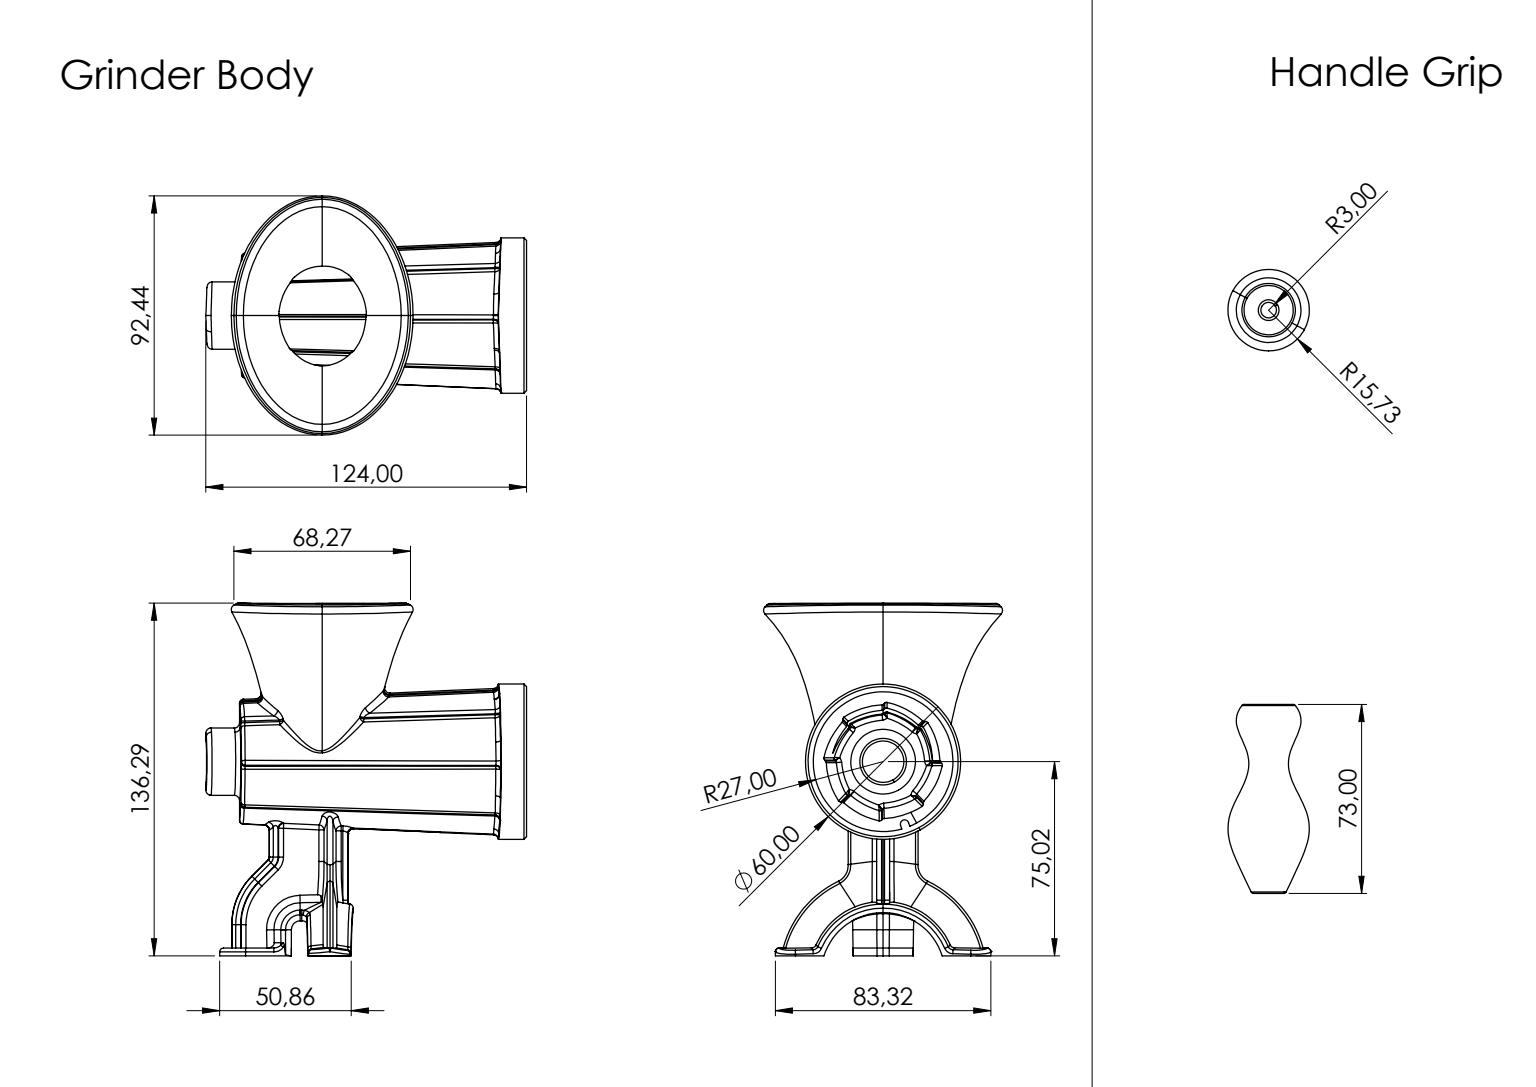
ISO-10303-21;
HEADER;
FILE_DESCRIPTION (('STEP AP214'),
    '1' );
FILE_NAME ('Grinder Body.step',
    '2026-10-06T09:49:54',
    ( '' ),
    ( '' ),
    'SwSTEP 2.0',
    'SolidWorks 2020',
    '' );
FILE_SCHEMA (( 'AUTOMOTIVE_DESIGN' ));
ENDSEC;

DATA;
#1=CARTESIAN_POINT ( 'NONE',  ( 0.9799183408087254188, 1466.964356560554961, 235.3982928250779310 ) ) ;
#5=CARTESIAN_POINT ( 'NONE',  ( -18.76815915579999938, 1485.949708182629820, 189.5055391954980166 ) ) ;
#7=CARTESIAN_POINT ( 'NONE',  ( -29.55438145523249815, 1510.073575141020228, 200.5476930356480239 ) ) ;
#9=CARTESIAN_POINT ( 'NONE',  ( 24.07566136850000049, 1410.921070243630083, 209.6344585171510175 ) ) ;
#11=CARTESIAN_POINT ( 'NONE',  ( 25.61451705386228284, 1436.639619060958239, 137.1797875125824362 ) ) ;
#13=CARTESIAN_POINT ( 'NONE',  ( 11.94438321470466136, 1435.361109817459010, 151.2115117280330310 ) ) ;
#18=CARTESIAN_POINT ( 'NONE',  ( 0.1771307642749359867, 1476.157344213379929, 182.2594403546649744 ) ) ;
#22=CARTESIAN_POINT ( 'NONE',  ( -25.18254675756193350, 1451.154070787092223, 137.5782062022625212 ) ) ;
#23=CARTESIAN_POINT ( 'NONE',  ( -22.28696231330000188, 1506.798305107829947, 208.8466800722590051 ) ) ;
#24=DIRECTION ( 'NONE',  ( -8.590429545572335868E-16, 0.9993908270191126375, 0.03489949670201628051 ) ) ;
#25=CARTESIAN_POINT ( 'NONE',  ( -41.44976345434149323, 1445.539178997049930, 134.0999999985149884 ) ) ;
#30=CARTESIAN_POINT ( 'NONE',  ( -14.66127766699999846, 1415.087974640030097, 218.7479844957980220 ) ) ;
#34=CARTESIAN_POINT ( 'NONE',  ( -2.760778634279479782, 1409.009468901610035, 188.0459411385839985 ) ) ;
#36=CARTESIAN_POINT ( 'NONE',  ( 21.19319384159999942, 1471.316885394430074, 209.8523956812749702 ) ) ;
#37=CARTESIAN_POINT ( 'NONE',  ( -5.360823448879425079, 1422.265545810137382, 143.1524318712457386 ) ) ;
#43=CARTESIAN_POINT ( 'NONE',  ( -32.69752361389999606, 1451.315419473630072, 135.9818030182980237 ) ) ;
#44=B_SPLINE_CURVE_WITH_KNOTS ( 'NONE', 3,
 ( #57452, #23800, #13187, #57991, #23253, #13738, #47922, #73698, #82058, #91579, #47375, #49043, #49590, #81500, #38947, #22130, #75882, #17028, #102702, #69152, #101057, #50145, #84272, #85931, #75348, #9234, #24355, #33305, #34970, #15944, #34425, #33864, #66948, #110030, #59640, #58541, #43391, #25996 ),
 .UNSPECIFIED., .F., .F.,
 ( 4, 2, 2, 2, 2, 2, 1, 1, 1, 1, 2, 2, 2, 2, 2, 1, 1, 1, 1, 2, 2, 2, 4 ),
 ( 0.000000000000000000, 0.1250000000000115463, 0.2500000000000230926, 0.3750000000000346390, 0.4375000000000425215, 0.4687500000000464073, 0.4843750000000510147, 0.4921875000000533462, 0.4960937500000545120, 0.4980468750000577316, 0.4990234375000622280, 0.5000000000000668354, 0.6250000000003189671, 0.6875000000004490852, 0.7187500000005095924, 0.7343750000005350165, 0.7421875000005526690, 0.7460937500005614398, 0.7480468750005607736, 0.7490234375005655476, 0.7500000000005703216, 0.8750000000002852163, 1.000000000000000000 ),
 .UNSPECIFIED. ) ;
#45=CARTESIAN_POINT ( 'NONE',  ( 17.11746647137171706, 1443.086052842848176, 162.7559337440806644 ) ) ;
#46=CARTESIAN_POINT ( 'NONE',  ( 8.598096571001718758, 1427.995879741943554, 137.0999999980979567 ) ) ;
#49=CARTESIAN_POINT ( 'NONE',  ( 25.83534073490000083, 1509.142433023230069, 218.8511637550280113 ) ) ;
#52=AXIS2_PLACEMENT_3D ( 'NONE', #79817, #89846, #28852 ) ;
#53=CARTESIAN_POINT ( 'NONE',  ( 39.02162918670904901, 1452.247899825818649, 269.5933113026415526 ) ) ;
#55=CARTESIAN_POINT ( 'NONE',  ( 5.639077273239999855, 1396.170382960830011, 219.3208623031979982 ) ) ;
#58=DIRECTION ( 'NONE',  ( 0.8730704095473449389, 0.4873619484741930075, 0.01504630028510589926 ) ) ;
#62=CARTESIAN_POINT ( 'NONE',  ( 4.260142758989999834, 1446.575475407549902, 159.4573513494979693 ) ) ;
#64=CARTESIAN_POINT ( 'NONE',  ( 13.58235818350000024, 1416.828044802929981, 196.3349386415980007 ) ) ;
#66=EDGE_LOOP ( 'NONE', ( #105431, #26314, #4870, #3833, #51565, #60481, #89456, #79002, #97316, #37692 ) ) ;
#68=ORIENTED_EDGE ( 'NONE', *, *, #43172, .F. ) ;
#70=ADVANCED_FACE ( 'NONE', ( #49805 ), #75938, .T. ) ;
#71=CARTESIAN_POINT ( 'NONE',  ( -23.55087209330000064, 1410.914164826029946, 206.5508649875179970 ) ) ;
#72=CARTESIAN_POINT ( 'NONE',  ( -10.49968249828000033, 1425.371007265300022, 102.3058044465100096 ) ) ;
#73=CARTESIAN_POINT ( 'NONE',  ( 16.84666619867320136, 1410.587845839309921, 191.9034688781510170 ) ) ;
#74=ADVANCED_FACE ( 'NONE', ( #10550 ), #8899, .T. ) ;
#76=CARTESIAN_POINT ( 'NONE',  ( 23.39541812081691674, 1509.845305380639729, 190.2643963894789181 ) ) ;
#80=B_SPLINE_CURVE_WITH_KNOTS ( 'NONE', 5,
 ( #89898, #13169, #47358, #81485, #38932, #107253 ),
 .UNSPECIFIED., .F., .F.,
 ( 6, 6 ),
 ( 0.000000000000000000, 1.000000000000000000 ),
 .UNSPECIFIED. ) ;
#81=CARTESIAN_POINT ( 'NONE',  ( -39.02581108420000078, 1422.344276296430053, 266.4771448061979982 ) ) ;
#84=CARTESIAN_POINT ( 'NONE',  ( 16.07415551216847049, 1461.167067577646549, 229.3519873809775333 ) ) ;
#90=CARTESIAN_POINT ( 'NONE',  ( 10.26791835527880004, 1396.449850368310081, 216.1922904392330338 ) ) ;
#93=CARTESIAN_POINT ( 'NONE',  ( -17.53303485170000187, 1459.032577061930169, 228.4504051497980015 ) ) ;
#94=ORIENTED_EDGE ( 'NONE', *, *, #44106, .T. ) ;
#105=CARTESIAN_POINT ( 'NONE',  ( 3.199785385034799923, 1421.555840881979975, 183.4721396264059763 ) ) ;
#107=CARTESIAN_POINT ( 'NONE',  ( 17.11714618744633754, 1443.086052842848630, 162.7561046190426737 ) ) ;
#114=CARTESIAN_POINT ( 'NONE',  ( 10.79382126600000014, 1414.913060387329779, 222.1041115775979904 ) ) ;
#116=ORIENTED_EDGE ( 'NONE', *, *, #25867, .F. ) ;
#117=CARTESIAN_POINT ( 'NONE',  ( -14.19373553490000006, 1416.535385209630022, 221.7254479851980022 ) ) ;
#118=CARTESIAN_POINT ( 'NONE',  ( -12.93811130839999812, 1442.831169986189934, 169.4238961894979809 ) ) ;
#122=CARTESIAN_POINT ( 'NONE',  ( -5.139599399479999775, 1425.322806783530041, 186.3313725629980127 ) ) ;
#126=CARTESIAN_POINT ( 'NONE',  ( -15.90471755817952548, 1410.840444494871690, 191.2727014167670916 ) ) ;
#128=CARTESIAN_POINT ( 'NONE',  ( 22.53878404599999641, 1411.058442739730026, 206.1986151668880041 ) ) ;
#129=CARTESIAN_POINT ( 'NONE',  ( 17.81158319340000062, 1457.914457808930138, 229.9274238559980006 ) ) ;
#131=CARTESIAN_POINT ( 'NONE',  ( -4.952890104507372548, 1423.293534163835830, 184.7224492574210615 ) ) ;
#133=B_SPLINE_SURFACE_WITH_KNOTS ( 'NONE', 5, 3, ( 
 ( #34867, #77434, #42173, #67396 ),
 ( #93646, #52248, #60652, #69055 ),
 ( #103155, #43831, #101494, #16929 ),
 ( #41622, #26457, #43287, #93111 ),
 ( #86374, #34317, #94776, #76885 ),
 ( #8007, #734, #1283, #85822 ),
 ( #35424, #50030, #76324, #8554 ),
 ( #51130, #69611, #84159, #18053 ),
 ( #24248, #109929, #16382, #42726 ) ),
 .UNSPECIFIED., .F., .F., .F.,
 ( 6, 3, 6 ),
 ( 4, 4 ),
 ( 0.000000000000000000, 5.782490304330000441, 11.25975508159999983 ),
 ( 37.69911184309999896, 40.20365518519999881 ),
 .UNSPECIFIED. ) ;
#136=CARTESIAN_POINT ( 'NONE',  ( -2.793439186891359949, 1486.025328193850100, 182.0741020391329812 ) ) ;
#138=CARTESIAN_POINT ( 'NONE',  ( -2.931110993877138249, 1485.094118085803984, 183.0973985693935617 ) ) ;
#139=CARTESIAN_POINT ( 'NONE',  ( 5.979558325686289422, 1406.768155905330104, 269.6447222190780053 ) ) ;
#141=ORIENTED_EDGE ( 'NONE', *, *, #18307, .F. ) ;
#142=CARTESIAN_POINT ( 'NONE',  ( 0.9041354327699999693, 1416.839648768630013, 190.2140802940980109 ) ) ;
#145=CARTESIAN_POINT ( 'NONE',  ( -11.74804893329999800, 1426.270137612329790, 145.0346010018980110 ) ) ;
#146=DIRECTION ( 'NONE',  ( -1.110223024629289185E-15, -0.7071067811865475727, -0.7071067811865475727 ) ) ;
#147=CARTESIAN_POINT ( 'NONE',  ( 0.000000000000000000, 1511.163060387329779, 209.1218459616979999 ) ) ;
#148=DIRECTION ( 'NONE',  ( 1.000000000000000000, 5.309750374689999822E-19, 2.343158368729999945E-19 ) ) ;
#151=CARTESIAN_POINT ( 'NONE',  ( 9.215280650669999574, 1410.394055827930060, 230.1315963332980061 ) ) ;
#152=CARTESIAN_POINT ( 'NONE',  ( -25.75006378359999815, 1482.723232260229906, 211.9130519178279997 ) ) ;
#157=CARTESIAN_POINT ( 'NONE',  ( 27.01536995560000065, 1412.459480457830068, 266.9350197775979723 ) ) ;
#159=CARTESIAN_POINT ( 'NONE',  ( 22.53781764839999724, 1430.293776123330190, 201.7931574036180109 ) ) ;
#160=CARTESIAN_POINT ( 'NONE',  ( -0.2682927907274870183, 1508.576597181550142, 237.9003827947630043 ) ) ;
#162=CARTESIAN_POINT ( 'NONE',  ( 21.91792426780000369, 1509.678451168330184, 227.8819284857980279 ) ) ;
#166=CARTESIAN_POINT ( 'NONE',  ( -13.11944326200000077, 1446.139497881190209, 187.9998882741980140 ) ) ;
#173=CARTESIAN_POINT ( 'NONE',  ( -12.50898706442170116, 1409.349883841199926, 217.3002069970499974 ) ) ;
#177=CARTESIAN_POINT ( 'NONE',  ( -23.55147266200000189, 1470.760850431830022, 269.0841978914980359 ) ) ;
#181=CARTESIAN_POINT ( 'NONE',  ( -24.15092527543778189, 1444.494566185576332, 211.6397483413928455 ) ) ;
#185=CARTESIAN_POINT ( 'NONE',  ( 11.29240053233250052, 1415.034069327070029, 222.6155400430430120 ) ) ;
#187=CARTESIAN_POINT ( 'NONE',  ( -14.61131892634599971, 1485.012037849769968, 224.2679068592169926 ) ) ;
#188=CARTESIAN_POINT ( 'NONE',  ( -22.86536645260000000, 1410.206636297830073, 204.9906524142479896 ) ) ;
#190=CARTESIAN_POINT ( 'NONE',  ( 13.83520663969999909, 1414.913060387329779, 199.8641522158279997 ) ) ;
#192=ADVANCED_FACE ( 'NONE', ( #107906 ), #49678, .T. ) ;
#198=CARTESIAN_POINT ( 'NONE',  ( -22.57636395089999937, 1411.060965688729766, 211.7929440282880194 ) ) ;
#200=CARTESIAN_POINT ( 'NONE',  ( 10.79382269979189957, 1414.913060387349788, 222.1041130917409987 ) ) ;
#201=CARTESIAN_POINT ( 'NONE',  ( 11.69274081191520054, 1426.725035085969921, 141.0012239352140000 ) ) ;
#205=CARTESIAN_POINT ( 'NONE',  ( -12.02002121700249937, 1447.120365805550136, 187.5076542713389927 ) ) ;
#206=CIRCLE ( 'NONE', #57435, 2.000000000000001776 ) ;
#208=CARTESIAN_POINT ( 'NONE',  ( -4.941360932494764491, 1398.060275951993162, 221.1476519450009164 ) ) ;
#209=CARTESIAN_POINT ( 'NONE',  ( -3.034707026709789979, 1440.440247136690004, 157.2489849372729793 ) ) ;
#211=CARTESIAN_POINT ( 'NONE',  ( 1.951029617469999922, 1508.751449870530223, 237.3205679125979941 ) ) ;
#213=EDGE_LOOP ( 'NONE', ( #57511, #100598, #97650, #95419, #60917 ) ) ;
#215=CARTESIAN_POINT ( 'NONE',  ( 11.97689773866060037, 1433.612225593400126, 149.9683442909959865 ) ) ;
#222=DIRECTION ( 'NONE',  ( 0.7071067811870476172, 0.000000000000000000, -0.7071067811860475283 ) ) ;
#223=CARTESIAN_POINT ( 'NONE',  ( 1.188177619867464285, 1416.835288280217583, 190.1185025207718695 ) ) ;
#224=CARTESIAN_POINT ( 'NONE',  ( 16.85900957629469943, 1498.111060690920112, 230.7389555287900009 ) ) ;
#225=AXIS2_PLACEMENT_3D ( 'NONE', #60606, #95291, #28634 ) ;
#226=CARTESIAN_POINT ( 'NONE',  ( 2.328600095410000126, 1488.173045798130033, 182.1148965703980025 ) ) ;
#227=CARTESIAN_POINT ( 'NONE',  ( 13.43167025587599817, 1509.382104656720003, 235.1752264429409820 ) ) ;
#231=CARTESIAN_POINT ( 'NONE',  ( 13.54623987573500088, 1415.059973085240017, 197.7769859117730107 ) ) ;
#232=CARTESIAN_POINT ( 'NONE',  ( 11.57525528770000101, 1432.243446488439986, 151.1962572209980067 ) ) ;
#235=CARTESIAN_POINT ( 'NONE',  ( 13.94902171141210090, 1435.073072362720040, 149.1168395385139718 ) ) ;
#239=CARTESIAN_POINT ( 'NONE',  ( 13.40011037178709330, 1444.420227106130369, 169.3684798139838676 ) ) ;
#240=CARTESIAN_POINT ( 'NONE',  ( -11.01696037870000033, 1462.338713412430252, 233.0647636304979926 ) ) ;
#244=AXIS2_PLACEMENT_3D ( 'NONE', #101072, #98882, #31677 ) ;
#246=LINE ( 'NONE', #1902, #99740 ) ;
#252=CARTESIAN_POINT ( 'NONE',  ( 21.27308478715089990, 1440.913060387330006, 223.7805658757509946 ) ) ;
#253=CARTESIAN_POINT ( 'NONE',  ( -18.65749898560000020, 1509.387464492830077, 230.8014192534980111 ) ) ;
#254=EDGE_LOOP ( 'NONE', ( #74179, #87875, #88245, #39917, #100540, #44653, #57226, #30791 ) ) ;
#255=FACE_OUTER_BOUND ( 'NONE', #49988, .T. ) ;
#259=CARTESIAN_POINT ( 'NONE',  ( 23.78270988279999898, 1434.944176083839920, 215.5045224494480181 ) ) ;
#264=CARTESIAN_POINT ( 'NONE',  ( -24.62269181266490037, 1457.704162723289983, 212.0269868133230204 ) ) ;
#271=CARTESIAN_POINT ( 'NONE',  ( 14.81130958389999996, 1410.375311269529902, 191.5354464119980094 ) ) ;
#272=AXIS2_PLACEMENT_3D ( 'NONE', #31208, #50242, #83816 ) ;
#273=CARTESIAN_POINT ( 'NONE',  ( -16.59643141521007692, 1486.110667197937119, 187.3981733332393844 ) ) ;
#277=CARTESIAN_POINT ( 'NONE',  ( 33.67855476909999624, 1460.266122003729834, 261.9078250184979879 ) ) ;
#279=CARTESIAN_POINT ( 'NONE',  ( -29.22959469711409852, 1509.933780326070064, 211.7723416727030212 ) ) ;
#280=CARTESIAN_POINT ( 'NONE',  ( -7.422625755698760486, 1509.173068315250021, 237.5382155034599805 ) ) ;
#281=CARTESIAN_POINT ( 'NONE',  ( -23.72450110970000026, 1447.345343915189915, 214.6425533432180259 ) ) ;
#283=LINE ( 'NONE', #53444, #107281 ) ;
#284=CARTESIAN_POINT ( 'NONE',  ( 17.19105300219910148, 1409.567693813439973, 222.3521885693010063 ) ) ;
#291=CARTESIAN_POINT ( 'NONE',  ( 29.02628104170000256, 1509.926680456829899, 206.2525988583179810 ) ) ;
#292=CARTESIAN_POINT ( 'NONE',  ( 24.56509571990000040, 1440.948426447710062, 213.0043250210379995 ) ) ;
#295=VECTOR ( 'NONE', #1841, 999.9999999999998863 ) ;
#296=CARTESIAN_POINT ( 'NONE',  ( 27.60463613754729906, 1435.937341596739998, 136.4952273551159863 ) ) ;
#297=CARTESIAN_POINT ( 'NONE',  ( 36.19701834746070546, 1449.940556718190010, 136.2509691137539960 ) ) ;
#300=CARTESIAN_POINT ( 'NONE',  ( -16.09127082379999862, 1410.842149181930154, 226.7264691084980086 ) ) ;
#305=ORIENTED_EDGE ( 'NONE', *, *, #65971, .T. ) ;
#306=CARTESIAN_POINT ( 'NONE',  ( 0.8090580814599999115, 1427.166763959530044, 147.9649995502979891 ) ) ;
#307=CARTESIAN_POINT ( 'NONE',  ( 3.902542035141590038, 1426.015650130040058, 185.2953857556300079 ) ) ;
#311=CARTESIAN_POINT ( 'NONE',  ( -0.5392968480769999573, 1417.272289817929959, 235.8882545161980033 ) ) ;
#314=CARTESIAN_POINT ( 'NONE',  ( -12.99045328924907139, 1444.881939451659264, 186.2719392246208656 ) ) ;
#317=AXIS2_PLACEMENT_3D ( 'NONE', #43515, #103956, #9895 ) ;
#319=CARTESIAN_POINT ( 'NONE',  ( -38.49765372626540483, 1444.525112228479884, 137.1053225085370002 ) ) ;
#321=CARTESIAN_POINT ( 'NONE',  ( 25.44234826850000175, 1436.623918441529895, 137.2992118829979802 ) ) ;
#322=CARTESIAN_POINT ( 'NONE',  ( -10.92603999506069989, 1396.294606111510120, 207.3491235618079997 ) ) ;
#325=CARTESIAN_POINT ( 'NONE',  ( -16.89772930833600029, 1410.137463210610122, 226.0661309239629873 ) ) ;
#326=CARTESIAN_POINT ( 'NONE',  ( 2.488082932330000219, 1441.600846913620217, 150.5962877614979902 ) ) ;
#327=ORIENTED_EDGE ( 'NONE', *, *, #30892, .T. ) ;
#331=FACE_OUTER_BOUND ( 'NONE', #57581, .T. ) ;
#333=CARTESIAN_POINT ( 'NONE',  ( 23.36041073559999859, 1411.089115351430110, 212.3712601659579775 ) ) ;
#334=CARTESIAN_POINT ( 'NONE',  ( 4.215774578864469824, 1425.101385327330036, 185.2788908656129934 ) ) ;
#335=CARTESIAN_POINT ( 'NONE',  ( -2.852637967456935986, 1419.721280333027380, 186.1746705150881098 ) ) ;
#340=CARTESIAN_POINT ( 'NONE',  ( 2.852330403769999911, 1449.230534335530137, 183.5545985393980004 ) ) ;
#343=CARTESIAN_POINT ( 'NONE',  ( -4.951136445669599511E-10, 1417.070352045260051, 236.6937895817889910 ) ) ;
#344=ORIENTED_EDGE ( 'NONE', *, *, #61935, .F. ) ;
#346=CARTESIAN_POINT ( 'NONE',  ( -41.48252549709999926, 1444.135617533290088, 136.5500651578979898 ) ) ;
#347=DIRECTION ( 'NONE',  ( 0.000000000000000000, 1.000000000000000000, 0.000000000000000000 ) ) ;
#348=CARTESIAN_POINT ( 'NONE',  ( -0.4691143273430000149, 1471.436294014529949, 269.3346704442980126 ) ) ;
#349=CARTESIAN_POINT ( 'NONE',  ( 12.17607342826484818, 1434.037890756064598, 147.4852139652959693 ) ) ;
#351=CARTESIAN_POINT ( 'NONE',  ( 20.46339790889999932, 1475.513060387329915, 205.2504343647379983 ) ) ;
#352=ADVANCED_FACE ( 'NONE', ( #86566 ), #108998, .T. ) ;
#354=CARTESIAN_POINT ( 'NONE',  ( 22.51991254300000023, 1410.619212212730190, 206.2037069855880134 ) ) ;
#355=CARTESIAN_POINT ( 'NONE',  ( -20.80119636470000088, 1475.513060387329915, 204.3591166435880098 ) ) ;
#357=CARTESIAN_POINT ( 'NONE',  ( -5.603383157293649656E-09, 1406.911841289329914, 196.1218459609980300 ) ) ;
#358=CARTESIAN_POINT ( 'NONE',  ( -12.11929752427059981, 1407.056436474629891, 267.1741674207860342 ) ) ;
#360=CARTESIAN_POINT ( 'NONE',  ( -13.80543509878039998, 1434.979598264029846, 148.5369193816260065 ) ) ;
#363=CARTESIAN_POINT ( 'NONE',  ( 13.57336059360000036, 1443.191372133680034, 188.8849899699980028 ) ) ;
#364=EDGE_LOOP ( 'NONE', ( #86550, #29612, #108325, #100325 ) ) ;
#366=EDGE_CURVE ( 'NONE', #43369, #37055, #92016, .T. ) ;
#368=CARTESIAN_POINT ( 'NONE',  ( 4.479677203900762628, 1422.012945122907468, 183.9385808951501531 ) ) ;
#369=CARTESIAN_POINT ( 'NONE',  ( 3.034145577506000446, 1440.440283345010130, 157.2495443575080003 ) ) ;
#371=CARTESIAN_POINT ( 'NONE',  ( -18.11868862529999902, 1485.487861948229920, 188.9570397301980051 ) ) ;
#376=( BOUNDED_CURVE ( )  B_SPLINE_CURVE ( 3, ( #102045, #83062, #101486, #40501 ),
 .UNSPECIFIED., .F., .T. ) 
 B_SPLINE_CURVE_WITH_KNOTS ( ( 4, 4 ),
 ( 4.045555810179484624, 4.691360937121570096 ),
 .UNSPECIFIED. ) 
 CURVE ( )  GEOMETRIC_REPRESENTATION_ITEM ( )  RATIONAL_B_SPLINE_CURVE ( ( 1.000000000000000000, 0.9655455809096770148, 0.9655455809096770148, 1.000000000000000000 ) ) 
 REPRESENTATION_ITEM ( '' )  );
#380=CARTESIAN_POINT ( 'NONE',  ( -29.75011777940000002, 1509.993906963430163, 208.5595589157580036 ) ) ;
#383=CARTESIAN_POINT ( 'NONE',  ( -1.344035116579999967, 1408.775599479229868, 195.0461770646979858 ) ) ;
#384=CARTESIAN_POINT ( 'NONE',  ( -26.58019104509060071, 1469.327027323300172, 208.7773797362419828 ) ) ;
#385=CARTESIAN_POINT ( 'NONE',  ( 15.37090799315269152, 1506.446781340675443, 193.3909299311295626 ) ) ;
#386=ORIENTED_EDGE ( 'NONE', *, *, #99268, .F. ) ;
#387=CARTESIAN_POINT ( 'NONE',  ( -27.41515663979030037, 1488.740012749160087, 208.8186931342820003 ) ) ;
#388=CARTESIAN_POINT ( 'NONE',  ( 26.30775428189999943, 1469.245646012430143, 210.8538279144680132 ) ) ;
#391=CARTESIAN_POINT ( 'NONE',  ( -23.95553108059999659, 1435.340102472350054, 136.9960523771979979 ) ) ;
#400=ORIENTED_EDGE ( 'NONE', *, *, #22203, .T. ) ;
#401=DIRECTION ( 'NONE',  ( -0.03489949670255338560, 0.9993908270190677845, 2.284588940413689109E-07 ) ) ;
#402=CARTESIAN_POINT ( 'NONE',  ( 5.375553136205760474, 1441.026369937100071, 154.8319413496199957 ) ) ;
#405=ORIENTED_EDGE ( 'NONE', *, *, #65155, .F. ) ;
#408=CARTESIAN_POINT ( 'NONE',  ( 12.69127487099669871, 1434.626206151899851, 149.6849692847659981 ) ) ;
#409=CARTESIAN_POINT ( 'NONE',  ( 14.76180801577280022, 1459.302556161789880, 230.0031883768110106 ) ) ;
#410=CARTESIAN_POINT ( 'NONE',  ( -21.86081811034360101, 1508.398734063270012, 226.4470915494329972 ) ) ;
#412=DIRECTION ( 'NONE',  ( -0.9999999999999995559, -4.156278225545078260E-11, 3.325661287725353434E-08 ) ) ;
#415=CARTESIAN_POINT ( 'NONE',  ( -3.619432601040000197, 1421.014464036429899, 186.0219392937979990 ) ) ;
#416=CARTESIAN_POINT ( 'NONE',  ( 20.30888173789999840, 1509.664622709230116, 187.3912422546979997 ) ) ;
#418=ORIENTED_EDGE ( 'NONE', *, *, #83682, .T. ) ;
#419=CARTESIAN_POINT ( 'NONE',  ( -12.45665494490000214, 1416.827520077930103, 194.7672771341979967 ) ) ;
#421=ORIENTED_EDGE ( 'NONE', *, *, #109564, .F. ) ;
#422=CARTESIAN_POINT ( 'NONE',  ( 3.316185754920000228, 1421.597412442629775, 183.5076398005980138 ) ) ;
#423=B_SPLINE_CURVE_WITH_KNOTS ( 'NONE', 3,
 ( #95450, #45072, #95995, #54035, #1393, #107007, #19264, #35533, #28242, #53467, #78091, #854, #10331, #70288 ),
 .UNSPECIFIED., .F., .F.,
 ( 4, 2, 1, 1, 1, 1, 2, 2, 4 ),
 ( 0.000000000000000000, 0.2500000000014274693, 0.3750000000021411761, 0.4375000000024389935, 0.4687500000025079938, 0.4843750000025635605, 0.4921875000025116020, 0.5000000000024596991, 1.000000000000000000 ),
 .UNSPECIFIED. ) ;
#426=CARTESIAN_POINT ( 'NONE',  ( 1275.711986934499919, 50.13405481564039690, 10006.43705117350146 ) ) ;
#429=CARTESIAN_POINT ( 'NONE',  ( 18.88067404609999755, 1416.254459047329874, 210.2603107721379843 ) ) ;
#432=DIRECTION ( 'NONE',  ( -0.9417419115949053898, 0.3363363969979660806, 0.000000000000000000 ) ) ;
#433=CARTESIAN_POINT ( 'NONE',  ( 26.36916589390109777, 1446.546730984839769, 137.7167331325649968 ) ) ;
#436=CARTESIAN_POINT ( 'NONE',  ( 10.91311011200522962, 1428.352194749460068, 150.6639344388404140 ) ) ;
#438=CARTESIAN_POINT ( 'NONE',  ( 14.25731394439999988, 1435.139839336880186, 149.2707523579979920 ) ) ;
#439=CARTESIAN_POINT ( 'NONE',  ( 25.70326353240000117, 1469.149937121330140, 207.3826394511280000 ) ) ;
#440=CARTESIAN_POINT ( 'NONE',  ( -29.19056928059999834, 1509.932417528530095, 211.8176115312480192 ) ) ;
#441=CARTESIAN_POINT ( 'NONE',  ( 7.731075332760467766, 1410.555903148826246, 187.4988090489762271 ) ) ;
#443=CARTESIAN_POINT ( 'NONE',  ( 3.439855069772169809E-11, 1452.913060387330006, 150.8032249182200246 ) ) ;
#445=CARTESIAN_POINT ( 'NONE',  ( 12.98226561589999939, 1414.913060387329779, 198.3280246956980193 ) ) ;
#448=CARTESIAN_POINT ( 'NONE',  ( -27.06966532493517974, 1508.822569575641182, 212.0394344631261561 ) ) ;
#452=CARTESIAN_POINT ( 'NONE',  ( -1.547463840030000037, 1414.913060387329779, 225.9340782259980074 ) ) ;
#454=CARTESIAN_POINT ( 'NONE',  ( -16.19086242769280304, 1409.478452467050147, 225.0103265570539861 ) ) ;
#459=CARTESIAN_POINT ( 'NONE',  ( 36.82437600794989407, 1437.810818275439942, 136.5532457654989855 ) ) ;
#460=CARTESIAN_POINT ( 'NONE',  ( 19.64184507190000062, 1452.819461535530081, 208.8935671266810061 ) ) ;
#464=CARTESIAN_POINT ( 'NONE',  ( -11.83623787450240528, 1435.250172798539779, 151.2634934636774346 ) ) ;
#466=CARTESIAN_POINT ( 'NONE',  ( 2.320227349930000127, 1408.994084511829897, 187.0163958760979881 ) ) ;
#467=CARTESIAN_POINT ( 'NONE',  ( 1.374098705546139998, 1508.999826499959909, 179.4761476500559922 ) ) ;
#468=CARTESIAN_POINT ( 'NONE',  ( -11.04138758999999936, 1437.532134338300011, 152.0929086130979897 ) ) ;
#469=LINE ( 'NONE', #52518, #42544 ) ;
#472=CARTESIAN_POINT ( 'NONE',  ( 11.86716023049999968, 1432.353341358199941, 147.6509521729980179 ) ) ;
#473=CARTESIAN_POINT ( 'NONE',  ( 0.6083087506080000484, 1465.081050579229895, 236.9567715190979982 ) ) ;
#474=ORIENTED_EDGE ( 'NONE', *, *, #24074, .F. ) ;
#476=CARTESIAN_POINT ( 'NONE',  ( -38.87545285710000087, 1457.142118430129813, 270.1626018656980364 ) ) ;
#477=CARTESIAN_POINT ( 'NONE',  ( -23.74108753817469974, 1436.296634041249945, 212.5883363871789982 ) ) ;
#478=CARTESIAN_POINT ( 'NONE',  ( 16.19492459430000153, 1409.478599616029896, 224.1775087544979783 ) ) ;
#480=CARTESIAN_POINT ( 'NONE',  ( -1.371587748774959908E-10, 1469.646809014170003, 253.0669417465539652 ) ) ;
#482=CARTESIAN_POINT ( 'NONE',  ( -19.88572122277579979, 1484.728771715989751, 191.0592865161910083 ) ) ;
#483=CARTESIAN_POINT ( 'NONE',  ( -0.7692391029760000665, 1415.628674266529742, 227.3871686175980074 ) ) ;
#484=CARTESIAN_POINT ( 'NONE',  ( -9.817298943409999978, 1418.814616626229963, 230.3607498785979999 ) ) ;
#487=CARTESIAN_POINT ( 'NONE',  ( -0.05082592258669504232, 1486.215346117376839, 181.8157142799529993 ) ) ;
#489=CARTESIAN_POINT ( 'NONE',  ( -45.95836323909989574, 1437.680972842699703, 268.2109776636490324 ) ) ;
#494=CARTESIAN_POINT ( 'NONE',  ( -2.478898695439999855, 1433.170136607830045, 157.5403501404979920 ) ) ;
#497=CARTESIAN_POINT ( 'NONE',  ( -26.35325170641180037, 1451.992872967969788, 135.0462968633300136 ) ) ;
#500=CARTESIAN_POINT ( 'NONE',  ( 25.99468486090000141, 1435.718168598109969, 225.6861378082980139 ) ) ;
#504=CARTESIAN_POINT ( 'NONE',  ( -2.479184146860000096E-08, 1422.360590008429881, 211.7205299278780046 ) ) ;
#505=EDGE_CURVE ( 'NONE', #59255, #100495, #12716, .T. ) ;
#509=CARTESIAN_POINT ( 'NONE',  ( -4.218478457446350305, 1409.928425769410069, 270.0721727225960080 ) ) ;
#511=CARTESIAN_POINT ( 'NONE',  ( 13.49846100598660037, 1421.214292344940077, 231.0218097068720056 ) ) ;
#514=ORIENTED_EDGE ( 'NONE', *, *, #3680, .F. ) ;
#516=CARTESIAN_POINT ( 'NONE',  ( -22.79252858209050103, 1409.718716787750054, 209.5234536894689938 ) ) ;
#517=CARTESIAN_POINT ( 'NONE',  ( -0.6532819063196209086, 1409.103086040569906, 185.7260927124030161 ) ) ;
#519=PLANE ( 'NONE',  #38439 ) ;
#520=CARTESIAN_POINT ( 'NONE',  ( -19.03551611759530005, 1443.980599388390146, 194.2018241821600100 ) ) ;
#521=CARTESIAN_POINT ( 'NONE',  ( -19.69872028629999861, 1420.831966503530111, 222.5429556983980035 ) ) ;
#522=CARTESIAN_POINT ( 'NONE',  ( 36.52219476372820850, 1461.495432610050102, 269.2158760797449872 ) ) ;
#523=CARTESIAN_POINT ( 'NONE',  ( -15.46700379407589843, 1461.188231737419756, 228.6959062608830209 ) ) ;
#524=CARTESIAN_POINT ( 'NONE',  ( -2.907264515414449857, 1451.960119877520128, 184.7556101994359778 ) ) ;
#527=ORIENTED_EDGE ( 'NONE', *, *, #22644, .F. ) ;
#528=CARTESIAN_POINT ( 'NONE',  ( -11.74481771089999960, 1433.726929579510170, 150.9290601731980246 ) ) ;
#531=ORIENTED_EDGE ( 'NONE', *, *, #98190, .F. ) ;
#533=CARTESIAN_POINT ( 'NONE',  ( 26.74533639559809828, 1450.888433640950097, 136.4325763836939984 ) ) ;
#537=CARTESIAN_POINT ( 'NONE',  ( 18.05634065199999938, 1410.467697827129996, 193.5994654289980019 ) ) ;
#539=CARTESIAN_POINT ( 'NONE',  ( 5.158526775084939509, 1409.093200111750093, 187.9627302490250145 ) ) ;
#541=CARTESIAN_POINT ( 'NONE',  ( -22.82877908214457463, 1432.437248394402786, 215.4934721305570520 ) ) ;
#542=CARTESIAN_POINT ( 'NONE',  ( 1.324223389204969958, 1452.129545857950006, 183.4093034293840105 ) ) ;
#545=CARTESIAN_POINT ( 'NONE',  ( 7.912312578985590150, 1418.799544019259883, 233.2448588504591669 ) ) ;
#546=ORIENTED_EDGE ( 'NONE', *, *, #47982, .F. ) ;
#547=CARTESIAN_POINT ( 'NONE',  ( 12.66409680412649941, 1415.935475482089942, 221.7747898017080104 ) ) ;
#548=FACE_OUTER_BOUND ( 'NONE', #82906, .T. ) ;
#549=FACE_OUTER_BOUND ( 'NONE', #106760, .T. ) ;
#553=CARTESIAN_POINT ( 'NONE',  ( 13.04266739719999890, 1417.449502458830011, 221.6520488708979713 ) ) ;
#556=CARTESIAN_POINT ( 'NONE',  ( 11.74567502190000035, 1433.530944218069862, 150.8654047345980018 ) ) ;
#557=CARTESIAN_POINT ( 'NONE',  ( 2.984513020910000147, 1453.913060387330006, 209.1218459616979999 ) ) ;
#562=CARTESIAN_POINT ( 'NONE',  ( 22.70509004431190192, 1409.705939603270053, 209.2982552845940063 ) ) ;
#564=CARTESIAN_POINT ( 'NONE',  ( -15.28951669910000000, 1509.578191272730010, 236.7286881490979908 ) ) ;
#565=CARTESIAN_POINT ( 'NONE',  ( 23.54254250440000007, 1430.351957799930005, 214.4849305350980160 ) ) ;
#567=CARTESIAN_POINT ( 'NONE',  ( 26.16840185550843856, 1436.693591485223578, 136.8912855551424173 ) ) ;
#569=CARTESIAN_POINT ( 'NONE',  ( 17.42808535260000014, 1431.113060387329824, 216.7347523923079962 ) ) ;
#573=CARTESIAN_POINT ( 'NONE',  ( 0.1665927539581550099, 1482.335989075430234, 181.9940412649720258 ) ) ;
#574=DIRECTION ( 'NONE',  ( -0.5412924984493711067, 0.1391731009598990432, -0.8292365640103210866 ) ) ;
#575=VERTEX_POINT ( 'NONE', #42240 ) ;
#576=CARTESIAN_POINT ( 'NONE',  ( -1.546869375780000055, 1416.835808399930102, 228.0212684633979734 ) ) ;
#577=CARTESIAN_POINT ( 'NONE',  ( -16.90742456144258909, 1444.994950788469623, 162.4348202098878744 ) ) ;
#579=CARTESIAN_POINT ( 'NONE',  ( -35.35021333641900299, 1451.550776711729895, 134.0999999984329918 ) ) ;
#581=ORIENTED_EDGE ( 'NONE', *, *, #68778, .F. ) ;
#585=FACE_OUTER_BOUND ( 'NONE', #42425, .T. ) ;
#596=CARTESIAN_POINT ( 'NONE',  ( 16.90809753623369360, 1442.831169986191526, 162.4344573440251338 ) ) ;
#604=DIRECTION ( 'NONE',  ( -1.592428286118737079E-10, -0.9689480427665004836, 0.2472644139761486504 ) ) ;
#606=CARTESIAN_POINT ( 'NONE',  ( 15.82611567847458289, 1431.600131786831980, 218.9583281995740833 ) ) ;
#609=CARTESIAN_POINT ( 'NONE',  ( -20.15452302159999931, 1507.845791376729949, 228.9024215066979764 ) ) ;
#613=CARTESIAN_POINT ( 'NONE',  ( 4.220927954709999597, 1446.217199771959940, 167.4561886970979856 ) ) ;
#614=CARTESIAN_POINT ( 'NONE',  ( -15.74187958907210039, 1412.794802208900137, 226.7867534266219991 ) ) ;
#622=CARTESIAN_POINT ( 'NONE',  ( -21.91488071189999687, 1449.791133988690035, 197.9993651584979943 ) ) ;
#623=CARTESIAN_POINT ( 'NONE',  ( -11.54936350167399972, 1426.401857134930196, 130.8094922821749719 ) ) ;
#624=CARTESIAN_POINT ( 'NONE',  ( 16.85667268330360002, 1410.729706438800122, 191.8820313785110159 ) ) ;
#627=CARTESIAN_POINT ( 'NONE',  ( -4.518180742295140181E-06, 1509.047264790930058, 179.1218459713510072 ) ) ;
#629=CARTESIAN_POINT ( 'NONE',  ( -21.30047364560000034, 1471.312091222029949, 208.2102265936800336 ) ) ;
#630=CARTESIAN_POINT ( 'NONE',  ( -41.56051824640000092, 1438.341700612089880, 261.5689736386979689 ) ) ;
#631=CARTESIAN_POINT ( 'NONE',  ( 19.31522993011370204, 1509.613100981719981, 231.6083989249460160 ) ) ;
#636=CARTESIAN_POINT ( 'NONE',  ( -39.46926012269349826, 1440.456819381679907, 136.7723882296410238 ) ) ;
#637=ORIENTED_EDGE ( 'NONE', *, *, #18509, .F. ) ;
#638=CARTESIAN_POINT ( 'NONE',  ( 12.86231746777660057, 1396.538691440989851, 207.1246007041149824 ) ) ;
#641=ORIENTED_EDGE ( 'NONE', *, *, #103472, .F. ) ;
#643=CARTESIAN_POINT ( 'NONE',  ( -29.24222457024196586, 1509.934245987175927, 211.7448869334152164 ) ) ;
#644=CARTESIAN_POINT ( 'NONE',  ( -9.298374131422571409, 1424.634617889919809, 149.7551454182870145 ) ) ;
#646=CARTESIAN_POINT ( 'NONE',  ( -1.116585105924089969E-07, 1397.914279478820163, 196.1218459578329885 ) ) ;
#649=CARTESIAN_POINT ( 'NONE',  ( -4.656690245969999253, 1461.191637107629958, 234.3103256880980041 ) ) ;
#658=CARTESIAN_POINT ( 'NONE',  ( 11.73986278517180182, 1426.693600150729935, 144.3691362286979825 ) ) ;
#660=VERTEX_POINT ( 'NONE', #93714 ) ;
#661=DIRECTION ( 'NONE',  ( 0.7067701421949666996, -0.03085961869104518474, 0.7067698706339636816 ) ) ;
#663=CARTESIAN_POINT ( 'NONE',  ( 9.406666111339999858, 1509.241548406330139, 236.7319732460980219 ) ) ;
#665=CARTESIAN_POINT ( 'NONE',  ( -5.256547791280000048, 1424.521933614530099, 186.2316258165979832 ) ) ;
#666=CARTESIAN_POINT ( 'NONE',  ( 7.984655233845471045, 1410.580038844309911, 269.8705203775900259 ) ) ;
#669=CARTESIAN_POINT ( 'NONE',  ( -11.54583652347674416, 1410.690064926147897, 189.0055360890668510 ) ) ;
#672=CARTESIAN_POINT ( 'NONE',  ( 24.92729647353190003, 1464.542099455490188, 206.2188305520340066 ) ) ;
#674=FACE_OUTER_BOUND ( 'NONE', #24207, .T. ) ;
#675=CARTESIAN_POINT ( 'NONE',  ( -5.010265762299249914, 1422.725625646132585, 184.8437789348542424 ) ) ;
#676=CARTESIAN_POINT ( 'NONE',  ( -5.370514330159649852, 1422.356910281434239, 139.1416123588654727 ) ) ;
#678=ORIENTED_EDGE ( 'NONE', *, *, #80484, .T. ) ;
#679=CARTESIAN_POINT ( 'NONE',  ( 18.07417247534460003, 1424.494734117629832, 224.1841365583740071 ) ) ;
#681=CARTESIAN_POINT ( 'NONE',  ( -2.959734820789013288, 1485.424150447127658, 182.8872198570792591 ) ) ;
#683=CARTESIAN_POINT ( 'NONE',  ( -17.60627216660330063, 1410.895669502700230, 193.4350316886979897 ) ) ;
#685=EDGE_LOOP ( 'NONE', ( #51444, #69652, #66163, #14641 ) ) ;
#687=CARTESIAN_POINT ( 'NONE',  ( -15.13342374508840038, 1507.606285602760181, 191.8462590464540085 ) ) ;
#688=CARTESIAN_POINT ( 'NONE',  ( -11.83486911239999984, 1430.209948791529769, 149.5656396673979884 ) ) ;
#689=CARTESIAN_POINT ( 'NONE',  ( 0.000000000000000000, 1405.413060387330006, 209.1218459616979999 ) ) ;
#695=CARTESIAN_POINT ( 'NONE',  ( -20.11321007749999978, 1508.016902856529896, 228.9715373177980098 ) ) ;
#697=CARTESIAN_POINT ( 'NONE',  ( -16.61466320086400117, 1459.965743753311926, 228.4923931122799843 ) ) ;
#699=CARTESIAN_POINT ( 'NONE',  ( 18.25484434299999847, 1409.004537368329920, 269.1701810006979940 ) ) ;
#700=CARTESIAN_POINT ( 'NONE',  ( 0.2895775691657055395, 1465.119059868797649, 238.1348893659934163 ) ) ;
#701=CARTESIAN_POINT ( 'NONE',  ( 19.27463171960000210, 1449.732551075340098, 192.4184640539980080 ) ) ;
#702=CARTESIAN_POINT ( 'NONE',  ( 24.65284846709989708, 1440.998862877870124, 212.5088464049670165 ) ) ;
#704=CARTESIAN_POINT ( 'NONE',  ( 7.659302844740099481, 1423.043197802409850, 144.1531582648829897 ) ) ;
#705=CARTESIAN_POINT ( 'NONE',  ( -40.27308333479999902, 1443.612076741559804, 137.1163319701979901 ) ) ;
#706=CARTESIAN_POINT ( 'NONE',  ( -10.16044903509999919, 1409.267871086030027, 197.9277695215979804 ) ) ;
#708=CARTESIAN_POINT ( 'NONE',  ( -13.22118898579999957, 1444.932341167249888, 187.3828105311979755 ) ) ;
#716=CARTESIAN_POINT ( 'NONE',  ( -13.94158961581099909, 1409.399911424660104, 214.4877138614390049 ) ) ;
#719=CARTESIAN_POINT ( 'NONE',  ( -27.07554453849999732, 1469.469472506630154, 267.2274423915979469 ) ) ;
#722=CARTESIAN_POINT ( 'NONE',  ( -24.69949338820000051, 1509.552011439729995, 222.6391731870980095 ) ) ;
#725=CARTESIAN_POINT ( 'NONE',  ( 18.26877678840750008, 1425.191339344029757, 225.8970440910269701 ) ) ;
#726=CARTESIAN_POINT ( 'NONE',  ( 12.08615242671140066, 1415.948038442619918, 223.4005273077049765 ) ) ;
#727=CARTESIAN_POINT ( 'NONE',  ( -25.76956215509200021, 1482.721195220700110, 211.7561243727609792 ) ) ;
#729=CARTESIAN_POINT ( 'NONE',  ( 15.57748978360000081, 1507.212883781729943, 225.5460497861979832 ) ) ;
#730=CARTESIAN_POINT ( 'NONE',  ( -22.96623755599999939, 1411.075251688929939, 204.6605450660979955 ) ) ;
#731=CARTESIAN_POINT ( 'NONE',  ( 16.64491405800000123, 1416.823872462129884, 201.3696481352879744 ) ) ;
#734=CARTESIAN_POINT ( 'NONE',  ( 0.8217888514169999770, 1435.943783413959864, 150.5249316333980119 ) ) ;
#740=CARTESIAN_POINT ( 'NONE',  ( -22.98253258309999936, 1410.218983115129959, 210.7724375874179827 ) ) ;
#742=CARTESIAN_POINT ( 'NONE',  ( 11.73122089892409825, 1426.699629391450117, 143.7537667490180127 ) ) ;
#747=CARTESIAN_POINT ( 'NONE',  ( -16.78507759299379742, 1507.483737884730090, 224.6466592809620124 ) ) ;
#752=CARTESIAN_POINT ( 'NONE',  ( 2.347965563550000301, 1508.995053151729962, 237.7725118035979790 ) ) ;
#755=AXIS2_PLACEMENT_3D ( 'NONE', #2441, #37107, #38202 ) ;
#758=VERTEX_POINT ( 'NONE', #45580 ) ;
#759=CARTESIAN_POINT ( 'NONE',  ( 11.75556087652499926, 1433.789100478620185, 150.9322770634290123 ) ) ;
#760=CARTESIAN_POINT ( 'NONE',  ( 27.31421232490000151, 1509.629811259429971, 216.2265006051580087 ) ) ;
#765=CARTESIAN_POINT ( 'NONE',  ( 16.02929450434690040, 1422.680592063800077, 191.1517350126889880 ) ) ;
#766=CARTESIAN_POINT ( 'NONE',  ( 11.44291537990000052, 1428.994970000029980, 123.0297916884979941 ) ) ;
#767=CARTESIAN_POINT ( 'NONE',  ( 17.01221803259009846, 1498.111302379200197, 230.6454121440009999 ) ) ;
#768=CARTESIAN_POINT ( 'NONE',  ( 1.117474349349999896, 1507.642466864929929, 181.0315143037979908 ) ) ;
#770=CARTESIAN_POINT ( 'NONE',  ( 16.66093349880000218, 1410.867388286930009, 226.5061864343979892 ) ) ;
#772=B_SPLINE_SURFACE_WITH_KNOTS ( 'NONE', 2, 5, ( 
 ( #84505, #49271, #41415, #48725, #102402, #40297 ),
 ( #32462, #76660, #83398, #67178, #6696, #41961 ),
 ( #75582, #40851, #68295, #25685, #42502, #34103 ) ),
 .UNSPECIFIED., .F., .F., .F.,
 ( 3, 3 ),
 ( 6, 6 ),
 ( 110.5970879970000027, 111.5653054569999938 ),
 ( 0.000000000000000000, 2.000000000000000000 ),
 .UNSPECIFIED. ) ;
#774=CARTESIAN_POINT ( 'NONE',  ( 34.51820589317019738, 1435.725758536269950, 134.0999999979759707 ) ) ;
#775=CARTESIAN_POINT ( 'NONE',  ( 11.86065779849999835, 1431.955919823459908, 149.9698378302979904 ) ) ;
#778=CARTESIAN_POINT ( 'NONE',  ( 13.87416642867090033, 1435.529565567879899, 149.9384610393090043 ) ) ;
#780=ORIENTED_EDGE ( 'NONE', *, *, #54473, .F. ) ;
#781=ORIENTED_EDGE ( 'NONE', *, *, #58768, .F. ) ;
#783=CARTESIAN_POINT ( 'NONE',  ( -1.085556744230000037, 1465.968794482429985, 235.6834014363979861 ) ) ;
#787=B_SPLINE_SURFACE_WITH_KNOTS ( 'NONE', 5, 5, ( 
 ( #32606, #26391, #34802, #33141, #68434, #7942 ),
 ( #84645, #17418, #9047, #50521, #109323, #110407 ),
 ( #25828, #7398, #92491, #43221, #42111, #33686 ),
 ( #68990, #67330, #77370, #67881, #103091, #76258 ),
 ( #60586, #101990, #101427, #25276, #59477, #40994 ),
 ( #93588, #66783, #100882, #42658, #15760, #49961 ) ),
 .UNSPECIFIED., .F., .F., .F.,
 ( 6, 6 ),
 ( 6, 6 ),
 ( 78.28065062529999807, 157.9815185129999975 ),
 ( -1.387778780779999841E-17, 1.000000000000000000 ),
 .UNSPECIFIED. ) ;
#793=ORIENTED_EDGE ( 'NONE', *, *, #35735, .T. ) ;
#797=CARTESIAN_POINT ( 'NONE',  ( -11.02381067019999961, 1409.298020338630067, 190.3753894067980070 ) ) ;
#800=EDGE_LOOP ( 'NONE', ( #73155, #27198, #21110, #74200 ) ) ;
#801=CARTESIAN_POINT ( 'NONE',  ( 24.19772972739999872, 1436.897348058309944, 213.7003709038880004 ) ) ;
#808=B_SPLINE_SURFACE_WITH_KNOTS ( 'NONE', 5, 5, ( 
 ( #65474, #14479, #6091, #93945, #7205, #59825 ),
 ( #25077, #84991, #67126, #76062, #24526, #85539 ),
 ( #58714, #68240, #110759, #101226, #33478, #86113 ),
 ( #15566, #92847, #49767, #17212, #1032, #8835 ),
 ( #102889, #16125, #42448, #8286, #59280, #51408 ),
 ( #25633, #67680, #50330, #84457, #7743, #93398 ) ),
 .UNSPECIFIED., .F., .F., .F.,
 ( 6, 6 ),
 ( 6, 6 ),
 ( 31.15146009760000112, 168.5477119569999900 ),
 ( 0.000000000000000000, 2.000000000000000000 ),
 .UNSPECIFIED. ) ;
#813=CARTESIAN_POINT ( 'NONE',  ( 28.24318409530000196, 1508.132100788830030, 208.6373738428400202 ) ) ;
#815=CARTESIAN_POINT ( 'NONE',  ( 13.04207770780000075, 1409.368499776629960, 192.3005056216980222 ) ) ;
#816=CARTESIAN_POINT ( 'NONE',  ( -18.12145421590813044, 1486.178648751641958, 188.5740549209106405 ) ) ;
#819=CARTESIAN_POINT ( 'NONE',  ( 38.63863155180000319, 1453.572278011729850, 261.7057835891980631 ) ) ;
#822=CARTESIAN_POINT ( 'NONE',  ( -3.857078437385809799, 1508.816503730140084, 237.6133849306840204 ) ) ;
#823=CARTESIAN_POINT ( 'NONE',  ( -20.12017060440000193, 1455.134694269430156, 226.3336132045979809 ) ) ;
#825=B_SPLINE_CURVE_WITH_KNOTS ( 'NONE', 3,
 ( #47399, #92685, #7583, #51245, #24372, #75897, #76443, #110598, #102187, #51810, #15416, #50694, #110049, #101619, #24907, #15960, #58007, #49607, #34444, #25467, #26016, #84292, #75365, #33322, #67518, #68620, #77560, #102722, #60213, #66420, #58557, #7036, #59115, #32780, #85378, #50164, #93240, #41738, #109504, #16506, #84824, #8126, #94331, #17609, #83739, #85951, #66964 ),
 .UNSPECIFIED., .F., .F.,
 ( 4, 2, 2, 2, 1, 1, 1, 1, 1, 1, 2, 2, 2, 2, 2, 1, 1, 1, 1, 2, 2, 2, 2, 2, 1, 1, 1, 2, 2, 4 ),
 ( 0.000000000000000000, 0.1249999999994302891, 0.1874999999991454336, 0.2187499999990033250, 0.2343749999989332422, 0.2421874999988981869, 0.2460937499988812005, 0.2480468749988732624, 0.2490234374988696819, 0.2495117187488680166, 0.2497558593738682942, 0.2499999999988685717, 0.3749999999990826782, 0.4374999999991906474, 0.4687499999992447708, 0.4843749999992725264, 0.4921874999992852939, 0.4960937499992913446, 0.4980468749992940647, 0.4990234374992957855, 0.4999999999992974509, 0.6249999999994888533, 0.6874999999995836664, 0.7187499999996309619, 0.7343749999996548317, 0.7421874999996680433, 0.7460937499996733724, 0.7480468749996770361, 0.7499999999996806999, 1.000000000000000000 ),
 .UNSPECIFIED. ) ;
#826=CARTESIAN_POINT ( 'NONE',  ( 11.86750639809999974, 1432.440573318600173, 149.9822236389979935 ) ) ;
#827=CARTESIAN_POINT ( 'NONE',  ( 17.53216825571119841, 1409.785550747969864, 222.6111406110179871 ) ) ;
#828=CARTESIAN_POINT ( 'NONE',  ( 14.94707557629999961, 1464.413060387330006, 194.8657129345979797 ) ) ;
#833=CARTESIAN_POINT ( 'NONE',  ( 1.802378746250000008E-09, 1405.842710276529942, 267.2349610868979539 ) ) ;
#834=CARTESIAN_POINT ( 'NONE',  ( 27.68516841690000163, 1508.595246553930110, 207.6423249425380106 ) ) ;
#835=CIRCLE ( 'NONE', #7915, 0.5000000000000000000 ) ;
#836=EDGE_CURVE ( 'NONE', #3563, #58739, #41250, .T. ) ;
#837=CARTESIAN_POINT ( 'NONE',  ( 12.73048906560000049, 1416.839648772530154, 223.1309759830980113 ) ) ;
#843=CARTESIAN_POINT ( 'NONE',  ( 26.80761308193400083, 1435.433708684199928, 135.7240834635020121 ) ) ;
#844=CARTESIAN_POINT ( 'NONE',  ( 36.51307952743290031, 1449.798342968150109, 136.2643497551869984 ) ) ;
#851=CARTESIAN_POINT ( 'NONE',  ( 1.618115094650000030, 1427.197104430330000, 147.9439864917980287 ) ) ;
#852=CARTESIAN_POINT ( 'NONE',  ( 13.80586431050000051, 1434.979615221880067, 146.9208280877979860 ) ) ;
#853=ADVANCED_FACE ( 'NONE', ( #80261 ), #34845, .T. ) ;
#854=CARTESIAN_POINT ( 'NONE',  ( -1.041174743597367502, 1450.833881364289255, 181.5282326196627594 ) ) ;
#855=CARTESIAN_POINT ( 'NONE',  ( 16.89419322268659940, 1506.223051208969991, 188.1395524883149903 ) ) ;
#856=CARTESIAN_POINT ( 'NONE',  ( -2.024352074859999871E-09, 1476.050155969130174, 268.4837719564979466 ) ) ;
#859=CARTESIAN_POINT ( 'NONE',  ( -29.25495648809999949, 1509.872423546730033, 208.6412349914980098 ) ) ;
#864=CARTESIAN_POINT ( 'NONE',  ( -11.09572995843272025, 1418.539393402124688, 229.3725684295395411 ) ) ;
#865=CARTESIAN_POINT ( 'NONE',  ( -18.88067404609999755, 1416.254459047329874, 207.9833811512579871 ) ) ;
#867=CARTESIAN_POINT ( 'NONE',  ( 24.98946546190000007, 1435.376445165819860, 135.9357081857980063 ) ) ;
#868=CARTESIAN_POINT ( 'NONE',  ( -6.019553345473489969, 1396.123267822159733, 199.8697773833820008 ) ) ;
#869=ORIENTED_EDGE ( 'NONE', *, *, #24347, .T. ) ;
#872=CARTESIAN_POINT ( 'NONE',  ( -16.31993864512639902, 1409.491010191830128, 225.1742793860710208 ) ) ;
#873=CARTESIAN_POINT ( 'NONE',  ( 4.967309476820000569, 1440.444625599219989, 150.3089546883979892 ) ) ;
#879=CARTESIAN_POINT ( 'NONE',  ( 10.92028016000000079, 1426.083762019530013, 93.45830742669778601 ) ) ;
#882=CARTESIAN_POINT ( 'NONE',  ( -11.62823626630000184, 1433.009257201529863, 151.0297253050979975 ) ) ;
#883=CARTESIAN_POINT ( 'NONE',  ( -2.882041267162114728, 1419.632841759689200, 186.1906303718482434 ) ) ;
#887=CARTESIAN_POINT ( 'NONE',  ( 3.452230076589999808, 1448.972367684420078, 184.0844731014979914 ) ) ;
#888=EDGE_CURVE ( 'NONE', #28394, #99599, #66657, .T. ) ;
#893=CARTESIAN_POINT ( 'NONE',  ( -41.65927775779999820, 1443.915297666309925, 135.6909731803980037 ) ) ;
#895=CARTESIAN_POINT ( 'NONE',  ( -1.417330028740000136, 1471.777279435030096, 269.8655828747980081 ) ) ;
#900=CARTESIAN_POINT ( 'NONE',  ( -22.84654337453140016, 1507.483738429109962, 208.2307034531480099 ) ) ;
#902=CARTESIAN_POINT ( 'NONE',  ( -0.03232803257987929696, 1407.837594159410173, 195.9367397066039871 ) ) ;
#903=CARTESIAN_POINT ( 'NONE',  ( -24.18583280233420041, 1410.839831453439956, 268.2351350556830312 ) ) ;
#904=CARTESIAN_POINT ( 'NONE',  ( -13.81131977446409920, 1434.989890545529988, 148.7892102494269864 ) ) ;
#905=ORIENTED_EDGE ( 'NONE', *, *, #70766, .T. ) ;
#906=FACE_OUTER_BOUND ( 'NONE', #101893, .T. ) ;
#907=CARTESIAN_POINT ( 'NONE',  ( 13.76098194390000096, 1443.039742490210074, 189.2009281145979855 ) ) ;
#916=CARTESIAN_POINT ( 'NONE',  ( -16.49868107950000251, 1485.484778815929985, 187.9250925817980260 ) ) ;
#917=B_SPLINE_SURFACE_WITH_KNOTS ( 'NONE', 5, 4, ( 
 ( #86063, #103389, #26695, #52480, #50808 ),
 ( #76552, #25027, #8785, #9902, #78209 ),
 ( #58665, #1521, #16073, #35654, #69844 ),
 ( #50276, #101739, #33428, #76004, #84405 ),
 ( #110708, #33998, #7692, #68191, #110157 ),
 ( #67625, #17159, #59229, #93346, #51352 ),
 ( #16611, #102295, #25580, #59773, #27259 ),
 ( #105074, #3195, #70400, #38407, #87738 ),
 ( #36767, #27816, #37875, #55240, #61442 ) ),
 .UNSPECIFIED., .F., .F., .F.,
 ( 6, 3, 6 ),
 ( 5, 5 ),
 ( 0.000000000000000000, 5.782490304330000441, 11.25975508159999983 ),
 ( 40.20365518519999881, 50.26548245740000453 ),
 .UNSPECIFIED. ) ;
#921=EDGE_CURVE ( 'NONE', #25855, #45625, #9330, .T. ) ;
#924=CARTESIAN_POINT ( 'NONE',  ( -27.91817790900000062, 1509.614502511829869, 204.0422066038080118 ) ) ;
#929=CARTESIAN_POINT ( 'NONE',  ( -6.294750371550000168, 1408.079328834029866, 197.5408074072979900 ) ) ;
#931=CARTESIAN_POINT ( 'NONE',  ( -8.892386117350001840, 1446.653515387309881, 186.0933241611980122 ) ) ;
#932=ORIENTED_EDGE ( 'NONE', *, *, #44106, .F. ) ;
#934=CARTESIAN_POINT ( 'NONE',  ( 27.66125109210000232, 1508.130528729329853, 212.4510895349179975 ) ) ;
#935=CARTESIAN_POINT ( 'NONE',  ( 20.54804277566730164, 1497.617938160230096, 225.9533463448229895 ) ) ;
#937=CARTESIAN_POINT ( 'NONE',  ( -25.25411696669999984, 1436.161966705209807, 137.2604574136979920 ) ) ;
#944=VERTEX_POINT ( 'NONE', #19645 ) ;
#945=DIRECTION ( 'NONE',  ( -1.139478816419269183E-15, -0.7071067811865474617, -0.7071067811865474617 ) ) ;
#946=CARTESIAN_POINT ( 'NONE',  ( -12.69028397900000016, 1410.293270958429957, 227.9608284046979918 ) ) ;
#948=EDGE_LOOP ( 'NONE', ( #55161, #35565, #39412, #54250 ) ) ;
#952=CARTESIAN_POINT ( 'NONE',  ( 12.17388030439999902, 1434.392357979209919, 150.5457779309980140 ) ) ;
#953=CARTESIAN_POINT ( 'NONE',  ( 17.06601014015459938, 1459.307105401880108, 228.6469079145479952 ) ) ;
#955=CARTESIAN_POINT ( 'NONE',  ( -24.97341835772749974, 1509.778186992499968, 223.4246975716070267 ) ) ;
#958=CARTESIAN_POINT ( 'NONE',  ( 3.055333763765900386E-13, 1547.913060387330006, 209.1218459616979999 ) ) ;
#959=CARTESIAN_POINT ( 'NONE',  ( 4.223877582933059927, 1441.585397622020082, 166.9011155059120028 ) ) ;
#962=CARTESIAN_POINT ( 'NONE',  ( 19.75079307820000096, 1509.023212949429990, 188.3853951167980085 ) ) ;
#965=CARTESIAN_POINT ( 'NONE',  ( -11.96392952312879920, 1414.971349104640012, 197.5065749685350340 ) ) ;
#968=CARTESIAN_POINT ( 'NONE',  ( 2.967683387859999744, 1419.631902151829991, 185.2975656967979887 ) ) ;
#973=CARTESIAN_POINT ( 'NONE',  ( -16.64381284196683097, 1410.502069620746624, 191.7858560727107715 ) ) ;
#974=CARTESIAN_POINT ( 'NONE',  ( -3.143430252119999935, 1447.188759692610120, 156.1111700446979853 ) ) ;
#975=CARTESIAN_POINT ( 'NONE',  ( 18.88375791580248730, 1507.757577934934034, 229.9162092553959837 ) ) ;
#977=CYLINDRICAL_SURFACE ( 'NONE', #41279, 23.99999999999999289 ) ;
#979=CARTESIAN_POINT ( 'NONE',  ( 15.92242058219999912, 1419.011245157130134, 191.2650185718979685 ) ) ;
#981=CARTESIAN_POINT ( 'NONE',  ( -5.003798055078270579, 1509.217832977240050, 179.4360497324900052 ) ) ;
#982=ORIENTED_EDGE ( 'NONE', *, *, #84481, .T. ) ;
#984=CARTESIAN_POINT ( 'NONE',  ( 24.30724142280000066, 1449.842033426479929, 206.4729385141180273 ) ) ;
#985=ADVANCED_FACE ( 'NONE', ( #24529 ), #51856, .F. ) ;
#986=CARTESIAN_POINT ( 'NONE',  ( -27.94676419710000204, 1509.200065883529760, 210.6896604893480003 ) ) ;
#987=CARTESIAN_POINT ( 'NONE',  ( 10.30115261902779089, 1410.643515217512459, 188.8098223140025027 ) ) ;
#1000=CARTESIAN_POINT ( 'NONE',  ( -1.499372387922010219, 1414.913526845469960, 226.2260460821569836 ) ) ;
#1002=CARTESIAN_POINT ( 'NONE',  ( 19.95567201858020212, 1508.916776747199947, 229.6244079712500081 ) ) ;
#1003=ORIENTED_EDGE ( 'NONE', *, *, #66990, .T. ) ;
#1005=CARTESIAN_POINT ( 'NONE',  ( 19.48180575948950022, 1507.796555935530250, 229.4922617073300160 ) ) ;
#1006=CARTESIAN_POINT ( 'NONE',  ( 18.80464302510000252, 1425.801049065629968, 225.6039134470979945 ) ) ;
#1007=CARTESIAN_POINT ( 'NONE',  ( 39.59123454348529947, 1440.695445213330004, 136.7962490760550054 ) ) ;
#1009=FACE_OUTER_BOUND ( 'NONE', #20638, .T. ) ;
#1010=B_SPLINE_CURVE_WITH_KNOTS ( 'NONE', 3,
 ( #7991, #34299, #67381, #75763 ),
 .UNSPECIFIED., .F., .F.,
 ( 4, 4 ),
 ( -21.04253309989999821, -13.35595807039999983 ),
 .UNSPECIFIED. ) ;
#1014=CARTESIAN_POINT ( 'NONE',  ( -0.5200257809521398045, 1450.894900823177750, 181.6063032256765553 ) ) ;
#1015=CARTESIAN_POINT ( 'NONE',  ( -20.31333848799999942, 1485.909380060430067, 191.0034922223980232 ) ) ;
#1016=CARTESIAN_POINT ( 'NONE',  ( 4.136067035069999953, 1409.224821449829960, 186.6613252426980125 ) ) ;
#1018=CARTESIAN_POINT ( 'NONE',  ( -8.778727802480000619, 1440.670317285799911, 153.7060890884979756 ) ) ;
#1022=CARTESIAN_POINT ( 'NONE',  ( 0.8791005338980000250, 1507.105016923229869, 237.2044774393979765 ) ) ;
#1023=CARTESIAN_POINT ( 'NONE',  ( -16.09752958667184330, 1409.475198507421055, 193.0827175891761271 ) ) ;
#1025=CARTESIAN_POINT ( 'NONE',  ( -18.64672481365220236, 1416.851343896850040, 208.5597484336410048 ) ) ;
#1028=CARTESIAN_POINT ( 'NONE',  ( -41.68718522609999155, 1445.343426362629998, 269.6415487380980380 ) ) ;
#1029=CARTESIAN_POINT ( 'NONE',  ( -12.27023110815660090, 1416.839692126590080, 194.6640136892829958 ) ) ;
#1030=( BOUNDED_CURVE ( )  B_SPLINE_CURVE ( 3, ( #18335, #33476, #17766, #17209 ),
 .UNSPECIFIED., .F., .T. ) 
 B_SPLINE_CURVE_WITH_KNOTS ( ( 4, 4 ),
 ( 1.455430482180659846, 1.955768190241684801 ),
 .UNSPECIFIED. ) 
 CURVE ( )  GEOMETRIC_REPRESENTATION_ITEM ( )  RATIONAL_B_SPLINE_CURVE ( ( 1.000000000000000000, 0.9792470884949975307, 0.9792470884949975307, 1.000000000000000000 ) ) 
 REPRESENTATION_ITEM ( '' )  );
#1031=CARTESIAN_POINT ( 'NONE',  ( 17.59077139289999892, 1410.452734695029903, 223.9185061424979892 ) ) ;
#1032=CARTESIAN_POINT ( 'NONE',  ( 16.67080554670000225, 1468.816899178029871, 189.7273712455979933 ) ) ;
#1033=CARTESIAN_POINT ( 'NONE',  ( 7.215398911020000305, 1408.913060387329779, 192.6378332269979978 ) ) ;
#1035=CARTESIAN_POINT ( 'NONE',  ( -0.5943821362719999835, 1416.311719779230089, 227.7090535903980140 ) ) ;
#1036=CARTESIAN_POINT ( 'NONE',  ( -4.868964994320000628, 1417.652559593630031, 232.9301174602979927 ) ) ;
#1037=VECTOR ( 'NONE', #102245, 1000.000000000000114 ) ;
#1040=CARTESIAN_POINT ( 'NONE',  ( -45.89749746886590032, 1438.271440801009931, 268.5002330264039756 ) ) ;
#1041=CARTESIAN_POINT ( 'NONE',  ( -4.155669689119999788, 1439.704322410179884, 185.4969487639980059 ) ) ;
#1047=CARTESIAN_POINT ( 'NONE',  ( 2.173590492602480051, 1419.636778193369992, 225.2801662438579910 ) ) ;
#1049=CARTESIAN_POINT ( 'NONE',  ( -26.63614110428829918, 1451.915376940910164, 135.4244124481140261 ) ) ;
#1050=ORIENTED_EDGE ( 'NONE', *, *, #94463, .T. ) ;
#1051=CARTESIAN_POINT ( 'NONE',  ( -16.90339957579946883, 1409.749894849624980, 225.4593229189988222 ) ) ;
#1053=CARTESIAN_POINT ( 'NONE',  ( 14.72846402789999942, 1488.814055421829835, 193.8574964441980057 ) ) ;
#1056=CARTESIAN_POINT ( 'NONE',  ( 9286.692186617183324, 54.07981494723826188, 5933.209537376913431 ) ) ;
#1058=CARTESIAN_POINT ( 'NONE',  ( -4.923540592713549380, 1408.758099391689939, 270.4264005896910135 ) ) ;
#1060=CARTESIAN_POINT ( 'NONE',  ( 12.66870000556460063, 1420.756754707929758, 231.4278130761680075 ) ) ;
#1061=CARTESIAN_POINT ( 'NONE',  ( -2.820595776548121325, 1448.944293396918511, 184.2202240992435236 ) ) ;
#1063=ORIENTED_EDGE ( 'NONE', *, *, #85947, .T. ) ;
#1064=ORIENTED_EDGE ( 'NONE', *, *, #95879, .F. ) ;
#1065=CARTESIAN_POINT ( 'NONE',  ( -23.55029577264210161, 1410.981915973860168, 210.4743339238279987 ) ) ;
#1066=CARTESIAN_POINT ( 'NONE',  ( -0.2881951457637970115, 1409.862531581090025, 185.0446401549079951 ) ) ;
#1067=CARTESIAN_POINT ( 'NONE',  ( 8.742163716520650412E-12, 1408.913060387359792, 224.1216835645979870 ) ) ;
#1068=CARTESIAN_POINT ( 'NONE',  ( -10.60629226371171363, 1406.913668871433856, 266.9166996103302836 ) ) ;
#1069=CARTESIAN_POINT ( 'NONE',  ( -19.79232061065411230, 1436.421083345947181, 145.6892389591389758 ) ) ;
#1070=CARTESIAN_POINT ( 'NONE',  ( -20.24778872499999949, 1425.809854017930093, 221.9168427389980138 ) ) ;
#1072=CARTESIAN_POINT ( 'NONE',  ( 28.26910033551460089, 1468.093474929750073, 269.2153630842319672 ) ) ;
#1073=CIRCLE ( 'NONE', #8153, 2.000001664945928237 ) ;
#1074=CARTESIAN_POINT ( 'NONE',  ( -2.606055286189628450, 1466.874310772752096, 235.1271370871118336 ) ) ;
#1075=CARTESIAN_POINT ( 'NONE',  ( -16.93175146515636698, 1421.930406924298040, 226.8423588672406481 ) ) ;
#1078=CARTESIAN_POINT ( 'NONE',  ( 22.30287194801498529, 1411.052071534360493, 215.4069906866415067 ) ) ;
#1079=CARTESIAN_POINT ( 'NONE',  ( 1.478215794333419986, 1479.409301536299836, 182.3215185385770098 ) ) ;
#1080=CARTESIAN_POINT ( 'NONE',  ( 22.81124892260000081, 1409.735994817030132, 208.6040538833909750 ) ) ;
#1083=CARTESIAN_POINT ( 'NONE',  ( 25.70093099836839912, 1451.138728924780025, 136.7959740386000078 ) ) ;
#1088=CARTESIAN_POINT ( 'NONE',  ( 17.47690429329999873, 1409.523367334130171, 194.5251149749979902 ) ) ;
#1089=CARTESIAN_POINT ( 'NONE',  ( 13.14421740897469704, 1444.740067931810472, 164.8757063741590230 ) ) ;
#1090=CARTESIAN_POINT ( 'NONE',  ( 3.464405900125376192, 1439.692844575363779, 184.4811232741128606 ) ) ;
#1092=CARTESIAN_POINT ( 'NONE',  ( -19.21510248855428671, 1425.233830981570009, 223.8702727496656166 ) ) ;
#1094=CARTESIAN_POINT ( 'NONE',  ( -0.2712433553410000253, 1477.454346902830139, 230.1237008569979992 ) ) ;
#1096=CARTESIAN_POINT ( 'NONE',  ( 12.36909147134636200, 1420.627402783089792, 231.5461179624636827 ) ) ;
#1099=CARTESIAN_POINT ( 'NONE',  ( 11.86610049460949945, 1432.336025080309810, 149.9824239092829998 ) ) ;
#1100=CARTESIAN_POINT ( 'NONE',  ( -0.3086018725757560532, 1408.964127551420006, 232.0914413854790155 ) ) ;
#1104=ADVANCED_FACE ( 'NONE', ( #87795 ), #91996, .T. ) ;
#1105=CARTESIAN_POINT ( 'NONE',  ( -8.800012970690000103, 1452.709869713229864, 209.1218459616979999 ) ) ;
#1107=CARTESIAN_POINT ( 'NONE',  ( 11.03413976350000070, 1433.575028546920066, 151.7351373796979885 ) ) ;
#1109=CARTESIAN_POINT ( 'NONE',  ( 3.268607919819999985, 1455.844446582929777, 219.6133833292979887 ) ) ;
#1112=CARTESIAN_POINT ( 'NONE',  ( 22.92687821287369943, 1507.614846683499991, 210.5904746357119848 ) ) ;
#1114=CARTESIAN_POINT ( 'NONE',  ( -9.700213616599999256, 1486.381094227929907, 183.3052980329979960 ) ) ;
#1116=CARTESIAN_POINT ( 'NONE',  ( -29.14871631793969797, 1509.943938004060101, 200.6668815711279876 ) ) ;
#1117=CARTESIAN_POINT ( 'NONE',  ( 21.05081438130000038, 1449.791259190219989, 221.6945081341980313 ) ) ;
#1119=CARTESIAN_POINT ( 'NONE',  ( 2.500000000000000000, 1448.210448412289907, 170.5244215879980061 ) ) ;
#1120=CARTESIAN_POINT ( 'NONE',  ( 25.18702156009318927, 1436.605886283166228, 137.6040374641183348 ) ) ;
#1128=CARTESIAN_POINT ( 'NONE',  ( -0.9043165181340000469, 1416.826388557929931, 228.0290525373980017 ) ) ;
#1131=CARTESIAN_POINT ( 'NONE',  ( -37.84675541842290158, 1450.538956397279890, 134.0999999985309898 ) ) ;
#1132=ORIENTED_EDGE ( 'NONE', *, *, #72781, .T. ) ;
#1149=CARTESIAN_POINT ( 'NONE',  ( -15.78459950990369975, 1409.489682787220090, 225.5863767987009965 ) ) ;
#1153=ORIENTED_EDGE ( 'NONE', *, *, #25538, .F. ) ;
#1158=CARTESIAN_POINT ( 'NONE',  ( 35.60280822696602598, 1457.100005120390506, 269.5399490414274055 ) ) ;
#1162=CARTESIAN_POINT ( 'NONE',  ( 21.56441682630240209, 1490.297454983860234, 209.3949090393569747 ) ) ;
#1163=CARTESIAN_POINT ( 'NONE',  ( -20.79162153139938951, 1507.840283869027871, 228.0156022542989263 ) ) ;
#1168=CARTESIAN_POINT ( 'NONE',  ( -2.500000000000000000, 1438.826994403640128, 157.7142568068980211 ) ) ;
#1171=EDGE_LOOP ( 'NONE', ( #75646, #66184, #110162, #28068 ) ) ;
#1172=AXIS2_PLACEMENT_3D ( 'NONE', #32306, #7103, #49123 ) ;
#1176=CARTESIAN_POINT ( 'NONE',  ( -24.70281712020000242, 1449.797141331690000, 204.5697651700980089 ) ) ;
#1177=CARTESIAN_POINT ( 'NONE',  ( -11.57305820287779952, 1425.905705694889775, 139.7073144656000068 ) ) ;
#1178=CARTESIAN_POINT ( 'NONE',  ( 16.82553512313559807, 1410.448925550840158, 191.9397864464299914 ) ) ;
#1180=CARTESIAN_POINT ( 'NONE',  ( 24.41443735958936401, 1509.880090222447734, 191.6102450087062152 ) ) ;
#1181=CARTESIAN_POINT ( 'NONE',  ( 12.53380499169999851, 1442.773887286369927, 169.4755105685979970 ) ) ;
#1182=CARTESIAN_POINT ( 'NONE',  ( -13.60515979240000028, 1408.134947171630074, 264.8398025118980286 ) ) ;
#1183=CARTESIAN_POINT ( 'NONE',  ( 15.67891837840150160, 1509.462974027039991, 234.0097172023010046 ) ) ;
#1184=CARTESIAN_POINT ( 'NONE',  ( 18.22805055419890152, 1459.311389626190021, 227.8763770136359881 ) ) ;
#1186=CARTESIAN_POINT ( 'NONE',  ( -34.47180251477740143, 1437.054646050100018, 136.5467630333359921 ) ) ;
#1187=ORIENTED_EDGE ( 'NONE', *, *, #109085, .T. ) ;
#1188=CARTESIAN_POINT ( 'NONE',  ( 6.220296828871760830, 1397.477110675040194, 220.4683221253430077 ) ) ;
#1190=CARTESIAN_POINT ( 'NONE',  ( -16.32194098420000117, 1459.453082325529977, 228.9511321261979901 ) ) ;
#1194=CARTESIAN_POINT ( 'NONE',  ( -3.134082760970000159, 1421.411057458130017, 144.1516174827979739 ) ) ;
#1199=CARTESIAN_POINT ( 'NONE',  ( -3.859940384109999734, 1461.192844946329842, 234.5475963274979847 ) ) ;
#1204=EDGE_LOOP ( 'NONE', ( #64781, #77382, #86140, #102380, #14395, #88297, #13141, #23084, #98114, #72274 ) ) ;
#1207=ORIENTED_EDGE ( 'NONE', *, *, #69473, .T. ) ;
#1208=CARTESIAN_POINT ( 'NONE',  ( 11.75126242882070038, 1426.765985215520004, 145.1646422661519864 ) ) ;
#1209=DIRECTION ( 'NONE',  ( 1.000000000000000000, 0.000000000000000000, 0.000000000000000000 ) ) ;
#1211=CARTESIAN_POINT ( 'NONE',  ( -1.440135193375450040, 1453.598502451769946, 183.7985014132709978 ) ) ;
#1212=CARTESIAN_POINT ( 'NONE',  ( -13.14421740897469704, 1443.086052842850677, 164.8757063741590230 ) ) ;
#1213=CARTESIAN_POINT ( 'NONE',  ( 4.916348328289999792, 1507.184349319130206, 235.7144663231979962 ) ) ;
#1215=CARTESIAN_POINT ( 'NONE',  ( -4.976708597980000093, 1421.169633119030095, 186.3323561761980045 ) ) ;
#1216=CARTESIAN_POINT ( 'NONE',  ( 3.048590950930369914, 1410.469311925999818, 269.3357931879770035 ) ) ;
#1223=CARTESIAN_POINT ( 'NONE',  ( 15.32936212569999945, 1453.152003547329969, 195.3739065139980084 ) ) ;
#1225=CARTESIAN_POINT ( 'NONE',  ( 17.95685989722359821, 1422.251379684970061, 225.1386422400370009 ) ) ;
#1226=CARTESIAN_POINT ( 'NONE',  ( -10.70847609427080016, 1506.854789404229905, 189.5201119528840081 ) ) ;
#1230=CARTESIAN_POINT ( 'NONE',  ( -2.898745121111036660, 1484.370110010407188, 183.3086963780446581 ) ) ;
#1235=CARTESIAN_POINT ( 'NONE',  ( -24.23599894299999846, 1443.366957020490190, 211.5779768989180241 ) ) ;
#1236=CARTESIAN_POINT ( 'NONE',  ( -11.81055660949999897, 1428.757038210530027, 148.7013752713980068 ) ) ;
#1240=CARTESIAN_POINT ( 'NONE',  ( 13.16277144537490074, 1428.831732683049950, 222.5358085910779948 ) ) ;
#1242=CARTESIAN_POINT ( 'NONE',  ( 11.16993257140000040, 1412.737055366430013, 229.4626520222979877 ) ) ;
#1244=CARTESIAN_POINT ( 'NONE',  ( -16.80253214529999894, 1461.096644362530014, 228.2779737265979918 ) ) ;
#1246=CARTESIAN_POINT ( 'NONE',  ( 23.35190786599999768, 1411.509783186830191, 269.4730611836980074 ) ) ;
#1247=CARTESIAN_POINT ( 'NONE',  ( 23.17024198529999879, 1435.306528354219836, 138.2719568257980143 ) ) ;
#1248=CARTESIAN_POINT ( 'NONE',  ( 18.06189968659999678, 1430.309388431030129, 192.0308204566979953 ) ) ;
#1249=CARTESIAN_POINT ( 'NONE',  ( -23.46079095940000059, 1434.934186800890075, 213.0598433132079776 ) ) ;
#1253=CARTESIAN_POINT ( 'NONE',  ( -41.66134498533040187, 1443.796928201230003, 135.6885309535949773 ) ) ;
#1254=CARTESIAN_POINT ( 'NONE',  ( -6.244762112600730219, 1407.784308377609932, 197.6511685975619912 ) ) ;
#1256=CARTESIAN_POINT ( 'NONE',  ( -12.41994595579999938, 1442.757755574029943, 186.2442043369979956 ) ) ;
#1257=ADVANCED_FACE ( 'NONE', ( #14112 ), #32095, .T. ) ;
#1259=CARTESIAN_POINT ( 'NONE',  ( -30.79851420400000350, 1435.573204670519999, 135.5995097962980083 ) ) ;
#1261=EDGE_LOOP ( 'NONE', ( #28337, #104669, #33068, #9186 ) ) ;
#1263=CARTESIAN_POINT ( 'NONE',  ( -12.51401920766459952, 1409.350059567480230, 200.9511622912029907 ) ) ;
#1267=CARTESIAN_POINT ( 'NONE',  ( -12.67405358299999918, 1474.477408728030014, 268.9829747063979539 ) ) ;
#1270=CARTESIAN_POINT ( 'NONE',  ( -24.51545692169827362, 1444.726069595008994, 210.9879020001179697 ) ) ;
#1273=CARTESIAN_POINT ( 'NONE',  ( 18.27461809169380302, 1424.830734655089827, 227.7279702984320124 ) ) ;
#1274=CARTESIAN_POINT ( 'NONE',  ( 21.32829263799999708, 1509.431654392129985, 227.8062006340979906 ) ) ;
#1275=CARTESIAN_POINT ( 'NONE',  ( 14.47057979809999928, 1463.299097360029918, 223.0641482907979878 ) ) ;
#1276=CARTESIAN_POINT ( 'NONE',  ( -26.33121976050560065, 1495.363534167619946, 211.7508342357739934 ) ) ;
#1278=CARTESIAN_POINT ( 'NONE',  ( -8.125988388849998856, 1509.268893885830039, 180.2859049925980059 ) ) ;
#1279=CARTESIAN_POINT ( 'NONE',  ( -23.87261416360000155, 1410.668553464130127, 207.8050958171579907 ) ) ;
#1280=CARTESIAN_POINT ( 'NONE',  ( 16.76079635960000047, 1415.087818611729972, 206.4452941520080174 ) ) ;
#1283=CARTESIAN_POINT ( 'NONE',  ( 1.643576684049999903, 1435.943783413959864, 150.4860296878979682 ) ) ;
#1290=CARTESIAN_POINT ( 'NONE',  ( 0.7174281048909999514, 1414.384036990830054, 233.3111233936980113 ) ) ;
#1298=CARTESIAN_POINT ( 'NONE',  ( 2.798741256239999586, 1509.010794585629810, 238.1786444319979807 ) ) ;
#1303=ORIENTED_EDGE ( 'NONE', *, *, #97292, .F. ) ;
#1304=VERTEX_POINT ( 'NONE', #22492 ) ;
#1305=CARTESIAN_POINT ( 'NONE',  ( 11.94418194357199958, 1433.568413397649920, 150.1854698904059831 ) ) ;
#1307=EDGE_LOOP ( 'NONE', ( #102465, #35282, #41395, #32770 ) ) ;
#1309=CARTESIAN_POINT ( 'NONE',  ( -22.39336929169999735, 1508.437846497230112, 193.8456439799980160 ) ) ;
#1311=CARTESIAN_POINT ( 'NONE',  ( 10.96946812545280103, 1432.347663862999980, 151.7701354189910035 ) ) ;
#1312=CARTESIAN_POINT ( 'NONE',  ( 2.205156445730000137, 1428.435894572430016, 91.31218443469779800 ) ) ;
#1313=CARTESIAN_POINT ( 'NONE',  ( 13.28903619059999919, 1507.808443900629982, 233.1137254224979927 ) ) ;
#1314=CARTESIAN_POINT ( 'NONE',  ( 3.162092520659999906, 1488.171764278530190, 182.3076926873980028 ) ) ;
#1316=CARTESIAN_POINT ( 'NONE',  ( -24.43504968562070445, 1444.778680445579994, 211.0911670020710176 ) ) ;
#1318=CARTESIAN_POINT ( 'NONE',  ( 36.90142499543770072, 1436.372079654780009, 134.0999999968939846 ) ) ;
#1321=EDGE_LOOP ( 'NONE', ( #91856, #48422, #19864, #38432, #109528, #81310, #103020, #40751, #105848, #86397, #80547, #54136, #50283, #42213, #34449, #7573, #54234, #106974, #18075, #43433 ) ) ;
#1322=CARTESIAN_POINT ( 'NONE',  ( 14.38916750008629997, 1435.820125812520018, 149.8242534154239820 ) ) ;
#1325=VERTEX_POINT ( 'NONE', #56693 ) ;
#1328=CARTESIAN_POINT ( 'NONE',  ( 5.157704406284129827E-09, 1406.911841301380036, 222.1218459627310153 ) ) ;
#1332=DIRECTION ( 'NONE',  ( -0.9993779840591179298, 0.0009463129470705568952, 0.03525265195329010254 ) ) ;
#1334=CARTESIAN_POINT ( 'NONE',  ( 4.221309089957250293, 1446.219906947470236, 169.0695559285369995 ) ) ;
#1335=( BOUNDED_CURVE ( )  B_SPLINE_CURVE ( 3, ( #24512, #18735, #33463, #84443 ),
 .UNSPECIFIED., .F., .F. ) 
 B_SPLINE_CURVE_WITH_KNOTS ( ( 4, 4 ),
 ( 4.625649227539959440, 4.863861644479719359 ),
 .UNSPECIFIED. ) 
 CURVE ( )  GEOMETRIC_REPRESENTATION_ITEM ( )  RATIONAL_B_SPLINE_CURVE ( ( 1.000000000000000000, 0.9952768246915880690, 0.9952768246915880690, 1.000000000000000000 ) ) 
 REPRESENTATION_ITEM ( '' )  );
#1339=ORIENTED_EDGE ( 'NONE', *, *, #56860, .T. ) ;
#1340=CARTESIAN_POINT ( 'NONE',  ( 23.15392403432699808, 1440.913060387330006, 232.3890819680619870 ) ) ;
#1341=CARTESIAN_POINT ( 'NONE',  ( -20.05348316079999904, 1509.507670961230133, 230.4164826494980218 ) ) ;
#1344=CARTESIAN_POINT ( 'NONE',  ( -13.85637388489999999, 1409.898955760130093, 190.3611264359980169 ) ) ;
#1345=CARTESIAN_POINT ( 'NONE',  ( -24.91017436590000145, 1441.730135535790168, 210.4543706807980072 ) ) ;
#1347=CARTESIAN_POINT ( 'NONE',  ( 0.0002660152826350496214, 1396.305602673456860, 196.9300748754315293 ) ) ;
#1348=CARTESIAN_POINT ( 'NONE',  ( -13.80599379854099951, 1434.979619881170038, 146.4346930281899972 ) ) ;
#1356=DIRECTION ( 'NONE',  ( 0.1115146187057051708, 0.9937625037592048294, -0.0007589052364158857143 ) ) ;
#1357=CARTESIAN_POINT ( 'NONE',  ( 28.56957134109999785, 1509.608813749330011, 207.7212829969979850 ) ) ;
#1359=CARTESIAN_POINT ( 'NONE',  ( 13.61519732589999876, 1409.388513550129801, 192.1720528023979853 ) ) ;
#1360=CARTESIAN_POINT ( 'NONE',  ( -18.73404851560655615, 1486.221193578838211, 189.0895470789506305 ) ) ;
#1363=CARTESIAN_POINT ( 'NONE',  ( 43.15854606300000285, 1446.267111671710154, 263.9123177541979999 ) ) ;
#1366=CARTESIAN_POINT ( 'NONE',  ( -1.628803710539000082, 1508.952962138009980, 238.4908458976950101 ) ) ;
#1367=CARTESIAN_POINT ( 'NONE',  ( -20.01739162620000201, 1456.480130098429981, 225.1960475761980263 ) ) ;
#1369=CARTESIAN_POINT ( 'NONE',  ( 11.58215542740000181, 1432.723885441809898, 151.1956759764979950 ) ) ;
#1370=CARTESIAN_POINT ( 'NONE',  ( 17.99896784699780383, 1410.879795390830168, 222.9861481690849985 ) ) ;
#1371=CARTESIAN_POINT ( 'NONE',  ( -0.3789282637219999472, 1488.814055421429885, 187.9137241168980097 ) ) ;
#1373=ORIENTED_EDGE ( 'NONE', *, *, #31031, .F. ) ;
#1375=CARTESIAN_POINT ( 'NONE',  ( 0.5589011644189999517, 1405.751811759530028, 267.5370429348980110 ) ) ;
#1376=CARTESIAN_POINT ( 'NONE',  ( 27.92328160759999989, 1509.198544193830003, 207.5288794971980053 ) ) ;
#1378=CARTESIAN_POINT ( 'NONE',  ( 24.59810391050000078, 1443.913212907020124, 213.1604229849380090 ) ) ;
#1379=CARTESIAN_POINT ( 'NONE',  ( -24.15153490410000359, 1438.063247892820073, 212.1983423404379892 ) ) ;
#1382=CARTESIAN_POINT ( 'NONE',  ( -37.98804544047590070, 1440.913060390229930, 256.2617115235140091 ) ) ;
#1383=CARTESIAN_POINT ( 'NONE',  ( 37.45767776268139926, 1449.247412760440056, 136.3260996822840241 ) ) ;
#1384=CARTESIAN_POINT ( 'NONE',  ( -1.171202044737849945, 1450.815562201780040, 154.2439547528010166 ) ) ;
#1389=CARTESIAN_POINT ( 'NONE',  ( 19.74164504280149757, 1455.376031929259852, 226.0788368184279875 ) ) ;
#1391=CARTESIAN_POINT ( 'NONE',  ( 0.8066080222970000158, 1426.500992774829911, 146.0666368882980066 ) ) ;
#1392=CARTESIAN_POINT ( 'NONE',  ( 12.06136797880000167, 1433.903288664979982, 146.9203525914979878 ) ) ;
#1393=CARTESIAN_POINT ( 'NONE',  ( -1.387456962977127395, 1450.687505278765684, 181.9496466349601747 ) ) ;
#1394=CARTESIAN_POINT ( 'NONE',  ( 14.91734427364780124, 1443.896427911540059, 190.0889645647779957 ) ) ;
#1395=CARTESIAN_POINT ( 'NONE',  ( -0.8945447425290000698, 1417.298088064829926, 235.8147206259980067 ) ) ;
#1401=CARTESIAN_POINT ( 'NONE',  ( -18.50064172359999759, 1416.067629290630066, 208.4803912601460070 ) ) ;
#1402=CARTESIAN_POINT ( 'NONE',  ( -16.70118312301810093, 1414.971390223319986, 209.0342377526849873 ) ) ;
#1403=CARTESIAN_POINT ( 'NONE',  ( -9.960850764644041178, 1396.260900962979804, 204.3086104707440143 ) ) ;
#1405=CARTESIAN_POINT ( 'NONE',  ( -17.28133596328079946, 1410.461149824280028, 225.8190134910500149 ) ) ;
#1406=CARTESIAN_POINT ( 'NONE',  ( 2.455820327400000114, 1434.541746329560056, 150.3615916412979914 ) ) ;
#1408=ORIENTED_EDGE ( 'NONE', *, *, #89707, .F. ) ;
#1411=CARTESIAN_POINT ( 'NONE',  ( 11.05913215650000048, 1426.494667556230070, 94.99634540869780608 ) ) ;
#1413=DIRECTION ( 'NONE',  ( 0.1159387279768451934, 0.9932563673871469545, 0.000000000000000000 ) ) ;
#1414=CARTESIAN_POINT ( 'NONE',  ( -11.71296687490000110, 1433.008354761999954, 150.8502298933980228 ) ) ;
#1417=CARTESIAN_POINT ( 'NONE',  ( -2.708795395750633439, 1420.182185210162970, 186.0140258646650864 ) ) ;
#1420=CARTESIAN_POINT ( 'NONE',  ( 8.353214826769999490, 1509.201657029630042, 181.3236374839979987 ) ) ;
#1424=ORIENTED_EDGE ( 'NONE', *, *, #96163, .T. ) ;
#1426=CARTESIAN_POINT ( 'NONE',  ( -41.48601633919999188, 1444.048446191809944, 136.5661428469979910 ) ) ;
#1428=CARTESIAN_POINT ( 'NONE',  ( -2.230923574740000248, 1471.396667871830005, 269.3352507041980175 ) ) ;
#1430=CARTESIAN_POINT ( 'NONE',  ( -0.5791816274180000557, 1486.229018827529899, 181.7900702770979819 ) ) ;
#1434=CARTESIAN_POINT ( 'NONE',  ( -2.500000000000000000, 1448.206111001999943, 170.1385578322760068 ) ) ;
#1436=CARTESIAN_POINT ( 'NONE',  ( 13.11441086409999990, 1409.193432151429988, 216.3239404139079909 ) ) ;
#1437=CARTESIAN_POINT ( 'NONE',  ( -0.7694941353355659874, 1406.265043692640120, 269.2947833301390119 ) ) ;
#1439=VERTEX_POINT ( 'NONE', #8465 ) ;
#1440=CARTESIAN_POINT ( 'NONE',  ( -11.86550948169999842, 1432.301447584650077, 150.3971867772980033 ) ) ;
#1441=CARTESIAN_POINT ( 'NONE',  ( 13.54476740079999963, 1443.929709051740019, 188.0927821155979984 ) ) ;
#1442=ORIENTED_EDGE ( 'NONE', *, *, #72907, .T. ) ;
#1444=EDGE_LOOP ( 'NONE', ( #20128, #45401, #22569, #42921 ) ) ;
#1451=AXIS2_PLACEMENT_3D ( 'NONE', #97655, #36648, #80859 ) ;
#1453=ADVANCED_FACE ( 'NONE', ( #67858 ), #93650, .F. ) ;
#1458=ADVANCED_FACE ( 'NONE', ( #94687 ), #103644, .T. ) ;
#1459=B_SPLINE_CURVE_WITH_KNOTS ( 'NONE', 3,
 ( #105967, #71293, #62904, #97014, #89149, #20276, #46071, #54480, #3520, #65482, #71851, #12434, #99591, #48118, #102360, #101798, #25088, #66038, #110215, #7213, #32414, #17223, #93958, #91754, #15029, #75536, #83353, #110770, #51419, #49776, #100698, #49228, #76074, #76618, #7753, #85550, #50872, #66594, #6652, #85002, #109671, #59835, #109132 ),
 .UNSPECIFIED., .F., .F.,
 ( 4, 3, 3, 3, 3, 3, 3, 3, 3, 3, 3, 3, 3, 3, 4 ),
 ( -2.000000000000000000, -1.936215008427339956, -1.791913135960270020, -1.645609380878030104, -1.498043589331059966, -1.348593918407889891, -1.198178442218299944, -1.047113558058780036, -0.8957606298038101045, -0.7380121483472110722, -0.5877609036753239646, -0.4386042209462979180, -0.2908102820543170264, -0.1445690464712710011, 0.000000000000000000 ),
 .UNSPECIFIED. ) ;
#1460=CARTESIAN_POINT ( 'NONE',  ( 7.292853372139999735, 1414.971279908829956, 224.4496626855979855 ) ) ;
#1462=B_SPLINE_CURVE_WITH_KNOTS ( 'NONE', 5,
 ( #85322, #26530, #8071, #43357, #77504, #102127 ),
 .UNSPECIFIED., .F., .F.,
 ( 6, 6 ),
 ( -1.020724565110000093, 5.536280491323250175 ),
 .UNSPECIFIED. ) ;
#1463=CARTESIAN_POINT ( 'NONE',  ( -29.17336326509999722, 1509.870405653630087, 207.9069865368680041 ) ) ;
#1465=CARTESIAN_POINT ( 'NONE',  ( -0.5920813016230001002, 1487.765345405229937, 230.8947267201980083 ) ) ;
#1469=( BOUNDED_SURFACE ( )  B_SPLINE_SURFACE ( 3, 2, ( 
 ( #99789, #74073, #14692 ),
 ( #48881, #91415, #47213 ),
 ( #106559, #13573, #56157 ),
 ( #90292, #81893, #72427 ),
 ( #29846, #5196, #81339 ),
 ( #83007, #65671, #39351 ),
 ( #82464, #99234, #4120 ),
 ( #32049, #90848, #56713 ),
 ( #73527, #31491, #6299 ),
 ( #40446, #107661, #4653 ),
 ( #30947, #65122, #22511 ),
 ( #66238, #89206, #46682 ) ),
 .UNSPECIFIED., .F., .F., .T. ) 
 B_SPLINE_SURFACE_WITH_KNOTS ( ( 4, 2, 2, 2, 2, 4 ),
 ( 3, 3 ),
 ( 0.000000000000000000, 0.001069581499716159949, 0.001604372249574239923, 0.002139162999432319898, 0.003208744499148479846, 0.004278325998864639795 ),
 ( 0.000000000000000000, 1.000000000000000000 ),
 .UNSPECIFIED. ) 
 GEOMETRIC_REPRESENTATION_ITEM ( )  RATIONAL_B_SPLINE_SURFACE ( (
 ( 1.000000000000000000, 0.7071067811863054331, 1.000000000000000000),
 ( 1.000000000000000000, 0.7227602064011806604, 1.000000000000000000),
 ( 1.000000000000000000, 0.7381100937480321589, 1.000000000000000000),
 ( 1.000000000000000000, 0.7607230651862928461, 1.000000000000000000),
 ( 1.000000000000000000, 0.7681914495759601946, 1.000000000000000000),
 ( 1.000000000000000000, 0.7829826642569391870, 1.000000000000000000),
 ( 1.000000000000000000, 0.7903039095410622217, 1.000000000000000000),
 ( 1.000000000000000000, 0.8113823828798899518, 1.000000000000000000),
 ( 1.000000000000000000, 0.8244993778341390689, 1.000000000000000000),
 ( 1.000000000000000000, 0.8485230146284407082, 1.000000000000000000),
 ( 1.000000000000000000, 0.8591868199085809232, 1.000000000000000000),
 ( 1.000000000000000000, 0.8676549144810682401, 1.000000000000000000) ) ) 
 REPRESENTATION_ITEM ( '' )  SURFACE ( )  );
#1470=CARTESIAN_POINT ( 'NONE',  ( -6.244762126029999472, 1407.784308383030066, 197.6511686028979966 ) ) ;
#1472=CARTESIAN_POINT ( 'NONE',  ( -10.63892929799999898, 1445.506293354350191, 185.8359387749980272 ) ) ;
#1475=CARTESIAN_POINT ( 'NONE',  ( -25.85373363512699996, 1440.913060485959932, 221.0820133274520174 ) ) ;
#1476=CARTESIAN_POINT ( 'NONE',  ( 19.65515833015399849, 1477.262508678489894, 226.0632499707639909 ) ) ;
#1477=CARTESIAN_POINT ( 'NONE',  ( -24.35667143039999516, 1435.422350721090197, 137.0292528702979951 ) ) ;
#1478=AXIS2_PLACEMENT_3D ( 'NONE', #2381, #34836, #69582 ) ;
#1486=CARTESIAN_POINT ( 'NONE',  ( 4.363122647530000009, 1417.926080483629903, 166.9581667359979917 ) ) ;
#1493=CARTESIAN_POINT ( 'NONE',  ( 12.12127920967330041, 1433.956690957220189, 149.8582645731989942 ) ) ;
#1495=CARTESIAN_POINT ( 'NONE',  ( 16.68871050416229807, 1478.708306862099789, 229.8628164125950093 ) ) ;
#1497=CARTESIAN_POINT ( 'NONE',  ( -24.69773639504949969, 1509.761573056400039, 223.9593781233639902 ) ) ;
#1500=CARTESIAN_POINT ( 'NONE',  ( -0.04532349001890000062, 1409.423585831229957, 233.0275901203980027 ) ) ;
#1501=VECTOR ( 'NONE', #9818, 1000.000000000000114 ) ;
#1503=CARTESIAN_POINT ( 'NONE',  ( -3.770547026519999623, 1420.469916612930092, 186.2929298669980085 ) ) ;
#1504=CARTESIAN_POINT ( 'NONE',  ( 18.70459387589999878, 1509.566239198529956, 186.5372755683980017 ) ) ;
#1507=CARTESIAN_POINT ( 'NONE',  ( -12.73136601901759946, 1416.225364278609959, 196.2684121632169933 ) ) ;
#1509=CARTESIAN_POINT ( 'NONE',  ( -20.49035733430000050, 1504.313428628929842, 189.6781957060979948 ) ) ;
#1512=CARTESIAN_POINT ( 'NONE',  ( 2.677300865789999929, 1420.709102647230111, 184.9509449586979883 ) ) ;
#1517=CARTESIAN_POINT ( 'NONE',  ( -16.31009655498456823, 1409.653544930775070, 192.3727841784286738 ) ) ;
#1518=CARTESIAN_POINT ( 'NONE',  ( 17.56720881609999907, 1415.048591087029763, 210.3588846212080057 ) ) ;
#1519=CARTESIAN_POINT ( 'NONE',  ( -17.96296818009999896, 1424.130910211129958, 225.8903661153979954 ) ) ;
#1520=FACE_OUTER_BOUND ( 'NONE', #99932, .T. ) ;
#1521=CARTESIAN_POINT ( 'NONE',  ( -4.978523888090000682, 1441.600846913620217, 150.3430135618980046 ) ) ;
#1527=CARTESIAN_POINT ( 'NONE',  ( 1.556457968405000170, 1415.007830321620077, 191.6742979189480138 ) ) ;
#1529=CARTESIAN_POINT ( 'NONE',  ( -23.88515968680000157, 1436.380149434200121, 211.3762814741380112 ) ) ;
#1530=CARTESIAN_POINT ( 'NONE',  ( 8.915053209252663535, 1410.596227120273625, 188.0708813341610437 ) ) ;
#1533=CARTESIAN_POINT ( 'NONE',  ( -11.90000415720300175, 1434.913060496859998, 147.6452464505769910 ) ) ;
#1540=CARTESIAN_POINT ( 'NONE',  ( 21.54229287260000092, 1452.160786943630228, 141.5333698742980175 ) ) ;
#1541=ADVANCED_FACE ( 'NONE', ( #10697 ), #23125, .F. ) ;
#1543=CARTESIAN_POINT ( 'NONE',  ( 14.20882688731320975, 1410.783320216355833, 191.3835041209767951 ) ) ;
#1546=CARTESIAN_POINT ( 'NONE',  ( -18.07191983094158161, 1459.591554196664219, 227.9854841469545192 ) ) ;
#1551=FACE_OUTER_BOUND ( 'NONE', #21340, .T. ) ;
#1553=CARTESIAN_POINT ( 'NONE',  ( 39.14220602846550179, 1439.921242502060068, 136.7207080452419916 ) ) ;
#1554=CARTESIAN_POINT ( 'NONE',  ( 18.05542495219999921, 1416.825784017130218, 208.7596466302459817 ) ) ;
#1555=CARTESIAN_POINT ( 'NONE',  ( -40.57811314119999935, 1448.614249393429873, 261.6156832257979659 ) ) ;
#1559=CARTESIAN_POINT ( 'NONE',  ( -0.3197736172905292218, 1452.655606759615466, 183.2748911063349055 ) ) ;
#1560=CARTESIAN_POINT ( 'NONE',  ( -19.88544360889999751, 1484.719772526229917, 191.4492701382980044 ) ) ;
#1561=TOROIDAL_SURFACE ( 'NONE', #51590, 2.030931026690000252, 0.5000000000000000000 ) ;
#1562=CARTESIAN_POINT ( 'NONE',  ( 1.734313731699999916, 1409.141427551030120, 185.9428025286979960 ) ) ;
#1563=CARTESIAN_POINT ( 'NONE',  ( 5.808871921319999743, 1423.519516101330055, 186.0672565399979987 ) ) ;
#1564=CARTESIAN_POINT ( 'NONE',  ( -7.733451861169999830, 1440.968359749710089, 154.0956080340980066 ) ) ;
#1569=EDGE_LOOP ( 'NONE', ( #50451, #68937, #11902, #3529 ) ) ;
#1570=CARTESIAN_POINT ( 'NONE',  ( -2.398688105316478580, 1426.758990796949320, 141.3562649765487436 ) ) ;
#1572=CARTESIAN_POINT ( 'NONE',  ( -39.29615804430000026, 1457.459686057429963, 269.7910478776980199 ) ) ;
#1574=CARTESIAN_POINT ( 'NONE',  ( 6.510459374210000760, 1435.947057077009958, 154.7340827710979738 ) ) ;
#1578=CARTESIAN_POINT ( 'NONE',  ( 2.924524102719100238, 1410.358758242020031, 231.6291648917529926 ) ) ;
#1579=CARTESIAN_POINT ( 'NONE',  ( -1.455250893790000166, 1415.140114704729967, 226.9749634510980059 ) ) ;
#1580=CARTESIAN_POINT ( 'NONE',  ( -3.026978396589999676, 1416.096969111230010, 232.7842076799979907 ) ) ;
#1581=CARTESIAN_POINT ( 'NONE',  ( -1.068647241811354398, 1484.851163306396302, 182.1517477618084229 ) ) ;
#1583=CARTESIAN_POINT ( 'NONE',  ( -45.58450343905819580, 1439.256682012769943, 268.9762893008089577 ) ) ;
#1590=CARTESIAN_POINT ( 'NONE',  ( 19.26602811997136655, 1456.117940503140971, 225.0698710879842110 ) ) ;
#1591=CARTESIAN_POINT ( 'NONE',  ( -11.38922736439999994, 1425.413087568229912, 188.2682818651980199 ) ) ;
#1593=B_SPLINE_SURFACE_WITH_KNOTS ( 'NONE', 5, 5, ( 
 ( #91827, #49848, #15105, #82335, #66115, #75608, #109738, #107530, #49296, #22953, #91283, #100764 ),
 ( #83424, #64458, #90166, #39785, #73944, #108075, #39218, #48197, #6170, #99114, #31370, #6720 ),
 ( #73394, #30819, #64996, #108635, #40876, #65553, #57159, #14564, #48754, #82877, #75054, #27983 ),
 ( #41990, #85622, #93470, #16202, #102427, #34681, #50406, #86189, #61026, #76140, #9481, #110284 ),
 ( #77798, #68319, #85073, #8365, #24598, #556, #42533, #76686, #78349, #101304, #25158, #77257 ),
 ( #18409, #84532, #44205, #95149, #59910, #34131, #102972, #67754, #25709, #103536, #52607, #68869 ),
 ( #94031, #26270, #86743, #8921, #60460, #35235, #94578, #43645, #17295, #51491, #59362, #1107 ),
 ( #17854, #43096, #7820, #10035, #52054, #69423, #26839, #33019, #16741, #67206, #58791, #92930 ),
 ( #50948, #33560, #101865, #62125, #54817, #88942, #80000, #55365, #29052, #1658, #20614, #71648 ),
 ( #36337, #44766, #11694, #3324, #104095, #72182, #63238, #37449, #106301, #87870, #27944, #70530 ),
 ( #20083, #89498, #97344, #71083, #105208, #104647, #29584, #45867, #53732, #105767, #12234, #2223 ),
 ( #27386, #46424, #36889, #11160, #45321, #61565, #80556, #79459, #2769, #46969, #69979, #96252 ) ),
 .UNSPECIFIED., .F., .F., .F.,
 ( 6, 3, 3, 6 ),
 ( 6, 3, 3, 6 ),
 ( 8.878046405300000998, 9.092838726940000171, 9.522423370220000294, 9.923260654589999064 ),
 ( 0.000000000000000000, 0.6020156018279999577, 1.679451024060000019, 2.218168735169999906 ),
 .UNSPECIFIED. ) ;
#1597=CARTESIAN_POINT ( 'NONE',  ( 14.17386987649999952, 1470.816980702629962, 194.4171917781980028 ) ) ;
#1598=EDGE_CURVE ( 'NONE', #58469, #46920, #64728, .T. ) ;
#1599=CARTESIAN_POINT ( 'NONE',  ( 1.802870145850000050, 1411.461756991529910, 232.2427255196980127 ) ) ;
#1600=CARTESIAN_POINT ( 'NONE',  ( -11.50670236126252810, 1425.933829454640545, 139.0400858972396918 ) ) ;
#1605=CARTESIAN_POINT ( 'NONE',  ( -6.833925870029700533, 1408.295428044619939, 270.2841559995019907 ) ) ;
#1607=CARTESIAN_POINT ( 'NONE',  ( 4.139239280457269743, 1417.946269731450002, 233.0858131667390012 ) ) ;
#1610=ORIENTED_EDGE ( 'NONE', *, *, #15204, .F. ) ;
#1613=EDGE_CURVE ( 'NONE', #46627, #39656, #1849, .T. ) ;
#1614=CARTESIAN_POINT ( 'NONE',  ( -4.287767397939999725, 1424.648436861230039, 185.9532686480980033 ) ) ;
#1615=CARTESIAN_POINT ( 'NONE',  ( 3.709069522732904911, 1425.316856860248663, 185.1233798031099980 ) ) ;
#1616=CARTESIAN_POINT ( 'NONE',  ( -0.01642798734072890149, 1408.968555449449923, 186.0689978232310011 ) ) ;
#1618=CIRCLE ( 'NONE', #23085, 2.000000000000001776 ) ;
#1620=CARTESIAN_POINT ( 'NONE',  ( -20.52576279630359579, 1436.445955288497771, 144.8643394113350666 ) ) ;
#1621=CARTESIAN_POINT ( 'NONE',  ( -18.04944458410000152, 1425.819836014529983, 225.8836100296980192 ) ) ;
#1622=CARTESIAN_POINT ( 'NONE',  ( 29.82179391674280211, 1467.143751206999923, 269.1831960069300180 ) ) ;
#1623=CARTESIAN_POINT ( 'NONE',  ( -14.43048377810894500, 1462.029581583880372, 229.5409151307926265 ) ) ;
#1624=CARTESIAN_POINT ( 'NONE',  ( 8.735250064049999708, 1446.655199166789998, 185.9308358984979748 ) ) ;
#1627=FACE_OUTER_BOUND ( 'NONE', #78029, .T. ) ;
#1629=CARTESIAN_POINT ( 'NONE',  ( 22.66310764289999824, 1409.704358029729974, 208.7414267666439969 ) ) ;
#1631=CARTESIAN_POINT ( 'NONE',  ( -1.369904464291739954, 1457.995076032020052, 229.8762231575159944 ) ) ;
#1632=CARTESIAN_POINT ( 'NONE',  ( 24.51785944913020288, 1452.041301548709953, 136.2948944376120153 ) ) ;
#1636=CARTESIAN_POINT ( 'NONE',  ( 18.27919210119999960, 1410.914348715230062, 193.9485672390979971 ) ) ;
#1638=CARTESIAN_POINT ( 'NONE',  ( 3.920879176457659820, 1439.701872010520219, 184.6839060028229937 ) ) ;
#1639=CARTESIAN_POINT ( 'NONE',  ( 0.1494614725679999923, 1415.405923509830018, 233.4379070838980113 ) ) ;
#1640=CARTESIAN_POINT ( 'NONE',  ( -18.81494228913341971, 1424.684930363856893, 224.5303940569564531 ) ) ;
#1641=ADVANCED_FACE ( 'NONE', ( #64847 ), #92910, .F. ) ;
#1643=CARTESIAN_POINT ( 'NONE',  ( 18.22805055419890152, 1459.311389626190021, 227.8763770136359881 ) ) ;
#1644=VECTOR ( 'NONE', #9431, 999.9999999999998863 ) ;
#1647=EDGE_CURVE ( 'NONE', #19483, #69912, #41409, .T. ) ;
#1656=CARTESIAN_POINT ( 'NONE',  ( -19.46212512329999811, 1448.109899945180132, 224.8635561905979898 ) ) ;
#1657=CARTESIAN_POINT ( 'NONE',  ( -2.646139193785439936, 1458.417740263149881, 184.4338440838500333 ) ) ;
#1658=CARTESIAN_POINT ( 'NONE',  ( 11.14906425410000068, 1433.235768261610247, 151.6390481664980143 ) ) ;
#1659=CARTESIAN_POINT ( 'NONE',  ( 25.52872275119999657, 1450.634754197290022, 248.0989693098979956 ) ) ;
#1660=CARTESIAN_POINT ( 'NONE',  ( 26.67910011776079671, 1440.913060392740135, 225.3147551850250068 ) ) ;
#1663=CARTESIAN_POINT ( 'NONE',  ( 24.45953054869999832, 1435.631735371460081, 137.6709130696980026 ) ) ;
#1664=CARTESIAN_POINT ( 'NONE',  ( -9.684780809540001201, 1486.248617649129983, 183.3457608578980000 ) ) ;
#1666=CARTESIAN_POINT ( 'NONE',  ( -29.28791600580530030, 1509.974769825920021, 200.6261233647479969 ) ) ;
#1668=CARTESIAN_POINT ( 'NONE',  ( 24.09077679649999837, 1449.794656634499916, 215.4601383587679777 ) ) ;
#1670=CARTESIAN_POINT ( 'NONE',  ( 26.34431982013864015, 1436.712149879578192, 136.8400218608261127 ) ) ;
#1676=CARTESIAN_POINT ( 'NONE',  ( 0.1633892455278690148, 1484.235898642210259, 181.9124132699890026 ) ) ;
#1682=CARTESIAN_POINT ( 'NONE',  ( -35.74845714583440071, 1451.452973098360189, 134.0999999985519935 ) ) ;
#1683=ORIENTED_EDGE ( 'NONE', *, *, #98768, .F. ) ;
#1691=ADVANCED_FACE ( 'NONE', ( #49136 ), #52131, .T. ) ;
#1694=CARTESIAN_POINT ( 'NONE',  ( 14.50852758997319825, 1409.419709334970094, 205.5898239192270012 ) ) ;
#1697=CARTESIAN_POINT ( 'NONE',  ( -17.22534334500000242, 1417.728649700130063, 191.7604894772980231 ) ) ;
#1698=DIRECTION ( 'NONE',  ( 0.000000000000000000, -1.000000000000000000, 0.000000000000000000 ) ) ;
#1699=ORIENTED_EDGE ( 'NONE', *, *, #62887, .F. ) ;
#1702=CARTESIAN_POINT ( 'NONE',  ( -1.547462741870939906, 1414.913060391199906, 225.9340804956229931 ) ) ;
#1703=ORIENTED_EDGE ( 'NONE', *, *, #71721, .T. ) ;
#1705=CIRCLE ( 'NONE', #83677, 6.988489866870006395 ) ;
#1706=ORIENTED_EDGE ( 'NONE', *, *, #85099, .F. ) ;
#1707=CARTESIAN_POINT ( 'NONE',  ( 24.21955345239999957, 1509.534796804930011, 222.9919670691980116 ) ) ;
#1711=CARTESIAN_POINT ( 'NONE',  ( 25.36436853360955368, 1465.298048299637685, 269.4265643490046500 ) ) ;
#1713=CARTESIAN_POINT ( 'NONE',  ( 3.851850563460000210, 1397.715876698029888, 221.6434075889979738 ) ) ;
#1714=B_SPLINE_CURVE_WITH_KNOTS ( 'NONE', 3,
 ( #52850, #103786, #61271, #9715, #95386, #51175, #25391, #60141, #93698, #36040, #52300, #85873, #70228, #9175, #8054, #104333, #78025, #27626, #43340, #16976, #86425, #85305, #43881, #8602, #42775, #34373, #18651, #77488, #102646, #106534, #72403, #3008, #62364, #104888, #97589, #10837, #106001, #29823, #12476, #28179, #80790, #11392, #37681, #13004, #21396, #38221, #64010, #89182, #98121, #19769, #79153, #105444, #2462, #55606, #29277, #54517, #47190, #88652, #19196, #38768, #46658, #81315 ),
 .UNSPECIFIED., .F., .F.,
 ( 4, 2, 1, 1, 1, 1, 1, 2, 2, 2, 1, 1, 1, 1, 1, 2, 2, 2, 2, 1, 1, 1, 1, 1, 2, 2, 2, 2, 2, 1, 1, 1, 1, 1, 2, 2, 2, 2, 2, 2, 4 ),
 ( 0.000000000000000000, 0.06249999999613299606, 0.09374999999417588104, 0.1093749999931755840, 0.1171874999926754285, 0.1210937499924412686, 0.1230468749923069038, 0.1240234374922550842, 0.1249999999922032645, 0.1874999999915968607, 0.2187499999912936588, 0.2343749999911442228, 0.2421874999910673953, 0.2460937499910139659, 0.2480468749909872650, 0.2490234374909866266, 0.2499999999909859882, 0.3749999999922498661, 0.4374999999928675942, 0.4687499999931619699, 0.4843749999933071870, 0.4921874999933816830, 0.4960937499934078287, 0.4980468749934336969, 0.4990234374934356398, 0.4999999999934376937, 0.6249999999958949504, 0.6874999999971151965, 0.7187499999977342569, 0.7343749999980366816, 0.7421874999981893373, 0.7460937499982656096, 0.7480468749983038013, 0.7490234374983243404, 0.7495117187483266719, 0.7499999999983288923, 0.8124999999987432275, 0.8437499999989501731, 0.8593749999990548671, 0.8749999999991596722, 1.000000000000000000 ),
 .UNSPECIFIED. ) ;
#1715=CARTESIAN_POINT ( 'NONE',  ( 2.632641773180000477, 1417.642867858430009, 234.7516729256979886 ) ) ;
#1722=CARTESIAN_POINT ( 'NONE',  ( -12.94800087099079988, 1434.761335965779836, 149.4045837073300049 ) ) ;
#1723=B_SPLINE_CURVE_WITH_KNOTS ( 'NONE', 3,
 ( #35580, #37799, #61924, #53513, #18212, #79259, #10375, #88205, #2569, #97149, #11499, #78131, #52408, #9827, #20418, #36146, #88756, #44548, #19873, #45117, #3119, #105562, #54080, #104442, #95491, #94943, #45675, #79813, #18759, #87656, #43996, #86533, #12039, #27189, #80355, #37247, #71445, #28848, #46221, #3671, #103314, #2010, #26622, #1434, #60818, #69772 ),
 .UNSPECIFIED., .F., .F.,
 ( 4, 3, 3, 3, 3, 3, 3, 3, 3, 3, 3, 3, 3, 3, 3, 4 ),
 ( 10.13148339209999982, 11.92987739649050027, 12.20407613010000070, 14.42827119532750046, 16.14045415531399996, 17.68759836607059910, 19.09865219163459926, 19.90566978349999872, 21.14179169827090021, 22.42859032020150067, 23.78131544472190129, 25.30278979458900324, 26.99779043053199956, 29.30852037210000560, 29.67356826380000001, 30.47641535120000356 ),
 .UNSPECIFIED. ) ;
#1725=CARTESIAN_POINT ( 'NONE',  ( -10.81507089441019964, 1424.921187596680056, 144.1620444830689962 ) ) ;
#1726=CARTESIAN_POINT ( 'NONE',  ( 44.07821130980000390, 1452.218472917530107, 269.0164675534979892 ) ) ;
#1728=ORIENTED_EDGE ( 'NONE', *, *, #7058, .T. ) ;
#1732=CARTESIAN_POINT ( 'NONE',  ( -27.27473106140000070, 1488.690404415530111, 208.0215548677279855 ) ) ;
#1733=CARTESIAN_POINT ( 'NONE',  ( -10.90364899684709954, 1425.308507793300123, 127.8401879169430089 ) ) ;
#1734=CARTESIAN_POINT ( 'NONE',  ( 16.18670465684310145, 1409.478287066380062, 193.0621080980399995 ) ) ;
#1736=DIRECTION ( 'NONE',  ( -0.1402804634180439824, 0.9901118076173108795, 3.469446951951086598E-18 ) ) ;
#1738=CARTESIAN_POINT ( 'NONE',  ( 1.763299156880000132E-09, 1413.741945241729809, 248.5896189551980058 ) ) ;
#1740=CARTESIAN_POINT ( 'NONE',  ( 28.25247054925810275, 1508.179583159759886, 209.3874533882519984 ) ) ;
#1741=EDGE_CURVE ( 'NONE', #35056, #37407, #61947, .T. ) ;
#1743=FACE_OUTER_BOUND ( 'NONE', #8453, .T. ) ;
#1745=CARTESIAN_POINT ( 'NONE',  ( 5.519893427111519202, 1440.499866072189889, 154.7645221071819890 ) ) ;
#1748=CARTESIAN_POINT ( 'NONE',  ( -16.94875024379999928, 1459.649199545330021, 228.5285952991980025 ) ) ;
#1750=ORIENTED_EDGE ( 'NONE', *, *, #94245, .T. ) ;
#1755=CARTESIAN_POINT ( 'NONE',  ( -0.7091552652710000348, 1410.300368832030017, 185.1037611371980063 ) ) ;
#1756=CARTESIAN_POINT ( 'NONE',  ( 9.348425627764461510, 1446.614265060813068, 153.6205959845594577 ) ) ;
#1759=CARTESIAN_POINT ( 'NONE',  ( -0.5626263542969999198, 1461.199651506930195, 235.3168487328979950 ) ) ;
#1766=ORIENTED_EDGE ( 'NONE', *, *, #67993, .T. ) ;
#1767=CARTESIAN_POINT ( 'NONE',  ( 11.86158182214910006, 1432.020402734500067, 149.9731981294450236 ) ) ;
#1768=AXIS2_PLACEMENT_3D ( 'NONE', #65477, #83348, #91749 ) ;
#1769=CARTESIAN_POINT ( 'NONE',  ( 12.71821945952179256, 1445.010168364093943, 186.4037021029734547 ) ) ;
#1773=CARTESIAN_POINT ( 'NONE',  ( 2.890489020249999985, 1507.108937781629947, 235.9439513813980227 ) ) ;
#1775=B_SPLINE_CURVE_WITH_KNOTS ( 'NONE', 3,
 ( #104351, #46129, #43897, #86441, #95403, #9732, #19787, #71903, #27644, #29295, #79173, #18666, #2480, #45027, #95952, #88122, #53988, #96507, #61830, #61287, #28195, #78040, #53415, #1348 ),
 .UNSPECIFIED., .F., .F.,
 ( 4, 2, 2, 2, 2, 1, 2, 2, 2, 1, 2, 2, 4 ),
 ( 0.000000000000000000, 0.1249999999999030775, 0.1874999999999517608, 0.2500000000000004441, 0.3750000000002716716, 0.4375000000004031775, 0.4687500000004693468, 0.5000000000005355716, 0.6250000000005783152, 0.6875000000005520029, 0.7187500000005322409, 0.7500000000005124789, 1.000000000000000000 ),
 .UNSPECIFIED. ) ;
#1776=CARTESIAN_POINT ( 'NONE',  ( -5.752888337419999942, 1422.114707807429795, 186.4775914538980146 ) ) ;
#1777=CIRCLE ( 'NONE', #8847, 1.000002395377252107 ) ;
#1778=CARTESIAN_POINT ( 'NONE',  ( 2.236972126526609816, 1410.279550646489952, 269.6153997192959650 ) ) ;
#1779=CARTESIAN_POINT ( 'NONE',  ( -2.370970874524632510, 1427.002265528473799, 137.0999999980979851 ) ) ;
#1782=CARTESIAN_POINT ( 'NONE',  ( 0.03096724798627218528, 1410.169160866321590, 233.2107615507483445 ) ) ;
#1783=CARTESIAN_POINT ( 'NONE',  ( -17.87013932006249917, 1448.191556807570123, 190.6845719629749851 ) ) ;
#1785=CARTESIAN_POINT ( 'NONE',  ( 17.92235813230709951, 1421.133839370329952, 225.1061056996060188 ) ) ;
#1786=EDGE_CURVE ( 'NONE', #39621, #5728, #110104, .T. ) ;
#1787=CARTESIAN_POINT ( 'NONE',  ( -2.499950883797279921, 1420.112351832789955, 91.39149109222310585 ) ) ;
#1789=CARTESIAN_POINT ( 'NONE',  ( 4.290289617690000057, 1420.418457356630142, 243.9198229205979942 ) ) ;
#1791=CARTESIAN_POINT ( 'NONE',  ( 13.00933603280000028, 1434.785429338880022, 149.1498346358980029 ) ) ;
#1794=ADVANCED_FACE ( 'NONE', ( #6010 ), #43808, .F. ) ;
#1807=CARTESIAN_POINT ( 'NONE',  ( 15.39869794680000048, 1410.406122991029861, 227.2465235211980144 ) ) ;
#1809=CARTESIAN_POINT ( 'NONE',  ( -16.16510620389999886, 1460.221770685330057, 228.5003369000980058 ) ) ;
#1810=AXIS2_PLACEMENT_3D ( 'NONE', #25428, #9218, #51212 ) ;
#1812=CARTESIAN_POINT ( 'NONE',  ( 18.34911816089999803, 1408.676262367329855, 267.0969396382980108 ) ) ;
#1814=CARTESIAN_POINT ( 'NONE',  ( 24.21241066229999817, 1488.577768217629909, 198.4900566605979861 ) ) ;
#1815=CARTESIAN_POINT ( 'NONE',  ( -20.35145834579999757, 1427.842720165429682, 222.5291350759979991 ) ) ;
#1819=B_SPLINE_CURVE_WITH_KNOTS ( 'NONE', 3,
 ( #30359, #12465, #46648, #5161, #89719, #12996, #55596, #65087, #4088, #38212 ),
 .UNSPECIFIED., .F., .F.,
 ( 4, 2, 2, 2, 4 ),
 ( 0.000000000000000000, 0.2500000000000224265, 0.3750000000000168754, 0.5000000000000113243, 1.000000000000000000 ),
 .UNSPECIFIED. ) ;
#1820=FACE_OUTER_BOUND ( 'NONE', #94074, .T. ) ;
#1823=CARTESIAN_POINT ( 'NONE',  ( -13.11094645300000039, 1442.914509522559911, 187.2395568284980243 ) ) ;
#1825=CARTESIAN_POINT ( 'NONE',  ( -33.13365710820000487, 1436.983726026989871, 136.5854365510979846 ) ) ;
#1826=CARTESIAN_POINT ( 'NONE',  ( -0.3973340087122340103, 1418.672806152889962, 184.7148007238050127 ) ) ;
#1829=CARTESIAN_POINT ( 'NONE',  ( -14.78586735916750072, 1409.429394253109876, 211.1975209631870030 ) ) ;
#1830=B_SPLINE_SURFACE_WITH_KNOTS ( 'NONE', 4, 5, ( 
 ( #33681, #84640, #14686, #84092, #109319, #23639 ),
 ( #32602, #7936, #15755, #82458, #66779, #39897 ),
 ( #67875, #48874, #33136, #100878, #24171, #7393 ),
 ( #56707, #14127, #41558, #57281, #22505, #75713 ),
 ( #109859, #16315, #74066, #67324, #5755, #74616 ) ),
 .UNSPECIFIED., .F., .F., .F.,
 ( 5, 5 ),
 ( 6, 6 ),
 ( 4.528383477379999356, 21.94916619720000028 ),
 ( 0.000000000000000000, 1.000000000000000000 ),
 .UNSPECIFIED. ) ;
#1833=CARTESIAN_POINT ( 'NONE',  ( -30.03533176510000047, 1467.264374321729974, 268.9518348310980400 ) ) ;
#1835=CARTESIAN_POINT ( 'NONE',  ( 0.1985875301063339815, 1419.813287738610143, 184.1956569253020177 ) ) ;
#1836=LINE ( 'NONE', #44943, #68305 ) ;
#1839=CARTESIAN_POINT ( 'NONE',  ( 17.85778552263929697, 1424.389883610459719, 228.2680410153979835 ) ) ;
#1840=CARTESIAN_POINT ( 'NONE',  ( 13.50674874259999925, 1414.971287085330005, 218.9120235863680080 ) ) ;
#1841=DIRECTION ( 'NONE',  ( -0.9993902469249968945, -0.03489947640978578736, 0.001077449542479110099 ) ) ;
#1842=CARTESIAN_POINT ( 'NONE',  ( -27.08645728671159958, 1507.996806876479923, 211.2375099390570199 ) ) ;
#1844=CARTESIAN_POINT ( 'NONE',  ( -9.985313959770000025, 1508.918243844630069, 181.8527837295979737 ) ) ;
#1845=CARTESIAN_POINT ( 'NONE',  ( -22.70634968689999766, 1409.870434428829867, 205.6103426976079902 ) ) ;
#1846=CARTESIAN_POINT ( 'NONE',  ( 16.17135635129999827, 1414.913060387329779, 206.5448528754380106 ) ) ;
#1849=B_SPLINE_CURVE_WITH_KNOTS ( 'NONE', 3,
 ( #523, #1623, #2189, #26236, #59869, #52016, #79426, #60425, #104615, #18377, #10559, #35759, #52573, #70498, #53128, #27350, #69387, #86707, #27911, #10000, #9449, #18932, #62093, #87838, #43614, #93997, #77763, #17261, #51453, #85585, #61534, #34648, #95664, #68832, #1074, #102934, #94543, #35200, #103498, #71616, #79969, #90008, #28464, #55335, #21128, #54244, #106269, #56428 ),
 .UNSPECIFIED., .F., .F.,
 ( 4, 2, 2, 1, 1, 1, 1, 1, 2, 2, 2, 1, 1, 1, 2, 2, 2, 2, 2, 2, 2, 2, 2, 2, 2, 2, 2, 4 ),
 ( 0.000000000000000000, 0.2500000000005769274, 0.3750000000008642531, 0.4375000000010069168, 0.4687500000010855206, 0.4843750000011176615, 0.4921875000011337598, 0.4960937500011416978, 0.4980468750011447510, 0.5000000000011477486, 0.6250000000009476864, 0.6875000000008416601, 0.7187500000007887024, 0.7343750000007658318, 0.7421875000007500667, 0.7500000000007343015, 0.8125000000005889733, 0.8437500000005155876, 0.8593750000004759526, 0.8671875000004583001, 0.8710937500004467537, 0.8750000000004350964, 0.9062500000003413936, 0.9218750000002963185, 0.9296875000002715606, 0.9335937500002587930, 0.9375000000002459144, 1.000000000000000000 ),
 .UNSPECIFIED. ) ;
#1851=B_SPLINE_SURFACE_WITH_KNOTS ( 'NONE', 5, 5, ( 
 ( #43005, #53633, #53069, #87776, #1560, #77163 ),
 ( #68774, #35692, #70438, #52514, #102875, #26173 ),
 ( #87206, #69882, #60359, #94481, #2126, #17754 ),
 ( #51957, #1015, #35141, #60926, #95056, #18323 ),
 ( #9940, #36250, #27295, #103998, #29492, #72618 ),
 ( #72095, #2680, #79918, #64230, #12146, #38988 ),
 ( #79366, #105678, #3231, #63687, #55832, #80467 ),
 ( #54733, #88861, #90499, #106210, #46337, #73164 ),
 ( #13775, #37914, #97798, #105114, #55281, #97251 ),
 ( #89411, #107309, #98354, #54185, #28405, #96719 ),
 ( #3782, #28962, #62604, #71559, #19992, #30038 ),
 ( #37358, #21076, #63151, #70996, #38444, #106749 ) ),
 .UNSPECIFIED., .F., .F., .F.,
 ( 6, 3, 3, 6 ),
 ( 6, 6 ),
 ( 0.9635945383279999055, 4.198788347969999890, 5.913340936670000048, 6.825063656079999319 ),
 ( 0.000000000000000000, 2.000000000000000000 ),
 .UNSPECIFIED. ) ;
#1856=CARTESIAN_POINT ( 'NONE',  ( -21.92806448420000009, 1409.678805267029929, 210.7898312680979984 ) ) ;
#1866=CARTESIAN_POINT ( 'NONE',  ( -14.26747435372389994, 1485.844175363280101, 186.1892725996659976 ) ) ;
#1867=CARTESIAN_POINT ( 'NONE',  ( -18.24639174359999672, 1430.281446294329953, 193.9508323147979922 ) ) ;
#1873=ORIENTED_EDGE ( 'NONE', *, *, #366, .T. ) ;
#1874=CARTESIAN_POINT ( 'NONE',  ( 11.73806480614890013, 1433.731339164239898, 150.9439538071720222 ) ) ;
#1877=DIRECTION ( 'NONE',  ( 0.03489949655844001852, 0.9993908270241265157, 1.111776183576166572E-08 ) ) ;
#1880=CARTESIAN_POINT ( 'NONE',  ( 11.30500403589999792, 1428.976642997429963, 112.4493539157979995 ) ) ;
#1884=CARTESIAN_POINT ( 'NONE',  ( -24.39284326694200189, 1444.780737751010065, 211.1468293442990216 ) ) ;
#1887=CARTESIAN_POINT ( 'NONE',  ( 34.72084050058860072, 1435.748200648169814, 134.0999999979019890 ) ) ;
#1890=ORIENTED_EDGE ( 'NONE', *, *, #68688, .F. ) ;
#1891=CARTESIAN_POINT ( 'NONE',  ( 14.32178456671769951, 1435.822963899329807, 149.8685163660410069 ) ) ;
#1896=CARTESIAN_POINT ( 'NONE',  ( 12.78525141209750871, 1444.986522992021037, 169.4510567559931644 ) ) ;
#1897=CARTESIAN_POINT ( 'NONE',  ( -1.674556947779999971, 1464.910406147030017, 237.1062727332979989 ) ) ;
#1898=VECTOR ( 'NONE', #41052, 1000.000000000000000 ) ;
#1899=CARTESIAN_POINT ( 'NONE',  ( 25.25200551730000242, 1450.804230319249882, 137.6134878989979882 ) ) ;
#1902=CARTESIAN_POINT ( 'NONE',  ( 40.27308137180000358, 1443.612049545939954, 137.1163288300980128 ) ) ;
#1904=CARTESIAN_POINT ( 'NONE',  ( 4.272474999264660234, 1446.725045888410023, 157.6426782973369995 ) ) ;
#1906=CARTESIAN_POINT ( 'NONE',  ( 0.4073663215339999866, 1508.683555889429954, 238.1699978998979930 ) ) ;
#1910=CARTESIAN_POINT ( 'NONE',  ( 25.66502446409790039, 1440.913060387330006, 241.2077300345669926 ) ) ;
#1912=CARTESIAN_POINT ( 'NONE',  ( -13.70491113640000158, 1508.146349762730097, 184.2329986728979918 ) ) ;
#1916=CARTESIAN_POINT ( 'NONE',  ( -14.51125708719999885, 1410.352142336630095, 190.4994541838979956 ) ) ;
#1917=CARTESIAN_POINT ( 'NONE',  ( -24.35464616639999846, 1441.602688108240045, 211.7287004059179765 ) ) ;
#1918=CARTESIAN_POINT ( 'NONE',  ( -2.370970874524632510, 1427.002265528473799, 137.0999999980979851 ) ) ;
#1923=CARTESIAN_POINT ( 'NONE',  ( -25.77261374515159886, 1483.519019013160005, 212.0189592763409792 ) ) ;
#1928=CARTESIAN_POINT ( 'NONE',  ( 28.26084317239999777, 1508.649017702329957, 208.6067999643450150 ) ) ;
#1930=CARTESIAN_POINT ( 'NONE',  ( 14.54195235379999929, 1410.802016681730038, 191.4776931444980050 ) ) ;
#1931=ADVANCED_FACE ( 'NONE', ( #27226 ), #69810, .F. ) ;
#1935=CARTESIAN_POINT ( 'NONE',  ( -0.5943821362719999835, 1416.311719779230089, 227.7090535903980140 ) ) ;
#1936=CARTESIAN_POINT ( 'NONE',  ( 26.69977470740000314, 1442.651301016559955, 225.7788486252980249 ) ) ;
#1939=CARTESIAN_POINT ( 'NONE',  ( -5.309335150381779833, 1508.059062283110052, 236.4392518008919808 ) ) ;
#1941=CARTESIAN_POINT ( 'NONE',  ( 11.77874534290000064, 1433.007534236340007, 150.8097953682980119 ) ) ;
#1942=CARTESIAN_POINT ( 'NONE',  ( 19.24310214189999968, 1455.949671055829867, 226.1911111612980108 ) ) ;
#1945=VERTEX_POINT ( 'NONE', #102263 ) ;
#1947=CARTESIAN_POINT ( 'NONE',  ( 0.2161160260170000014, 1405.776202818429965, 268.4837592986979757 ) ) ;
#1949=CARTESIAN_POINT ( 'NONE',  ( 28.66995857139999870, 1509.914237401530045, 206.7534942493879839 ) ) ;
#1950=CARTESIAN_POINT ( 'NONE',  ( 30.57166591494479846, 1464.042419567909974, 270.1181552200280294 ) ) ;
#1951=CARTESIAN_POINT ( 'NONE',  ( 5.405732451549999595, 1434.707887834109897, 154.6595955769979867 ) ) ;
#1954=CARTESIAN_POINT ( 'NONE',  ( -36.06691658716020044, 1440.913060387480073, 252.9701890490810285 ) ) ;
#1955=CARTESIAN_POINT ( 'NONE',  ( 33.91369266730000476, 1450.440660192670066, 136.2454535554979884 ) ) ;
#1958=CARTESIAN_POINT ( 'NONE',  ( 2.500592263345220001, 1448.944489456090196, 154.5202628404780114 ) ) ;
#1964=CARTESIAN_POINT ( 'NONE',  ( -12.85916294159999929, 1411.892799971530167, 268.3665355202980436 ) ) ;
#1968=CARTESIAN_POINT ( 'NONE',  ( -1.331593054780000118, 1475.969838803829816, 267.2342691169980640 ) ) ;
#1969=CARTESIAN_POINT ( 'NONE',  ( -33.91369114349999592, 1451.728768196330066, 134.7155300131979914 ) ) ;
#1970=CARTESIAN_POINT ( 'NONE',  ( -27.79064038249999768, 1508.605033447930055, 210.4916515659980121 ) ) ;
#1973=CARTESIAN_POINT ( 'NONE',  ( -18.41105348850000212, 1415.553739807329976, 208.0605876747880245 ) ) ;
#1977=CARTESIAN_POINT ( 'NONE',  ( 26.66179749201589644, 1435.630288477099839, 136.0743949063709977 ) ) ;
#1978=CARTESIAN_POINT ( 'NONE',  ( -5.343479917770609156, 1396.099658817820000, 199.4684377796870081 ) ) ;
#1981=CARTESIAN_POINT ( 'NONE',  ( -17.21443206581249896, 1410.737832039549858, 226.0138299294659987 ) ) ;
#1982=CARTESIAN_POINT ( 'NONE',  ( 7.450897614389999646, 1442.756953654919926, 149.7755488681980012 ) ) ;
#1986=FACE_OUTER_BOUND ( 'NONE', #45042, .T. ) ;
#1987=CARTESIAN_POINT ( 'NONE',  ( 9.946025746629999276, 1425.248710433229917, 91.15452341569790917 ) ) ;
#1990=CARTESIAN_POINT ( 'NONE',  ( 4.237000157206120221, 1423.967056607189988, 184.0491610448669917 ) ) ;
#1994=CARTESIAN_POINT ( 'NONE',  ( -23.79000955475941836, 1411.113042535969726, 210.2403600569826096 ) ) ;
#1996=CARTESIAN_POINT ( 'NONE',  ( 3.264324498270000152, 1450.280157591569832, 183.9712559857979954 ) ) ;
#2001=PLANE ( 'NONE',  #78383 ) ;
#2002=CARTESIAN_POINT ( 'NONE',  ( -0.3541148012579999893, 1466.691116367230052, 235.5895199573979824 ) ) ;
#2003=CARTESIAN_POINT ( 'NONE',  ( -0.4843842464630000455, 1473.264972808229913, 270.4290818601980391 ) ) ;
#2005=( BOUNDED_CURVE ( )  B_SPLINE_CURVE ( 3, ( #34455, #41747, #68630, #75906 ),
 .UNSPECIFIED., .F., .F. ) 
 B_SPLINE_CURVE_WITH_KNOTS ( ( 4, 4 ),
 ( 4.612172254335380472, 4.862528044142459649 ),
 .UNSPECIFIED. ) 
 CURVE ( )  GEOMETRIC_REPRESENTATION_ITEM ( )  RATIONAL_B_SPLINE_CURVE ( ( 1.000000000000000000, 0.9947836483532912499, 0.9947836483532912499, 1.000000000000000000 ) ) 
 REPRESENTATION_ITEM ( '' )  );
#2009=CARTESIAN_POINT ( 'NONE',  ( 12.48640425065659976, 1423.660394517820123, 223.7918487953089937 ) ) ;
#2010=CARTESIAN_POINT ( 'NONE',  ( -2.500000000000000000, 1448.204021880610071, 169.8582428316960033 ) ) ;
#2011=CARTESIAN_POINT ( 'NONE',  ( 9.222591024579390506, 1396.235120365410012, 215.2291610791590131 ) ) ;
#2012=CARTESIAN_POINT ( 'NONE',  ( 3.205045813472149785, 1408.488127767880087, 195.5730862361089919 ) ) ;
#2013=DIRECTION ( 'NONE',  ( 0.2020439943617916845, -0.9583089389155642346, 0.2020450492757928096 ) ) ;
#2014=CARTESIAN_POINT ( 'NONE',  ( -10.93238010534558313, 1414.913060581097170, 195.9940915879461159 ) ) ;
#2015=ORIENTED_EDGE ( 'NONE', *, *, #26089, .F. ) ;
#2016=CARTESIAN_POINT ( 'NONE',  ( 3.827327205999999649, 1424.046157813729906, 183.3886489380980152 ) ) ;
#2017=CARTESIAN_POINT ( 'NONE',  ( 12.85143379750000037, 1446.481137621939979, 188.4927750485979914 ) ) ;
#2020=B_SPLINE_CURVE_WITH_KNOTS ( 'NONE', 3,
 ( #107977, #22849, #101210, #92280, #83329, #22292, #15549, #55945, #31274, #13903, #6625, #48090, #32384, #65458, #40779, #99565, #74955, #66567, #49749, #90066, #13348, #47541, #41882, #78240, #7722, #85518, #459, #33457, #93923, #92829, #103424, #8264, #16104, #86637, #9932, #77696, #68220, #84970, #44102, #50839, #34581, #50308, #8814, #102325, #84438, #24506, #25611, #102869, #59803, #76587, #60920, #1553, #35134, #17190, #51386, #42997, #77155, #1007, #68766, #26166, #60352, #93376, #52508, #76041, #42428, #34029, #110186, #58697, #67659, #110738, #35685, #94475, #17748, #86092, #51950, #69876, #9386, #25056, #95049 ),
 .UNSPECIFIED., .F., .F.,
 ( 4, 3, 3, 3, 3, 3, 3, 3, 3, 3, 3, 3, 3, 3, 3, 3, 3, 3, 3, 3, 3, 3, 3, 3, 3, 3, 4 ),
 ( 0.000000000000000000, 0.4548555274129320036, 0.9190079891053550831, 1.398119237412919880, 1.886365508051579987, 2.387648495461230258, 2.516896244989999865, 3.033433463757130077, 3.554872652308640024, 4.076782264074299889, 4.594593341653459895, 5.099843107827240374, 5.596159927621140007, 6.077963950408490135, 6.410372910170000438, 7.036818067524451159, 7.682305271035700933, 8.346433156759069050, 9.030012755689879711, 9.715260639136369392, 10.38844028647699780, 10.64487668199999959, 11.49777674247360082, 12.38410586200980035, 13.29134611626929896, 14.23087319025490061, 14.62789107123472121 ),
 .UNSPECIFIED. ) ;
#2028=B_SPLINE_CURVE_WITH_KNOTS ( 'NONE', 3,
 ( #5077, #83430, #49305, #5644, #14573, #57169 ),
 .UNSPECIFIED., .F., .F.,
 ( 4, 2, 4 ),
 ( -0.2778631976372760159, -0.1390217908135579772, -1.347131930007350320E-06 ),
 .UNSPECIFIED. ) ;
#2030=CARTESIAN_POINT ( 'NONE',  ( 10.07457632729999908, 1416.825421876529845, 224.7882279959979996 ) ) ;
#2033=CARTESIAN_POINT ( 'NONE',  ( -5425.877332847427169, 54.28084076250834755, 8448.741457306947268 ) ) ;
#2037=CARTESIAN_POINT ( 'NONE',  ( -5.943866765360000137, 1409.623546987629879, 231.2954894698980013 ) ) ;
#2038=CARTESIAN_POINT ( 'NONE',  ( -8.896201126819999416, 1446.954173154499813, 186.2107498446980003 ) ) ;
#2040=CARTESIAN_POINT ( 'NONE',  ( -14.56153818869126049, 1435.986600758549912, 149.8060885009444974 ) ) ;
#2041=CARTESIAN_POINT ( 'NONE',  ( 1.734605482336269988, 1474.701058242480030, 235.0720777047329761 ) ) ;
#2042=CARTESIAN_POINT ( 'NONE',  ( 20.73258896465929979, 1507.783937758249749, 226.5135743084329931 ) ) ;
#2043=DIRECTION ( 'NONE',  ( -0.9211327884476211425, -0.3892484888175031799, 0.000000000000000000 ) ) ;
#2044=CARTESIAN_POINT ( 'NONE',  ( -25.23204818860000032, 1435.454757579879924, 136.2099880446980080 ) ) ;
#2048=CARTESIAN_POINT ( 'NONE',  ( -3.659368786598335088, 1424.416642863884363, 227.7607030046739283 ) ) ;
#2053=CARTESIAN_POINT ( 'NONE',  ( 2.500000000000000000, 1432.393161327160215, 157.4962941367979852 ) ) ;
#2054=CARTESIAN_POINT ( 'NONE',  ( -0.4885209890020000834, 1412.847411980229936, 233.2840911246979942 ) ) ;
#2058=VECTOR ( 'NONE', #84789, 1000.000000000000000 ) ;
#2060=CARTESIAN_POINT ( 'NONE',  ( 11.99823785417749988, 1434.648096261249975, 150.9684152172500262 ) ) ;
#2061=CARTESIAN_POINT ( 'NONE',  ( 10.31468017153819972, 1478.700932630890065, 232.9778818359829984 ) ) ;
#2063=CARTESIAN_POINT ( 'NONE',  ( -24.30765313494389801, 1509.765688098410010, 225.8104982504189877 ) ) ;
#2064=CARTESIAN_POINT ( 'NONE',  ( -2.445261619629999661, 1408.998450803630021, 187.5560518005979986 ) ) ;
#2065=DIRECTION ( 'NONE',  ( 0.7067700363771036720, 0.03085824620770448445, -0.7067700363771035610 ) ) ;
#2066=CARTESIAN_POINT ( 'NONE',  ( 0.06322423967616179474, 1420.447901757230056, 182.6808383609890143 ) ) ;
#2068=CARTESIAN_POINT ( 'NONE',  ( -3.075414810399999865, 1420.210582609129915, 186.1942670208979962 ) ) ;
#2069=CARTESIAN_POINT ( 'NONE',  ( 18.84890159040000057, 1508.241238762730291, 188.4656274554980087 ) ) ;
#2070=CARTESIAN_POINT ( 'NONE',  ( 18.24053064527407741, 1425.259887461422977, 223.9475156348823646 ) ) ;
#2071=VERTEX_POINT ( 'NONE', #86573 ) ;
#2072=CARTESIAN_POINT ( 'NONE',  ( -12.66409680412509964, 1415.935475482089942, 196.4689021216840104 ) ) ;
#2074=ORIENTED_EDGE ( 'NONE', *, *, #106146, .T. ) ;
#2077=CARTESIAN_POINT ( 'NONE',  ( 10.02841049835654275, 1435.644464287910068, 152.4726594247936191 ) ) ;
#2083=CARTESIAN_POINT ( 'NONE',  ( -2.500000000000000000, 1448.685390522050056, 157.9322779416980040 ) ) ;
#2085=CARTESIAN_POINT ( 'NONE',  ( -14.75023390800000023, 1435.013611184930141, 147.9283531795979911 ) ) ;
#2087=CARTESIAN_POINT ( 'NONE',  ( 17.61169129089999785, 1418.990866690829989, 192.1965113226980293 ) ) ;
#2088=CARTESIAN_POINT ( 'NONE',  ( 1.138216366218499864, 1409.887084221469877, 232.8382466657240002 ) ) ;
#2091=ORIENTED_EDGE ( 'NONE', *, *, #110275, .F. ) ;
#2092=CARTESIAN_POINT ( 'NONE',  ( 1.468632314148109907, 1507.614846007670167, 186.1949685577550042 ) ) ;
#2093=CARTESIAN_POINT ( 'NONE',  ( -5399.190729149936487, 50.28429875023819307, -8134.791976861672083 ) ) ;
#2094=CARTESIAN_POINT ( 'NONE',  ( -24.68077715769999969, 1437.736179642080060, 210.5119845752080039 ) ) ;
#2097=CARTESIAN_POINT ( 'NONE',  ( -3.503594166644271368, 1426.007756115946222, 185.8779573887631216 ) ) ;
#2099=CARTESIAN_POINT ( 'NONE',  ( 2.496055909974519427, 1410.375802592201580, 231.6937116688994820 ) ) ;
#2100=CARTESIAN_POINT ( 'NONE',  ( -3.827327205999999649, 1418.913060387330006, 172.2701767054979882 ) ) ;
#2110=VERTEX_POINT ( 'NONE', #30527 ) ;
#2111=CARTESIAN_POINT ( 'NONE',  ( -18.72407526530000155, 1458.246115540929850, 227.3156487912980026 ) ) ;
#2113=CARTESIAN_POINT ( 'NONE',  ( 20.55900035540929949, 1509.660753117409968, 230.5261133655430115 ) ) ;
#2114=VERTEX_POINT ( 'NONE', #98835 ) ;
#2117=CARTESIAN_POINT ( 'NONE',  ( -10.96946876072200006, 1432.347663854339999, 151.7701362700559855 ) ) ;
#2118=CARTESIAN_POINT ( 'NONE',  ( 13.41954733660536370, 1443.449734802816920, 169.3662105687162978 ) ) ;
#2120=CARTESIAN_POINT ( 'NONE',  ( -41.23304476799999918, 1446.065281864440067, 261.5842295713979979 ) ) ;
#2123=B_SPLINE_CURVE_WITH_KNOTS ( 'NONE', 3,
 ( #81265, #28680, #62313, #72353, #98073, #87493, #29768, #54460, #72890, #4581, #38715, #19714, #88598, #29229 ),
 .UNSPECIFIED., .F., .F.,
 ( 4, 2, 2, 2, 2, 2, 4 ),
 ( 0.000000000000000000, 0.001128757102284214499, 0.002257514204568428998, 0.002821892755710748643, 0.003386271306853069155, 0.003950649857995389667, 0.004515028409137709746 ),
 .UNSPECIFIED. ) ;
#2124=CIRCLE ( 'NONE', #91458, 1.999999999999942935 ) ;
#2125=CARTESIAN_POINT ( 'NONE',  ( 25.23662664879999795, 1509.794342810929948, 195.3591958783979976 ) ) ;
#2126=CARTESIAN_POINT ( 'NONE',  ( -19.90114970400000161, 1485.011347091429798, 190.9790800808980009 ) ) ;
#2128=CARTESIAN_POINT ( 'NONE',  ( 5.557914828519999517, 1420.826195899929871, 186.0956685246979987 ) ) ;
#2129=CARTESIAN_POINT ( 'NONE',  ( -9.548319411750000540, 1438.548742442639877, 152.9855554426980007 ) ) ;
#2132=CARTESIAN_POINT ( 'NONE',  ( -19.71294296389999801, 1452.081684968429954, 145.2800229328979924 ) ) ;
#2137=CARTESIAN_POINT ( 'NONE',  ( -44.56544972020000728, 1444.219545419719907, 269.9128112642979431 ) ) ;
#2139=CARTESIAN_POINT ( 'NONE',  ( -23.75705825515298031, 1436.072652686797028, 211.7065605907733357 ) ) ;
#2140=CARTESIAN_POINT ( 'NONE',  ( 17.54329103400000278, 1410.021606951229842, 223.3339101244980043 ) ) ;
#2141=CARTESIAN_POINT ( 'NONE',  ( -14.05027195639999960, 1463.289392627530106, 223.4969360966980219 ) ) ;
#2144=CARTESIAN_POINT ( 'NONE',  ( 2.852115976134160125, 1409.175191729200151, 230.8570650992599838 ) ) ;
#2145=CARTESIAN_POINT ( 'NONE',  ( 2.173985094599999890, 1508.988976439630051, 238.5378654763979966 ) ) ;
#2146=CARTESIAN_POINT ( 'NONE',  ( -7.617228954449999812, 1417.322863989330017, 231.1379649406979979 ) ) ;
#2147=EDGE_CURVE ( 'NONE', #10764, #80757, #107327, .T. ) ;
#2149=CARTESIAN_POINT ( 'NONE',  ( -1.435153818974767237, 1484.396021952602950, 182.4491198709524724 ) ) ;
#2151=CARTESIAN_POINT ( 'NONE',  ( -45.64771259127410019, 1435.560685441120086, 266.9890804707069378 ) ) ;
#2154=CARTESIAN_POINT ( 'NONE',  ( 24.40199393649999848, 1435.349635217629839, 136.1409814179979776 ) ) ;
#2158=CARTESIAN_POINT ( 'NONE',  ( -4.026786250540000722, 1422.913060387330006, 172.2701767054979882 ) ) ;
#2159=CARTESIAN_POINT ( 'NONE',  ( -21.92443624460000251, 1509.678678571630144, 190.3581774935979922 ) ) ;
#2160=FACE_OUTER_BOUND ( 'NONE', #37349, .T. ) ;
#2164=CARTESIAN_POINT ( 'NONE',  ( -17.38127759599958466, 1410.742336404525759, 225.7780505793990926 ) ) ;
#2165=CARTESIAN_POINT ( 'NONE',  ( 0.5697990016583959205, 1450.893162567740092, 181.2939912002310052 ) ) ;
#2173=CARTESIAN_POINT ( 'NONE',  ( -12.95209671980339827, 1411.808719174920043, 269.3556024724110216 ) ) ;
#2179=ORIENTED_EDGE ( 'NONE', *, *, #106940, .T. ) ;
#2180=CARTESIAN_POINT ( 'NONE',  ( -23.51878303699330175, 1410.727184521670097, 210.4338679270009891 ) ) ;
#2181=CARTESIAN_POINT ( 'NONE',  ( -4.526843557140001195, 1425.874817585629899, 186.1888505123980053 ) ) ;
#2183=CARTESIAN_POINT ( 'NONE',  ( -3.818068226668779541, 1406.099103250517146, 266.9557811492330757 ) ) ;
#2185=CARTESIAN_POINT ( 'NONE',  ( -20.42021094099999701, 1430.789239710730044, 222.0598896059980234 ) ) ;
#2187=CARTESIAN_POINT ( 'NONE',  ( 5.341374517573029834, 1476.050173402869859, 268.4837847659439944 ) ) ;
#2188=B_SPLINE_CURVE_WITH_KNOTS ( 'NONE', 5,
 ( #32849, #39617, #23350, #75442, #7114, #75969 ),
 .UNSPECIFIED., .F., .F.,
 ( 6, 6 ),
 ( 0.000000000000000000, 1.000000000000000000 ),
 .UNSPECIFIED. ) ;
#2189=CARTESIAN_POINT ( 'NONE',  ( -13.34651281871636286, 1462.782296786469715, 230.3199898465639990 ) ) ;
#2190=CARTESIAN_POINT ( 'NONE',  ( 10.26047870550000063, 1446.726006776589884, 186.8445627053979763 ) ) ;
#2193=CARTESIAN_POINT ( 'NONE',  ( 24.08426297012860218, 1411.115209414830133, 209.6325633951909708 ) ) ;
#2194=CARTESIAN_POINT ( 'NONE',  ( 1.475845351969280017, 1481.308154728749969, 182.2386903793839963 ) ) ;
#2197=CARTESIAN_POINT ( 'NONE',  ( 25.37084254212440371, 1451.310454143999777, 137.0122259544509973 ) ) ;
#2198=CARTESIAN_POINT ( 'NONE',  ( 13.79555462530000121, 1416.822690122329959, 196.3351664771980154 ) ) ;
#2200=CARTESIAN_POINT ( 'NONE',  ( -18.65749898563134579, 1509.387464492826666, 230.8014192534890014 ) ) ;
#2201=CARTESIAN_POINT ( 'NONE',  ( 19.05936272150000121, 1410.940464818530018, 195.3780893796979967 ) ) ;
#2203=CARTESIAN_POINT ( 'NONE',  ( 2.903677228125761900, 1439.669927704568863, 183.9752002117523091 ) ) ;
#2204=CARTESIAN_POINT ( 'NONE',  ( 0.7916551353930000312, 1417.386977067530097, 235.1101550285980011 ) ) ;
#2205=CARTESIAN_POINT ( 'NONE',  ( -18.63621073208100398, 1424.448676634511685, 224.8155311996966930 ) ) ;
#2206=CARTESIAN_POINT ( 'NONE',  ( 0.8296033197978609497, 1451.436690953809830, 182.8542985698300072 ) ) ;
#2217=CARTESIAN_POINT ( 'NONE',  ( -34.75239981097760023, 1450.355854787910175, 136.2303794071760024 ) ) ;
#2220=CARTESIAN_POINT ( 'NONE',  ( -13.21926163380000041, 1460.466222979229997, 248.0989693022980020 ) ) ;
#2222=CARTESIAN_POINT ( 'NONE',  ( 44.66359154829995504, 1448.409698723047768, 266.2173270182975671 ) ) ;
#2223=CARTESIAN_POINT ( 'NONE',  ( 10.98204826459999950, 1433.094938567290001, 151.7693906807980113 ) ) ;
#2224=CARTESIAN_POINT ( 'NONE',  ( -32.54472331756920767, 1464.064700655210117, 269.9033746748029898 ) ) ;
#2227=ORIENTED_EDGE ( 'NONE', *, *, #30453, .T. ) ;
#2229=CARTESIAN_POINT ( 'NONE',  ( 25.00977876991279913, 1436.598012848749931, 137.9330263815630246 ) ) ;
#2230=CARTESIAN_POINT ( 'NONE',  ( -12.27295469420000096, 1486.509335314930013, 184.4397015064979826 ) ) ;
#2233=EDGE_CURVE ( 'NONE', #93915, #86873, #79381, .T. ) ;
#2235=CARTESIAN_POINT ( 'NONE',  ( 24.75581127549999749, 1430.360917243230006, 210.2728189765479954 ) ) ;
#2242=B_SPLINE_CURVE_WITH_KNOTS ( 'NONE', 3,
 ( #64901, #20109, #29611, #46449 ),
 .UNSPECIFIED., .F., .F.,
 ( 4, 4 ),
 ( 0.000000000000000000, 1.000000000000000000 ),
 .UNSPECIFIED. ) ;
#2244=CARTESIAN_POINT ( 'NONE',  ( 0.1678350090582330090, 1481.603268379459905, 182.0255188484140092 ) ) ;
#2245=EDGE_CURVE ( 'NONE', #101350, #84627, #84705, .T. ) ;
#2247=EDGE_LOOP ( 'NONE', ( #62076, #91279, #55048, #2892, #99074, #45713, #80231, #44012, #64267 ) ) ;
#2250=CARTESIAN_POINT ( 'NONE',  ( -5.375553179505209833, 1441.026369770150040, 154.8319413312549955 ) ) ;
#2252=ORIENTED_EDGE ( 'NONE', *, *, #54613, .T. ) ;
#2256=CARTESIAN_POINT ( 'NONE',  ( -17.84204423069999734, 1415.932840167130053, 209.4661914366780024 ) ) ;
#2257=CARTESIAN_POINT ( 'NONE',  ( -5.524058921557154278, 1509.111545497368979, 238.0554591568478031 ) ) ;
#2262=CARTESIAN_POINT ( 'NONE',  ( 13.71176819436150041, 1409.391885883779878, 203.1931630247410112 ) ) ;
#2265=CARTESIAN_POINT ( 'NONE',  ( -17.91583404220000020, 1424.173795738829995, 192.2475373850980134 ) ) ;
#2271=VERTEX_POINT ( 'NONE', #94565 ) ;
#2273=CARTESIAN_POINT ( 'NONE',  ( 25.84050225520000055, 1509.815430613229864, 221.3404165686980036 ) ) ;
#2275=CARTESIAN_POINT ( 'NONE',  ( -12.00426221419999884, 1433.697247254759986, 150.2718049272980068 ) ) ;
#2276=CARTESIAN_POINT ( 'NONE',  ( 29.51415436607676313, 1509.963328502264176, 211.7137289823847652 ) ) ;
#2278=CARTESIAN_POINT ( 'NONE',  ( 2.349396271509999856, 1396.056274664130115, 220.6130876232980143 ) ) ;
#2280=CARTESIAN_POINT ( 'NONE',  ( 19.52793876076239954, 1443.814291013210095, 209.3879297421120214 ) ) ;
#2281=FACE_OUTER_BOUND ( 'NONE', #55547, .T. ) ;
#2283=CARTESIAN_POINT ( 'NONE',  ( -26.66311519709438116, 1436.746818294333934, 136.7889187690164761 ) ) ;
#2284=EDGE_CURVE ( 'NONE', #99393, #77212, #39309, .T. ) ;
#2286=CARTESIAN_POINT ( 'NONE',  ( -13.13860279428170053, 1434.935977728519902, 149.7031307944440073 ) ) ;
#2287=CARTESIAN_POINT ( 'NONE',  ( 9.061759573819999858, 1423.804867913830094, 133.5337813787979826 ) ) ;
#2292=EDGE_LOOP ( 'NONE', ( #38318, #90683, #29383, #41414 ) ) ;
#2294=CARTESIAN_POINT ( 'NONE',  ( -26.12765557870000066, 1469.244184481629873, 206.5858184781079956 ) ) ;
#2295=CARTESIAN_POINT ( 'NONE',  ( -10.68704931835589989, 1425.705646839379824, 93.54238571512179590 ) ) ;
#2296=CARTESIAN_POINT ( 'NONE',  ( 16.24908062485310012, 1409.480479830250033, 193.1391318611629799 ) ) ;
#2298=CARTESIAN_POINT ( 'NONE',  ( 0.4003602064798469917, 1395.927041273810119, 198.1267992979170174 ) ) ;
#2300=CARTESIAN_POINT ( 'NONE',  ( -28.33103133930000084, 1431.247806717810136, 240.1819618842980049 ) ) ;
#2302=CARTESIAN_POINT ( 'NONE',  ( 29.03159036030189810, 1509.651961614089942, 209.5599309260780103 ) ) ;
#2304=CARTESIAN_POINT ( 'NONE',  ( -24.02849098739518041, 1410.733038014311205, 208.6273191338911772 ) ) ;
#2308=CARTESIAN_POINT ( 'NONE',  ( -16.12485330519999849, 1459.081998215830026, 229.9878740626980118 ) ) ;
#2309=ORIENTED_EDGE ( 'NONE', *, *, #87057, .F. ) ;
#2312=CARTESIAN_POINT ( 'NONE',  ( -9.330551624163069491, 1426.784211110280012, 151.9956449679999935 ) ) ;
#2313=VERTEX_POINT ( 'NONE', #78901 ) ;
#2314=CARTESIAN_POINT ( 'NONE',  ( 0.1022255644269999819, 1415.641329274630152, 184.7537210817980338 ) ) ;
#2315=CARTESIAN_POINT ( 'NONE',  ( 9.883113931189466683, 1446.592767805756466, 153.4333270483208196 ) ) ;
#2316=CARTESIAN_POINT ( 'NONE',  ( 17.22592475670000312, 1443.913060387330006, 162.9227486557980171 ) ) ;
#2317=FACE_OUTER_BOUND ( 'NONE', #41238, .T. ) ;
#2319=CARTESIAN_POINT ( 'NONE',  ( 1.211738532285810077, 1420.845824148819929, 182.9724934397759739 ) ) ;
#2322=CARTESIAN_POINT ( 'NONE',  ( 0.04809667444139999887, 1420.202366602630036, 183.9005171462980002 ) ) ;
#2323=EDGE_LOOP ( 'NONE', ( #105995, #70389, #91707, #39981 ) ) ;
#2327=CARTESIAN_POINT ( 'NONE',  ( 11.86603321975120018, 1432.331321816350055, 149.9824224880240138 ) ) ;
#2328=CARTESIAN_POINT ( 'NONE',  ( 13.30719000516407391, 1444.579980391261415, 187.5321241343243059 ) ) ;
#2331=CARTESIAN_POINT ( 'NONE',  ( -13.31970894439942832, 1443.086052842850449, 169.4013815678669346 ) ) ;
#2332=CARTESIAN_POINT ( 'NONE',  ( 5.138925822920000108, 1509.092515631430160, 237.3859384438979987 ) ) ;
#2334=CARTESIAN_POINT ( 'NONE',  ( -5.656371325420000318, 1421.415623769629747, 186.5737237497980061 ) ) ;
#2335=CARTESIAN_POINT ( 'NONE',  ( 4.903601556030229958, 1409.407506479329868, 270.3706464830609661 ) ) ;
#2342=CARTESIAN_POINT ( 'NONE',  ( -2.500000000000000000, 1426.966631815929986, 170.4008037693979816 ) ) ;
#2345=CARTESIAN_POINT ( 'NONE',  ( 17.88485182696830122, 1419.918979540250120, 225.0707500705920268 ) ) ;
#2347=ORIENTED_EDGE ( 'NONE', *, *, #88292, .T. ) ;
#2348=CARTESIAN_POINT ( 'NONE',  ( 22.74199304079999706, 1435.511682894840078, 234.3916895645979821 ) ) ;
#2349=CARTESIAN_POINT ( 'NONE',  ( 13.67952642077979952, 1434.971887304759775, 148.6457544281230128 ) ) ;
#2353=CARTESIAN_POINT ( 'NONE',  ( 39.86227344171260256, 1422.528661024590292, 269.1410521188619782 ) ) ;
#2358=CARTESIAN_POINT ( 'NONE',  ( -24.15641795129999991, 1444.538778010680062, 211.4627077540479831 ) ) ;
#2360=CARTESIAN_POINT ( 'NONE',  ( -2.332679820760331424, 1449.698752274461867, 154.4191734171435257 ) ) ;
#2364=CARTESIAN_POINT ( 'NONE',  ( 21.50779739108499911, 1509.664126782800167, 229.6171678230790008 ) ) ;
#2367=CARTESIAN_POINT ( 'NONE',  ( -13.31005321830910049, 1421.758539284290009, 222.0611081425300029 ) ) ;
#2368=CARTESIAN_POINT ( 'NONE',  ( 16.67088892840000014, 1415.091340903430137, 226.7043766012980370 ) ) ;
#2370=LINE ( 'NONE', #21301, #78244 ) ;
#2372=CARTESIAN_POINT ( 'NONE',  ( 35.49642997870000016, 1419.115857373830067, 269.2425788070980275 ) ) ;
#2374=CARTESIAN_POINT ( 'NONE',  ( 18.54481337859999712, 1435.291263500080049, 145.9381164648980018 ) ) ;
#2375=CARTESIAN_POINT ( 'NONE',  ( 21.33248983229999851, 1469.154932495629964, 194.2950544196980047 ) ) ;
#2376=CARTESIAN_POINT ( 'NONE',  ( -23.20318700179999993, 1433.765057477279925, 215.6666483125179923 ) ) ;
#2380=CARTESIAN_POINT ( 'NONE',  ( 20.85715831679999965, 1508.960610662329827, 227.8108772789979923 ) ) ;
#2381=CARTESIAN_POINT ( 'NONE',  ( -17.79016152762200065, 1578.884136531910144, 256.3461289262040168 ) ) ;
#2383=CARTESIAN_POINT ( 'NONE',  ( -13.40137408230000027, 1443.240311850900071, 187.4864273396979968 ) ) ;
#2386=CARTESIAN_POINT ( 'NONE',  ( -31.78593504660000235, 1435.767691617939818, 136.0101313228979905 ) ) ;
#2389=EDGE_CURVE ( 'NONE', #104546, #62931, #33940, .T. ) ;
#2391=CARTESIAN_POINT ( 'NONE',  ( -13.26148688360019889, 1409.376161713930060, 215.9976612687219983 ) ) ;
#2393=ADVANCED_FACE ( 'NONE', ( #13301 ), #4921, .F. ) ;
#2395=CARTESIAN_POINT ( 'NONE',  ( -30.02861084270000092, 1467.289302230230078, 266.6068817451980522 ) ) ;
#2397=CARTESIAN_POINT ( 'NONE',  ( 0.2074656164648590040, 1420.466249280530064, 183.0472788335430039 ) ) ;
#2398=CARTESIAN_POINT ( 'NONE',  ( 3.835404308833624043, 1396.046995657106436, 216.1425064568209677 ) ) ;
#2401=CARTESIAN_POINT ( 'NONE',  ( 17.72398368343529995, 1424.436447516579847, 227.0786475391319925 ) ) ;
#2402=CARTESIAN_POINT ( 'NONE',  ( 20.59563400740000105, 1507.764823632930074, 227.7386540762980189 ) ) ;
#2403=CARTESIAN_POINT ( 'NONE',  ( 14.22148428500000072, 1463.290759296229908, 223.5797348918979992 ) ) ;
#2409=CARTESIAN_POINT ( 'NONE',  ( 16.02395358489999921, 1414.971262582530017, 204.1331252983779905 ) ) ;
#2410=CARTESIAN_POINT ( 'NONE',  ( -12.72965162820000096, 1416.819756528429934, 195.1130951807980125 ) ) ;
#2412=CARTESIAN_POINT ( 'NONE',  ( 23.64646709530000024, 1410.660431756829894, 211.3066953406180346 ) ) ;
#2413=CARTESIAN_POINT ( 'NONE',  ( -12.58535514000000077, 1434.516889947230084, 149.4256401672980132 ) ) ;
#2415=CARTESIAN_POINT ( 'NONE',  ( -15.80894762269999987, 1421.035220212730110, 227.0411592943979997 ) ) ;
#2416=CARTESIAN_POINT ( 'NONE',  ( -10.97117066409999886, 1432.448735918919965, 151.7701026906980246 ) ) ;
#2418=CARTESIAN_POINT ( 'NONE',  ( 0.7147005917380000461, 1413.022813240129835, 233.2540336019980032 ) ) ;
#2421=ADVANCED_FACE ( 'NONE', ( #67608 ), #17297, .T. ) ;
#2422=DIRECTION ( 'NONE',  ( 0.000000000000000000, 1.000000000000000000, 0.000000000000000000 ) ) ;
#2425=CARTESIAN_POINT ( 'NONE',  ( -18.26675480510339966, 1424.840341062940070, 227.6848255537819909 ) ) ;
#2426=CARTESIAN_POINT ( 'NONE',  ( -12.99662007391709828, 1486.035101518850070, 185.1546605780280004 ) ) ;
#2427=EDGE_CURVE ( 'NONE', #57154, #5163, #43285, .T. ) ;
#2429=CARTESIAN_POINT ( 'NONE',  ( -4.267907479344899890, 1441.147145201229932, 158.2247601545199984 ) ) ;
#2432=B_SPLINE_CURVE_WITH_KNOTS ( 'NONE', 3,
 ( #2111, #9379, #60345, #70424, #78233, #34573, #45212, #2665, #17183, #35127, #68758, #53619, #69309, #96139, #94467, #102316, #78795, #51377, #17740, #1546, #36237, #52501, #27280, #87192, #95041, #19418, #102862, #26159, #51941, #104543, #93916, #27839, #42989, #86085, #87761 ),
 .UNSPECIFIED., .F., .F.,
 ( 4, 2, 2, 1, 1, 1, 2, 2, 2, 2, 1, 1, 2, 2, 2, 2, 1, 1, 2, 2, 4 ),
 ( 0.000000000000000000, 0.1250000000010763057, 0.1875000000015372703, 0.2187500000018319513, 0.2343750000020440594, 0.2421875000021461444, 0.2460937500021343760, 0.2500000000021225799, 0.3125000000017883472, 0.3750000000014541146, 0.4375000000011198265, 0.4687500000009520162, 0.4843750000009499623, 0.5000000000009479084, 0.6250000000006392664, 0.6875000000004880540, 0.7187500000005031531, 0.7343750000006038503, 0.7421875000006541434, 0.7500000000007044365, 1.000000000000000000 ),
 .UNSPECIFIED. ) ;
#2434=CARTESIAN_POINT ( 'NONE',  ( 11.94589852435660049, 1433.532020350129869, 150.0906635879709938 ) ) ;
#2435=CARTESIAN_POINT ( 'NONE',  ( 27.59571790329999885, 1509.876735559930012, 217.1915671101180010 ) ) ;
#2436=ORIENTED_EDGE ( 'NONE', *, *, #3034, .T. ) ;
#2438=CARTESIAN_POINT ( 'NONE',  ( 1.441539424170000139, 1414.983771850430003, 191.7394860166979811 ) ) ;
#2439=CARTESIAN_POINT ( 'NONE',  ( 15.92079754877469888, 1418.953290843069908, 191.2668077924519991 ) ) ;
#2440=CARTESIAN_POINT ( 'NONE',  ( 7.097634907420000694, 1427.571433844230114, 133.6118001900980232 ) ) ;
#2441=CARTESIAN_POINT ( 'NONE',  ( 1.600048698852036821, 1402.754281879943164, 135.5999999980979851 ) ) ;
#2442=CARTESIAN_POINT ( 'NONE',  ( 2.807222226979999569, 1507.639813928429930, 181.3621223444980046 ) ) ;
#2444=CARTESIAN_POINT ( 'NONE',  ( 15.60455980150000066, 1409.457983623130076, 225.4781096464980124 ) ) ;
#2445=SHAPE_REPRESENTATION_RELATIONSHIP ( 'NONE' , 'NONE' ,  #49395, #43980 ) ;
#2447=CARTESIAN_POINT ( 'NONE',  ( 14.02570581375280057, 1415.492117401590122, 197.2936844647439898 ) ) ;
#2449=DIRECTION ( 'NONE',  ( 0.9993908264651745199, 0.03489951250826475032, -1.985168277816197220E-06 ) ) ;
#2451=CARTESIAN_POINT ( 'NONE',  ( 14.41724164474389980, 1435.959222008799998, 149.8873962520480063 ) ) ;
#2452=CARTESIAN_POINT ( 'NONE',  ( -0.2658540493943280514, 1507.120020986029886, 237.3289608297170048 ) ) ;
#2453=ORIENTED_EDGE ( 'NONE', *, *, #40652, .F. ) ;
#2455=ORIENTED_EDGE ( 'NONE', *, *, #89035, .F. ) ;
#2458=CARTESIAN_POINT ( 'NONE',  ( -1.450401227179999974, 1465.036285835330091, 237.9109516336980334 ) ) ;
#2459=CARTESIAN_POINT ( 'NONE',  ( 15.21996770522959075, 1451.144474064526321, 149.5789455636493983 ) ) ;
#2462=CARTESIAN_POINT ( 'NONE',  ( -17.29202514838780047, 1448.661259662438624, 218.6898848943429812 ) ) ;
#2464=CARTESIAN_POINT ( 'NONE',  ( 4.234072258626359719, 1446.327634590550133, 164.0209402114229817 ) ) ;
#2469=CARTESIAN_POINT ( 'NONE',  ( 24.18808457932529876, 1440.913060387330006, 236.3222631112920169 ) ) ;
#2471=CARTESIAN_POINT ( 'NONE',  ( -20.35720481940000326, 1509.285579243329948, 188.5733115188980094 ) ) ;
#2474=CARTESIAN_POINT ( 'NONE',  ( -14.27671737280000031, 1409.578295415130015, 190.9808476275980240 ) ) ;
#2476=CARTESIAN_POINT ( 'NONE',  ( -24.67047192240000086, 1440.997076622129725, 210.6883048062180137 ) ) ;
#2480=CARTESIAN_POINT ( 'NONE',  ( -12.45980060270386325, 1434.393920058226058, 147.3155158375118106 ) ) ;
#2482=CARTESIAN_POINT ( 'NONE',  ( 23.17024198529999879, 1435.306528354219836, 138.2719568257980143 ) ) ;
#2483=CARTESIAN_POINT ( 'NONE',  ( 6.312923550360000746, 1466.069290330830199, 233.5697152015980009 ) ) ;
#2488=CARTESIAN_POINT ( 'NONE',  ( 28.77213281849999760, 1509.917805405330000, 206.8662417206580244 ) ) ;
#2490=CARTESIAN_POINT ( 'NONE',  ( -22.28696231330000188, 1506.798305107930219, 208.8466800722590051 ) ) ;
#2491=CARTESIAN_POINT ( 'NONE',  ( -15.47297587689426557, 1486.079131676784073, 186.6300910287472448 ) ) ;
#2495=CARTESIAN_POINT ( 'NONE',  ( 31.95512683279999777, 1442.955673907409846, 244.1805851208980300 ) ) ;
#2496=CARTESIAN_POINT ( 'NONE',  ( -17.07358046210000069, 1458.578126118629825, 230.5958457830979853 ) ) ;
#2498=CARTESIAN_POINT ( 'NONE',  ( 2.424144924439999738, 1411.756412224629912, 231.8070165610980098 ) ) ;
#2499=CARTESIAN_POINT ( 'NONE',  ( -19.55701159389999688, 1456.127805513129942, 228.1967745823979783 ) ) ;
#2500=CARTESIAN_POINT ( 'NONE',  ( 11.77285469709999965, 1432.580854644329975, 150.8112884974979977 ) ) ;
#2501=CARTESIAN_POINT ( 'NONE',  ( 5.360343482560489647, 1422.243226290559960, 144.1300244169619873 ) ) ;
#2502=CARTESIAN_POINT ( 'NONE',  ( -0.08582555699890000167, 1434.820761659839945, 190.2315579290979883 ) ) ;
#2504=ORIENTED_EDGE ( 'NONE', *, *, #99232, .F. ) ;
#2506=CARTESIAN_POINT ( 'NONE',  ( 0.8891455584299999826, 1405.782266041229832, 268.4834380686980353 ) ) ;
#2508=CARTESIAN_POINT ( 'NONE',  ( 6.451457836568720516, 1472.045055758229864, 270.0713883367370727 ) ) ;
#2509=CARTESIAN_POINT ( 'NONE',  ( 5.449707646490000279, 1437.831544062859848, 154.7230940508980268 ) ) ;
#2510=CARTESIAN_POINT ( 'NONE',  ( -27.95267559379999867, 1445.173348659859812, 137.3670106800980193 ) ) ;
#2511=EDGE_CURVE ( 'NONE', #36154, #43673, #59211, .T. ) ;
#2512=CARTESIAN_POINT ( 'NONE',  ( -39.04178053251449398, 1440.913060396100036, 257.8928201085430487 ) ) ;
#2513=CARTESIAN_POINT ( 'NONE',  ( 35.96429464762940142, 1450.032176740089881, 136.2433800175030001 ) ) ;
#2517=CARTESIAN_POINT ( 'NONE',  ( -1.280362375963175925, 1451.774120661134702, 183.7183834684909129 ) ) ;
#2519=FACE_OUTER_BOUND ( 'NONE', #17744, .T. ) ;
#2525=CARTESIAN_POINT ( 'NONE',  ( -1.323475895380000100, 1475.548043385830169, 269.2940999293979871 ) ) ;
#2527=CARTESIAN_POINT ( 'NONE',  ( -28.14152818990000071, 1508.624282259429947, 209.9763561811920169 ) ) ;
#2528=CARTESIAN_POINT ( 'NONE',  ( -3.160714151128600768, 1448.277390616477760, 184.6271217223835208 ) ) ;
#2531=B_SPLINE_SURFACE_WITH_KNOTS ( 'NONE', 5, 5, ( 
 ( #105964, #29242, #12431, #27583, #86936, #36538 ),
 ( #80752, #37086, #53931, #4060, #11353, #27043 ),
 ( #69620, #45524, #70735, #61230, #104848, #95344 ),
 ( #79665, #71290, #70187, #18605, #10227, #104296 ),
 ( #90788, #39844, #99726, #5699, #93403, #48260 ),
 ( #30879, #59285, #76066, #106498, #13513, #98635 ) ),
 .UNSPECIFIED., .F., .F., .F.,
 ( 6, 6 ),
 ( 6, 6 ),
 ( 30.28564970649999921, 65.26196872020000228 ),
 ( -5.551115123129999410E-17, 2.000000000000000000 ),
 .UNSPECIFIED. ) ;
#2532=CARTESIAN_POINT ( 'NONE',  ( -18.73327636269999985, 1416.067629296030191, 207.5724925610480227 ) ) ;
#2533=CARTESIAN_POINT ( 'NONE',  ( 11.87347576087729983, 1432.890358733870244, 149.9808790610170206 ) ) ;
#2534=CARTESIAN_POINT ( 'NONE',  ( 26.42364260034900170, 1435.420366583209898, 135.3851555990079873 ) ) ;
#2535=CARTESIAN_POINT ( 'NONE',  ( -4.748065736170270057, 1396.078866497700119, 219.0788021602359663 ) ) ;
#2536=CARTESIAN_POINT ( 'NONE',  ( -14.92155151709999927, 1422.314549104929938, 229.4637292825979955 ) ) ;
#2537=CARTESIAN_POINT ( 'NONE',  ( -16.22807784372640327, 1409.487890249900147, 225.2828359470929627 ) ) ;
#2538=CARTESIAN_POINT ( 'NONE',  ( 7.362632729190000447, 1435.943783413959864, 149.6281905168980302 ) ) ;
#2543=CARTESIAN_POINT ( 'NONE',  ( 11.06146551219999985, 1426.045375945929891, 103.4405617616979924 ) ) ;
#2546=CARTESIAN_POINT ( 'NONE',  ( 4.342007114105989274, 1423.862343561519765, 183.6384043889740099 ) ) ;
#2550=CARTESIAN_POINT ( 'NONE',  ( 7.105603315319999780, 1508.968284067629838, 181.5155069444980143 ) ) ;
#2552=CARTESIAN_POINT ( 'NONE',  ( 3.686444929539999915, 1449.169999442819972, 184.1879160448980031 ) ) ;
#2557=ORIENTED_EDGE ( 'NONE', *, *, #36332, .F. ) ;
#2561=CARTESIAN_POINT ( 'NONE',  ( 4.063550476549999679, 1497.713060387329961, 230.5763704537980061 ) ) ;
#2564=CARTESIAN_POINT ( 'NONE',  ( -0.5757066863040000149, 1486.369792037530033, 181.7416807582980027 ) ) ;
#2565=ADVANCED_FACE ( 'NONE', ( #42380 ), #83049, .T. ) ;
#2569=CARTESIAN_POINT ( 'NONE',  ( -2.500000000000000000, 1448.666881541910243, 158.2772778262040276 ) ) ;
#2570=CARTESIAN_POINT ( 'NONE',  ( 7.480565282176630859, 1396.174287483810076, 217.2553306272309896 ) ) ;
#2571=CARTESIAN_POINT ( 'NONE',  ( 13.95725854910000052, 1409.400458595830059, 216.7863739448980027 ) ) ;
#2572=CARTESIAN_POINT ( 'NONE',  ( -0.7741896587115789652, 1405.842756057490078, 267.2348683375010410 ) ) ;
#2573=CARTESIAN_POINT ( 'NONE',  ( 41.14953079480000042, 1443.861296646169876, 136.9341326470980107 ) ) ;
#2575=CARTESIAN_POINT ( 'NONE',  ( -11.30152483640000050, 1432.323726368159896, 151.5220244150980307 ) ) ;
#2576=CARTESIAN_POINT ( 'NONE',  ( 12.77277809070000103, 1442.800511918249867, 187.2257584126980134 ) ) ;
#2577=VERTEX_POINT ( 'NONE', #101166 ) ;
#2583=ORIENTED_EDGE ( 'NONE', *, *, #102915, .T. ) ;
#2588=CARTESIAN_POINT ( 'NONE',  ( -23.46990153750000019, 1440.913060387330006, 234.5287104542979932 ) ) ;
#2591=CARTESIAN_POINT ( 'NONE',  ( -2.820494496349999825, 1409.011554225530062, 231.0801550522980108 ) ) ;
#2592=CARTESIAN_POINT ( 'NONE',  ( -7.473911413859999797, 1445.831988935439767, 184.4657707173980157 ) ) ;
#2595=DIRECTION ( 'NONE',  ( 0.03489949670250328678, -0.9993908270190956511, 0.000000000000000000 ) ) ;
#2599=CARTESIAN_POINT ( 'NONE',  ( -25.68312509100000085, 1435.472708640420024, 135.9883602099980067 ) ) ;
#2600=CARTESIAN_POINT ( 'NONE',  ( 36.10026286240969995, 1420.948621320099846, 270.1974792939670351 ) ) ;
#2603=CIRCLE ( 'NONE', #108064, 0.5000000000000000000 ) ;
#2604=CARTESIAN_POINT ( 'NONE',  ( 0.01879578147808497537, 1507.445532545652668, 237.3948011092800527 ) ) ;
#2606=CARTESIAN_POINT ( 'NONE',  ( 19.19561268899386164, 1410.945033757853935, 195.6515498416322885 ) ) ;
#2609=CARTESIAN_POINT ( 'NONE',  ( -1.837422785889859966, 1451.937235225580025, 184.2647726144609805 ) ) ;
#2610=CARTESIAN_POINT ( 'NONE',  ( -2.354922572530000036, 1415.377356045230044, 232.9301894368979902 ) ) ;
#2612=ORIENTED_EDGE ( 'NONE', *, *, #24045, .T. ) ;
#2615=PRODUCT_DEFINITION_SHAPE ( 'NONE', 'NONE',  #63131 ) ;
#2616=CARTESIAN_POINT ( 'NONE',  ( 7.976687763616449267, 1478.700324351950030, 233.7293620187649879 ) ) ;
#2617=CARTESIAN_POINT ( 'NONE',  ( -23.16109911851550152, 1509.676460279360299, 226.5529115091270000 ) ) ;
#2618=CARTESIAN_POINT ( 'NONE',  ( -2.680555363329999885, 1409.943153559129996, 186.5983026406979945 ) ) ;
#2619=CARTESIAN_POINT ( 'NONE',  ( -0.3489575399770000197, 1409.432092532930028, 233.0021930383979907 ) ) ;
#2620=DIRECTION ( 'NONE',  ( 0.000000000000000000, 0.000000000000000000, 1.000000000000000000 ) ) ;
#2622=CARTESIAN_POINT ( 'NONE',  ( -3.895671750679999601, 1421.575785769229924, 185.6035415176980052 ) ) ;
#2623=CARTESIAN_POINT ( 'NONE',  ( 18.85941592800000066, 1507.948893524529922, 188.5324247627980014 ) ) ;
#2624=CARTESIAN_POINT ( 'NONE',  ( -10.73514660131351839, 1424.973046421745494, 139.1354236205272343 ) ) ;
#2625=ORIENTED_EDGE ( 'NONE', *, *, #23915, .T. ) ;
#2626=CARTESIAN_POINT ( 'NONE',  ( -12.70695307632060000, 1416.230844595159851, 196.1160997689679846 ) ) ;
#2636=CARTESIAN_POINT ( 'NONE',  ( -17.60627563539920004, 1410.895669414250051, 194.0661810348550205 ) ) ;
#2637=CARTESIAN_POINT ( 'NONE',  ( -18.46184065339999592, 1425.292999754929951, 225.8901492113980112 ) ) ;
#2638=CARTESIAN_POINT ( 'NONE',  ( -18.60903282430000161, 1435.578292681360153, 146.4159160996979949 ) ) ;
#2640=DIRECTION ( 'NONE',  ( 0.000000000000000000, -1.000000000000000000, 0.000000000000000000 ) ) ;
#2646=CARTESIAN_POINT ( 'NONE',  ( 27.24409202460000046, 1507.989521382530029, 207.2276950740879897 ) ) ;
#2651=CARTESIAN_POINT ( 'NONE',  ( 11.31902516476188403, 1434.496189561966730, 151.5389523139992036 ) ) ;
#2652=B_SPLINE_SURFACE_WITH_KNOTS ( 'NONE', 5, 1, ( 
 ( #62206, #72793 ),
 ( #106920, #19611 ),
 ( #53813, #54354 ),
 ( #87949, #105845 ),
 ( #79541, #98523 ),
 ( #21789, #2844 ),
 ( #38075, #71159 ),
 ( #105282, #88485 ),
 ( #37526, #62773 ),
 ( #72252, #20158 ),
 ( #97429, #66612 ),
 ( #49796, #91772 ),
 ( #31870, #57104 ),
 ( #66059, #85432 ),
 ( #58193, #15050 ),
 ( #23466, #100183 ),
 ( #99610, #42910 ),
 ( #81709, #90669 ),
 ( #49248, #68676 ),
 ( #77067, #92321 ),
 ( #108584, #40271 ),
 ( #75002, #47584 ),
 ( #48142, #32436 ),
 ( #109152, #15592 ) ),
 .UNSPECIFIED., .F., .F., .F.,
 ( 6, 3, 3, 3, 3, 3, 3, 6 ),
 ( 2, 2 ),
 ( 21.22849039669999982, 21.28303926239999910, 21.63383848259999809, 29.22288786549999884, 33.07574020050000030, 38.86051041610000567, 44.90455290039999880, 44.92448007948200228 ),
 ( 0.000000000000000000, 4.091690576229590093 ),
 .UNSPECIFIED. ) ;
#2653=CARTESIAN_POINT ( 'NONE',  ( -24.89734149463049917, 1440.895437401190065, 210.4282814422280126 ) ) ;
#2654=CARTESIAN_POINT ( 'NONE',  ( -22.48884418427819654, 1509.698386039090110, 189.0638421303760026 ) ) ;
#2658=EDGE_CURVE ( 'NONE', #75744, #32788, #24653, .T. ) ;
#2661=FACE_OUTER_BOUND ( 'NONE', #7524, .T. ) ;
#2665=CARTESIAN_POINT ( 'NONE',  ( -18.44192439828749386, 1458.893192691106606, 227.6840821340426828 ) ) ;
#2668=ADVANCED_FACE ( 'NONE', ( #103945 ), #50924, .F. ) ;
#2671=CARTESIAN_POINT ( 'NONE',  ( 18.24633262864339756, 1416.842625005220043, 209.2839319684169936 ) ) ;
#2673=CARTESIAN_POINT ( 'NONE',  ( 13.05900637259455088, 1442.991450065072740, 169.4123328598832927 ) ) ;
#2674=CARTESIAN_POINT ( 'NONE',  ( 38.89664643686552381, 1429.356341322375329, 269.5911935481951218 ) ) ;
#2675=CARTESIAN_POINT ( 'NONE',  ( -45.67178388729999483, 1443.699401684990107, 266.1886045289979847 ) ) ;
#2678=FACE_OUTER_BOUND ( 'NONE', #50434, .T. ) ;
#2680=CARTESIAN_POINT ( 'NONE',  ( -19.74739994659999809, 1486.108233622730040, 190.1528327617980096 ) ) ;
#2681=CARTESIAN_POINT ( 'NONE',  ( 13.85929416610000153, 1410.325638497430191, 191.1496551215980162 ) ) ;
#2682=CARTESIAN_POINT ( 'NONE',  ( 5.419569259119999316, 1423.396285514930014, 185.7614624571979789 ) ) ;
#2684=CARTESIAN_POINT ( 'NONE',  ( -6.070028495709999916, 1440.055555071880008, 154.5780773277979847 ) ) ;
#2685=CARTESIAN_POINT ( 'NONE',  ( 7.539474771970000155, 1438.620589226539778, 153.9375993584980051 ) ) ;
#2693=CARTESIAN_POINT ( 'NONE',  ( -42.28244123120000353, 1440.913087102529971, 269.8809842803979677 ) ) ;
#2695=CARTESIAN_POINT ( 'NONE',  ( 17.84692852179999889, 1410.032953050229935, 222.8512888978980016 ) ) ;
#2697=CARTESIAN_POINT ( 'NONE',  ( 9.202936508599998788, 1519.913060387329779, 187.9174701372980110 ) ) ;
#2701=CARTESIAN_POINT ( 'NONE',  ( -43.64288401327429767, 1430.870968838220051, 269.0307669793850209 ) ) ;
#2702=FACE_OUTER_BOUND ( 'NONE', #87860, .T. ) ;
#2705=ORIENTED_EDGE ( 'NONE', *, *, #13807, .F. ) ;
#2709=CARTESIAN_POINT ( 'NONE',  ( -21.92423686329999910, 1509.678671609130106, 190.3411753249980052 ) ) ;
#2710=CARTESIAN_POINT ( 'NONE',  ( -11.93035415709999825, 1425.413819132130129, 188.4997697822980172 ) ) ;
#2714=CARTESIAN_POINT ( 'NONE',  ( 11.60004869885203860, 1425.798524488559224, 137.3564486607050128 ) ) ;
#2721=CARTESIAN_POINT ( 'NONE',  ( -22.30921403175210216, 1414.773190229989950, 269.6722363558229745 ) ) ;
#2723=CARTESIAN_POINT ( 'NONE',  ( 2.075990293979999676E-15, 1427.305457135430061, 123.0297916884979941 ) ) ;
#2726=ORIENTED_EDGE ( 'NONE', *, *, #17330, .T. ) ;
#2727=ORIENTED_EDGE ( 'NONE', *, *, #2658, .T. ) ;
#2728=CARTESIAN_POINT ( 'NONE',  ( 45.58236131563670313, 1442.587618990865167, 268.9762474203030820 ) ) ;
#2730=CARTESIAN_POINT ( 'NONE',  ( 3.631811699416766182, 1424.449122815756482, 184.4189500110305744 ) ) ;
#2731=CARTESIAN_POINT ( 'NONE',  ( -0.7722883701989260441, 1405.989080711971610, 266.9611463895769248 ) ) ;
#2732=B_SPLINE_SURFACE_WITH_KNOTS ( 'NONE', 3, 5, ( 
 ( #62215, #96341, #54364, #87960, #11249, #45410 ),
 ( #36976, #71168, #88494, #46509, #69516, #103637 ),
 ( #26934, #61125, #48152, #63859, #64956, #23476 ),
 ( #5589, #39738, #107479, #65510, #57113, #72260 ) ),
 .UNSPECIFIED., .F., .F., .F.,
 ( 4, 4 ),
 ( 6, 6 ),
 ( 9.885439000899999940, 20.49136985950000067 ),
 ( -1.110223024629999900E-16, 1.000000000000000000 ),
 .UNSPECIFIED. ) ;
#2733=CARTESIAN_POINT ( 'NONE',  ( -21.03310440946566118, 1506.473666153777458, 215.6352647881066389 ) ) ;
#2734=CARTESIAN_POINT ( 'NONE',  ( -19.33962896530000108, 1430.793376614329873, 224.1389769688979925 ) ) ;
#2735=CARTESIAN_POINT ( 'NONE',  ( -14.45783241110000006, 1416.839692138830060, 221.3920770704979759 ) ) ;
#2738=CARTESIAN_POINT ( 'NONE',  ( 5.582246511119999255, 1448.050470245740144, 184.8003903095979865 ) ) ;
#2740=ORIENTED_EDGE ( 'NONE', *, *, #68131, .T. ) ;
#2742=CARTESIAN_POINT ( 'NONE',  ( 1.470748360624610118, 1485.779233187629870, 182.0437263276170086 ) ) ;
#2745=CARTESIAN_POINT ( 'NONE',  ( 26.02147390689500028, 1451.119159405719984, 136.5906395866829826 ) ) ;
#2747=CARTESIAN_POINT ( 'NONE',  ( 13.58235846979999906, 1416.828040475229955, 196.3349388281980055 ) ) ;
#2750=CARTESIAN_POINT ( 'NONE',  ( 17.53069353509999928, 1410.450030956830005, 192.7292893744979949 ) ) ;
#2751=CARTESIAN_POINT ( 'NONE',  ( 16.90742463041998178, 1444.994950788469168, 162.4348201727410981 ) ) ;
#2752=CARTESIAN_POINT ( 'NONE',  ( 16.19062492770000006, 1409.478449468330155, 224.9177422266980102 ) ) ;
#2753=CARTESIAN_POINT ( 'NONE',  ( -19.39313673858097786, 1425.487805292472331, 223.5657354981669016 ) ) ;
#2754=CARTESIAN_POINT ( 'NONE',  ( 0.4857184740991669636, 1450.960785378189939, 181.9315177450459942 ) ) ;
#2757=CARTESIAN_POINT ( 'NONE',  ( 26.02532873005809932, 1446.299728326420109, 138.3445498427680036 ) ) ;
#2763=CARTESIAN_POINT ( 'NONE',  ( -1275.711986934299830, 50.13405481578730161, 10006.43705117240097 ) ) ;
#2765=CARTESIAN_POINT ( 'NONE',  ( -38.10256990246180209, 1448.730340511050144, 136.3926152995410064 ) ) ;
#2767=CARTESIAN_POINT ( 'NONE',  ( -4.540901342749999792, 1462.614442895030152, 248.0989693022980020 ) ) ;
#2769=CARTESIAN_POINT ( 'NONE',  ( 11.21203837859999908, 1433.014098020569918, 151.5746018212979891 ) ) ;
#2776=CARTESIAN_POINT ( 'NONE',  ( -2.500000000000000000, 1425.929641636930000, 184.1455913746980002 ) ) ;
#2778=CARTESIAN_POINT ( 'NONE',  ( -3.521375377790000094, 1486.251522346130059, 181.9026547285980087 ) ) ;
#2779=CARTESIAN_POINT ( 'NONE',  ( 0.9465674214180413992, 1397.942249001653408, 196.1218459535367344 ) ) ;
#2781=CARTESIAN_POINT ( 'NONE',  ( 24.62246550709999937, 1430.359249624430277, 210.8418034199980013 ) ) ;
#2783=CARTESIAN_POINT ( 'NONE',  ( -14.23402513019999915, 1509.239477817229954, 233.4640051292979877 ) ) ;
#2786=CARTESIAN_POINT ( 'NONE',  ( 2.499937251232230206, 1420.100124192889780, 93.04876811845220175 ) ) ;
#2791=CARTESIAN_POINT ( 'NONE',  ( -0.5621806315070000393, 1416.843576368729828, 227.7683147415980045 ) ) ;
#2794=EDGE_CURVE ( 'NONE', #62471, #93599, #3249, .T. ) ;
#2795=CARTESIAN_POINT ( 'NONE',  ( -35.54866228632759828, 1451.502040174180138, 134.0999999984919668 ) ) ;
#2800=( BOUNDED_CURVE ( )  B_SPLINE_CURVE ( 3, ( #65459, #91182, #14462, #48656 ),
 .UNSPECIFIED., .F., .T. ) 
 B_SPLINE_CURVE_WITH_KNOTS ( ( 4, 4 ),
 ( 1.569840739599899893, 1.584370187438904898 ),
 .UNSPECIFIED. ) 
 CURVE ( )  GEOMETRIC_REPRESENTATION_ITEM ( )  RATIONAL_B_SPLINE_CURVE ( ( 1.000000000000000000, 0.9999824080061611165, 0.9999824080061611165, 1.000000000000000000 ) ) 
 REPRESENTATION_ITEM ( '' )  );
#2803=CARTESIAN_POINT ( 'NONE',  ( 23.52438575543722266, 1410.744643456190261, 207.8036212700959027 ) ) ;
#2806=CARTESIAN_POINT ( 'NONE',  ( 10.95613331925090073, 1409.295656986259928, 219.2973035561870176 ) ) ;
#2809=CARTESIAN_POINT ( 'NONE',  ( -18.21532205240000124, 1430.623180213430032, 192.4625600593979868 ) ) ;
#2811=FACE_OUTER_BOUND ( 'NONE', #36135, .T. ) ;
#2814=CARTESIAN_POINT ( 'NONE',  ( -11.48964235823120106, 1415.152886232609944, 195.4311914138980057 ) ) ;
#2816=CARTESIAN_POINT ( 'NONE',  ( 29.63432559401041644, 1509.974525581411626, 210.8805246852537891 ) ) ;
#2818=CARTESIAN_POINT ( 'NONE',  ( 3.843918134389999963, 1397.403951559329926, 221.5816238264980029 ) ) ;
#2819=CARTESIAN_POINT ( 'NONE',  ( 1.704993463989999958, 1417.527066604930042, 233.7744655226979944 ) ) ;
#2821=CARTESIAN_POINT ( 'NONE',  ( -0.5133842287350000033, 1453.574655232029954, 183.2220989632980093 ) ) ;
#2826=CARTESIAN_POINT ( 'NONE',  ( -12.88529584148609963, 1435.823228682630088, 150.7601930830520018 ) ) ;
#2827=CARTESIAN_POINT ( 'NONE',  ( 3.047790189539999695, 1421.605827388129910, 133.5221414154979698 ) ) ;
#2830=CARTESIAN_POINT ( 'NONE',  ( 40.82021089259919933, 1444.183590552639998, 136.9680080752169999 ) ) ;
#2832=CARTESIAN_POINT ( 'NONE',  ( -23.31685689360000069, 1508.124115171030098, 195.2425524244979727 ) ) ;
#2833=CARTESIAN_POINT ( 'NONE',  ( -11.03890283615240087, 1426.504156864669994, 93.54506299971779981 ) ) ;
#2835=CARTESIAN_POINT ( 'NONE',  ( -0.6474865636856289575, 1507.275793736380137, 231.8019763530149930 ) ) ;
#2838=CARTESIAN_POINT ( 'NONE',  ( -18.32011680670000331, 1412.375216495030145, 259.8063326943979519 ) ) ;
#2840=CARTESIAN_POINT ( 'NONE',  ( -26.09332909799999811, 1435.428316942780157, 135.6095828681980038 ) ) ;
#2841=CARTESIAN_POINT ( 'NONE',  ( 2.516438831412172394, 1448.700965663029820, 154.6256843495723103 ) ) ;
#2842=CARTESIAN_POINT ( 'NONE',  ( 12.51099983133400073, 1416.825784014559986, 196.0986189223339977 ) ) ;
#2844=CARTESIAN_POINT ( 'NONE',  ( -5.386055587696130686, 1432.253251891989976, 154.6059980213289862 ) ) ;
#2846=CARTESIAN_POINT ( 'NONE',  ( 5.886744298249999119, 1509.118630028029884, 238.1980421559979959 ) ) ;
#2851=EDGE_LOOP ( 'NONE', ( #82408, #92311, #63309, #90861 ) ) ;
#2852=CARTESIAN_POINT ( 'NONE',  ( -0.3231955925520000328, 1419.319817403729985, 184.6083566393980107 ) ) ;
#2855=CARTESIAN_POINT ( 'NONE',  ( -3.210018582440000046, 1470.482941419229974, 235.1373499011980073 ) ) ;
#2860=CARTESIAN_POINT ( 'NONE',  ( 11.15489169059999952, 1425.160568487430055, 144.1681086605980227 ) ) ;
#2866=ORIENTED_EDGE ( 'NONE', *, *, #53184, .T. ) ;
#2867=CARTESIAN_POINT ( 'NONE',  ( 11.86420161318850042, 1432.203304325139925, 149.9807413596300023 ) ) ;
#2869=CARTESIAN_POINT ( 'NONE',  ( 13.39865035957124029, 1444.421645391301581, 187.7321514735085088 ) ) ;
#2871=ORIENTED_EDGE ( 'NONE', *, *, #47610, .T. ) ;
#2872=CARTESIAN_POINT ( 'NONE',  ( 5.370527602886283169, 1422.356908813907012, 139.1416118586824666 ) ) ;
#2873=EDGE_CURVE ( 'NONE', #49524, #3437, #29264, .T. ) ;
#2875=CARTESIAN_POINT ( 'NONE',  ( 10.88110552090000027, 1508.288216035629830, 234.3544958320979958 ) ) ;
#2879=CARTESIAN_POINT ( 'NONE',  ( 20.20676118117160058, 1452.207424737969859, 143.0075041318320075 ) ) ;
#2880=CARTESIAN_POINT ( 'NONE',  ( 3.409543808716749780, 1410.339071755739951, 269.6161397029929958 ) ) ;
#2890=CARTESIAN_POINT ( 'NONE',  ( 17.73489863255730015, 1415.061873231259824, 224.9295571200040058 ) ) ;
#2892=ORIENTED_EDGE ( 'NONE', *, *, #104822, .F. ) ;
#2893=CARTESIAN_POINT ( 'NONE',  ( 28.05448519009999941, 1420.250147135629959, 265.6112251771979800 ) ) ;
#2894=CARTESIAN_POINT ( 'NONE',  ( 13.20531104009999979, 1434.869042435399933, 149.0170821157980185 ) ) ;
#2898=CARTESIAN_POINT ( 'NONE',  ( 45.63714000780699820, 1434.626146812550132, 268.9747433262190270 ) ) ;
#2903=CARTESIAN_POINT ( 'NONE',  ( -24.35236995230000190, 1444.655896658020083, 211.1425131463980165 ) ) ;
#2904=CARTESIAN_POINT ( 'NONE',  ( -2.319649531331190229, 1449.727814782791029, 154.4137922862332459 ) ) ;
#2906=CARTESIAN_POINT ( 'NONE',  ( 18.28372774912679688, 1419.974404435409951, 223.2769049341759739 ) ) ;
#2907=CARTESIAN_POINT ( 'NONE',  ( -10.93437594629999943, 1442.547277881270020, 185.2874795750979899 ) ) ;
#2908=EDGE_CURVE ( 'NONE', #11508, #65085, #80, .T. ) ;
#2909=CARTESIAN_POINT ( 'NONE',  ( 30.40044630675230053, 1510.013553480240034, 213.6863598775470052 ) ) ;
#2911=CARTESIAN_POINT ( 'NONE',  ( 12.71481701828757949, 1434.614953001262847, 149.3394185820198743 ) ) ;
#2912=ADVANCED_FACE ( 'NONE', ( #30547 ), #64736, .T. ) ;
#2913=CARTESIAN_POINT ( 'NONE',  ( 13.93256980790000021, 1412.742330145629921, 228.1707926741980259 ) ) ;
#2915=CARTESIAN_POINT ( 'NONE',  ( -15.88332445569999862, 1459.702822082929970, 228.9589543435980090 ) ) ;
#2917=CARTESIAN_POINT ( 'NONE',  ( 41.36157324430000415, 1425.216340838630003, 268.6469744794979988 ) ) ;
#2918=CARTESIAN_POINT ( 'NONE',  ( -17.99881233489999843, 1409.541592764029929, 221.8083273357979976 ) ) ;
#2919=CARTESIAN_POINT ( 'NONE',  ( 20.43352477559999869, 1435.211929165099946, 143.2813443149979946 ) ) ;
#2921=CARTESIAN_POINT ( 'NONE',  ( 20.06092942580000127, 1488.587903410330000, 190.6166884224980151 ) ) ;
#2922=CARTESIAN_POINT ( 'NONE',  ( 29.22958591724099975, 1509.933780020319773, 206.4713313096740137 ) ) ;
#2925=CARTESIAN_POINT ( 'NONE',  ( -15.97706642740000227, 1420.887606515729885, 227.0366021596980204 ) ) ;
#2927=CARTESIAN_POINT ( 'NONE',  ( -40.67505929589849956, 1440.823025992459861, 136.6075842068449901 ) ) ;
#2928=CARTESIAN_POINT ( 'NONE',  ( -7.881523990731260199, 1408.659461760370050, 198.0058231072500234 ) ) ;
#2930=CARTESIAN_POINT ( 'NONE',  ( -12.80028686799999882, 1442.828808077900021, 186.6514660660979814 ) ) ;
#2931=CARTESIAN_POINT ( 'NONE',  ( -27.86688904147829859, 1508.626580732350021, 210.5580440514449947 ) ) ;
#2932=CARTESIAN_POINT ( 'NONE',  ( -30.80657653509999605, 1436.049661374800053, 136.3951857664980025 ) ) ;
#2933=DIRECTION ( 'NONE',  ( 0.3892484888175031799, -0.9211327884476211425, 0.000000000000000000 ) ) ;
#2936=CARTESIAN_POINT ( 'NONE',  ( -4.827031846966990614, 1409.081624053799942, 223.3000366672669941 ) ) ;
#2939=FACE_OUTER_BOUND ( 'NONE', #88360, .T. ) ;
#2940=CARTESIAN_POINT ( 'NONE',  ( -42.28308919219999495, 1455.990853814730144, 268.6218227887980561 ) ) ;
#2942=CARTESIAN_POINT ( 'NONE',  ( -2.382436964801009083, 1426.901689560119166, 137.0999999980979567 ) ) ;
#2943=CARTESIAN_POINT ( 'NONE',  ( -26.47494755039999959, 1509.166824640230061, 216.3301573140479945 ) ) ;
#2946=CARTESIAN_POINT ( 'NONE',  ( -5.992819232552549558, 1405.413060387330006, 198.1520639380683235 ) ) ;
#2947=CARTESIAN_POINT ( 'NONE',  ( 22.52523981570000089, 1509.699659094630078, 227.7647078266979861 ) ) ;
#2948=CARTESIAN_POINT ( 'NONE',  ( 14.91982466159999987, 1485.050512577729933, 224.1086942190979983 ) ) ;
#2949=ADVANCED_FACE ( 'NONE', ( #65276 ), #49574, .T. ) ;
#2951=CARTESIAN_POINT ( 'NONE',  ( -26.68246396532270026, 1495.347229232020027, 211.0255316263900056 ) ) ;
#2954=CARTESIAN_POINT ( 'NONE',  ( -3.567504847130000378, 1508.690878337329877, 180.4372022099980200 ) ) ;
#2958=CARTESIAN_POINT ( 'NONE',  ( -11.53430538779999992, 1415.163755998629995, 195.3861979139979894 ) ) ;
#2960=CARTESIAN_POINT ( 'NONE',  ( 23.75575072150000011, 1410.664328360029913, 210.9000785660479949 ) ) ;
#2963=CARTESIAN_POINT ( 'NONE',  ( -5.360093979568320677, 1422.720973808630106, 147.5125564607829745 ) ) ;
#2970=CARTESIAN_POINT ( 'NONE',  ( -1.288412296889219766, 1419.848508814950264, 185.1203347260929775 ) ) ;
#2974=CARTESIAN_POINT ( 'NONE',  ( -16.67081401233100024, 1485.422209799639859, 187.9724624971670153 ) ) ;
#2978=ORIENTED_EDGE ( 'NONE', *, *, #90427, .T. ) ;
#2980=CARTESIAN_POINT ( 'NONE',  ( 29.12655685680000062, 1509.869978479729980, 210.7036736057679889 ) ) ;
#2984=( BOUNDED_CURVE ( )  B_SPLINE_CURVE ( 3, ( #106814, #3295, #47486, #37427 ),
 .UNSPECIFIED., .F., .F. ) 
 B_SPLINE_CURVE_WITH_KNOTS ( ( 4, 4 ),
 ( 3.106755518160905005, 3.118534288586135350 ),
 .UNSPECIFIED. ) 
 CURVE ( )  GEOMETRIC_REPRESENTATION_ITEM ( )  RATIONAL_B_SPLINE_CURVE ( ( 1.000000000000000000, 0.9999884384140235172, 0.9999884384140235172, 1.000000000000000000 ) ) 
 REPRESENTATION_ITEM ( '' )  );
#2985=CARTESIAN_POINT ( 'NONE',  ( 15.88602804442459870, 1417.757759938499930, 191.3037173568610001 ) ) ;
#2986=CARTESIAN_POINT ( 'NONE',  ( 24.61702284729999946, 1442.198266432479841, 213.4925807370779864 ) ) ;
#2987=CARTESIAN_POINT ( 'NONE',  ( -0.8945946638535250406, 1417.298095655010002, 235.8147265033050246 ) ) ;
#2989=CARTESIAN_POINT ( 'NONE',  ( -25.31584570420000091, 1451.871603816930246, 136.1751615687979893 ) ) ;
#2990=CARTESIAN_POINT ( 'NONE',  ( 8.178501070643639181, 1441.152429762079919, 153.9860758848200248 ) ) ;
#2991=CARTESIAN_POINT ( 'NONE',  ( 5.659654762769999792, 1409.110699888030013, 230.1372059342980094 ) ) ;
#2993=CARTESIAN_POINT ( 'NONE',  ( 41.63894744325380515, 1444.312235791039939, 134.0999999983169744 ) ) ;
#2995=CARTESIAN_POINT ( 'NONE',  ( -0.5635418445434529078, 1419.788636389980184, 227.8982600517779815 ) ) ;
#2996=ORIENTED_EDGE ( 'NONE', *, *, #78745, .F. ) ;
#3004=CARTESIAN_POINT ( 'NONE',  ( -1.499470402960000115, 1465.333991039530019, 236.0689215525979705 ) ) ;
#3005=CARTESIAN_POINT ( 'NONE',  ( 21.08599079332655890, 1450.945512302869247, 144.3583723772087808 ) ) ;
#3008=CARTESIAN_POINT ( 'NONE',  ( -18.54137802971740001, 1445.596289520634400, 214.4230706237874813 ) ) ;
#3010=CARTESIAN_POINT ( 'NONE',  ( 4.254108446939370403, 1446.519541462919960, 160.4550363066709906 ) ) ;
#3013=ORIENTED_EDGE ( 'NONE', *, *, #19215, .F. ) ;
#3017=CARTESIAN_POINT ( 'NONE',  ( 24.29942712596140098, 1440.913060387330006, 236.7211978293100003 ) ) ;
#3018=CARTESIAN_POINT ( 'NONE',  ( -15.81194716269999923, 1509.534088746730049, 183.7661278115980110 ) ) ;
#3021=CARTESIAN_POINT ( 'NONE',  ( 25.87535885525390000, 1449.883803224160147, 136.9992940508379888 ) ) ;
#3022=CARTESIAN_POINT ( 'NONE',  ( -14.55035415250000064, 1409.421169950730018, 191.6335217687980048 ) ) ;
#3026=CARTESIAN_POINT ( 'NONE',  ( 22.53780194058930064, 1411.035674245950077, 206.1988793083210112 ) ) ;
#3028=CARTESIAN_POINT ( 'NONE',  ( 1.356522472024429993, 1410.335674015750101, 232.6399073486850000 ) ) ;
#3029=CARTESIAN_POINT ( 'NONE',  ( -13.50104314780000081, 1434.968970217379820, 148.5641363387979936 ) ) ;
#3031=CARTESIAN_POINT ( 'NONE',  ( 6.227622670500000623, 1464.007336795129959, 235.2942956369979868 ) ) ;
#3034=EDGE_CURVE ( 'NONE', #80762, #8717, #17270, .T. ) ;
#3036=ADVANCED_FACE ( 'NONE', ( #102150 ), #41040, .F. ) ;
#3045=CARTESIAN_POINT ( 'NONE',  ( 24.64758684679999945, 1455.655050828230060, 240.2509105760980219 ) ) ;
#3047=CARTESIAN_POINT ( 'NONE',  ( -25.94248324348950163, 1509.818991864719919, 222.8344883908499980 ) ) ;
#3049=ADVANCED_FACE ( 'NONE', ( #13044 ), #33926, .F. ) ;
#3050=CARTESIAN_POINT ( 'NONE',  ( -20.89412605160000069, 1454.104942495830073, 223.6452089798980012 ) ) ;
#3051=CARTESIAN_POINT ( 'NONE',  ( 10.97117078989999861, 1432.448750475399947, 151.7701039698980026 ) ) ;
#3052=CARTESIAN_POINT ( 'NONE',  ( 5.386275313190370007, 1432.307805056000007, 154.6069887461920018 ) ) ;
#3057=CARTESIAN_POINT ( 'NONE',  ( 0.5545655831749999320, 1406.267234724929949, 269.2946136120979759 ) ) ;
#3058=EDGE_CURVE ( 'NONE', #99066, #109412, #62977, .T. ) ;
#3060=CARTESIAN_POINT ( 'NONE',  ( 38.52648929541060596, 1455.895828382030004, 270.1643681006679572 ) ) ;
#3061=CARTESIAN_POINT ( 'NONE',  ( 5.519877061429999898, 1440.499830656789982, 154.7645262406979896 ) ) ;
#3062=CARTESIAN_POINT ( 'NONE',  ( 11.60004869885203682, 1425.894345409931248, 137.5113366366250034 ) ) ;
#3063=B_SPLINE_CURVE_WITH_KNOTS ( 'NONE', 3,
 ( #18293, #2092, #52486, #79334, #86614, #10462, #88280, #44077, #19395, #77671, #44636, #78777 ),
 .UNSPECIFIED., .F., .F.,
 ( 4, 2, 2, 2, 2, 4 ),
 ( -0.1123552135074580016, -0.09789198044012829836, -0.08346214397256018769, -0.05408911794985069715, -0.02844460996696679400, -2.821931098934138404E-07 ),
 .UNSPECIFIED. ) ;
#3064=CARTESIAN_POINT ( 'NONE',  ( -36.36844575302269789, 1440.913060387330006, 253.5188197989739933 ) ) ;
#3065=CARTESIAN_POINT ( 'NONE',  ( -25.71870319980000019, 1450.791960742989886, 136.8495502446980083 ) ) ;
#3068=CARTESIAN_POINT ( 'NONE',  ( 1.459574821760450059, 1450.689303316930136, 154.7904039106100242 ) ) ;
#3071=CARTESIAN_POINT ( 'NONE',  ( -1.546949757679999760, 1416.828040475729949, 228.0209010782980101 ) ) ;
#3072=VERTEX_POINT ( 'NONE', #38264 ) ;
#3073=CARTESIAN_POINT ( 'NONE',  ( -22.74199304079999706, 1435.511682894840078, 234.3916895436979928 ) ) ;
#3076=CARTESIAN_POINT ( 'NONE',  ( -1.333808752909999784, 1476.063104645729936, 267.5364536224980156 ) ) ;
#3078=CARTESIAN_POINT ( 'NONE',  ( -27.93158978740000009, 1508.017348977630036, 210.2982006691480024 ) ) ;
#3082=CARTESIAN_POINT ( 'NONE',  ( -18.79647799810000208, 1416.822690122329959, 208.4084635082059833 ) ) ;
#3084=CARTESIAN_POINT ( 'NONE',  ( 26.56954545285969616, 1436.266953136529992, 136.6620164141489795 ) ) ;
#3085=CARTESIAN_POINT ( 'NONE',  ( -10.84999001794609974, 1396.291950387739917, 211.3263223283950083 ) ) ;
#3086=CARTESIAN_POINT ( 'NONE',  ( -15.81043287432200017, 1421.035995845646084, 227.0411833758840032 ) ) ;
#3087=CARTESIAN_POINT ( 'NONE',  ( -16.59998697850549831, 1410.444752549930172, 226.4425751357730121 ) ) ;
#3088=CARTESIAN_POINT ( 'NONE',  ( -45.62036884359999789, 1439.936247324329770, 268.9752023951979822 ) ) ;
#3093=CARTESIAN_POINT ( 'NONE',  ( 11.17341440289999888, 1425.629743028729990, 126.2832056323980083 ) ) ;
#3100=CARTESIAN_POINT ( 'NONE',  ( -11.86716023049999968, 1432.353341358199941, 147.6509521729980179 ) ) ;
#3101=CARTESIAN_POINT ( 'NONE',  ( 7.312123808780000012, 1507.578463809529921, 182.6814736750980046 ) ) ;
#3108=DIRECTION ( 'NONE',  ( 1.000000000000000000, 0.000000000000000000, 0.000000000000000000 ) ) ;
#3109=FACE_OUTER_BOUND ( 'NONE', #94071, .T. ) ;
#3116=CARTESIAN_POINT ( 'NONE',  ( 13.15366522099999891, 1428.703228679929907, 223.0784815109979888 ) ) ;
#3117=CARTESIAN_POINT ( 'NONE',  ( -40.26396339707969219, 1444.186527608570032, 137.1012300132789790 ) ) ;
#3118=B_SPLINE_CURVE_WITH_KNOTS ( 'NONE', 5,
 ( #70328, #25504, #77046, #59694, #60814, #34479 ),
 .UNSPECIFIED., .F., .F.,
 ( 6, 6 ),
 ( 0.000000000000000000, 1.000000000000000000 ),
 .UNSPECIFIED. ) ;
#3119=CARTESIAN_POINT ( 'NONE',  ( -2.500000000000000000, 1448.375148597939869, 162.6885153068710110 ) ) ;
#3120=CARTESIAN_POINT ( 'NONE',  ( 26.79414481833639883, 1435.433178084320161, 135.2874577367330176 ) ) ;
#3121=FACE_OUTER_BOUND ( 'NONE', #50968, .T. ) ;
#3122=CARTESIAN_POINT ( 'NONE',  ( -3.804492251863449859, 1406.371137055889903, 269.2897714392109947 ) ) ;
#3123=CARTESIAN_POINT ( 'NONE',  ( -18.64588652299999794, 1416.828040475229955, 208.5593769277110141 ) ) ;
#3125=CARTESIAN_POINT ( 'NONE',  ( 4.095657388320000258, 1423.950325605830130, 183.4778182170979903 ) ) ;
#3126=CARTESIAN_POINT ( 'NONE',  ( 12.24860663770000002, 1442.680101602390096, 186.9125332272980131 ) ) ;
#3127=ORIENTED_EDGE ( 'NONE', *, *, #89493, .F. ) ;
#3140=CARTESIAN_POINT ( 'NONE',  ( -41.02245140317685212, 1434.148376033890372, 269.6289973472830184 ) ) ;
#3142=CARTESIAN_POINT ( 'NONE',  ( -9.486449742109998695, 1409.244334512030036, 228.2930016836979803 ) ) ;
#3144=CARTESIAN_POINT ( 'NONE',  ( -8.965713971590000497, 1447.579297599270149, 186.2691576776979900 ) ) ;
#3145=ORIENTED_EDGE ( 'NONE', *, *, #8545, .T. ) ;
#3146=DIRECTION ( 'NONE',  ( 0.000000000000000000, 0.000000000000000000, 1.000000000000000000 ) ) ;
#3150=CARTESIAN_POINT ( 'NONE',  ( 15.56138138183905362, 1506.691119442913987, 224.9532563058226913 ) ) ;
#3151=ADVANCED_FACE ( 'NONE', ( #91438 ), #28602, .F. ) ;
#3152=CARTESIAN_POINT ( 'NONE',  ( 27.75956368386599848, 1417.581732837509890, 269.7078427950669948 ) ) ;
#3157=CARTESIAN_POINT ( 'NONE',  ( 0.01643980240737619863, 1507.683248503670711, 237.4603286191148754 ) ) ;
#3159=CARTESIAN_POINT ( 'NONE',  ( 18.70421975728147501, 1410.928392002681903, 194.6991403882563532 ) ) ;
#3162=CARTESIAN_POINT ( 'NONE',  ( 0.1179895432987919934, 1424.305365874710105, 227.5542676486180085 ) ) ;
#3163=CARTESIAN_POINT ( 'NONE',  ( -6.550474571240000543, 1420.442131291729993, 231.7423262060979994 ) ) ;
#3168=CARTESIAN_POINT ( 'NONE',  ( 2.816976817413889833, 1488.404750540059922, 235.1213689463969843 ) ) ;
#3169=CARTESIAN_POINT ( 'NONE',  ( -24.04894046811064712, 1437.994949862434623, 211.5653030982465452 ) ) ;
#3171=CARTESIAN_POINT ( 'NONE',  ( -0.1980233633810000171, 1409.427787100730029, 233.0227887172979990 ) ) ;
#3172=CARTESIAN_POINT ( 'NONE',  ( -0.05438287574095269916, 1420.446865887249942, 182.6846654475669993 ) ) ;
#3183=ORIENTED_EDGE ( 'NONE', *, *, #94264, .T. ) ;
#3184=CARTESIAN_POINT ( 'NONE',  ( -0.1710941967680000009, 1506.802866821829866, 231.3049357514979931 ) ) ;
#3185=B_SPLINE_CURVE_WITH_KNOTS ( 'NONE', 5,
 ( #15559, #100143, #57065, #64360, #30728, #81128, #91190, #99024, #4446, #38573, #82238, #56502 ),
 .UNSPECIFIED., .F., .F.,
 ( 6, 3, 3, 6 ),
 ( 0.000000000000000000, 0.4244931604951553972, 0.5659654508551994478, 1.000000000000000000 ),
 .UNSPECIFIED. ) ;
#3190=CARTESIAN_POINT ( 'NONE',  ( -26.50966091029689764, 1508.705881461730087, 201.4781748968639761 ) ) ;
#3191=CARTESIAN_POINT ( 'NONE',  ( 19.39445793089999981, 1410.873186823329888, 196.0569557394979938 ) ) ;
#3192=FACE_OUTER_BOUND ( 'NONE', #35869, .T. ) ;
#3193=CARTESIAN_POINT ( 'NONE',  ( -17.73224984459999831, 1423.865196787429795, 226.2326530843979810 ) ) ;
#3194=CARTESIAN_POINT ( 'NONE',  ( -23.11088550610000070, 1435.448731366229822, 140.2466043785979934 ) ) ;
#3195=CARTESIAN_POINT ( 'NONE',  ( -4.906228319039999342, 1433.447543843880112, 150.0987928807979870 ) ) ;
#3197=CARTESIAN_POINT ( 'NONE',  ( 0.6901592941706589102, 1408.937161280970031, 231.9235919190410300 ) ) ;
#3198=CARTESIAN_POINT ( 'NONE',  ( -17.29007009959331143, 1433.653063861127976, 216.8064808204674421 ) ) ;
#3204=CARTESIAN_POINT ( 'NONE',  ( -23.95903483410000234, 1435.875769846390085, 211.1525007611679712 ) ) ;
#3206=CARTESIAN_POINT ( 'NONE',  ( -18.59896194139999892, 1509.326147591629933, 230.4813394039980210 ) ) ;
#3208=CARTESIAN_POINT ( 'NONE',  ( -17.33645362950000290, 1414.996442546130083, 207.8511177337479978 ) ) ;
#3213=FACE_OUTER_BOUND ( 'NONE', #87331, .T. ) ;
#3216=CARTESIAN_POINT ( 'NONE',  ( 20.60471804940000240, 1508.365513109829863, 189.9195030953979710 ) ) ;
#3221=ORIENTED_EDGE ( 'NONE', *, *, #85035, .T. ) ;
#3223=CARTESIAN_POINT ( 'NONE',  ( 27.68253994085160130, 1507.989615297080036, 207.6661388942010262 ) ) ;
#3225=CARTESIAN_POINT ( 'NONE',  ( 12.58542764725278396, 1442.782369552073305, 169.4702723407457370 ) ) ;
#3226=CARTESIAN_POINT ( 'NONE',  ( 33.74927008391222216, 1422.757720856681317, 269.5148346472382173 ) ) ;
#3227=CARTESIAN_POINT ( 'NONE',  ( 3.493530715499999673E-09, 1465.143864312329924, 238.2947549826980094 ) ) ;
#3228=CARTESIAN_POINT ( 'NONE',  ( -19.92516257929999668, 1505.117484763329912, 189.0508382488979748 ) ) ;
#3229=CARTESIAN_POINT ( 'NONE',  ( -11.37747002660000106, 1433.840278266459791, 151.4434446340980003 ) ) ;
#3230=CARTESIAN_POINT ( 'NONE',  ( 28.18475875730000269, 1509.897293851330005, 206.0721245515180158 ) ) ;
#3231=CARTESIAN_POINT ( 'NONE',  ( -19.57242333670000178, 1486.003043799229999, 190.0103911238980174 ) ) ;
#3232=CARTESIAN_POINT ( 'NONE',  ( 12.57381168289999884, 1409.852089639629867, 190.4288237261979759 ) ) ;
#3233=CARTESIAN_POINT ( 'NONE',  ( 5.138704292839999965, 1423.280612878629881, 185.3401477795979986 ) ) ;
#3234=CARTESIAN_POINT ( 'NONE',  ( -24.36523719230000040, 1440.927839248139890, 211.6868766829179833 ) ) ;
#3235=CARTESIAN_POINT ( 'NONE',  ( 6.070028637900000135, 1440.055554934649763, 154.5780772664979850 ) ) ;
#3236=DIRECTION ( 'NONE',  ( 1.000000000000000000, 0.000000000000000000, 0.000000000000000000 ) ) ;
#3238=CARTESIAN_POINT ( 'NONE',  ( -6.229759787779999947, 1452.550331331829966, 152.9826722968979880 ) ) ;
#3240=ORIENTED_EDGE ( 'NONE', *, *, #58344, .F. ) ;
#3243=VECTOR ( 'NONE', #20861, 1000.000000000000000 ) ;
#3245=CARTESIAN_POINT ( 'NONE',  ( -28.88176192769999773, 1466.008130076530051, 270.2667557415980468 ) ) ;
#3247=CARTESIAN_POINT ( 'NONE',  ( 7.549516567449999513E-15, 1441.600846913620217, 155.7224805731980268 ) ) ;
#3248=CARTESIAN_POINT ( 'NONE',  ( -22.60252397918324618, 1411.062741196104980, 211.6173965618407351 ) ) ;
#3249=B_SPLINE_CURVE_WITH_KNOTS ( 'NONE', 3,
 ( #35085, #45171, #87150, #51903, #79312, #36748, #70941, #77107, #78191, #93876 ),
 .UNSPECIFIED., .F., .F.,
 ( 4, 3, 3, 4 ),
 ( -157.4228417709999803, -134.4932908349400122, -78.88178533201940468, -29.50720979964130208 ),
 .UNSPECIFIED. ) ;
#3251=CARTESIAN_POINT ( 'NONE',  ( -13.27194800760000071, 1421.356218534429900, 229.3113483544979943 ) ) ;
#3254=CARTESIAN_POINT ( 'NONE',  ( -45.16571290676200334, 1435.656948718850117, 266.2028280709869819 ) ) ;
#3255=ORIENTED_EDGE ( 'NONE', *, *, #26901, .F. ) ;
#3257=ORIENTED_EDGE ( 'NONE', *, *, #89991, .F. ) ;
#3259=CYLINDRICAL_SURFACE ( 'NONE', #34042, 1.999999999999913181 ) ;
#3260=CIRCLE ( 'NONE', #56869, 1.999998625699862753 ) ;
#3262=CARTESIAN_POINT ( 'NONE',  ( -4.228066225910000142, 1425.410669922729767, 186.1178616580979792 ) ) ;
#3271=CARTESIAN_POINT ( 'NONE',  ( -12.98904541243399891, 1411.656893195809971, 269.6326585443520116 ) ) ;
#3273=CARTESIAN_POINT ( 'NONE',  ( 2.895864789156030294, 1417.780720963150088, 233.2805537130719813 ) ) ;
#3276=EDGE_LOOP ( 'NONE', ( #55028, #24641, #38474, #82690, #56008, #92096, #97428 ) ) ;
#3277=ORIENTED_EDGE ( 'NONE', *, *, #64427, .F. ) ;
#3278=CARTESIAN_POINT ( 'NONE',  ( 42.20684054510284255, 1453.921873302082531, 269.0702141739801618 ) ) ;
#3280=CARTESIAN_POINT ( 'NONE',  ( -10.71662182846777611, 1438.669127598729347, 152.4922056935914725 ) ) ;
#3282=CARTESIAN_POINT ( 'NONE',  ( -37.29571716481897425, 1420.414000716506052, 266.4271095758174965 ) ) ;
#3283=CARTESIAN_POINT ( 'NONE',  ( -13.36997666210000091, 1416.851343894929869, 221.9096085505980227 ) ) ;
#3284=CARTESIAN_POINT ( 'NONE',  ( 5.386772287290000349, 1432.443201990170110, 154.6097844173980036 ) ) ;
#3286=CARTESIAN_POINT ( 'NONE',  ( -14.35483098210000108, 1416.837177098929942, 221.5788728580980091 ) ) ;
#3287=CARTESIAN_POINT ( 'NONE',  ( 12.72965162820000096, 1416.819756528429934, 223.1305967425979873 ) ) ;
#3288=CARTESIAN_POINT ( 'NONE',  ( 8.781051467919999354, 1447.572322149110050, 186.1084250623979983 ) ) ;
#3292=CARTESIAN_POINT ( 'NONE',  ( 1.488643740577330066, 1472.261774644039861, 182.6335304928790038 ) ) ;
#3294=CARTESIAN_POINT ( 'NONE',  ( 6.928690003924570462, 1456.700621706041602, 227.7321335879927346 ) ) ;
#3295=CARTESIAN_POINT ( 'NONE',  ( -18.89942244622886491, 1416.835807149959237, 207.5749765851556674 ) ) ;
#3297=CARTESIAN_POINT ( 'NONE',  ( -15.29528072393560123, 1489.809333300280059, 194.3627042033380121 ) ) ;
#3300=CARTESIAN_POINT ( 'NONE',  ( 22.53878019769999952, 1411.058442714830107, 206.1986153634379946 ) ) ;
#3301=CARTESIAN_POINT ( 'NONE',  ( 18.43688931543651321, 1444.994950788469851, 161.6100378850028676 ) ) ;
#3302=CARTESIAN_POINT ( 'NONE',  ( 16.57803282680000123, 1409.491978020829947, 225.2035548608979809 ) ) ;
#3305=CARTESIAN_POINT ( 'NONE',  ( 0.9110504335954089372, 1450.859124385219957, 181.7304192028629757 ) ) ;
#3307=CIRCLE ( 'NONE', #64056, 26.99999999999999645 ) ;
#3314=CARTESIAN_POINT ( 'NONE',  ( -12.32904923379281392, 1414.913060387329779, 219.9538042439937726 ) ) ;
#3315=CIRCLE ( 'NONE', #58754, 2.000000000000075495 ) ;
#3317=( BOUNDED_CURVE ( )  B_SPLINE_CURVE ( 3, ( #53153, #105197, #11148, #87861 ),
 .UNSPECIFIED., .F., .F. ) 
 B_SPLINE_CURVE_WITH_KNOTS ( ( 4, 4 ),
 ( 1.916439914372829456, 2.295463455679393583 ),
 .UNSPECIFIED. ) 
 CURVE ( )  GEOMETRIC_REPRESENTATION_ITEM ( )  RATIONAL_B_SPLINE_CURVE ( ( 1.000000000000000000, 0.9880642163529229638, 0.9880642163529229638, 1.000000000000000000 ) ) 
 REPRESENTATION_ITEM ( '' )  );
#3318=CARTESIAN_POINT ( 'NONE',  ( -35.83299582265050276, 1450.078159482010051, 136.2400848972689857 ) ) ;
#3319=ADVANCED_FACE ( 'NONE', ( #22819, #101742 ), #68194, .T. ) ;
#3322=CARTESIAN_POINT ( 'NONE',  ( -7.553102827650000961, 1458.344558659830000, 234.3916895958979865 ) ) ;
#3323=CARTESIAN_POINT ( 'NONE',  ( -2.904356733534350088, 1464.880529238149848, 184.1795813031409921 ) ) ;
#3324=CARTESIAN_POINT ( 'NONE',  ( 11.85605537800000064, 1433.090874555759910, 150.3159297862979997 ) ) ;
#3325=CARTESIAN_POINT ( 'NONE',  ( -42.68574267046690096, 1451.691555868290152, 269.7334229991980123 ) ) ;
#3326=CARTESIAN_POINT ( 'NONE',  ( -17.98939368576640163, 1410.465184060849879, 195.2754043433779998 ) ) ;
#3330=ORIENTED_EDGE ( 'NONE', *, *, #90583, .T. ) ;
#3334=CARTESIAN_POINT ( 'NONE',  ( 8.491925884367525157, 1398.165181957728691, 199.2754951843434412 ) ) ;
#3335=CARTESIAN_POINT ( 'NONE',  ( 1.914485657349999981, 1482.804926797230110, 235.2460200716980125 ) ) ;
#3336=AXIS2_PLACEMENT_3D ( 'NONE', #42739, #25909, #50591 ) ;
#3338=CARTESIAN_POINT ( 'NONE',  ( -13.79885730810000055, 1508.398156089429904, 232.7146120173979966 ) ) ;
#3341=CARTESIAN_POINT ( 'NONE',  ( 2.499938418426329800, 1420.065636441539937, 97.17118231416419860 ) ) ;
#3343=CARTESIAN_POINT ( 'NONE',  ( 1.549411822890000234, 1466.670383311630076, 234.9066445244980059 ) ) ;
#3344=CARTESIAN_POINT ( 'NONE',  ( -41.65927775779999820, 1443.915297666309925, 135.6909731803980037 ) ) ;
#3346=CARTESIAN_POINT ( 'NONE',  ( -1.608997026699999777, 1450.560824856070212, 182.3064528867980130 ) ) ;
#3348=CARTESIAN_POINT ( 'NONE',  ( -5.401672965901620493, 1440.924418141449905, 154.8182599540220110 ) ) ;
#3355=CARTESIAN_POINT ( 'NONE',  ( -4.500000000000000000, 1411.429641636930000, 146.1721969590979882 ) ) ;
#3356=CARTESIAN_POINT ( 'NONE',  ( -11.86629848740000170, 1432.349867584279991, 149.9824238681979978 ) ) ;
#3358=CARTESIAN_POINT ( 'NONE',  ( 19.68017795844365381, 1509.620912528763256, 186.9948578458423469 ) ) ;
#3359=CARTESIAN_POINT ( 'NONE',  ( 14.51762396736629945, 1409.420026987000028, 212.6122462860219855 ) ) ;
#3366=EDGE_LOOP ( 'NONE', ( #41879, #9222, #17343, #38774, #60912 ) ) ;
#3368=CARTESIAN_POINT ( 'NONE',  ( -11.93592535262589927, 1415.651572961190141, 194.9902245485579897 ) ) ;
#3370=CARTESIAN_POINT ( 'NONE',  ( 16.41865139929206308, 1468.993348773691878, 269.3709366672832743 ) ) ;
#3373=CARTESIAN_POINT ( 'NONE',  ( -19.08184036181711818, 1486.257387795368004, 189.3980559289429664 ) ) ;
#3375=CARTESIAN_POINT ( 'NONE',  ( 2.890489020090289962, 1507.108937781499890, 235.9439513786750240 ) ) ;
#3378=CARTESIAN_POINT ( 'NONE',  ( -12.89606705209609849, 1434.724827189529833, 149.2205627886980039 ) ) ;
#3380=CARTESIAN_POINT ( 'NONE',  ( 0.5621803949210000262, 1416.843576337130116, 190.4753774197980078 ) ) ;
#3384=ORIENTED_EDGE ( 'NONE', *, *, #73344, .T. ) ;
#3387=CARTESIAN_POINT ( 'NONE',  ( -25.71796661899999847, 1449.805629481410051, 208.5932933947370032 ) ) ;
#3388=CARTESIAN_POINT ( 'NONE',  ( -10.34929248509440036, 1425.419910064279975, 92.74534805534860027 ) ) ;
#3389=CARTESIAN_POINT ( 'NONE',  ( -1.421471790896170040, 1507.619497854750080, 232.0556091900969875 ) ) ;
#3390=CARTESIAN_POINT ( 'NONE',  ( -1.875976467151887928, 1407.675044305313577, 270.1370780915658543 ) ) ;
#3391=CARTESIAN_POINT ( 'NONE',  ( -27.24390625379999875, 1427.221042094029826, 244.3119004031979955 ) ) ;
#3393=CARTESIAN_POINT ( 'NONE',  ( 1.149726251327802373, 1415.652443921420854, 233.0560295573103815 ) ) ;
#3394=CARTESIAN_POINT ( 'NONE',  ( 33.52142426879999704, 1450.454466855290093, 136.2569758902980084 ) ) ;
#3396=CARTESIAN_POINT ( 'NONE',  ( -0.07152548254896469448, 1397.597842456309991, 196.1220356218829863 ) ) ;
#3398=CARTESIAN_POINT ( 'NONE',  ( 5.994894223190000204, 1509.255434487730099, 238.7615784654979905 ) ) ;
#3400=VERTEX_POINT ( 'NONE', #50279 ) ;
#3404=CARTESIAN_POINT ( 'NONE',  ( 0.4901633952960000040, 1417.479174814430053, 184.7651825110980326 ) ) ;
#3406=CARTESIAN_POINT ( 'NONE',  ( 10.80134480061129842, 1446.564900598669965, 153.0805715986590201 ) ) ;
#3408=CARTESIAN_POINT ( 'NONE',  ( -1.478497299709999879, 1479.774927945029958, 235.9387637257979975 ) ) ;
#3409=CARTESIAN_POINT ( 'NONE',  ( 5.473890272918479738, 1440.659206135580007, 154.7842680422769774 ) ) ;
#3410=ORIENTED_EDGE ( 'NONE', *, *, #83296, .T. ) ;
#3411=CARTESIAN_POINT ( 'NONE',  ( 10.81515773970000005, 1424.921120067930133, 144.1684135303979986 ) ) ;
#3412=CARTESIAN_POINT ( 'NONE',  ( -12.82280136242419921, 1414.971993471370070, 220.5247844368900019 ) ) ;
#3413=B_SPLINE_CURVE_WITH_KNOTS ( 'NONE', 3,
 ( #73421, #105928, #29207, #99688, #65019, #107557, #63396, #81245, #39809, #97512, #82363, #108100, #90190, #89106, #22980, #57185, #54981, #46580, #80714, #4023, #72331, #106461, #29745, #63933, #98046, #21320, #55524, #4560, #38693, #72869, #30292, #25736, #15130, #6196, #50432, #102450, #40348, #31948, #42015, #57736, #7846, #58816, #48779, #58271, #75080, #83446, #108660, #59938, #41471, #24082, #42560, #91854, #94055, #7305, #109766, #74529, #24620, #66685, #33586, #23544, #15667, #75631, #66142, #100265, #8391, #92394, #49320, #82904, #34158, #6741, #59387, #40899, #25, #92955, #109230, #67779, #16228, #32514, #100791, #49871, #33046, #67234, #16769, #84005, #101330, #101891, #25184, #85102, #84557, #76164, #110311, #93498, #50972, #76713, #68344, #95723, #18431, #104120, #36915, #87895, #52631, #79487, #1131, #52081, #77282, #27408, #27967, #70006, #71109, #86768, #96278, #43671, #43123, #1682, #2795, #579, #35261, #61590, #26865, #61053, #18988, #60486, #11186, #77823 ),
 .UNSPECIFIED., .F., .F.,
 ( 4, 3, 3, 3, 3, 3, 3, 3, 3, 3, 3, 3, 3, 3, 3, 3, 3, 3, 3, 3, 3, 3, 3, 3, 3, 3, 3, 3, 3, 3, 3, 3, 3, 3, 3, 3, 3, 3, 3, 3, 3, 4 ),
 ( 1.527661073586570062E-12, 0.7233976231403740353, 1.453179569883080058, 2.189205328784380011, 2.931232241550089768, 3.681692766877309619, 4.436664690839419833, 5.195519430183240139, 5.957507373442520127, 6.722615321679190181, 7.488461883525279639, 8.253940120566859662, 8.872098166340000702, 9.627621989370730660, 10.37987637255229956, 11.12818954179939901, 11.87201083100580057, 12.60808579036049792, 13.25493342740159974, 13.90338778565579858, 14.62763214506709986, 14.71347576958129899, 15.43831616431399922, 16.16939285698139983, 16.92109434517130140, 17.66675291283500115, 18.41722696808670179, 19.17198454146360120, 19.93209661842169922, 20.69429497015770281, 21.45845625511120147, 22.18300476250000131, 22.94765126354310070, 23.71051285761900118, 24.46875717884919865, 25.22311653746220017, 25.97295705762990181, 26.71776956198449682, 27.45421737720040056, 28.18570414294039850, 28.90920563930189857, 29.42721171550000392 ),
 .UNSPECIFIED. ) ;
#3414=CARTESIAN_POINT ( 'NONE',  ( 14.23707600319999855, 1463.795787833229952, 224.1834224494979821 ) ) ;
#3415=ORIENTED_EDGE ( 'NONE', *, *, #94459, .T. ) ;
#3418=CARTESIAN_POINT ( 'NONE',  ( 11.86184899506429957, 1432.039039536349947, 149.9742464043579844 ) ) ;
#3419=CARTESIAN_POINT ( 'NONE',  ( 12.56175195062177607, 1445.048273880567194, 186.1342204703917673 ) ) ;
#3421=ORIENTED_EDGE ( 'NONE', *, *, #105523, .F. ) ;
#3423=CARTESIAN_POINT ( 'NONE',  ( -1.725662463192670248, 1484.236887848700007, 182.7463278875050037 ) ) ;
#3424=CARTESIAN_POINT ( 'NONE',  ( -20.70884933757140089, 1409.636229341499984, 202.4398936187430138 ) ) ;
#3426=CARTESIAN_POINT ( 'NONE',  ( 22.49191412916869837, 1452.127625438600035, 139.6794960788859896 ) ) ;
#3427=CARTESIAN_POINT ( 'NONE',  ( 3.113156245266410327, 1409.286500863440097, 270.3710781324699610 ) ) ;
#3430=CARTESIAN_POINT ( 'NONE',  ( -19.53035325068421812, 1509.611020418987209, 231.3334718708714206 ) ) ;
#3433=CARTESIAN_POINT ( 'NONE',  ( 16.04354243109999700, 1471.309244717529964, 194.9556777362979858 ) ) ;
#3435=CARTESIAN_POINT ( 'NONE',  ( 18.00557643216280113, 1423.829347998640060, 225.1846075778630052 ) ) ;
#3437=VERTEX_POINT ( 'NONE', #32357 ) ;
#3438=CARTESIAN_POINT ( 'NONE',  ( 8.518323188990001071, 1421.108130355529966, 243.9198229205979942 ) ) ;
#3439=CARTESIAN_POINT ( 'NONE',  ( 18.68654020979418817, 1509.565608750526735, 186.8439702850651543 ) ) ;
#3446=ORIENTED_EDGE ( 'NONE', *, *, #70043, .F. ) ;
#3449=AXIS2_PLACEMENT_3D ( 'NONE', #65561, #99672, #14721 ) ;
#3453=CARTESIAN_POINT ( 'NONE',  ( -7.375172166690000530, 1440.187291567539887, 186.1370477051980004 ) ) ;
#3454=CARTESIAN_POINT ( 'NONE',  ( 6.531016915288740066, 1509.181447638889949, 179.3779377418509853 ) ) ;
#3456=CARTESIAN_POINT ( 'NONE',  ( -7.215398911020000305, 1408.913060387329779, 225.6058586963979735 ) ) ;
#3457=CARTESIAN_POINT ( 'NONE',  ( 16.82235843289999977, 1415.092068029630127, 226.6094184117980319 ) ) ;
#3462=CARTESIAN_POINT ( 'NONE',  ( 44.15636045789999287, 1429.838460442230144, 267.0405866975980302 ) ) ;
#3463=CARTESIAN_POINT ( 'NONE',  ( -17.71696417089999898, 1409.531750409229971, 223.2909357272980060 ) ) ;
#3464=CARTESIAN_POINT ( 'NONE',  ( 17.33494591590000056, 1435.104201471239776, 146.4861191636979925 ) ) ;
#3466=CARTESIAN_POINT ( 'NONE',  ( 21.98314659799999760, 1488.582363539229846, 193.7203962354979865 ) ) ;
#3467=CARTESIAN_POINT ( 'NONE',  ( 29.71786509910646146, 1509.988056437398200, 208.1828936582288065 ) ) ;
#3470=CARTESIAN_POINT ( 'NONE',  ( -1.328227237909999969, 1475.823473844229966, 266.9604901357979543 ) ) ;
#3473=CARTESIAN_POINT ( 'NONE',  ( -10.00906774830520085, 1407.931115486439921, 200.5109140070470062 ) ) ;
#3475=CARTESIAN_POINT ( 'NONE',  ( -13.40958089250450058, 1414.996442620860080, 220.3303868550709694 ) ) ;
#3477=CARTESIAN_POINT ( 'NONE',  ( 13.80590739080000162, 1434.979616766929894, 146.7593012265980121 ) ) ;
#3478=CARTESIAN_POINT ( 'NONE',  ( 24.08426297012860218, 1411.115209414830133, 209.6325633951909708 ) ) ;
#3480=ORIENTED_EDGE ( 'NONE', *, *, #87025, .F. ) ;
#3482=CARTESIAN_POINT ( 'NONE',  ( -8.449237503979869501, 1409.208114262609797, 221.4678425924969929 ) ) ;
#3484=CARTESIAN_POINT ( 'NONE',  ( -5.370514330159649852, 1422.356910281434239, 139.1416123588654727 ) ) ;
#3485=CARTESIAN_POINT ( 'NONE',  ( -31.61404177300000029, 1466.402308574429981, 266.8259062747980010 ) ) ;
#3493=CARTESIAN_POINT ( 'NONE',  ( 21.92272425139999825, 1509.678618787829919, 227.7933223883979963 ) ) ;
#3494=CARTESIAN_POINT ( 'NONE',  ( 15.64624339340000070, 1506.809279343430035, 224.6411995677980258 ) ) ;
#3499=EDGE_CURVE ( 'NONE', #35766, #99633, #74407, .T. ) ;
#3500=DIRECTION ( 'NONE',  ( 1.000000000000000000, 0.000000000000000000, 0.000000000000000000 ) ) ;
#3506=EDGE_CURVE ( 'NONE', #83462, #77212, #56914, .T. ) ;
#3507=CARTESIAN_POINT ( 'NONE',  ( 23.35095090740000146, 1410.223686913330084, 211.6910680449280164 ) ) ;
#3508=CARTESIAN_POINT ( 'NONE',  ( -4.146782895030730387, 1426.018316030089863, 186.1121555109529879 ) ) ;
#3511=CARTESIAN_POINT ( 'NONE',  ( -15.63365311440000127, 1422.686384262629872, 229.4762402829979919 ) ) ;
#3512=CARTESIAN_POINT ( 'NONE',  ( -11.77676754959999883, 1432.864147235409973, 150.8103446100980136 ) ) ;
#3513=CARTESIAN_POINT ( 'NONE',  ( -11.72666526949699950, 1426.702413974029923, 143.4268556625789870 ) ) ;
#3514=CARTESIAN_POINT ( 'NONE',  ( -0.4957217136000000024, 1415.745301206330168, 233.4042774855979872 ) ) ;
#3515=CARTESIAN_POINT ( 'NONE',  ( 0.3803835583100000362, 1496.712195753129890, 230.6756913771979782 ) ) ;
#3520=CARTESIAN_POINT ( 'NONE',  ( 13.38995414329220068, 1507.947836362450062, 233.1180173837540224 ) ) ;
#3521=CARTESIAN_POINT ( 'NONE',  ( -16.30638770610000066, 1484.820604609629981, 187.8396872195979768 ) ) ;
#3526=ORIENTED_EDGE ( 'NONE', *, *, #49371, .T. ) ;
#3528=CARTESIAN_POINT ( 'NONE',  ( 28.32766665009999940, 1509.601337745830051, 212.4145138620280022 ) ) ;
#3529=ORIENTED_EDGE ( 'NONE', *, *, #6660, .F. ) ;
#3532=CARTESIAN_POINT ( 'NONE',  ( 15.76264809293400226, 1413.510787989959908, 191.4348339044099987 ) ) ;
#3533=CARTESIAN_POINT ( 'NONE',  ( 1.206391046180000037, 1508.614280349730052, 180.4667425254979776 ) ) ;
#3534=CARTESIAN_POINT ( 'NONE',  ( 11.86590139589999815, 1432.348266868109931, 151.0567667964980103 ) ) ;
#3535=EDGE_CURVE ( 'NONE', #75001, #94600, #101498, .T. ) ;
#3537=CARTESIAN_POINT ( 'NONE',  ( -25.15969574395609953, 1451.151030661709910, 137.5686878300720082 ) ) ;
#3539=CARTESIAN_POINT ( 'NONE',  ( 5.824346749060000050, 1409.620982476830022, 230.9132778911979926 ) ) ;
#3542=EDGE_CURVE ( 'NONE', #67049, #17568, #84135, .T. ) ;
#3543=CARTESIAN_POINT ( 'NONE',  ( 40.44958274758150196, 1439.458628678830109, 134.0999999981179940 ) ) ;
#3545=EDGE_LOOP ( 'NONE', ( #86504, #13255, #25222, #109789 ) ) ;
#3546=CARTESIAN_POINT ( 'NONE',  ( 0.1681681984989999989, 1420.473120458229914, 172.2701767054979882 ) ) ;
#3553=CARTESIAN_POINT ( 'NONE',  ( 13.46945357809454613, 1410.756328442758104, 228.3088036694626624 ) ) ;
#3555=CARTESIAN_POINT ( 'NONE',  ( 10.56616917823093793, 1451.302389960884284, 152.0481050481907630 ) ) ;
#3561=CARTESIAN_POINT ( 'NONE',  ( 4.237127598589969679, 1446.355009009640071, 163.3939598556469832 ) ) ;
#3562=CARTESIAN_POINT ( 'NONE',  ( 1.406911967200000113, 1508.853878877429906, 238.2247902776979913 ) ) ;
#3563=VERTEX_POINT ( 'NONE', #44074 ) ;
#3566=CARTESIAN_POINT ( 'NONE',  ( 31.14199524840240230, 1440.913060387330006, 254.3632966892320155 ) ) ;
#3567=CARTESIAN_POINT ( 'NONE',  ( -18.89418430779999980, 1508.334383760630089, 187.8348365672979980 ) ) ;
#3569=CARTESIAN_POINT ( 'NONE',  ( 25.71819509060329878, 1450.790613536419869, 136.8498688079899921 ) ) ;
#3570=CARTESIAN_POINT ( 'NONE',  ( -13.62085029079999998, 1409.388710960530034, 191.1271092111979897 ) ) ;
#3572=CARTESIAN_POINT ( 'NONE',  ( -24.90078896880000059, 1441.036975945570020, 210.4313365108079950 ) ) ;
#3574=CARTESIAN_POINT ( 'NONE',  ( 22.13036493270980287, 1410.097162861090055, 206.2644002183290013 ) ) ;
#3575=CARTESIAN_POINT ( 'NONE',  ( 0.0002637436312147029959, 1396.476788460397984, 196.7304488273350387 ) ) ;
#3577=CARTESIAN_POINT ( 'NONE',  ( -11.87502393270000134, 1433.007271228389982, 149.9804723947979994 ) ) ;
#3578=CARTESIAN_POINT ( 'NONE',  ( -14.56318188130000024, 1489.452917662129948, 192.4089202742979978 ) ) ;
#3579=CARTESIAN_POINT ( 'NONE',  ( -0.2272535083270984524, 1465.118792751454293, 238.1338994539894145 ) ) ;
#3580=CARTESIAN_POINT ( 'NONE',  ( 0.3086485800401259638, 1457.828016588880018, 228.9774103206889890 ) ) ;
#3581=AXIS2_PLACEMENT_3D ( 'NONE', #29767, #90773, #64504 ) ;
#3586=CARTESIAN_POINT ( 'NONE',  ( 2.189546061933858478, 1407.000065118299290, 222.1218459836267698 ) ) ;
#3591=ORIENTED_EDGE ( 'NONE', *, *, #5748, .T. ) ;
#3594=CARTESIAN_POINT ( 'NONE',  ( 28.09269446629999933, 1440.913060388880012, 231.9538848061980048 ) ) ;
#3595=CARTESIAN_POINT ( 'NONE',  ( -11.86652821809999914, 1432.377789890399981, 150.3970469068979980 ) ) ;
#3597=CARTESIAN_POINT ( 'NONE',  ( 1.797565579689999860, 1415.903556134429891, 232.4419632246980143 ) ) ;
#3600=FACE_OUTER_BOUND ( 'NONE', #27914, .T. ) ;
#3601=CARTESIAN_POINT ( 'NONE',  ( 19.01728017970000195, 1456.599257794629921, 225.8866418926980089 ) ) ;
#3602=CARTESIAN_POINT ( 'NONE',  ( -0.2331618352820000184, 1488.813684182529869, 187.9057016649980199 ) ) ;
#3606=CARTESIAN_POINT ( 'NONE',  ( 2.110812721519999879, 1405.784960767830171, 267.5353002013980017 ) ) ;
#3607=EDGE_CURVE ( 'NONE', #82900, #104987, #86066, .T. ) ;
#3609=B_SPLINE_CURVE_WITH_KNOTS ( 'NONE', 3,
 ( #106022, #37157, #89205, #11951, #10858, #80263, #81338, #13026, #61834, #12500 ),
 .UNSPECIFIED., .F., .F.,
 ( 4, 2, 2, 2, 4 ),
 ( 0.000000000000000000, 0.2500000000000000000, 0.5000000000000000000, 0.7500000000000000000, 1.000000000000000000 ),
 .UNSPECIFIED. ) ;
#3610=CARTESIAN_POINT ( 'NONE',  ( 38.08045545485799721, 1455.559130441839898, 269.8109766600500166 ) ) ;
#3611=DIRECTION ( 'NONE',  ( -0.7142107836478398530, 0.4827861023098918847, -0.5067746401878859830 ) ) ;
#3615=EDGE_CURVE ( 'NONE', #37055, #77021, #38719, .T. ) ;
#3616=DIRECTION ( 'NONE',  ( -0.7067707787425930865, 0.03085829008194152304, 0.7067692920952404201 ) ) ;
#3620=ORIENTED_EDGE ( 'NONE', *, *, #20513, .T. ) ;
#3622=CARTESIAN_POINT ( 'NONE',  ( -23.42675388609999843, 1440.913060387330006, 234.3916895593979746 ) ) ;
#3624=CARTESIAN_POINT ( 'NONE',  ( -0.2135896670159999899, 1475.319218785530211, 269.4986771182980192 ) ) ;
#3625=CARTESIAN_POINT ( 'NONE',  ( -4.254265649320910114, 1446.521173488880095, 160.4300573142469943 ) ) ;
#3627=CARTESIAN_POINT ( 'NONE',  ( -3.531993496884077377, 1448.289151893011649, 184.8902033554412299 ) ) ;
#3632=CARTESIAN_POINT ( 'NONE',  ( 26.48169467979350244, 1435.504490709530046, 135.8310255694130149 ) ) ;
#3633=EDGE_CURVE ( 'NONE', #32165, #85866, #104172, .T. ) ;
#3635=CARTESIAN_POINT ( 'NONE',  ( -11.00962827163180080, 1396.297525078389981, 210.2710635922789777 ) ) ;
#3636=EDGE_CURVE ( 'NONE', #72154, #74077, #29398, .T. ) ;
#3637=B_SPLINE_CURVE_WITH_KNOTS ( 'NONE', 3,
 ( #100646, #92259, #49179, #57031, #109620, #76561, #91158, #109081, #75486, #8239, #59237, #32362, #15529, #76012, #40205 ),
 .UNSPECIFIED., .F., .F.,
 ( 4, 2, 2, 1, 1, 1, 2, 2, 4 ),
 ( 0.000000000000000000, 0.2499999999999727440, 0.3749999999999591438, 0.4374999999999514277, 0.4687499999999488742, 0.4843749999999449329, 0.4921874999999458211, 0.4999999999999468203, 1.000000000000000000 ),
 .UNSPECIFIED. ) ;
#3638=CARTESIAN_POINT ( 'NONE',  ( -14.74910871950000057, 1422.312372933829920, 229.1172104516980141 ) ) ;
#3639=CARTESIAN_POINT ( 'NONE',  ( -44.78530908650000697, 1438.258924716540150, 269.6939408608980671 ) ) ;
#3642=FACE_OUTER_BOUND ( 'NONE', #105448, .T. ) ;
#3643=CARTESIAN_POINT ( 'NONE',  ( -11.76196280667599936, 1425.587142435169881, 146.3421825698729890 ) ) ;
#3644=CARTESIAN_POINT ( 'NONE',  ( 11.30143738019999944, 1426.878411159930010, 112.6515547669980037 ) ) ;
#3647=CARTESIAN_POINT ( 'NONE',  ( 4.285305835930380169, 1423.903434674070013, 183.8442863319299931 ) ) ;
#3653=CARTESIAN_POINT ( 'NONE',  ( 2.338461260499999916, 1507.140901839730077, 181.2734692156980145 ) ) ;
#3659=EDGE_LOOP ( 'NONE', ( #92733, #50325, #24117, #77022 ) ) ;
#3661=CARTESIAN_POINT ( 'NONE',  ( -6.170313909579999923, 1397.182081570829951, 197.8857380438980158 ) ) ;
#3662=CARTESIAN_POINT ( 'NONE',  ( -0.2817902298945799688, 1499.041747040399741, 236.9809926041430117 ) ) ;
#3663=CARTESIAN_POINT ( 'NONE',  ( 3.294994957250000134, 1408.913060387329779, 226.6118641217979928 ) ) ;
#3666=CARTESIAN_POINT ( 'NONE',  ( 11.71997758784366184, 1414.913060387329779, 198.0465748933708880 ) ) ;
#3668=CARTESIAN_POINT ( 'NONE',  ( 2.931305164040000300, 1429.770167287230151, 184.8385999854980071 ) ) ;
#3670=CARTESIAN_POINT ( 'NONE',  ( -41.65407651957470136, 1444.067054679140028, 136.1145617669420176 ) ) ;
#3671=CARTESIAN_POINT ( 'NONE',  ( -2.500000000000000000, 1448.203018870860205, 169.6830894382590031 ) ) ;
#3672=CARTESIAN_POINT ( 'NONE',  ( -12.89608512423069975, 1434.724840024559853, 149.2206170422699927 ) ) ;
#3673=CARTESIAN_POINT ( 'NONE',  ( 1.342110557989999897, 1416.822690122629865, 190.1636845438980004 ) ) ;
#3674=CARTESIAN_POINT ( 'NONE',  ( -3.827756660372859887, 1405.952650783709942, 267.2292680377810257 ) ) ;
#3678=CARTESIAN_POINT ( 'NONE',  ( 12.53124724090000086, 1441.827068648660088, 188.3849333394979908 ) ) ;
#3680=EDGE_CURVE ( 'NONE', #97278, #44414, #58766, .T. ) ;
#3688=CARTESIAN_POINT ( 'NONE',  ( -2.961869365206950100, 1509.113818662810218, 179.2106785136219855 ) ) ;
#3690=CARTESIAN_POINT ( 'NONE',  ( 18.20160569639999792, 1416.825421875629900, 213.0758509618380003 ) ) ;
#3696=CARTESIAN_POINT ( 'NONE',  ( -3.448199307399999913, 1409.033474160629794, 231.3476878950980051 ) ) ;
#3699=CARTESIAN_POINT ( 'NONE',  ( -14.59279134157089963, 1436.244781760590058, 149.8708244536879874 ) ) ;
#3701=CARTESIAN_POINT ( 'NONE',  ( 20.28308613678659711, 1497.601638836400070, 226.7150518706519904 ) ) ;
#3702=CARTESIAN_POINT ( 'NONE',  ( 16.61094140337936409, 1423.052547370200500, 227.3764671272628277 ) ) ;
#3703=CARTESIAN_POINT ( 'NONE',  ( 42.28239094362500339, 1436.755401113810194, 269.8809666808659813 ) ) ;
#3706=CARTESIAN_POINT ( 'NONE',  ( 23.55087631299999984, 1411.110694763729953, 207.7642880164279973 ) ) ;
#3709=CARTESIAN_POINT ( 'NONE',  ( -11.60004869885203682, 1422.586199384407792, 135.5999999980976440 ) ) ;
#3712=CARTESIAN_POINT ( 'NONE',  ( 4.299342307242959293, 1420.540376342569971, 185.6306603416350072 ) ) ;
#3713=CARTESIAN_POINT ( 'NONE',  ( -12.88074797900000057, 1417.902816224529943, 228.2418185653980061 ) ) ;
#3720=CARTESIAN_POINT ( 'NONE',  ( -24.91259172930000076, 1441.818365303380006, 210.4560922370480114 ) ) ;
#3721=CARTESIAN_POINT ( 'NONE',  ( -0.4274041271319999891, 1409.096031326030015, 232.6209024892979755 ) ) ;
#3722=CARTESIAN_POINT ( 'NONE',  ( 0.04366022373244289601, 1420.445819799160063, 182.6759295617300154 ) ) ;
#3723=ADVANCED_FACE ( 'NONE', ( #29457 ), #100025, .F. ) ;
#3734=DIRECTION ( 'NONE',  ( 1.988619772330852129E-13, 0.03085824620771311644, -0.9995237709234254808 ) ) ;
#3737=CARTESIAN_POINT ( 'NONE',  ( -27.30178126419649942, 1509.643183905199976, 201.1665203492270280 ) ) ;
#3739=EDGE_CURVE ( 'NONE', #68673, #108385, #26617, .T. ) ;
#3740=CARTESIAN_POINT ( 'NONE',  ( -3.116049926250000102, 1446.579647253840221, 167.4613962610980025 ) ) ;
#3742=CARTESIAN_POINT ( 'NONE',  ( -16.81191884579999751, 1435.084986459429956, 146.9484194988980050 ) ) ;
#3744=CARTESIAN_POINT ( 'NONE',  ( 18.35614473489999909, 1445.354571529839859, 191.3429017699980079 ) ) ;
#3746=CARTESIAN_POINT ( 'NONE',  ( -18.93441063164366511, 1438.881150600395131, 210.4529607928175494 ) ) ;
#3752=CARTESIAN_POINT ( 'NONE',  ( -10.73514660131351839, 1424.973046421745494, 139.1354236205272343 ) ) ;
#3753=CARTESIAN_POINT ( 'NONE',  ( -24.26965460479999948, 1437.030983368090119, 210.8923187080280002 ) ) ;
#3756=CARTESIAN_POINT ( 'NONE',  ( -2.500000000000000000, 1425.929641636930000, 184.1455913746980002 ) ) ;
#3757=CARTESIAN_POINT ( 'NONE',  ( 22.59376922909999763, 1497.713060387329961, 210.1004891184930159 ) ) ;
#3765=CARTESIAN_POINT ( 'NONE',  ( 21.59676349220000091, 1508.920392562430152, 190.9891518189980104 ) ) ;
#3772=CARTESIAN_POINT ( 'NONE',  ( 26.92641998615820143, 1490.346006921080061, 207.6803555114329924 ) ) ;
#3774=CARTESIAN_POINT ( 'NONE',  ( 12.75948692019158948, 1442.829946663825012, 169.4538695351947410 ) ) ;
#3775=CARTESIAN_POINT ( 'NONE',  ( 38.88871891119339352, 1429.342410219364410, 269.5910596282614051 ) ) ;
#3776=CARTESIAN_POINT ( 'NONE',  ( -31.95512683359999428, 1442.955673910089899, 244.1805851163980208 ) ) ;
#3779=CARTESIAN_POINT ( 'NONE',  ( -11.93261574969999828, 1433.458717525199972, 150.0079056965979873 ) ) ;
#3781=CARTESIAN_POINT ( 'NONE',  ( 26.86205050240000247, 1508.007394640929988, 206.2315947028279766 ) ) ;
#3782=CARTESIAN_POINT ( 'NONE',  ( -19.05388999639999881, 1486.255215324529900, 189.3722275761979859 ) ) ;
#3784=CARTESIAN_POINT ( 'NONE',  ( 13.86092680780000030, 1410.765486841630263, 191.1266656171980003 ) ) ;
#3785=CARTESIAN_POINT ( 'NONE',  ( 5.031515383899999527, 1423.012122006030040, 184.4169789091980078 ) ) ;
#3787=CARTESIAN_POINT ( 'NONE',  ( 16.95499469859999664, 1419.905063748630027, 226.7592642413980002 ) ) ;
#3789=AXIS2_PLACEMENT_3D ( 'NONE', #101960, #93560, #7368 ) ;
#3790=EDGE_CURVE ( 'NONE', #92672, #11723, #41367, .T. ) ;
#3792=CARTESIAN_POINT ( 'NONE',  ( 9.286020759454600352E-09, 1409.388281829009884, 259.9969200755350585 ) ) ;
#3795=CARTESIAN_POINT ( 'NONE',  ( -11.85886382813039930, 1431.831096394299948, 149.9589654793649913 ) ) ;
#3797=CARTESIAN_POINT ( 'NONE',  ( -10.46129436240000032, 1470.510090683430008, 269.3483239609980160 ) ) ;
#3799=FACE_OUTER_BOUND ( 'NONE', #95481, .T. ) ;
#3801=CARTESIAN_POINT ( 'NONE',  ( -15.32324661150000011, 1495.926233386129979, 224.3776978810979870 ) ) ;
#3802=CARTESIAN_POINT ( 'NONE',  ( 0.3404056040617879364, 1450.948218928229835, 181.6983794943430155 ) ) ;
#3806=CARTESIAN_POINT ( 'NONE',  ( -1.056358525591428288, 1484.867159798215653, 182.1438065072321137 ) ) ;
#3808=CARTESIAN_POINT ( 'NONE',  ( -44.63471219002420298, 1432.172276597919790, 266.7236482179810082 ) ) ;
#3810=CARTESIAN_POINT ( 'NONE',  ( -3.543446017492749789, 1501.284872974150176, 181.2258732813619986 ) ) ;
#3811=EDGE_CURVE ( 'NONE', #48668, #45663, #28011, .T. ) ;
#3815=AXIS2_PLACEMENT_3D ( 'NONE', #40082, #109501, #99974 ) ;
#3816=CARTESIAN_POINT ( 'NONE',  ( -17.22592475670000312, 1443.913060387330006, 162.9227486557980171 ) ) ;
#3818=CARTESIAN_POINT ( 'NONE',  ( -22.52564151099999989, 1509.699673122230024, 190.3321270482979912 ) ) ;
#3819=CARTESIAN_POINT ( 'NONE',  ( -14.69814578489999946, 1425.419041251630006, 189.8691658534980036 ) ) ;
#3828=CARTESIAN_POINT ( 'NONE',  ( -13.03876375938340004, 1411.451441007050107, 269.8787200598279696 ) ) ;
#3829=CARTESIAN_POINT ( 'NONE',  ( -1.554562095370000119, 1427.328278510630071, 123.0297916884979941 ) ) ;
#3832=ORIENTED_EDGE ( 'NONE', *, *, #55659, .F. ) ;
#3833=ORIENTED_EDGE ( 'NONE', *, *, #97972, .F. ) ;
#3834=CARTESIAN_POINT ( 'NONE',  ( 45.58493676572534525, 1442.547795422105082, 268.9761766335485618 ) ) ;
#3836=CARTESIAN_POINT ( 'NONE',  ( -14.45215659597139890, 1436.253647968190080, 149.9616404399920100 ) ) ;
#3837=CARTESIAN_POINT ( 'NONE',  ( -0.03623977524627750024, 1409.497123560340015, 185.3062518060349930 ) ) ;
#3839=CARTESIAN_POINT ( 'NONE',  ( -17.44754804248470137, 1415.007830321539814, 207.5653879932930295 ) ) ;
#3840=CARTESIAN_POINT ( 'NONE',  ( -18.30677928060000070, 1435.778268302339939, 226.2504290301980063 ) ) ;
#3841=CARTESIAN_POINT ( 'NONE',  ( 10.66852226406069981, 1475.487520392919805, 267.5060550787330271 ) ) ;
#3842=CARTESIAN_POINT ( 'NONE',  ( 11.75715125319999999, 1415.140114695929924, 222.5039781239979959 ) ) ;
#3843=CARTESIAN_POINT ( 'NONE',  ( -17.37005806175103473, 1422.637693141805130, 226.5733611387645965 ) ) ;
#3846=CARTESIAN_POINT ( 'NONE',  ( -38.81202640297369300, 1450.612734557460044, 135.6928040505150079 ) ) ;
#3847=CARTESIAN_POINT ( 'NONE',  ( -22.45016027724620855, 1451.714353191599685, 219.6156308778561765 ) ) ;
#3849=CARTESIAN_POINT ( 'NONE',  ( 0.2331202188386839735, 1408.921201124740037, 186.4825399812679905 ) ) ;
#3854=CARTESIAN_POINT ( 'NONE',  ( 19.12232319319999618, 1410.076634111130033, 195.9544771405979873 ) ) ;
#3855=CARTESIAN_POINT ( 'NONE',  ( 22.77810580590000100, 1410.208903622529988, 207.2750177385480015 ) ) ;
#3856=CARTESIAN_POINT ( 'NONE',  ( -23.80235451360000098, 1435.328707481769925, 136.9030858810979794 ) ) ;
#3858=CARTESIAN_POINT ( 'NONE',  ( 20.28305703155452733, 1455.773760547615893, 223.2321826931089106 ) ) ;
#3859=CARTESIAN_POINT ( 'NONE',  ( 2.500000000000000000, 1439.466623694439932, 162.9904177469239812 ) ) ;
#3864=CARTESIAN_POINT ( 'NONE',  ( -44.79032719779999638, 1444.249662561040168, 269.6864475883979821 ) ) ;
#3865=CARTESIAN_POINT ( 'NONE',  ( -11.22085813611739979, 1414.913060387329779, 220.6193216859199993 ) ) ;
#3867=CARTESIAN_POINT ( 'NONE',  ( -40.23101736414809437, 1444.600352321709806, 137.0308947161730089 ) ) ;
#3869=CARTESIAN_POINT ( 'NONE',  ( 11.60004869885203682, 1425.965608304797797, 137.6301247321180483 ) ) ;
#3870=CARTESIAN_POINT ( 'NONE',  ( -3.274920518576323377E-16, 1418.913060387330006, 172.2701767054979882 ) ) ;
#3871=CARTESIAN_POINT ( 'NONE',  ( 17.88228687367667646, 1423.788287748384391, 225.8724688183563671 ) ) ;
#3873=CARTESIAN_POINT ( 'NONE',  ( -44.01000096382649929, 1448.211628717079975, 269.7085006184129838 ) ) ;
#3877=ORIENTED_EDGE ( 'NONE', *, *, #58344, .T. ) ;
#3880=CIRCLE ( 'NONE', #57513, 1.999999999992389865 ) ;
#3882=CARTESIAN_POINT ( 'NONE',  ( -2.409586283469999923, 1426.663880916129983, 144.1938086916980239 ) ) ;
#3884=CARTESIAN_POINT ( 'NONE',  ( -14.53877746969999940, 1509.420765683830041, 233.9657681612980014 ) ) ;
#3887=CARTESIAN_POINT ( 'NONE',  ( 18.64672481363430379, 1416.851343896850040, 209.6839434896919840 ) ) ;
#3889=CARTESIAN_POINT ( 'NONE',  ( 1.358137423290000090, 1466.377668926530077, 235.0851387380980100 ) ) ;
#3891=ORIENTED_EDGE ( 'NONE', *, *, #55132, .T. ) ;
#3892=CARTESIAN_POINT ( 'NONE',  ( -0.9433386499399999403, 1452.411361074829983, 183.4747736275980117 ) ) ;
#3897=CARTESIAN_POINT ( 'NONE',  ( -18.34590453789999742, 1416.851343897030119, 208.8605687093670156 ) ) ;
#3900=ORIENTED_EDGE ( 'NONE', *, *, #100121, .F. ) ;
#3902=CARTESIAN_POINT ( 'NONE',  ( 11.74015320060000001, 1428.979986575930070, 144.1938086916980239 ) ) ;
#3903=FACE_OUTER_BOUND ( 'NONE', #75801, .T. ) ;
#3907=CARTESIAN_POINT ( 'NONE',  ( 14.85649457888519898, 1409.431860609890009, 210.6024228449819873 ) ) ;
#3908=FACE_OUTER_BOUND ( 'NONE', #1261, .T. ) ;
#3910=CARTESIAN_POINT ( 'NONE',  ( -18.11933796430000143, 1437.050887716040052, 191.5172096114979752 ) ) ;
#3912=CIRCLE ( 'NONE', #317, 20.12638776789572503 ) ;
#3915=ORIENTED_EDGE ( 'NONE', *, *, #80879, .T. ) ;
#3916=ORIENTED_EDGE ( 'NONE', *, *, #24375, .F. ) ;
#3920=CARTESIAN_POINT ( 'NONE',  ( 29.04422735952528356, 1509.932355432719078, 214.2352895502645822 ) ) ;
#3921=CARTESIAN_POINT ( 'NONE',  ( -20.18061928985329700, 1494.280760705760031, 190.7832826676969660 ) ) ;
#3927=CARTESIAN_POINT ( 'NONE',  ( -19.39871373709999958, 1468.954201919629895, 192.1830138438979816 ) ) ;
#3929=CARTESIAN_POINT ( 'NONE',  ( -13.16556780021149820, 1435.937898916229869, 150.6367019297510126 ) ) ;
#3933=CARTESIAN_POINT ( 'NONE',  ( 0.7132214971689999627, 1416.830000968330069, 190.3250594539979943 ) ) ;
#3937=CARTESIAN_POINT ( 'NONE',  ( 10.01186952689999821, 1415.800370255129792, 244.5548898179980029 ) ) ;
#3938=CARTESIAN_POINT ( 'NONE',  ( -21.52036872800000111, 1488.680653138530261, 194.1608577479979942 ) ) ;
#3939=CARTESIAN_POINT ( 'NONE',  ( -10.67517646397909914, 1425.711402707339857, 92.74368930566500069 ) ) ;
#3940=CARTESIAN_POINT ( 'NONE',  ( -16.99430611709999894, 1409.506514629130152, 195.5583755198979929 ) ) ;
#3943=CARTESIAN_POINT ( 'NONE',  ( -31.20802388730000132, 1430.369980854730102, 248.1710554681980057 ) ) ;
#3945=CARTESIAN_POINT ( 'NONE',  ( 2.595924361719925244, 1448.352474427002562, 154.6961829228227145 ) ) ;
#3946=CARTESIAN_POINT ( 'NONE',  ( -24.07938165869598635, 1410.986708706416493, 208.6133297288818653 ) ) ;
#3947=ORIENTED_EDGE ( 'NONE', *, *, #888, .T. ) ;
#3948=CARTESIAN_POINT ( 'NONE',  ( 3.433722984520000132, 1396.093883862429948, 197.4759704522980144 ) ) ;
#3952=ORIENTED_EDGE ( 'NONE', *, *, #50407, .F. ) ;
#3957=CARTESIAN_POINT ( 'NONE',  ( -1.083446969300000173, 1419.332833902230050, 184.9378854065980136 ) ) ;
#3959=CARTESIAN_POINT ( 'NONE',  ( -0.7728793615600000333, 1479.776535910530129, 236.0727651660979802 ) ) ;
#3961=ORIENTED_EDGE ( 'NONE', *, *, #103402, .F. ) ;
#3962=CARTESIAN_POINT ( 'NONE',  ( 11.15486294749999985, 1425.160588235329897, 144.1660541351980100 ) ) ;
#3963=CARTESIAN_POINT ( 'NONE',  ( -12.28605913130100014, 1415.088506334920112, 220.9685418577669793 ) ) ;
#3964=CARTESIAN_POINT ( 'NONE',  ( 15.25203479360000181, 1496.671131138630017, 225.4162514494980201 ) ) ;
#3966=( BOUNDED_CURVE ( )  B_SPLINE_CURVE ( 3, ( #54667, #63085, #97184, #80398 ),
 .UNSPECIFIED., .F., .F. ) 
 B_SPLINE_CURVE_WITH_KNOTS ( ( 4, 4 ),
 ( 2.226350983651550042, 2.864757500696315073 ),
 .UNSPECIFIED. ) 
 CURVE ( )  GEOMETRIC_REPRESENTATION_ITEM ( )  RATIONAL_B_SPLINE_CURVE ( ( 1.000000000000000000, 0.9663238299975769330, 0.9663238299975769330, 1.000000000000000000 ) ) 
 REPRESENTATION_ITEM ( '' )  );
#3969=CARTESIAN_POINT ( 'NONE',  ( 0.000000000000000000, 1408.913060387329779, 217.9908631324380224 ) ) ;
#3971=CARTESIAN_POINT ( 'NONE',  ( 13.50539683911128108, 1444.074071570348224, 187.9928544899986775 ) ) ;
#3972=ORIENTED_EDGE ( 'NONE', *, *, #93708, .T. ) ;
#3973=ORIENTED_EDGE ( 'NONE', *, *, #65486, .F. ) ;
#3976=CARTESIAN_POINT ( 'NONE',  ( -22.42121221859999736, 1409.696026370929985, 207.7819003571480039 ) ) ;
#3978=CARTESIAN_POINT ( 'NONE',  ( 14.98330790116689926, 1452.389831745899983, 147.8685068122100006 ) ) ;
#3983=CARTESIAN_POINT ( 'NONE',  ( 0.03647752878835780477, 1409.823935006122611, 233.1203796024890380 ) ) ;
#3986=CARTESIAN_POINT ( 'NONE',  ( -24.07281716570090069, 1508.277182899829995, 222.3373729421060148 ) ) ;
#3989=CARTESIAN_POINT ( 'NONE',  ( 3.804422481160000036, 1422.873164470030133, 234.3916895958979865 ) ) ;
#3990=CIRCLE ( 'NONE', #54111, 2.000000000000008882 ) ;
#3991=CARTESIAN_POINT ( 'NONE',  ( 41.66134420550000073, 1443.796851579070108, 135.6885409488979803 ) ) ;
#4002=CARTESIAN_POINT ( 'NONE',  ( 27.79924491104030082, 1510.012621779409983, 222.8077676732789882 ) ) ;
#4005=CARTESIAN_POINT ( 'NONE',  ( 9.414868078959999664, 1419.756125693529839, 230.5038554507980280 ) ) ;
#4009=CARTESIAN_POINT ( 'NONE',  ( 44.24543032989999602, 1429.800888227629912, 267.6618094214979919 ) ) ;
#4010=CARTESIAN_POINT ( 'NONE',  ( -18.02631345340000024, 1410.039226335029980, 224.3300098786980072 ) ) ;
#4011=CARTESIAN_POINT ( 'NONE',  ( 19.94495958220000276, 1435.193444768860218, 143.8622995873980130 ) ) ;
#4012=CARTESIAN_POINT ( 'NONE',  ( 21.33447918899999962, 1508.013007766330020, 191.0177302433980344 ) ) ;
#4013=CARTESIAN_POINT ( 'NONE',  ( 29.73445058744768588, 1509.991226363751821, 208.3164907507077714 ) ) ;
#4014=CARTESIAN_POINT ( 'NONE',  ( -26.93323766929999863, 1469.218382335129945, 266.6753116650979791 ) ) ;
#4016=CARTESIAN_POINT ( 'NONE',  ( -40.58566290280030131, 1442.151355276100048, 136.9330292898360142 ) ) ;
#4017=CARTESIAN_POINT ( 'NONE',  ( 0.2174939161106619889, 1453.161012291630186, 183.2464846872150304 ) ) ;
#4018=CARTESIAN_POINT ( 'NONE',  ( -15.29352652250000055, 1409.447122101729974, 207.7760784791980200 ) ) ;
#4023=CARTESIAN_POINT ( 'NONE',  ( -37.65468647916719647, 1436.753545005770093, 134.0999999968539953 ) ) ;
#4027=CARTESIAN_POINT ( 'NONE',  ( -4.185613592979979813, 1409.059225234809901, 223.5095492053650048 ) ) ;
#4030=CARTESIAN_POINT ( 'NONE',  ( 15.87566433304780311, 1507.597587122909999, 231.8003883547650048 ) ) ;
#4031=CARTESIAN_POINT ( 'NONE',  ( -27.10654211919999668, 1469.521092463829973, 267.5396841185980179 ) ) ;
#4033=CARTESIAN_POINT ( 'NONE',  ( 18.79734767819999774, 1416.844618642430078, 209.8348600039379903 ) ) ;
#4034=CARTESIAN_POINT ( 'NONE',  ( -27.50473206080000210, 1509.873546795530046, 216.5854941500080031 ) ) ;
#4038=CARTESIAN_POINT ( 'NONE',  ( 20.61567397870000207, 1508.364961461330040, 227.6869092844980003 ) ) ;
#4039=CARTESIAN_POINT ( 'NONE',  ( -27.28051563420000036, 1451.961389759230087, 135.3445407374979936 ) ) ;
#4040=CARTESIAN_POINT ( 'NONE',  ( 33.91369110979979951, 1435.681798629080049, 135.0664268281979901 ) ) ;
#4046=B_SPLINE_CURVE_WITH_KNOTS ( 'NONE', 3,
 ( #45936, #72249, #3393, #105842, #46498, #38072, #21231, #12861, #82820, #40821, #67152, #41388, #82278 ),
 .UNSPECIFIED., .F., .F.,
 ( 4, 2, 2, 1, 2, 2, 4 ),
 ( 0.000000000000000000, 0.2499999999998752664, 0.3749999999998002709, 0.4374999999998336331, 0.4687499999998503974, 0.4999999999998672173, 1.000000000000000000 ),
 .UNSPECIFIED. ) ;
#4048=CARTESIAN_POINT ( 'NONE',  ( -12.22173834910000068, 1416.311719782429918, 194.7110039421980048 ) ) ;
#4051=CARTESIAN_POINT ( 'NONE',  ( 22.29596073799999800, 1409.691652492829917, 210.9314411838980163 ) ) ;
#4054=CARTESIAN_POINT ( 'NONE',  ( -15.95047594089999876, 1421.629085502230055, 227.1824928441980092 ) ) ;
#4055=CARTESIAN_POINT ( 'NONE',  ( -11.87124624760000025, 1432.722071916729874, 149.9814472446979892 ) ) ;
#4057=CARTESIAN_POINT ( 'NONE',  ( 28.25140913253650155, 1508.152706006489780, 209.3868776241489797 ) ) ;
#4060=CARTESIAN_POINT ( 'NONE',  ( -22.99101922890000083, 1415.988654013429823, 211.3100808865079898 ) ) ;
#4061=B_SPLINE_CURVE_WITH_KNOTS ( 'NONE', 5,
 ( #8258, #49197, #100666, #42423, #101206, #42992, #17185, #109100, #84432, #16100, #77150, #68760, #15545, #110733, #67654, #34023, #454 ),
 .UNSPECIFIED., .F., .F.,
 ( 6, 2, 3, 3, 3, 6 ),
 ( 50.96205257140000100, 60.48206970939999394, 67.46372249629999374, 67.82259044730000141, 68.73290467190000186, 70.00206443017889058 ),
 .UNSPECIFIED. ) ;
#4064=CARTESIAN_POINT ( 'NONE',  ( -18.97892456421369900, 1485.957843142680076, 189.4647141020179788 ) ) ;
#4071=CARTESIAN_POINT ( 'NONE',  ( 28.28536618100000055, 1509.154939139430098, 210.5349106460980124 ) ) ;
#4072=ORIENTED_EDGE ( 'NONE', *, *, #106151, .T. ) ;
#4075=CARTESIAN_POINT ( 'NONE',  ( 15.77284072136830240, 1413.861949724670012, 191.4239925061509950 ) ) ;
#4076=CARTESIAN_POINT ( 'NONE',  ( 1.126797019860000137, 1507.655509662929717, 181.0315140402979921 ) ) ;
#4078=CARTESIAN_POINT ( 'NONE',  ( -23.91746435257450187, 1452.077846361179809, 136.8095616623199930 ) ) ;
#4079=CARTESIAN_POINT ( 'NONE',  ( 10.67939883587730066, 1438.711029782762353, 152.5177852837198600 ) ) ;
#4080=CARTESIAN_POINT ( 'NONE',  ( 5.754827835269999525, 1409.281567319030046, 230.5672434926979975 ) ) ;
#4082=( NAMED_UNIT ( * ) PLANE_ANGLE_UNIT ( ) SI_UNIT ( $, .RADIAN. ) );
#4084=CARTESIAN_POINT ( 'NONE',  ( 40.38917806159109603, 1448.047423120819985, 134.0999999983369833 ) ) ;
#4088=CARTESIAN_POINT ( 'NONE',  ( -16.02330256640034634, 1410.858424892926678, 226.7269707842006881 ) ) ;
#4089=VERTEX_POINT ( 'NONE', #17991 ) ;
#4090=ORIENTED_EDGE ( 'NONE', *, *, #91097, .F. ) ;
#4094=CARTESIAN_POINT ( 'NONE',  ( 15.15576445393604033, 1451.146651684196740, 149.6210827369275762 ) ) ;
#4097=LINE ( 'NONE', #37131, #3243 ) ;
#4100=CARTESIAN_POINT ( 'NONE',  ( -0.7397222527619999877, 1507.631725827129912, 231.9097525726980109 ) ) ;
#4101=CARTESIAN_POINT ( 'NONE',  ( 3.747720459029999951, 1415.426091369230107, 191.4590206283980081 ) ) ;
#4103=VERTEX_POINT ( 'NONE', #62253 ) ;
#4106=CARTESIAN_POINT ( 'NONE',  ( 23.86424463509850113, 1440.913060387330006, 235.1402480613069770 ) ) ;
#4108=EDGE_LOOP ( 'NONE', ( #11879, #6944, #90929, #2996 ) ) ;
#4110=CARTESIAN_POINT ( 'NONE',  ( -16.31417794970000301, 1410.855162238230150, 191.5236355156980039 ) ) ;
#4111=CARTESIAN_POINT ( 'NONE',  ( -22.75992825160000166, 1415.999881831630091, 212.0429175123080086 ) ) ;
#4112=CARTESIAN_POINT ( 'NONE',  ( -24.36543176699999691, 1441.018317148199912, 211.6908555921579875 ) ) ;
#4113=LINE ( 'NONE', #31338, #74209 ) ;
#4114=CARTESIAN_POINT ( 'NONE',  ( 22.53630099147500232, 1411.012929146719898, 206.1992209292300231 ) ) ;
#4115=CARTESIAN_POINT ( 'NONE',  ( -20.99191405665301247, 1509.583341913562435, 229.4942967042139799 ) ) ;
#4116=CARTESIAN_POINT ( 'NONE',  ( 23.58347146439999875, 1410.948704344629959, 266.7402917337980170 ) ) ;
#4119=CARTESIAN_POINT ( 'NONE',  ( 4.576117726849999734, 1464.329345424329858, 235.6418306423979914 ) ) ;
#4120=CARTESIAN_POINT ( 'NONE',  ( -11.60004869885203682, 1424.140773632030005, 136.0101406525482162 ) ) ;
#4122=CARTESIAN_POINT ( 'NONE',  ( -27.74152896854549866, 1446.393007474169963, 137.1637341980870133 ) ) ;
#4124=CARTESIAN_POINT ( 'NONE',  ( 19.22487415824295098, 1443.387065727409436, 213.3559128720396529 ) ) ;
#4126=EDGE_CURVE ( 'NONE', #68079, #18109, #30589, .T. ) ;
#4127=CARTESIAN_POINT ( 'NONE',  ( -18.05542495219999921, 1416.825784017130218, 209.4840452931509844 ) ) ;
#4132=CARTESIAN_POINT ( 'NONE',  ( 29.14244786389999931, 1446.680133728120154, 238.0755343184980006 ) ) ;
#4133=EDGE_CURVE ( 'NONE', #94093, #78014, #64274, .T. ) ;
#4137=CARTESIAN_POINT ( 'NONE',  ( 8.373664385848250902, 1414.913060387329779, 195.2168834859115236 ) ) ;
#4139=CARTESIAN_POINT ( 'NONE',  ( -21.42362349770000307, 1457.441058934229886, 222.6620133773979830 ) ) ;
#4140=CARTESIAN_POINT ( 'NONE',  ( 19.74164165809999716, 1455.376033653930108, 226.0788330262979855 ) ) ;
#4141=CARTESIAN_POINT ( 'NONE',  ( -2.793441807180000236, 1486.025323702830065, 182.0741001059980135 ) ) ;
#4144=CARTESIAN_POINT ( 'NONE',  ( 2.076955596959999983, 1406.811590412529995, 269.6487031941979922 ) ) ;
#4146=CARTESIAN_POINT ( 'NONE',  ( 42.89777864911530258, 1451.794179102650105, 270.1114872296610088 ) ) ;
#4147=DIRECTION ( 'NONE',  ( 0.000000000000000000, -1.000000000000000000, 0.000000000000000000 ) ) ;
#4148=CARTESIAN_POINT ( 'NONE',  ( -4.500000000000000000, 1411.429641636930000, 137.0999999980979851 ) ) ;
#4151=CARTESIAN_POINT ( 'NONE',  ( -1.612833274716345411, 1450.726624143510662, 183.2858275704341793 ) ) ;
#4152=CARTESIAN_POINT ( 'NONE',  ( 2.425481792534780023, 1449.557072643099900, 154.2478782046509878 ) ) ;
#4153=CARTESIAN_POINT ( 'NONE',  ( -14.44521984438740070, 1416.640375558069991, 221.3789857444529900 ) ) ;
#4154=CARTESIAN_POINT ( 'NONE',  ( 17.88677872281977344, 1428.781882675516044, 191.8785727744143799 ) ) ;
#4157=CARTESIAN_POINT ( 'NONE',  ( 5.773159728049999117E-15, 1422.873164470030133, 234.3916895801979763 ) ) ;
#4158=CARTESIAN_POINT ( 'NONE',  ( 2.500000000000000000, 1439.615672362369878, 170.5246407132979982 ) ) ;
#4159=CARTESIAN_POINT ( 'NONE',  ( -0.2158985180920000024, 1475.983168668529743, 267.2349487566980315 ) ) ;
#4160=CARTESIAN_POINT ( 'NONE',  ( -27.26775404520000023, 1451.960960096730105, 134.9110166487979825 ) ) ;
#4162=CARTESIAN_POINT ( 'NONE',  ( -2.981021339944338155, 1448.268954114771532, 184.4415419840244681 ) ) ;
#4166=CARTESIAN_POINT ( 'NONE',  ( -6.206590242792029422, 1396.129799296749752, 218.2548821234479988 ) ) ;
#4168=CARTESIAN_POINT ( 'NONE',  ( -45.63712941939999723, 1440.913060387330006, 268.9747522934979997 ) ) ;
#4172=CARTESIAN_POINT ( 'NONE',  ( 2.935740814629999917, 1409.954265555830034, 231.6094213276980156 ) ) ;
#4174=CARTESIAN_POINT ( 'NONE',  ( 11.03988486929999979, 1426.047781454529968, 101.9056521216979974 ) ) ;
#4176=CARTESIAN_POINT ( 'NONE',  ( -12.37499353609999986, 1445.063428794549964, 151.6327898328030130 ) ) ;
#4180=CARTESIAN_POINT ( 'NONE',  ( 2.641544985019999903, 1509.028982294729985, 179.6267714488979834 ) ) ;
#4187=CARTESIAN_POINT ( 'NONE',  ( -13.37869501641699621, 1446.597784270054717, 188.1529856935966336 ) ) ;
#4191=CARTESIAN_POINT ( 'NONE',  ( 8.486299124169999430, 1519.913060387329779, 230.6230627099979813 ) ) ;
#4195=CARTESIAN_POINT ( 'NONE',  ( 2.112541014579999654, 1410.305346947330008, 185.4714011601980133 ) ) ;
#4198=CARTESIAN_POINT ( 'NONE',  ( 41.01675760900570111, 1440.827364353530129, 136.2625528850119849 ) ) ;
#4199=CARTESIAN_POINT ( 'NONE',  ( 8.051433653212120234, 1396.194222647300194, 216.6959449344469988 ) ) ;
#4200=CARTESIAN_POINT ( 'NONE',  ( 1.546949757679999760, 1416.828040475729949, 190.2227908450980181 ) ) ;
#4201=CARTESIAN_POINT ( 'NONE',  ( 11.27689108819999930, 1430.486160747730082, 151.2803084875980062 ) ) ;
#4202=CYLINDRICAL_SURFACE ( 'NONE', #48337, 12.50000000000001066 ) ;
#4203=EDGE_LOOP ( 'NONE', ( #36861, #13976, #3900, #60788 ) ) ;
#4205=CARTESIAN_POINT ( 'NONE',  ( 12.60696393929999992, 1442.571107480210003, 187.6656753080980025 ) ) ;
#4207=VERTEX_POINT ( 'NONE', #99516 ) ;
#4210=CARTESIAN_POINT ( 'NONE',  ( -14.05757250470000130, 1460.648840866229875, 232.1449230562979835 ) ) ;
#4211=CARTESIAN_POINT ( 'NONE',  ( -15.56469051740000076, 1506.798305107229908, 193.1680121121979994 ) ) ;
#4212=EDGE_CURVE ( 'NONE', #87841, #64698, #103156, .T. ) ;
#4216=B_SPLINE_SURFACE_WITH_KNOTS ( 'NONE', 2, 5, ( 
 ( #29177, #20211, #54410, #97483, #88542, #52193 ),
 ( #86322, #9606, #77927, #95284, #86874, #20751 ),
 ( #31919, #106434, #22388, #106975, #89622, #66111 ) ),
 .UNSPECIFIED., .F., .F., .F.,
 ( 3, 3 ),
 ( 6, 6 ),
 ( 1.399803019379999958, 2.016961153080000013 ),
 ( 0.000000000000000000, 1.000000000000000000 ),
 .UNSPECIFIED. ) ;
#4218=CARTESIAN_POINT ( 'NONE',  ( -14.39828244561829962, 1509.511548947660003, 182.8869702195129889 ) ) ;
#4220=CARTESIAN_POINT ( 'NONE',  ( 2.628012963020000203, 1414.971287085229960, 225.5952605496979970 ) ) ;
#4224=CARTESIAN_POINT ( 'NONE',  ( -37.99384790316972982, 1427.843275130108395, 269.5760518878157086 ) ) ;
#4225=CARTESIAN_POINT ( 'NONE',  ( -2.903727783739999957, 1409.519113742730042, 232.3413682034979786 ) ) ;
#4226=CARTESIAN_POINT ( 'NONE',  ( -6.940379574320000522, 1431.113060387329824, 191.4151908640980082 ) ) ;
#4228=CARTESIAN_POINT ( 'NONE',  ( -0.01304059463119639981, 1452.815422809060010, 183.2381944397329789 ) ) ;
#4229=CARTESIAN_POINT ( 'NONE',  ( -31.46900625217390157, 1440.913060388669919, 242.6984041783090049 ) ) ;
#4232=EDGE_CURVE ( 'NONE', #101078, #99658, #20918, .T. ) ;
#4233=CARTESIAN_POINT ( 'NONE',  ( 43.48861604073940157, 1436.533985799180073, 270.3367144192989713 ) ) ;
#4236=CARTESIAN_POINT ( 'NONE',  ( 22.61598442209999860, 1409.702807929629898, 208.8472236539830078 ) ) ;
#4237=CARTESIAN_POINT ( 'NONE',  ( -7.738877702543442538, 1425.750511251113039, 225.8955623955143039 ) ) ;
#4242=CARTESIAN_POINT ( 'NONE',  ( 28.15443155984639745, 1509.896245780209938, 217.4026704617729990 ) ) ;
#4243=CARTESIAN_POINT ( 'NONE',  ( -8.414414886229998558, 1415.366749018530072, 230.7044676890980099 ) ) ;
#4250=EDGE_CURVE ( 'NONE', #21185, #25603, #101356, .T. ) ;
#4251=CARTESIAN_POINT ( 'NONE',  ( -20.32972594443840109, 1508.870366473410058, 229.0186719067029912 ) ) ;
#4252=CARTESIAN_POINT ( 'NONE',  ( -24.90010528315330163, 1441.007489120919900, 210.4306619437199970 ) ) ;
#4259=CARTESIAN_POINT ( 'NONE',  ( -25.82242192641380640, 1450.787213346408635, 136.8648991040845431 ) ) ;
#4261=ORIENTED_EDGE ( 'NONE', *, *, #105010, .F. ) ;
#4264=ORIENTED_EDGE ( 'NONE', *, *, #83036, .T. ) ;
#4273=CARTESIAN_POINT ( 'NONE',  ( -27.12205470637029947, 1509.520315501660207, 201.2360477619779999 ) ) ;
#4274=CARTESIAN_POINT ( 'NONE',  ( -3.115733350010000180, 1446.573609257150110, 168.9983159514980002 ) ) ;
#4275=CARTESIAN_POINT ( 'NONE',  ( -19.63221898369999963, 1426.793815849529892, 223.9042199868979992 ) ) ;
#4276=CARTESIAN_POINT ( 'NONE',  ( -24.00430195510000075, 1435.335597340879985, 137.4619936623980152 ) ) ;
#4278=CARTESIAN_POINT ( 'NONE',  ( 17.67025347690000103, 1478.544842878630106, 189.4270408572980102 ) ) ;
#4280=CARTESIAN_POINT ( 'NONE',  ( -18.93601566932215974, 1438.893878115886309, 210.4432051349708104 ) ) ;
#4281=ADVANCED_FACE ( 'NONE', ( #102821 ), #24028, .F. ) ;
#4291=CARTESIAN_POINT ( 'NONE',  ( -18.52446843519999931, 1509.559949079530043, 231.7134234805980100 ) ) ;
#4293=CARTESIAN_POINT ( 'NONE',  ( -12.90241536995782923, 1442.892915964137273, 186.4197113181899397 ) ) ;
#4294=CARTESIAN_POINT ( 'NONE',  ( -16.81223226430000039, 1414.913060387329779, 207.5743821216680089 ) ) ;
#4303=FACE_OUTER_BOUND ( 'NONE', #46274, .T. ) ;
#4309=CARTESIAN_POINT ( 'NONE',  ( 13.42980330897129271, 1443.474176595161225, 169.3652270005678133 ) ) ;
#4310=CARTESIAN_POINT ( 'NONE',  ( 28.45946923949786012, 1418.491042720496353, 269.4551673254863431 ) ) ;
#4311=CARTESIAN_POINT ( 'NONE',  ( -36.81312676959999663, 1443.228346179749906, 254.5659337120980013 ) ) ;
#4312=CARTESIAN_POINT ( 'NONE',  ( -20.32961525440000017, 1499.106861559730078, 190.3279599699980054 ) ) ;
#4313=CARTESIAN_POINT ( 'NONE',  ( -11.91439454699999878, 1433.379825245419852, 150.0311634427979754 ) ) ;
#4314=LINE ( 'NONE', #13774, #71436 ) ;
#4315=CARTESIAN_POINT ( 'NONE',  ( 11.63970458439030153, 1426.761200432619944, 137.2142808755380088 ) ) ;
#4316=CARTESIAN_POINT ( 'NONE',  ( -1.725662463192670248, 1484.236887848700007, 182.7463278875050037 ) ) ;
#4317=FACE_OUTER_BOUND ( 'NONE', #25471, .T. ) ;
#4319=CARTESIAN_POINT ( 'NONE',  ( 16.66094735743510213, 1410.867388111209948, 226.5061907891179942 ) ) ;
#4324=CARTESIAN_POINT ( 'NONE',  ( 1.482666866830270077E-09, 1410.677261243919929, 256.9622107588730273 ) ) ;
#4327=CARTESIAN_POINT ( 'NONE',  ( -11.86428414876309922, 1432.209070943210008, 149.9808888289879860 ) ) ;
#4330=CARTESIAN_POINT ( 'NONE',  ( -28.03279905679999828, 1464.673443976430008, 270.1137655723980515 ) ) ;
#4334=CARTESIAN_POINT ( 'NONE',  ( 0.2178157486290130118, 1452.982786607829894, 183.2541296479709843 ) ) ;
#4335=CARTESIAN_POINT ( 'NONE',  ( -12.29554385710000020, 1419.827449229430158, 228.7908442235979862 ) ) ;
#4339=CARTESIAN_POINT ( 'NONE',  ( -44.47864120876400307, 1432.224334038000052, 266.4559105170700377 ) ) ;
#4341=CARTESIAN_POINT ( 'NONE',  ( -3.538009167994560222, 1496.111029204799934, 181.4461849933530004 ) ) ;
#4342=CIRCLE ( 'NONE', #82972, 6.988489866870006395 ) ;
#4349=CARTESIAN_POINT ( 'NONE',  ( -8.015707256689999838, 1470.460698177329732, 184.9071038282980055 ) ) ;
#4351=LINE ( 'NONE', #91087, #37570 ) ;
#4352=B_SPLINE_SURFACE_WITH_KNOTS ( 'NONE', 5, 5, ( 
 ( #24216, #49997, #41596, #75751, #109897, #67367 ),
 ( #84678, #90883, #14170, #24753, #58950, #93082 ),
 ( #16355, #7976, #42144, #110445, #69581, #103698 ),
 ( #18565, #61188, #93619, #16897, #104255, #95305 ),
 ( #43796, #60622, #76852, #85228, #35955, #43254 ),
 ( #77401, #10188, #94183, #34835, #35392, #26998 ) ),
 .UNSPECIFIED., .F., .F., .F.,
 ( 6, 6 ),
 ( 6, 6 ),
 ( 5.770254232290000118, 6.424361107539999338 ),
 ( 0.000000000000000000, 2.000000000000000000 ),
 .UNSPECIFIED. ) ;
#4353=EDGE_LOOP ( 'NONE', ( #61123, #106543, #39984, #54937 ) ) ;
#4355=ADVANCED_FACE ( 'NONE', ( #57438 ), #32207, .T. ) ;
#4359=CARTESIAN_POINT ( 'NONE',  ( -26.95138969526639983, 1414.522592307069999, 270.1541509808739647 ) ) ;
#4360=CARTESIAN_POINT ( 'NONE',  ( 3.460649750935970381, 1417.553534582059910, 232.5463249240959840 ) ) ;
#4362=EDGE_CURVE ( 'NONE', #93315, #20179, #49242, .T. ) ;
#4364=ORIENTED_EDGE ( 'NONE', *, *, #57291, .F. ) ;
#4366=CARTESIAN_POINT ( 'NONE',  ( 45.62325630519739406, 1441.755915269380012, 268.9751291415536230 ) ) ;
#4368=CARTESIAN_POINT ( 'NONE',  ( -13.45539595447709935, 1436.151332559189996, 150.5285823830119796 ) ) ;
#4371=CARTESIAN_POINT ( 'NONE',  ( -18.49337492746660061, 1415.724942517919999, 207.5698429335219828 ) ) ;
#4372=CARTESIAN_POINT ( 'NONE',  ( -14.56134018280000042, 1420.166564076130044, 221.4975583820979921 ) ) ;
#4373=CARTESIAN_POINT ( 'NONE',  ( 11.53430538779999992, 1415.163755998629995, 222.8574940093980103 ) ) ;
#4376=VERTEX_POINT ( 'NONE', #6456 ) ;
#4380=CARTESIAN_POINT ( 'NONE',  ( -12.86122366611309964, 1416.830086716310007, 196.3807296669870084 ) ) ;
#4381=EDGE_LOOP ( 'NONE', ( #1303, #84850, #25958, #73510, #92359 ) ) ;
#4382=CARTESIAN_POINT ( 'NONE',  ( 7.356817058030821421, 1456.556113374074812, 227.5920619859562350 ) ) ;
#4384=CARTESIAN_POINT ( 'NONE',  ( 25.15894589063669784, 1451.153250808739813, 137.5682474387959928 ) ) ;
#4385=CARTESIAN_POINT ( 'NONE',  ( 13.29661090509999966, 1415.048591087029763, 197.5746719060980183 ) ) ;
#4387=CARTESIAN_POINT ( 'NONE',  ( 21.35641278199999959, 1409.658842758330138, 204.9228439656180285 ) ) ;
#4389=CARTESIAN_POINT ( 'NONE',  ( -4.220676207128734703, 1446.230049502166139, 170.5366217123670083 ) ) ;
#4390=CARTESIAN_POINT ( 'NONE',  ( -24.67107306660000177, 1435.359038600570102, 135.9357527513979846 ) ) ;
#4391=CARTESIAN_POINT ( 'NONE',  ( -24.00203106780000084, 1421.760869654530097, 210.4932335677079891 ) ) ;
#4393=CARTESIAN_POINT ( 'NONE',  ( 1.000433738244750126, 1452.575225918920069, 183.3871588569680284 ) ) ;
#4395=CARTESIAN_POINT ( 'NONE',  ( 2.500000000000000000, 1439.450741841849776, 162.6867541768519914 ) ) ;
#4402=FACE_OUTER_BOUND ( 'NONE', #81841, .T. ) ;
#4403=CARTESIAN_POINT ( 'NONE',  ( -38.26793863361420733, 1448.575033566829916, 136.4135971887010044 ) ) ;
#4404=CARTESIAN_POINT ( 'NONE',  ( 11.18796758460170615, 1425.276586956789288, 138.5633102189376018 ) ) ;
#4405=CARTESIAN_POINT ( 'NONE',  ( 2.567982850141544926, 1417.735512785670153, 233.8238498394635201 ) ) ;
#4406=CARTESIAN_POINT ( 'NONE',  ( -2.141398646916960136, 1471.330659375019877, 183.6643496123579951 ) ) ;
#4409=CARTESIAN_POINT ( 'NONE',  ( 36.09585466289570377, 1440.913060387229962, 253.0262047010989761 ) ) ;
#4413=EDGE_CURVE ( 'NONE', #43546, #93315, #18458, .T. ) ;
#4414=AXIS2_PLACEMENT_3D ( 'NONE', #92463, #60002, #33658 ) ;
#4418=CARTESIAN_POINT ( 'NONE',  ( 1.734605482469999904, 1474.701058102730030, 235.0720776984979921 ) ) ;
#4419=VECTOR ( 'NONE', #35940, 999.9999999999998863 ) ;
#4420=EDGE_CURVE ( 'NONE', #61381, #25667, #44294, .T. ) ;
#4422=CARTESIAN_POINT ( 'NONE',  ( -17.92485939079999824, 1509.539010270229937, 231.4769768637980007 ) ) ;
#4424=CARTESIAN_POINT ( 'NONE',  ( 21.03123203779729877, 1507.789098030329797, 226.0655639048319756 ) ) ;
#4425=CARTESIAN_POINT ( 'NONE',  ( 1.363639811660000145, 1415.765555525229956, 232.8698637559979829 ) ) ;
#4427=CARTESIAN_POINT ( 'NONE',  ( 1.586086858110000053, 1465.659878105630014, 235.1389441440979908 ) ) ;
#4430=CARTESIAN_POINT ( 'NONE',  ( -0.9209488051710000844, 1450.858101657689758, 181.8220196252979974 ) ) ;
#4439=CARTESIAN_POINT ( 'NONE',  ( -18.04214300190000131, 1416.520646107730045, 209.4829339742140064 ) ) ;
#4442=CARTESIAN_POINT ( 'NONE',  ( -18.11157280723839946, 1509.545530446499924, 231.7129765844609892 ) ) ;
#4443=CARTESIAN_POINT ( 'NONE',  ( 19.50214312291780416, 1509.609062993781436, 186.8947548611758407 ) ) ;
#4444=CARTESIAN_POINT ( 'NONE',  ( 12.10652582572050129, 1409.335829585050078, 200.3615976011700184 ) ) ;
#4445=FACE_OUTER_BOUND ( 'NONE', #2323, .T. ) ;
#4446=CARTESIAN_POINT ( 'NONE',  ( 1.506876827590000190, 1419.080345689929800, 184.9340756889980071 ) ) ;
#4447=CARTESIAN_POINT ( 'NONE',  ( 3995.588063464740117, 778.1435596157219834, 210.2211552457290225 ) ) ;
#4449=CARTESIAN_POINT ( 'NONE',  ( -2.647176844829699949, 1448.931638480319862, 183.9391811989769678 ) ) ;
#4450=EDGE_LOOP ( 'NONE', ( #106162, #109811, #97788, #44855 ) ) ;
#4455=CARTESIAN_POINT ( 'NONE',  ( -12.48153481890000016, 1434.603604361780071, 150.3555482973980020 ) ) ;
#4457=CARTESIAN_POINT ( 'NONE',  ( -20.45011936773050110, 1503.010088104919987, 190.5302468752080074 ) ) ;
#4460=CARTESIAN_POINT ( 'NONE',  ( -0.8791753874670000801, 1462.362773244929940, 182.9702177369979950 ) ) ;
#4463=CARTESIAN_POINT ( 'NONE',  ( -20.04223814320000230, 1488.365800429130104, 192.0903004145979764 ) ) ;
#4466=CARTESIAN_POINT ( 'NONE',  ( -11.93818408299999945, 1433.480074519959999, 149.8972116839979947 ) ) ;
#4467=CARTESIAN_POINT ( 'NONE',  ( -13.79088340914820066, 1435.084318818310066, 149.2846745635849857 ) ) ;
#4469=B_SPLINE_SURFACE_WITH_KNOTS ( 'NONE', 2, 5, ( 
 ( #30931, #5182, #32595, #55616, #13013, #81325 ),
 ( #73511, #65108, #99220, #22498, #59465, #76246 ),
 ( #93034, #17406, #77356, #84631, #114, #67316 ) ),
 .UNSPECIFIED., .F., .F., .F.,
 ( 3, 3 ),
 ( 6, 6 ),
 ( 1.399803019469999965, 2.016961153420000041 ),
 ( 0.000000000000000000, 1.000000000000000000 ),
 .UNSPECIFIED. ) ;
#4470=CARTESIAN_POINT ( 'NONE',  ( 0.7133821232520000111, 1416.822694190629818, 190.3253679279979735 ) ) ;
#4472=CARTESIAN_POINT ( 'NONE',  ( -16.46632221292249909, 1492.699621139769988, 229.6814607386230023 ) ) ;
#4473=ORIENTED_EDGE ( 'NONE', *, *, #96434, .T. ) ;
#4474=CARTESIAN_POINT ( 'NONE',  ( -2.034726938789999869E-09, 1411.425360646529953, 255.2684106118979912 ) ) ;
#4475=CARTESIAN_POINT ( 'NONE',  ( -27.39969416010000103, 1508.129222247830057, 204.7535242178479962 ) ) ;
#4476=CARTESIAN_POINT ( 'NONE',  ( -10.66340896497400159, 1425.717702253409925, 91.95185177473790361 ) ) ;
#4477=CARTESIAN_POINT ( 'NONE',  ( -1.514738108749209999, 1507.606285622480073, 232.0384771855580084 ) ) ;
#4478=CARTESIAN_POINT ( 'NONE',  ( -4.375890055962693204, 1407.803708330174459, 270.1335399949743987 ) ) ;
#4479=CARTESIAN_POINT ( 'NONE',  ( -20.03573726089999596, 1421.675448602630013, 240.3194873213979861 ) ) ;
#4481=CARTESIAN_POINT ( 'NONE',  ( -12.98226713004480004, 1414.913060387349788, 219.9156686614909972 ) ) ;
#4482=CARTESIAN_POINT ( 'NONE',  ( 28.25319277509999694, 1450.638438602809856, 136.4121326236979996 ) ) ;
#4483=ORIENTED_EDGE ( 'NONE', *, *, #87792, .F. ) ;
#4484=CARTESIAN_POINT ( 'NONE',  ( -0.006135675924780000130, 1395.974572295429880, 197.4936679463980056 ) ) ;
#4487=ORIENTED_EDGE ( 'NONE', *, *, #6990, .F. ) ;
#4491=CARTESIAN_POINT ( 'NONE',  ( -22.92752184622879952, 1409.723336632170231, 208.9617817198769671 ) ) ;
#4495=CARTESIAN_POINT ( 'NONE',  ( -4.707600842899999805, 1479.769858085930082, 235.1404652853979940 ) ) ;
#4498=CARTESIAN_POINT ( 'NONE',  ( 10.81509838440000060, 1424.921163249430037, 144.1641696251980136 ) ) ;
#4499=CARTESIAN_POINT ( 'NONE',  ( -13.15726445900019925, 1415.090956648730071, 220.8192894451659924 ) ) ;
#4500=CARTESIAN_POINT ( 'NONE',  ( 14.44508776610000034, 1485.704772158630021, 225.7184853347980038 ) ) ;
#4502=EDGE_LOOP ( 'NONE', ( #30495, #1703, #91330, #94161 ) ) ;
#4504=EDGE_CURVE ( 'NONE', #18765, #44739, #106843, .T. ) ;
#4505=DIRECTION ( 'NONE',  ( -0.1402804634174202869, 0.9901118076173992533, 0.000000000000000000 ) ) ;
#4509=EDGE_CURVE ( 'NONE', #26609, #67105, #69280, .T. ) ;
#4511=CARTESIAN_POINT ( 'NONE',  ( -22.51439127229999926, 1409.699280255230178, 208.1503399454410328 ) ) ;
#4513=CARTESIAN_POINT ( 'NONE',  ( 12.79875861287509942, 1452.466117888040117, 149.2463358307309989 ) ) ;
#4517=CARTESIAN_POINT ( 'NONE',  ( -18.70459388414779767, 1509.566239243649989, 231.7064163625079800 ) ) ;
#4518=DIRECTION ( 'NONE',  ( 0.000000000000000000, 1.000000000000000000, 0.000000000000000000 ) ) ;
#4519=CARTESIAN_POINT ( 'NONE',  ( -16.71917355490290191, 1412.654832539980134, 191.6875434529309814 ) ) ;
#4522=CARTESIAN_POINT ( 'NONE',  ( -24.02854066789229748, 1507.902906607559999, 222.3115874531950169 ) ) ;
#4525=CARTESIAN_POINT ( 'NONE',  ( 19.62446893450000118, 1438.771933937429822, 214.3676144197979738 ) ) ;
#4528=VECTOR ( 'NONE', #7696, 1000.000000000000000 ) ;
#4532=ORIENTED_EDGE ( 'NONE', *, *, #99080, .F. ) ;
#4535=CARTESIAN_POINT ( 'NONE',  ( -14.00886230499999918, 1416.826388551330183, 221.8518116138980076 ) ) ;
#4538=CARTESIAN_POINT ( 'NONE',  ( 1.047411759368620077, 1450.818007791970103, 181.4574043003410111 ) ) ;
#4540=CARTESIAN_POINT ( 'NONE',  ( -4.159508860199999880, 1408.913060387329779, 226.9541261483979895 ) ) ;
#4541=CARTESIAN_POINT ( 'NONE',  ( 4.446767511710000065, 1419.755698973330027, 231.8271342798979902 ) ) ;
#4544=CARTESIAN_POINT ( 'NONE',  ( 45.69700908059999733, 1436.916749176230041, 266.4179775685979621 ) ) ;
#4545=CARTESIAN_POINT ( 'NONE',  ( -18.78014126040000065, 1409.733562993129908, 222.2006764194979951 ) ) ;
#4546=ADVANCED_FACE ( 'NONE', ( #51214 ), #93203, .T. ) ;
#4547=CARTESIAN_POINT ( 'NONE',  ( 14.60160452979999945, 1435.005028509159956, 148.0399068081979976 ) ) ;
#4548=CARTESIAN_POINT ( 'NONE',  ( -0.7136739638169999900, 1418.680438739629835, 228.0000072166980090 ) ) ;
#4549=CARTESIAN_POINT ( 'NONE',  ( -16.10803554549259786, 1409.475565386449944, 193.1216181386560038 ) ) ;
#4550=CARTESIAN_POINT ( 'NONE',  ( 12.45685414969999805, 1416.832348306829999, 223.4765384881980026 ) ) ;
#4552=CARTESIAN_POINT ( 'NONE',  ( -40.49282606110470084, 1439.396725205129769, 135.6940988356820128 ) ) ;
#4554=CARTESIAN_POINT ( 'NONE',  ( 0.2139245209313919704, 1455.148420693890102, 183.1612303901350174 ) ) ;
#4555=CARTESIAN_POINT ( 'NONE',  ( -9.354904844460000035, 1409.239740863030192, 221.4829250259980142 ) ) ;
#4556=CARTESIAN_POINT ( 'NONE',  ( 2.382436964801011303, 1426.901689560120076, 137.0999999980980135 ) ) ;
#4558=CARTESIAN_POINT ( 'NONE',  ( -28.26636407291830011, 1509.425358601070229, 210.9265341182299949 ) ) ;
#4559=CARTESIAN_POINT ( 'NONE',  ( 13.50093264849999919, 1434.968966241960061, 149.0260858328979907 ) ) ;
#4560=CARTESIAN_POINT ( 'NONE',  ( -39.02661178205909920, 1437.758897876949959, 134.0999999974839909 ) ) ;
#4564=CARTESIAN_POINT ( 'NONE',  ( -6.087041179825980031, 1409.125624549270015, 222.8042030212700126 ) ) ;
#4568=CARTESIAN_POINT ( 'NONE',  ( 31.76117549946924612, 1416.371467029696760, 269.3206785931494665 ) ) ;
#4569=CARTESIAN_POINT ( 'NONE',  ( 19.70592387150000135, 1434.997135647629875, 210.0287612964809796 ) ) ;
#4574=CARTESIAN_POINT ( 'NONE',  ( -24.74145858110844642, 1444.127034557292745, 210.7303339034181988 ) ) ;
#4575=CARTESIAN_POINT ( 'NONE',  ( -27.01382318160000295, 1450.681613999719957, 136.4483333615980030 ) ) ;
#4580=VECTOR ( 'NONE', #40352, 999.9999999999998863 ) ;
#4581=CARTESIAN_POINT ( 'NONE',  ( 5.098960260437297443, 1422.101870575426801, 138.2838502392716862 ) ) ;
#4585=CARTESIAN_POINT ( 'NONE',  ( 0.003688949178799999940, 1466.041018883930064, 235.8553854185979901 ) ) ;
#4586=CARTESIAN_POINT ( 'NONE',  ( 21.08090099129999828, 1409.649221671529858, 214.5855264853080087 ) ) ;
#4590=CARTESIAN_POINT ( 'NONE',  ( -15.59773506849999869, 1422.361982635230106, 227.8242805376979732 ) ) ;
#4592=CARTESIAN_POINT ( 'NONE',  ( -11.73701141503820011, 1426.696005490819971, 144.1689084034089774 ) ) ;
#4596=CARTESIAN_POINT ( 'NONE',  ( -1.828265859660000103, 1416.270454245330029, 233.1889656714979822 ) ) ;
#4599=CARTESIAN_POINT ( 'NONE',  ( -10.40111706681060078, 1485.527135515960026, 184.6835754761009696 ) ) ;
#4605=ORIENTED_EDGE ( 'NONE', *, *, #8081, .T. ) ;
#4606=CARTESIAN_POINT ( 'NONE',  ( 28.08128577580000140, 1509.609363975330098, 213.5608712337979966 ) ) ;
#4609=CARTESIAN_POINT ( 'NONE',  ( 1.326919697849999968, 1414.988015876730060, 191.7691690367979902 ) ) ;
#4610=CARTESIAN_POINT ( 'NONE',  ( 15.79333902952730107, 1414.567926746569810, 191.4021969136939845 ) ) ;
#4611=CARTESIAN_POINT ( 'NONE',  ( 15.73512419572140075, 1409.471149252580062, 192.7531534643019882 ) ) ;
#4613=( BOUNDED_CURVE ( )  B_SPLINE_CURVE ( 3, ( #71939, #89242, #97646, #20915 ),
 .UNSPECIFIED., .F., .T. ) 
 B_SPLINE_CURVE_WITH_KNOTS ( ( 4, 4 ),
 ( 0.8490841261708470533, 1.097941757445210165 ),
 .UNSPECIFIED. ) 
 CURVE ( )  GEOMETRIC_REPRESENTATION_ITEM ( )  RATIONAL_B_SPLINE_CURVE ( ( 1.000000000000000000, 0.9948458117537219980, 0.9948458117537219980, 1.000000000000000000 ) ) 
 REPRESENTATION_ITEM ( '' )  );
#4614=CARTESIAN_POINT ( 'NONE',  ( -24.99671999555539870, 1451.592871286339914, 137.2106111822299965 ) ) ;
#4615=CARTESIAN_POINT ( 'NONE',  ( -11.63668813159999971, 1425.864839735429769, 144.1681848196979843 ) ) ;
#4616=CARTESIAN_POINT ( 'NONE',  ( 13.06456701529999975, 1409.369285120729955, 227.4078810651980120 ) ) ;
#4619=CARTESIAN_POINT ( 'NONE',  ( 41.25063694425699623, 1441.159963067259923, 134.0999999980680002 ) ) ;
#4620=AXIS2_PLACEMENT_3D ( 'NONE', #57541, #83814, #52323 ) ;
#4621=CARTESIAN_POINT ( 'NONE',  ( -40.14620926511650367, 1442.319073519450058, 136.9682662247859923 ) ) ;
#4622=ORIENTED_EDGE ( 'NONE', *, *, #51179, .T. ) ;
#4625=ORIENTED_EDGE ( 'NONE', *, *, #80622, .F. ) ;
#4628=CARTESIAN_POINT ( 'NONE',  ( -0.06979896196049999169, 1450.915497820830069, 181.2403767423980128 ) ) ;
#4633=CARTESIAN_POINT ( 'NONE',  ( 28.24318409530000196, 1508.132100788830030, 208.6373738428400202 ) ) ;
#4634=CARTESIAN_POINT ( 'NONE',  ( 3.236790408180000078, 1414.913060387329779, 192.7926995017980119 ) ) ;
#4641=CARTESIAN_POINT ( 'NONE',  ( 19.34500396569999836, 1467.214498603729908, 226.4572167402979801 ) ) ;
#4643=CARTESIAN_POINT ( 'NONE',  ( -0.4702569809430000025, 1450.896638651699959, 181.9239822119980090 ) ) ;
#4644=CARTESIAN_POINT ( 'NONE',  ( -16.23065921520000288, 1409.981629652129868, 191.7102031687979888 ) ) ;
#4646=CARTESIAN_POINT ( 'NONE',  ( -24.39257549919999946, 1441.120364142740073, 211.3418877072379871 ) ) ;
#4647=CARTESIAN_POINT ( 'NONE',  ( 22.52918858713469774, 1410.933109781309895, 206.2006944076529749 ) ) ;
#4649=CARTESIAN_POINT ( 'NONE',  ( 45.67178753498799182, 1438.934170743232244, 266.1885948232590522 ) ) ;
#4650=CARTESIAN_POINT ( 'NONE',  ( -13.19898084229999924, 1434.900407900599930, 147.1505653820979944 ) ) ;
#4652=CARTESIAN_POINT ( 'NONE',  ( 2.994687017620000447, 1464.609795535930061, 236.6065848807980103 ) ) ;
#4653=CARTESIAN_POINT ( 'NONE',  ( -11.60004869885203682, 1425.464090738186542, 136.9270719929736515 ) ) ;
#4656=CARTESIAN_POINT ( 'NONE',  ( -0.1235785668905619999, 1507.996910569370129, 180.6531142414899875 ) ) ;
#4660=AXIS2_PLACEMENT_3D ( 'NONE', #7664, #67596, #110128 ) ;
#4663=CARTESIAN_POINT ( 'NONE',  ( 0.000000000000000000, 1395.913060387330006, 201.1218459616980283 ) ) ;
#4666=CARTESIAN_POINT ( 'NONE',  ( 24.96471540929999833, 1444.223829899530074, 217.4975133951479904 ) ) ;
#4668=CARTESIAN_POINT ( 'NONE',  ( -11.30178248569999866, 1432.341675826490018, 151.5222233993980012 ) ) ;
#4671=CARTESIAN_POINT ( 'NONE',  ( 12.37689147640000087, 1445.074465208020001, 186.3522911324980100 ) ) ;
#4673=CARTESIAN_POINT ( 'NONE',  ( -23.87373140470000266, 1444.795516104289845, 213.3892174405480091 ) ) ;
#4674=CARTESIAN_POINT ( 'NONE',  ( 2.500000000000000000, 1432.287109468649987, 157.4934292187979850 ) ) ;
#4675=CARTESIAN_POINT ( 'NONE',  ( -2.950048403249999840, 1486.007024737429902, 182.1215898259980293 ) ) ;
#4676=ORIENTED_EDGE ( 'NONE', *, *, #55094, .F. ) ;
#4678=CARTESIAN_POINT ( 'NONE',  ( 0.8822908926409999131, 1406.271154717829859, 269.2944284930979961 ) ) ;
#4680=AXIS2_PLACEMENT_3D ( 'NONE', #79873, #11559, #20478 ) ;
#4681=CARTESIAN_POINT ( 'NONE',  ( 24.33107475527064167, 1437.296842069204786, 213.0379144650110845 ) ) ;
#4685=CARTESIAN_POINT ( 'NONE',  ( -0.8755637974877499285, 1450.882485025779943, 155.3353162938959997 ) ) ;
#4686=CARTESIAN_POINT ( 'NONE',  ( -1.699825449855114634, 1451.801988038905392, 184.1305289709272586 ) ) ;
#4687=CARTESIAN_POINT ( 'NONE',  ( -19.75226155591039401, 1486.000263447242787, 190.2095123751601022 ) ) ;
#4688=CARTESIAN_POINT ( 'NONE',  ( -14.17422268755229986, 1415.724942524879907, 221.1012049180340000 ) ) ;
#4689=LINE ( 'NONE', #73007, #76490 ) ;
#4690=CARTESIAN_POINT ( 'NONE',  ( -20.74408967690000338, 1436.077466332870017, 224.8635562271979893 ) ) ;
#4691=CARTESIAN_POINT ( 'NONE',  ( -26.86204968941349946, 1508.007394745769943, 212.0120970035400205 ) ) ;
#4692=CARTESIAN_POINT ( 'NONE',  ( 2.710683911340000307, 1440.403613791419957, 159.2736478902979798 ) ) ;
#4693=CARTESIAN_POINT ( 'NONE',  ( -3.744984048050000069, 1475.448291240629942, 269.2893923236980527 ) ) ;
#4695=DIRECTION ( 'NONE',  ( 0.000000000000000000, 1.000000000000000000, 0.000000000000000000 ) ) ;
#4697=DIRECTION ( 'NONE',  ( -0.9417419115949662300, -0.2378257470769920556, 0.2378257470769920556 ) ) ;
#4701=CARTESIAN_POINT ( 'NONE',  ( -5.283839841746620358, 1396.097576142400158, 218.8113393475669852 ) ) ;
#4702=CARTESIAN_POINT ( 'NONE',  ( -15.05376510940000045, 1421.406871761930233, 227.2858920301979992 ) ) ;
#4703=CARTESIAN_POINT ( 'NONE',  ( 19.47931728987103739, 1455.585788024227668, 225.7017591050554017 ) ) ;
#4705=DIRECTION ( 'NONE',  ( 0.9417419115949662300, -0.2378257470769920556, 0.2378257470769920556 ) ) ;
#4708=CARTESIAN_POINT ( 'NONE',  ( 10.97133660469999938, 1425.661190073130001, 112.6510004812979986 ) ) ;
#4710=CARTESIAN_POINT ( 'NONE',  ( -9286.692186988937465, 54.07981494722830718, 5933.209537134458515 ) ) ;
#4715=CARTESIAN_POINT ( 'NONE',  ( 5.458328288009999696, 1507.507604181929992, 182.0472652214980087 ) ) ;
#4716=CARTESIAN_POINT ( 'NONE',  ( -20.59684415639999955, 1507.762623716630060, 190.3921826403979765 ) ) ;
#4719=CARTESIAN_POINT ( 'NONE',  ( 16.99888975204404673, 1410.874132688714326, 191.9700510342732684 ) ) ;
#4721=ORIENTED_EDGE ( 'NONE', *, *, #51473, .T. ) ;
#4722=CARTESIAN_POINT ( 'NONE',  ( -12.08430580090000106, 1397.963661761730009, 203.2737820671979705 ) ) ;
#4723=CARTESIAN_POINT ( 'NONE',  ( 2.927202511967800014, 1410.063496054050120, 231.5773537391340255 ) ) ;
#4724=CARTESIAN_POINT ( 'NONE',  ( -1.383992982630000146, 1414.983773852929744, 226.4898643104980067 ) ) ;
#4725=CARTESIAN_POINT ( 'NONE',  ( 7.019973835868021340E-09, 1395.913060387101041, 220.3433455203826838 ) ) ;
#4726=CARTESIAN_POINT ( 'NONE',  ( -14.75025451881061755, 1435.013611857857086, 147.9283386685173411 ) ) ;
#4729=CARTESIAN_POINT ( 'NONE',  ( -1.357842376853849897, 1411.328796458540182, 185.5617438169070113 ) ) ;
#4733=CARTESIAN_POINT ( 'NONE',  ( 9.026700659202800736, 1396.228279763480032, 202.7331491456050117 ) ) ;
#4734=CARTESIAN_POINT ( 'NONE',  ( 0.5624690339869999889, 1416.828040475229955, 190.4759594386979984 ) ) ;
#4736=CARTESIAN_POINT ( 'NONE',  ( 41.65674243270000687, 1443.992462215730029, 135.6790809909979885 ) ) ;
#4737=VERTEX_POINT ( 'NONE', #58525 ) ;
#4739=CARTESIAN_POINT ( 'NONE',  ( 12.57940213210000024, 1442.756379237810052, 186.9445026950980093 ) ) ;
#4741=ORIENTED_EDGE ( 'NONE', *, *, #16575, .T. ) ;
#4749=ORIENTED_EDGE ( 'NONE', *, *, #61669, .T. ) ;
#4751=CARTESIAN_POINT ( 'NONE',  ( -2.948549143151390162, 1509.071337496469823, 179.3632791091939964 ) ) ;
#4753=CARTESIAN_POINT ( 'NONE',  ( 4.988721302020000081, 1414.971262582530017, 225.1457994249980175 ) ) ;
#4756=CARTESIAN_POINT ( 'NONE',  ( -20.84357928160000029, 1509.537325856430016, 229.6909426013980067 ) ) ;
#4757=CARTESIAN_POINT ( 'NONE',  ( -35.24250836817223842, 1424.318067564319335, 269.5348774294620284 ) ) ;
#4758=CARTESIAN_POINT ( 'NONE',  ( -0.5133638609530000174, 1410.311096994530089, 233.1717005261980091 ) ) ;
#4759=CARTESIAN_POINT ( 'NONE',  ( -8.099819236969999281, 1497.713060387329961, 188.5692696260980199 ) ) ;
#4760=ORIENTED_EDGE ( 'NONE', *, *, #92439, .F. ) ;
#4761=CARTESIAN_POINT ( 'NONE',  ( 2.500000000000000000, 1420.168334228329968, 149.0935893383980044 ) ) ;
#4762=CARTESIAN_POINT ( 'NONE',  ( -33.00779162925590526, 1440.913060389950033, 246.6090774808910169 ) ) ;
#4764=CARTESIAN_POINT ( 'NONE',  ( -0.2830760018822799928, 1465.096848926169969, 236.9997508814410025 ) ) ;
#4765=B_SPLINE_CURVE_WITH_KNOTS ( 'NONE', 3,
 ( #96116, #54697, #61443, #26696 ),
 .UNSPECIFIED., .F., .F.,
 ( 4, 4 ),
 ( -128.3330504390000044, -82.60381054909998966 ),
 .UNSPECIFIED. ) ;
#4766=CARTESIAN_POINT ( 'NONE',  ( 27.88456862112260026, 1417.385368265699753, 269.9356247533810347 ) ) ;
#4769=CARTESIAN_POINT ( 'NONE',  ( 23.53857934830000076, 1410.839771826630113, 207.7860714048179887 ) ) ;
#4771=CARTESIAN_POINT ( 'NONE',  ( -11.60004869885203682, 1425.691647225251245, 137.2114480028974413 ) ) ;
#4773=CARTESIAN_POINT ( 'NONE',  ( 4.240641006030480220, 1420.805731536519943, 185.5174961375570319 ) ) ;
#4774=CARTESIAN_POINT ( 'NONE',  ( -1.715370464160000052, 1415.379143890329942, 233.0965786315979926 ) ) ;
#4776=ORIENTED_EDGE ( 'NONE', *, *, #43168, .T. ) ;
#4784=CARTESIAN_POINT ( 'NONE',  ( -0.1681676274470000065, 1420.473121337229941, 182.7663689088979879 ) ) ;
#4786=CARTESIAN_POINT ( 'NONE',  ( 25.07506534592078395, 1507.939511209920283, 220.0842285648270718 ) ) ;
#4793=CARTESIAN_POINT ( 'NONE',  ( 0.000000000000000000, 1395.913060387330006, 201.1218459616980283 ) ) ;
#4794=CIRCLE ( 'NONE', #67414, 1.999999999999951594 ) ;
#4795=CARTESIAN_POINT ( 'NONE',  ( 20.94619202359999832, 1453.740811735230182, 222.3286468221979817 ) ) ;
#4796=CARTESIAN_POINT ( 'NONE',  ( 8.429635107905490088, 1437.624008729415664, 153.4535873770691126 ) ) ;
#4799=CARTESIAN_POINT ( 'NONE',  ( -28.15442856212169787, 1509.896234822020006, 200.8410265843269826 ) ) ;
#4800=CARTESIAN_POINT ( 'NONE',  ( -3.116758655539999534, 1446.591766556430002, 170.5446539902980021 ) ) ;
#4801=CARTESIAN_POINT ( 'NONE',  ( -18.94750420209999930, 1425.709852022430141, 224.6216987348980183 ) ) ;
#4802=CARTESIAN_POINT ( 'NONE',  ( -23.79554767710000007, 1435.472948733359999, 138.9787834592980005 ) ) ;
#4804=CARTESIAN_POINT ( 'NONE',  ( 15.46929474969999951, 1508.458304026830092, 186.6659617994979783 ) ) ;
#4805=CARTESIAN_POINT ( 'NONE',  ( 0.004826507542732910543, 1408.913229183870044, 232.2214716291990158 ) ) ;
#4806=CARTESIAN_POINT ( 'NONE',  ( 28.79939865120000064, 1509.589074241529943, 209.5214322619669929 ) ) ;
#4814=CARTESIAN_POINT ( 'NONE',  ( -12.29727565780000020, 1497.713060387329961, 227.1658498148980243 ) ) ;
#4817=CIRCLE ( 'NONE', #97849, 2.000055855578698250 ) ;
#4818=CARTESIAN_POINT ( 'NONE',  ( -12.86841135482259801, 1442.875644955115831, 186.3777548099945420 ) ) ;
#4819=CARTESIAN_POINT ( 'NONE',  ( 3.827327205999999649, 1416.243718512830128, 162.3415388335980083 ) ) ;
#4821=DIRECTION ( 'NONE',  ( 0.000000000000000000, 0.000000000000000000, -1.000000000000000000 ) ) ;
#4826=ORIENTED_EDGE ( 'NONE', *, *, #85308, .T. ) ;
#4827=B_SPLINE_CURVE_WITH_KNOTS ( 'NONE', 5,
 ( #71566, #97257, #53076, #1022, #87214, #10504 ),
 .UNSPECIFIED., .F., .F.,
 ( 6, 6 ),
 ( 0.000000000000000000, 1.000000000000000000 ),
 .UNSPECIFIED. ) ;
#4832=CARTESIAN_POINT ( 'NONE',  ( 18.07834331186310095, 1415.943166310999914, 209.4111036143110027 ) ) ;
#4835=CARTESIAN_POINT ( 'NONE',  ( 38.71733486712167860, 1429.045209714008251, 269.5881714454281450 ) ) ;
#4836=CARTESIAN_POINT ( 'NONE',  ( -5.301749019849999911, 1468.084175535429949, 248.5896189551980058 ) ) ;
#4837=CARTESIAN_POINT ( 'NONE',  ( -20.14880953469999980, 1505.117035552629886, 189.2730550177980149 ) ) ;
#4838=CARTESIAN_POINT ( 'NONE',  ( -11.89516891659999942, 1433.269307931430149, 149.9552190595979937 ) ) ;
#4840=CARTESIAN_POINT ( 'NONE',  ( 11.68956516707849858, 1426.727195071810002, 140.7743839025759769 ) ) ;
#4843=CARTESIAN_POINT ( 'NONE',  ( -25.58021156830000109, 1438.607539758289931, 137.7510881711980062 ) ) ;
#4844=CARTESIAN_POINT ( 'NONE',  ( -24.49620807289999647, 1440.956473104630049, 210.9946877109179866 ) ) ;
#4849=CARTESIAN_POINT ( 'NONE',  ( 5.854860788615310809E-11, 1411.443096976360039, 255.0304971312720284 ) ) ;
#4856=CARTESIAN_POINT ( 'NONE',  ( -19.98019444420000212, 1468.125272135429896, 269.6585770649980418 ) ) ;
#4857=CARTESIAN_POINT ( 'NONE',  ( -19.16951723229999871, 1456.627470220629903, 228.8719212425980061 ) ) ;
#4860=CARTESIAN_POINT ( 'NONE',  ( 0.2432523447182529941, 1451.431949927530013, 182.6146734826490103 ) ) ;
#4863=EDGE_CURVE ( 'NONE', #29539, #30233, #56757, .T. ) ;
#4864=CARTESIAN_POINT ( 'NONE',  ( -16.17567622148224871, 1459.146940454415244, 230.7169173019193806 ) ) ;
#4867=CARTESIAN_POINT ( 'NONE',  ( -43.33566613482280161, 1430.149811106979996, 269.0393173100790136 ) ) ;
#4870=ORIENTED_EDGE ( 'NONE', *, *, #37390, .F. ) ;
#4877=CARTESIAN_POINT ( 'NONE',  ( -2.780728806079999949, 1455.446097032029911, 184.5837736821980002 ) ) ;
#4878=VECTOR ( 'NONE', #9392, 1000.000000000000000 ) ;
#4879=CARTESIAN_POINT ( 'NONE',  ( -2.487880308650109118, 1449.152950345517183, 183.0833625634865029 ) ) ;
#4881=CARTESIAN_POINT ( 'NONE',  ( -26.80800901980000006, 1435.516554886219865, 135.8282728032980060 ) ) ;
#4882=ADVANCED_FACE ( 'NONE', ( #87017 ), #67009, .F. ) ;
#4887=CARTESIAN_POINT ( 'NONE',  ( -44.70567049325760678, 1435.628793295649984, 269.9105676632909763 ) ) ;
#4889=CARTESIAN_POINT ( 'NONE',  ( -1.233882608030000050, 1397.950738654029919, 196.1137546483980145 ) ) ;
#4891=ORIENTED_EDGE ( 'NONE', *, *, #57291, .T. ) ;
#4894=CARTESIAN_POINT ( 'NONE',  ( 45.63712937690380755, 1440.913060387330006, 268.9747523971630017 ) ) ;
#4897=CARTESIAN_POINT ( 'NONE',  ( -1.654395288670000186, 1485.634623599329871, 182.1583419804979940 ) ) ;
#4903=CARTESIAN_POINT ( 'NONE',  ( 12.54660221610000193, 1415.996778984329922, 223.0356910586980064 ) ) ;
#4905=ORIENTED_EDGE ( 'NONE', *, *, #45967, .T. ) ;
#4908=ORIENTED_EDGE ( 'NONE', *, *, #95207, .T. ) ;
#4909=CARTESIAN_POINT ( 'NONE',  ( -36.37832866295120482, 1451.642701157629745, 135.6928041510159915 ) ) ;
#4911=ORIENTED_EDGE ( 'NONE', *, *, #104138, .T. ) ;
#4912=CARTESIAN_POINT ( 'NONE',  ( 8.469983976807428760, 1456.145527513871912, 227.1991206335947595 ) ) ;
#4914=CARTESIAN_POINT ( 'NONE',  ( -4.090588468780437914, 1440.341105203780216, 185.3471663033907362 ) ) ;
#4916=CARTESIAN_POINT ( 'NONE',  ( 19.57944302010000115, 1410.092255016530089, 196.9053163625980005 ) ) ;
#4919=CARTESIAN_POINT ( 'NONE',  ( 24.51476220920747195, 1444.144828869601270, 213.4463787509066606 ) ) ;
#4921=SPHERICAL_SURFACE ( 'NONE', #19321, 2.000000000000000000 ) ;
#4923=VERTEX_POINT ( 'NONE', #73551 ) ;
#4926=CARTESIAN_POINT ( 'NONE',  ( -3.090336956749999864, 1448.965793307639842, 184.6975808967980015 ) ) ;
#4927=CARTESIAN_POINT ( 'NONE',  ( 0.3740406207303079711, 1452.976564550639978, 183.2744760995269928 ) ) ;
#4929=CARTESIAN_POINT ( 'NONE',  ( -40.26304726651319754, 1444.203404886970020, 137.0983463635160149 ) ) ;
#4932=CARTESIAN_POINT ( 'NONE',  ( 18.00000152313205248, 1424.173982496956569, 225.4517810533038471 ) ) ;
#4935=CARTESIAN_POINT ( 'NONE',  ( 36.96116112992849878, 1440.913060387089899, 254.5581055479269708 ) ) ;
#4942=ADVANCED_FACE ( 'NONE', ( #21986 ), #50009, .F. ) ;
#4944=CARTESIAN_POINT ( 'NONE',  ( -1.232506167737122516, 1409.632636740825774, 185.7525785795714341 ) ) ;
#4947=CARTESIAN_POINT ( 'NONE',  ( 15.06903345039999920, 1410.389868239730049, 191.5311856341979819 ) ) ;
#4952=CARTESIAN_POINT ( 'NONE',  ( 16.19492434978379691, 1409.478599607480191, 224.1775087544979783 ) ) ;
#4954=CARTESIAN_POINT ( 'NONE',  ( 2.281074820099999734, 1464.713448700129902, 235.8689246865980067 ) ) ;
#4956=ORIENTED_EDGE ( 'NONE', *, *, #72866, .T. ) ;
#4957=CARTESIAN_POINT ( 'NONE',  ( -0.6004483790419999911, 1452.607490234929855, 183.3312902083980021 ) ) ;
#4964=EDGE_LOOP ( 'NONE', ( #95945, #97531, #89699, #54523 ) ) ;
#4968=CARTESIAN_POINT ( 'NONE',  ( -11.60004869885203505, 1426.591398205465111, 134.9942363669703695 ) ) ;
#4971=VECTOR ( 'NONE', #79904, 1000.000000000000227 ) ;
#4972=CARTESIAN_POINT ( 'NONE',  ( 6.463161920097060253, 1409.138758974899929, 195.6150904016829770 ) ) ;
#4973=DIRECTION ( 'NONE',  ( -4.137698748469999823E-18, -2.750577543510000101E-14, -1.000000000000000000 ) ) ;
#4980=EDGE_CURVE ( 'NONE', #42879, #48892, #80009, .T. ) ;
#4982=CARTESIAN_POINT ( 'NONE',  ( -12.12507211471189805, 1416.051481378869994, 194.8051867232880170 ) ) ;
#4983=CARTESIAN_POINT ( 'NONE',  ( -11.84681311729999820, 1434.711927244070012, 151.1872562620980034 ) ) ;
#4985=CARTESIAN_POINT ( 'NONE',  ( -8.184993690210469467E-10, 1468.121328536410147, 248.6278164530129970 ) ) ;
#4986=CARTESIAN_POINT ( 'NONE',  ( -20.15323670362180053, 1493.393816397240016, 190.8089475466459817 ) ) ;
#4989=CARTESIAN_POINT ( 'NONE',  ( 0.1648048234879999907, 1483.385634709730084, 181.9489519295979676 ) ) ;
#4991=CARTESIAN_POINT ( 'NONE',  ( -45.88148358874209976, 1440.468640267019964, 266.4123968719909499 ) ) ;
#4992=CARTESIAN_POINT ( 'NONE',  ( 13.92249237623939884, 1452.656259886599855, 223.1400375642430163 ) ) ;
#4999=CARTESIAN_POINT ( 'NONE',  ( -13.52518119320440171, 1435.051496296169944, 149.4677306140820008 ) ) ;
#5003=EDGE_CURVE ( 'NONE', #34701, #14678, #26360, .T. ) ;
#5005=CARTESIAN_POINT ( 'NONE',  ( 32.79493994350000463, 1434.501496568570019, 248.1152222124979971 ) ) ;
#5007=CARTESIAN_POINT ( 'NONE',  ( -2.484903766530000002, 1458.411121269429941, 182.9125316254979907 ) ) ;
#5008=CARTESIAN_POINT ( 'NONE',  ( -1.325823302270159987, 1507.620489792419903, 232.0621709551870140 ) ) ;
#5009=CARTESIAN_POINT ( 'NONE',  ( 21.91250632045888125, 1506.380977038693800, 207.4373042671960548 ) ) ;
#5010=CARTESIAN_POINT ( 'NONE',  ( -3.773954403609999897, 1421.529510570530192, 216.2239751100380261 ) ) ;
#5012=CARTESIAN_POINT ( 'NONE',  ( -4.967560240179940578, 1452.739589361249955, 152.0866475748709945 ) ) ;
#5013=CARTESIAN_POINT ( 'NONE',  ( -18.95839814150000180, 1416.827520077830059, 207.7798181853180211 ) ) ;
#5014=VERTEX_POINT ( 'NONE', #91978 ) ;
#5016=DIRECTION ( 'NONE',  ( -1.000000000000000000, 0.000000000000000000, 0.000000000000000000 ) ) ;
#5018=ORIENTED_EDGE ( 'NONE', *, *, #103442, .T. ) ;
#5020=EDGE_CURVE ( 'NONE', #101781, #28929, #94173, .T. ) ;
#5023=ORIENTED_EDGE ( 'NONE', *, *, #28403, .F. ) ;
#5029=CARTESIAN_POINT ( 'NONE',  ( -6.753454085369999582, 1489.056761658230016, 234.9017483617980133 ) ) ;
#5031=ORIENTED_EDGE ( 'NONE', *, *, #64741, .T. ) ;
#5033=CARTESIAN_POINT ( 'NONE',  ( 45.63691652665460197, 1441.836777326350102, 268.9749693829069770 ) ) ;
#5034=CARTESIAN_POINT ( 'NONE',  ( -12.73594778875919964, 1416.524489948229984, 221.9712528552830122 ) ) ;
#5035=CARTESIAN_POINT ( 'NONE',  ( 0.05678182167189999713, 1418.511462927230014, 184.6660934127980340 ) ) ;
#5039=CARTESIAN_POINT ( 'NONE',  ( 12.91984442206437578, 1442.902292219558149, 187.0613185807262084 ) ) ;
#5041=ORIENTED_EDGE ( 'NONE', *, *, #63813, .F. ) ;
#5044=CARTESIAN_POINT ( 'NONE',  ( 12.89273669479999995, 1508.859229393329997, 233.8778408584979900 ) ) ;
#5046=CARTESIAN_POINT ( 'NONE',  ( 21.41738597313630166, 1452.165148788659963, 141.3889158671639734 ) ) ;
#5050=CARTESIAN_POINT ( 'NONE',  ( -18.95791602736232306, 1509.575124649889176, 231.6168982108185901 ) ) ;
#5051=CARTESIAN_POINT ( 'NONE',  ( 0.02347612988675716952, 1409.045439741765676, 232.3809737551641774 ) ) ;
#5052=CARTESIAN_POINT ( 'NONE',  ( -16.83010722181489882, 1416.063878291570290, 191.5921218490719866 ) ) ;
#5053=CARTESIAN_POINT ( 'NONE',  ( 17.01808896600000054, 1507.624369720630057, 193.6805215186979865 ) ) ;
#5056=CARTESIAN_POINT ( 'NONE',  ( -25.38913556476300215, 1509.752285549599947, 222.9524089379939653 ) ) ;
#5067=CARTESIAN_POINT ( 'NONE',  ( -1.639582970820000041, 1434.541746329560056, 150.4377894671980016 ) ) ;
#5074=CARTESIAN_POINT ( 'NONE',  ( 2.938302457570000303, 1419.757091722530049, 232.0470454606980013 ) ) ;
#5076=CARTESIAN_POINT ( 'NONE',  ( -3.469833849039999683E-16, 1426.566393376330097, 144.1938086916980239 ) ) ;
#5077=CARTESIAN_POINT ( 'NONE',  ( 10.80134480061119895, 1441.261220175989820, 153.0805715986579969 ) ) ;
#5078=CARTESIAN_POINT ( 'NONE',  ( -18.59938032009999986, 1409.727296728430019, 222.5591327112979911 ) ) ;
#5080=CARTESIAN_POINT ( 'NONE',  ( 20.59733728950000042, 1508.015129919730043, 189.9429528794979944 ) ) ;
#5086=CARTESIAN_POINT ( 'NONE',  ( -6.194271847559999600, 1415.931669658129977, 226.1787850318980020 ) ) ;
#5087=CARTESIAN_POINT ( 'NONE',  ( 0.2104582539746929770, 1457.090827936239975, 183.0778992351330032 ) ) ;
#5088=CARTESIAN_POINT ( 'NONE',  ( -9.160204422789998802, 1409.232941774529991, 221.2278796158979901 ) ) ;
#5091=ADVANCED_FACE ( 'NONE', ( #92518 ), #32995, .F. ) ;
#5093=CARTESIAN_POINT ( 'NONE',  ( 11.87527449220000086, 1433.007027006299950, 149.0256347040979961 ) ) ;
#5094=DIRECTION ( 'NONE',  ( 0.9536973727975270876, 0.1200132783607290032, -0.2757863922244979671 ) ) ;
#5095=CARTESIAN_POINT ( 'NONE',  ( 11.97824860639999933, 1442.481624454889925, 187.4134949571979973 ) ) ;
#5099=CARTESIAN_POINT ( 'NONE',  ( -10.35541825330239973, 1409.274679561159928, 219.9120658599189824 ) ) ;
#5101=CARTESIAN_POINT ( 'NONE',  ( -15.41079858738659958, 1501.813619937609928, 192.8668813100890134 ) ) ;
#5102=CARTESIAN_POINT ( 'NONE',  ( 43.55237166414823236, 1430.623344126982829, 269.0332385863825948 ) ) ;
#5104=CARTESIAN_POINT ( 'NONE',  ( -19.62842490763629399, 1495.540557520950642, 189.3275510559486179 ) ) ;
#5111=CARTESIAN_POINT ( 'NONE',  ( -27.54194134069999933, 1451.798912744530071, 135.7745631451980159 ) ) ;
#5113=CARTESIAN_POINT ( 'NONE',  ( -15.91558000873799905, 1409.468827912599863, 225.2516522794149978 ) ) ;
#5114=CARTESIAN_POINT ( 'NONE',  ( 0.5122327485485929088, 1410.651863534059885, 185.0574092668310016 ) ) ;
#5116=CARTESIAN_POINT ( 'NONE',  ( -9.845241469799999479, 1507.507259092430104, 182.3675330799979974 ) ) ;
#5123=CARTESIAN_POINT ( 'NONE',  ( 22.68241477640000170, 1411.065318295730094, 214.3862589840079806 ) ) ;
#5124=CARTESIAN_POINT ( 'NONE',  ( -1.984486858693230493, 1410.354035999710050, 186.2309706543619825 ) ) ;
#5128=CARTESIAN_POINT ( 'NONE',  ( 16.19188814560000012, 1409.478493580929808, 223.7357041228979995 ) ) ;
#5129=CARTESIAN_POINT ( 'NONE',  ( 24.65388594573819958, 1430.511875713700192, 208.0202360571709903 ) ) ;
#5131=EDGE_CURVE ( 'NONE', #36118, #72991, #2370, .T. ) ;
#5133=CARTESIAN_POINT ( 'NONE',  ( -0.9888743217240001382, 1417.038468317130310, 234.0372654507980030 ) ) ;
#5138=CARTESIAN_POINT ( 'NONE',  ( -3.344054220715769965, 1485.138363243759841, 183.2114304489670076 ) ) ;
#5140=CARTESIAN_POINT ( 'NONE',  ( 14.35483100429999936, 1416.837177087930058, 196.6648189961979938 ) ) ;
#5142=VERTEX_POINT ( 'NONE', #5076 ) ;
#5143=EDGE_CURVE ( 'NONE', #94751, #77737, #27812, .T. ) ;
#5145=CARTESIAN_POINT ( 'NONE',  ( 26.91098882550000226, 1508.590122467729998, 215.2366165824080042 ) ) ;
#5148=CARTESIAN_POINT ( 'NONE',  ( -18.68355584089999866, 1410.903490300429894, 196.1540984432980110 ) ) ;
#5149=CARTESIAN_POINT ( 'NONE',  ( -11.59426166675470071, 1425.891398669320097, 141.1919140291859947 ) ) ;
#5150=CARTESIAN_POINT ( 'NONE',  ( 1.361079355559999815, 1508.999526997630028, 179.4746003585979963 ) ) ;
#5152=CARTESIAN_POINT ( 'NONE',  ( -25.43901382002360023, 1451.305424502000051, 136.9267323982909659 ) ) ;
#5153=CARTESIAN_POINT ( 'NONE',  ( -11.63663615270000129, 1425.864876078829866, 144.1644678891980220 ) ) ;
#5154=CARTESIAN_POINT ( 'NONE',  ( 11.56026858080000075, 1410.250182171229881, 229.1792121341979964 ) ) ;
#5157=CARTESIAN_POINT ( 'NONE',  ( 39.33777287878179862, 1438.052711710340191, 134.0999999977100003 ) ) ;
#5158=CARTESIAN_POINT ( 'NONE',  ( -39.81703491479910184, 1441.203410251259811, 136.8482318521629963 ) ) ;
#5159=ORIENTED_EDGE ( 'NONE', *, *, #5131, .F. ) ;
#5161=CARTESIAN_POINT ( 'NONE',  ( -17.00631957490619683, 1410.874949912819375, 226.2321320020102462 ) ) ;
#5163=VERTEX_POINT ( 'NONE', #29188 ) ;
#5166=CARTESIAN_POINT ( 'NONE',  ( 0.2078300974330000161, 1450.905802800400124, 181.2506496984979947 ) ) ;
#5167=CARTESIAN_POINT ( 'NONE',  ( -3.212068473500000465, 1485.523016082529921, 182.9307348487979823 ) ) ;
#5176=CARTESIAN_POINT ( 'NONE',  ( 11.61528297179999925, 1414.971352895729979, 197.1579143274979913 ) ) ;
#5182=CARTESIAN_POINT ( 'NONE',  ( 11.24049413620000060, 1414.988015881329829, 222.4824404014979962 ) ) ;
#5184=CARTESIAN_POINT ( 'NONE',  ( 19.25108290950000267, 1467.194595399430000, 227.2294850399980248 ) ) ;
#5185=EDGE_LOOP ( 'NONE', ( #86439, #100951, #9561, #15847 ) ) ;
#5186=CARTESIAN_POINT ( 'NONE',  ( 0.06655362833503029873, 1450.915384491239820, 181.8858670609800186 ) ) ;
#5187=CARTESIAN_POINT ( 'NONE',  ( -15.83337727950000229, 1409.465974096930040, 192.3897112323980139 ) ) ;
#5188=DIRECTION ( 'NONE',  ( 0.9751355587651674428, 0.000000000000000000, 0.2216092101690377847 ) ) ;
#5192=CARTESIAN_POINT ( 'NONE',  ( -2.164025747320000193, 1508.926860436930156, 179.8555707243980066 ) ) ;
#5195=CARTESIAN_POINT ( 'NONE',  ( 15.48256451790000021, 1460.897023939530072, 229.7631170700979908 ) ) ;
#5196=CARTESIAN_POINT ( 'NONE',  ( -11.60004869885203505, 1423.252811911736217, 137.0073056665461309 ) ) ;
#5202=CARTESIAN_POINT ( 'NONE',  ( 0.03632882829513719297, 1486.486083103770170, 181.8024630677937523 ) ) ;
#5203=CARTESIAN_POINT ( 'NONE',  ( -0.1417130572052019977, 1507.672022827310002, 180.7972791130320047 ) ) ;
#5205=CARTESIAN_POINT ( 'NONE',  ( 18.70435367232109058, 1445.431086849344638, 214.8978195684285879 ) ) ;
#5207=CARTESIAN_POINT ( 'NONE',  ( 18.59896181469999732, 1509.326147590929850, 187.7623525226980234 ) ) ;
#5213=CARTESIAN_POINT ( 'NONE',  ( -10.96572839600000115, 1432.076500672689917, 151.7663020546979737 ) ) ;
#5214=CARTESIAN_POINT ( 'NONE',  ( 19.22285271143139695, 1456.937641708669844, 224.8075632610019738 ) ) ;
#5216=CARTESIAN_POINT ( 'NONE',  ( 3.218260586992740091, 1432.346978324299926, 155.4230415804039751 ) ) ;
#5220=CARTESIAN_POINT ( 'NONE',  ( -21.84276879380000125, 1457.439937068030076, 221.7697786318980206 ) ) ;
#5226=CARTESIAN_POINT ( 'NONE',  ( 4.982688416889999417, 1406.041084510129849, 267.2248725163979657 ) ) ;
#5229=CARTESIAN_POINT ( 'NONE',  ( 21.88093256148639654, 1429.722962281219907, 218.2777509189953093 ) ) ;
#5233=CARTESIAN_POINT ( 'NONE',  ( -1.462738481218180064, 1450.687750463569955, 155.0630832256589997 ) ) ;
#5234=CARTESIAN_POINT ( 'NONE',  ( -1.598127250451339076, 1450.771782104136264, 183.3389037459045880 ) ) ;
#5235=CARTESIAN_POINT ( 'NONE',  ( -19.84652166835276432, 1485.605575737134131, 190.5233726884732732 ) ) ;
#5236=CARTESIAN_POINT ( 'NONE',  ( -14.30082345506849961, 1416.007771869980161, 221.2306877730480039 ) ) ;
#5238=CARTESIAN_POINT ( 'NONE',  ( -25.65427092280000210, 1434.769004650220268, 243.9198229650980068 ) ) ;
#5239=CARTESIAN_POINT ( 'NONE',  ( -26.98839749300549684, 1508.001257810110019, 211.5020470289859986 ) ) ;
#5241=CARTESIAN_POINT ( 'NONE',  ( -6.177389037570000241, 1475.457658709629868, 269.0307152584979917 ) ) ;
#5243=B_SPLINE_CURVE_WITH_KNOTS ( 'NONE', 3,
 ( #14043, #91320, #39819, #71818, #29217, #39259, #54993, #5104, #73980, #108110, #72342, #98611 ),
 .UNSPECIFIED., .F., .F.,
 ( 4, 2, 2, 2, 2, 4 ),
 ( 0.000000000000000000, 0.2500000000000155431, 0.3750000000000233147, 0.5000000000000310862, 0.7500000000000155431, 1.000000000000000000 ),
 .UNSPECIFIED. ) ;
#5244=CARTESIAN_POINT ( 'NONE',  ( -18.60876427879999895, 1443.367094472220060, 192.4891415986979837 ) ) ;
#5245=CARTESIAN_POINT ( 'NONE',  ( -6.524649951413074689, 1486.518242610188963, 182.3718320799524975 ) ) ;
#5248=CARTESIAN_POINT ( 'NONE',  ( -17.21411445179911581, 1414.941240495250440, 207.5657464664730583 ) ) ;
#5252=CARTESIAN_POINT ( 'NONE',  ( -1.270728281904929924, 1414.996443537369942, 226.4582996361970118 ) ) ;
#5253=CARTESIAN_POINT ( 'NONE',  ( -22.18770510819999942, 1409.852309958130036, 204.0989260225280191 ) ) ;
#5257=CARTESIAN_POINT ( 'NONE',  ( 19.68098305160793515, 1455.410563046006473, 226.0042006104999075 ) ) ;
#5259=ORIENTED_EDGE ( 'NONE', *, *, #33197, .F. ) ;
#5260=CARTESIAN_POINT ( 'NONE',  ( -8.919353607585813748, 1410.596373793224302, 230.1706237015127954 ) ) ;
#5263=CARTESIAN_POINT ( 'NONE',  ( 11.63658902509999926, 1425.864914507529875, 144.1610765019980249 ) ) ;
#5265=CARTESIAN_POINT ( 'NONE',  ( 27.65015272131789814, 1446.921108212359968, 137.0757173949590140 ) ) ;
#5275=ORIENTED_EDGE ( 'NONE', *, *, #78745, .T. ) ;
#5276=ORIENTED_EDGE ( 'NONE', *, *, #70145, .F. ) ;
#5277=EDGE_CURVE ( 'NONE', #88595, #59778, #46067, .T. ) ;
#5278=CARTESIAN_POINT ( 'NONE',  ( -10.60671173099999898, 1397.919176979029999, 200.8919131671280240 ) ) ;
#5279=CARTESIAN_POINT ( 'NONE',  ( -21.99779390299999804, 1409.845345892729711, 211.9582520095080156 ) ) ;
#5280=CARTESIAN_POINT ( 'NONE',  ( -1.052431931479999916, 1415.163755984229965, 226.8636908286979974 ) ) ;
#5281=CARTESIAN_POINT ( 'NONE',  ( -13.18815759610568605, 1444.720196239782808, 169.3929182581312887 ) ) ;
#5282=CARTESIAN_POINT ( 'NONE',  ( 47.22425680062420383, 1578.884105819039860, 226.9120406781360089 ) ) ;
#5285=CARTESIAN_POINT ( 'NONE',  ( 16.92682308619999887, 1419.037090534729941, 226.7348578532979957 ) ) ;
#5286=CARTESIAN_POINT ( 'NONE',  ( 3.219365683689999980, 1429.769570239930090, 184.9205627192980330 ) ) ;
#5287=CARTESIAN_POINT ( 'NONE',  ( -11.30589511670000036, 1414.913060387329779, 196.4146731187979924 ) ) ;
#5288=EDGE_CURVE ( 'NONE', #86711, #1325, #81140, .T. ) ;
#5289=CARTESIAN_POINT ( 'NONE',  ( -40.04713527513419535, 1448.341380581330213, 135.9090988750369888 ) ) ;
#5290=CARTESIAN_POINT ( 'NONE',  ( 10.99103875765120009, 1396.296875918300202, 210.4629671561480109 ) ) ;
#5291=CARTESIAN_POINT ( 'NONE',  ( 1.350316101520000256, 1416.274718424630009, 190.2409646149980063 ) ) ;
#5292=CARTESIAN_POINT ( 'NONE',  ( 11.55624295700000026, 1430.790237445429966, 151.0224672601980274 ) ) ;
#5295=CARTESIAN_POINT ( 'NONE',  ( 3.961598046809999829, 1423.998203942029932, 183.4328845819979961 ) ) ;
#5297=VERTEX_POINT ( 'NONE', #66123 ) ;
#5298=ORIENTED_EDGE ( 'NONE', *, *, #43218, .F. ) ;
#5307=CARTESIAN_POINT ( 'NONE',  ( 2.500000000000000000, 1448.507635988019956, 160.4651386227409944 ) ) ;
#5310=CARTESIAN_POINT ( 'NONE',  ( 5.061321880549999541, 1415.087745006229852, 225.4285409366979991 ) ) ;
#5314=CIRCLE ( 'NONE', #33914, 22.86690257359991207 ) ;
#5315=CARTESIAN_POINT ( 'NONE',  ( -20.10853138519999916, 1509.039643839130122, 229.5731426189979913 ) ) ;
#5316=CARTESIAN_POINT ( 'NONE',  ( -29.84310692597631842, 1419.462045361091214, 269.4691403088048105 ) ) ;
#5318=CARTESIAN_POINT ( 'NONE',  ( -4.884981308350000102E-15, 1408.913060387329779, 191.3838116191980134 ) ) ;
#5320=CARTESIAN_POINT ( 'NONE',  ( -0.01271949248029489998, 1452.441493942580109, 183.1886361936269907 ) ) ;
#5321=CARTESIAN_POINT ( 'NONE',  ( -33.18846733439090002, 1440.913060389980046, 247.0360926224090292 ) ) ;
#5323=CARTESIAN_POINT ( 'NONE',  ( -0.1242689031270829830, 1466.391594368360074, 235.6938023998040137 ) ) ;
#5324=CARTESIAN_POINT ( 'NONE',  ( 7.478702110549999560, 1409.021897787929902, 270.4228357812979766 ) ) ;
#5327=CARTESIAN_POINT ( 'NONE',  ( 23.71731968020000281, 1410.130348990129960, 209.4170045476479913 ) ) ;
#5328=CARTESIAN_POINT ( 'NONE',  ( -20.13259047659999723, 1508.866004122629874, 188.8141438244979895 ) ) ;
#5329=CARTESIAN_POINT ( 'NONE',  ( -7.262210027532643331, 1423.020617356984985, 139.1422465717866146 ) ) ;
#5333=CARTESIAN_POINT ( 'NONE',  ( 15.10324330609999954, 1409.440477264029823, 192.5109551743979921 ) ) ;
#5339=DIRECTION ( 'NONE',  ( 0.000000000000000000, 1.000000000000000000, 1.036208156316812031E-12 ) ) ;
#5340=CARTESIAN_POINT ( 'NONE',  ( 0.1366081833359999997, 1416.109320291729773, 233.5463589650980225 ) ) ;
#5342=CARTESIAN_POINT ( 'NONE',  ( -20.76201028965770234, 1508.885069966210040, 228.4351800535669952 ) ) ;
#5356=CARTESIAN_POINT ( 'NONE',  ( 19.44861509849999948, 1455.533462210330072, 225.7267910435979843 ) ) ;
#5360=CARTESIAN_POINT ( 'NONE',  ( 16.20463669235772386, 1421.461506550293507, 227.3035140667420251 ) ) ;
#5361=DIRECTION ( 'NONE',  ( 0.000000000000000000, 1.000000000000000000, -0.000000000000000000 ) ) ;
#5362=CARTESIAN_POINT ( 'NONE',  ( -19.24690813209999973, 1426.102494106830136, 224.1205169862979858 ) ) ;
#5363=CARTESIAN_POINT ( 'NONE',  ( -25.00976051679999657, 1436.598010167069788, 137.9330532114979917 ) ) ;
#5365=CARTESIAN_POINT ( 'NONE',  ( 19.35574166329999812, 1498.080849027529894, 189.0919305048980164 ) ) ;
#5367=CARTESIAN_POINT ( 'NONE',  ( -18.45403838167598209, 1436.531269343617168, 212.9422139639101772 ) ) ;
#5368=CARTESIAN_POINT ( 'NONE',  ( -29.82636534510967508, 1462.376341263100585, 269.4689657811763368 ) ) ;
#5374=CARTESIAN_POINT ( 'NONE',  ( -0.9776412681320001408, 1475.513060387329915, 230.7453403689980007 ) ) ;
#5376=CARTESIAN_POINT ( 'NONE',  ( 1.461235200690810032, 1494.741996085649816, 181.6529089755349844 ) ) ;
#5378=CARTESIAN_POINT ( 'NONE',  ( -13.24008678843756925, 1444.663275562806803, 186.6390711729250711 ) ) ;
#5383=CARTESIAN_POINT ( 'NONE',  ( -1.810647825301244129, 1415.577673978943039, 233.0806231791490291 ) ) ;
#5387=CARTESIAN_POINT ( 'NONE',  ( -14.72054864259999896, 1409.427113273230134, 225.7256316435980068 ) ) ;
#5391=ORIENTED_EDGE ( 'NONE', *, *, #14745, .T. ) ;
#5392=VERTEX_POINT ( 'NONE', #7827 ) ;
#5393=CARTESIAN_POINT ( 'NONE',  ( 16.49832412793039893, 1414.913057855109855, 209.6477601274349922 ) ) ;
#5394=CARTESIAN_POINT ( 'NONE',  ( 12.86976130269999885, 1508.080714966730056, 233.3011978812979805 ) ) ;
#5396=CARTESIAN_POINT ( 'NONE',  ( -10.01186952459999802, 1466.025750520630027, 244.5548898232979980 ) ) ;
#5398=CARTESIAN_POINT ( 'NONE',  ( -11.90032380669999945, 1433.331458429630175, 150.1435198483980287 ) ) ;
#5401=CARTESIAN_POINT ( 'NONE',  ( -25.47645757409999945, 1436.566927373820135, 137.1740747294979883 ) ) ;
#5403=CARTESIAN_POINT ( 'NONE',  ( -4.500000000000000000, 1448.210448412289907, 183.1418046154980175 ) ) ;
#5404=CARTESIAN_POINT ( 'NONE',  ( 12.86636877496950149, 1428.376440794390192, 223.7743079858460078 ) ) ;
#5406=CARTESIAN_POINT ( 'NONE',  ( -1.365576857718376003, 1509.093805881863091, 239.1218459691334033 ) ) ;
#5407=CARTESIAN_POINT ( 'NONE',  ( 1.395903919076789877E-08, 1408.640860330559917, 261.6452554441709708 ) ) ;
#5413=CARTESIAN_POINT ( 'NONE',  ( -14.72002262839999887, 1469.537467531630227, 269.3627926194980091 ) ) ;
#5416=B_SPLINE_CURVE_WITH_KNOTS ( 'NONE', 3,
 ( #51264, #44532, #43429, #42875, #1994, #36129 ),
 .UNSPECIFIED., .F., .F.,
 ( 4, 2, 4 ),
 ( 0.000000000000000000, 0.5000000000000000000, 1.000000000000000000 ),
 .UNSPECIFIED. ) ;
#5417=CARTESIAN_POINT ( 'NONE',  ( 33.93383603481760247, 1451.270696425840015, 135.9469434958280090 ) ) ;
#5419=CARTESIAN_POINT ( 'NONE',  ( 0.3830348160098190347, 1450.899684516809884, 181.3422595746110062 ) ) ;
#5421=EDGE_CURVE ( 'NONE', #89175, #36972, #105152, .T. ) ;
#5425=CARTESIAN_POINT ( 'NONE',  ( -39.67050070681160179, 1422.888949612689885, 266.6045514581650195 ) ) ;
#5427=VERTEX_POINT ( 'NONE', #83987 ) ;
#5428=CARTESIAN_POINT ( 'NONE',  ( -24.24612263075051288, 1442.627844462843541, 211.5705962792871446 ) ) ;
#5436=CARTESIAN_POINT ( 'NONE',  ( -16.51001495079999870, 1425.424181616729811, 190.9332292383980132 ) ) ;
#5437=CARTESIAN_POINT ( 'NONE',  ( -1.992696810621175540, 1450.242131535874478, 182.8294641353408281 ) ) ;
#5438=ORIENTED_EDGE ( 'NONE', *, *, #46699, .T. ) ;
#5439=CARTESIAN_POINT ( 'NONE',  ( -26.41196673809999851, 1435.620866968539985, 136.0816445379979882 ) ) ;
#5441=DIRECTION ( 'NONE',  ( -0.001183870442918495778, 0.9989952321583787098, 0.04480094391417914490 ) ) ;
#5442=CARTESIAN_POINT ( 'NONE',  ( 2.294541319819646041, 1508.993187694497465, 238.4785069940606661 ) ) ;
#5443=CARTESIAN_POINT ( 'NONE',  ( -43.48865640085159612, 1435.886059616880175, 270.3367133951149981 ) ) ;
#5445=CARTESIAN_POINT ( 'NONE',  ( -4.717969115980000794, 1396.259831671730126, 198.0836446571979934 ) ) ;
#5448=ORIENTED_EDGE ( 'NONE', *, *, #6645, .F. ) ;
#5449=CARTESIAN_POINT ( 'NONE',  ( 0.4364087686210000316, 1450.897820657319926, 181.2764007302979792 ) ) ;
#5450=CARTESIAN_POINT ( 'NONE',  ( 32.26066749790219745, 1465.087609890807016, 269.3103000282806647 ) ) ;
#5454=CARTESIAN_POINT ( 'NONE',  ( -0.03560127825697149279, 1409.432827519930242, 185.3548041051600137 ) ) ;
#5457=CARTESIAN_POINT ( 'NONE',  ( 2.596345137909159551, 1439.736139237240195, 157.6563016627050047 ) ) ;
#5458=CARTESIAN_POINT ( 'NONE',  ( 0.000000000000000000, 1445.052233488290085, 126.8032249175980155 ) ) ;
#5465=CARTESIAN_POINT ( 'NONE',  ( -23.83497567388974048, 1446.573076643067225, 213.8261868645313655 ) ) ;
#5467=CARTESIAN_POINT ( 'NONE',  ( 18.22805055419890152, 1459.311389626190021, 227.8763770136359881 ) ) ;
#5468=AXIS2_PLACEMENT_3D ( 'NONE', #29059, #96820, #20089 ) ;
#5470=CARTESIAN_POINT ( 'NONE',  ( -4.114495368158031852, 1440.063097891708139, 185.4396243348899986 ) ) ;
#5471=CARTESIAN_POINT ( 'NONE',  ( -2.922186645726760013, 1413.437602691799839, 186.4765809533099912 ) ) ;
#5472=CARTESIAN_POINT ( 'NONE',  ( 22.33897096189999942, 1410.187224096529917, 206.2328832085579791 ) ) ;
#5476=CARTESIAN_POINT ( 'NONE',  ( 4.247461698663549612, 1441.373656070180004, 161.5375685151940104 ) ) ;
#5480=ORIENTED_EDGE ( 'NONE', *, *, #3607, .F. ) ;
#5482=CARTESIAN_POINT ( 'NONE',  ( -7.595213676849999374, 1473.705021973730027, 270.1248737330980134 ) ) ;
#5483=CARTESIAN_POINT ( 'NONE',  ( 0.3641805758275279969, 1424.317995888269934, 227.5054904079770211 ) ) ;
#5485=CARTESIAN_POINT ( 'NONE',  ( -6.037828305847510180, 1422.573108036489884, 122.8777291217150065 ) ) ;
#5488=CARTESIAN_POINT ( 'NONE',  ( 11.60004869885015211, 1426.082545937270424, 138.9242053348294519 ) ) ;
#5489=CARTESIAN_POINT ( 'NONE',  ( 2.790610563364870789, 1417.787132752280741, 234.0645936422330919 ) ) ;
#5490=CARTESIAN_POINT ( 'NONE',  ( -2.500000000000000000, 1432.241594156859946, 157.4925871266979982 ) ) ;
#5491=ADVANCED_FACE ( 'NONE', ( #33568 ), #41967, .F. ) ;
#5495=CARTESIAN_POINT ( 'NONE',  ( 32.33429827083980257, 1440.913060383199991, 244.9699483744109898 ) ) ;
#5496=EDGE_CURVE ( 'NONE', #33774, #83258, #42473, .T. ) ;
#5499=CARTESIAN_POINT ( 'NONE',  ( 13.05081502930000070, 1422.960060114630096, 222.0524190261979811 ) ) ;
#5500=VERTEX_POINT ( 'NONE', #52062 ) ;
#5502=FACE_OUTER_BOUND ( 'NONE', #99984, .T. ) ;
#5503=CARTESIAN_POINT ( 'NONE',  ( -19.10636532737555626, 1485.521373224806439, 189.6418533252866894 ) ) ;
#5504=CARTESIAN_POINT ( 'NONE',  ( -0.9810412822912069064, 1409.219255427743292, 186.0188850891012464 ) ) ;
#5513=CARTESIAN_POINT ( 'NONE',  ( -13.90890181880000043, 1453.165958253930057, 194.3940701926979955 ) ) ;
#5516=CARTESIAN_POINT ( 'NONE',  ( 2.157288638769999878, 1464.754106553530164, 235.9996813455979918 ) ) ;
#5517=LINE ( 'NONE', #28515, #65828 ) ;
#5519=CARTESIAN_POINT ( 'NONE',  ( -0.3328288701460000443, 1452.976686003830082, 183.2631395458980137 ) ) ;
#5527=AXIS2_PLACEMENT_3D ( 'NONE', #70412, #34010, #44643 ) ;
#5531=CARTESIAN_POINT ( 'NONE',  ( -11.60004869884828338, 1426.567386193286893, 135.1569321345708090 ) ) ;
#5535=AXIS2_PLACEMENT_3D ( 'NONE', #104140, #79506, #94628 ) ;
#5536=CARTESIAN_POINT ( 'NONE',  ( -3.885780586189999829E-16, 1420.943991414029824, 179.3023655596979893 ) ) ;
#5537=CARTESIAN_POINT ( 'NONE',  ( 2.955851087435179991, 1409.016280981779801, 194.4300961132470036 ) ) ;
#5538=CARTESIAN_POINT ( 'NONE',  ( 18.03390783410000253, 1424.747035879229998, 225.0015027529979932 ) ) ;
#5540=CARTESIAN_POINT ( 'NONE',  ( -19.64105509870000077, 1485.638507108129943, 190.1260793311979853 ) ) ;
#5541=CARTESIAN_POINT ( 'NONE',  ( 11.86561512750000169, 1432.302095436430136, 149.9824189746979926 ) ) ;
#5542=CARTESIAN_POINT ( 'NONE',  ( -4.115857443736018695, 1425.929640604822680, 186.1083528362279651 ) ) ;
#5543=EDGE_LOOP ( 'NONE', ( #5031, #21279, #102810, #92614 ) ) ;
#5546=CARTESIAN_POINT ( 'NONE',  ( 19.03157125241660097, 1457.060517503149867, 226.1452829519230079 ) ) ;
#5547=B_SPLINE_CURVE_WITH_KNOTS ( 'NONE', 3,
 ( #94936, #62479, #26615, #69767, #45113, #87651 ),
 .UNSPECIFIED., .F., .F.,
 ( 4, 2, 4 ),
 ( 0.000000000000000000, 0.5000000000000000000, 1.000000000000000000 ),
 .UNSPECIFIED. ) ;
#5551=CARTESIAN_POINT ( 'NONE',  ( -20.32074529087200077, 1498.819556202739932, 190.6518178786860176 ) ) ;
#5553=DIRECTION ( 'NONE',  ( -0.9417419115949053898, -0.3363363969979660806, -9.559255346349042767E-16 ) ) ;
#5555=CARTESIAN_POINT ( 'NONE',  ( -1.465047864650000031, 1483.408900079630030, 182.5218640156980143 ) ) ;
#5557=CARTESIAN_POINT ( 'NONE',  ( -46.16552303099769716, 1440.463954059739990, 266.9715276195660181 ) ) ;
#5558=CARTESIAN_POINT ( 'NONE',  ( -19.52413277859999852, 1426.414269502929756, 225.5212833970979887 ) ) ;
#5559=CARTESIAN_POINT ( 'NONE',  ( 13.89554995500000167, 1452.733480491630189, 223.3956528723979886 ) ) ;
#5563=CARTESIAN_POINT ( 'NONE',  ( -13.64440718200000013, 1435.322370893529978, 149.8642038458980323 ) ) ;
#5564=FILL_AREA_STYLE ('',( #31856 ) ) ;
#5567=ORIENTED_EDGE ( 'NONE', *, *, #29783, .F. ) ;
#5568=CARTESIAN_POINT ( 'NONE',  ( 36.81312681789999885, 1440.913060384859818, 254.5659338001980529 ) ) ;
#5569=CARTESIAN_POINT ( 'NONE',  ( 4.500000000000000000, 1426.966631815929986, 170.4008037693979816 ) ) ;
#5570=CARTESIAN_POINT ( 'NONE',  ( 0.4937778921180000502, 1478.160124056830000, 182.1794214162979983 ) ) ;
#5571=CARTESIAN_POINT ( 'NONE',  ( -17.63079341550000123, 1410.452321969430159, 194.5845618450980226 ) ) ;
#5572=( BOUNDED_CURVE ( )  B_SPLINE_CURVE ( 3, ( #41935, #7770, #50892, #77746 ),
 .UNSPECIFIED., .F., .T. ) 
 B_SPLINE_CURVE_WITH_KNOTS ( ( 4, 4 ),
 ( 1.036306020146634088, 2.105308394323555099 ),
 .UNSPECIFIED. ) 
 CURVE ( )  GEOMETRIC_REPRESENTATION_ITEM ( )  RATIONAL_B_SPLINE_CURVE ( ( 1.000000000000000000, 0.9070152250226227730, 0.9070152250226227730, 1.000000000000000000 ) ) 
 REPRESENTATION_ITEM ( '' )  );
#5573=CARTESIAN_POINT ( 'NONE',  ( -27.08076141661259939, 1414.294488336634686, 269.9731936574717110 ) ) ;
#5574=CARTESIAN_POINT ( 'NONE',  ( -22.49770453780000068, 1429.484910292730092, 225.2498666484979992 ) ) ;
#5576=CARTESIAN_POINT ( 'NONE',  ( -0.9757794191400900319, 1452.878985419150013, 152.5158834087430080 ) ) ;
#5577=CARTESIAN_POINT ( 'NONE',  ( 28.27349493010000003, 1451.471014347730033, 136.1137886329979949 ) ) ;
#5578=ORIENTED_EDGE ( 'NONE', *, *, #33188, .F. ) ;
#5580=CARTESIAN_POINT ( 'NONE',  ( 2.098309414416280126E-05, 1407.650889052649973, 270.1377145618209283 ) ) ;
#5581=CARTESIAN_POINT ( 'NONE',  ( -0.04885444012580000134, 1508.952077801630139, 238.8419334758980028 ) ) ;
#5583=EDGE_LOOP ( 'NONE', ( #76471, #6925, #47180, #75560, #86734, #55615 ) ) ;
#5586=CARTESIAN_POINT ( 'NONE',  ( -24.07954513569999833, 1411.114689535729894, 209.5888749416580197 ) ) ;
#5589=CARTESIAN_POINT ( 'NONE',  ( -0.2612701254520000127, 1416.813004075730078, 227.4660694200979947 ) ) ;
#5592=CARTESIAN_POINT ( 'NONE',  ( -21.10399601188239416, 1436.465560437122576, 144.1929280529386972 ) ) ;
#5595=CARTESIAN_POINT ( 'NONE',  ( 44.34415660218949284, 1449.868985015139742, 268.8027473384019572 ) ) ;
#5596=CARTESIAN_POINT ( 'NONE',  ( -13.15726442530000107, 1416.237488680629895, 221.8313562556980116 ) ) ;
#5597=CARTESIAN_POINT ( 'NONE',  ( -0.1147355858779999932, 1419.163093610929991, 184.6463452042980009 ) ) ;
#5602=CARTESIAN_POINT ( 'NONE',  ( 13.51299049401507091, 1444.004812340696390, 188.0184190261968524 ) ) ;
#5604=VERTEX_POINT ( 'NONE', #39085 ) ;
#5608=CARTESIAN_POINT ( 'NONE',  ( 4.724549302593670674, 1452.748075490200108, 152.1309929677310038 ) ) ;
#5609=CARTESIAN_POINT ( 'NONE',  ( -1.651001239120279923E-05, 1410.239988154289904, 269.6149086386799922 ) ) ;
#5613=CARTESIAN_POINT ( 'NONE',  ( -6.896890933126118993E-05, 1408.913065613199933, 231.7784170915439859 ) ) ;
#5615=CARTESIAN_POINT ( 'NONE',  ( 17.27619071350000013, 1507.625766668030110, 193.9878102724979954 ) ) ;
#5618=CARTESIAN_POINT ( 'NONE',  ( -24.02956139221189957, 1507.932518080230011, 222.3125113693119772 ) ) ;
#5620=CARTESIAN_POINT ( 'NONE',  ( 4.882003189570000679, 1430.559178934629927, 150.0077195948979920 ) ) ;
#5622=FACE_OUTER_BOUND ( 'NONE', #26224, .T. ) ;
#5635=CARTESIAN_POINT ( 'NONE',  ( -12.78690713350000152, 1416.828040475229955, 195.5394874918979724 ) ) ;
#5636=CARTESIAN_POINT ( 'NONE',  ( 20.14739811709999984, 1469.497636830730016, 271.1218459616979999 ) ) ;
#5637=CARTESIAN_POINT ( 'NONE',  ( 0.5697990016583959205, 1450.893162567740092, 181.2939912002310052 ) ) ;
#5641=CARTESIAN_POINT ( 'NONE',  ( 15.40374502139999890, 1422.106951872629907, 227.8157797934979953 ) ) ;
#5643=DIRECTION ( 'NONE',  ( 0.000000000000000000, 0.000000000000000000, 1.000000000000000000 ) ) ;
#5644=CARTESIAN_POINT ( 'NONE',  ( 9.064548041611230289, 1441.200071122209920, 153.7187301893350195 ) ) ;
#5645=CARTESIAN_POINT ( 'NONE',  ( -17.68297954760000223, 1410.894413715530163, 225.3003200628979812 ) ) ;
#5648=CARTESIAN_POINT ( 'NONE',  ( -1.544578923920000069, 1422.347071476030123, 228.2660149837979873 ) ) ;
#5650=CARTESIAN_POINT ( 'NONE',  ( 31.03138121380739989, 1441.878430465370002, 137.2367898306910092 ) ) ;
#5652=CARTESIAN_POINT ( 'NONE',  ( -1.538891143356439777E-07, 1406.985163805290085, 196.1207725567600164 ) ) ;
#5655=CARTESIAN_POINT ( 'NONE',  ( -3.954003734500000089, 1416.825421876529845, 227.3234521733980102 ) ) ;
#5657=CARTESIAN_POINT ( 'NONE',  ( -13.35131665876559914, 1408.061408147960037, 210.5533457943919871 ) ) ;
#5658=CARTESIAN_POINT ( 'NONE',  ( -13.25708502290000013, 1414.913060387329779, 199.5091795105679751 ) ) ;
#5660=CARTESIAN_POINT ( 'NONE',  ( 13.80577029839999881, 1434.979611850010087, 147.2734062573980225 ) ) ;
#5661=DIRECTION ( 'NONE',  ( -0.2495203814060049652, -0.1962602150479464402, -0.9482729075811118236 ) ) ;
#5662=CARTESIAN_POINT ( 'NONE',  ( 8.745088717699999847, 1441.583345737160016, 186.1462670829980084 ) ) ;
#5669=EDGE_CURVE ( 'NONE', #86466, #77021, #79780, .T. ) ;
#5670=CARTESIAN_POINT ( 'NONE',  ( 20.52383114756580085, 1473.184610000140083, 208.7461008354759997 ) ) ;
#5671=CARTESIAN_POINT ( 'NONE',  ( 15.67984159504549879, 1509.462706413110027, 234.0183160927130075 ) ) ;
#5672=CARTESIAN_POINT ( 'NONE',  ( 41.65685823593407378, 1426.928113394742468, 269.0850263944785752 ) ) ;
#5675=DIRECTION ( 'NONE',  ( -0.9211327884476214756, -0.3892484888175026247, 0.000000000000000000 ) ) ;
#5680=EDGE_CURVE ( 'NONE', #8387, #93417, #107924, .T. ) ;
#5681=CARTESIAN_POINT ( 'NONE',  ( -28.91692647416590134, 1509.557647291290095, 208.7049441970110308 ) ) ;
#5682=CARTESIAN_POINT ( 'NONE',  ( -15.80103170504700039, 1409.464838628420011, 225.2833922138719913 ) ) ;
#5685=CARTESIAN_POINT ( 'NONE',  ( -14.35518634559999818, 1509.483852653929944, 182.9676329983980168 ) ) ;
#5689=CARTESIAN_POINT ( 'NONE',  ( -11.24049419400000005, 1414.988017874730076, 195.7612516212979870 ) ) ;
#5690=CARTESIAN_POINT ( 'NONE',  ( 0.2042600169000000077, 1465.101704582730235, 237.0131066117980083 ) ) ;
#5691=CARTESIAN_POINT ( 'NONE',  ( 22.49646906260000279, 1410.193735020430040, 214.3055066545979912 ) ) ;
#5692=CARTESIAN_POINT ( 'NONE',  ( -2.667363771992699473, 1417.233457082500081, 186.2697805505230235 ) ) ;
#5694=CARTESIAN_POINT ( 'NONE',  ( -16.36294508339999965, 1422.940422817830040, 227.7580329737979810 ) ) ;
#5696=CARTESIAN_POINT ( 'NONE',  ( 26.50595462180590189, 1469.329495983640072, 208.3089406750970056 ) ) ;
#5698=CARTESIAN_POINT ( 'NONE',  ( 22.68380688229993680, 1509.726051394556407, 190.0734992207788991 ) ) ;
#5699=CARTESIAN_POINT ( 'NONE',  ( -23.65270513040000111, 1430.813106381330044, 211.2966596496080172 ) ) ;
#5704=CARTESIAN_POINT ( 'NONE',  ( 0.8265244082521410185, 1408.941923255679967, 231.1644249228330068 ) ) ;
#5705=CARTESIAN_POINT ( 'NONE',  ( -4.228853213262760313, 1441.542194655879939, 165.2229178842150077 ) ) ;
#5708=ORIENTED_EDGE ( 'NONE', *, *, #60246, .F. ) ;
#5714=CARTESIAN_POINT ( 'NONE',  ( -10.37251529557829954, 1441.250888918300006, 153.2543604180100090 ) ) ;
#5715=CARTESIAN_POINT ( 'NONE',  ( 15.94138077806149845, 1410.571769083230038, 191.5578847893440013 ) ) ;
#5717=EDGE_CURVE ( 'NONE', #63851, #10428, #85098, .T. ) ;
#5720=CARTESIAN_POINT ( 'NONE',  ( 10.81507089421240053, 1424.921187596799882, 144.1620444706739761 ) ) ;
#5722=CARTESIAN_POINT ( 'NONE',  ( 37.66742087362709412, 1450.649596001800091, 134.0999999985879754 ) ) ;
#5723=( BOUNDED_CURVE ( )  B_SPLINE_CURVE ( 3, ( #68525, #85853, #223, #61250 ),
 .UNSPECIFIED., .F., .T. ) 
 B_SPLINE_CURVE_WITH_KNOTS ( ( 4, 4 ),
 ( 4.177675889938866405, 5.247004472095339267 ),
 .UNSPECIFIED. ) 
 CURVE ( )  GEOMETRIC_REPRESENTATION_ITEM ( )  RATIONAL_B_SPLINE_CURVE ( ( 1.000000000000000000, 0.9069598259872098112, 0.9069598259872098112, 1.000000000000000000 ) ) 
 REPRESENTATION_ITEM ( '' )  );
#5724=DIRECTION ( 'NONE',  ( 0.03489949670246857150, 0.9993908270190969834, 0.000000000000000000 ) ) ;
#5727=CARTESIAN_POINT ( 'NONE',  ( -18.37766962349999744, 1457.945728469830101, 227.9374886095980060 ) ) ;
#5728=VERTEX_POINT ( 'NONE', #22826 ) ;
#5729=ORIENTED_EDGE ( 'NONE', *, *, #107778, .F. ) ;
#5731=CARTESIAN_POINT ( 'NONE',  ( -3.218260648026030069, 1432.346989537609943, 155.4230417355269935 ) ) ;
#5732=EDGE_CURVE ( 'NONE', #4376, #7383, #3637, .T. ) ;
#5735=CARTESIAN_POINT ( 'NONE',  ( -2.500000000000000000, 1439.621710174999862, 168.1588803299280244 ) ) ;
#5736=AXIS2_PLACEMENT_3D ( 'NONE', #42697, #18022, #34285 ) ;
#5738=CARTESIAN_POINT ( 'NONE',  ( 36.37832868398670172, 1435.767865609760065, 135.3769914889309973 ) ) ;
#5741=CARTESIAN_POINT ( 'NONE',  ( 9.959064829120000795, 1415.087818611729972, 195.3775652628979742 ) ) ;
#5746=ORIENTED_EDGE ( 'NONE', *, *, #79495, .T. ) ;
#5747=CARTESIAN_POINT ( 'NONE',  ( 34.44779686536719510, 1440.913060387330006, 260.0104300309679957 ) ) ;
#5748=EDGE_CURVE ( 'NONE', #95283, #62471, #72986, .T. ) ;
#5749=CARTESIAN_POINT ( 'NONE',  ( -0.002357574298573597137, 1451.791738093121467, 154.0465204539138142 ) ) ;
#5751=CARTESIAN_POINT ( 'NONE',  ( -15.06280282045160135, 1422.388303761650150, 229.4662100962750060 ) ) ;
#5753=PLANE ( 'NONE',  #77812 ) ;
#5755=CARTESIAN_POINT ( 'NONE',  ( -12.61812115819999924, 1416.825245919430245, 222.0544627597980138 ) ) ;
#5757=CARTESIAN_POINT ( 'NONE',  ( -20.61690376153225301, 1509.299818264167243, 229.2235484916167820 ) ) ;
#5758=CARTESIAN_POINT ( 'NONE',  ( 0.5565654927739999147, 1405.991402147929875, 266.9610393333979914 ) ) ;
#5761=CARTESIAN_POINT ( 'NONE',  ( 14.93370170679999909, 1461.288361491829846, 230.0893540134979958 ) ) ;
#5762=CARTESIAN_POINT ( 'NONE',  ( -24.20882859423510070, 1435.739118765830199, 210.8967395777180229 ) ) ;
#5765=VERTEX_POINT ( 'NONE', #28239 ) ;
#5766=CARTESIAN_POINT ( 'NONE',  ( -0.5533431911963668792, 1486.379993417803689, 181.7748704520617480 ) ) ;
#5767=CARTESIAN_POINT ( 'NONE',  ( -0.08976027792670869532, 1508.421112912959870, 180.3398118522160019 ) ) ;
#5768=CARTESIAN_POINT ( 'NONE',  ( 18.25525582808161218, 1446.597240889685281, 216.0033427005020030 ) ) ;
#5770=CARTESIAN_POINT ( 'NONE',  ( 18.55970574510000048, 1508.848287786029914, 188.2531264885979851 ) ) ;
#5773=ORIENTED_EDGE ( 'NONE', *, *, #71836, .F. ) ;
#5774=B_SPLINE_CURVE_WITH_KNOTS ( 'NONE', 3,
 ( #44237, #19561, #86775, #52088, #2257, #78950, #20116, #104127, #45898, #27973, #103571, #62157, #52638, #28528, #54308, #10064, #78381 ),
 .UNSPECIFIED., .F., .F.,
 ( 4, 2, 2, 1, 1, 1, 1, 1, 2, 2, 4 ),
 ( 0.000000000000000000, 0.2500000000000363598, 0.5000000000000727196, 0.6250000000000900391, 0.6875000000000995870, 0.7187500000001053602, 0.7343750000001072475, 0.7421875000001063594, 0.7460937500001042499, 0.7500000000001021405, 1.000000000000000000 ),
 .UNSPECIFIED. ) ;
#5778=CARTESIAN_POINT ( 'NONE',  ( -11.85676285999999990, 1431.648968933459855, 150.3599054133979962 ) ) ;
#5781=CARTESIAN_POINT ( 'NONE',  ( 9.400735431060539327, 1432.346466415740224, 153.1462980661239897 ) ) ;
#5782=ADVANCED_FACE ( 'NONE', ( #2519 ), #11991, .T. ) ;
#5786=CARTESIAN_POINT ( 'NONE',  ( -23.17373061810000223, 1444.794561936630089, 216.5813394841780166 ) ) ;
#5787=CARTESIAN_POINT ( 'NONE',  ( -9.459818323764448422, 1424.144492356367664, 137.0999999969407099 ) ) ;
#5791=CARTESIAN_POINT ( 'NONE',  ( 9.883432818870000247, 1406.823613192530047, 269.0083561828979555 ) ) ;
#5793=CARTESIAN_POINT ( 'NONE',  ( 19.26869546180000015, 1410.873740538630045, 195.8008840898980054 ) ) ;
#5794=ADVANCED_FACE ( 'NONE', ( #95992 ), #12143, .F. ) ;
#5795=CARTESIAN_POINT ( 'NONE',  ( 24.00668311305575742, 1435.609311454352110, 213.8188581933794410 ) ) ;
#5796=CARTESIAN_POINT ( 'NONE',  ( -24.10313149040000269, 1452.071361778829896, 136.4709151672980170 ) ) ;
#5797=DIRECTION ( 'NONE',  ( -0.000000000000000000, -0.000000000000000000, 1.000000000000000000 ) ) ;
#5799=CARTESIAN_POINT ( 'NONE',  ( -2.437740576677990489, 1449.518193424200035, 155.3362125304199992 ) ) ;
#5800=CARTESIAN_POINT ( 'NONE',  ( -12.72147812920000121, 1445.025642375379903, 185.9027152744980071 ) ) ;
#5801=CARTESIAN_POINT ( 'NONE',  ( -19.75663087343670909, 1485.988119119562953, 190.2206659241704756 ) ) ;
#5802=CARTESIAN_POINT ( 'NONE',  ( -14.34456629294319896, 1416.134159100620082, 221.2755357109419947 ) ) ;
#5804=CARTESIAN_POINT ( 'NONE',  ( -7.707668447030600056, 1409.182218100520004, 196.2912339717319981 ) ) ;
#5807=CARTESIAN_POINT ( 'NONE',  ( 2.499999998570000326, 1439.824558940259976, 159.3162087218979934 ) ) ;
#5808=CARTESIAN_POINT ( 'NONE',  ( -6.106286103040000413, 1474.752488639329840, 269.6381986971979927 ) ) ;
#5809=CARTESIAN_POINT ( 'NONE',  ( -4.244916217095670241, 1446.427620833529772, 161.9653756394929758 ) ) ;
#5811=EDGE_CURVE ( 'NONE', #86293, #63851, #29000, .T. ) ;
#5816=CARTESIAN_POINT ( 'NONE',  ( 16.93613030662569940, 1507.562497965019929, 193.6637058848310176 ) ) ;
#5819=CARTESIAN_POINT ( 'NONE',  ( -18.44228220140000118, 1409.721884562830155, 196.7777138713979923 ) ) ;
#5820=CARTESIAN_POINT ( 'NONE',  ( -15.49718189712599958, 1421.634728641663969, 227.2930083201289904 ) ) ;
#5821=CARTESIAN_POINT ( 'NONE',  ( -37.09487445649999415, 1421.897761927629972, 269.8322594516980075 ) ) ;
#5822=ORIENTED_EDGE ( 'NONE', *, *, #86219, .T. ) ;
#5823=CARTESIAN_POINT ( 'NONE',  ( -2.336386348569962745, 1410.372884070141026, 232.7140726396572745 ) ) ;
#5829=CARTESIAN_POINT ( 'NONE',  ( 7.768471907389999487, 1409.184341404130009, 189.0606530832980070 ) ) ;
#5830=FACE_OUTER_BOUND ( 'NONE', #11616, .T. ) ;
#5834=CARTESIAN_POINT ( 'NONE',  ( -12.61716434588512037, 1398.287096944733094, 212.2535635707003507 ) ) ;
#5838=CARTESIAN_POINT ( 'NONE',  ( 20.04660124756710005, 1509.276552014090157, 229.7844253363949747 ) ) ;
#5841=ORIENTED_EDGE ( 'NONE', *, *, #83719, .T. ) ;
#5842=CARTESIAN_POINT ( 'NONE',  ( 0.01233345008840000014, 1396.097901039130193, 221.0480490693979903 ) ) ;
#5843=CARTESIAN_POINT ( 'NONE',  ( -19.17428229720000132, 1409.582641083130056, 220.3285384914979943 ) ) ;
#5844=ORIENTED_EDGE ( 'NONE', *, *, #34494, .T. ) ;
#5845=CARTESIAN_POINT ( 'NONE',  ( -13.51602633418888821, 1443.948650972781479, 169.3503399069581121 ) ) ;
#5846=CARTESIAN_POINT ( 'NONE',  ( 21.56377605174612100, 1509.708111594535012, 229.5989167562945852 ) ) ;
#5848=FACE_OUTER_BOUND ( 'NONE', #28299, .T. ) ;
#5849=CARTESIAN_POINT ( 'NONE',  ( 17.17836974400000116, 1416.259463228930144, 226.4421905685979937 ) ) ;
#5850=CARTESIAN_POINT ( 'NONE',  ( 1.034090463059999854, 1410.308950726829835, 185.1959119782980281 ) ) ;
#5853=CARTESIAN_POINT ( 'NONE',  ( 10.69511309515409891, 1396.286541966780078, 206.2627936616379998 ) ) ;
#5854=CARTESIAN_POINT ( 'NONE',  ( 14.39446395561900083, 1416.321686235030029, 196.9169130221449961 ) ) ;
#5855=CARTESIAN_POINT ( 'NONE',  ( 11.52956870459999905, 1428.865126643429903, 150.2645387300980246 ) ) ;
#5856=CARTESIAN_POINT ( 'NONE',  ( 16.90742456150000095, 1442.831169986189934, 162.4348202098979925 ) ) ;
#5858=CARTESIAN_POINT ( 'NONE',  ( 13.11860189580039915, 1435.347307412770078, 150.3412794832900090 ) ) ;
#5859=CARTESIAN_POINT ( 'NONE',  ( 1.930489070153026399, 1450.295778691457372, 181.9128711244939325 ) ) ;
#5869=CARTESIAN_POINT ( 'NONE',  ( 2.500000000000000000, 1448.626811758040049, 158.8049822478760120 ) ) ;
#5874=CARTESIAN_POINT ( 'NONE',  ( -20.38220705570000035, 1509.051558519629907, 229.2949352805979970 ) ) ;
#5875=CARTESIAN_POINT ( 'NONE',  ( -32.57952228147021145, 1421.659236551914319, 269.5001856740272501 ) ) ;
#5876=CARTESIAN_POINT ( 'NONE',  ( -0.8957367667660000032, 1409.883006492629875, 233.0638040154979933 ) ) ;
#5877=CARTESIAN_POINT ( 'NONE',  ( -0.1496009369319929727, 1415.938742849230039, 227.0988434848029840 ) ) ;
#5878=ORIENTED_EDGE ( 'NONE', *, *, #107533, .F. ) ;
#5879=FACE_OUTER_BOUND ( 'NONE', #7172, .T. ) ;
#5880=CARTESIAN_POINT ( 'NONE',  ( -27.91175324445159944, 1440.913060390089868, 230.7978836448200184 ) ) ;
#5882=CARTESIAN_POINT ( 'NONE',  ( -0.3530909465895950006, 1467.116854953090069, 235.6078142961000026 ) ) ;
#5883=CARTESIAN_POINT ( 'NONE',  ( 10.97762738470000166, 1408.611869070129842, 270.1116084948980074 ) ) ;
#5885=CARTESIAN_POINT ( 'NONE',  ( 23.31696727199999941, 1409.831874797830096, 209.1795042131419962 ) ) ;
#5891=CARTESIAN_POINT ( 'NONE',  ( 15.10371975099999986, 1409.440493903229935, 192.9533947891980006 ) ) ;
#5892=CARTESIAN_POINT ( 'NONE',  ( -15.36992167882205429, 1486.076716614789348, 186.5633141537735753 ) ) ;
#5894=EDGE_LOOP ( 'NONE', ( #57752, #110494, #17510, #35887 ) ) ;
#5896=EDGE_CURVE ( 'NONE', #9209, #75410, #40698, .T. ) ;
#5897=CARTESIAN_POINT ( 'NONE',  ( 17.52111108772825432, 1410.887420319047806, 225.4767960855723743 ) ) ;
#5899=CARTESIAN_POINT ( 'NONE',  ( -10.80134480061119895, 1446.564900598669965, 153.0805715986579969 ) ) ;
#5900=CARTESIAN_POINT ( 'NONE',  ( 18.80339027203730140, 1425.953307585449693, 225.0197318394450008 ) ) ;
#5901=CARTESIAN_POINT ( 'NONE',  ( -7.121584071090000023, 1409.161751583130126, 195.9581075130980139 ) ) ;
#5907=CARTESIAN_POINT ( 'NONE',  ( 10.16550028177676168, 1422.464185489443253, 137.0999999980980988 ) ) ;
#5910=CARTESIAN_POINT ( 'NONE',  ( -13.58256619105009477, 1416.843574567863016, 221.9093686888480192 ) ) ;
#5912=CARTESIAN_POINT ( 'NONE',  ( 0.08876556219990000551, 1487.215267144130166, 230.3027642732979814 ) ) ;
#5914=B_SPLINE_CURVE_WITH_KNOTS ( 'NONE', 5,
 ( #57432, #99384, #84251, #41702, #109469, #14833, #91558, #74228, #110012, #49022, #108358, #101037, #92647, #22660, #58518, #56862, #14282, #82610 ),
 .UNSPECIFIED., .F., .F.,
 ( 6, 3, 3, 3, 3, 6 ),
 ( 14.02535798500000119, 16.90079360149999843, 18.14364336469999728, 21.12354018079999918, 24.53920724549999832, 25.26141249534510180 ),
 .UNSPECIFIED. ) ;
#5915=CARTESIAN_POINT ( 'NONE',  ( 22.79799990230000262, 1450.565005821530121, 218.5548369444179855 ) ) ;
#5920=CARTESIAN_POINT ( 'NONE',  ( 15.57895570635746729, 1420.991873654417759, 227.6562969275110504 ) ) ;
#5921=CARTESIAN_POINT ( 'NONE',  ( 5.250757762980000187, 1425.396628029330259, 185.7731830333980270 ) ) ;
#5922=CARTESIAN_POINT ( 'NONE',  ( -19.53581944440000129, 1426.498310938329951, 223.6168261148980037 ) ) ;
#5923=CARTESIAN_POINT ( 'NONE',  ( -24.39260298050000131, 1436.577174086429977, 139.3086241096980018 ) ) ;
#5925=CARTESIAN_POINT ( 'NONE',  ( 18.05311534039999799, 1478.533517822129852, 189.4273905463979872 ) ) ;
#5927=CARTESIAN_POINT ( 'NONE',  ( -29.81576564734521995, 1462.384100490245146, 269.4688546054820790 ) ) ;
#5928=ORIENTED_EDGE ( 'NONE', *, *, #77821, .F. ) ;
#5930=CARTESIAN_POINT ( 'NONE',  ( -40.87222264588623943, 1425.533548234441241, 269.1063209156467906 ) ) ;
#5932=CARTESIAN_POINT ( 'NONE',  ( -11.16733641199999916, 1453.313060387329870, 225.4924597496980141 ) ) ;
#5933=CARTESIAN_POINT ( 'NONE',  ( -0.1157347679000000074, 1416.431691060530056, 233.7196346762979999 ) ) ;
#5934=CARTESIAN_POINT ( 'NONE',  ( -12.92866756046528742, 1442.907176575177346, 186.4521622979591768 ) ) ;
#5935=ADVANCED_FACE ( 'NONE', ( #89792 ), #107701, .T. ) ;
#5938=CARTESIAN_POINT ( 'NONE',  ( -0.8307656363412412315, 1415.466171952180275, 233.3157467582985305 ) ) ;
#5940=CARTESIAN_POINT ( 'NONE',  ( 23.84671661830000033, 1435.330256084430175, 136.8235927701979904 ) ) ;
#5941=CARTESIAN_POINT ( 'NONE',  ( -12.57626553825837057, 1442.780697748498824, 169.4711281103210183 ) ) ;
#5943=CARTESIAN_POINT ( 'NONE',  ( -15.10371725490000117, 1409.440493816029857, 225.2902966875980155 ) ) ;
#5944=ORIENTED_EDGE ( 'NONE', *, *, #12567, .F. ) ;
#5948=ORIENTED_EDGE ( 'NONE', *, *, #35114, .T. ) ;
#5952=CARTESIAN_POINT ( 'NONE',  ( -7.835336891880000820, 1460.591301111030134, 220.7785084851980173 ) ) ;
#5954=CARTESIAN_POINT ( 'NONE',  ( -11.10223665490000045, 1433.397901385839987, 151.6819397502979712 ) ) ;
#5957=CARTESIAN_POINT ( 'NONE',  ( 33.91369110979999846, 1435.681798629080049, 135.0664268281979901 ) ) ;
#5958=CARTESIAN_POINT ( 'NONE',  ( -14.15746895765553148, 1429.524163386080772, 222.2892373711416667 ) ) ;
#5960=CARTESIAN_POINT ( 'NONE',  ( 1.131674255589999900, 1451.349625404129938, 182.9318192675980299 ) ) ;
#5962=CARTESIAN_POINT ( 'NONE',  ( -11.10591547028436210, 1509.425967423228713, 236.9904550492935869 ) ) ;
#5963=CARTESIAN_POINT ( 'NONE',  ( 1.012732680628119953E-08, 1406.631737762240164, 265.7406131533139728 ) ) ;
#5965=EDGE_LOOP ( 'NONE', ( #80360, #67781, #4261, #92596 ) ) ;
#5966=CARTESIAN_POINT ( 'NONE',  ( -11.86416350221509930, 1432.200641232820089, 149.9806832619509862 ) ) ;
#5968=CARTESIAN_POINT ( 'NONE',  ( -7.320734367630000072, 1471.591706303030151, 270.0738322358980099 ) ) ;
#5971=CARTESIAN_POINT ( 'NONE',  ( 37.04734811236939862, 1450.866104830520044, 135.5959735071040200 ) ) ;
#5972=CARTESIAN_POINT ( 'NONE',  ( 0.2217422282631729968, 1451.716230971589766, 182.8672561695299805 ) ) ;
#5977=CARTESIAN_POINT ( 'NONE',  ( -43.82815393974300378, 1429.932399413429948, 268.2833890840869913 ) ) ;
#5978=ORIENTED_EDGE ( 'NONE', *, *, #61644, .T. ) ;
#5979=CARTESIAN_POINT ( 'NONE',  ( -3.533055825017940244, 1491.511335076580053, 181.6418872453359938 ) ) ;
#5984=CARTESIAN_POINT ( 'NONE',  ( 3.118627138969999990, 1507.020746158230168, 237.9289388427980043 ) ) ;
#5986=CARTESIAN_POINT ( 'NONE',  ( -14.38276615813130022, 1509.537722091349906, 182.7943691049900110 ) ) ;
#5987=CARTESIAN_POINT ( 'NONE',  ( -2.722115699650000220, 1440.429139517749945, 185.2447042016979992 ) ) ;
#5988=CARTESIAN_POINT ( 'NONE',  ( -2.147779505350395191, 1450.027952981308999, 182.8955025268928978 ) ) ;
#5989=ORIENTED_EDGE ( 'NONE', *, *, #43929, .F. ) ;
#5990=CARTESIAN_POINT ( 'NONE',  ( -26.59118184279999753, 1435.506208013240212, 135.8223177419979777 ) ) ;
#5992=CARTESIAN_POINT ( 'NONE',  ( -39.13294649639051670, 1449.732215464259525, 134.8602047732755693 ) ) ;
#5993=CARTESIAN_POINT ( 'NONE',  ( 1.261852030525026258, 1508.993026050927256, 238.7550003759345998 ) ) ;
#5994=CARTESIAN_POINT ( 'NONE',  ( -27.23383974134830154, 1417.435118850199842, 269.7057695636269727 ) ) ;
#5996=CARTESIAN_POINT ( 'NONE',  ( -2.560623336209999934, 1397.364455864229967, 196.3367421450979862 ) ) ;
#6000=DIRECTION ( 'NONE',  ( 0.000000000000000000, 0.000000000000000000, 1.000000000000000000 ) ) ;
#6004=CARTESIAN_POINT ( 'NONE',  ( -2.500000000000000000, 1419.383254857029897, 144.0944172368980105 ) ) ;
#6005=CARTESIAN_POINT ( 'NONE',  ( -1.465793849540000027, 1484.360957265730121, 182.4810413031979976 ) ) ;
#6007=LINE ( 'NONE', #32317, #98441 ) ;
#6010=FACE_OUTER_BOUND ( 'NONE', #25973, .T. ) ;
#6013=VERTEX_POINT ( 'NONE', #98188 ) ;
#6014=CARTESIAN_POINT ( 'NONE',  ( -33.91369117178599879, 1451.728768195329849, 134.4203408260499941 ) ) ;
#6016=CARTESIAN_POINT ( 'NONE',  ( -23.49708866447455691, 1448.323603619134701, 215.7384060670668759 ) ) ;
#6019=CARTESIAN_POINT ( 'NONE',  ( 11.99125049862840164, 1436.336701747860161, 149.2203835722019960 ) ) ;
#6020=B_SPLINE_SURFACE_WITH_KNOTS ( 'NONE', 5, 5, ( 
 ( #65952, #7125, #83277, #33404, #74355, #32331, #75454, #6575, #50779, #40724, #74896, #48595 ),
 ( #109590, #14402, #32859, #58094, #7667, #101158, #108483, #25000, #31766, #84912, #24452, #58640 ),
 ( #92773, #67599, #16049, #50252, #75979, #8205, #42372, #76527, #110678, #33970, #22790, #56995 ),
 ( #82729, #8759, #51895, #408, #104491, #60867, #59744, #52455, #26105, #103364, #94993, #60295 ),
 ( #35077, #27784, #34525, #87141, #36192, #77100, #18260, #102273, #68706, #17133, #42940, #43496 ),
 ( #86034, #102811, #44044, #44601, #25553, #85459, #69257, #77639, #93865, #53007, #61416, #95539 ),
 ( #35625, #26667, #9334, #94413, #17690, #952, #18812, #2060, #51323, #10431, #86584, #9876 ),
 ( #78183, #1493, #78744, #70376, #69820, #103938, #27236, #84183, #33229, #102617, #59009, #91493 ),
 ( #75799, #101517, #76908, #14773, #41643, #42196, #7482, #16948, #59555, #83090, #6383, #25917 ),
 ( #51150, #66320, #33776, #25363, #50055, #48959, #40531, #66865, #6926, #76347, #74707, #23720 ),
 ( #15850, #109409, #24804, #32135, #93669, #85277, #110496, #108838, #109950, #100438, #93136, #8576 ),
 ( #41083, #67418, #57906, #92040, #42746, #15312, #92578, #67972, #49505, #16404, #32685, #83630 ),
 ( #75260, #215, #50598, #34340, #102080, #68518, #58451, #100974, #24270, #84730, #8027, #35445 ),
 ( #72774, #78558, #51706, #104306, #86395, #10240, #36008, #9684, #43308, #52817, #38595, #60675 ),
 ( #81152, #103177, #70200, #106902, #26479, #85846, #759, #103756, #27057, #77999, #94801, #61781 ),
 ( #60115, #9145, #95357, #1305, #94233, #79126, #87518, #10807, #44977, #27597, #61243, #43852 ),
 ( #17508, #77457, #2434, #97946, #34887, #18076, #18617, #21214, #36549, #29647, #86948, #52271 ),
 ( #95905, #19166, #69633, #70746, #44416, #53372, #1874, #106361, #63834, #55423, #12845, #89556 ) ),
 .UNSPECIFIED., .F., .F., .F.,
 ( 6, 3, 3, 3, 3, 6 ),
 ( 6, 3, 3, 6 ),
 ( 8.580843589984830544, 11.93617684059999995, 16.46680586349999942, 17.68033087479999921, 18.28709338049999999, 18.73288479507320048 ),
 ( -0.0007644201731544349393, 0.4984688824269999929, 1.495406647280000056, 2.064389376412830046 ),
 .UNSPECIFIED. ) ;
#6021=CARTESIAN_POINT ( 'NONE',  ( 13.65307821729999915, 1415.140114704729967, 197.5268032949979897 ) ) ;
#6023=CARTESIAN_POINT ( 'NONE',  ( 1.704192342800000001E-13, 1475.048391919030109, 269.6500679772980220 ) ) ;
#6026=CARTESIAN_POINT ( 'NONE',  ( -0.3175620501786377559, 1506.436298853426024, 187.1391428864371846 ) ) ;
#6027=CARTESIAN_POINT ( 'NONE',  ( 24.32234920051570626, 1445.577642606156360, 214.2383469815599142 ) ) ;
#6029=CARTESIAN_POINT ( 'NONE',  ( 16.40119952638874068, 1409.652464920799048, 226.0181189573841891 ) ) ;
#6032=ORIENTED_EDGE ( 'NONE', *, *, #62416, .F. ) ;
#6035=CARTESIAN_POINT ( 'NONE',  ( 0.4933970490180000779, 1420.589273614029935, 183.4078724835979983 ) ) ;
#6038=CARTESIAN_POINT ( 'NONE',  ( 1.270728227940000066, 1414.996442546130083, 191.7853923321980005 ) ) ;
#6039=CARTESIAN_POINT ( 'NONE',  ( -0.04745950029138250315, 1508.924973538250015, 179.5474405769929831 ) ) ;
#6041=CARTESIAN_POINT ( 'NONE',  ( 2.058017575162654822, 1417.326595624436550, 233.1728886830721876 ) ) ;
#6042=CARTESIAN_POINT ( 'NONE',  ( 17.98726295721315793, 1424.120998220819729, 225.5226115392007955 ) ) ;
#6044=EDGE_CURVE ( 'NONE', #52345, #89175, #4689, .T. ) ;
#6045=CARTESIAN_POINT ( 'NONE',  ( -5.311472889528250303E-07, 1407.436814443840149, 222.1874709566379806 ) ) ;
#6046=CARTESIAN_POINT ( 'NONE',  ( 33.71363641244969500, 1440.913060384090159, 248.2283521579210230 ) ) ;
#6049=CARTESIAN_POINT ( 'NONE',  ( -0.3788333198289999815, 1408.926289538330138, 186.6322588406980003 ) ) ;
#6053=CARTESIAN_POINT ( 'NONE',  ( -19.79281846730729200, 1484.923549257670402, 190.6224826566608783 ) ) ;
#6056=CARTESIAN_POINT ( 'NONE',  ( -2.500000000000000000, 1419.383100980419840, 144.1003751433630100 ) ) ;
#6062=CARTESIAN_POINT ( 'NONE',  ( -14.87725549029999961, 1489.466917449729863, 192.6664679402979914 ) ) ;
#6067=CARTESIAN_POINT ( 'NONE',  ( -1.376413794940000157, 1450.856769977960084, 182.9787630389979824 ) ) ;
#6070=ORIENTED_EDGE ( 'NONE', *, *, #83645, .T. ) ;
#6071=EDGE_LOOP ( 'NONE', ( #100719, #67842, #79528, #86986 ) ) ;
#6076=AXIS2_PLACEMENT_3D ( 'NONE', #20156, #36966, #71157 ) ;
#6081=CARTESIAN_POINT ( 'NONE',  ( 4.258779903668019173, 1409.061780258630051, 194.7559829868740167 ) ) ;
#6082=CARTESIAN_POINT ( 'NONE',  ( 18.28847123799999963, 1425.325025442230071, 225.4709929694980133 ) ) ;
#6087=CARTESIAN_POINT ( 'NONE',  ( -3.617662457638250117, 1448.976550491250009, 184.9371969260439812 ) ) ;
#6088=ORIENTED_EDGE ( 'NONE', *, *, #32338, .T. ) ;
#6090=CARTESIAN_POINT ( 'NONE',  ( -8.593470627377898907, 1428.030732904877141, 134.0999999980980135 ) ) ;
#6091=CARTESIAN_POINT ( 'NONE',  ( 14.29468422029999886, 1410.759725256029924, 191.3977978341980020 ) ) ;
#6093=CARTESIAN_POINT ( 'NONE',  ( -20.37362044233400127, 1500.532225497879836, 190.6021518776060191 ) ) ;
#6098=CARTESIAN_POINT ( 'NONE',  ( -19.28416521189999955, 1426.095206623730064, 225.9565170197979853 ) ) ;
#6099=CARTESIAN_POINT ( 'NONE',  ( -20.76266710848580033, 1464.825012654529928, 208.5383817516119791 ) ) ;
#6101=CARTESIAN_POINT ( 'NONE',  ( 2.930076095445649731, 1409.015380899219963, 223.9343627405490054 ) ) ;
#6105=ORIENTED_EDGE ( 'NONE', *, *, #97262, .T. ) ;
#6106=CARTESIAN_POINT ( 'NONE',  ( -4.212364877099999840E-09, 1416.130848190830193, 240.4142140047979694 ) ) ;
#6107=CARTESIAN_POINT ( 'NONE',  ( -28.11157287190000176, 1508.133875831329760, 208.0042757565580018 ) ) ;
#6108=CARTESIAN_POINT ( 'NONE',  ( 1.469976146670000094, 1486.449623437230002, 182.0144994357980011 ) ) ;
#6110=CARTESIAN_POINT ( 'NONE',  ( -13.69364981090000022, 1418.910360879329801, 238.2645903702979808 ) ) ;
#6111=CYLINDRICAL_SURFACE ( 'NONE', #8919, 1.999999999999915179 ) ;
#6112=CARTESIAN_POINT ( 'NONE',  ( -21.42407812907550024, 1452.164915093389936, 141.3791819868360164 ) ) ;
#6113=CARTESIAN_POINT ( 'NONE',  ( -18.96350866050000050, 1416.837080243330092, 208.0006276345779952 ) ) ;
#6117=CARTESIAN_POINT ( 'NONE',  ( 15.82007826961449837, 1421.163257332559851, 227.5271101461229932 ) ) ;
#6122=CARTESIAN_POINT ( 'NONE',  ( -22.80833251699839792, 1409.709435844829841, 209.2324790707910154 ) ) ;
#6123=CARTESIAN_POINT ( 'NONE',  ( -3.961468203580000402, 1423.998250314630013, 184.1718454746980171 ) ) ;
#6126=CARTESIAN_POINT ( 'NONE',  ( -6.895798589700000925, 1507.635187917330086, 235.7209506179980281 ) ) ;
#6127=CARTESIAN_POINT ( 'NONE',  ( -22.76667043220000153, 1415.847673962129875, 211.9494722144779928 ) ) ;
#6130=CARTESIAN_POINT ( 'NONE',  ( 46.04304765074009964, 1443.742661411660038, 266.9755472754490029 ) ) ;
#6131=CARTESIAN_POINT ( 'NONE',  ( -1.126474399395450021, 1424.149452017869862, 228.3764236718020015 ) ) ;
#6132=CARTESIAN_POINT ( 'NONE',  ( 0.01346536989209999938, 1420.212931417629989, 183.8948729780979932 ) ) ;
#6134=ORIENTED_EDGE ( 'NONE', *, *, #58907, .T. ) ;
#6137=CARTESIAN_POINT ( 'NONE',  ( 12.53380745427929988, 1442.773887455719887, 186.4115735415020083 ) ) ;
#6139=VERTEX_POINT ( 'NONE', #90331 ) ;
#6141=FACE_OUTER_BOUND ( 'NONE', #107255, .T. ) ;
#6143=CARTESIAN_POINT ( 'NONE',  ( 1.364635942960239934, 1452.865406250129809, 152.5018568859900085 ) ) ;
#6145=CARTESIAN_POINT ( 'NONE',  ( 16.93202667939999984, 1409.669517366430000, 192.7683719188979978 ) ) ;
#6150=PLANE ( 'NONE',  #12439 ) ;
#6151=CARTESIAN_POINT ( 'NONE',  ( -13.55647141870050021, 1434.955288304769965, 148.7473005004320044 ) ) ;
#6156=CARTESIAN_POINT ( 'NONE',  ( 7.214502255410000231, 1427.316505021429975, 144.1938086916980239 ) ) ;
#6158=CARTESIAN_POINT ( 'NONE',  ( 21.37693747720000204, 1440.913060387330006, 224.8635562088979896 ) ) ;
#6168=CARTESIAN_POINT ( 'NONE',  ( 4.122931283589999374E-15, 1438.194204504490017, 150.6035180695979818 ) ) ;
#6169=CARTESIAN_POINT ( 'NONE',  ( -13.58245609809999976, 1416.835809823829777, 221.9090836517979994 ) ) ;
#6170=CARTESIAN_POINT ( 'NONE',  ( 11.35166415849999844, 1433.891578315870220, 151.4717738640979974 ) ) ;
#6172=CARTESIAN_POINT ( 'NONE',  ( 31.32742178679999512, 1440.913060387330006, 255.3819207742980097 ) ) ;
#6178=CARTESIAN_POINT ( 'NONE',  ( -18.15222296039999961, 1485.954920948629933, 188.9255103041979851 ) ) ;
#6180=CARTESIAN_POINT ( 'NONE',  ( 18.64588652299999794, 1416.828040475229955, 209.6843149956849857 ) ) ;
#6185=CARTESIAN_POINT ( 'NONE',  ( 12.61594199600000188, 1416.825532269230052, 223.3236178109980017 ) ) ;
#6186=CARTESIAN_POINT ( 'NONE',  ( 11.21621798026153449, 1434.249418731722926, 151.6036331528934795 ) ) ;
#6187=CARTESIAN_POINT ( 'NONE',  ( -9.959882553640550640, 1432.347050749440086, 152.5237167886959924 ) ) ;
#6188=CARTESIAN_POINT ( 'NONE',  ( 14.03757890547870169, 1511.404489521279856, 234.8174622444540205 ) ) ;
#6189=CIRCLE ( 'NONE', #31215, 1.999999999914150450 ) ;
#6190=CARTESIAN_POINT ( 'NONE',  ( 0.2102264332707180217, 1457.221076095949911, 183.0723111843419986 ) ) ;
#6193=CARTESIAN_POINT ( 'NONE',  ( -12.93811130839999812, 1444.994950788469851, 169.4238961894979809 ) ) ;
#6194=CARTESIAN_POINT ( 'NONE',  ( -28.74510110280450093, 1509.809709161739875, 211.3508879095350039 ) ) ;
#6195=CARTESIAN_POINT ( 'NONE',  ( 11.87523146630000070, 1433.007068934590052, 149.1894884818979676 ) ) ;
#6196=CARTESIAN_POINT ( 'NONE',  ( -39.90438676673540641, 1438.693166632869861, 134.0999999980629980 ) ) ;
#6203=EDGE_CURVE ( 'NONE', #22181, #59085, #97210, .T. ) ;
#6205=CARTESIAN_POINT ( 'NONE',  ( 31.98568811499627529, 1416.535344689362319, 269.3160153020001530 ) ) ;
#6208=CARTESIAN_POINT ( 'NONE',  ( 3.906311210379999732, 1428.753781860530125, 185.1730557025980204 ) ) ;
#6211=CARTESIAN_POINT ( 'NONE',  ( -26.79977994216764259, 1436.581364966177944, 136.7606519021615554 ) ) ;
#6213=CARTESIAN_POINT ( 'NONE',  ( -28.86205551545040038, 1509.507027965300040, 208.7152694674689997 ) ) ;
#6214=CARTESIAN_POINT ( 'NONE',  ( -16.29200499093240140, 1410.123450363890015, 226.4300118576410057 ) ) ;
#6215=CARTESIAN_POINT ( 'NONE',  ( 0.5077272017738569954, 1412.024639619329946, 184.9986638035829856 ) ) ;
#6217=CARTESIAN_POINT ( 'NONE',  ( -27.68254001883949655, 1507.989615300039986, 210.5775529569929745 ) ) ;
#6220=CARTESIAN_POINT ( 'NONE',  ( 21.03123271209999956, 1507.789097944330024, 226.0655642189979915 ) ) ;
#6223=CARTESIAN_POINT ( 'NONE',  ( 0.2597461834470000119, 1465.026886499829970, 237.7737181796979939 ) ) ;
#6224=CARTESIAN_POINT ( 'NONE',  ( 18.72649884289999989, 1410.063202272829813, 221.6652856211979952 ) ) ;
#6225=CARTESIAN_POINT ( 'NONE',  ( -17.98886881720000019, 1424.630730734530061, 227.7167155485979890 ) ) ;
#6229=CARTESIAN_POINT ( 'NONE',  ( 23.60905104348515593, 1509.747275849248581, 191.3746876935084060 ) ) ;
#6230=CARTESIAN_POINT ( 'NONE',  ( -0.4792592228059999737, 1416.456888389930100, 233.6761958929980096 ) ) ;
#6234=CARTESIAN_POINT ( 'NONE',  ( -8.629181194863379645, 1486.004047916040008, 183.3125379289229784 ) ) ;
#6237=CARTESIAN_POINT ( 'NONE',  ( 14.23445134770000031, 1463.710773101130144, 224.1807475960980298 ) ) ;
#6238=CARTESIAN_POINT ( 'NONE',  ( -4.224005846046000379, 1441.584137753169898, 166.8519868219619866 ) ) ;
#6242=ORIENTED_EDGE ( 'NONE', *, *, #109065, .T. ) ;
#6244=ORIENTED_EDGE ( 'NONE', *, *, #52966, .T. ) ;
#6246=EDGE_CURVE ( 'NONE', #62909, #101516, #66511, .T. ) ;
#6247=CARTESIAN_POINT ( 'NONE',  ( -20.32611051789999834, 1410.902622711730146, 198.7319329392979910 ) ) ;
#6248=CARTESIAN_POINT ( 'NONE',  ( -11.64413779052331854, 1425.860397285439376, 144.6913732887203992 ) ) ;
#6249=CARTESIAN_POINT ( 'NONE',  ( 16.18216864280910272, 1410.860672406080084, 191.5684563615119771 ) ) ;
#6250=ADVANCED_FACE ( 'NONE', ( #28659 ), #45487, .F. ) ;
#6252=CARTESIAN_POINT ( 'NONE',  ( 37.53898081716540247, 1436.541061908490065, 135.4800556696710032 ) ) ;
#6254=CARTESIAN_POINT ( 'NONE',  ( -11.73648056819999930, 1426.280364960429779, 144.1673147898980005 ) ) ;
#6257=CARTESIAN_POINT ( 'NONE',  ( 15.10766868565390730, 1461.886987926997563, 229.9399717845676605 ) ) ;
#6260=CARTESIAN_POINT ( 'NONE',  ( 34.74890047445369845, 1451.658442319180040, 134.0999999982409747 ) ) ;
#6261=CARTESIAN_POINT ( 'NONE',  ( 5.343479918049999888, 1396.099658817830004, 218.7752541424879951 ) ) ;
#6263=CARTESIAN_POINT ( 'NONE',  ( -18.76032074160000107, 1456.949267706729870, 228.3571107660980033 ) ) ;
#6269=CARTESIAN_POINT ( 'NONE',  ( 0.1579620925989999869, 1450.907544229120049, 181.8932541306980113 ) ) ;
#6272=CARTESIAN_POINT ( 'NONE',  ( -41.14066433057620031, 1444.183247621620012, 136.8991340826939904 ) ) ;
#6273=CARTESIAN_POINT ( 'NONE',  ( 40.71747596589879947, 1448.637563225589929, 134.7402674100779905 ) ) ;
#6274=CARTESIAN_POINT ( 'NONE',  ( 12.78690713350000152, 1416.828040475229955, 222.7042044314979989 ) ) ;
#6276=DIRECTION ( 'NONE',  ( -0.8926073982886787439, 0.000000000000000000, 0.4508348173337058951 ) ) ;
#6278=EDGE_CURVE ( 'NONE', #50772, #11318, #43668, .T. ) ;
#6284=CARTESIAN_POINT ( 'NONE',  ( 41.33116270185299612, 1440.913060387330006, 268.8666020839340263 ) ) ;
#6285=CARTESIAN_POINT ( 'NONE',  ( -0.0006570779929211399998, 1451.938362507649117, 153.9926151582928071 ) ) ;
#6293=CARTESIAN_POINT ( 'NONE',  ( -4.405926214540000885, 1420.984874813729903, 186.2222319335980103 ) ) ;
#6295=CARTESIAN_POINT ( 'NONE',  ( 2.101979435200000079, 1406.024670839530017, 266.9594151837979439 ) ) ;
#6296=EDGE_CURVE ( 'NONE', #101169, #75664, #86348, .T. ) ;
#6298=CARTESIAN_POINT ( 'NONE',  ( 16.43421760069999848, 1460.517322140429997, 229.1132056239979704 ) ) ;
#6299=CARTESIAN_POINT ( 'NONE',  ( -11.60004869885203682, 1424.920234268488002, 136.4497806812309193 ) ) ;
#6300=CARTESIAN_POINT ( 'NONE',  ( -4.479448571171882776, 1422.019686008850385, 184.5739666799692600 ) ) ;
#6305=CARTESIAN_POINT ( 'NONE',  ( -0.8197074128579011632, 1486.333374263157339, 181.7749019119357570 ) ) ;
#6306=CARTESIAN_POINT ( 'NONE',  ( -0.1482922428603659915, 1507.522720463130099, 180.8421728092000080 ) ) ;
#6310=CARTESIAN_POINT ( 'NONE',  ( 1.632486301776860348E-07, 1509.047264794319972, 239.1218459617020073 ) ) ;
#6314=CARTESIAN_POINT ( 'NONE',  ( 25.21572900089999791, 1445.966631079429817, 221.6528564213980133 ) ) ;
#6315=CARTESIAN_POINT ( 'NONE',  ( -11.85988639909999875, 1431.881489348090099, 150.3806999221980050 ) ) ;
#6318=CARTESIAN_POINT ( 'NONE',  ( 3.199225641321900238, 1428.849793147289802, 155.3746604249230074 ) ) ;
#6320=CARTESIAN_POINT ( 'NONE',  ( 12.13323926729999869, 1445.693284459350025, 187.5259842820979941 ) ) ;
#6321=CARTESIAN_POINT ( 'NONE',  ( -22.24587359499999906, 1495.367887861130157, 224.6596000937979909 ) ) ;
#6322=CARTESIAN_POINT ( 'NONE',  ( -3.921313488591959384, 1421.968803082632803, 139.1411894385240942 ) ) ;
#6326=CARTESIAN_POINT ( 'NONE',  ( 14.64774519859999913, 1407.477793284829886, 267.7626194198979874 ) ) ;
#6327=CARTESIAN_POINT ( 'NONE',  ( -0.3074737364230000214, 1409.850186678229875, 185.0722532870979933 ) ) ;
#6330=CARTESIAN_POINT ( 'NONE',  ( 24.55543445757494325, 1439.121178053543872, 212.5561943058436327 ) ) ;
#6334=CARTESIAN_POINT ( 'NONE',  ( -12.94448954231350513, 1511.163060387329779, 185.4271167906579478 ) ) ;
#6337=CARTESIAN_POINT ( 'NONE',  ( -12.02000798989999986, 1447.120367794319918, 187.5076484450979990 ) ) ;
#6338=CARTESIAN_POINT ( 'NONE',  ( 2.314829377092709972, 1449.816261417490068, 155.0640813294609757 ) ) ;
#6339=CARTESIAN_POINT ( 'NONE',  ( -14.41907353321770024, 1416.449138231110055, 221.3520838159390109 ) ) ;
#6341=B_SPLINE_CURVE_WITH_KNOTS ( 'NONE', 5,
 ( #33615, #75658, #33077, #67812, #66174, #91887 ),
 .UNSPECIFIED., .F., .F.,
 ( 6, 6 ),
 ( 123.8981302308609997, 143.2822930469999960 ),
 .UNSPECIFIED. ) ;
#6342=CARTESIAN_POINT ( 'NONE',  ( -9.881922048573189343, 1409.258144709340058, 197.8933969988160015 ) ) ;
#6344=CARTESIAN_POINT ( 'NONE',  ( 20.59269117493390056, 1507.766073655780019, 227.7908423917359926 ) ) ;
#6345=CARTESIAN_POINT ( 'NONE',  ( 3.140603745509999989, 1440.712167354720123, 157.0498910118980120 ) ) ;
#6346=CARTESIAN_POINT ( 'NONE',  ( -3.774131035769999976, 1475.960033162130003, 267.5310482922980100 ) ) ;
#6347=CARTESIAN_POINT ( 'NONE',  ( -4.238698856969680406, 1446.369308287780086, 163.0896733719079919 ) ) ;
#6351=CARTESIAN_POINT ( 'NONE',  ( 13.58268853708210067, 1416.851343896850040, 196.3340833727469885 ) ) ;
#6352=CARTESIAN_POINT ( 'NONE',  ( 15.10371975099999986, 1409.440493903229935, 192.9533947891980006 ) ) ;
#6357=CARTESIAN_POINT ( 'NONE',  ( -18.50671984590000108, 1409.559329285129934, 198.4601733219979849 ) ) ;
#6360=CARTESIAN_POINT ( 'NONE',  ( -6.691255413100000382, 1406.996319227029971, 269.6355722701979403 ) ) ;
#6361=ORIENTED_EDGE ( 'NONE', *, *, #60271, .F. ) ;
#6364=VECTOR ( 'NONE', #90126, 1000.000000000000000 ) ;
#6367=CARTESIAN_POINT ( 'NONE',  ( 10.80393815379999900, 1424.927943689529911, 143.4644770969979959 ) ) ;
#6369=CARTESIAN_POINT ( 'NONE',  ( -15.83291935337495815, 1409.465937342200732, 225.2763755258536662 ) ) ;
#6371=ADVANCED_FACE ( 'NONE', ( #10195 ), #48224, .T. ) ;
#6372=CARTESIAN_POINT ( 'NONE',  ( 26.99540884559359810, 1450.681726017589881, 136.4489477893459934 ) ) ;
#6379=CARTESIAN_POINT ( 'NONE',  ( 21.21721392852580124, 1509.704275884970230, 230.0128098300520207 ) ) ;
#6382=ORIENTED_EDGE ( 'NONE', *, *, #9110, .F. ) ;
#6383=CARTESIAN_POINT ( 'NONE',  ( 11.40220705808729917, 1434.449209149890066, 151.4764968396059999 ) ) ;
#6384=CARTESIAN_POINT ( 'NONE',  ( -7.907916001329999389, 1397.529048966930077, 219.9234842523979978 ) ) ;
#6385=CARTESIAN_POINT ( 'NONE',  ( -18.85211735460000071, 1409.571390833930081, 221.0529096949979930 ) ) ;
#6387=CARTESIAN_POINT ( 'NONE',  ( -13.51311000297323339, 1443.997929519461877, 169.3513768787690026 ) ) ;
#6391=CARTESIAN_POINT ( 'NONE',  ( 35.00335893190000291, 1443.851131231850104, 135.3147355765980251 ) ) ;
#6392=CARTESIAN_POINT ( 'NONE',  ( -13.76157194526980021, 1508.323015833239879, 184.1190294504459928 ) ) ;
#6393=B_SPLINE_CURVE_WITH_KNOTS ( 'NONE', 3,
 ( #84558, #7847, #110312, #33587, #101892, #68345 ),
 .UNSPECIFIED., .F., .F.,
 ( 4, 2, 4 ),
 ( 0.000000000000000000, 0.4987707156545279630, 0.9977421829108459317 ),
 .UNSPECIFIED. ) ;
#6394=CARTESIAN_POINT ( 'NONE',  ( 0.1761655985929999890, 1468.710735116929982, 182.5349289889980184 ) ) ;
#6395=ADVANCED_FACE ( 'NONE', ( #72870 ), #42899, .T. ) ;
#6397=CARTESIAN_POINT ( 'NONE',  ( 42.85031101989900293, 1440.913053629049955, 270.2009481551980343 ) ) ;
#6399=CARTESIAN_POINT ( 'NONE',  ( 10.62399481180199956, 1396.284058461849781, 206.0104454596539938 ) ) ;
#6400=CARTESIAN_POINT ( 'NONE',  ( 2.500000000000000000, 1419.401689857129895, 143.2540567177979938 ) ) ;
#6401=CARTESIAN_POINT ( 'NONE',  ( 11.50749625859999981, 1427.423291567529986, 149.3076215910979840 ) ) ;
#6404=CARTESIAN_POINT ( 'NONE',  ( 13.11477892927669942, 1435.900992455230153, 150.6555893957250021 ) ) ;
#6406=VERTEX_POINT ( 'NONE', #38152 ) ;
#6408=CARTESIAN_POINT ( 'NONE',  ( -18.42347945445600033, 1478.095089849470014, 228.7109761469720013 ) ) ;
#6409=CARTESIAN_POINT ( 'NONE',  ( -12.96438286449999922, 1461.237399744029972, 232.5537136377980119 ) ) ;
#6425=CARTESIAN_POINT ( 'NONE',  ( -35.09211443864747793, 1424.151985311556473, 269.5327834166636194 ) ) ;
#6427=CARTESIAN_POINT ( 'NONE',  ( -1.027470347570780040, 1414.913060387399810, 225.5111429998570145 ) ) ;
#6429=CARTESIAN_POINT ( 'NONE',  ( -0.008271327469596450460, 1451.342692138500297, 182.5054642300370062 ) ) ;
#6430=CARTESIAN_POINT ( 'NONE',  ( -28.38246044266520229, 1440.913060387269979, 232.6696485458210191 ) ) ;
#6432=CARTESIAN_POINT ( 'NONE',  ( -0.2944423246913550063, 1465.427648891259878, 236.3065114702050096 ) ) ;
#6433=CARTESIAN_POINT ( 'NONE',  ( 6.198203255362690456, 1410.719740469389990, 269.3394747697590219 ) ) ;
#6436=CARTESIAN_POINT ( 'NONE',  ( 23.02287022260000171, 1409.743200923030145, 209.1790448026619913 ) ) ;
#6439=CIRCLE ( 'NONE', #52895, 1.999998160074185627 ) ;
#6443=CARTESIAN_POINT ( 'NONE',  ( 0.1409679171009999843, 1419.780819256630139, 184.3745687884979816 ) ) ;
#6456=CARTESIAN_POINT ( 'NONE',  ( -15.27152961130000008, 1506.433683729329914, 224.9338604266980326 ) ) ;
#6462=CARTESIAN_POINT ( 'NONE',  ( 21.97919311359999739, 1451.781877468529956, 220.8331905986980246 ) ) ;
#6466=CARTESIAN_POINT ( 'NONE',  ( 9.442266983135132463, 1417.594392525823650, 230.3524224733923802 ) ) ;
#6467=CARTESIAN_POINT ( 'NONE',  ( 39.47629592728779357, 1446.978162307669891, 136.6467521598829649 ) ) ;
#6468=CARTESIAN_POINT ( 'NONE',  ( -19.53850950879999715, 1426.169861875230026, 223.3587345906979920 ) ) ;
#6469=CARTESIAN_POINT ( 'NONE',  ( -23.03159172119999809, 1435.301732086840275, 138.5817198000980000 ) ) ;
#6471=CARTESIAN_POINT ( 'NONE',  ( 13.70990347210000060, 1507.817794156229866, 185.7059265823980070 ) ) ;
#6473=CARTESIAN_POINT ( 'NONE',  ( 8.410267065803780360E-17, 1471.436294031830130, 269.3346704751489824 ) ) ;
#6475=CARTESIAN_POINT ( 'NONE',  ( 2.446787376320000096, 1432.353341358199941, 150.2884730787980061 ) ) ;
#6476=CARTESIAN_POINT ( 'NONE',  ( -42.13563646669874885, 1427.775737239709770, 269.0721146450511583 ) ) ;
#6478=CARTESIAN_POINT ( 'NONE',  ( -10.03739716579999808, 1408.913060387329779, 223.8190696839980092 ) ) ;
#6479=CARTESIAN_POINT ( 'NONE',  ( -15.52964687406499955, 1451.324136384999974, 222.4830579234560162 ) ) ;
#6480=CARTESIAN_POINT ( 'NONE',  ( -12.78293219662820057, 1442.837713915257837, 186.2730944851466575 ) ) ;
#6482=CARTESIAN_POINT ( 'NONE',  ( 11.86629848900230044, 1432.349867578880094, 149.9824231379060109 ) ) ;
#6483=CARTESIAN_POINT ( 'NONE',  ( -0.4967073565345429542, 1415.438070636819930, 233.3911243540180180 ) ) ;
#6486=CARTESIAN_POINT ( 'NONE',  ( -12.68854658940551339, 1442.806680916267851, 169.4609767598299470 ) ) ;
#6487=CARTESIAN_POINT ( 'NONE',  ( 18.80462376713409967, 1425.802750969149884, 225.5973978925190124 ) ) ;
#6490=CARTESIAN_POINT ( 'NONE',  ( 1.457047359303009992, 1414.913057819779851, 191.9717114511999796 ) ) ;
#6491=CARTESIAN_POINT ( 'NONE',  ( -3.314356077729999406, 1409.028800251930079, 230.9273595247980211 ) ) ;
#6494=CARTESIAN_POINT ( 'NONE',  ( 18.09118544614330304, 1416.225364278609959, 209.2081609163089979 ) ) ;
#6496=CARTESIAN_POINT ( 'NONE',  ( -11.65615920360559699, 1428.981702016564896, 138.1374390033664383 ) ) ;
#6497=CARTESIAN_POINT ( 'NONE',  ( -25.01541332120000050, 1440.913060508280068, 216.4497915762179900 ) ) ;
#6499=CARTESIAN_POINT ( 'NONE',  ( -11.19195527129999945, 1433.382885624610026, 151.6055787587979751 ) ) ;
#6501=CARTESIAN_POINT ( 'NONE',  ( 25.71166857904860237, 1449.089649366449976, 209.5200665649139751 ) ) ;
#6502=CARTESIAN_POINT ( 'NONE',  ( -25.20182348799999872, 1437.586142492700219, 138.0414809568979990 ) ) ;
#6503=CARTESIAN_POINT ( 'NONE',  ( -14.06820649347891283, 1429.461423307730911, 222.2989188825169151 ) ) ;
#6505=CARTESIAN_POINT ( 'NONE',  ( 2.325461800109999810, 1451.292411637130044, 183.5656961689980164 ) ) ;
#6507=CARTESIAN_POINT ( 'NONE',  ( -29.04773278458495156, 1510.038324495063989, 216.6204971033638458 ) ) ;
#6513=CARTESIAN_POINT ( 'NONE',  ( -11.79189761063040010, 1427.869643660999827, 147.7507972342360176 ) ) ;
#6515=CARTESIAN_POINT ( 'NONE',  ( -7.260537799720000685, 1471.133396844229992, 269.6205813391980541 ) ) ;
#6518=CARTESIAN_POINT ( 'NONE',  ( 36.71369698479820443, 1450.233298359589753, 136.1820598115060079 ) ) ;
#6519=CARTESIAN_POINT ( 'NONE',  ( 10.70848634212536865, 1506.855035729306792, 228.7236287190453936 ) ) ;
#6520=EDGE_CURVE ( 'NONE', #59778, #88595, #51471, .T. ) ;
#6525=CARTESIAN_POINT ( 'NONE',  ( -27.32593768275089730, 1412.870037644089962, 266.6661490471050229 ) ) ;
#6527=EDGE_CURVE ( 'NONE', #96120, #48466, #17462, .T. ) ;
#6528=ORIENTED_EDGE ( 'NONE', *, *, #97271, .T. ) ;
#6531=ORIENTED_EDGE ( 'NONE', *, *, #24347, .F. ) ;
#6534=CARTESIAN_POINT ( 'NONE',  ( 38.51619765980534993, 1444.740067931809790, 136.9081133514089288 ) ) ;
#6538=CARTESIAN_POINT ( 'NONE',  ( -18.34539076389999934, 1455.459263898130075, 190.6407490677979979 ) ) ;
#6539=EDGE_CURVE ( 'NONE', #47514, #19483, #6393, .T. ) ;
#6542=CARTESIAN_POINT ( 'NONE',  ( -26.29952725040000061, 1435.947996908099867, 136.5136938088979832 ) ) ;
#6543=( BOUNDED_SURFACE ( )  B_SPLINE_SURFACE ( 4, 2, ( 
 ( #68361, #15685, #60504, #24639, #102467, #58837, #42581 ),
 ( #596, #92972, #76733, #33604, #94627, #84023, #43688 ),
 ( #110332, #45, #25757, #17341, #69465, #16245, #49891 ),
 ( #84574, #51536, #68915, #7866, #67800, #101909, #59404 ),
 ( #93516, #35841, #96859, #12273, #80043, #104689, #95740 ) ),
 .UNSPECIFIED., .F., .F., .F. ) 
 B_SPLINE_SURFACE_WITH_KNOTS ( ( 5, 5 ),
 ( 3, 2, 2, 3 ),
 ( 1.967616199060000071, 3.613988937050000239 ),
 ( 11.46118682297159985, 11.46128530315550087, 12.56637061435916003, 12.57442343279920038 ),
 .UNSPECIFIED. ) 
 GEOMETRIC_REPRESENTATION_ITEM ( )  RATIONAL_B_SPLINE_SURFACE ( (
 ( 0.8778316440755170591, 0.8778241674203509648, 0.8778166930676719604, 0.7939440089458740246, 1.000000000000000000, 0.9984984584740950186, 0.9970123125040389889),
 ( 0.8778316440755170591, 0.8778241674203509648, 0.8778166930676719604, 0.7939440089458740246, 1.000000000000000000, 0.9984984584740950186, 0.9970123125040389889),
 ( 0.8778316440755170591, 0.8778241674203509648, 0.8778166930676719604, 0.7939440089458740246, 1.000000000000000000, 0.9984984584740950186, 0.9970123125040389889),
 ( 0.8778316440755170591, 0.8778241674203509648, 0.8778166930676719604, 0.7939440089458740246, 1.000000000000000000, 0.9984984584740950186, 0.9970123125040389889),
 ( 0.8778316440755170591, 0.8778241674203509648, 0.8778166930676719604, 0.7939440089458740246, 1.000000000000000000, 0.9984984584740950186, 0.9970123125040389889) ) ) 
 REPRESENTATION_ITEM ( '' )  SURFACE ( )  );
#6546=CARTESIAN_POINT ( 'NONE',  ( 1.546869376546317509, 1416.835807149388984, 190.2224235154945404 ) ) ;
#6548=CARTESIAN_POINT ( 'NONE',  ( -33.44468239324360326, 1421.725958844539946, 269.5026010579289846 ) ) ;
#6550=CARTESIAN_POINT ( 'NONE',  ( -5.086423039969999671, 1397.753029223729982, 197.0860517657980040 ) ) ;
#6551=FACE_OUTER_BOUND ( 'NONE', #65063, .T. ) ;
#6552=ORIENTED_EDGE ( 'NONE', *, *, #48270, .F. ) ;
#6554=CARTESIAN_POINT ( 'NONE',  ( -11.86629850686009924, 1432.349867577580198, 149.9824227077560010 ) ) ;
#6557=CARTESIAN_POINT ( 'NONE',  ( -23.69417716570000110, 1435.324924696049948, 137.3225688245979654 ) ) ;
#6558=CARTESIAN_POINT ( 'NONE',  ( -24.37286542989999916, 1441.888782162479856, 211.3878437502879990 ) ) ;
#6562=CARTESIAN_POINT ( 'NONE',  ( -2.825590008402790065, 1484.262936871399916, 183.3074027492610298 ) ) ;
#6565=CARTESIAN_POINT ( 'NONE',  ( 3.034663161748390348, 1440.440203176670138, 157.2490260270419924 ) ) ;
#6569=CARTESIAN_POINT ( 'NONE',  ( -33.91369117178599879, 1435.681798755369982, 134.4203392960459951 ) ) ;
#6571=( BOUNDED_CURVE ( )  B_SPLINE_CURVE ( 3, ( #57163, #58252, #16206, #92373 ),
 .UNSPECIFIED., .F., .T. ) 
 B_SPLINE_CURVE_WITH_KNOTS ( ( 4, 4 ),
 ( 5.307843187739740287, 5.956424869281669920 ),
 .UNSPECIFIED. ) 
 CURVE ( )  GEOMETRIC_REPRESENTATION_ITEM ( )  RATIONAL_B_SPLINE_CURVE ( ( 1.000000000000000000, 0.9652512859188302485, 0.9652512859188302485, 1.000000000000000000 ) ) 
 REPRESENTATION_ITEM ( '' )  );
#6575=CARTESIAN_POINT ( 'NONE',  ( 13.01189198590000018, 1435.390145910219871, 150.4640032787939958 ) ) ;
#6576=CARTESIAN_POINT ( 'NONE',  ( 14.15566883900000050, 1416.254459047329874, 196.5762094978979917 ) ) ;
#6577=CARTESIAN_POINT ( 'NONE',  ( 17.55898010899999662, 1488.218443485430043, 189.1283882809980241 ) ) ;
#6578=CARTESIAN_POINT ( 'NONE',  ( -11.44789780662239664, 1425.801310437136181, 139.0691777563419578 ) ) ;
#6579=CARTESIAN_POINT ( 'NONE',  ( 3.933438035067677863, 1449.506699156169361, 184.2458349000845601 ) ) ;
#6582=CARTESIAN_POINT ( 'NONE',  ( 24.58878164341058792, 1443.302558083091526, 213.0807573783872613 ) ) ;
#6583=CARTESIAN_POINT ( 'NONE',  ( 41.66793168306197259, 1443.219043443782311, 135.6262769008947089 ) ) ;
#6584=CARTESIAN_POINT ( 'NONE',  ( -1.835536242490369840, 1450.383119622699951, 182.7750508701979868 ) ) ;
#6593=CARTESIAN_POINT ( 'NONE',  ( 1.810458008787178885, 1416.704060343818810, 232.7176022638104200 ) ) ;
#6594=CARTESIAN_POINT ( 'NONE',  ( 17.47617717604931542, 1422.886529812959225, 226.4807061310582128 ) ) ;
#6597=CARTESIAN_POINT ( 'NONE',  ( 35.65332322675680388, 1440.913060386850020, 252.2033051962219758 ) ) ;
#6600=CARTESIAN_POINT ( 'NONE',  ( 13.07088740030000018, 1426.021987528729824, 222.4234160755980270 ) ) ;
#6602=VERTEX_POINT ( 'NONE', #79848 ) ;
#6606=CARTESIAN_POINT ( 'NONE',  ( 16.06428792994640276, 1414.913060387329779, 208.9262477894010033 ) ) ;
#6609=DIRECTION ( 'NONE',  ( 0.000000000000000000, 0.000000000000000000, 1.000000000000000000 ) ) ;
#6613=CARTESIAN_POINT ( 'NONE',  ( 24.63041548480000031, 1451.910759679029979, 137.3284484590980128 ) ) ;
#6620=CARTESIAN_POINT ( 'NONE',  ( 19.84207428532359785, 1508.528044499219959, 229.4304224270640020 ) ) ;
#6622=ORIENTED_EDGE ( 'NONE', *, *, #97190, .T. ) ;
#6623=AXIS2_PLACEMENT_3D ( 'NONE', #82180, #66521, #22801 ) ;
#6625=CARTESIAN_POINT ( 'NONE',  ( 35.12919938944479270, 1437.169777039490100, 136.5372291599819903 ) ) ;
#6632=CARTESIAN_POINT ( 'NONE',  ( 12.30091743380850033, 1409.342617889579969, 200.6317861282630020 ) ) ;
#6633=CARTESIAN_POINT ( 'NONE',  ( 18.80464347163499994, 1425.799926482960018, 225.6082800063759919 ) ) ;
#6636=CARTESIAN_POINT ( 'NONE',  ( -2.499999999569840092, 1440.150708319569958, 165.1395380847510239 ) ) ;
#6637=AXIS2_PLACEMENT_3D ( 'NONE', #26441, #68481, #35406 ) ;
#6638=CARTESIAN_POINT ( 'NONE',  ( -2.933306627113769771, 1448.953742279190010, 184.4303279486910014 ) ) ;
#6639=EDGE_LOOP ( 'NONE', ( #92995, #5708, #96221, #76584 ) ) ;
#6641=CARTESIAN_POINT ( 'NONE',  ( 18.62804149895199757, 1457.295705444719943, 227.7225047233159785 ) ) ;
#6642=CARTESIAN_POINT ( 'NONE',  ( -12.65123529389999923, 1435.857297067140053, 150.8939753325980178 ) ) ;
#6643=B_SPLINE_CURVE_WITH_KNOTS ( 'NONE', 3,
 ( #82689, #46909, #31169, #98380, #72649, #20552, #30630, #54756, #64818, #65358, #3810, #12728, #81032, #22744, #12170, #63175, #106236, #46360, #98926, #48552, #22196, #55303, #4341, #106774, #28987, #37941, #80495, #99466, #29522, #63713, #97823, #56948, #64256, #91077, #5979, #105705, #21101, #89437, #30065, #21651, #55859, #89978, #13252 ),
 .UNSPECIFIED., .F., .F.,
 ( 4, 3, 3, 3, 3, 3, 3, 3, 3, 3, 3, 3, 3, 3, 4 ),
 ( 31.69285774156780278, 33.86896628700200296, 36.91232095655669809, 39.42219942477719741, 41.51453054943480225, 43.42754320367789944, 45.18198672082530010, 46.87502985914650111, 48.51047212527600294, 50.14591439140560425, 51.70904730156200202, 53.35035321201050351, 55.10040584591209978, 57.14372345036669998, 60.99056492696890075 ),
 .UNSPECIFIED. ) ;
#6644=CARTESIAN_POINT ( 'NONE',  ( -1.176169269157790113E-08, 1473.984312740150017, 263.3285085788550077 ) ) ;
#6645=EDGE_CURVE ( 'NONE', #16155, #63851, #24999, .T. ) ;
#6646=CARTESIAN_POINT ( 'NONE',  ( 20.51827461483625825, 1436.445738427861443, 144.8727729820485592 ) ) ;
#6647=CARTESIAN_POINT ( 'NONE',  ( 3.500000000000000000, 1407.163060387330006, 146.1721969590979882 ) ) ;
#6652=CARTESIAN_POINT ( 'NONE',  ( 14.00200617152209936, 1509.378643023580025, 234.5785651225629636 ) ) ;
#6655=CARTESIAN_POINT ( 'NONE',  ( 5.805057908697529356, 1409.115777476449921, 223.0048059185109821 ) ) ;
#6656=CIRCLE ( 'NONE', #42383, 1.500000000000001332 ) ;
#6657=CARTESIAN_POINT ( 'NONE',  ( 8.902411381149999414, 1424.022968669029979, 122.9077991975980098 ) ) ;
#6660=EDGE_CURVE ( 'NONE', #6800, #32914, #70276, .T. ) ;
#6661=CARTESIAN_POINT ( 'NONE',  ( 13.69365034059999964, 1418.910360381229793, 238.2645940840980074 ) ) ;
#6662=CARTESIAN_POINT ( 'NONE',  ( -2.522360636850000226, 1478.162778754029887, 182.0787142752979832 ) ) ;
#6663=CARTESIAN_POINT ( 'NONE',  ( -17.64684345579999913, 1410.891992815630147, 194.5765879308980004 ) ) ;
#6665=CARTESIAN_POINT ( 'NONE',  ( -4.804950797150000064, 1416.130848188830214, 240.4142140068979927 ) ) ;
#6668=CARTESIAN_POINT ( 'NONE',  ( -5.464307007782710279, 1452.722242581880209, 151.9884548250850003 ) ) ;
#6669=CARTESIAN_POINT ( 'NONE',  ( -18.64672481350000055, 1416.851343894929869, 208.5597484335680178 ) ) ;
#6673=CARTESIAN_POINT ( 'NONE',  ( 14.65055688039350024, 1420.306699661070070, 228.1705606154760062 ) ) ;
#6678=CARTESIAN_POINT ( 'NONE',  ( -24.14171740887259787, 1410.987097078699890, 209.1436450758499745 ) ) ;
#6683=B_SPLINE_CURVE_WITH_KNOTS ( 'NONE', 4,
 ( #106769, #89973, #104155, #4864, #18468, #52664, #30060, #98374, #86801 ),
 .UNSPECIFIED., .F., .F.,
 ( 5, 4, 5 ),
 ( 0.000000000000000000, 2.461317144287991862E-05, 1.000000000000000000 ),
 .UNSPECIFIED. ) ;
#6684=CARTESIAN_POINT ( 'NONE',  ( -0.4783097240599999966, 1498.354913959829901, 236.9202977269980011 ) ) ;
#6685=CARTESIAN_POINT ( 'NONE',  ( -19.36978574289999955, 1410.873293175530080, 222.2371973171979960 ) ) ;
#6686=CARTESIAN_POINT ( 'NONE',  ( 45.13182480330119972, 1448.544769101459906, 267.0067098273050306 ) ) ;
#6688=CARTESIAN_POINT ( 'NONE',  ( -0.06123813080619999044, 1419.142829484630056, 184.6462053571979993 ) ) ;
#6692=CARTESIAN_POINT ( 'NONE',  ( 18.49876145869168553, 1458.769598805399028, 227.6223408758116307 ) ) ;
#6695=ORIENTED_EDGE ( 'NONE', *, *, #7012, .T. ) ;
#6696=CARTESIAN_POINT ( 'NONE',  ( 3.440243711449999964, 1448.632170455610094, 184.1390994748980177 ) ) ;
#6703=CARTESIAN_POINT ( 'NONE',  ( 1.821213500400669982, 1408.976658564170066, 186.8790236249210182 ) ) ;
#6704=CARTESIAN_POINT ( 'NONE',  ( -16.67282884602620285, 1411.231623680630037, 191.7273266183159990 ) ) ;
#6705=CARTESIAN_POINT ( 'NONE',  ( -18.51078443728962597, 1424.286743862528056, 225.0123096373268936 ) ) ;
#6708=CARTESIAN_POINT ( 'NONE',  ( 2.424063131930000115, 1427.257651041929876, 147.9020499575979954 ) ) ;
#6709=ORIENTED_EDGE ( 'NONE', *, *, #32585, .T. ) ;
#6710=CARTESIAN_POINT ( 'NONE',  ( 12.77825866169999891, 1416.543503932829935, 222.2791103846979865 ) ) ;
#6711=DIRECTION ( 'NONE',  ( -1.000000000000000000, 0.000000000000000000, -0.000000000000000000 ) ) ;
#6712=AXIS2_PLACEMENT_3D ( 'NONE', #63183, #10533, #71028 ) ;
#6718=CARTESIAN_POINT ( 'NONE',  ( -39.48812356950000435, 1450.238330950499858, 268.3665355202980436 ) ) ;
#6720=CARTESIAN_POINT ( 'NONE',  ( 11.13410507230000057, 1433.980233170309930, 151.6623994222979945 ) ) ;
#6721=CARTESIAN_POINT ( 'NONE',  ( 3.330669073880000049E-15, 1465.000168611230038, 255.3819207742980097 ) ) ;
#6722=FACE_OUTER_BOUND ( 'NONE', #86787, .T. ) ;
#6726=CARTESIAN_POINT ( 'NONE',  ( -15.65156082859999920, 1486.025561616130062, 186.7146735895979930 ) ) ;
#6728=CARTESIAN_POINT ( 'NONE',  ( -17.12887326659999943, 1409.676338055229962, 225.1570305523979982 ) ) ;
#6729=CARTESIAN_POINT ( 'NONE',  ( 5.205339508856989816, 1440.970228299569953, 155.0076768800470006 ) ) ;
#6731=CARTESIAN_POINT ( 'NONE',  ( -17.50306819544480064, 1410.886025037689933, 192.6233946069430090 ) ) ;
#6732=CARTESIAN_POINT ( 'NONE',  ( 3.393535723931189676E-07, 1408.913060375439727, 194.3872976811450144 ) ) ;
#6734=CARTESIAN_POINT ( 'NONE',  ( -7.951679572020000641, 1415.087745006229852, 224.2313155807979683 ) ) ;
#6735=CARTESIAN_POINT ( 'NONE',  ( 0.2051860993799010102, 1460.061070970760056, 182.9504558288110161 ) ) ;
#6737=ORIENTED_EDGE ( 'NONE', *, *, #107025, .F. ) ;
#6738=CARTESIAN_POINT ( 'NONE',  ( -17.22592482065197927, 1444.324653571828776, 162.9227486220069920 ) ) ;
#6739=CARTESIAN_POINT ( 'NONE',  ( -29.01179239785159680, 1509.906542726809903, 211.5837526005719837 ) ) ;
#6740=CARTESIAN_POINT ( 'NONE',  ( 13.19848402559999911, 1434.900413493669930, 149.4779621765979982 ) ) ;
#6741=CARTESIAN_POINT ( 'NONE',  ( -41.56943536072299850, 1444.920853409440042, 134.0999999984259716 ) ) ;
#6750=CARTESIAN_POINT ( 'NONE',  ( 31.99848188241270108, 1416.544741823263621, 269.3157487230474771 ) ) ;
#6753=CARTESIAN_POINT ( 'NONE',  ( 2.500000000000000000, 1434.142768478290236, 183.0182394750980279 ) ) ;
#6757=VERTEX_POINT ( 'NONE', #59062 ) ;
#6758=CARTESIAN_POINT ( 'NONE',  ( -28.53738215540000311, 1450.628365292199987, 136.4035485695980014 ) ) ;
#6759=CARTESIAN_POINT ( 'NONE',  ( -15.88324579074509835, 1409.493232073089985, 225.5703039524069879 ) ) ;
#6761=ORIENTED_EDGE ( 'NONE', *, *, #54326, .T. ) ;
#6764=CARTESIAN_POINT ( 'NONE',  ( -21.04604312829590995, 1411.007314980063711, 218.1938530540165857 ) ) ;
#6767=CARTESIAN_POINT ( 'NONE',  ( 18.50818375480000100, 1409.559380405929915, 219.7813082434980174 ) ) ;
#6769=CARTESIAN_POINT ( 'NONE',  ( -17.46811834570000244, 1424.002211962029833, 227.1199482243980015 ) ) ;
#6773=CARTESIAN_POINT ( 'NONE',  ( 22.98705083096197654, 1509.732498449673130, 190.4850602025729813 ) ) ;
#6779=CARTESIAN_POINT ( 'NONE',  ( -11.46119733878520108, 1485.818205503899890, 184.7882622351909845 ) ) ;
#6781=CARTESIAN_POINT ( 'NONE',  ( -4.222410926209430038, 1441.597235995280016, 167.7030612426750054 ) ) ;
#6782=AXIS2_PLACEMENT_3D ( 'NONE', #57334, #38834, #65166 ) ;
#6784=VERTEX_POINT ( 'NONE', #109457 ) ;
#6786=ORIENTED_EDGE ( 'NONE', *, *, #89707, .T. ) ;
#6790=CARTESIAN_POINT ( 'NONE',  ( -11.43729212106539883, 1425.481250161560183, 144.1595925846119997 ) ) ;
#6791=CARTESIAN_POINT ( 'NONE',  ( 16.18564167855010183, 1410.718174707190201, 191.5748361957220141 ) ) ;
#6793=CARTESIAN_POINT ( 'NONE',  ( 37.45063484360860429, 1436.678284271650227, 135.9172768678939747 ) ) ;
#6795=CARTESIAN_POINT ( 'NONE',  ( -11.15483420530000025, 1425.160608745730087, 144.1639996088979956 ) ) ;
#6796=CARTESIAN_POINT ( 'NONE',  ( -1.870694922257569948, 1509.048000892659957, 179.3712176469529993 ) ) ;
#6799=CARTESIAN_POINT ( 'NONE',  ( 39.48448845331249402, 1449.205409213759822, 134.0999999980729740 ) ) ;
#6800=VERTEX_POINT ( 'NONE', #33277 ) ;
#6802=CARTESIAN_POINT ( 'NONE',  ( 4.219439013950669448, 1441.595895969210005, 182.7715284958480026 ) ) ;
#6806=CARTESIAN_POINT ( 'NONE',  ( 11.60004869885203682, 1426.170871907920400, 138.0044153181233071 ) ) ;
#6807=CARTESIAN_POINT ( 'NONE',  ( 15.13342375178309851, 1507.606285622089899, 226.3974328904010065 ) ) ;
#6808=CARTESIAN_POINT ( 'NONE',  ( 0.2421685061019999974, 1451.163597886330081, 182.5480898430980119 ) ) ;
#6814=CARTESIAN_POINT ( 'NONE',  ( 36.37832874669670247, 1435.767865795960006, 134.4205480902799934 ) ) ;
#6815=CARTESIAN_POINT ( 'NONE',  ( 2.268814847818510394, 1421.223351404420100, 183.2269488433420008 ) ) ;
#6816=CARTESIAN_POINT ( 'NONE',  ( 26.72206613759999883, 1436.390045543859969, 136.7408624964980106 ) ) ;
#6824=CARTESIAN_POINT ( 'NONE',  ( -0.002327269815061227144, 1451.794865080891896, 154.0455392037681293 ) ) ;
#6826=CARTESIAN_POINT ( 'NONE',  ( -13.38213216230000135, 1415.140114695929924, 220.8789972148979928 ) ) ;
#6828=B_SPLINE_CURVE_WITH_KNOTS ( 'NONE', 3,
 ( #97454, #3419, #26949, #53271, #27488, #80099, #89044, #1769, #105867, #62797, #19634, #77902, #29147, #52712, #87410, #61676, #63334, #95799, #86847, #19067, #87975, #11263, #10140, #35906, #70090, #104203, #79027, #20181, #2328, #45425, #79568, #2869, #36989, #105305, #96913, #88512, #13417, #108606, #57126, #3971, #5602, #99083, #38095, #22361, #91252, #39753, #56562, #90690, #108043, #82304, #97989, #21811, #106946, #56010, #65524, #38638, #90134, #13978, #48166, #73915, #66080, #64968, #47606, #81731, #64423, #89594, #63873, #21256, #48722, #31340, #40294, #55467, #14533, #5039, #30232, #72272, #99631, #22919, #74479, #12886, #100206, #82847, #39184, #47064, #6137 ),
 .UNSPECIFIED., .F., .F.,
 ( 4, 2, 1, 1, 2, 2, 2, 1, 1, 2, 2, 2, 2, 1, 1, 2, 2, 2, 2, 1, 2, 2, 2, 2, 2, 2, 2, 2, 2, 2, 2, 1, 2, 2, 2, 1, 1, 2, 2, 2, 1, 1, 1, 2, 2, 2, 2, 2, 4 ),
 ( 0.000000000000000000, 0.03124999999979321402, 0.04687499999968981756, 0.05468749999963812281, 0.05859374999961227543, 0.06249999999958642805, 0.09374999999943356421, 0.1093749999993740563, 0.1171874999993623018, 0.1210937499993691435, 0.1249999999993759714, 0.1874999999992264521, 0.2187499999991654176, 0.2343749999991026067, 0.2421874999990496768, 0.2460937499990234201, 0.2499999999989971911, 0.3124999999987780330, 0.3437499999986242671, 0.3593749999985473287, 0.3671874999985022536, 0.3749999999984571231, 0.4374999999983198995, 0.4687499999981770138, 0.4999999999980341281, 0.5624999999977483567, 0.5937499999976966203, 0.6093749999976747489, 0.6249999999976528775, 0.6874999999980238030, 0.7187499999982092103, 0.7343749999982962517, 0.7421874999983337773, 0.7499999999983713028, 0.7812499999987206900, 0.7968749999989165334, 0.8046874999989963584, 0.8085937499990306643, 0.8124999999990649702, 0.8437499999992383870, 0.8593749999993495203, 0.8671874999993995914, 0.8710937499994046984, 0.8730468749993932631, 0.8749999999993817168, 0.9062499999995329292, 0.9218749999996082023, 0.9374999999996835864, 1.000000000000000000 ),
 .UNSPECIFIED. ) ;
#6830=CARTESIAN_POINT ( 'NONE',  ( 21.19109013666399832, 1409.653069700570086, 206.4065099927269955 ) ) ;
#6833=CARTESIAN_POINT ( 'NONE',  ( -11.87558183880000051, 1433.006727494650022, 147.8551147428979959 ) ) ;
#6834=CARTESIAN_POINT ( 'NONE',  ( 23.26829263668760106, 1427.370071165639956, 206.2054270095080142 ) ) ;
#6835=EDGE_CURVE ( 'NONE', #17250, #7904, #33834, .T. ) ;
#6836=CARTESIAN_POINT ( 'NONE',  ( 12.79059621819999926, 1461.442156363629920, 233.1425226920979696 ) ) ;
#6838=CARTESIAN_POINT ( 'NONE',  ( -4.694043468504164096, 1422.166103873277052, 184.6933998799214578 ) ) ;
#6839=CARTESIAN_POINT ( 'NONE',  ( 0.3402564618027850152, 1410.306538916012187, 185.0315799371184653 ) ) ;
#6845=CARTESIAN_POINT ( 'NONE',  ( 18.53418647859999879, 1507.620785850130005, 188.5293807644980006 ) ) ;
#6846=CARTESIAN_POINT ( 'NONE',  ( -10.98821264772629469, 1424.974956303378349, 138.3384972958762660 ) ) ;
#6849=CARTESIAN_POINT ( 'NONE',  ( 1.320018090259999832, 1507.624001450029937, 186.1627566462979928 ) ) ;
#6851=CARTESIAN_POINT ( 'NONE',  ( -10.95162904410000060, 1431.051873458699902, 151.6569759818979719 ) ) ;
#6858=CARTESIAN_POINT ( 'NONE',  ( -26.30997306620000131, 1508.005173063729899, 215.7207955781479995 ) ) ;
#6861=ORIENTED_EDGE ( 'NONE', *, *, #39266, .T. ) ;
#6864=CARTESIAN_POINT ( 'NONE',  ( 12.72968732700000061, 1407.074333243529964, 268.4159762977980108 ) ) ;
#6865=CARTESIAN_POINT ( 'NONE',  ( -0.08525575416679999352, 1408.910083189030047, 186.0349129820979783 ) ) ;
#6866=AXIS2_PLACEMENT_3D ( 'NONE', #12829, #100147, #83341 ) ;
#6870=CARTESIAN_POINT ( 'NONE',  ( 24.50944912269722664, 1438.648100259966668, 212.6421093072691235 ) ) ;
#6873=( BOUNDED_CURVE ( )  B_SPLINE_CURVE ( 3, ( #3375, #28553, #45918, #20139 ),
 .UNSPECIFIED., .F., .F. ) 
 B_SPLINE_CURVE_WITH_KNOTS ( ( 4, 4 ),
 ( 5.644024340868369904, 5.936278781197910526 ),
 .UNSPECIFIED. ) 
 CURVE ( )  GEOMETRIC_REPRESENTATION_ITEM ( )  RATIONAL_B_SPLINE_CURVE ( ( 1.000000000000000000, 0.9928949349872718821, 0.9928949349872718821, 1.000000000000000000 ) ) 
 REPRESENTATION_ITEM ( '' )  );
#6874=CARTESIAN_POINT ( 'NONE',  ( 27.78931436370000085, 1508.066562786630129, 211.8879754161380333 ) ) ;
#6875=ADVANCED_FACE ( 'NONE', ( #6551 ), #47597, .F. ) ;
#6878=CARTESIAN_POINT ( 'NONE',  ( -13.96458816240000012, 1446.023138053109960, 188.4738050279979973 ) ) ;
#6880=CARTESIAN_POINT ( 'NONE',  ( -19.88180708459617207, 1485.246950916194237, 190.7624080160636595 ) ) ;
#6884=CARTESIAN_POINT ( 'NONE',  ( 1.998401444330000344E-15, 1425.981674191730008, 219.6133832206979832 ) ) ;
#6886=CARTESIAN_POINT ( 'NONE',  ( -2.744509240469999778, 1475.260335887530118, 269.4960840521980572 ) ) ;
#6890=CARTESIAN_POINT ( 'NONE',  ( 17.83371091504290007, 1414.294633887780037, 223.5299421325470064 ) ) ;
#6893=B_SPLINE_CURVE_WITH_KNOTS ( 'NONE', 3,
 ( #74775, #5907, #57976, #14840, #90446, #49029, #50129, #15928, #30549, #92110 ),
 .UNSPECIFIED., .F., .F.,
 ( 4, 2, 2, 2, 4 ),
 ( 0.000000000000000000, 0.0007408354861221088392, 0.001481670972244217678, 0.002222506458366326626, 0.002963341944488435357 ),
 .UNSPECIFIED. ) ;
#6894=CARTESIAN_POINT ( 'NONE',  ( -17.01308424645448980, 1414.913060581098534, 207.5694819292969271 ) ) ;
#6895=CARTESIAN_POINT ( 'NONE',  ( -25.40163730124199759, 1470.069713657840111, 211.2641496062430235 ) ) ;
#6897=CARTESIAN_POINT ( 'NONE',  ( 2.918143513847768445E-16, 1426.814114634534008, 137.0999999980979851 ) ) ;
#6898=CARTESIAN_POINT ( 'NONE',  ( -22.18401561299999969, 1410.609167765330085, 202.6466877633079946 ) ) ;
#6901=CARTESIAN_POINT ( 'NONE',  ( -15.97833203511600253, 1420.726030562786036, 227.0316138336059737 ) ) ;
#6904=CARTESIAN_POINT ( 'NONE',  ( -4.107001541143308287, 1410.432827086315910, 232.1774397938114589 ) ) ;
#6908=CARTESIAN_POINT ( 'NONE',  ( 4.602958218326069779E-16, 1426.918876943007945, 134.0999999980979851 ) ) ;
#6909=CARTESIAN_POINT ( 'NONE',  ( 11.71693939160000042, 1426.292619179529993, 142.7697690241979842 ) ) ;
#6911=CARTESIAN_POINT ( 'NONE',  ( -15.73574044604409927, 1409.462552572229924, 225.2910003602459881 ) ) ;
#6914=CARTESIAN_POINT ( 'NONE',  ( 28.11203376910000173, 1444.250560465929993, 137.5208087134980133 ) ) ;
#6917=DIRECTION ( 'NONE',  ( 0.000000000000000000, 1.000000000000000000, 0.000000000000000000 ) ) ;
#6918=CARTESIAN_POINT ( 'NONE',  ( -7.615348975238497076, 1398.139300407672863, 198.4687090422606275 ) ) ;
#6922=CARTESIAN_POINT ( 'NONE',  ( 20.82055072771269977, 1509.307918567249999, 229.0039304369510091 ) ) ;
#6924=VERTEX_POINT ( 'NONE', #34506 ) ;
#6925=ORIENTED_EDGE ( 'NONE', *, *, #9707, .T. ) ;
#6926=CARTESIAN_POINT ( 'NONE',  ( 11.52705822141970060, 1434.294195329290005, 151.3489372875870060 ) ) ;
#6927=CARTESIAN_POINT ( 'NONE',  ( -12.55568685759999958, 1398.285279232130051, 212.9384880290180320 ) ) ;
#6928=CARTESIAN_POINT ( 'NONE',  ( -19.69385343140000444, 1409.600784903429940, 217.8674699180880054 ) ) ;
#6930=CARTESIAN_POINT ( 'NONE',  ( -13.12297772262875029, 1444.782698483078320, 169.4025063443241095 ) ) ;
#6931=CARTESIAN_POINT ( 'NONE',  ( 22.30235455686514712, 1509.698861494391622, 228.4320621754980607 ) ) ;
#6933=CARTESIAN_POINT ( 'NONE',  ( 1.581901184577762853, 1426.946688134061105, 137.0999999980979851 ) ) ;
#6934=CARTESIAN_POINT ( 'NONE',  ( 17.71884614950000270, 1424.302129513130012, 226.3668682875980096 ) ) ;
#6935=CARTESIAN_POINT ( 'NONE',  ( 0.5045109264089999712, 1429.776885342730111, 184.2481756784980291 ) ) ;
#6936=CARTESIAN_POINT ( 'NONE',  ( -9.507368510479999202, 1414.971339025629959, 194.7268509206979843 ) ) ;
#6939=B_SPLINE_SURFACE_WITH_KNOTS ( 'NONE', 5, 5, ( 
 ( #24378, #6490, #84831, #109509, #74813, #40641, #108959, #100542, #41200 ),
 ( #15421, #23277, #101624, #23822, #58013, #75902, #31683, #84297, #92692 ),
 ( #49613, #42297, #15967, #8131, #50700, #99985, #57473, #91598, #42860 ),
 ( #32246, #24913, #49066, #32785, #68082, #83201, #76449, #17053, #92149 ),
 ( #51250, #66969, #101079, #75370, #66426, #83745, #7041, #14874, #58562 ),
 ( #50170, #7588, #102193, #65865, #41743, #110604, #59122, #110054, #33328 ) ),
 .UNSPECIFIED., .F., .F., .F.,
 ( 6, 6 ),
 ( 6, 3, 6 ),
 ( 0.4666582264849999939, 2.797885342226240191 ),
 ( -1.082960624482799909E-05, 1.000000000000000000, 2.000000000000000000 ),
 .UNSPECIFIED. ) ;
#6940=CARTESIAN_POINT ( 'NONE',  ( 8.265387638122250635, 1396.201694164710034, 201.7848193804910011 ) ) ;
#6941=CARTESIAN_POINT ( 'NONE',  ( 2.500000000000000000, 1419.503957648720871, 138.2096356918212905 ) ) ;
#6942=CARTESIAN_POINT ( 'NONE',  ( 10.95984484989999963, 1431.648774854440035, 151.7380654299980165 ) ) ;
#6944=ORIENTED_EDGE ( 'NONE', *, *, #64219, .T. ) ;
#6945=CARTESIAN_POINT ( 'NONE',  ( 13.51212582107970128, 1435.883254532899855, 150.4097860975269896 ) ) ;
#6948=CARTESIAN_POINT ( 'NONE',  ( -19.64522922078770151, 1497.936653429400167, 228.8931875647859897 ) ) ;
#6949=CARTESIAN_POINT ( 'NONE',  ( -10.87454802859999781, 1463.204792800929908, 232.0658476886979713 ) ) ;
#6954=B_SPLINE_SURFACE_WITH_KNOTS ( 'NONE', 3, 5, ( 
 ( #76204, #110349, #33625, #11221, #71712, #28558 ),
 ( #80617, #37508, #21774, #47030, #20142, #3380 ),
 ( #45384, #105830, #62756, #55428, #3933, #29108 ),
 ( #81155, #54337, #63294, #38060, #4470, #11753 ) ),
 .UNSPECIFIED., .F., .F., .F.,
 ( 4, 4 ),
 ( 6, 6 ),
 ( 5.479561955150000330, 5.505632801049999969 ),
 ( 0.000000000000000000, 1.000000000000000000 ),
 .UNSPECIFIED. ) ;
#6955=AXIS2_PLACEMENT_3D ( 'NONE', #33066, #85671, #76183 ) ;
#6956=ORIENTED_EDGE ( 'NONE', *, *, #106940, .F. ) ;
#6961=ORIENTED_EDGE ( 'NONE', *, *, #85737, .F. ) ;
#6966=CARTESIAN_POINT ( 'NONE',  ( -12.21036482539999923, 1409.841853000129959, 189.5541482494979846 ) ) ;
#6967=CARTESIAN_POINT ( 'NONE',  ( -2.261018246749999960, 1409.497062291729890, 232.5268568490979817 ) ) ;
#6968=CARTESIAN_POINT ( 'NONE',  ( -0.6362176846849959544, 1414.913060387399810, 225.3300418929160003 ) ) ;
#6969=VERTEX_POINT ( 'NONE', #92205 ) ;
#6970=CARTESIAN_POINT ( 'NONE',  ( 19.06118660449999780, 1425.780408082830036, 222.6829976502980060 ) ) ;
#6973=CARTESIAN_POINT ( 'NONE',  ( -0.1209835420493560049, 1465.026716009449956, 237.7730318938839957 ) ) ;
#6974=EDGE_CURVE ( 'NONE', #6784, #50075, #13600, .T. ) ;
#6976=EDGE_CURVE ( 'NONE', #11504, #106239, #107717, .T. ) ;
#6977=CARTESIAN_POINT ( 'NONE',  ( 7.520399230329999796, 1408.700311873330065, 270.3839821972980531 ) ) ;
#6979=CARTESIAN_POINT ( 'NONE',  ( 23.98652862120000151, 1410.713095165929872, 208.5703825711269985 ) ) ;
#6980=CARTESIAN_POINT ( 'NONE',  ( -2.500574544111449971, 1448.942056179399970, 154.5733147259969940 ) ) ;
#6985=CARTESIAN_POINT ( 'NONE',  ( 0.2691385670090000182, 1419.231489590830051, 184.6448893939979996 ) ) ;
#6986=CARTESIAN_POINT ( 'NONE',  ( 2.456308003337250412, 1421.792674159936951, 137.0999999980978714 ) ) ;
#6990=EDGE_CURVE ( 'NONE', #87156, #95283, #30152, .T. ) ;
#6991=CARTESIAN_POINT ( 'NONE',  ( 7.132065395029999699, 1475.995241008230096, 267.2559760689979953 ) ) ;
#6996=CARTESIAN_POINT ( 'NONE',  ( 0.8010214712846820406, 1452.931212010089894, 183.3398705925079923 ) ) ;
#7003=CARTESIAN_POINT ( 'NONE',  ( 11.93818824289999903, 1433.480083226980014, 149.8972169559980046 ) ) ;
#7004=CARTESIAN_POINT ( 'NONE',  ( 15.81201445386249915, 1506.433683730510211, 224.3933755863170063 ) ) ;
#7007=CARTESIAN_POINT ( 'NONE',  ( 22.75126231049999959, 1450.312999748930224, 218.7949445992479980 ) ) ;
#7009=LINE ( 'NONE', #41167, #18058 ) ;
#7010=CARTESIAN_POINT ( 'NONE',  ( 26.81178797887219645, 1450.703257649033958, 136.4517338180884849 ) ) ;
#7011=CARTESIAN_POINT ( 'NONE',  ( 3.918670472299999208, 1441.329835342249908, 183.9132893515979958 ) ) ;
#7012=EDGE_CURVE ( 'NONE', #23487, #86024, #109392, .T. ) ;
#7013=CARTESIAN_POINT ( 'NONE',  ( 29.16088018400000337, 1435.515811254470009, 135.2139231482979937 ) ) ;
#7015=CARTESIAN_POINT ( 'NONE',  ( 38.22332642270760061, 1448.618965483920192, 136.4075853064549904 ) ) ;
#7016=CARTESIAN_POINT ( 'NONE',  ( -23.53722878629999826, 1435.319033575220146, 213.4336055579080380 ) ) ;
#7017=CARTESIAN_POINT ( 'NONE',  ( -12.78776258895079998, 1416.851343896850040, 195.5391574246120001 ) ) ;
#7019=CARTESIAN_POINT ( 'NONE',  ( 10.17004918770000010, 1507.385806824230031, 183.8335291379979992 ) ) ;
#7021=CARTESIAN_POINT ( 'NONE',  ( -2.751978043620916026, 1471.436294014188888, 269.3346704505487992 ) ) ;
#7024=CARTESIAN_POINT ( 'NONE',  ( -42.08860907271759544, 1427.691514611570938, 269.0733891839905141 ) ) ;
#7025=ADVANCED_FACE ( 'NONE', ( #95518 ), #26815, .T. ) ;
#7029=CARTESIAN_POINT ( 'NONE',  ( -15.02666660005860244, 1451.829519320988311, 222.9333663745973411 ) ) ;
#7030=CARTESIAN_POINT ( 'NONE',  ( -13.10582615840648479, 1444.796545787240802, 186.4375160407790588 ) ) ;
#7033=VECTOR ( 'NONE', #94551, 1000.000000000000000 ) ;
#7035=CARTESIAN_POINT ( 'NONE',  ( -4.037103925677953953, 1415.961567342583521, 232.4510850075154451 ) ) ;
#7036=CARTESIAN_POINT ( 'NONE',  ( -16.26938466631711933, 1451.108877157205370, 148.8960758721039781 ) ) ;
#7037=CARTESIAN_POINT ( 'NONE',  ( 25.69726023690000005, 1436.490352274229963, 137.0663831747980055 ) ) ;
#7038=CARTESIAN_POINT ( 'NONE',  ( -12.80739992162959240, 1442.848094250957729, 169.4485940490470739 ) ) ;
#7039=CARTESIAN_POINT ( 'NONE',  ( 18.01711958838799887, 1424.180322377740140, 225.4683465207770041 ) ) ;
#7041=CARTESIAN_POINT ( 'NONE',  ( -0.2033579075130829972, 1416.218865267220053, 191.1379978179999739 ) ) ;
#7042=CARTESIAN_POINT ( 'NONE',  ( -11.90005270625540135, 1409.328619384790045, 226.7881248095609976 ) ) ;
#7043=EDGE_LOOP ( 'NONE', ( #96909, #88078, #105508, #32308 ) ) ;
#7045=CARTESIAN_POINT ( 'NONE',  ( 17.19251027932519804, 1415.089118586289942, 209.7053761061400223 ) ) ;
#7049=CARTESIAN_POINT ( 'NONE',  ( -20.54560411990000190, 1453.269583021529797, 220.8539909785980058 ) ) ;
#7051=ADVANCED_FACE ( 'NONE', ( #12619 ), #8245, .T. ) ;
#7052=CARTESIAN_POINT ( 'NONE',  ( -11.86372866770000023, 1433.130351995409910, 150.2717319648980094 ) ) ;
#7054=CIRCLE ( 'NONE', #23108, 39.03564169359999170 ) ;
#7057=CARTESIAN_POINT ( 'NONE',  ( -12.77587743780000018, 1416.568813547830132, 195.5427461491979955 ) ) ;
#7058=EDGE_CURVE ( 'NONE', #109848, #72154, #27937, .T. ) ;
#7060=CARTESIAN_POINT ( 'NONE',  ( 3.057433871810000259, 1450.174788091120035, 183.8252404729979901 ) ) ;
#7062=CARTESIAN_POINT ( 'NONE',  ( -21.39654334329791396, 1509.777343320284899, 230.1584121880257783 ) ) ;
#7063=CARTESIAN_POINT ( 'NONE',  ( -2.296399283793280044E-09, 1415.822370859000102, 241.4911618200540033 ) ) ;
#7065=VERTEX_POINT ( 'NONE', #72011 ) ;
#7066=CARTESIAN_POINT ( 'NONE',  ( -11.82359547739990013, 1429.509793761799983, 149.2101411770329946 ) ) ;
#7068=CARTESIAN_POINT ( 'NONE',  ( -5.402393449050000740, 1473.936434490630063, 270.1311850751980046 ) ) ;
#7071=CARTESIAN_POINT ( 'NONE',  ( 38.63621758546330653, 1450.019455539890032, 134.8311675663850053 ) ) ;
#7073=CARTESIAN_POINT ( 'NONE',  ( -13.71477132504269925, 1421.034959706790005, 222.0387691072829739 ) ) ;
#7078=CARTESIAN_POINT ( 'NONE',  ( -8.361732071192520266, 1406.610899605839904, 269.0188235946120585 ) ) ;
#7082=VERTEX_POINT ( 'NONE', #73647 ) ;
#7085=CARTESIAN_POINT ( 'NONE',  ( 4.974056298193653802, 1423.234490133592544, 184.3173436926480520 ) ) ;
#7088=CARTESIAN_POINT ( 'NONE',  ( -2.571340789771010549, 1440.211241685782170, 170.5281974536487439 ) ) ;
#7089=CARTESIAN_POINT ( 'NONE',  ( -18.39440931229999876, 1485.488557115530057, 189.1449212182980091 ) ) ;
#7090=CARTESIAN_POINT ( 'NONE',  ( -17.34910718890199988, 1498.334872555480160, 229.4722646656200027 ) ) ;
#7091=B_SPLINE_SURFACE_WITH_KNOTS ( 'NONE', 4, 5, ( 
 ( #80441, #97227, #64203, #72594, #19401, #37334 ),
 ( #4291, #53604, #105085, #45755, #55809, #89385 ),
 ( #71530, #46856, #89926, #28374, #87748, #105650 ),
 ( #106722, #96693, #3206, #11578, #45197, #28935 ),
 ( #30013, #13201, #21604, #78783, #36225, #63125 ) ),
 .UNSPECIFIED., .F., .F., .F.,
 ( 5, 5 ),
 ( 6, 6 ),
 ( 0.8555274230859999385, 1.128731558089999920 ),
 ( 0.000000000000000000, 2.000000000000000000 ),
 .UNSPECIFIED. ) ;
#7096=B_SPLINE_SURFACE_WITH_KNOTS ( 'NONE', 4, 5, ( 
 ( #2735, #3286, #105735, #96778, #72681, #20049 ),
 ( #4372, #72149, #11659, #71615, #45834, #79968 ),
 ( #29019, #63205, #97312, #106268, #29554, #63739 ),
 ( #106805, #30095, #64290, #109036, #23351, #48022 ),
 ( #91115, #40162, #22228, #108471, #31207, #24443 ) ),
 .UNSPECIFIED., .F., .F., .F.,
 ( 5, 5 ),
 ( 6, 6 ),
 ( 29.43575841650000058, 48.27399281030000111 ),
 ( -1.387778780779999841E-17, 1.000000000000000000 ),
 .UNSPECIFIED. ) ;
#7099=CARTESIAN_POINT ( 'NONE',  ( -41.51852662024420226, 1431.123461163979982, 270.1901905831499562 ) ) ;
#7101=CARTESIAN_POINT ( 'NONE',  ( -24.18363701780000241, 1464.258769156330118, 212.1671259816380086 ) ) ;
#7103=DIRECTION ( 'NONE',  ( 0.000000000000000000, 1.000000000000000000, 0.000000000000000000 ) ) ;
#7107=CARTESIAN_POINT ( 'NONE',  ( 3.771101265954107884, 1425.575893895815852, 185.2173869927980832 ) ) ;
#7109=ADVANCED_FACE ( 'NONE', ( #54651 ), #9835, .T. ) ;
#7110=CARTESIAN_POINT ( 'NONE',  ( -24.40603932400000176, 1441.493461285830108, 212.0691197944780129 ) ) ;
#7114=CARTESIAN_POINT ( 'NONE',  ( -0.07726447814961530380, 1452.995338318107770, 183.2382765434469434 ) ) ;
#7116=CARTESIAN_POINT ( 'NONE',  ( 18.80463396749128435, 1425.801069675071858, 225.6039139557115902 ) ) ;
#7118=ORIENTED_EDGE ( 'NONE', *, *, #44010, .T. ) ;
#7121=CARTESIAN_POINT ( 'NONE',  ( -19.87427776918198674, 1456.662545660512478, 225.4134381264325668 ) ) ;
#7122=ORIENTED_EDGE ( 'NONE', *, *, #33674, .F. ) ;
#7124=EDGE_CURVE ( 'NONE', #52007, #105623, #98821, .T. ) ;
#7125=CARTESIAN_POINT ( 'NONE',  ( 12.92481085168819988, 1434.740917461700064, 149.3164734981210131 ) ) ;
#7126=CARTESIAN_POINT ( 'NONE',  ( 6.152613576320070443, 1468.998513094850068, 233.7412649376300067 ) ) ;
#7128=CARTESIAN_POINT ( 'NONE',  ( 12.78690713350000152, 1416.828040475229955, 222.7042044314979989 ) ) ;
#7131=CARTESIAN_POINT ( 'NONE',  ( 4.026786250540000722, 1422.913060387330006, 179.4243885131980107 ) ) ;
#7135=CARTESIAN_POINT ( 'NONE',  ( -11.86590139589999815, 1432.348266868109931, 151.0567667964980103 ) ) ;
#7138=VERTEX_POINT ( 'NONE', #15353 ) ;
#7140=CARTESIAN_POINT ( 'NONE',  ( 15.87406479873239995, 1409.467378496833362, 192.9778776010643071 ) ) ;
#7141=CARTESIAN_POINT ( 'NONE',  ( 0.8259447189419999447, 1418.827400219930041, 184.7842358559980198 ) ) ;
#7149=ADVANCED_FACE ( 'NONE', ( #16987 ), #35774, .F. ) ;
#7151=CARTESIAN_POINT ( 'NONE',  ( 37.28204567502979927, 1440.913060386509869, 255.1050374929049838 ) ) ;
#7154=CARTESIAN_POINT ( 'NONE',  ( 13.31375889959999803, 1429.098084184829986, 222.1181957922979961 ) ) ;
#7157=ORIENTED_EDGE ( 'NONE', *, *, #63723, .T. ) ;
#7159=CARTESIAN_POINT ( 'NONE',  ( -19.64841113585741539, 1485.306958117290833, 190.2729878873239215 ) ) ;
#7162=CARTESIAN_POINT ( 'NONE',  ( 2.483039259372770591, 1508.999772102527686, 238.0619777347729666 ) ) ;
#7163=CARTESIAN_POINT ( 'NONE',  ( -3.321447364419999548, 1484.261043626330093, 183.3707343507980170 ) ) ;
#7164=ADVANCED_FACE ( 'NONE', ( #19210 ), #103709, .F. ) ;
#7168=CARTESIAN_POINT ( 'NONE',  ( -13.90870118630000007, 1453.159462792929844, 194.1873857778979868 ) ) ;
#7169=DIRECTION ( 'NONE',  ( 0.000000000000000000, -1.000000000000000000, -0.000000000000000000 ) ) ;
#7172=EDGE_LOOP ( 'NONE', ( #88279, #42626, #45662, #531 ) ) ;
#7176=B_SPLINE_SURFACE_WITH_KNOTS ( 'NONE', 5, 5, ( 
 ( #47746, #82994, #72955, #40984, #29834, #38779 ),
 ( #32036, #13014, #47200, #5184, #81326, #4641 ),
 ( #30381, #98690, #30932, #21950, #90279, #39339 ),
 ( #51055, #66773, #85186, #43208, #102525, #8472 ),
 ( #60015, #34238, #49950, #84632, #58904, #7930 ),
 ( #101416, #42099, #42646, #76800, #68423, #17968 ) ),
 .UNSPECIFIED., .F., .F., .F.,
 ( 6, 6 ),
 ( 6, 6 ),
 ( 17.24302740239999920, 89.20802345619999585 ),
 ( -2.775557561569999727E-17, 2.000000000410000034 ),
 .UNSPECIFIED. ) ;
#7179=EDGE_LOOP ( 'NONE', ( #73607, #78031, #95120, #54723, #17130, #89487 ) ) ;
#7180=EDGE_LOOP ( 'NONE', ( #84068, #48104, #2557, #66954 ) ) ;
#7183=DIRECTION ( 'NONE',  ( -0.004026485253183625761, 0.9999913661844073154, 0.001027118858031680253 ) ) ;
#7186=ADVANCED_FACE ( 'NONE', ( #86990 ), #86722, .T. ) ;
#7193=CARTESIAN_POINT ( 'NONE',  ( 0.7988375143999999484, 1409.446852857530075, 185.3482159754979932 ) ) ;
#7197=CARTESIAN_POINT ( 'NONE',  ( -4.243814737821510086, 1441.427819818469970, 162.1743596817549928 ) ) ;
#7198=AXIS2_PLACEMENT_3D ( 'NONE', #30074, #22755, #73199 ) ;
#7199=CARTESIAN_POINT ( 'NONE',  ( -2.104349271192939685, 1450.141963089990213, 182.8680826352290012 ) ) ;
#7200=VERTEX_POINT ( 'NONE', #107654 ) ;
#7202=EDGE_CURVE ( 'NONE', #16155, #12333, #78372, .T. ) ;
#7205=CARTESIAN_POINT ( 'NONE',  ( 14.79572149000000003, 1410.747178327829943, 191.5201547110980016 ) ) ;
#7206=CARTESIAN_POINT ( 'NONE',  ( -6.443502200292150068E-09, 1472.319935551380013, 259.7298202287869913 ) ) ;
#7207=CARTESIAN_POINT ( 'NONE',  ( 20.44283505528667888, 1436.443178919755610, 144.9572787325427328 ) ) ;
#7210=CARTESIAN_POINT ( 'NONE',  ( 0.1246760915043968326, 1486.459310424578462, 181.8129998335755317 ) ) ;
#7212=CARTESIAN_POINT ( 'NONE',  ( -46.27659351362679985, 1440.462201645729920, 267.5895223780760261 ) ) ;
#7213=CARTESIAN_POINT ( 'NONE',  ( 13.52332530298609825, 1508.669884114960041, 233.4688069057430084 ) ) ;
#7218=B_SPLINE_SURFACE_WITH_KNOTS ( 'NONE', 5, 5, ( 
 ( #80788, #21394, #55605, #53968, #88101, #71328 ),
 ( #89728, #105441, #11388, #28730, #48853, #72940 ),
 ( #40968, #82437, #107632, #13003, #100330, #56130 ),
 ( #99207, #90265, #5167, #56686, #90823, #14104 ),
 ( #107079, #22486, #15197, #91924, #74594, #40417 ),
 ( #30367, #48294, #64557, #57801, #81866, #109296 ) ),
 .UNSPECIFIED., .F., .F., .F.,
 ( 6, 6 ),
 ( 6, 6 ),
 ( 13.29217618510000065, 14.75807319179999944 ),
 ( 0.000000000000000000, 2.000000000000000000 ),
 .UNSPECIFIED. ) ;
#7221=CARTESIAN_POINT ( 'NONE',  ( -26.57297411396899989, 1451.985062530020059, 135.0132826329440263 ) ) ;
#7223=CARTESIAN_POINT ( 'NONE',  ( 25.18659394999999890, 1435.864776774990105, 221.5022687698979951 ) ) ;
#7224=CARTESIAN_POINT ( 'NONE',  ( 1.461742694410000043, 1494.215630625830045, 181.6758722823980179 ) ) ;
#7226=CARTESIAN_POINT ( 'NONE',  ( -24.17505645849999851, 1437.686240857209896, 211.9528072102179976 ) ) ;
#7228=CARTESIAN_POINT ( 'NONE',  ( -18.87589743271229992, 1452.253899524100007, 144.5155550433779865 ) ) ;
#7232=CARTESIAN_POINT ( 'NONE',  ( 13.12206485389999955, 1420.327681803430096, 229.1659002618980026 ) ) ;
#7237=CARTESIAN_POINT ( 'NONE',  ( -23.92522223069349963, 1410.731318646559885, 209.8608519489140178 ) ) ;
#7238=ORIENTED_EDGE ( 'NONE', *, *, #57100, .T. ) ;
#7240=CARTESIAN_POINT ( 'NONE',  ( -45.35511022099471035, 1436.791113516306268, 266.1975110343311712 ) ) ;
#7241=CARTESIAN_POINT ( 'NONE',  ( -25.00976051679999657, 1436.598010167069788, 137.9330532114979917 ) ) ;
#7243=ORIENTED_EDGE ( 'NONE', *, *, #41858, .F. ) ;
#7244=CARTESIAN_POINT ( 'NONE',  ( 45.61112093737630602, 1446.140457532640085, 266.6912352721849970 ) ) ;
#7246=CARTESIAN_POINT ( 'NONE',  ( -16.91308933013565508, 1421.902804263020471, 226.8507505944365619 ) ) ;
#7249=CARTESIAN_POINT ( 'NONE',  ( 18.56582872426456632, 1458.623439932988958, 227.5449210459607059 ) ) ;
#7251=AXIS2_PLACEMENT_3D ( 'NONE', #29628, #63812, #65468 ) ;
#7255=CARTESIAN_POINT ( 'NONE',  ( 26.92459677059870060, 1451.501184678159916, 136.0683855680960050 ) ) ;
#7261=CARTESIAN_POINT ( 'NONE',  ( 3.377914574041609885, 1409.031019763529912, 187.3393513309910077 ) ) ;
#7262=CARTESIAN_POINT ( 'NONE',  ( 1.803096684420000040, 1417.508280449130098, 234.1739293872979886 ) ) ;
#7263=DIRECTION ( 'NONE',  ( 0.9995237679829612754, -0.03085834145158970754, -2.563637404923585686E-08 ) ) ;
#7264=CARTESIAN_POINT ( 'NONE',  ( 4.051730709047915546, 1441.572134815625986, 170.5366858379989310 ) ) ;
#7266=CARTESIAN_POINT ( 'NONE',  ( 9.609284535499998725, 1429.602790706330097, 148.1400166355980161 ) ) ;
#7267=EDGE_LOOP ( 'NONE', ( #39811, #86125, #42482, #44787 ) ) ;
#7268=CARTESIAN_POINT ( 'NONE',  ( 11.22551998620189906, 1414.913060387399810, 220.6642913648300066 ) ) ;
#7269=AXIS2_PLACEMENT_3D ( 'NONE', #110647, #7632, #51293 ) ;
#7271=CARTESIAN_POINT ( 'NONE',  ( 17.40764059099999628, 1414.996444526030018, 210.6782161193179945 ) ) ;
#7276=CARTESIAN_POINT ( 'NONE',  ( -23.03655027839999647, 1458.194572356429944, 255.3819207742980097 ) ) ;
#7286=CARTESIAN_POINT ( 'NONE',  ( -18.98347673960000037, 1486.208000860629909, 189.2831150523980170 ) ) ;
#7289=CARTESIAN_POINT ( 'NONE',  ( -17.58360215189999920, 1410.891091606730015, 225.4625532605979856 ) ) ;
#7294=CARTESIAN_POINT ( 'NONE',  ( 12.72996564059999969, 1416.826388557929931, 223.1307082869980150 ) ) ;
#7297=DIRECTION ( 'NONE',  ( 0.1976594630508882178, -0.9325252259461312976, 0.3022043011615674901 ) ) ;
#7299=CARTESIAN_POINT ( 'NONE',  ( 0.2060721707870890040, 1459.560850903249730, 182.9719205269209965 ) ) ;
#7302=CARTESIAN_POINT ( 'NONE',  ( -27.23063139319997816, 1443.913060387329097, 161.8596747266978753 ) ) ;
#7303=CARTESIAN_POINT ( 'NONE',  ( -37.73093663436678469, 1445.052233488290085, 136.8111089660027062 ) ) ;
#7305=CARTESIAN_POINT ( 'NONE',  ( -41.54171725205129917, 1442.308966536679918, 134.0999999980950008 ) ) ;
#7307=ORIENTED_EDGE ( 'NONE', *, *, #14442, .F. ) ;
#7314=CYLINDRICAL_SURFACE ( 'NONE', #107244, 1.463110112869996149 ) ;
#7315=CARTESIAN_POINT ( 'NONE',  ( 22.78790659570000088, 1507.631725798030175, 209.8615682015409902 ) ) ;
#7317=CARTESIAN_POINT ( 'NONE',  ( 2.500000000000000000, 1436.879499792069964, 182.8948590173980051 ) ) ;
#7319=ADVANCED_FACE ( 'NONE', ( #32043 ), #1830, .F. ) ;
#7323=CARTESIAN_POINT ( 'NONE',  ( -32.07934838669999777, 1451.337335293929982, 136.0002333985979988 ) ) ;
#7324=CARTESIAN_POINT ( 'NONE',  ( -15.80146386689030003, 1410.855256520919966, 226.7268951530490142 ) ) ;
#7325=DIRECTION ( 'NONE',  ( 3.085874980950000024E-15, -2.120525977030000242E-14, -1.000000000000000000 ) ) ;
#7328=ADVANCED_FACE ( 'NONE', ( #108196 ), #78705, .F. ) ;
#7329=CARTESIAN_POINT ( 'NONE',  ( -19.19237350200172187, 1410.944925138707504, 222.5985789656905638 ) ) ;
#7331=CARTESIAN_POINT ( 'NONE',  ( -0.3290055904713540258, 1418.886737140139985, 184.6767946731409893 ) ) ;
#7332=CARTESIAN_POINT ( 'NONE',  ( 41.48540613818578038, 1445.929842224576305, 269.6377302435102479 ) ) ;
#7333=CARTESIAN_POINT ( 'NONE',  ( 16.90258613670328813, 1433.073112335133601, 217.3043047566771122 ) ) ;
#7334=CARTESIAN_POINT ( 'NONE',  ( 1.956921220169999698, 1417.602764174529966, 233.5179091431980112 ) ) ;
#7337=CARTESIAN_POINT ( 'NONE',  ( 4.063550476549999679, 1497.713060387329961, 230.5763704537980061 ) ) ;
#7340=CARTESIAN_POINT ( 'NONE',  ( 2.500000000000000000, 1448.989771342329959, 154.5778231068980233 ) ) ;
#7342=VECTOR ( 'NONE', #75145, 1000.000000000000000 ) ;
#7344=CARTESIAN_POINT ( 'NONE',  ( -4.232926184839439721, 1441.503792767389996, 164.1558557344339988 ) ) ;
#7348=ORIENTED_EDGE ( 'NONE', *, *, #59133, .T. ) ;
#7351=CARTESIAN_POINT ( 'NONE',  ( -11.43885624517646526, 1425.480338822508202, 144.2656653268024343 ) ) ;
#7352=CARTESIAN_POINT ( 'NONE',  ( 15.97954657421199798, 1409.471061115830025, 193.0248343784320184 ) ) ;
#7355=CARTESIAN_POINT ( 'NONE',  ( 39.86835271869999531, 1441.199396608850066, 136.8459542608980257 ) ) ;
#7356=B_SPLINE_CURVE_WITH_KNOTS ( 'NONE', 3,
 ( #63107, #97204, #98307, #46293, #55791, #37866, #21583, #89906, #88266, #54688, #97758, #96105, #106167, #44621, #78762, #29444, #2077, #19380, #21029, #89364, #53584, #12657, #80965, #105066, #27804, #36207, #61989, #40062, #47916, #75340, #32758, #4796, #56322, #107263, #38941, #31106, #101049, #74242, #73121, #82624, #99398, #65285, #22676, #57983, #83714, #30558, #15393, #57445, #108372, #64746, #109481, #13731, #39516, #14846 ),
 .UNSPECIFIED., .F., .F.,
 ( 4, 2, 2, 1, 1, 2, 2, 2, 2, 1, 1, 1, 1, 2, 2, 2, 2, 2, 2, 2, 2, 2, 1, 1, 2, 2, 1, 1, 1, 1, 2, 2, 4 ),
 ( 0.000000000000000000, 0.06249999999991798227, 0.09374999999990608901, 0.1093749999998750166, 0.1171874999998856054, 0.1210937499998925304, 0.1249999999998994693, 0.1875000000009550416, 0.2187500000015098200, 0.2343750000017873758, 0.2421875000019497182, 0.2460937500020323188, 0.2480468750020981550, 0.2490234375021571356, 0.2500000000022161162, 0.3750000000027837177, 0.4375000000030658254, 0.4687500000032305825, 0.5000000000033952841, 0.5625000000037223558, 0.5937500000039129811, 0.6093750000040102366, 0.6171875000040586423, 0.6210937500040828452, 0.6230468750040973891, 0.6250000000041118220, 0.6875000000031932235, 0.7187500000027338132, 0.7343750000024805713, 0.7421875000023285818, 0.7460937500022526425, 0.7500000000021767033, 1.000000000000000000 ),
 .UNSPECIFIED. ) ;
#7358=CARTESIAN_POINT ( 'NONE',  ( 14.87107281846884455, 1462.053534961335572, 230.0773967180462876 ) ) ;
#7361=CARTESIAN_POINT ( 'NONE',  ( -37.82787436099530254, 1438.484237118849933, 136.5974028198669998 ) ) ;
#7365=B_SPLINE_CURVE_WITH_KNOTS ( 'NONE', 5,
 ( #70727, #55010, #52795, #2413, #105956, #20265, #62892, #19722, #20812, #86927, #36530, #10218 ),
 .UNSPECIFIED., .F., .F.,
 ( 6, 3, 3, 6 ),
 ( 0.000000000000000000, 0.3925153839664296540, 0.7975051279878269117, 1.000000000000000000 ),
 .UNSPECIFIED. ) ;
#7366=ORIENTED_EDGE ( 'NONE', *, *, #47219, .F. ) ;
#7368=DIRECTION ( 'NONE',  ( -0.7067700363774163108, -0.03085824620771824081, 0.7067700363767903671 ) ) ;
#7369=DIRECTION ( 'NONE',  ( 0.6906235816661250304, -0.2466512791670444904, -0.6798545542481230219 ) ) ;
#7371=DIRECTION ( 'NONE',  ( 0.000000000000000000, 0.000000000000000000, -1.000000000000000000 ) ) ;
#7374=CARTESIAN_POINT ( 'NONE',  ( 11.78238356083980065, 1440.882651838439870, 188.1224447589279976 ) ) ;
#7375=CARTESIAN_POINT ( 'NONE',  ( 40.71747597329999735, 1438.773003763650195, 134.0999987698980078 ) ) ;
#7376=FACE_OUTER_BOUND ( 'NONE', #75524, .T. ) ;
#7377=CARTESIAN_POINT ( 'NONE',  ( 27.11300533590000228, 1438.407748754029853, 136.9651466902979848 ) ) ;
#7383=VERTEX_POINT ( 'NONE', #96362 ) ;
#7384=CARTESIAN_POINT ( 'NONE',  ( 11.77725414648410052, 1427.326574604300049, 146.8862230489449985 ) ) ;
#7387=ORIENTED_EDGE ( 'NONE', *, *, #20315, .T. ) ;
#7389=CARTESIAN_POINT ( 'NONE',  ( -16.68463233076019492, 1442.773887286370609, 162.0935120523188857 ) ) ;
#7391=VECTOR ( 'NONE', #16740, 1000.000000000000227 ) ;
#7392=CARTESIAN_POINT ( 'NONE',  ( 24.15268678416311587, 1411.115268795248767, 208.9542267914210925 ) ) ;
#7393=CARTESIAN_POINT ( 'NONE',  ( -12.70045074689999964, 1422.978954057429974, 222.3368426438979952 ) ) ;
#7398=CARTESIAN_POINT ( 'NONE',  ( -16.12193243460000147, 1473.842759945530133, 223.3670126793980160 ) ) ;
#7399=CARTESIAN_POINT ( 'NONE',  ( 15.59938138249999895, 1461.167668198130059, 229.6381429124979832 ) ) ;
#7401=CARTESIAN_POINT ( 'NONE',  ( 13.37887034578663048, 1473.256410945989728, 270.1124231610745596 ) ) ;
#7403=ORIENTED_EDGE ( 'NONE', *, *, #110402, .T. ) ;
#7404=CIRCLE ( 'NONE', #73604, 1.997270720800846444 ) ;
#7409=CARTESIAN_POINT ( 'NONE',  ( -11.60004869885203860, 1425.963618636351384, 138.7040202299609462 ) ) ;
#7414=CARTESIAN_POINT ( 'NONE',  ( -11.66015940019999952, 1426.002483172329903, 146.0081277900980012 ) ) ;
#7419=DIRECTION ( 'NONE',  ( 0.000000000000000000, 0.000000000000000000, -1.000000000000000000 ) ) ;
#7420=CARTESIAN_POINT ( 'NONE',  ( -21.43773211839999959, 1495.369928931229879, 226.0474949278979864 ) ) ;
#7422=CARTESIAN_POINT ( 'NONE',  ( -16.16762553486000087, 1459.157033785442081, 229.6200968447579953 ) ) ;
#7425=CARTESIAN_POINT ( 'NONE',  ( 14.60988619030000102, 1407.613819657329941, 267.1471522769979856 ) ) ;
#7426=CARTESIAN_POINT ( 'NONE',  ( 1.665334536940000074E-16, 1408.913060387329779, 186.4687945730979948 ) ) ;
#7427=CARTESIAN_POINT ( 'NONE',  ( 17.47809751519999821, 1410.883709062829894, 192.6106407635979849 ) ) ;
#7428=EDGE_CURVE ( 'NONE', #46291, #99393, #101196, .T. ) ;
#7431=CARTESIAN_POINT ( 'NONE',  ( -0.5077264128435760027, 1412.020084291579906, 233.2448261540379804 ) ) ;
#7433=CARTESIAN_POINT ( 'NONE',  ( 12.94229023090000119, 1461.456462053329915, 233.4393938603979848 ) ) ;
#7435=CARTESIAN_POINT ( 'NONE',  ( -13.52564516290000007, 1444.429216800270069, 187.6720164552979782 ) ) ;
#7440=CARTESIAN_POINT ( 'NONE',  ( 1.448679645196929933, 1507.129709964000085, 181.1126013477120011 ) ) ;
#7442=CARTESIAN_POINT ( 'NONE',  ( 11.64966881943793808, 1425.711239460408251, 138.1863722522803641 ) ) ;
#7444=CIRCLE ( 'NONE', #14632, 4.004820216691862278 ) ;
#7445=CARTESIAN_POINT ( 'NONE',  ( -23.58453086489999961, 1470.876928620230046, 266.7402721287979830 ) ) ;
#7448=CARTESIAN_POINT ( 'NONE',  ( -17.36863403203877709, 1486.486724665740667, 187.7553479223266777 ) ) ;
#7451=CARTESIAN_POINT ( 'NONE',  ( 11.94473499015900053, 1415.666200591219877, 223.2621103331699999 ) ) ;
#7455=CARTESIAN_POINT ( 'NONE',  ( -0.7469581576472559270, 1395.939144740979827, 220.1009958539310105 ) ) ;
#7458=CARTESIAN_POINT ( 'NONE',  ( -15.03991797343599934, 1422.464147859393734, 228.7611401550659878 ) ) ;
#7460=CARTESIAN_POINT ( 'NONE',  ( -1.600048698852036821, 1402.754281879943164, 137.0999999980979851 ) ) ;
#7473=CARTESIAN_POINT ( 'NONE',  ( -12.92123606608499564, 1398.295999377893168, 210.5944397367629506 ) ) ;
#7481=ORIENTED_EDGE ( 'NONE', *, *, #21895, .F. ) ;
#7482=CARTESIAN_POINT ( 'NONE',  ( 11.87854472459999933, 1434.090690883939942, 150.8572398186979626 ) ) ;
#7483=CARTESIAN_POINT ( 'NONE',  ( -12.90425718179999848, 1398.295578896729921, 211.5077388498779953 ) ) ;
#7485=CARTESIAN_POINT ( 'NONE',  ( 1.475648591298595717E-05, 1397.578653621796548, 222.1218461011892771 ) ) ;
#7486=CARTESIAN_POINT ( 'NONE',  ( 0.2223009155142280091, 1416.826860677879949, 227.1890218400880030 ) ) ;
#7489=CARTESIAN_POINT ( 'NONE',  ( 17.94031933599999817, 1421.715617410530058, 225.1230053650979812 ) ) ;
#7490=CARTESIAN_POINT ( 'NONE',  ( 17.30154577271699878, 1488.410570188420024, 229.9719745730320142 ) ) ;
#7491=CARTESIAN_POINT ( 'NONE',  ( 1.840176472590000056, 1468.706575379429978, 182.8606869624980220 ) ) ;
#7492=CARTESIAN_POINT ( 'NONE',  ( -9.986922776509999267, 1415.932617989529945, 193.6517757706980092 ) ) ;
#7496=CARTESIAN_POINT ( 'NONE',  ( 1.184716195880000100, 1415.245980409429876, 191.1061508846980246 ) ) ;
#7497=CARTESIAN_POINT ( 'NONE',  ( 11.86609764940000034, 1432.335824637460064, 149.9825529227980212 ) ) ;
#7498=CARTESIAN_POINT ( 'NONE',  ( 4.146234843596174002, 1509.069516669909945, 179.8708435902544238 ) ) ;
#7500=CARTESIAN_POINT ( 'NONE',  ( 13.20527699253010034, 1434.869030501559791, 149.0170173390359878 ) ) ;
#7501=ORIENTED_EDGE ( 'NONE', *, *, #45307, .T. ) ;
#7503=CARTESIAN_POINT ( 'NONE',  ( 13.14776788045321609, 1444.759486401034792, 169.3987463143653258 ) ) ;
#7504=CARTESIAN_POINT ( 'NONE',  ( -9.617209207600001974, 1463.011625836029907, 234.9738963373979743 ) ) ;
#7508=VERTEX_POINT ( 'NONE', #29697 ) ;
#7510=LINE ( 'NONE', #75830, #85819 ) ;
#7512=B_SPLINE_CURVE_WITH_KNOTS ( 'NONE', 3,
 ( #99073, #13970, #3409, #56553, #37539, #63325 ),
 .UNSPECIFIED., .F., .F.,
 ( 4, 2, 4 ),
 ( 0.000000000000000000, 0.02504328917203360247, 0.04927314457962859995 ),
 .UNSPECIFIED. ) ;
#7514=ORIENTED_EDGE ( 'NONE', *, *, #98951, .F. ) ;
#7516=ORIENTED_EDGE ( 'NONE', *, *, #22039, .T. ) ;
#7517=CARTESIAN_POINT ( 'NONE',  ( 19.52188586753710098, 1440.913060387330006, 213.1792421281620022 ) ) ;
#7519=EDGE_CURVE ( 'NONE', #92476, #68340, #95620, .T. ) ;
#7520=CARTESIAN_POINT ( 'NONE',  ( -12.59263084910000075, 1409.352804746330094, 190.6087445503980007 ) ) ;
#7523=CARTESIAN_POINT ( 'NONE',  ( 0.3443494227334849556, 1415.932840154009909, 226.9638899044090010 ) ) ;
#7524=EDGE_LOOP ( 'NONE', ( #45606, #56564, #83485, #89018, #89075 ) ) ;
#7525=CARTESIAN_POINT ( 'NONE',  ( 21.53595778569999908, 1429.715726643929884, 219.1980677462979941 ) ) ;
#7530=CARTESIAN_POINT ( 'NONE',  ( 12.94490868551340057, 1411.836793529460010, 269.3560162488220158 ) ) ;
#7532=B_SPLINE_CURVE_WITH_KNOTS ( 'NONE', 5,
 ( #104108, #76698, #44219, #8936, #102985, #17309, #101879, #69993, #18977, #84544, #33574, #60473 ),
 .UNSPECIFIED., .F., .F.,
 ( 6, 3, 3, 6 ),
 ( 0.000000000000000000, 0.2618501547404907814, 0.6384622943148291485, 1.000000000000000000 ),
 .UNSPECIFIED. ) ;
#7533=CARTESIAN_POINT ( 'NONE',  ( 23.56365677970000050, 1409.992931709729874, 209.3923694546319894 ) ) ;
#7537=DIRECTION ( 'NONE',  ( 7.524247891465669597E-10, -7.387944558779740342E-11, 1.000000000000000000 ) ) ;
#7540=CARTESIAN_POINT ( 'NONE',  ( 1.330041181847649856, 1409.969615095589916, 232.6005830404007213 ) ) ;
#7545=CARTESIAN_POINT ( 'NONE',  ( 38.77643282620000065, 1448.325309301239713, 259.1405302821979717 ) ) ;
#7546=CARTESIAN_POINT ( 'NONE',  ( -16.81223434880759982, 1414.913060387349788, 207.5743820648510223 ) ) ;
#7547=CARTESIAN_POINT ( 'NONE',  ( -8.733798672629999871, 1419.056601762730224, 233.0476203166980156 ) ) ;
#7549=CARTESIAN_POINT ( 'NONE',  ( -24.05825847430000053, 1444.359855996980059, 212.4695695426480029 ) ) ;
#7552=CARTESIAN_POINT ( 'NONE',  ( -35.00335893040000457, 1443.851131231850104, 135.3147355765980251 ) ) ;
#7558=CARTESIAN_POINT ( 'NONE',  ( -27.01380866140000236, 1450.681584507220123, 136.4483241423979791 ) ) ;
#7559=CARTESIAN_POINT ( 'NONE',  ( 12.45806603379999977, 1422.765585813930102, 223.7640243073979889 ) ) ;
#7560=CARTESIAN_POINT ( 'NONE',  ( 38.22966134442160069, 1444.824641043079964, 137.0630644299180005 ) ) ;
#7562=CARTESIAN_POINT ( 'NONE',  ( 26.08557971843411138, 1450.768665719140927, 136.6909322435282377 ) ) ;
#7563=CARTESIAN_POINT ( 'NONE',  ( 0.000000000000000000, 1443.913060387330006, 126.8032249175980155 ) ) ;
#7564=CARTESIAN_POINT ( 'NONE',  ( 29.17443018255550058, 1436.411321637160199, 136.6577757746120199 ) ) ;
#7565=CARTESIAN_POINT ( 'NONE',  ( -38.64468767635309376, 1444.005792560380087, 137.1818110982019903 ) ) ;
#7566=CARTESIAN_POINT ( 'NONE',  ( -21.73794315169999791, 1429.924065208830143, 218.8049817396780270 ) ) ;
#7569=EDGE_CURVE ( 'NONE', #46920, #9209, #87710, .T. ) ;
#7570=CARTESIAN_POINT ( 'NONE',  ( 13.97274253350000173, 1508.900194118629997, 185.2208288689979838 ) ) ;
#7572=CARTESIAN_POINT ( 'NONE',  ( -16.15327634166941095, 1469.074778267816782, 269.3697231530343288 ) ) ;
#7573=ORIENTED_EDGE ( 'NONE', *, *, #93872, .F. ) ;
#7574=CARTESIAN_POINT ( 'NONE',  ( -26.31257376103580370, 1482.825501787880057, 210.8488302918380271 ) ) ;
#7577=CARTESIAN_POINT ( 'NONE',  ( 13.86092937120069912, 1410.765486813650114, 191.1266627561969926 ) ) ;
#7578=CARTESIAN_POINT ( 'NONE',  ( -1.802301101800737992, 1409.910657974563946, 186.0681198055114862 ) ) ;
#7579=CARTESIAN_POINT ( 'NONE',  ( -12.86383581051971525, 1444.953095748689520, 186.0976155970778052 ) ) ;
#7582=CARTESIAN_POINT ( 'NONE',  ( -12.68222283512827353, 1419.450370853951199, 228.4188145333208411 ) ) ;
#7583=CARTESIAN_POINT ( 'NONE',  ( -3.387022137372330821, 1451.546079549640808, 153.9286616154712419 ) ) ;
#7584=CARTESIAN_POINT ( 'NONE',  ( -18.04214276402350237, 1416.520646088689773, 209.4829372689819706 ) ) ;
#7585=CARTESIAN_POINT ( 'NONE',  ( 25.62964228539999922, 1435.682999602769996, 136.4541818545979766 ) ) ;
#7588=CARTESIAN_POINT ( 'NONE',  ( -0.2210724871084639997, 1414.913057862230062, 192.7532066038650100 ) ) ;
#7589=CARTESIAN_POINT ( 'NONE',  ( 21.22517422831483458, 1508.705765652955961, 226.2458636531372633 ) ) ;
#7595=CARTESIAN_POINT ( 'NONE',  ( -12.77219964900000093, 1461.479478047029943, 231.7859092782980213 ) ) ;
#7597=CARTESIAN_POINT ( 'NONE',  ( -11.87549035710000034, 1433.045081316169899, 150.0791374503980080 ) ) ;
#7600=CARTESIAN_POINT ( 'NONE',  ( -2.681752544285345596, 1420.275109781218589, 185.9665801933430487 ) ) ;
#7602=CARTESIAN_POINT ( 'NONE',  ( -14.52664492645137351, 1429.813426209209183, 222.1557458822846627 ) ) ;
#7604=CARTESIAN_POINT ( 'NONE',  ( 1.530053592280000041, 1452.704408633029971, 183.4894966516980048 ) ) ;
#7606=CARTESIAN_POINT ( 'NONE',  ( -27.54257285163602020, 1509.986926926110982, 197.2303957788377318 ) ) ;
#7607=CARTESIAN_POINT ( 'NONE',  ( -2.797860769668700114E-09, 1414.981275559920050, 244.4714746855989915 ) ) ;
#7608=VERTEX_POINT ( 'NONE', #97624 ) ;
#7610=CARTESIAN_POINT ( 'NONE',  ( -11.74434471530499913, 1426.711920943479981, 144.6829737354520091 ) ) ;
#7611=DIRECTION ( 'NONE',  ( -0.01734307837366609595, 0.9988445490243716973, 0.04481946582484658964 ) ) ;
#7612=CARTESIAN_POINT ( 'NONE',  ( -4.146669009850000975, 1471.900945888130082, 270.0721599525979855 ) ) ;
#7613=CARTESIAN_POINT ( 'NONE',  ( 12.21136012500357637, 1434.092705541917667, 147.4644113196944204 ) ) ;
#7615=CARTESIAN_POINT ( 'NONE',  ( 18.65529551030000022, 1453.313060387329870, 201.7949864999779948 ) ) ;
#7621=CARTESIAN_POINT ( 'NONE',  ( -6.126475865403940624, 1406.019691185119882, 267.8379111553729786 ) ) ;
#7622=CARTESIAN_POINT ( 'NONE',  ( -13.07119275721439955, 1435.903469544349946, 150.6799624932950223 ) ) ;
#7623=VERTEX_POINT ( 'NONE', #72437 ) ;
#7632=DIRECTION ( 'NONE',  ( 0.000000000000000000, 0.000000000000000000, -1.000000000000000000 ) ) ;
#7633=VERTEX_POINT ( 'NONE', #4663 ) ;
#7640=CARTESIAN_POINT ( 'NONE',  ( -1.117292507960000014, 1467.878890391829827, 230.3293191710980068 ) ) ;
#7643=CARTESIAN_POINT ( 'NONE',  ( -2.590851938810000199, 1407.641758401829975, 196.2196012994980094 ) ) ;
#7644=CARTESIAN_POINT ( 'NONE',  ( -24.08426305480000451, 1411.115211393229856, 208.6111285346999864 ) ) ;
#7646=ORIENTED_EDGE ( 'NONE', *, *, #107638, .T. ) ;
#7647=CARTESIAN_POINT ( 'NONE',  ( -26.29896967323349699, 1469.338024908179932, 210.2737814497969850 ) ) ;
#7648=CARTESIAN_POINT ( 'NONE',  ( 26.64485081109999953, 1469.250187268130048, 209.0988510226020196 ) ) ;
#7652=CARTESIAN_POINT ( 'NONE',  ( -13.08109920040210028, 1436.034850317789960, 150.7074356796669861 ) ) ;
#7653=CARTESIAN_POINT ( 'NONE',  ( 0.1595995995380000143, 1486.508831850330125, 181.8147405652979671 ) ) ;
#7656=CARTESIAN_POINT ( 'NONE',  ( -2.065269763300760175, 1484.249225516169872, 183.0195811470669867 ) ) ;
#7658=CARTESIAN_POINT ( 'NONE',  ( 18.80463394749709138, 1425.801072080043696, 225.6039047707025134 ) ) ;
#7661=CARTESIAN_POINT ( 'NONE',  ( -38.81202645930000017, 1450.612734574169963, 134.0999998922980012 ) ) ;
#7664=CARTESIAN_POINT ( 'NONE',  ( 10.78872034293299897, 1416.913057013769958, 222.2791104510660034 ) ) ;
#7667=CARTESIAN_POINT ( 'NONE',  ( 12.92083169069850079, 1434.847021224489936, 149.8557914971470097 ) ) ;
#7668=CARTESIAN_POINT ( 'NONE',  ( 7.829103442970730242, 1468.998337108560008, 233.3189757471670021 ) ) ;
#7669=EDGE_CURVE ( 'NONE', #68439, #8198, #47635, .T. ) ;
#7671=CARTESIAN_POINT ( 'NONE',  ( -11.11039799191612509, 1425.147017898752893, 138.4692043722531594 ) ) ;
#7675=CARTESIAN_POINT ( 'NONE',  ( 4.232343036945110271, 1441.513652504289894, 164.4116054800499853 ) ) ;
#7677=CARTESIAN_POINT ( 'NONE',  ( -7.000000000000000000, 1432.413060387330006, 146.1721969590979882 ) ) ;
#7678=CARTESIAN_POINT ( 'NONE',  ( 21.01954381400000216, 1509.698214756829884, 188.0278171981979938 ) ) ;
#7681=CARTESIAN_POINT ( 'NONE',  ( -12.45685420760000106, 1416.832348283729971, 194.7671534681980177 ) ) ;
#7684=CARTESIAN_POINT ( 'NONE',  ( 1.192913453829999915, 1420.839100914329947, 183.5603160090979884 ) ) ;
#7687=CARTESIAN_POINT ( 'NONE',  ( -11040.89558200930696, 2833.596074015641989, -8386.665009981023104 ) ) ;
#7689=CARTESIAN_POINT ( 'NONE',  ( -16.17568633703940151, 1459.146939663510011, 230.7169128052520080 ) ) ;
#7690=CARTESIAN_POINT ( 'NONE',  ( 17.31687731428424115, 1422.595274621808130, 226.6249846890611650 ) ) ;
#7692=CARTESIAN_POINT ( 'NONE',  ( -7.390160694869999602, 1438.194204504490017, 149.6789596403979772 ) ) ;
#7693=CARTESIAN_POINT ( 'NONE',  ( 42.25133546600230261, 1440.913060352949969, 262.2708174827409948 ) ) ;
#7696=DIRECTION ( 'NONE',  ( 0.000000000000000000, 0.000000000000000000, -1.000000000000000000 ) ) ;
#7698=ORIENTED_EDGE ( 'NONE', *, *, #33959, .F. ) ;
#7699=CARTESIAN_POINT ( 'NONE',  ( 14.43915977099999992, 1435.431951939009878, 149.5788185351979962 ) ) ;
#7700=CARTESIAN_POINT ( 'NONE',  ( -19.42676974918696331, 1485.587889656283323, 189.9363221898242671 ) ) ;
#7702=CARTESIAN_POINT ( 'NONE',  ( 2.294753475282899302, 1410.371478230091043, 185.5182217525652675 ) ) ;
#7703=LINE ( 'NONE', #41863, #55387 ) ;
#7704=CARTESIAN_POINT ( 'NONE',  ( 16.06472692613853681, 1509.595107636989042, 234.5263603880145524 ) ) ;
#7706=CARTESIAN_POINT ( 'NONE',  ( 33.91369120210129751, 1435.681798817170147, 134.0999999980979851 ) ) ;
#7709=CARTESIAN_POINT ( 'NONE',  ( -0.01367056625530000021, 1452.767332469330086, 153.3854620859980002 ) ) ;
#7714=ORIENTED_EDGE ( 'NONE', *, *, #33706, .T. ) ;
#7715=FACE_OUTER_BOUND ( 'NONE', #30958, .T. ) ;
#7719=ORIENTED_EDGE ( 'NONE', *, *, #74104, .T. ) ;
#7720=CARTESIAN_POINT ( 'NONE',  ( -13.50563910776669907, 1440.103950034289710, 194.8057323916819996 ) ) ;
#7722=CARTESIAN_POINT ( 'NONE',  ( 36.58809064867419636, 1437.689614402119787, 136.5472558022989915 ) ) ;
#7724=DIRECTION ( 'NONE',  ( 0.03489949670250495212, 0.9993908270190956511, 0.000000000000000000 ) ) ;
#7729=CARTESIAN_POINT ( 'NONE',  ( -3.827327205999999649, 1422.542708386029972, 168.6405287067979941 ) ) ;
#7732=CARTESIAN_POINT ( 'NONE',  ( 2.322154075020000263, 1410.372404442829975, 185.5255194826980016 ) ) ;
#7733=CARTESIAN_POINT ( 'NONE',  ( 1.031331416711620097, 1508.991934534589973, 179.4420581554169871 ) ) ;
#7735=CARTESIAN_POINT ( 'NONE',  ( -3.116664625471300187, 1441.244075315679993, 166.9150288857020143 ) ) ;
#7737=CARTESIAN_POINT ( 'NONE',  ( -24.24033364359999965, 1452.066569283630088, 137.1576854437979875 ) ) ;
#7738=ORIENTED_EDGE ( 'NONE', *, *, #11122, .T. ) ;
#7740=FACE_OUTER_BOUND ( 'NONE', #30378, .T. ) ;
#7741=CARTESIAN_POINT ( 'NONE',  ( 19.58792912137019826, 1456.031451223419936, 227.9529518234539864 ) ) ;
#7742=DIRECTION ( 'NONE',  ( -0.9822959463214659959, 0.1391731009602450164, 0.1254014426134129889 ) ) ;
#7743=CARTESIAN_POINT ( 'NONE',  ( 17.91320533999999753, 1507.617064948130064, 188.5294956351980318 ) ) ;
#7745=CARTESIAN_POINT ( 'NONE',  ( -9.767263980911179754E-11, 1470.490992744460073, 255.3083357207799793 ) ) ;
#7750=CARTESIAN_POINT ( 'NONE',  ( -0.2620786904165167130, 1485.927256572733086, 181.8391900102611203 ) ) ;
#7752=CARTESIAN_POINT ( 'NONE',  ( -46.12691182732100259, 1439.415857468709874, 266.9728105068039667 ) ) ;
#7753=CARTESIAN_POINT ( 'NONE',  ( 13.88631813555559980, 1509.307012642660084, 234.3182586601199944 ) ) ;
#7758=CARTESIAN_POINT ( 'NONE',  ( 12.63038619288439968, 1428.207532477410041, 223.9332333053530135 ) ) ;
#7760=CARTESIAN_POINT ( 'NONE',  ( -25.92826244057819807, 1451.942608940840046, 135.5698208547320007 ) ) ;
#7761=ORIENTED_EDGE ( 'NONE', *, *, #26199, .T. ) ;
#7762=CARTESIAN_POINT ( 'NONE',  ( 11.60711259459999845, 1422.283843339130044, 221.4360218614980340 ) ) ;
#7767=CARTESIAN_POINT ( 'NONE',  ( -20.40418802293068623, 1454.957320664023200, 226.6330256283032725 ) ) ;
#7769=EDGE_CURVE ( 'NONE', #20179, #73741, #107496, .T. ) ;
#7770=CARTESIAN_POINT ( 'NONE',  ( -13.95553461971410414, 1416.818673879764901, 221.9083874777307130 ) ) ;
#7772=CARTESIAN_POINT ( 'NONE',  ( -4.820018915960121220, 1409.974924445299848, 270.0724225275779418 ) ) ;
#7773=CARTESIAN_POINT ( 'NONE',  ( 15.99884507355850083, 1421.963095027500003, 227.5209166517219899 ) ) ;
#7774=CARTESIAN_POINT ( 'NONE',  ( -0.2746046721839675020, 1507.636717399409008, 237.3923158053290763 ) ) ;
#7775=ORIENTED_EDGE ( 'NONE', *, *, #2245, .F. ) ;
#7776=ORIENTED_EDGE ( 'NONE', *, *, #10600, .F. ) ;
#7777=B_SPLINE_CURVE_WITH_KNOTS ( 'NONE', 5,
 ( #88083, #89162, #52825, #87525, #11371, #2987 ),
 .UNSPECIFIED., .F., .F.,
 ( 6, 6 ),
 ( 0.000000000000000000, 1.000000000000000000 ),
 .UNSPECIFIED. ) ;
#7778=CARTESIAN_POINT ( 'NONE',  ( -23.94120819599999805, 1410.421789068329872, 209.3772794782499886 ) ) ;
#7783=EDGE_CURVE ( 'NONE', #90951, #54360, #98182, .T. ) ;
#7784=CARTESIAN_POINT ( 'NONE',  ( -2.833554060450000023, 1507.639777131729943, 236.8757964686979847 ) ) ;
#7785=CARTESIAN_POINT ( 'NONE',  ( -17.85390903009999874, 1410.880990427929873, 225.0173061825979914 ) ) ;
#7786=CARTESIAN_POINT ( 'NONE',  ( 45.81235299787979898, 1442.782150107359939, 268.7577288735689649 ) ) ;
#7787=CARTESIAN_POINT ( 'NONE',  ( -0.8768788928080630818, 1424.155975923929873, 228.3063952870599849 ) ) ;
#7788=CARTESIAN_POINT ( 'NONE',  ( -16.94513000609982356, 1421.950298552636241, 226.8362257794649111 ) ) ;
#7791=CARTESIAN_POINT ( 'NONE',  ( 19.00830952430770893, 1457.291692359948456, 226.5122007821947818 ) ) ;
#7793=LINE ( 'NONE', #68838, #62312 ) ;
#7796=CARTESIAN_POINT ( 'NONE',  ( 27.02941372530000308, 1451.801869924330049, 135.6489090826979975 ) ) ;
#7803=CARTESIAN_POINT ( 'NONE',  ( 1.762714104866460074, 1408.974615720260090, 186.8633000340620072 ) ) ;
#7804=CARTESIAN_POINT ( 'NONE',  ( 1.265494006419999984, 1415.708214660429803, 232.9654935851980042 ) ) ;
#7805=DIRECTION ( 'NONE',  ( -1.000000000000000000, 0.000000000000000000, 0.000000000000000000 ) ) ;
#7806=CARTESIAN_POINT ( 'NONE',  ( 15.26168084529999902, 1409.446010026229715, 225.6870430949980175 ) ) ;
#7809=CARTESIAN_POINT ( 'NONE',  ( 17.22592475670000312, 1444.324653571829913, 162.9227486557980171 ) ) ;
#7810=ORIENTED_EDGE ( 'NONE', *, *, #25761, .T. ) ;
#7811=CARTESIAN_POINT ( 'NONE',  ( 12.60587301698949858, 1415.938742849230039, 221.9392866525910222 ) ) ;
#7812=CARTESIAN_POINT ( 'NONE',  ( 11.50213335426050065, 1432.340329806790123, 151.2059253680629922 ) ) ;
#7818=CARTESIAN_POINT ( 'NONE',  ( -37.18025134340000193, 1449.733372748519969, 265.6112251771979800 ) ) ;
#7820=CARTESIAN_POINT ( 'NONE',  ( 11.88085280169999969, 1433.210362566009962, 150.1928659671980029 ) ) ;
#7821=CARTESIAN_POINT ( 'NONE',  ( 31.32742178079999462, 1444.517716078169997, 255.3819207742980097 ) ) ;
#7822=CARTESIAN_POINT ( 'NONE',  ( 12.50239138351419932, 1416.520646088689773, 196.1087943541830043 ) ) ;
#7827=CARTESIAN_POINT ( 'NONE',  ( 2.370970874524633398, 1427.002265528473799, 137.0999999980980135 ) ) ;
#7829=CARTESIAN_POINT ( 'NONE',  ( -17.03047024470000181, 1409.672928417430057, 225.3166904351979838 ) ) ;
#7830=CARTESIAN_POINT ( 'NONE',  ( 23.92333147209999922, 1430.353917304629931, 213.3463240754979893 ) ) ;
#7833=CARTESIAN_POINT ( 'NONE',  ( -1.085894894499999928E-15, 1432.353341358199941, 150.3995506339979897 ) ) ;
#7840=CARTESIAN_POINT ( 'NONE',  ( 0.1690262106856909863, 1480.902069235160070, 182.0556410569679997 ) ) ;
#7843=CARTESIAN_POINT ( 'NONE',  ( -13.26516604059999693, 1444.994950788470987, 176.9857848810979704 ) ) ;
#7846=CARTESIAN_POINT ( 'NONE',  ( -40.66293689394410649, 1439.821779689789992, 134.0999999980979851 ) ) ;
#7847=CARTESIAN_POINT ( 'NONE',  ( -29.38941616001999790, 1446.173485192630096, 137.1432708197739885 ) ) ;
#7849=B_SPLINE_SURFACE_WITH_KNOTS ( 'NONE', 5, 5, ( 
 ( #110363, #33640, #25233, #86262, #52133, #9550 ),
 ( #52682, #86818, #26919, #34760, #78996, #35312 ),
 ( #87381, #43176, #95771, #19037, #105275, #9003 ),
 ( #104171, #19603, #62198, #629, #68947, #103047 ),
 ( #10110, #43720, #36410, #60543, #44282, #78426 ),
 ( #26345, #95223, #69498, #104720, #20151, #77873 ) ),
 .UNSPECIFIED., .F., .F., .F.,
 ( 6, 6 ),
 ( 6, 6 ),
 ( 29.52656374780000093, 158.0439293190000001 ),
 ( 0.000000000000000000, 1.000000000000000000 ),
 .UNSPECIFIED. ) ;
#7853=CARTESIAN_POINT ( 'NONE',  ( -28.84709929359999947, 1507.919204203629988, 212.2396942135479776 ) ) ;
#7857=CARTESIAN_POINT ( 'NONE',  ( 7.650637082874630401, 1409.180226521390068, 221.9865298110669869 ) ) ;
#7858=CARTESIAN_POINT ( 'NONE',  ( 2.500000002320000192, 1428.690610018730013, 183.7723879534980256 ) ) ;
#7865=CARTESIAN_POINT ( 'NONE',  ( -30.94580556280000039, 1451.832637120030085, 135.2368415506980170 ) ) ;
#7866=CARTESIAN_POINT ( 'NONE',  ( 13.35741048202589809, 1443.501467202830099, 164.9741927960640453 ) ) ;
#7870=CARTESIAN_POINT ( 'NONE',  ( -18.70871766619247722, 1410.928537324267609, 223.5363647290388940 ) ) ;
#7872=CARTESIAN_POINT ( 'NONE',  ( -0.1681676274470000065, 1420.473121337229941, 182.7663689088979879 ) ) ;
#7873=CARTESIAN_POINT ( 'NONE',  ( 38.93029842025811860, 1452.410457501353221, 269.5917637810125598 ) ) ;
#7874=CARTESIAN_POINT ( 'NONE',  ( 17.95066969181503325, 1434.914995825377446, 215.4365105091481496 ) ) ;
#7875=CARTESIAN_POINT ( 'NONE',  ( 1.797565579689999860, 1415.903556134529936, 232.4419632246980143 ) ) ;
#7877=CARTESIAN_POINT ( 'NONE',  ( -23.79097509939970934, 1507.893976353429935, 222.8398596609989966 ) ) ;
#7878=CARTESIAN_POINT ( 'NONE',  ( 3.679272716979999913, 1453.313060387329870, 228.5941172881979924 ) ) ;
#7881=CARTESIAN_POINT ( 'NONE',  ( 2.704615531860000033, 1447.046937274380070, 168.9986710020979785 ) ) ;
#7884=CARTESIAN_POINT ( 'NONE',  ( 13.44384801999999901, 1473.247726564130062, 270.1124235791980368 ) ) ;
#7890=CARTESIAN_POINT ( 'NONE',  ( -25.29760786810000184, 1449.800867303260020, 206.6892432500980306 ) ) ;
#7891=CARTESIAN_POINT ( 'NONE',  ( -11.18153660112279901, 1426.464409952729966, 103.8952900393150003 ) ) ;
#7892=CARTESIAN_POINT ( 'NONE',  ( 16.15008297119439717, 1409.578690898410059, 192.4543258895550082 ) ) ;
#7894=CARTESIAN_POINT ( 'NONE',  ( 40.62990447646500058, 1439.681968513619950, 135.2802037849949954 ) ) ;
#7897=CARTESIAN_POINT ( 'NONE',  ( -11.15477664960000048, 1425.160652183429875, 144.1598853320980140 ) ) ;
#7899=CARTESIAN_POINT ( 'NONE',  ( 17.11202944081011168, 1460.312853445443579, 228.6673605825106392 ) ) ;
#7904=VERTEX_POINT ( 'NONE', #9350 ) ;
#7910=CARTESIAN_POINT ( 'NONE',  ( -29.71787946601863339, 1509.988004069222825, 210.0607825035318115 ) ) ;
#7915=AXIS2_PLACEMENT_3D ( 'NONE', #31833, #4973, #40788 ) ;
#7918=CARTESIAN_POINT ( 'NONE',  ( 40.71747596589879947, 1438.773003663980035, 134.7402664639769796 ) ) ;
#7921=CARTESIAN_POINT ( 'NONE',  ( 25.40031078099999817, 1438.607438808799998, 138.1536180571980026 ) ) ;
#7924=ORIENTED_EDGE ( 'NONE', *, *, #106730, .T. ) ;
#7927=ORIENTED_EDGE ( 'NONE', *, *, #85881, .F. ) ;
#7930=CARTESIAN_POINT ( 'NONE',  ( 20.28670476199999939, 1497.716955700230073, 227.3610620833980249 ) ) ;
#7932=CARTESIAN_POINT ( 'NONE',  ( -13.79060599709999835, 1416.547221146729953, 221.8961093151980037 ) ) ;
#7933=CARTESIAN_POINT ( 'NONE',  ( -11.83148324045470012, 1432.336210885780019, 150.3814747831369800 ) ) ;
#7936=CARTESIAN_POINT ( 'NONE',  ( -13.30235076369999980, 1426.047137753730112, 222.1935098235980206 ) ) ;
#7938=CARTESIAN_POINT ( 'NONE',  ( -8.568239406770191025, 1446.651419842080713, 153.8735861858707210 ) ) ;
#7939=CARTESIAN_POINT ( 'NONE',  ( -0.03625434476629999653, 1508.564801718729768, 180.3428531422979972 ) ) ;
#7942=CARTESIAN_POINT ( 'NONE',  ( -14.66954656289999903, 1451.336034133729981, 222.9742526267980054 ) ) ;
#7945=CARTESIAN_POINT ( 'NONE',  ( -4.546321247799015808, 1423.767664050271151, 184.3780306669439426 ) ) ;
#7947=CARTESIAN_POINT ( 'NONE',  ( -5.365571251823850751, 1422.412084457530000, 136.7230467533039757 ) ) ;
#7949=CARTESIAN_POINT ( 'NONE',  ( -1.307006097452011906, 1486.249936161337018, 181.8003811105465104 ) ) ;
#7952=CARTESIAN_POINT ( 'NONE',  ( -2.902304511463737136, 1484.512052158883762, 183.2899361315264741 ) ) ;
#7954=CARTESIAN_POINT ( 'NONE',  ( -11.60004869885203860, 1426.112400841504041, 139.0398264042692063 ) ) ;
#7960=CARTESIAN_POINT ( 'NONE',  ( -11.44957079769999986, 1425.470528643129910, 145.1412166744979970 ) ) ;
#7961=CARTESIAN_POINT ( 'NONE',  ( -10.84547348403736322, 1425.250141514038660, 146.5429171640950585 ) ) ;
#7962=CARTESIAN_POINT ( 'NONE',  ( -4.055165558009999671, 1441.344553830540008, 184.7145706676980126 ) ) ;
#7963=CARTESIAN_POINT ( 'NONE',  ( 14.38071331779389794, 1509.494653947579991, 235.3234850005289900 ) ) ;
#7966=CARTESIAN_POINT ( 'NONE',  ( -20.02122337150000320, 1470.088377314129957, 226.2655331251979760 ) ) ;
#7968=CARTESIAN_POINT ( 'NONE',  ( -17.15404056067600180, 1460.895016437030108, 228.2717488779379948 ) ) ;
#7969=ORIENTED_EDGE ( 'NONE', *, *, #40056, .T. ) ;
#7971=CARTESIAN_POINT ( 'NONE',  ( 21.63331298869999841, 1410.785270426130182, 269.4984061937980186 ) ) ;
#7973=CARTESIAN_POINT ( 'NONE',  ( 19.33005223189999811, 1449.732321041979958, 192.5069533228979992 ) ) ;
#7974=CARTESIAN_POINT ( 'NONE',  ( -0.1513279769116150086, 1507.119540709420107, 237.3446492454640122 ) ) ;
#7976=CARTESIAN_POINT ( 'NONE',  ( -1.555019539419999930, 1450.617762354220076, 182.9982681214980005 ) ) ;
#7977=B_SPLINE_CURVE_WITH_KNOTS ( 'NONE', 3,
 ( #59570, #95371, #44991, #774, #1887, #94248, #34902, #76922, #85860, #53384, #36023, #18635, #52832, #69089, #103190, #1318, #86410, #9700, #25378, #78011, #70214, #35459, #87533, #104318, #10821, #79138, #20846, #88089, #64545, #5157, #79687, #12993, #98108, #104872, #97574, #96474, #11376, #30354, #3543, #37113, #105988, #88638, #12460, #62350, #63456, #55592, #71314, #4619, #81855, #55042, #63997, #62924, #89169, #45548, #46643, #38755, #47723, #105428, #89716, #47176, #107069, #37666, #21927, #19754, #80225, #72930, #2993, #56120, #98664, #53955, #28717, #71872, #97035, #90255, #13537, #54502, #20298, #11916, #28162, #46093, #29263, #72392, #70760, #80777, #81304, #4084, #38208, #106521, #29809, #21382, #15724, #40958, #6799, #48842, #82427, #49378, #74032, #82966, #50486, #90812, #58328, #14655, #33105, #5722, #84609, #108719, #100318, #56677, #67294, #39315, #48284, #92453, #66745, #73485, #66199, #65083, #14095, #109824, #6260, #39866, #74584, #57248, #91912, #30905 ),
 .UNSPECIFIED., .F., .F.,
 ( 4, 3, 3, 3, 3, 3, 3, 3, 3, 3, 3, 3, 3, 3, 3, 3, 3, 3, 3, 3, 3, 3, 3, 3, 3, 3, 3, 3, 3, 3, 3, 3, 3, 3, 3, 3, 3, 3, 3, 3, 3, 4 ),
 ( 1.525827422200500012E-12, 0.7233976230870560187, 1.453179569741549937, 2.189205328521389937, 2.931232241145099948, 3.681692766298920283, 4.436664690071680184, 5.195519429214390250, 5.957507372262750067, 6.722615320280829643, 7.488461881906269824, 8.253940118726170283, 8.872098167640000810, 9.627621990570389698, 10.37987637364419946, 11.12818954277669903, 11.87201083186580064, 12.60808579110319982, 13.25493343014260006, 13.90338779108970080, 14.62763215072740053, 14.71347577215040126, 15.43831616715549870, 16.16939286010799748, 16.92109434835699844, 17.66675291633200118, 18.41722697190180114, 19.17198454560039877, 19.93209662288229822, 20.69429497494040149, 21.45845626021019825, 22.18300476610000160, 22.94765126737859973, 23.71051286168500027, 24.46875718313560100, 25.22311654196029806, 25.97295706232930002, 26.71776956687309834, 27.45421738225800112, 28.18570414815399872, 28.90920564465159970, 29.42721172040000610 ),
 .UNSPECIFIED. ) ;
#7978=CARTESIAN_POINT ( 'NONE',  ( 2.994688454485729956, 1464.609795419120246, 236.6065850994260131 ) ) ;
#7981=CARTESIAN_POINT ( 'NONE',  ( -14.66018946070000162, 1444.034773379980152, 188.9384452558980172 ) ) ;
#7982=CARTESIAN_POINT ( 'NONE',  ( -17.35500899530000041, 1519.913060387329779, 225.0914276473980067 ) ) ;
#7985=CARTESIAN_POINT ( 'NONE',  ( 1.464604549361590013, 1491.527831886150125, 181.7930722882989869 ) ) ;
#7986=CARTESIAN_POINT ( 'NONE',  ( -9.562842837499999860, 1427.428384263329917, 219.6133833293980047 ) ) ;
#7987=B_SPLINE_CURVE_WITH_KNOTS ( 'NONE', 5,
 ( #63657, #39531, #30573, #21046, #37883, #38415, #97772, #29462, #55248, #22140, #47931, #37330 ),
 .UNSPECIFIED., .F., .F.,
 ( 6, 3, 3, 6 ),
 ( 0.000000000000000000, 3.329846645400000416, 4.930332151970000076, 12.58720418400000085 ),
 .UNSPECIFIED. ) ;
#7990=CARTESIAN_POINT ( 'NONE',  ( -14.47363261859999994, 1473.619884778130199, 269.4256078961980165 ) ) ;
#7991=CARTESIAN_POINT ( 'NONE',  ( 1.356522472024429993, 1410.335674015750101, 232.6399073486850000 ) ) ;
#7993=CARTESIAN_POINT ( 'NONE',  ( -25.78156413019999960, 1509.813372445429877, 223.1298229008980059 ) ) ;
#7997=CARTESIAN_POINT ( 'NONE',  ( -6.692947047070000544, 1442.760174925260117, 154.8612665581980252 ) ) ;
#7999=CARTESIAN_POINT ( 'NONE',  ( -24.15811863269659909, 1444.790571029629973, 211.5220723686269935 ) ) ;
#8002=CARTESIAN_POINT ( 'NONE',  ( -22.45312464719999923, 1409.861582708429978, 204.8525374248079913 ) ) ;
#8007=CARTESIAN_POINT ( 'NONE',  ( -4.714294778569999749E-15, 1435.943783413959864, 150.5249316333980119 ) ) ;
#8011=CARTESIAN_POINT ( 'NONE',  ( -22.55885438500000006, 1410.621632387330010, 211.7835870406779861 ) ) ;
#8013=CARTESIAN_POINT ( 'NONE',  ( 11.70658720183600110, 1426.715707391050046, 141.9907706309280115 ) ) ;
#8019=CARTESIAN_POINT ( 'NONE',  ( -12.60641157257676603, 1398.286779454209181, 212.2965709224484954 ) ) ;
#8020=FACE_OUTER_BOUND ( 'NONE', #56108, .T. ) ;
#8022=CARTESIAN_POINT ( 'NONE',  ( 1.457628745759999900, 1507.679360684230005, 236.7889182215979815 ) ) ;
#8027=CARTESIAN_POINT ( 'NONE',  ( 11.29013490629070127, 1434.173224897529963, 151.5467475927899841 ) ) ;
#8028=CARTESIAN_POINT ( 'NONE',  ( 0.006135582747789999729, 1395.974572298430076, 220.7500239725980009 ) ) ;
#8030=CARTESIAN_POINT ( 'NONE',  ( -0.0002528412978207496297, 1396.454035521046762, 221.4895412923443985 ) ) ;
#8033=CARTESIAN_POINT ( 'NONE',  ( 17.10397118209110090, 1459.366159650030113, 190.0191433627400102 ) ) ;
#8034=CARTESIAN_POINT ( 'NONE',  ( 17.75627633020000218, 1419.037206885730029, 225.8504925643980243 ) ) ;
#8035=CARTESIAN_POINT ( 'NONE',  ( 18.06964159120650137, 1488.412039253179955, 229.4705429282849991 ) ) ;
#8036=B_SPLINE_CURVE_WITH_KNOTS ( 'NONE', 3,
 ( #26796, #61531, #33516, #60984, #26232, #17813, #95660, #53125, #87262, #67718, #10556, #11123, #36854, #88367, #11657, #106803, #104612, #54241, #46938, #80523, #4371, #71047, #27906, #45832, #62090, #89463, #30093, #28460, #79423, #96215, #54779, #55331, #97310, #64287, #29552, #45282, #63737, #78880, #29017, #98408, #70494, #3839, #88911 ),
 .UNSPECIFIED., .F., .F.,
 ( 4, 3, 3, 3, 3, 3, 3, 3, 3, 3, 3, 3, 3, 3, 4 ),
 ( 0.7655572723440000615, 0.9910019269298769862, 1.224379706003839940, 1.462078625881179983, 1.704827365636400138, 1.793853281190000093, 2.038466594486210148, 2.281256481516179768, 2.316155491860000026, 2.583989317150000353, 2.855920922269310047, 3.139267324261280301, 3.387490793020000002, 3.680707212640610404, 3.835724788559999876 ),
 .UNSPECIFIED. ) ;
#8037=CARTESIAN_POINT ( 'NONE',  ( 4.249520622459999508, 1449.235034532409827, 184.3503851686980113 ) ) ;
#8038=CARTESIAN_POINT ( 'NONE',  ( -2.763735881080000123, 1415.425644477329797, 191.8448309814980064 ) ) ;
#8040=CARTESIAN_POINT ( 'NONE',  ( 3.067664574526319576, 1396.020185594800068, 198.5347274153989758 ) ) ;
#8041=CARTESIAN_POINT ( 'NONE',  ( 14.43002663333369995, 1416.512142030569976, 196.8803429896850048 ) ) ;
#8042=CIRCLE ( 'NONE', #101134, 1.999999954277524639 ) ;
#8043=CARTESIAN_POINT ( 'NONE',  ( 11.29278012259999997, 1431.667649477319856, 151.4912647795979979 ) ) ;
#8046=CARTESIAN_POINT ( 'NONE',  ( 13.22467655529630015, 1434.956598927620007, 149.6122180398979822 ) ) ;
#8049=CARTESIAN_POINT ( 'NONE',  ( 13.46491591593493631, 1444.254331750074925, 169.3609691702259852 ) ) ;
#8050=CARTESIAN_POINT ( 'NONE',  ( -8.808667445430000242, 1463.337573581429979, 235.3868220254979917 ) ) ;
#8054=CARTESIAN_POINT ( 'NONE',  ( -19.03146662611517925, 1442.920952512881286, 211.1498405880065548 ) ) ;
#8058=EDGE_LOOP ( 'NONE', ( #12887, #52962, #53977, #47483, #10445, #27618, #62663, #66338, #34292, #49746 ) ) ;
#8063=EDGE_CURVE ( 'NONE', #80510, #92712, #69123, .T. ) ;
#8064=CARTESIAN_POINT ( 'NONE',  ( -4.398465238590000048, 1410.004223061730045, 186.8505807875980054 ) ) ;
#8066=CARTESIAN_POINT ( 'NONE',  ( 0.2707663694632699847, 1415.088012641449950, 226.0844260569690221 ) ) ;
#8068=CARTESIAN_POINT ( 'NONE',  ( 19.02456972039999883, 1426.130241254430075, 222.9765850832980050 ) ) ;
#8071=CARTESIAN_POINT ( 'NONE',  ( 7.758583985612400369, 1432.346375769730230, 153.7649721816169972 ) ) ;
#8075=CARTESIAN_POINT ( 'NONE',  ( -20.37457945109999713, 1508.379714647830042, 189.3932127643979868 ) ) ;
#8079=FACE_OUTER_BOUND ( 'NONE', #32249, .T. ) ;
#8080=CARTESIAN_POINT ( 'NONE',  ( 15.05358515569999867, 1410.831827814130065, 191.5175410460979890 ) ) ;
#8081=EDGE_CURVE ( 'NONE', #43874, #49524, #20800, .T. ) ;
#8082=CARTESIAN_POINT ( 'NONE',  ( -12.40790004000990443, 1486.029326377792813, 184.8800518666174355 ) ) ;
#8087=CARTESIAN_POINT ( 'NONE',  ( 22.71362856800000074, 1462.471423918330174, 250.3594882937979946 ) ) ;
#8090=CARTESIAN_POINT ( 'NONE',  ( -23.68010693890000340, 1447.007135453729916, 214.9276627933680004 ) ) ;
#8095=CARTESIAN_POINT ( 'NONE',  ( 3.068292148129999717E-16, 1443.913060387330006, 150.8032249175980155 ) ) ;
#8098=CARTESIAN_POINT ( 'NONE',  ( 0.1080094079350000097, 1405.775964805630110, 268.4837719563980158 ) ) ;
#8101=CARTESIAN_POINT ( 'NONE',  ( 12.97071388079999998, 1422.777285505929967, 222.8915848212980109 ) ) ;
#8102=CARTESIAN_POINT ( 'NONE',  ( 37.79051012442420188, 1445.035584067519949, 137.0421779800970228 ) ) ;
#8104=CARTESIAN_POINT ( 'NONE',  ( 25.64308588377748421, 1450.800358157930759, 136.9756054736515694 ) ) ;
#8106=CARTESIAN_POINT ( 'NONE',  ( 32.00873375412530208, 1436.944025776200078, 136.6203492527909873 ) ) ;
#8107=CARTESIAN_POINT ( 'NONE',  ( 39.81773801718750150, 1446.247923821029872, 136.7608449633160035 ) ) ;
#8108=CARTESIAN_POINT ( 'NONE',  ( -4.162004322789402799, 1449.631395384008101, 185.0510854563681846 ) ) ;
#8110=CARTESIAN_POINT ( 'NONE',  ( 8.313286323959999891, 1507.316772408030147, 183.0869040499979974 ) ) ;
#8113=FACE_OUTER_BOUND ( 'NONE', #80434, .T. ) ;
#8114=ORIENTED_EDGE ( 'NONE', *, *, #43175, .F. ) ;
#8116=CARTESIAN_POINT ( 'NONE',  ( -42.47163414147675553, 1428.396231719419120, 269.0629786396675058 ) ) ;
#8118=CARTESIAN_POINT ( 'NONE',  ( 16.80488241574720121, 1503.399646969610103, 188.2277903123039948 ) ) ;
#8119=CARTESIAN_POINT ( 'NONE',  ( 13.78830459049999924, 1507.504417904530101, 224.4506042099979766 ) ) ;
#8121=CARTESIAN_POINT ( 'NONE',  ( -12.67125179517506695, 1445.026230862206148, 185.8434676868600945 ) ) ;
#8122=B_SPLINE_SURFACE_WITH_KNOTS ( 'NONE', 5, 5, ( 
 ( #3378, #79521, #1722, #37505, #35298, #71710, #96872, #96312, #61093, #11220, #2826, #12289 ),
 ( #62186, #10661, #19590, #44829, #35862, #105828, #87931, #29106, #103605, #70046, #45383, #95758 ),
 ( #19023, #36944, #78982, #54335, #2286, #62755, #71142, #105262, #90653, #47027, #7622, #67006 ),
 ( #55973, #109546, #30751, #29648, #64932, #101661, #33365, #80615, #32819, #24950, #3929, #21216 ),
 ( #13937, #64383, #50207, #99045, #73878, #106903, #48125, #22323, #56525, #84332, #82263, #101116 ),
 ( #97947, #90097, #55424, #24413, #4999, #59159, #5563, #41780, #92729, #30190, #58597, #16004 ),
 ( #75935, #98504, #110090, #67558, #38058, #93279, #46483, #72236, #39144, #21772, #106362, #63835 ),
 ( #89557, #12846, #81153, #13380, #4467, #73319, #38596, #47568, #72775, #81692, #107456, #39714 ),
 ( #33922, #69776, #36150, #8716, #52412, #51852, #35030, #68661, #68118, #76485, #102230, #77053 ),
 ( #60252, #18216, #904, #69209, #9831, #104446, #70334, #27738, #17651, #43450, #35584, #93812 ),
 ( #103318, #59700, #110637, #61376, #25509, #17091, #42895, #103894, #61929, #16542, #34486, #51283 ),
 ( #360, #10379, #27193, #84866, #52961, #95495, #44552, #85989, #102761, #50733, #87094, #44000 ) ),
 .UNSPECIFIED., .F., .F., .F.,
 ( 6, 3, 3, 6 ),
 ( 6, 3, 3, 6 ),
 ( 5.901444351240000330, 6.549836289219999941, 7.702803945130000329, 8.339062479686310425 ),
 ( -4.054862768222389734E-05, 0.3888358943340000096, 1.166507657809999987, 1.690645290116310040 ),
 .UNSPECIFIED. ) ;
#8125=CARTESIAN_POINT ( 'NONE',  ( -10.76135780955835131, 1418.364098519981781, 229.5605810891095473 ) ) ;
#8126=CARTESIAN_POINT ( 'NONE',  ( -21.00754753991050450, 1450.948176978987703, 144.4512443326310347 ) ) ;
#8128=CARTESIAN_POINT ( 'NONE',  ( 24.46423381230000160, 1435.351789881140121, 136.2073200738979892 ) ) ;
#8129=CARTESIAN_POINT ( 'NONE',  ( -12.75960595697487676, 1442.830007631229819, 169.4538581461608828 ) ) ;
#8131=CARTESIAN_POINT ( 'NONE',  ( 0.5835301444260361237, 1415.089118586289942, 191.9293356823729937 ) ) ;
#8138=CARTESIAN_POINT ( 'NONE',  ( -15.47578423070000042, 1455.753639292730213, 211.9081975729679925 ) ) ;
#8140=CARTESIAN_POINT ( 'NONE',  ( 4.187230966989369918, 1424.086676286679904, 184.3159420495250060 ) ) ;
#8142=CARTESIAN_POINT ( 'NONE',  ( -2.495937523808232861, 1421.225737875227424, 184.7764519901441531 ) ) ;
#8144=CARTESIAN_POINT ( 'NONE',  ( -24.50758153960000030, 1438.442324728890071, 210.7299082220580146 ) ) ;
#8148=CARTESIAN_POINT ( 'NONE',  ( -17.49344942435742567, 1509.643870198284048, 184.6887002396688899 ) ) ;
#8149=CARTESIAN_POINT ( 'NONE',  ( -2.798454660896469878E-09, 1414.971556725290156, 244.5047741046470264 ) ) ;
#8151=VERTEX_POINT ( 'NONE', #45179 ) ;
#8152=CARTESIAN_POINT ( 'NONE',  ( -11.80049257314770017, 1428.258320413980073, 148.2065752701799966 ) ) ;
#8153=AXIS2_PLACEMENT_3D ( 'NONE', #37239, #72503, #71438 ) ;
#8154=CARTESIAN_POINT ( 'NONE',  ( -19.87223104929999806, 1484.291808912129909, 191.2808552885979907 ) ) ;
#8155=CARTESIAN_POINT ( 'NONE',  ( -1.412138242519999975, 1471.571752635429903, 269.6151167561980060 ) ) ;
#8156=CARTESIAN_POINT ( 'NONE',  ( 11.95405219206525516, 1433.552936807464221, 147.6143242043138173 ) ) ;
#8158=CARTESIAN_POINT ( 'NONE',  ( 17.73803434250000066, 1408.913060387329779, 209.1218459616979999 ) ) ;
#8160=CARTESIAN_POINT ( 'NONE',  ( -15.28420222229999936, 1497.713060387329961, 193.8376437396979952 ) ) ;
#8163=CARTESIAN_POINT ( 'NONE',  ( -20.58955907263800000, 1409.512823798320142, 267.0592759364189988 ) ) ;
#8166=CYLINDRICAL_SURFACE ( 'NONE', #53805, 1.638701816490922836 ) ;
#8167=CARTESIAN_POINT ( 'NONE',  ( 14.26923756360000084, 1444.927653052269989, 189.5513799252980220 ) ) ;
#8169=ORIENTED_EDGE ( 'NONE', *, *, #76712, .F. ) ;
#8170=CARTESIAN_POINT ( 'NONE',  ( 4.647253597870006026, 1422.128807924814055, 184.1025069751984802 ) ) ;
#8173=CARTESIAN_POINT ( 'NONE',  ( -15.59759639429999822, 1470.467432881730019, 188.1491572198980009 ) ) ;
#8175=VERTEX_POINT ( 'NONE', #80421 ) ;
#8180=CARTESIAN_POINT ( 'NONE',  ( -27.28719766109999867, 1508.596937417230038, 204.2391279096780181 ) ) ;
#8181=FACE_OUTER_BOUND ( 'NONE', #105706, .T. ) ;
#8183=CIRCLE ( 'NONE', #13538, 2.000000000000001776 ) ;
#8184=CARTESIAN_POINT ( 'NONE',  ( -6.448255178740000204, 1408.606950374030021, 197.2260920491980016 ) ) ;
#8187=ORIENTED_EDGE ( 'NONE', *, *, #49516, .T. ) ;
#8189=CARTESIAN_POINT ( 'NONE',  ( 27.89257148229999927, 1508.131979115830063, 211.4058184921079828 ) ) ;
#8192=CARTESIAN_POINT ( 'NONE',  ( -13.12992410348680039, 1436.052586817060046, 150.6851515388850089 ) ) ;
#8195=CARTESIAN_POINT ( 'NONE',  ( -14.45007549780000033, 1415.597377782830108, 226.9959651844980044 ) ) ;
#8198=VERTEX_POINT ( 'NONE', #96672 ) ;
#8200=CARTESIAN_POINT ( 'NONE',  ( 5.429027314403359838, 1440.820888945739853, 154.8047238334139877 ) ) ;
#8201=CARTESIAN_POINT ( 'NONE',  ( -20.52956604201131086, 1455.629392789516260, 224.1961909860604862 ) ) ;
#8205=CARTESIAN_POINT ( 'NONE',  ( 12.82193894433369863, 1434.943467189540115, 150.1840956961830216 ) ) ;
#8206=B_SPLINE_CURVE_WITH_KNOTS ( 'NONE', 5,
 ( #95820, #63895, #1791, #28620, #2894, #19088, #37012, #35928, #2349, #44898, #87431, #70112 ),
 .UNSPECIFIED., .F., .F.,
 ( 6, 3, 3, 6 ),
 ( 5.812629425579999953, 6.561021380799999747, 7.569428689259999565, 8.073601757938709156 ),
 .UNSPECIFIED. ) ;
#8207=CARTESIAN_POINT ( 'NONE',  ( 2.706310507869800208, 1459.298787099630090, 233.8407132922810092 ) ) ;
#8209=CARTESIAN_POINT ( 'NONE',  ( -11.43336139241818827, 1425.764428307910975, 138.9802830098579420 ) ) ;
#8212=CARTESIAN_POINT ( 'NONE',  ( -15.09681984919999920, 1409.610690840030202, 226.1751760239980058 ) ) ;
#8216=CARTESIAN_POINT ( 'NONE',  ( 20.99960916279999878, 1509.542875961329855, 188.7432993302979867 ) ) ;
#8218=ORIENTED_EDGE ( 'NONE', *, *, #73439, .F. ) ;
#8228=CARTESIAN_POINT ( 'NONE',  ( 17.36968966387737723, 1422.689908039817965, 226.5801647642350076 ) ) ;
#8232=CARTESIAN_POINT ( 'NONE',  ( 41.06518263065470364, 1440.913060356710048, 260.7453200965900351 ) ) ;
#8234=CARTESIAN_POINT ( 'NONE',  ( 8.313287170068500487, 1507.316777277299934, 183.0869016502879845 ) ) ;
#8235=CARTESIAN_POINT ( 'NONE',  ( 10.95929498157123483, 1431.610953951363172, 151.7698544105677456 ) ) ;
#8239=CARTESIAN_POINT ( 'NONE',  ( -8.972797484658892486, 1506.569407359554816, 229.3146644943394676 ) ) ;
#8241=CARTESIAN_POINT ( 'NONE',  ( 3.931910744533549718, 1448.296755838050103, 184.2998928686550073 ) ) ;
#8242=CARTESIAN_POINT ( 'NONE',  ( -3.059934833509219576, 1425.992208071485948, 185.5324912608258785 ) ) ;
#8245=TOROIDAL_SURFACE ( 'NONE', #74469, 8.500000000000000000, 1.500000000000000000 ) ;
#8249=ADVANCED_FACE ( 'NONE', ( #54138 ), #28355, .F. ) ;
#8250=CARTESIAN_POINT ( 'NONE',  ( 10.34308214130000003, 1452.551872000029789, 150.8401898677979887 ) ) ;
#8251=CARTESIAN_POINT ( 'NONE',  ( 3.500000000000000000, 1424.163060387329779, 172.2701767054979882 ) ) ;
#8254=ORIENTED_EDGE ( 'NONE', *, *, #46258, .T. ) ;
#8257=EDGE_CURVE ( 'NONE', #21200, #75280, #7356, .T. ) ;
#8258=CARTESIAN_POINT ( 'NONE',  ( -21.13431252044160047, 1409.651086843229905, 211.8287216663260040 ) ) ;
#8259=ORIENTED_EDGE ( 'NONE', *, *, #22699, .T. ) ;
#8262=CARTESIAN_POINT ( 'NONE',  ( 20.59988588776639773, 1509.677360688819817, 230.5839048903779940 ) ) ;
#8264=CARTESIAN_POINT ( 'NONE',  ( 37.37547333107730196, 1438.147115316229929, 136.5735404978140082 ) ) ;
#8272=CARTESIAN_POINT ( 'NONE',  ( 4.526435456679999803, 1410.447042416829845, 186.2069608473979940 ) ) ;
#8273=CARTESIAN_POINT ( 'NONE',  ( 4.853127557110000545, 1425.657129708029970, 185.6214293445979990 ) ) ;
#8275=CARTESIAN_POINT ( 'NONE',  ( -2.499999942568179812, 1440.188496425770154, 170.5318011134379788 ) ) ;
#8276=B_SPLINE_CURVE_WITH_KNOTS ( 'NONE', 5,
 ( #54352, #3946, #87947, #2304, #18492, #89017, #45937, #11768, #12309, #80075, #63308, #70607 ),
 .UNSPECIFIED., .F., .F.,
 ( 6, 3, 3, 6 ),
 ( 0.000000000000000000, 0.2928450906018923439, 0.7539279110859780086, 1.000000000000000000 ),
 .UNSPECIFIED. ) ;
#8277=B_SPLINE_CURVE_WITH_KNOTS ( 'NONE', 3,
 ( #81039, #89445, #74321, #106245 ),
 .UNSPECIFIED., .F., .F.,
 ( 4, 4 ),
 ( 0.000000000000000000, 1.000000000000000000 ),
 .UNSPECIFIED. ) ;
#8278=CARTESIAN_POINT ( 'NONE',  ( -22.03365245649999693, 1451.714665305230028, 143.0874833212980093 ) ) ;
#8279=CARTESIAN_POINT ( 'NONE',  ( 1.790406358549999855, 1464.873382007230020, 236.3711796330979666 ) ) ;
#8280=ORIENTED_EDGE ( 'NONE', *, *, #46216, .T. ) ;
#8284=CARTESIAN_POINT ( 'NONE',  ( -12.26979726809049964, 1416.828039266780024, 194.6643405733680083 ) ) ;
#8285=CARTESIAN_POINT ( 'NONE',  ( -2.499999999859999988, 1439.640830480200293, 184.0873493999980042 ) ) ;
#8286=CARTESIAN_POINT ( 'NONE',  ( 17.02674992690000266, 1488.215563971529946, 189.0842524208980251 ) ) ;
#8287=CARTESIAN_POINT ( 'NONE',  ( -3.721063415729999695E-09, 1475.837061091930082, 266.9611530633980010 ) ) ;
#8288=CARTESIAN_POINT ( 'NONE',  ( 20.04791373445998204, 1436.429743172953977, 145.3885934355014342 ) ) ;
#8289=CARTESIAN_POINT ( 'NONE',  ( -0.5624690339869999889, 1416.828040475229955, 227.7677324846980014 ) ) ;
#8290=CARTESIAN_POINT ( 'NONE',  ( -8.733798672629999871, 1419.056601762730224, 233.0476203166980156 ) ) ;
#8293=EDGE_CURVE ( 'NONE', #94676, #44473, #27383, .T. ) ;
#8296=CARTESIAN_POINT ( 'NONE',  ( -45.61713505807430380, 1439.852003152469933, 268.9753901037370269 ) ) ;
#8300=ORIENTED_EDGE ( 'NONE', *, *, #20547, .T. ) ;
#8306=CARTESIAN_POINT ( 'NONE',  ( -26.01456120673969963, 1451.843691735240100, 135.7887858332240114 ) ) ;
#8308=CARTESIAN_POINT ( 'NONE',  ( 26.01030838259999811, 1431.980453045119930, 231.9333039360980138 ) ) ;
#8313=CARTESIAN_POINT ( 'NONE',  ( -19.36515920207871488, 1456.378690097197477, 228.5344338426573358 ) ) ;
#8315=CARTESIAN_POINT ( 'NONE',  ( -17.99954540876850118, 1410.904693920620048, 195.2564682659330231 ) ) ;
#8316=CARTESIAN_POINT ( 'NONE',  ( -25.37229503420000043, 1438.463288316339913, 138.1377907575980259 ) ) ;
#8318=CARTESIAN_POINT ( 'NONE',  ( -1.236138560472719972, 1408.568929830810248, 270.4289767352809690 ) ) ;
#8319=CARTESIAN_POINT ( 'NONE',  ( 7.805697987095799206, 1418.513168923040212, 231.5901604170679775 ) ) ;
#8321=VERTEX_POINT ( 'NONE', #10749 ) ;
#8323=CARTESIAN_POINT ( 'NONE',  ( -22.72614924474259723, 1409.716713977369864, 209.6046740144809917 ) ) ;
#8324=CARTESIAN_POINT ( 'NONE',  ( -0.8389850993970380255, 1409.109437246339894, 185.8522822715279972 ) ) ;
#8326=CARTESIAN_POINT ( 'NONE',  ( -6.629188914260000232, 1428.588785140030041, 91.31218443469779800 ) ) ;
#8327=CARTESIAN_POINT ( 'NONE',  ( -20.54885787271648567, 1436.446738464058399, 144.8383282339893299 ) ) ;
#8329=CARTESIAN_POINT ( 'NONE',  ( 41.27561781798189600, 1456.929397665800025, 267.7644989067840129 ) ) ;
#8331=CARTESIAN_POINT ( 'NONE',  ( -16.55054877997067209, 1421.400737720431835, 226.9740673232442134 ) ) ;
#8334=CARTESIAN_POINT ( 'NONE',  ( 18.33221555414402459, 1459.112549484824740, 227.7897102868277557 ) ) ;
#8336=CARTESIAN_POINT ( 'NONE',  ( 23.17738928069999815, 1409.983622293829967, 208.1777596987790275 ) ) ;
#8337=ORIENTED_EDGE ( 'NONE', *, *, #99685, .T. ) ;
#8343=CARTESIAN_POINT ( 'NONE',  ( 20.79403292647610257, 1409.639204018000100, 215.4572002851739967 ) ) ;
#8345=CARTESIAN_POINT ( 'NONE',  ( 2.164129514809030042, 1408.988633455270246, 186.9734320209399812 ) ) ;
#8346=CARTESIAN_POINT ( 'NONE',  ( 2.223260522209999923, 1417.626103841329723, 234.7006573303980019 ) ) ;
#8347=DIRECTION ( 'NONE',  ( -0.9445946449598763284, 0.000000000000000000, 0.3282391760791590340 ) ) ;
#8348=CARTESIAN_POINT ( 'NONE',  ( 1.039304647762639977, 1450.826060414650101, 181.7808938767670099 ) ) ;
#8351=EDGE_CURVE ( 'NONE', #46444, #104691, #110244, .T. ) ;
#8359=CARTESIAN_POINT ( 'NONE',  ( -34.14991619301339654, 1450.428381852520033, 136.2391939585110094 ) ) ;
#8361=B_SPLINE_CURVE_WITH_KNOTS ( 'NONE', 3,
 ( #54868, #19582, #54327, #104147, #80605, #3920, #61083, #95198, #53785, #95748, #19012, #87354, #78972, #2276, #36390, #87922, #79512, #2816, #36935, #39129 ),
 .UNSPECIFIED., .F., .F.,
 ( 4, 2, 1, 2, 2, 1, 1, 1, 1, 1, 2, 2, 4 ),
 ( 0.000000000000000000, 0.2500000000000632827, 0.3750000000000898170, 0.4375000000000980882, 0.5000000000001063594, 0.6250000000001328937, 0.6875000000001459943, 0.7187500000001525446, 0.7343750000001615375, 0.7421875000001608713, 0.7460937500001610934, 0.7500000000001613154, 1.000000000000000000 ),
 .UNSPECIFIED. ) ;
#8362=CARTESIAN_POINT ( 'NONE',  ( -0.8182520991989999937, 1433.447543843880112, 150.4377610267980003 ) ) ;
#8364=CARTESIAN_POINT ( 'NONE',  ( -21.22517433705326084, 1508.705765839073138, 191.9978281503293829 ) ) ;
#8365=CARTESIAN_POINT ( 'NONE',  ( 11.89989176039999919, 1433.416276115000073, 150.2672394752979983 ) ) ;
#8366=CARTESIAN_POINT ( 'NONE',  ( 27.19819524420000079, 1447.435760031770087, 248.0989693098979956 ) ) ;
#8367=CARTESIAN_POINT ( 'NONE',  ( 11.91079909304919937, 1414.913060387399810, 198.1107945471090090 ) ) ;
#8368=CARTESIAN_POINT ( 'NONE',  ( 0.5061640001184035675, 1467.094681707714244, 235.5773264646662710 ) ) ;
#8371=CARTESIAN_POINT ( 'NONE',  ( 12.81185530964379815, 1416.835419214280137, 221.9980326694370092 ) ) ;
#8372=CARTESIAN_POINT ( 'NONE',  ( 12.61713793920759663, 1398.287094680502605, 205.9900219852154351 ) ) ;
#8373=CARTESIAN_POINT ( 'NONE',  ( -15.22206364535530021, 1509.523931070260005, 236.6035046314040073 ) ) ;
#8385=CARTESIAN_POINT ( 'NONE',  ( 0.1798334447694739935, 1474.584573357990166, 182.3269854996729862 ) ) ;
#8386=CARTESIAN_POINT ( 'NONE',  ( -6.033397232889999628, 1408.942087272730078, 222.3801906342980033 ) ) ;
#8387=VERTEX_POINT ( 'NONE', #32581 ) ;
#8388=CARTESIAN_POINT ( 'NONE',  ( -25.25200574389469921, 1450.804213008409988, 137.6134964715130025 ) ) ;
#8390=CARTESIAN_POINT ( 'NONE',  ( 12.40397477760000022, 1434.420140970890088, 149.9806263996979965 ) ) ;
#8391=CARTESIAN_POINT ( 'NONE',  ( -41.66188030070010484, 1443.907795131759940, 134.0999999982419979 ) ) ;
#8392=DIRECTION ( 'NONE',  ( 0.7071068048245321425, 1.133496607279266283E-10, 0.7071067575485621148 ) ) ;
#8396=CARTESIAN_POINT ( 'NONE',  ( -17.29183738970000306, 1416.216252248629871, 214.4361153381880172 ) ) ;
#8399=DIRECTION ( 'NONE',  ( -0.9995237709234272572, -0.03085824620765321644, -1.897025751615122517E-13 ) ) ;
#8401=CARTESIAN_POINT ( 'NONE',  ( -5.360152366205530150, 1422.242722016050038, 144.1549655170190078 ) ) ;
#8407=CARTESIAN_POINT ( 'NONE',  ( -32.07183470040000373, 1450.932248063129919, 136.2258049830979871 ) ) ;
#8408=EDGE_CURVE ( 'NONE', #105450, #40901, #103533, .T. ) ;
#8416=CARTESIAN_POINT ( 'NONE',  ( -4.283857371189049523, 1440.956241081810049, 155.9231041381889895 ) ) ;
#8418=CARTESIAN_POINT ( 'NONE',  ( 13.94796568798376946, 1429.572418609742044, 221.4045584918379745 ) ) ;
#8419=CARTESIAN_POINT ( 'NONE',  ( 2.040662746359999780, 1417.628369438229811, 233.4326516709979842 ) ) ;
#8426=CIRCLE ( 'NONE', #94280, 95.87906523465393605 ) ;
#8427=CARTESIAN_POINT ( 'NONE',  ( 4.271711532569999470, 1446.704874179759827, 157.7711585643980072 ) ) ;
#8428=ADVANCED_FACE ( 'NONE', ( #41639 ), #93696, .F. ) ;
#8436=CARTESIAN_POINT ( 'NONE',  ( -24.07566136870000051, 1410.921070259630142, 208.6092334039690002 ) ) ;
#8437=CARTESIAN_POINT ( 'NONE',  ( -11.04544962402649944, 1426.046997354040059, 102.3020123086109976 ) ) ;
#8438=CARTESIAN_POINT ( 'NONE',  ( 16.05360826451080314, 1409.473653766179950, 193.0727167379100138 ) ) ;
#8444=CARTESIAN_POINT ( 'NONE',  ( 15.05249117875021270, 1461.926097438958323, 229.9722081114364869 ) ) ;
#8447=CARTESIAN_POINT ( 'NONE',  ( -34.12598879534539975, 1437.021307524110171, 136.5549898716600126 ) ) ;
#8448=ORIENTED_EDGE ( 'NONE', *, *, #11845, .T. ) ;
#8449=CARTESIAN_POINT ( 'NONE',  ( 10.77727084197429974, 1397.924324489370292, 200.3403619048980033 ) ) ;
#8451=CARTESIAN_POINT ( 'NONE',  ( -17.62109803770000127, 1460.304421794930022, 228.2025014059980208 ) ) ;
#8452=ORIENTED_EDGE ( 'NONE', *, *, #2233, .T. ) ;
#8453=EDGE_LOOP ( 'NONE', ( #28388, #56774, #780, #72782 ) ) ;
#8454=AXIS2_PLACEMENT_3D ( 'NONE', #15785, #75743, #67357 ) ;
#8461=LINE ( 'NONE', #76786, #30052 ) ;
#8463=DIRECTION ( 'NONE',  ( -0.9995237709234254808, 0.03085824620771311644, -1.986951185180850780E-13 ) ) ;
#8465=CARTESIAN_POINT ( 'NONE',  ( -2.370970874524632510, 1427.002265528473799, 137.0999999980979851 ) ) ;
#8467=ORIENTED_EDGE ( 'NONE', *, *, #53596, .F. ) ;
#8471=CARTESIAN_POINT ( 'NONE',  ( 11.74578019742499890, 1426.720260049070021, 144.7832389959820034 ) ) ;
#8472=CARTESIAN_POINT ( 'NONE',  ( 19.97280420420000269, 1487.549460532730109, 227.0589497365980094 ) ) ;
#8474=CARTESIAN_POINT ( 'NONE',  ( -13.68684928409999912, 1415.245980412430072, 220.9574426735980239 ) ) ;
#8475=CARTESIAN_POINT ( 'NONE',  ( -11.62445858788020026, 1432.338721124250014, 150.9950008028209822 ) ) ;
#8478=CARTESIAN_POINT ( 'NONE',  ( -4.599789036639999829, 1421.972502547630029, 185.2173717891980118 ) ) ;
#8481=CARTESIAN_POINT ( 'NONE',  ( 0.06584449245319999588, 1508.965707083629923, 179.3766826265980114 ) ) ;
#8482=CARTESIAN_POINT ( 'NONE',  ( -12.82501412541063601, 1410.734581749099561, 189.5959794609471487 ) ) ;
#8484=CARTESIAN_POINT ( 'NONE',  ( 23.61616453110579883, 1435.156076846089945, 206.2084620324950208 ) ) ;
#8487=CARTESIAN_POINT ( 'NONE',  ( -4.703918259281699044, 1423.649054296706709, 184.4972853060825173 ) ) ;
#8489=CARTESIAN_POINT ( 'NONE',  ( -5.360124858665960446, 1422.242564188120014, 144.1629134808320032 ) ) ;
#8490=ORIENTED_EDGE ( 'NONE', *, *, #93521, .T. ) ;
#8492=B_SPLINE_CURVE_WITH_KNOTS ( 'NONE', 3,
 ( #81251, #40355, #100272, #57192, #5670, #98608, #90759 ),
 .UNSPECIFIED., .F., .F.,
 ( 4, 3, 4 ),
 ( -157.7108139880000124, -101.4631914111549946, -30.86246212799579780 ),
 .UNSPECIFIED. ) ;
#8494=CARTESIAN_POINT ( 'NONE',  ( -2.907988962752879658, 1484.679952288234063, 183.2543140236687407 ) ) ;
#8495=( BOUNDED_CURVE ( )  B_SPLINE_CURVE ( 3, ( #62713, #96832, #97361, #106854 ),
 .UNSPECIFIED., .F., .F. ) 
 B_SPLINE_CURVE_WITH_KNOTS ( ( 4, 4 ),
 ( 1.268017777846622174, 1.928411132994934940 ),
 .UNSPECIFIED. ) 
 CURVE ( )  GEOMETRIC_REPRESENTATION_ITEM ( )  RATIONAL_B_SPLINE_CURVE ( ( 1.000000000000000000, 0.9639857288230757604, 0.9639857288230757604, 1.000000000000000000 ) ) 
 REPRESENTATION_ITEM ( '' )  );
#8499=CARTESIAN_POINT ( 'NONE',  ( 1.341949918430000110, 1416.837177098230086, 190.1629998231980210 ) ) ;
#8502=CARTESIAN_POINT ( 'NONE',  ( -10.93042732790000038, 1429.541181187929851, 151.2220225859979905 ) ) ;
#8503=CARTESIAN_POINT ( 'NONE',  ( -14.78895068404719915, 1427.485687361509918, 221.7293924355389834 ) ) ;
#8505=CARTESIAN_POINT ( 'NONE',  ( 11.22085813615770000, 1414.913060387329779, 197.6243702374680140 ) ) ;
#8508=CARTESIAN_POINT ( 'NONE',  ( -21.39747632310000114, 1482.727152785329963, 225.0468285881979966 ) ) ;
#8514=CARTESIAN_POINT ( 'NONE',  ( 31.26225106439999735, 1415.948784915929991, 269.3319312554980343 ) ) ;
#8515=CARTESIAN_POINT ( 'NONE',  ( 2.463295206089754608, 1464.794365557463379, 237.1801197134051336 ) ) ;
#8516=CARTESIAN_POINT ( 'NONE',  ( 22.48977040930000015, 1469.151985490530251, 196.6582214529979922 ) ) ;
#8517=CARTESIAN_POINT ( 'NONE',  ( -0.4212817365179999940, 1508.863410648129957, 238.3519434705980018 ) ) ;
#8519=CARTESIAN_POINT ( 'NONE',  ( -41.35142502486309724, 1442.058002965339938, 136.3890446465489958 ) ) ;
#8520=B_SPLINE_CURVE_WITH_KNOTS ( 'NONE', 3,
 ( #107887, #83243, #65915, #56957, #13259, #13809, #100033, #7088, #89986, #92193 ),
 .UNSPECIFIED., .F., .F.,
 ( 4, 2, 2, 2, 4 ),
 ( 0.000000000000000000, 0.2500000000000000000, 0.5000000000000000000, 0.7500000000000000000, 1.000000000000000000 ),
 .UNSPECIFIED. ) ;
#8521=CARTESIAN_POINT ( 'NONE',  ( 13.57704973455800079, 1430.332977960800008, 195.9178655745220112 ) ) ;
#8523=CARTESIAN_POINT ( 'NONE',  ( -14.34037905889999998, 1443.120642612440179, 188.8125533694979765 ) ) ;
#8527=CARTESIAN_POINT ( 'NONE',  ( 3.565775598909999733, 1407.753784349630223, 270.1349117941979898 ) ) ;
#8530=CARTESIAN_POINT ( 'NONE',  ( 1.453919372226760043, 1501.892033211519902, 181.3410715267950195 ) ) ;
#8531=CARTESIAN_POINT ( 'NONE',  ( -13.68648241757620099, 1409.391002885000034, 215.1022502297769847 ) ) ;
#8532=B_SPLINE_CURVE_WITH_KNOTS ( 'NONE', 5,
 ( #49054, #7578, #98878, #31122, #99415, #41187 ),
 .UNSPECIFIED., .F., .F.,
 ( 6, 6 ),
 ( 0.000000000000000000, 1.000000000000000000 ),
 .UNSPECIFIED. ) ;
#8536=CARTESIAN_POINT ( 'NONE',  ( -23.70279561169999738, 1471.127482098729843, 267.2984211408980286 ) ) ;
#8541=B_SPLINE_SURFACE_WITH_KNOTS ( 'NONE', 5, 5, ( 
 ( #44765, #78348, #96251, #103535, #53731, #29051 ),
 ( #9480, #1657, #87869, #11159, #35234, #62688 ),
 ( #3323, #37448, #71647, #82190, #21158, #100102 ),
 ( #12233, #22814, #73818, #4406, #64321, #55364 ),
 ( #63768, #81089, #38534, #107947, #22257, #65422 ),
 ( #37998, #89497, #80555, #30689, #46968, #72181 ) ),
 .UNSPECIFIED., .F., .F., .F.,
 ( 6, 6 ),
 ( 6, 6 ),
 ( 82.60151368457970023, 128.3333305958969959 ),
 ( -0.002296749680308819968, 2.002296750983780349 ),
 .UNSPECIFIED. ) ;
#8542=CARTESIAN_POINT ( 'NONE',  ( 19.02839246307539511, 1456.959193721570273, 225.8332742494027912 ) ) ;
#8544=CARTESIAN_POINT ( 'NONE',  ( -9.624350592200000776, 1441.605633920840091, 153.1179271311979733 ) ) ;
#8545=EDGE_CURVE ( 'NONE', #65361, #21837, #90235, .T. ) ;
#8548=DIRECTION ( 'NONE',  ( 1.442302170131585847E-09, -0.8818471531508758066, 0.4715353629153342663 ) ) ;
#8549=AXIS2_PLACEMENT_3D ( 'NONE', #58188, #25104, #75550 ) ;
#8550=CARTESIAN_POINT ( 'NONE',  ( -23.05373657170000001, 1411.078320233030126, 204.9169236815779982 ) ) ;
#8554=CARTESIAN_POINT ( 'NONE',  ( 2.455820327400000114, 1434.541746329560056, 150.3615916412979914 ) ) ;
#8558=CARTESIAN_POINT ( 'NONE',  ( -21.81077096749999811, 1409.674709292730086, 210.2046642649879971 ) ) ;
#8560=CARTESIAN_POINT ( 'NONE',  ( 11.71130021051819980, 1426.712571118619962, 142.3277864718619696 ) ) ;
#8567=CARTESIAN_POINT ( 'NONE',  ( -8.010882276929157442, 1398.150985990356958, 219.3602984231706330 ) ) ;
#8575=ORIENTED_EDGE ( 'NONE', *, *, #97509, .F. ) ;
#8576=CARTESIAN_POINT ( 'NONE',  ( 11.25278939239490050, 1434.345226179090105, 151.5801780830220196 ) ) ;
#8578=ORIENTED_EDGE ( 'NONE', *, *, #72151, .T. ) ;
#8579=CARTESIAN_POINT ( 'NONE',  ( -0.0002530612592032526744, 1396.486685308509095, 221.5233369264674650 ) ) ;
#8580=CARTESIAN_POINT ( 'NONE',  ( -22.37835337210000120, 1507.839481092230017, 193.8708192753979915 ) ) ;
#8583=CARTESIAN_POINT ( 'NONE',  ( 6.861707994109999653, 1428.078401598830169, 112.4493539157979995 ) ) ;
#8585=CARTESIAN_POINT ( 'NONE',  ( 18.22709068499189655, 1488.412411835820194, 229.3642029072559865 ) ) ;
#8586=CARTESIAN_POINT ( 'NONE',  ( 9.594803834039998591, 1488.165126248830120, 184.4998152664979898 ) ) ;
#8589=CARTESIAN_POINT ( 'NONE',  ( -12.78776258895079998, 1416.851343896850040, 195.5391574246120001 ) ) ;
#8590=CARTESIAN_POINT ( 'NONE',  ( 13.69065454780360014, 1415.152886232609944, 197.6322036034630116 ) ) ;
#8591=CARTESIAN_POINT ( 'NONE',  ( 11.56811281929999957, 1431.694744716809964, 151.1673513621979907 ) ) ;
#8594=CARTESIAN_POINT ( 'NONE',  ( 13.64099228464760039, 1434.977781978229814, 148.9109081837199824 ) ) ;
#8595=ORIENTED_EDGE ( 'NONE', *, *, #26521, .T. ) ;
#8597=CARTESIAN_POINT ( 'NONE',  ( 13.41809782280081897, 1444.381396344529094, 169.3665683494473910 ) ) ;
#8598=CARTESIAN_POINT ( 'NONE',  ( -5.041740361659999614, 1464.446899236929994, 235.7978687534979940 ) ) ;
#8601=CARTESIAN_POINT ( 'NONE',  ( -2.500000000000000000, 1448.210448412289907, 170.5244215879980061 ) ) ;
#8602=CARTESIAN_POINT ( 'NONE',  ( -18.94224506989981904, 1443.728200593167458, 212.0298136739947665 ) ) ;
#8603=CARTESIAN_POINT ( 'NONE',  ( 2.500000000000000000, 1448.251495160190188, 165.7055370936290046 ) ) ;
#8604=CARTESIAN_POINT ( 'NONE',  ( -20.15452302159999931, 1507.845791376729949, 228.9024215066979764 ) ) ;
#8606=ORIENTED_EDGE ( 'NONE', *, *, #65486, .T. ) ;
#8607=CARTESIAN_POINT ( 'NONE',  ( 22.31762535187430174, 1440.913060387330006, 228.8232858593530068 ) ) ;
#8608=CARTESIAN_POINT ( 'NONE',  ( -19.26331490529999968, 1508.281539162429908, 229.6732352803980177 ) ) ;
#8609=CARTESIAN_POINT ( 'NONE',  ( -11.55154600989999913, 1410.249881412029936, 189.0607701063979960 ) ) ;
#8613=CARTESIAN_POINT ( 'NONE',  ( 18.42577565999999933, 1424.509266043230127, 223.4215470970979993 ) ) ;
#8617=CARTESIAN_POINT ( 'NONE',  ( 0.001396730326707920156, 1465.018684410219976, 237.3906889929259876 ) ) ;
#8619=AXIS2_PLACEMENT_3D ( 'NONE', #46454, #38031, #29617 ) ;
#8623=CARTESIAN_POINT ( 'NONE',  ( 22.70509004431190192, 1409.705939603270053, 209.2982552845940063 ) ) ;
#8624=VECTOR ( 'NONE', #15767, 1000.000000000000000 ) ;
#8632=CARTESIAN_POINT ( 'NONE',  ( 5.442004255449999661, 1468.737548876029905, 250.5651368528980072 ) ) ;
#8633=CARTESIAN_POINT ( 'NONE',  ( 3.347294972025637527, 1451.126043403471158, 184.0057138541948802 ) ) ;
#8634=CARTESIAN_POINT ( 'NONE',  ( -28.85571497835669774, 1509.920724158590019, 214.5067048101039973 ) ) ;
#8636=CARTESIAN_POINT ( 'NONE',  ( -2.709137183217330325, 1508.767349011980059, 237.8404265817369776 ) ) ;
#8640=CARTESIAN_POINT ( 'NONE',  ( 17.73893480064900174, 1410.031254009529903, 222.7710511100789859 ) ) ;
#8646=CARTESIAN_POINT ( 'NONE',  ( 0.1078348715190000084, 1405.842710276629987, 267.2349610867980232 ) ) ;
#8647=CARTESIAN_POINT ( 'NONE',  ( 29.06854786870000140, 1509.928156446929961, 206.2948012444579717 ) ) ;
#8648=CARTESIAN_POINT ( 'NONE',  ( 12.78755496059999786, 1416.844618646730169, 222.9177554085979978 ) ) ;
#8649=CARTESIAN_POINT ( 'NONE',  ( -6.220539724137306159, 1424.583771648741731, 186.6152494251206235 ) ) ;
#8652=CARTESIAN_POINT ( 'NONE',  ( 33.29225716172200578, 1435.659897776519983, 135.5215965639700073 ) ) ;
#8653=DIRECTION ( 'NONE',  ( 0.000000000000000000, 1.000000000000000000, 0.000000000000000000 ) ) ;
#8656=CARTESIAN_POINT ( 'NONE',  ( 8.326538737159999926, 1507.918727144829973, 183.0016939534980338 ) ) ;
#8662=CARTESIAN_POINT ( 'NONE',  ( 11.87980743189999977, 1433.311001100440080, 146.5967650327979754 ) ) ;
#8664=CARTESIAN_POINT ( 'NONE',  ( 15.03006911687520031, 1447.439797465169931, 189.9780440897100107 ) ) ;
#8665=LINE ( 'NONE', #8119, #44685 ) ;
#8668=CARTESIAN_POINT ( 'NONE',  ( -29.74048408400000199, 1509.991911973829929, 210.0353904563160086 ) ) ;
#8671=CARTESIAN_POINT ( 'NONE',  ( -11.48552941940051220, 1418.748566887944889, 229.1496130817171775 ) ) ;
#8672=CARTESIAN_POINT ( 'NONE',  ( 17.99954443082109989, 1410.904693892220166, 222.9872220945560173 ) ) ;
#8675=CARTESIAN_POINT ( 'NONE',  ( 24.07357629730000070, 1435.356839239090050, 136.9693785357980005 ) ) ;
#8676=CARTESIAN_POINT ( 'NONE',  ( -10.83121030459200007, 1396.291294585879996, 206.8277440348720120 ) ) ;
#8677=ORIENTED_EDGE ( 'NONE', *, *, #91091, .T. ) ;
#8679=CARTESIAN_POINT ( 'NONE',  ( 21.77056714271089177, 1509.419234230875190, 226.6994063304933036 ) ) ;
#8684=DIRECTION ( 'NONE',  ( 0.000000000000000000, 0.000000000000000000, -1.000000000000000000 ) ) ;
#8685=CARTESIAN_POINT ( 'NONE',  ( 11.12372166200000123, 1426.894033309730048, 99.60654041669779701 ) ) ;
#8686=CARTESIAN_POINT ( 'NONE',  ( 4.363122647530000009, 1432.413060387330006, 146.1721969590979882 ) ) ;
#8687=CARTESIAN_POINT ( 'NONE',  ( 23.57985488250000117, 1410.231772307329948, 210.8506199998580257 ) ) ;
#8688=CARTESIAN_POINT ( 'NONE',  ( -11.87499642090000052, 1433.007151748719934, 150.0792799791980201 ) ) ;
#8690=CARTESIAN_POINT ( 'NONE',  ( -2.496155285332042784, 1421.191123497494345, 184.8720394902521207 ) ) ;
#8691=CIRCLE ( 'NONE', #85580, 1.999999999999973577 ) ;
#8695=CARTESIAN_POINT ( 'NONE',  ( 3.236908035719999965, 1449.131113800429830, 183.9272198847980064 ) ) ;
#8705=CARTESIAN_POINT ( 'NONE',  ( -0.4790278571090000326, 1472.619496933330083, 270.3713665238979615 ) ) ;
#8709=CARTESIAN_POINT ( 'NONE',  ( 15.55054316549999882, 1408.913060387329779, 199.4537366391079729 ) ) ;
#8711=CARTESIAN_POINT ( 'NONE',  ( 22.65427326300000033, 1411.066072244829911, 206.6969470652379925 ) ) ;
#8712=CARTESIAN_POINT ( 'NONE',  ( -22.81156273906369947, 1507.439214557219884, 208.2956905222379760 ) ) ;
#8714=CARTESIAN_POINT ( 'NONE',  ( 6.465563136336550443, 1408.607608635380075, 196.5438154157149881 ) ) ;
#8715=CARTESIAN_POINT ( 'NONE',  ( -18.72589922193079914, 1409.005224371739814, 266.8215888940370064 ) ) ;
#8716=CARTESIAN_POINT ( 'NONE',  ( -13.80919631936640002, 1435.007083571719932, 148.9152799103790130 ) ) ;
#8717=VERTEX_POINT ( 'NONE', #109268 ) ;
#8718=DIRECTION ( 'NONE',  ( 0.000000000000000000, 0.000000000000000000, 1.000000000000000000 ) ) ;
#8719=CARTESIAN_POINT ( 'NONE',  ( 13.41370794949999912, 1444.653901271769882, 188.3548391028979836 ) ) ;
#8722=CARTESIAN_POINT ( 'NONE',  ( 4.695345900855497412, 1422.169280887841296, 184.1494170363840510 ) ) ;
#8726=CARTESIAN_POINT ( 'NONE',  ( -17.41752696329999850, 1470.470948016929924, 189.2590027405980209 ) ) ;
#8727=CARTESIAN_POINT ( 'NONE',  ( -16.26545371259889805, 1479.765189095689948, 229.1142011118929815 ) ) ;
#8728=ORIENTED_EDGE ( 'NONE', *, *, #95396, .F. ) ;
#8730=CARTESIAN_POINT ( 'NONE',  ( -3.899071993169999590E-16, 1420.943991414029824, 172.2701767054979882 ) ) ;
#8732=CARTESIAN_POINT ( 'NONE',  ( -27.69670323179999727, 1508.056852025029912, 205.9292566894080210 ) ) ;
#8733=CARTESIAN_POINT ( 'NONE',  ( -0.7321517276410000052, 1477.822672531229955, 230.6006906680979966 ) ) ;
#8735=CARTESIAN_POINT ( 'NONE',  ( -2.867472949620000211, 1409.013194749230024, 194.6181666647979966 ) ) ;
#8736=CARTESIAN_POINT ( 'NONE',  ( -28.25086642335310216, 1508.135711581739997, 208.8579954535609886 ) ) ;
#8737=DIRECTION ( 'NONE',  ( 0.3363363969981701951, -0.9417419115948324482, 0.000000000000000000 ) ) ;
#8739=CARTESIAN_POINT ( 'NONE',  ( -27.33099940864819999, 1488.742651603209879, 209.9611524475739941 ) ) ;
#8740=CARTESIAN_POINT ( 'NONE',  ( 23.31685688550000179, 1508.124115173030077, 223.0011395122980105 ) ) ;
#8742=CARTESIAN_POINT ( 'NONE',  ( 19.02702702808590018, 1456.914964676220052, 225.6710515766719993 ) ) ;
#8747=CARTESIAN_POINT ( 'NONE',  ( -15.03087568459999979, 1418.003645312529898, 226.9475657730980060 ) ) ;
#8751=CARTESIAN_POINT ( 'NONE',  ( -36.37832876729999754, 1435.767865857450261, 134.0999984849980251 ) ) ;
#8752=CARTESIAN_POINT ( 'NONE',  ( -11.50267440360000037, 1412.829103654730034, 228.8848828364980079 ) ) ;
#8759=CARTESIAN_POINT ( 'NONE',  ( 12.65519453621029911, 1434.571286974429995, 149.4915664245209825 ) ) ;
#8761=CARTESIAN_POINT ( 'NONE',  ( 6.041208603222500528, 1459.296510909109884, 233.3208609013059913 ) ) ;
#8762=CARTESIAN_POINT ( 'NONE',  ( -23.63758762339999819, 1509.747673043829991, 226.8389689203980026 ) ) ;
#8768=CARTESIAN_POINT ( 'NONE',  ( 19.94909480960000181, 1508.591193236829895, 188.8781692952979938 ) ) ;
#8770=VERTEX_POINT ( 'NONE', #5704 ) ;
#8772=ORIENTED_EDGE ( 'NONE', *, *, #89921, .T. ) ;
#8782=CARTESIAN_POINT ( 'NONE',  ( 17.34090440699278091, 1422.638053189401944, 226.6050307785843074 ) ) ;
#8785=CARTESIAN_POINT ( 'NONE',  ( -7.450897614389999646, 1442.756953654919926, 149.7755488681980012 ) ) ;
#8786=CARTESIAN_POINT ( 'NONE',  ( 42.65467180383260626, 1440.913060353519995, 262.7680395952199888 ) ) ;
#8788=CARTESIAN_POINT ( 'NONE',  ( -19.70594995229999924, 1434.992946305789928, 207.5825935615879985 ) ) ;
#8789=CARTESIAN_POINT ( 'NONE',  ( 11.94174092869224069, 1433.516789646251709, 150.0943515355301088 ) ) ;
#8790=VERTEX_POINT ( 'NONE', #92432 ) ;
#8795=CARTESIAN_POINT ( 'NONE',  ( 11.79002570591860000, 1447.121451514569799, 187.8029540059399949 ) ) ;
#8797=B_SPLINE_SURFACE_WITH_KNOTS ( 'NONE', 5, 5, ( 
 ( #9139, #69626, #95351, #85271, #42741, #76902 ),
 ( #68513, #102611, #43301, #1867, #52811, #86943 ),
 ( #94793, #60109, #36001, #77451, #26473, #60667 ),
 ( #77993, #35439, #70192, #98500, #22319, #3927 ),
 ( #73874, #100162, #74436, #4463, #108562, #99592 ),
 ( #99041, #91207, #21768, #14489, #55969, #73315 ) ),
 .UNSPECIFIED., .F., .F., .F.,
 ( 6, 6 ),
 ( 6, 6 ),
 ( 30.36509140000000073, 167.7881597310000075 ),
 ( 0.000000000000000000, 2.000000000000000000 ),
 .UNSPECIFIED. ) ;
#8803=CARTESIAN_POINT ( 'NONE',  ( -27.40792122765466132, 1509.298960328587327, 212.0799651120152589 ) ) ;
#8806=VERTEX_POINT ( 'NONE', #31993 ) ;
#8807=CARTESIAN_POINT ( 'NONE',  ( -1.383993012750000196, 1414.983771848930019, 226.4898643371980143 ) ) ;
#8814=CARTESIAN_POINT ( 'NONE',  ( 38.29511879756229575, 1438.902673677490156, 136.6303356394320190 ) ) ;
#8819=CARTESIAN_POINT ( 'NONE',  ( -12.59663421299888952, 1435.821309450346234, 150.9177216549062450 ) ) ;
#8820=CARTESIAN_POINT ( 'NONE',  ( -19.08445480129999794, 1440.913060387330006, 209.8212738029720299 ) ) ;
#8821=CARTESIAN_POINT ( 'NONE',  ( 3.513330320889999747, 1409.035748585529973, 186.9170200111979625 ) ) ;
#8826=VECTOR ( 'NONE', #70650, 1000.000000000000114 ) ;
#8827=CARTESIAN_POINT ( 'NONE',  ( -1.816161586769259983, 1450.477603230480099, 183.3762537591580042 ) ) ;
#8828=CARTESIAN_POINT ( 'NONE',  ( 1.769009636590000101, 1464.859476624029867, 237.2742850304979925 ) ) ;
#8829=EDGE_LOOP ( 'NONE', ( #7924, #71453, #21652, #26337, #109582, #20371, #31744, #38232, #57977 ) ) ;
#8831=CARTESIAN_POINT ( 'NONE',  ( -41.96992763659999781, 1449.933563106350221, 270.3374075954979503 ) ) ;
#8832=CARTESIAN_POINT ( 'NONE',  ( -26.13694927001759893, 1446.561492601239934, 138.0017901643740004 ) ) ;
#8833=( BOUNDED_SURFACE ( )  B_SPLINE_SURFACE ( 1, 2, ( 
 ( #25020, #25573, #16067, #7687, #34544, #16605, #33422, #42391, #50802 ),
 ( #77120, #83297, #426, #15516, #17154, #110151, #49713, #74917, #109067 ) ),
 .UNSPECIFIED., .F., .T., .F. ) 
 B_SPLINE_SURFACE_WITH_KNOTS ( ( 2, 2 ),
 ( 3, 2, 2, 2, 3 ),
 ( -10000.00000000000000, 10000.00000000000000 ),
 ( 0.000000000000000000, 1.570796326794899889, 3.141592653589790007, 4.712388980384689674, 6.283185307179590673 ),
 .UNSPECIFIED. ) 
 GEOMETRIC_REPRESENTATION_ITEM ( )  RATIONAL_B_SPLINE_SURFACE ( (
 ( 1.000000000000000000, 0.7071067811865480168, 1.000000000000000000, 0.7071067811865480168, 1.000000000000000000, 0.7071067811865480168, 1.000000000000000000, 0.7071067811865480168, 1.000000000000000000),
 ( 1.000000000000000000, 0.7071067811865480168, 1.000000000000000000, 0.7071067811865480168, 1.000000000000000000, 0.7071067811865480168, 1.000000000000000000, 0.7071067811865480168, 1.000000000000000000) ) ) 
 REPRESENTATION_ITEM ( '' )  SURFACE ( )  );
#8835=CARTESIAN_POINT ( 'NONE',  ( 16.93412905219999942, 1468.808412830429916, 189.7276331636979876 ) ) ;
#8837=CARTESIAN_POINT ( 'NONE',  ( -6.910112620815310491E-10, 1470.927955446970145, 256.4164964148890249 ) ) ;
#8838=CARTESIAN_POINT ( 'NONE',  ( 20.51249426540298515, 1436.445542391833442, 144.8792686586828040 ) ) ;
#8839=CARTESIAN_POINT ( 'NONE',  ( -1.362314668290000030, 1416.021639799829927, 227.8893587007979988 ) ) ;
#8840=CARTESIAN_POINT ( 'NONE',  ( -8.457611602209999191, 1419.058770192229986, 232.4533566405980025 ) ) ;
#8845=CARTESIAN_POINT ( 'NONE',  ( -45.69545081991040547, 1437.710744842920121, 266.4180560666800375 ) ) ;
#8847=AXIS2_PLACEMENT_3D ( 'NONE', #39162, #40824, #107471 ) ;
#8851=CARTESIAN_POINT ( 'NONE',  ( -5.388310285459999349, 1432.653871653890064, 154.6144347680979934 ) ) ;
#8852=CARTESIAN_POINT ( 'NONE',  ( -25.98561794621749854, 1441.261220175949802, 138.2899389286700114 ) ) ;
#8855=CARTESIAN_POINT ( 'NONE',  ( -26.74532466102600026, 1451.223413308900035, 136.2813698317930005 ) ) ;
#8856=EDGE_LOOP ( 'NONE', ( #15872, #105713, #5822, #106759 ) ) ;
#8857=CARTESIAN_POINT ( 'NONE',  ( 29.14244744279999821, 1435.145987126659975, 238.0755329184979985 ) ) ;
#8861=CARTESIAN_POINT ( 'NONE',  ( 27.78452742954910093, 1508.000976259739900, 207.7754991261529938 ) ) ;
#8863=CARTESIAN_POINT ( 'NONE',  ( -17.60627563539920004, 1410.895669414250051, 194.0661810348550205 ) ) ;
#8864=CARTESIAN_POINT ( 'NONE',  ( -25.19103893129999960, 1437.530664664930100, 138.0353914523980166 ) ) ;
#8865=ORIENTED_EDGE ( 'NONE', *, *, #8257, .T. ) ;
#8866=CARTESIAN_POINT ( 'NONE',  ( -8.677567137620060933, 1408.534241456209884, 270.2786540372579793 ) ) ;
#8867=CARTESIAN_POINT ( 'NONE',  ( 10.82050651005049957, 1419.935650953779941, 231.8985719784330115 ) ) ;
#8869=CARTESIAN_POINT ( 'NONE',  ( -2.500000000000360156, 1439.188135388240198, 158.6514568555039943 ) ) ;
#8870=ORIENTED_EDGE ( 'NONE', *, *, #11242, .F. ) ;
#8872=CARTESIAN_POINT ( 'NONE',  ( -23.19576873519860172, 1410.004524903090214, 210.0850936017089907 ) ) ;
#8874=CARTESIAN_POINT ( 'NONE',  ( -2.923521517025829741, 1410.394928878200062, 186.6127595807840009 ) ) ;
#8876=CARTESIAN_POINT ( 'NONE',  ( -44.28110705741969610, 1432.290621434800414, 266.2283975843345729 ) ) ;
#8877=CARTESIAN_POINT ( 'NONE',  ( -18.28401409811200296, 1419.983726780179722, 194.9665186433740018 ) ) ;
#8878=CARTESIAN_POINT ( 'NONE',  ( -19.57049444700000151, 1420.832488470329963, 222.7981928031980203 ) ) ;
#8879=CARTESIAN_POINT ( 'NONE',  ( 40.86771873664179822, 1456.647620516569987, 268.9064048513220087 ) ) ;
#8885=CARTESIAN_POINT ( 'NONE',  ( -11.81944340819999972, 1433.674010844490113, 150.7526810563979893 ) ) ;
#8889=CARTESIAN_POINT ( 'NONE',  ( -1.205637028059169946, 1458.002444675669949, 229.8765855511719849 ) ) ;
#8892=CARTESIAN_POINT ( 'NONE',  ( 24.88318342085590018, 1452.039007177160101, 135.7900169370240064 ) ) ;
#8893=EDGE_CURVE ( 'NONE', #86228, #53112, #16636, .T. ) ;
#8896=B_SPLINE_CURVE_WITH_KNOTS ( 'NONE', 5,
 ( #35803, #69984, #53742, #26276, #45328, #79467 ),
 .UNSPECIFIED., .F., .F.,
 ( 6, 6 ),
 ( -106.8619706870000101, -30.32814661860000172 ),
 .UNSPECIFIED. ) ;
#8898=CARTESIAN_POINT ( 'NONE',  ( 16.85557976710000005, 1409.501670203030017, 194.3276026113979924 ) ) ;
#8899=B_SPLINE_SURFACE_WITH_KNOTS ( 'NONE', 5, 5, ( 
 ( #25670, #77757, #69937, #59863, #25116, #51446 ),
 ( #93988, #61528, #60417, #104051, #1066, #17809 ),
 ( #95656, #60981, #102927, #9442, #18923, #86149 ),
 ( #43606, #68280, #517, #53121, #87258, #85577 ),
 ( #44724, #78876, #8324, #102388, #36297, #69379 ),
 ( #70490, #43057, #59320, #35194, #17254, #93432 ) ),
 .UNSPECIFIED., .F., .F., .F.,
 ( 6, 6 ),
 ( 6, 6 ),
 ( 4.807626846469999826, 6.388845116620970543 ),
 ( 0.000000000000000000, 1.432659768743509865 ),
 .UNSPECIFIED. ) ;
#8901=CARTESIAN_POINT ( 'NONE',  ( 0.2331202188386839735, 1408.921201124740037, 186.4825399812679905 ) ) ;
#8908=ORIENTED_EDGE ( 'NONE', *, *, #48641, .T. ) ;
#8912=B_SPLINE_CURVE_WITH_KNOTS ( 'NONE', 3,
 ( #69563, #44344, #25291, #103682, #59493, #42128, #61172, #51633, #68449, #102552, #7961, #94725, #25845, #60047 ),
 .UNSPECIFIED., .F., .F.,
 ( 4, 2, 2, 2, 2, 2, 4 ),
 ( 0.000000000000000000, 0.2500000000000193179, 0.5000000000000386358, 0.6250000000000289768, 0.7500000000000193179, 0.8750000000000096589, 1.000000000000000000 ),
 .UNSPECIFIED. ) ;
#8913=B_SPLINE_SURFACE_WITH_KNOTS ( 'NONE', 5, 5, ( 
 ( #43827, #70722, #104834, #60091, #96438, #25892, #103726, #18592, #51680 ),
 ( #190, #10781, #26454, #34312, #28121, #62314, #95880, #86370, #103152 ),
 ( #69052, #52790, #19716, #9117, #19142, #35982, #78535, #53349, #731 ),
 ( #9655, #94206, #2409, #10215, #35421, #53919, #27029, #68492, #88053 ),
 ( #44393, #1846, #43281, #1280, #102592, #44954, #94771, #77430, #76880 ),
 ( #87494, #77974, #61217, #34863, #95332, #70172, #104283, #79100, #36526 ) ),
 .UNSPECIFIED., .F., .F., .F.,
 ( 6, 6 ),
 ( 6, 3, 6 ),
 ( 25.26539776070000087, 42.22154025839999747 ),
 ( 0.000000000000000000, 1.000000000000000000, 2.000000000000000000 ),
 .UNSPECIFIED. ) ;
#8916=CARTESIAN_POINT ( 'NONE',  ( -35.77265797339989462, 1450.098916315730094, 136.2386353496389688 ) ) ;
#8919=AXIS2_PLACEMENT_3D ( 'NONE', #74998, #109147, #74451 ) ;
#8921=CARTESIAN_POINT ( 'NONE',  ( 11.87922074009999918, 1433.306015784339934, 150.2908134751979787 ) ) ;
#8922=CARTESIAN_POINT ( 'NONE',  ( 13.21926163380000041, 1460.466222979229997, 248.0989693098979956 ) ) ;
#8924=CARTESIAN_POINT ( 'NONE',  ( 12.61115941410569974, 1416.521607925270018, 196.2004978253030174 ) ) ;
#8930=CARTESIAN_POINT ( 'NONE',  ( 22.71803131159999722, 1409.706390560829959, 209.2188350014689888 ) ) ;
#8931=CARTESIAN_POINT ( 'NONE',  ( 11.89222639830229156, 1398.265657350177207, 214.3730992004363713 ) ) ;
#8932=CARTESIAN_POINT ( 'NONE',  ( -30.01282678429459594, 1510.000041106939989, 208.7873087230510123 ) ) ;
#8934=CARTESIAN_POINT ( 'NONE',  ( 18.41411251730000131, 1430.349327995130125, 223.8639151150979956 ) ) ;
#8936=CARTESIAN_POINT ( 'NONE',  ( -41.53484662709239927, 1442.119007197383553, 135.5124903905762892 ) ) ;
#8938=CARTESIAN_POINT ( 'NONE',  ( 16.48401273470000206, 1408.913060387329779, 216.3372448727180313 ) ) ;
#8941=B_SPLINE_CURVE_WITH_KNOTS ( 'NONE', 5,
 ( #109382, #101488, #69048, #16376, #49476, #41053, #94204, #67390, #83598 ),
 .UNSPECIFIED., .F., .F.,
 ( 6, 3, 6 ),
 ( 0.000000000000000000, 0.5000001178084170217, 1.000000000000000000 ),
 .UNSPECIFIED. ) ;
#8943=CARTESIAN_POINT ( 'NONE',  ( 0.1654384182819229887, 1483.018567707959846, 181.9647163855690053 ) ) ;
#8947=DIRECTION ( 'NONE',  ( 0.000000000000000000, 0.000000000000000000, 1.000000000000000000 ) ) ;
#8955=CARTESIAN_POINT ( 'NONE',  ( -17.63393957150000091, 1415.931784855930118, 211.9458465498180146 ) ) ;
#8969=CARTESIAN_POINT ( 'NONE',  ( -15.80810346846800130, 1409.717633941269924, 226.1408703758089871 ) ) ;
#8973=ORIENTED_EDGE ( 'NONE', *, *, #64103, .F. ) ;
#8974=CARTESIAN_POINT ( 'NONE',  ( 23.61148526040000206, 1508.482535357130018, 222.5984954199980166 ) ) ;
#8977=VECTOR ( 'NONE', #45922, 1000.000000000000000 ) ;
#8978=CARTESIAN_POINT ( 'NONE',  ( 35.43993441567700131, 1457.286910017509399, 269.5376372890260654 ) ) ;
#8980=CARTESIAN_POINT ( 'NONE',  ( 18.99548197422359763, 1437.728065295126953, 213.2617020504292498 ) ) ;
#8981=CARTESIAN_POINT ( 'NONE',  ( 1.624355357520000043, 1415.847779888729974, 232.6127382033980098 ) ) ;
#8986=EDGE_CURVE ( 'NONE', #105450, #67100, #31339, .T. ) ;
#8988=CARTESIAN_POINT ( 'NONE',  ( 3.684086215580000268, 1446.644899200540067, 159.4624503042980166 ) ) ;
#8991=CARTESIAN_POINT ( 'NONE',  ( 13.63581072969999930, 1474.110335124630183, 269.6067227616979949 ) ) ;
#8993=ORIENTED_EDGE ( 'NONE', *, *, #70906, .F. ) ;
#8994=FACE_OUTER_BOUND ( 'NONE', #63743, .T. ) ;
#8997=CARTESIAN_POINT ( 'NONE',  ( -23.22702229119999728, 1430.350733269630155, 202.9151551450079864 ) ) ;
#8998=CARTESIAN_POINT ( 'NONE',  ( -10.74422203838610024, 1424.967024678149983, 139.7076782565099791 ) ) ;
#8999=CARTESIAN_POINT ( 'NONE',  ( 17.38493044761679940, 1410.884709072750184, 192.4605050727279831 ) ) ;
#9001=CARTESIAN_POINT ( 'NONE',  ( 28.88831231914572584, 1510.032855735962585, 201.0268679937729530 ) ) ;
#9003=CARTESIAN_POINT ( 'NONE',  ( -20.24918891140000099, 1453.165958253630151, 208.5428146401309846 ) ) ;
#9005=CARTESIAN_POINT ( 'NONE',  ( 17.48970627280642987, 1459.983305242940560, 228.4052134740612416 ) ) ;
#9008=CARTESIAN_POINT ( 'NONE',  ( -35.58396791106149948, 1437.290684582510039, 136.5355017401039959 ) ) ;
#9010=CARTESIAN_POINT ( 'NONE',  ( 7.539262298278820218, 1397.225239789469924, 197.6719658297510023 ) ) ;
#9013=CARTESIAN_POINT ( 'NONE',  ( -17.43253919180000011, 1460.024831443229914, 228.2391352219980263 ) ) ;
#9014=VERTEX_POINT ( 'NONE', #1725 ) ;
#9017=CARTESIAN_POINT ( 'NONE',  ( -29.26524805770378990, 1509.935219952241368, 211.6937577894515528 ) ) ;
#9018=CARTESIAN_POINT ( 'NONE',  ( -9.267034430364599729, 1423.582047745190039, 146.9531713541019826 ) ) ;
#9021=EDGE_CURVE ( 'NONE', #43805, #104880, #77316, .T. ) ;
#9030=ORIENTED_EDGE ( 'NONE', *, *, #64583, .F. ) ;
#9034=CARTESIAN_POINT ( 'NONE',  ( 11.80100415298899996, 1428.281167224610044, 148.2341325577170039 ) ) ;
#9035=EDGE_CURVE ( 'NONE', #101156, #61195, #15440, .T. ) ;
#9037=EDGE_LOOP ( 'NONE', ( #2252, #63462, #110091, #45254 ) ) ;
#9038=CARTESIAN_POINT ( 'NONE',  ( -13.15726448929999925, 1414.996444518330009, 220.4820292908979980 ) ) ;
#9040=DIRECTION ( 'NONE',  ( 0.000000000000000000, 1.000000000000000000, 0.000000000000000000 ) ) ;
#9042=CARTESIAN_POINT ( 'NONE',  ( -5.465716833969999300, 1421.576913351030043, 186.4279755057980026 ) ) ;
#9043=CARTESIAN_POINT ( 'NONE',  ( -7.613833802559419439, 1446.707927629628557, 154.1417109755026331 ) ) ;
#9047=CARTESIAN_POINT ( 'NONE',  ( -15.62174622799999923, 1462.582522095329978, 223.1630036629979941 ) ) ;
#9049=CARTESIAN_POINT ( 'NONE',  ( 17.80012153870000091, 1459.332523128830189, 228.1679591816979951 ) ) ;
#9050=DIRECTION ( 'NONE',  ( -0.7074300732568279404, -0.02470400251969399191, -0.7063514732138288510 ) ) ;
#9051=CARTESIAN_POINT ( 'NONE',  ( 15.54603130660830068, 1507.439213079509955, 225.8362344188779787 ) ) ;
#9053=CARTESIAN_POINT ( 'NONE',  ( -6.328696556262070949, 1422.647538939597780, 139.1419529473191972 ) ) ;
#9055=CARTESIAN_POINT ( 'NONE',  ( -0.03226023477341029982, 1410.297896964309984, 185.0217421575940193 ) ) ;
#9056=ORIENTED_EDGE ( 'NONE', *, *, #43961, .T. ) ;
#9057=EDGE_CURVE ( 'NONE', #59173, #36566, #25975, .T. ) ;
#9058=CARTESIAN_POINT ( 'NONE',  ( 18.17529663798200090, 1424.501927100039893, 223.8627669670750038 ) ) ;
#9060=CARTESIAN_POINT ( 'NONE',  ( -2.898382840419457818, 1484.352318093022632, 183.3103537128903895 ) ) ;
#9062=EDGE_CURVE ( 'NONE', #80364, #48449, #35863, .T. ) ;
#9064=ORIENTED_EDGE ( 'NONE', *, *, #20118, .F. ) ;
#9065=CARTESIAN_POINT ( 'NONE',  ( 0.9069153359830000038, 1434.997135647769937, 189.4159220886979824 ) ) ;
#9068=CARTESIAN_POINT ( 'NONE',  ( -11.82648314689999935, 1429.505905138129947, 149.6875397860980001 ) ) ;
#9069=CARTESIAN_POINT ( 'NONE',  ( -5.386185223340929973, 1432.347042777500064, 154.6076275972019971 ) ) ;
#9072=CARTESIAN_POINT ( 'NONE',  ( 7.121584085660000341, 1409.161751583630121, 222.2855843900980233 ) ) ;
#9075=EDGE_CURVE ( 'NONE', #61499, #97372, #94651, .T. ) ;
#9076=CARTESIAN_POINT ( 'NONE',  ( 13.36463437909999996, 1410.400759883430055, 228.3459572537979909 ) ) ;
#9077=CARTESIAN_POINT ( 'NONE',  ( -20.56562140180000142, 1508.015221763929958, 228.3467905896980028 ) ) ;
#9081=CARTESIAN_POINT ( 'NONE',  ( 23.65302801580000036, 1410.800135283929876, 267.0034940390980296 ) ) ;
#9083=ADVANCED_FACE ( 'NONE', ( #27445 ), #6954, .F. ) ;
#9084=CARTESIAN_POINT ( 'NONE',  ( 18.33825317269999999, 1449.737352364420076, 190.9873845589980021 ) ) ;
#9085=CARTESIAN_POINT ( 'NONE',  ( -0.2681387158619999433, 1507.638498121229759, 237.3507797630980178 ) ) ;
#9087=CARTESIAN_POINT ( 'NONE',  ( -41.15025406726699231, 1443.128258067170009, 136.8582507510139976 ) ) ;
#9088=CARTESIAN_POINT ( 'NONE',  ( -7.598474438054299895, 1407.528248760620045, 198.4581846281600122 ) ) ;
#9091=CARTESIAN_POINT ( 'NONE',  ( -13.45920590230000080, 1444.312827231819938, 187.2388222693979856 ) ) ;
#9092=CARTESIAN_POINT ( 'NONE',  ( -16.39250384509999847, 1431.113060387329824, 219.3475551130979966 ) ) ;
#9095=CARTESIAN_POINT ( 'NONE',  ( -6.040745412617011922, 1457.036252898433759, 228.2768262899412548 ) ) ;
#9098=CARTESIAN_POINT ( 'NONE',  ( -14.86811171559539879, 1409.432266289319841, 210.5260528434040168 ) ) ;
#9100=SPHERICAL_SURFACE ( 'NONE', #109916, 2.000000000680000056 ) ;
#9101=CARTESIAN_POINT ( 'NONE',  ( -14.63733634519999960, 1474.309184518629991, 267.4468043569979727 ) ) ;
#9104=CARTESIAN_POINT ( 'NONE',  ( -24.56423024638272778, 1444.748822478129341, 210.9347104645846116 ) ) ;
#9106=CARTESIAN_POINT ( 'NONE',  ( -24.40236318204969379, 1436.401018377404853, 210.7321041510820692 ) ) ;
#9108=CARTESIAN_POINT ( 'NONE',  ( -14.22405469409999945, 1409.409775322530095, 225.3473850829980165 ) ) ;
#9109=CARTESIAN_POINT ( 'NONE',  ( 12.13275115577349972, 1416.073666497539989, 223.4459935694849833 ) ) ;
#9110=EDGE_CURVE ( 'NONE', #12333, #10428, #15263, .T. ) ;
#9111=CARTESIAN_POINT ( 'NONE',  ( -26.40673502673280026, 1495.359935024549941, 211.4908345026910013 ) ) ;
#9114=CARTESIAN_POINT ( 'NONE',  ( -23.67432059500000108, 1410.661424214930094, 207.0403095298379981 ) ) ;
#9117=CARTESIAN_POINT ( 'NONE',  ( 15.60349182690000092, 1415.087797054229895, 201.7328695000580012 ) ) ;
#9124=CARTESIAN_POINT ( 'NONE',  ( -22.91694383419999781, 1410.643289684830052, 211.0883591864180175 ) ) ;
#9126=CARTESIAN_POINT ( 'NONE',  ( 10.93238010538601657, 1414.913060581095351, 222.2496003354920333 ) ) ;
#9127=CARTESIAN_POINT ( 'NONE',  ( 11.72537925141179826, 1426.703358321739870, 143.3352947567420017 ) ) ;
#9136=CARTESIAN_POINT ( 'NONE',  ( -4.295246787833081115, 1398.041196492937843, 221.3918056679002575 ) ) ;
#9138=FACE_OUTER_BOUND ( 'NONE', #28278, .T. ) ;
#9139=CARTESIAN_POINT ( 'NONE',  ( -17.99923967009999970, 1410.894937295029877, 195.2567800406980041 ) ) ;
#9141=CARTESIAN_POINT ( 'NONE',  ( 40.85596413570220165, 1446.221434197089820, 136.5631368516420139 ) ) ;
#9145=CARTESIAN_POINT ( 'NONE',  ( 11.95088893593300128, 1433.527687467219948, 149.9885903255629955 ) ) ;
#9146=CARTESIAN_POINT ( 'NONE',  ( 27.86052284579999849, 1509.876774252430096, 216.4221030366980187 ) ) ;
#9148=CARTESIAN_POINT ( 'NONE',  ( 2.522951803030079727E-08, 1397.914279477030050, 222.1218461579910297 ) ) ;
#9152=CARTESIAN_POINT ( 'NONE',  ( 2.409586283469999923, 1426.663880916129983, 144.1938086916980239 ) ) ;
#9153=CARTESIAN_POINT ( 'NONE',  ( 18.56073619233890071, 1498.114107680659799, 229.6370383981259806 ) ) ;
#9156=CARTESIAN_POINT ( 'NONE',  ( 3.154888307769999845, 1507.639342598330131, 181.4414887542980068 ) ) ;
#9157=CARTESIAN_POINT ( 'NONE',  ( -5.061321235330000334, 1415.087745006229852, 192.8151508637980101 ) ) ;
#9161=CARTESIAN_POINT ( 'NONE',  ( 14.34456629291880070, 1416.134159100540046, 196.9681562124789878 ) ) ;
#9162=CARTESIAN_POINT ( 'NONE',  ( 11.86050315890000029, 1431.927500028019949, 150.3837318091979967 ) ) ;
#9165=CARTESIAN_POINT ( 'NONE',  ( 13.99694514614609808, 1435.072495206890153, 149.0791654432190114 ) ) ;
#9169=CARTESIAN_POINT ( 'NONE',  ( 12.96262155038025554, 1444.899173449604177, 169.4271127342331908 ) ) ;
#9170=CARTESIAN_POINT ( 'NONE',  ( -0.4726074384389999938, 1465.085986095130011, 236.9699255896980219 ) ) ;
#9175=CARTESIAN_POINT ( 'NONE',  ( -19.05441023136656753, 1442.634723914723963, 210.8671806021638702 ) ) ;
#9178=( BOUNDED_CURVE ( )  B_SPLINE_CURVE ( 3, ( #74524, #101886, #76706, #40894 ),
 .UNSPECIFIED., .F., .F. ) 
 B_SPLINE_CURVE_WITH_KNOTS ( ( 4, 4 ),
 ( 6.031750314274309410, 6.430153894057509589 ),
 .UNSPECIFIED. ) 
 CURVE ( )  GEOMETRIC_REPRESENTATION_ITEM ( )  RATIONAL_B_SPLINE_CURVE ( ( 1.000000000000000000, 0.9868165636486558867, 0.9868165636486558867, 1.000000000000000000 ) ) 
 REPRESENTATION_ITEM ( '' )  );
#9179=B_SPLINE_CURVE_WITH_KNOTS ( 'NONE', 3,
 ( #26257, #86177, #9469, #41002, #43634, #78332, #1643 ),
 .UNSPECIFIED., .F., .F.,
 ( 4, 3, 4 ),
 ( -89.14624201249999658, -56.86225756220769512, -20.47911906334890375 ),
 .UNSPECIFIED. ) ;
#9183=CARTESIAN_POINT ( 'NONE',  ( 19.84271301760869832, 1440.913060387330006, 215.4053540786730139 ) ) ;
#9185=ADVANCED_FACE ( 'NONE', ( #19592 ), #100805, .F. ) ;
#9186=ORIENTED_EDGE ( 'NONE', *, *, #15352, .T. ) ;
#9187=CARTESIAN_POINT ( 'NONE',  ( -5.555854370870000558, 1409.107075097130291, 188.5359587977980027 ) ) ;
#9189=CARTESIAN_POINT ( 'NONE',  ( -11.24049413600000058, 1414.988015881329829, 195.7612515219979912 ) ) ;
#9191=CARTESIAN_POINT ( 'NONE',  ( 21.58388069929999986, 1429.957715527830032, 219.4703653642980044 ) ) ;
#9193=B_SPLINE_CURVE_WITH_KNOTS ( 'NONE', 5,
 ( #11023, #95024, #54154, #62569, #19960, #9365 ),
 .UNSPECIFIED., .F., .F.,
 ( 6, 6 ),
 ( 0.000000000000000000, 1.000000000000000000 ),
 .UNSPECIFIED. ) ;
#9207=CARTESIAN_POINT ( 'NONE',  ( -18.13278339737094669, 1486.179330754719786, 188.5833977309001739 ) ) ;
#9209=VERTEX_POINT ( 'NONE', #58181 ) ;
#9211=CARTESIAN_POINT ( 'NONE',  ( 34.21123855309999584, 1452.338600522630031, 254.6787333579979986 ) ) ;
#9212=CARTESIAN_POINT ( 'NONE',  ( 3.524967334472002278, 1450.792428028305494, 184.0702269475962680 ) ) ;
#9213=CARTESIAN_POINT ( 'NONE',  ( -11.79165762230000070, 1429.416862815430022, 146.4064176768980019 ) ) ;
#9214=CARTESIAN_POINT ( 'NONE',  ( -8.160870615792729765, 1509.019321687440197, 236.3691303609340082 ) ) ;
#9216=CARTESIAN_POINT ( 'NONE',  ( -23.83643911649999936, 1446.361787448990071, 213.8673211433680024 ) ) ;
#9218=DIRECTION ( 'NONE',  ( -0.7067700363771035610, 0.03085824620770448445, 0.7067700363771036720 ) ) ;
#9219=CARTESIAN_POINT ( 'NONE',  ( 17.27890247157979786, 1409.608338727829960, 222.4184771258499893 ) ) ;
#9222=ORIENTED_EDGE ( 'NONE', *, *, #46216, .F. ) ;
#9226=CARTESIAN_POINT ( 'NONE',  ( 27.70374302159999758, 1507.991978481930119, 207.6872388016580260 ) ) ;
#9227=CARTESIAN_POINT ( 'NONE',  ( 12.70878548640000005, 1419.800077408030120, 223.4159102764979821 ) ) ;
#9228=CARTESIAN_POINT ( 'NONE',  ( 5.387463376540000404, 1432.539377501929948, 154.6119119043980277 ) ) ;
#9229=CARTESIAN_POINT ( 'NONE',  ( -4.363122647530000009, 1423.854802298929826, 178.2623905312979957 ) ) ;
#9230=CARTESIAN_POINT ( 'NONE',  ( -20.35720354223120054, 1509.285576857579827, 188.5733128882430094 ) ) ;
#9232=CARTESIAN_POINT ( 'NONE',  ( 33.30036996651080017, 1435.821070638500032, 135.9642379680810222 ) ) ;
#9233=CARTESIAN_POINT ( 'NONE',  ( 36.78992615597000082, 1449.659024602699901, 136.2786194408189715 ) ) ;
#9234=CARTESIAN_POINT ( 'NONE',  ( -41.27798004816977340, 1455.501545579069443, 269.0951446923482990 ) ) ;
#9238=CARTESIAN_POINT ( 'NONE',  ( 10.10004869885203682, 1411.254281879943164, 137.0999999980979851 ) ) ;
#9239=ORIENTED_EDGE ( 'NONE', *, *, #33959, .T. ) ;
#9240=CARTESIAN_POINT ( 'NONE',  ( -6.832964021560000489, 1409.413060387330006, 271.1218459616979999 ) ) ;
#9243=CARTESIAN_POINT ( 'NONE',  ( 16.84953930043489834, 1504.811272959099824, 188.1836725605500078 ) ) ;
#9244=CARTESIAN_POINT ( 'NONE',  ( 11.01434323564089546, 1425.013952765832983, 138.3678689716161614 ) ) ;
#9251=CARTESIAN_POINT ( 'NONE',  ( -13.22973741984542784, 1419.796952795795278, 228.0648478904874139 ) ) ;
#9252=CARTESIAN_POINT ( 'NONE',  ( -37.66849514949689848, 1445.052233488579986, 137.0436250779820000 ) ) ;
#9254=CARTESIAN_POINT ( 'NONE',  ( 24.93943963239999917, 1435.368420818290133, 135.8598268128979782 ) ) ;
#9255=CARTESIAN_POINT ( 'NONE',  ( -11.04150331276600028, 1396.298638179350064, 208.3126073074500084 ) ) ;
#9257=CARTESIAN_POINT ( 'NONE',  ( -17.33055221583169825, 1410.741059433489909, 225.8597740937110245 ) ) ;
#9263=CARTESIAN_POINT ( 'NONE',  ( 10.66298931770000102, 1425.717966165029793, 91.92307070169779593 ) ) ;
#9265=CARTESIAN_POINT ( 'NONE',  ( -10.98202954919999996, 1433.094628001990031, 151.7694013171979748 ) ) ;
#9270=CARTESIAN_POINT ( 'NONE',  ( 3.202543372079999617, 1449.460684387319816, 183.9015485015980005 ) ) ;
#9272=CARTESIAN_POINT ( 'NONE',  ( -1.063679629813300442, 1465.068952270626824, 237.9910131846521892 ) ) ;
#9273=ORIENTED_EDGE ( 'NONE', *, *, #70145, .T. ) ;
#9275=LINE ( 'NONE', #35566, #1501 ) ;
#9277=CARTESIAN_POINT ( 'NONE',  ( 2.658194159920000229E-12, 1471.586156922030113, 269.6149382602980040 ) ) ;
#9279=CARTESIAN_POINT ( 'NONE',  ( -3.493700197999999979, 1486.025447731730083, 182.1170718226980227 ) ) ;
#9283=CARTESIAN_POINT ( 'NONE',  ( -22.78047381600000065, 1519.913060387329779, 203.9569696715980172 ) ) ;
#9285=CARTESIAN_POINT ( 'NONE',  ( 3.125347622798469782, 1407.037771531689941, 196.1218459610850005 ) ) ;
#9286=CARTESIAN_POINT ( 'NONE',  ( -12.14280743485850067, 1406.971422057159998, 268.4212961918660199 ) ) ;
#9289=CARTESIAN_POINT ( 'NONE',  ( -11.86572145370000086, 1432.317384755180001, 150.3971827880980072 ) ) ;
#9290=CARTESIAN_POINT ( 'NONE',  ( 12.96054471030000066, 1446.716588664140090, 188.5511171461979814 ) ) ;
#9294=CARTESIAN_POINT ( 'NONE',  ( 4.860846556981773148, 1422.361256645696585, 184.3086965326904760 ) ) ;
#9297=CARTESIAN_POINT ( 'NONE',  ( -12.90603589790000072, 1485.480164596930081, 186.0404649208980175 ) ) ;
#9299=CARTESIAN_POINT ( 'NONE',  ( -11.49747572423030029, 1414.913060387329779, 197.9009878255399997 ) ) ;
#9303=EDGE_CURVE ( 'NONE', #104433, #80324, #43467, .T. ) ;
#9304=CARTESIAN_POINT ( 'NONE',  ( -28.28536570780000048, 1509.154939129630066, 207.7087783032280015 ) ) ;
#9305=EDGE_CURVE ( 'NONE', #47913, #38319, #79352, .T. ) ;
#9312=CARTESIAN_POINT ( 'NONE',  ( -1.757532416683340148, 1451.933574871519795, 184.1885909450070073 ) ) ;
#9314=CARTESIAN_POINT ( 'NONE',  ( -24.16765274424039944, 1411.086006602699854, 209.4242098710629989 ) ) ;
#9315=CARTESIAN_POINT ( 'NONE',  ( 27.00673397879999982, 1508.127684930929945, 214.8638446572979888 ) ) ;
#9316=CARTESIAN_POINT ( 'NONE',  ( 19.96912209102779912, 1487.432069230659863, 226.3893998912439827 ) ) ;
#9317=CARTESIAN_POINT ( 'NONE',  ( -25.58013815969999882, 1435.410414332659911, 135.7415235870979870 ) ) ;
#9319=AXIS2_PLACEMENT_3D ( 'NONE', #50389, #61007, #101850 ) ;
#9321=EDGE_CURVE ( 'NONE', #58739, #84614, #29952, .T. ) ;
#9325=EDGE_LOOP ( 'NONE', ( #32015, #106924, #77408, #2309 ) ) ;
#9326=CARTESIAN_POINT ( 'NONE',  ( 2.500000000000000000, 1433.874165682790135, 157.5407159993979747 ) ) ;
#9330=B_SPLINE_CURVE_WITH_KNOTS ( 'NONE', 3,
 ( #33684, #9590, #51065, #66782, #67879, #33139 ),
 .UNSPECIFIED., .F., .F.,
 ( 4, 2, 4 ),
 ( -0.2938203139006840270, -0.1489810209828570098, -1.348803076839377724E-06 ),
 .UNSPECIFIED. ) ;
#9334=CARTESIAN_POINT ( 'NONE',  ( 12.22653077411650102, 1434.139770046449939, 149.8861139874390176 ) ) ;
#9335=CARTESIAN_POINT ( 'NONE',  ( -4.069613198648311503, 1440.892824350064529, 185.0069551270901229 ) ) ;
#9336=CARTESIAN_POINT ( 'NONE',  ( -23.79097876124399846, 1507.893941173470012, 222.8398483086459976 ) ) ;
#9337=CARTESIAN_POINT ( 'NONE',  ( -1.943613794290000030, 1409.147975346630119, 186.8816397165979879 ) ) ;
#9341=CARTESIAN_POINT ( 'NONE',  ( -3.266559724300000411, 1419.654073176930069, 186.2489323254980036 ) ) ;
#9344=ORIENTED_EDGE ( 'NONE', *, *, #22570, .T. ) ;
#9347=CARTESIAN_POINT ( 'NONE',  ( -0.7210096769089999746, 1490.513422156730030, 181.4676356941980089 ) ) ;
#9350=CARTESIAN_POINT ( 'NONE',  ( -4.363122647530000009, 1421.971318475729959, 172.2701767054979882 ) ) ;
#9355=DIRECTION ( 'NONE',  ( -1.000000000000000000, -8.350994020400001099E-15, -2.004238564900000104E-13 ) ) ;
#9356=CARTESIAN_POINT ( 'NONE',  ( 14.38488119590115488, 1507.535237583830849, 232.5758862642972247 ) ) ;
#9357=CARTESIAN_POINT ( 'NONE',  ( 11.79165762230000070, 1429.416862815430022, 146.4064176768980019 ) ) ;
#9358=CARTESIAN_POINT ( 'NONE',  ( 16.14995240670000243, 1471.299568758330224, 195.1298844619979889 ) ) ;
#9359=CARTESIAN_POINT ( 'NONE',  ( 39.73140103348869445, 1440.913060368030074, 258.9046876989520456 ) ) ;
#9360=CARTESIAN_POINT ( 'NONE',  ( 15.27152964737910068, 1506.433683733550197, 193.3098315259690025 ) ) ;
#9361=CARTESIAN_POINT ( 'NONE',  ( -2.793439186891359949, 1486.025328193850100, 182.0741020391329812 ) ) ;
#9362=CARTESIAN_POINT ( 'NONE',  ( 11.31406713481371362, 1433.949558832472121, 151.5135725724176439 ) ) ;
#9363=ORIENTED_EDGE ( 'NONE', *, *, #61122, .T. ) ;
#9364=CARTESIAN_POINT ( 'NONE',  ( 1.556187358146779998, 1415.184612915219986, 191.2576310833790103 ) ) ;
#9365=CARTESIAN_POINT ( 'NONE',  ( 28.15443155984639745, 1509.896245780209938, 217.4026704617729990 ) ) ;
#9366=CARTESIAN_POINT ( 'NONE',  ( -27.72455330040000021, 1507.994297257130029, 210.5349572574680224 ) ) ;
#9367=CARTESIAN_POINT ( 'NONE',  ( 4.060573924520632261, 1410.431253889573782, 186.0508650619275954 ) ) ;
#9368=CARTESIAN_POINT ( 'NONE',  ( -3.813754118949360894, 1426.014263033397583, 186.0222677740474069 ) ) ;
#9369=CARTESIAN_POINT ( 'NONE',  ( 2.109961980403928905, 1410.360755918536825, 231.8875558583745828 ) ) ;
#9374=CARTESIAN_POINT ( 'NONE',  ( 20.90601844020000044, 1451.753496920530097, 144.3735648103979941 ) ) ;
#9378=EDGE_LOOP ( 'NONE', ( #36220, #15546, #34385 ) ) ;
#9379=CARTESIAN_POINT ( 'NONE',  ( -18.69043176373318715, 1458.332274568611865, 227.3714872367983162 ) ) ;
#9381=CARTESIAN_POINT ( 'NONE',  ( -0.4920987264512118320, 1416.537162660588820, 233.7617262382077854 ) ) ;
#9382=ORIENTED_EDGE ( 'NONE', *, *, #50002, .F. ) ;
#9384=CARTESIAN_POINT ( 'NONE',  ( 11.79002570591860000, 1447.121451514569799, 187.8029540059399949 ) ) ;
#9385=CARTESIAN_POINT ( 'NONE',  ( 18.02093535799999913, 1424.326836137830014, 225.1991050518980160 ) ) ;
#9386=CARTESIAN_POINT ( 'NONE',  ( 40.27144807147075767, 1443.454046232561950, 137.0977477732117222 ) ) ;
#9387=CARTESIAN_POINT ( 'NONE',  ( 19.67719249089999778, 1452.817890304029788, 209.0349214551060015 ) ) ;
#9391=CARTESIAN_POINT ( 'NONE',  ( -0.5697963391879999895, 1450.893162800530263, 181.2886238165980046 ) ) ;
#9392=DIRECTION ( 'NONE',  ( 0.000000000000000000, 0.000000000000000000, -1.000000000000000000 ) ) ;
#9393=CARTESIAN_POINT ( 'NONE',  ( 4.000901505650000800, 1409.052774946530008, 187.0792394566980192 ) ) ;
#9394=CARTESIAN_POINT ( 'NONE',  ( -0.0001187281342228439996, 1508.967929526819944, 179.3767679645770272 ) ) ;
#9395=CARTESIAN_POINT ( 'NONE',  ( -7.134031852310000588, 1442.025630767510165, 154.4960303242980046 ) ) ;
#9396=CARTESIAN_POINT ( 'NONE',  ( 11.10313694099999893, 1434.937812064100171, 151.7082819323979948 ) ) ;
#9399=CARTESIAN_POINT ( 'NONE',  ( -2.038535907758979970, 1450.880163189499854, 184.1774945304460118 ) ) ;
#9400=CARTESIAN_POINT ( 'NONE',  ( 1.358136954149999909, 1466.377669086430160, 235.0851390371979903 ) ) ;
#9401=ORIENTED_EDGE ( 'NONE', *, *, #110707, .F. ) ;
#9404=CARTESIAN_POINT ( 'NONE',  ( -42.28243328599999273, 1442.407792791449992, 269.8809849862979604 ) ) ;
#9405=CARTESIAN_POINT ( 'NONE',  ( -26.80104139319950107, 1446.506287351420042, 137.4021342824260046 ) ) ;
#9406=CARTESIAN_POINT ( 'NONE',  ( 11.89522282729999958, 1434.541161981840105, 151.0452005854980086 ) ) ;
#9411=CARTESIAN_POINT ( 'NONE',  ( -7.555873979100000248, 1418.426267280130105, 231.8714557520980009 ) ) ;
#9412=B_SPLINE_CURVE_WITH_KNOTS ( 'NONE', 3,
 ( #60309, #94428, #17147, #93335 ),
 .UNSPECIFIED., .F., .F.,
 ( 4, 4 ),
 ( 2.359153149548954932E-13, 0.0008464750159282172573 ),
 .UNSPECIFIED. ) ;
#9414=CARTESIAN_POINT ( 'NONE',  ( -0.08237014995780950199, 1486.172125964604220, 181.8174796312961803 ) ) ;
#9416=CARTESIAN_POINT ( 'NONE',  ( -46.13232427859189499, 1439.830690899319961, 268.2051409423269774 ) ) ;
#9417=CARTESIAN_POINT ( 'NONE',  ( -3.603587107540000112, 1436.962766753449841, 185.5233392668979775 ) ) ;
#9421=DIRECTION ( 'NONE',  ( 0.000000000000000000, 0.000000000000000000, 1.000000000000000000 ) ) ;
#9422=CARTESIAN_POINT ( 'NONE',  ( 19.26390258110135534, 1456.145399297611448, 225.0436448590560587 ) ) ;
#9424=CARTESIAN_POINT ( 'NONE',  ( -25.31835743630890079, 1452.013124259819961, 135.5916582954220075 ) ) ;
#9426=CARTESIAN_POINT ( 'NONE',  ( -15.00920760809999877, 1488.805759878829804, 193.8727931445979777 ) ) ;
#9428=CARTESIAN_POINT ( 'NONE',  ( 13.98962170100000080, 1452.815214894029850, 195.1980501640979924 ) ) ;
#9431=DIRECTION ( 'NONE',  ( 0.000000000000000000, -0.9989866842452286289, 0.04500671839541338370 ) ) ;
#9434=CARTESIAN_POINT ( 'NONE',  ( -3.016912340155930128, 1409.850859107569931, 270.0717562529079601 ) ) ;
#9436=CARTESIAN_POINT ( 'NONE',  ( 4.721853743513210411, 1416.907067146989903, 231.6953472553319955 ) ) ;
#9437=CARTESIAN_POINT ( 'NONE',  ( -0.2886430721605260930, 1507.883296045167526, 237.4859371806405477 ) ) ;
#9441=CARTESIAN_POINT ( 'NONE',  ( -22.80095230299680154, 1409.739651980310100, 209.6803998413979855 ) ) ;
#9442=CARTESIAN_POINT ( 'NONE',  ( -0.5472265402873980333, 1409.436775872690077, 185.2931106816229772 ) ) ;
#9444=CARTESIAN_POINT ( 'NONE',  ( -4.665393456780000392, 1427.510941591930077, 123.0297916884979941 ) ) ;
#9445=CARTESIAN_POINT ( 'NONE',  ( -15.86142964305496328, 1436.287026273651236, 149.0794767532250376 ) ) ;
#9446=CARTESIAN_POINT ( 'NONE',  ( -17.82322816519999975, 1420.841307626830030, 225.8555466793980031 ) ) ;
#9448=CARTESIAN_POINT ( 'NONE',  ( 29.93888874088349894, 1467.326863092750045, 268.9541358474360209 ) ) ;
#9449=CARTESIAN_POINT ( 'NONE',  ( -4.904755620210820233, 1466.423659703103340, 234.4687970439992455 ) ) ;
#9453=DIRECTION ( 'NONE',  ( 0.03489949670250328678, 0.9993908270190956511, -1.802540234690167715E-19 ) ) ;
#9455=CARTESIAN_POINT ( 'NONE',  ( 23.52858676739999666, 1410.126050507929904, 208.3803572285970063 ) ) ;
#9458=CARTESIAN_POINT ( 'NONE',  ( 26.74166369658919962, 1451.062954263790061, 136.3717679156470126 ) ) ;
#9459=EDGE_CURVE ( 'NONE', #48606, #17250, #22917, .T. ) ;
#9463=CARTESIAN_POINT ( 'NONE',  ( 18.11184817270000025, 1410.042143777230194, 194.0622353138979861 ) ) ;
#9464=CARTESIAN_POINT ( 'NONE',  ( 27.48389906189999721, 1444.324653571829913, 168.8435737885979790 ) ) ;
#9465=CARTESIAN_POINT ( 'NONE',  ( 2.927892279132241260, 1439.671353555214864, 184.0067670968116715 ) ) ;
#9467=CARTESIAN_POINT ( 'NONE',  ( -18.74856935563128957, 1424.596591154755515, 224.6369667799821741 ) ) ;
#9468=CARTESIAN_POINT ( 'NONE',  ( 1.211734507026360097, 1452.507822344910210, 183.4303198485629878 ) ) ;
#9469=CARTESIAN_POINT ( 'NONE',  ( 19.29501924868120000, 1492.614329036100116, 228.8343218840969939 ) ) ;
#9471=CARTESIAN_POINT ( 'NONE',  ( 16.68463225900990210, 1445.052233488270076, 162.0935120915889911 ) ) ;
#9473=CARTESIAN_POINT ( 'NONE',  ( 12.92134813639719937, 1416.521607925270018, 221.7330053757000030 ) ) ;
#9474=LINE ( 'NONE', #34121, #89213 ) ;
#9475=CARTESIAN_POINT ( 'NONE',  ( -0.4819983852477000563, 1409.558626638459828, 232.9244056882299958 ) ) ;
#9478=CARTESIAN_POINT ( 'NONE',  ( 0.02610324308704914387, 1506.535970896533854, 231.1903710126655653 ) ) ;
#9479=CARTESIAN_POINT ( 'NONE',  ( -12.48077398090000045, 1459.371347868330076, 243.9198229205979942 ) ) ;
#9480=CARTESIAN_POINT ( 'NONE',  ( -2.906507337806380153, 1458.419515837879999, 184.4676491233109914 ) ) ;
#9481=CARTESIAN_POINT ( 'NONE',  ( 11.18751708150000113, 1433.873588989760037, 151.6203832400979934 ) ) ;
#9482=CARTESIAN_POINT ( 'NONE',  ( 7.553102823739999749, 1458.344558665030036, 234.3916895749979687 ) ) ;
#9483=CARTESIAN_POINT ( 'NONE',  ( 12.81744069099580052, 1415.938742849230039, 196.5159729447089774 ) ) ;
#9487=CARTESIAN_POINT ( 'NONE',  ( -13.70191729650000134, 1486.504808716829984, 185.2020610571979944 ) ) ;
#9488=CARTESIAN_POINT ( 'NONE',  ( 12.63310190591395887, 1398.287565835977830, 206.0545710329436133 ) ) ;
#9489=CARTESIAN_POINT ( 'NONE',  ( 1.928731171289999935, 1466.614202310529890, 234.5248722603980127 ) ) ;
#9490=CARTESIAN_POINT ( 'NONE',  ( 22.95381948220000012, 1410.909818696329921, 213.5977567476680008 ) ) ;
#9491=CARTESIAN_POINT ( 'NONE',  ( 2.499999999999999112, 1447.900700312901108, 170.5263301090720915 ) ) ;
#9492=CARTESIAN_POINT ( 'NONE',  ( 25.00977876991279913, 1436.598012848749931, 137.9330263815630246 ) ) ;
#9499=B_SPLINE_CURVE_WITH_KNOTS ( 'NONE', 5,
 ( #21781, #28008, #71151, #11231, #80067, #89012, #80626, #96323, #106913 ),
 .UNSPECIFIED., .F., .F.,
 ( 6, 3, 6 ),
 ( 0.000000000000000000, 0.5050532947643375792, 1.000000000000000000 ),
 .UNSPECIFIED. ) ;
#9502=CARTESIAN_POINT ( 'NONE',  ( -1.121268592569999889, 1416.831305870130109, 228.0850991587980161 ) ) ;
#9503=CARTESIAN_POINT ( 'NONE',  ( -16.68463225827361995, 1445.052233488289630, 162.0935120918203154 ) ) ;
#9504=CARTESIAN_POINT ( 'NONE',  ( -24.68077630836099701, 1437.736159206269804, 210.5119845322900005 ) ) ;
#9508=CARTESIAN_POINT ( 'NONE',  ( -38.60856581307790236, 1443.613625294319945, 137.1750438966080026 ) ) ;
#9510=CARTESIAN_POINT ( 'NONE',  ( -0.5805478584864469660, 1457.956445091640035, 229.5817085807559863 ) ) ;
#9517=CARTESIAN_POINT ( 'NONE',  ( -17.07255110680000243, 1412.953535666930065, 191.8935328429979847 ) ) ;
#9520=CARTESIAN_POINT ( 'NONE',  ( -15.69557462584969798, 1410.567954306330194, 226.7002212045480007 ) ) ;
#9523=CARTESIAN_POINT ( 'NONE',  ( 0.000000000000000000, 1443.913060387330006, 126.8032249175980155 ) ) ;
#9525=CARTESIAN_POINT ( 'NONE',  ( 26.60754018289999934, 1509.169817829930025, 216.8086175352880218 ) ) ;
#9529=CARTESIAN_POINT ( 'NONE',  ( 13.42479616400980014, 1453.338203267170002, 224.7140346886050111 ) ) ;
#9530=CARTESIAN_POINT ( 'NONE',  ( 6.170313737849999924, 1397.182081568630110, 220.3579539676979948 ) ) ;
#9537=CARTESIAN_POINT ( 'NONE',  ( 3.123967384229999755, 1446.720974403119953, 162.7331095090980000 ) ) ;
#9538=CARTESIAN_POINT ( 'NONE',  ( -2.500000000000000000, 1438.363963900590079, 157.6955293123980084 ) ) ;
#9542=CARTESIAN_POINT ( 'NONE',  ( 11.17472318946589382, 1414.941152333678701, 222.2292738415587223 ) ) ;
#9544=CARTESIAN_POINT ( 'NONE',  ( 12.45246148929999919, 1410.452081827329948, 259.9010045688979744 ) ) ;
#9545=CARTESIAN_POINT ( 'NONE',  ( -23.67770893750000027, 1410.915352782729997, 207.0119029875280035 ) ) ;
#9546=CARTESIAN_POINT ( 'NONE',  ( -10.66999429222479989, 1425.355950166579987, 113.0095011697890044 ) ) ;
#9547=CARTESIAN_POINT ( 'NONE',  ( 16.16924758266979723, 1409.477698513250061, 193.1979172417030099 ) ) ;
#9549=CARTESIAN_POINT ( 'NONE',  ( 18.38538203976483487, 1509.674347933654644, 185.4157845068922086 ) ) ;
#9550=CARTESIAN_POINT ( 'NONE',  ( -18.64672481370000057, 1416.851343898729965, 208.5597484337050105 ) ) ;
#9551=CARTESIAN_POINT ( 'NONE',  ( -21.01921848810000171, 1409.015076449529943, 267.0603558840980440 ) ) ;
#9553=CARTESIAN_POINT ( 'NONE',  ( 40.26002446930366574, 1457.179217869769673, 269.7777131889765769 ) ) ;
#9555=CARTESIAN_POINT ( 'NONE',  ( -39.08845109511560878, 1439.842738404589909, 136.7133373061289774 ) ) ;
#9556=EDGE_LOOP ( 'NONE', ( #60132, #58744, #68346, #47480, #38210 ) ) ;
#9557=CARTESIAN_POINT ( 'NONE',  ( 7.598730086320700572, 1396.178413889069816, 217.5432070791739818 ) ) ;
#9559=CARTESIAN_POINT ( 'NONE',  ( -16.77882483980000217, 1459.813925007329772, 228.5196583047979857 ) ) ;
#9560=EDGE_LOOP ( 'NONE', ( #91036, #35192, #42344 ) ) ;
#9561=ORIENTED_EDGE ( 'NONE', *, *, #6246, .T. ) ;
#9562=CARTESIAN_POINT ( 'NONE',  ( -29.33944776771571483, 1509.939423613863028, 211.5188534573150321 ) ) ;
#9563=CARTESIAN_POINT ( 'NONE',  ( -6.384249706610589215, 1425.832386075969907, 153.2928965425799959 ) ) ;
#9566=B_SPLINE_CURVE_WITH_KNOTS ( 'NONE', 5,
 ( #62670, #26813, #10013, #28477, #53140, #2200, #61001, #11137, #62105 ),
 .UNSPECIFIED., .F., .F.,
 ( 6, 3, 6 ),
 ( 0.000000000000000000, 0.5000000000000000000, 1.000000000000000000 ),
 .UNSPECIFIED. ) ;
#9577=VERTEX_POINT ( 'NONE', #37387 ) ;
#9580=ORIENTED_EDGE ( 'NONE', *, *, #46851, .T. ) ;
#9581=CARTESIAN_POINT ( 'NONE',  ( -1.441435334883619968, 1455.080613134490022, 183.7350912049300007 ) ) ;
#9582=ADVANCED_FACE ( 'NONE', ( #63718 ), #47130, .T. ) ;
#9586=CARTESIAN_POINT ( 'NONE',  ( -6.449257186580000578, 1423.216257312029938, 186.7332274999980086 ) ) ;
#9587=CARTESIAN_POINT ( 'NONE',  ( 2.245205672760550275, 1410.074017455439844, 269.8657980300729946 ) ) ;
#9590=CARTESIAN_POINT ( 'NONE',  ( 5.839375649711069372, 1441.004146644160073, 154.6877193062889830 ) ) ;
#9592=AXIS2_PLACEMENT_3D ( 'NONE', #30355, #99753, #48285 ) ;
#9593=CARTESIAN_POINT ( 'NONE',  ( 0.03068904745159911282, 1410.176690693337150, 233.2117524165238081 ) ) ;
#9594=CARTESIAN_POINT ( 'NONE',  ( 17.69067153579999996, 1458.123849909530009, 230.3917265491979833 ) ) ;
#9596=CARTESIAN_POINT ( 'NONE',  ( -4.452653756150430020, 1423.820617467126112, 184.3121917427432663 ) ) ;
#9597=CARTESIAN_POINT ( 'NONE',  ( 17.82218026611110062, 1417.888996552500203, 225.0117082750950033 ) ) ;
#9598=CARTESIAN_POINT ( 'NONE',  ( -2.499952405548359735, 1420.058982578270161, 97.99576999742468786 ) ) ;
#9600=CARTESIAN_POINT ( 'NONE',  ( 18.13455101590619734, 1424.499683988459992, 223.9684704944369855 ) ) ;
#9602=CARTESIAN_POINT ( 'NONE',  ( -3.030506966135566582, 1485.909268244792202, 182.3458070157814745 ) ) ;
#9605=ORIENTED_EDGE ( 'NONE', *, *, #32338, .F. ) ;
#9606=CARTESIAN_POINT ( 'NONE',  ( 17.11050544153610176, 1414.913527275050001, 210.6493517936639819 ) ) ;
#9607=CARTESIAN_POINT ( 'NONE',  ( -24.49494333239999833, 1443.910508108940121, 210.9673953710880028 ) ) ;
#9608=CARTESIAN_POINT ( 'NONE',  ( -10.89448555409999919, 1427.255301856029973, 149.7563259081979936 ) ) ;
#9611=DIRECTION ( 'NONE',  ( 0.4794255386042041711, 0.000000000000000000, 0.8775825618903720926 ) ) ;
#9612=CARTESIAN_POINT ( 'NONE',  ( 3.512785867830420180E-12, 1395.913060387330006, 198.1220674046479928 ) ) ;
#9615=CARTESIAN_POINT ( 'NONE',  ( 16.73302193210000155, 1412.751708530930046, 226.5522076595979968 ) ) ;
#9618=CARTESIAN_POINT ( 'NONE',  ( -16.12484297499999997, 1459.082000229730056, 229.9878769759980059 ) ) ;
#9620=CARTESIAN_POINT ( 'NONE',  ( 30.24521524950000284, 1414.226558136529775, 268.0936365245980255 ) ) ;
#9621=B_SPLINE_CURVE_WITH_KNOTS ( 'NONE', 4,
 ( #71813, #77555, #51239, #20243, #54444 ),
 .UNSPECIFIED., .F., .F.,
 ( 5, 5 ),
 ( 3.613988937050000239, 5.260361675040000407 ),
 .UNSPECIFIED. ) ;
#9622=CARTESIAN_POINT ( 'NONE',  ( 19.69322412969999903, 1430.301618381130083, 194.7952341051980056 ) ) ;
#9623=CARTESIAN_POINT ( 'NONE',  ( -23.25337057739999835, 1434.173748762760169, 214.1890449410079782 ) ) ;
#9624=CARTESIAN_POINT ( 'NONE',  ( 8.167113615893089928, 1506.588258981613308, 229.6708076605581823 ) ) ;
#9627=CYLINDRICAL_SURFACE ( 'NONE', #49757, 2.000000000000001776 ) ;
#9629=CARTESIAN_POINT ( 'NONE',  ( -13.81487708659999925, 1442.792748204340114, 188.4458667950979986 ) ) ;
#9631=CARTESIAN_POINT ( 'NONE',  ( -30.20925072189999838, 1435.551608164450045, 135.6183629175980059 ) ) ;
#9635=CARTESIAN_POINT ( 'NONE',  ( -14.89768408183259929, 1409.433298979099845, 208.1358299322530172 ) ) ;
#9638=CARTESIAN_POINT ( 'NONE',  ( -23.72712553860000284, 1471.175367018230190, 267.6119644152980186 ) ) ;
#9640=CARTESIAN_POINT ( 'NONE',  ( 0.1617910656812470149, 1420.267555168729814, 183.6005827977619731 ) ) ;
#9641=CARTESIAN_POINT ( 'NONE',  ( -24.34146701290755033, 1444.633454629505877, 211.2257049224041054 ) ) ;
#9644=CARTESIAN_POINT ( 'NONE',  ( 17.03853110007430161, 1423.468938760780247, 227.1882557915390066 ) ) ;
#9645=CARTESIAN_POINT ( 'NONE',  ( 11.73070209459999802, 1414.913060387329779, 220.5399151727980041 ) ) ;
#9646=CARTESIAN_POINT ( 'NONE',  ( 14.24758728489999982, 1463.294432896430180, 223.4356431231979911 ) ) ;
#9650=CARTESIAN_POINT ( 'NONE',  ( -3.549614846889999953, 1507.276796483229873, 180.9705030601980127 ) ) ;
#9652=CARTESIAN_POINT ( 'NONE',  ( -23.44454018040000065, 1410.653275362629984, 206.2180064241879904 ) ) ;
#9653=EDGE_CURVE ( 'NONE', #103213, #52345, #90033, .T. ) ;
#9655=CARTESIAN_POINT ( 'NONE',  ( 15.42960845380000023, 1414.913060387329779, 204.2857382735780050 ) ) ;
#9658=EDGE_CURVE ( 'NONE', #86873, #91513, #59333, .T. ) ;
#9671=EDGE_CURVE ( 'NONE', #60117, #40901, #8520, .T. ) ;
#9674=CARTESIAN_POINT ( 'NONE',  ( -5.960248613831936382, 1398.090355469260885, 220.6805375304444965 ) ) ;
#9675=CARTESIAN_POINT ( 'NONE',  ( -3.827178453834580552, 1440.905424146408222, 156.3821726451605514 ) ) ;
#9680=VECTOR ( 'NONE', #109241, 1000.000000000000000 ) ;
#9683=ORIENTED_EDGE ( 'NONE', *, *, #47980, .F. ) ;
#9684=CARTESIAN_POINT ( 'NONE',  ( 11.62114210317369967, 1433.932828604870110, 151.1840183943909892 ) ) ;
#9686=ORIENTED_EDGE ( 'NONE', *, *, #102204, .T. ) ;
#9691=CARTESIAN_POINT ( 'NONE',  ( 6.984406781949999754, 1427.831049039629988, 123.0297916884979941 ) ) ;
#9692=CARTESIAN_POINT ( 'NONE',  ( 17.44907805046609894, 1488.410848430800115, 229.8778797731829968 ) ) ;
#9694=CARTESIAN_POINT ( 'NONE',  ( 1.654058768690000125, 1488.174163428330075, 181.9749823065980081 ) ) ;
#9695=CARTESIAN_POINT ( 'NONE',  ( -5.332221971070000066, 1416.518532928429977, 191.7600702370979775 ) ) ;
#9696=CARTESIAN_POINT ( 'NONE',  ( -24.16428115052429959, 1444.791601846139883, 211.5724956969189918 ) ) ;
#9700=CARTESIAN_POINT ( 'NONE',  ( 37.28324835979699969, 1436.551445510500116, 134.0999999968369991 ) ) ;
#9703=ORIENTED_EDGE ( 'NONE', *, *, #110394, .T. ) ;
#9704=CARTESIAN_POINT ( 'NONE',  ( 14.13658382577439987, 1436.257447983569818, 150.1576428853639982 ) ) ;
#9705=CARTESIAN_POINT ( 'NONE',  ( -0.5620977654635980203, 1416.851343899799986, 227.7685710128770040 ) ) ;
#9707=EDGE_CURVE ( 'NONE', #85866, #47741, #21782, .T. ) ;
#9714=EDGE_CURVE ( 'NONE', #1439, #99476, #28568, .T. ) ;
#9715=CARTESIAN_POINT ( 'NONE',  ( -19.09068663893856055, 1441.686046601835869, 210.1346042266184782 ) ) ;
#9718=CARTESIAN_POINT ( 'NONE',  ( 0.9826203254349998861, 1507.899765146830077, 237.3510063151980205 ) ) ;
#9721=B_SPLINE_CURVE_WITH_KNOTS ( 'NONE', 3,
 ( #53192, #29083, #87334, #10630, #63267, #17889, #86218, #43678, #69453, #88975 ),
 .UNSPECIFIED., .F., .F.,
 ( 4, 2, 2, 2, 4 ),
 ( -1.402821835648833217E-05, 0.0002466997669630880004, 0.0005074277522826644042, 0.0007681557376022407537, 0.001028883722921816995 ),
 .UNSPECIFIED. ) ;
#9723=CARTESIAN_POINT ( 'NONE',  ( 20.81437694473750000, 1440.913060387330006, 221.3077511967070166 ) ) ;
#9724=CARTESIAN_POINT ( 'NONE',  ( -19.11260742820000047, 1509.007777199430166, 230.1654993297979956 ) ) ;
#9727=CARTESIAN_POINT ( 'NONE',  ( -14.73086949309999838, 1409.427473685330142, 191.7357518190979988 ) ) ;
#9728=CARTESIAN_POINT ( 'NONE',  ( -24.34449756709999946, 1441.851259293030125, 211.7501733141479860 ) ) ;
#9730=VERTEX_POINT ( 'NONE', #23865 ) ;
#9732=CARTESIAN_POINT ( 'NONE',  ( -12.00019380695538018, 1433.679412593930692, 147.5877376356537809 ) ) ;
#9737=B_SPLINE_SURFACE_WITH_KNOTS ( 'NONE', 5, 1, ( 
 ( #98764, #71963 ),
 ( #19849, #79787 ),
 ( #20393, #107167 ),
 ( #97124, #55693 ),
 ( #12563, #3643 ),
 ( #36667, #54597 ) ),
 .UNSPECIFIED., .F., .F., .F.,
 ( 6, 6 ),
 ( 2, 2 ),
 ( 0.000000000000000000, 11.48860674278019900 ),
 ( -1.500000000000000000, 1.500000000000000000 ),
 .UNSPECIFIED. ) ;
#9739=CARTESIAN_POINT ( 'NONE',  ( 23.54053115110000149, 1409.992431845630108, 209.4961337924339944 ) ) ;
#9740=CARTESIAN_POINT ( 'NONE',  ( -20.47737311789999737, 1507.835268392529997, 189.6592733436979756 ) ) ;
#9741=CARTESIAN_POINT ( 'NONE',  ( 28.04656794799999986, 1508.051246012029878, 208.1255033510109911 ) ) ;
#9747=ORIENTED_EDGE ( 'NONE', *, *, #74069, .F. ) ;
#9748=CARTESIAN_POINT ( 'NONE',  ( 35.25153999819999484, 1460.998002025230107, 264.2530495828980293 ) ) ;
#9751=CARTESIAN_POINT ( 'NONE',  ( -6.840494606030000035, 1507.559926465930175, 235.7307567964980137 ) ) ;
#9752=CARTESIAN_POINT ( 'NONE',  ( -19.24704176450000048, 1456.292361409630075, 227.8736337451979921 ) ) ;
#9753=CIRCLE ( 'NONE', #50926, 1.999999609710441106 ) ;
#9755=CARTESIAN_POINT ( 'NONE',  ( 11.86923165449999829, 1432.580340585790054, 150.3965903347979918 ) ) ;
#9756=CARTESIAN_POINT ( 'NONE',  ( 17.99954443082109989, 1410.904693892220166, 222.9872220945560173 ) ) ;
#9761=CARTESIAN_POINT ( 'NONE',  ( 0.3391062976460000322, 1405.843521269830035, 267.2349199626979726 ) ) ;
#9765=CARTESIAN_POINT ( 'NONE',  ( -4.986743168611350200E-06, 1473.589451234700164, 270.3925711489580408 ) ) ;
#9768=CARTESIAN_POINT ( 'NONE',  ( -20.13259443705889851, 1508.866006816849904, 188.8141325411800153 ) ) ;
#9769=CARTESIAN_POINT ( 'NONE',  ( -38.50736833418749683, 1440.913060392829948, 257.0794435389950081 ) ) ;
#9772=CARTESIAN_POINT ( 'NONE',  ( -0.5718103630240639612, 1450.893092329450155, 154.2421351031399865 ) ) ;
#9776=DIRECTION ( 'NONE',  ( 2.775557561562887961E-17, -0.7071067811865475727, -0.7071067811865475727 ) ) ;
#9779=CARTESIAN_POINT ( 'NONE',  ( 2.500000195207620290, 1448.894380947069976, 182.3534016008459844 ) ) ;
#9781=CARTESIAN_POINT ( 'NONE',  ( 2.500000000000000000, 1425.929641634319978, 183.3886485707629959 ) ) ;
#9783=CARTESIAN_POINT ( 'NONE',  ( -26.02647937380000087, 1444.708500955269983, 212.3004752285879988 ) ) ;
#9784=CARTESIAN_POINT ( 'NONE',  ( -0.5400825333060000899, 1417.004123502529865, 234.1403136323979766 ) ) ;
#9786=CARTESIAN_POINT ( 'NONE',  ( -29.39269380490000216, 1509.939475872329922, 211.4205234510380080 ) ) ;
#9789=CARTESIAN_POINT ( 'NONE',  ( -17.54299231450000107, 1415.063410489729904, 207.9622084005079898 ) ) ;
#9791=CARTESIAN_POINT ( 'NONE',  ( 18.91040668671516300, 1416.839570625551914, 209.9480928164305453 ) ) ;
#9793=CARTESIAN_POINT ( 'NONE',  ( -9.302637435961308654, 1396.237915646910096, 203.1362697860550099 ) ) ;
#9794=ORIENTED_EDGE ( 'NONE', *, *, #102136, .F. ) ;
#9796=CARTESIAN_POINT ( 'NONE',  ( -16.62504627205539975, 1409.593993787780164, 225.4105808336230155 ) ) ;
#9798=CARTESIAN_POINT ( 'NONE',  ( 9.804877192300001099, 1442.756953654919926, 148.8379299677979759 ) ) ;
#9799=VERTEX_POINT ( 'NONE', #2452 ) ;
#9806=CARTESIAN_POINT ( 'NONE',  ( -11.85865206170000086, 1433.007128070730232, 150.2761877906980033 ) ) ;
#9808=CARTESIAN_POINT ( 'NONE',  ( -2.566714976521826230, 1420.724238763095173, 185.6155453858885664 ) ) ;
#9816=ORIENTED_EDGE ( 'NONE', *, *, #47982, .T. ) ;
#9818=DIRECTION ( 'NONE',  ( -0.9993902469148121526, -0.03489947669269360953, 0.001077449825718530298 ) ) ;
#9819=DIRECTION ( 'NONE',  ( 0.3953879427268398583, -0.03432097994341943431, 0.9178727826240195009 ) ) ;
#9820=CARTESIAN_POINT ( 'NONE',  ( -8.571939095150000286E-11, 1471.791680839530045, 269.8654495162979856 ) ) ;
#9821=CARTESIAN_POINT ( 'NONE',  ( 13.51519562106584971, 1434.954339805268546, 146.6368354188692820 ) ) ;
#9823=CARTESIAN_POINT ( 'NONE',  ( -1.368191914778909890, 1419.344528075180278, 185.2221190139939893 ) ) ;
#9826=CARTESIAN_POINT ( 'NONE',  ( 22.63948220110000165, 1410.626538726429999, 206.7101357973980100 ) ) ;
#9827=CARTESIAN_POINT ( 'NONE',  ( -2.500000000000000000, 1448.505996463670044, 160.4897366963279808 ) ) ;
#9829=CARTESIAN_POINT ( 'NONE',  ( 14.11499368570000001, 1408.887749557829920, 212.0299715937679821 ) ) ;
#9830=CARTESIAN_POINT ( 'NONE',  ( -0.7754390136715150206, 1405.775973440009921, 268.4837770662310277 ) ) ;
#9831=CARTESIAN_POINT ( 'NONE',  ( -14.00371981653700004, 1435.086289393800143, 149.1230187904150171 ) ) ;
#9833=CARTESIAN_POINT ( 'NONE',  ( -11.87502386937130083, 1433.007271227619867, 149.9804723889419904 ) ) ;
#9834=CARTESIAN_POINT ( 'NONE',  ( 13.39320068580000012, 1444.488385957100036, 187.9681878425980130 ) ) ;
#9835=B_SPLINE_SURFACE_WITH_KNOTS ( 'NONE', 5, 4, ( 
 ( #5318, #21541, #80928, #55197, #89324 ),
 ( #82013, #106668, #4226, #81454, #64150 ),
 ( #22630, #37825, #63605, #38903, #29402 ),
 ( #97722, #107779, #14258, #20992, #29957 ),
 ( #55752, #89871, #4759, #48448, #12062 ),
 ( #73085, #82586, #107225, #65244, #63070 ) ),
 .UNSPECIFIED., .F., .F., .F.,
 ( 6, 6 ),
 ( 5, 5 ),
 ( 0.000000000000000000, 111.1101480259999903 ),
 ( 25.81581217359999769, 39.03307591160000101 ),
 .UNSPECIFIED. ) ;
#9837=EDGE_LOOP ( 'NONE', ( #84872, #51705, #24866, #31398 ) ) ;
#9838=ORIENTED_EDGE ( 'NONE', *, *, #33719, .T. ) ;
#9849=CARTESIAN_POINT ( 'NONE',  ( -28.34445769270000071, 1509.155937271930043, 208.0685711019380051 ) ) ;
#9850=B_SPLINE_SURFACE_WITH_KNOTS ( 'NONE', 5, 5, ( 
 ( #89454, #20571, #54770, #46929, #12188, #32305, #22217, #90544, #81585 ),
 ( #107899, #66488, #39605, #98397, #98942, #56415, #82707, #108459, #4889 ),
 ( #74872, #14927, #47463, #39030, #13822, #13272, #5996, #23337, #73209 ),
 ( #89997, #65379, #100049, #40148, #107353, #48008, #30649, #31741, #82146 ),
 ( #64835, #65927, #99482, #5445, #57529, #91653, #49122, #6550, #74331 ),
 ( #21670, #83255, #73775, #31192, #23876, #40701, #22764, #48572, #100595 ) ),
 .UNSPECIFIED., .F., .F., .F.,
 ( 6, 6 ),
 ( 6, 3, 6 ),
 ( 44.88737144639999599, 53.51437230290000002 ),
 ( 0.000000000000000000, 1.000000000000000000, 2.000000000000000000 ),
 .UNSPECIFIED. ) ;
#9856=CARTESIAN_POINT ( 'NONE',  ( -9.205317785249999218, 1445.523818337909915, 184.6644746700980022 ) ) ;
#9857=ORIENTED_EDGE ( 'NONE', *, *, #83689, .T. ) ;
#9859=CARTESIAN_POINT ( 'NONE',  ( 28.11157287220000001, 1508.133875833430011, 210.2394161656980032 ) ) ;
#9860=CARTESIAN_POINT ( 'NONE',  ( 19.38471501534730024, 1467.100108073059801, 225.4733628320850300 ) ) ;
#9861=CARTESIAN_POINT ( 'NONE',  ( -25.59041975919999601, 1436.636834531569775, 137.1827113295979927 ) ) ;
#9870=CARTESIAN_POINT ( 'NONE',  ( 5.992819232552550446, 1405.413060387330006, 220.0916279853276762 ) ) ;
#9871=FACE_OUTER_BOUND ( 'NONE', #80006, .T. ) ;
#9873=ORIENTED_EDGE ( 'NONE', *, *, #15782, .F. ) ;
#9876=CARTESIAN_POINT ( 'NONE',  ( 11.62509077527690060, 1435.026956746350152, 151.3666508164980087 ) ) ;
#9877=CARTESIAN_POINT ( 'NONE',  ( 4.603045327887139493, 1488.403330520399777, 234.9096270858480011 ) ) ;
#9878=CARTESIAN_POINT ( 'NONE',  ( -22.95450442767450028, 1508.996452064000096, 225.0504402230399990 ) ) ;
#9879=CARTESIAN_POINT ( 'NONE',  ( -1.881591706919999885, 1409.481719852029983, 186.4035628224980030 ) ) ;
#9881=CARTESIAN_POINT ( 'NONE',  ( -0.09674472009071061196, 1420.453443083549928, 182.7061723080140041 ) ) ;
#9884=CARTESIAN_POINT ( 'NONE',  ( -2.534204888539999700, 1421.318133561829882, 184.2270942479979965 ) ) ;
#9886=CARTESIAN_POINT ( 'NONE',  ( 18.32525213847251777, 1425.583872255219831, 224.3060837807782946 ) ) ;
#9888=CARTESIAN_POINT ( 'NONE',  ( -12.86029672965840120, 1416.218865267220053, 196.5491407428460207 ) ) ;
#9889=CARTESIAN_POINT ( 'NONE',  ( -16.32510252680000207, 1490.513422153330112, 186.1369888929979766 ) ) ;
#9890=VERTEX_POINT ( 'NONE', #9705 ) ;
#9891=CARTESIAN_POINT ( 'NONE',  ( 2.632631803615880450, 1417.642869435429930, 234.7516633181379859 ) ) ;
#9893=CARTESIAN_POINT ( 'NONE',  ( -16.81223434880759982, 1414.913060387349788, 207.5743820648510223 ) ) ;
#9895=DIRECTION ( 'NONE',  ( -0.5896169998278202318, 0.8072987820615146193, 0.02490923515557254622 ) ) ;
#9899=CARTESIAN_POINT ( 'NONE',  ( -2.713767578570000172, 1447.666021099130148, 156.1534018598979969 ) ) ;
#9902=CARTESIAN_POINT ( 'NONE',  ( -9.804877192300001099, 1442.756953654919926, 148.8379299677979759 ) ) ;
#9903=CARTESIAN_POINT ( 'NONE',  ( 17.64666381520000016, 1438.546942878890150, 190.9554714633979984 ) ) ;
#9907=VERTEX_POINT ( 'NONE', #72933 ) ;
#9908=CARTESIAN_POINT ( 'NONE',  ( 1.551584912920709991, 1415.778512721559764, 190.5885286268029972 ) ) ;
#9909=CARTESIAN_POINT ( 'NONE',  ( 23.40737871429999828, 1430.466916175329970, 206.2070977998880039 ) ) ;
#9910=CARTESIAN_POINT ( 'NONE',  ( -11.90004737883514885, 1434.917734999592540, 147.6452089151140683 ) ) ;
#9913=CARTESIAN_POINT ( 'NONE',  ( 33.91369266730000476, 1450.440660192670066, 136.2454535554979884 ) ) ;
#9914=DIRECTION ( 'NONE',  ( 0.000000000000000000, 1.000000000000000000, 0.000000000000000000 ) ) ;
#9920=CARTESIAN_POINT ( 'NONE',  ( -15.31956810097295296, 1506.436298843622581, 224.8905146749963819 ) ) ;
#9921=CARTESIAN_POINT ( 'NONE',  ( -23.35503329776611636, 1410.253263646306095, 210.2532719333120781 ) ) ;
#9923=VERTEX_POINT ( 'NONE', #105992 ) ;
#9924=CARTESIAN_POINT ( 'NONE',  ( -1.547463840030000037, 1414.913060387329779, 225.9340782259980074 ) ) ;
#9927=CARTESIAN_POINT ( 'NONE',  ( 20.32615318336489807, 1509.499165376259953, 230.1903333978989963 ) ) ;
#9928=VERTEX_POINT ( 'NONE', #56123 ) ;
#9929=EDGE_LOOP ( 'NONE', ( #45291, #37348, #100870, #105757 ) ) ;
#9930=CARTESIAN_POINT ( 'NONE',  ( 18.96125632730090160, 1509.596089392960039, 231.8852599957560017 ) ) ;
#9932=CARTESIAN_POINT ( 'NONE',  ( 37.67547422206740748, 1438.363447988549979, 136.5885122490469996 ) ) ;
#9939=CARTESIAN_POINT ( 'NONE',  ( -11.44352787233476043, 1434.730410361278018, 151.4668307198162438 ) ) ;
#9940=CARTESIAN_POINT ( 'NONE',  ( -20.21110395610000054, 1486.183523693229972, 190.5939432119980097 ) ) ;
#9941=CARTESIAN_POINT ( 'NONE',  ( 1.519174826900000053, 1408.966111141229931, 186.7972504656979993 ) ) ;
#9942=CARTESIAN_POINT ( 'NONE',  ( 4.677467455710000444, 1423.717330411029934, 184.5524840891980034 ) ) ;
#9943=CARTESIAN_POINT ( 'NONE',  ( -7.492225609940000197, 1440.568648358839937, 154.1013270938980213 ) ) ;
#9947=CARTESIAN_POINT ( 'NONE',  ( 2.867004424349999752E-15, 1452.913060387330006, 152.5211338456980172 ) ) ;
#9950=CARTESIAN_POINT ( 'NONE',  ( -18.64646848361585896, 1416.843574578169637, 208.5596655484202131 ) ) ;
#9952=CARTESIAN_POINT ( 'NONE',  ( -40.91723400889999596, 1454.696300030829889, 269.9723865689980471 ) ) ;
#9953=DIRECTION ( 'NONE',  ( 0.1402804634178727861, 0.9901118076173351934, 0.000000000000000000 ) ) ;
#9954=CARTESIAN_POINT ( 'NONE',  ( 11.96661585360000046, 1440.449248668989867, 150.8629738177980073 ) ) ;
#9955=CARTESIAN_POINT ( 'NONE',  ( -14.16989796120989986, 1420.440730658529901, 227.4201728071160176 ) ) ;
#9956=CARTESIAN_POINT ( 'NONE',  ( 10.03739716579999808, 1408.913060387329779, 194.4246222393980190 ) ) ;
#9957=CARTESIAN_POINT ( 'NONE',  ( 2.845478396016010159, 1409.147963385939875, 230.8055523966380065 ) ) ;
#9959=CARTESIAN_POINT ( 'NONE',  ( -4.836546735790000717, 1417.127067430429861, 232.4758270233980113 ) ) ;
#9960=AXIS2_PLACEMENT_3D ( 'NONE', #16842, #8463, #102517 ) ;
#9964=CARTESIAN_POINT ( 'NONE',  ( -46.03694284678339699, 1438.255879967419787, 266.9758360327800233 ) ) ;
#9965=CARTESIAN_POINT ( 'NONE',  ( -3.084747516479999785, 1428.738071243629975, 185.6021225283980129 ) ) ;
#9970=DIRECTION ( 'NONE',  ( 1.000000000000000000, 0.000000000000000000, 0.000000000000000000 ) ) ;
#9971=EDGE_CURVE ( 'NONE', #98841, #36566, #1819, .T. ) ;
#9972=CARTESIAN_POINT ( 'NONE',  ( 19.26056229662549413, 1456.232671275964321, 224.9627812116155781 ) ) ;
#9975=ORIENTED_EDGE ( 'NONE', *, *, #53523, .T. ) ;
#9976=CARTESIAN_POINT ( 'NONE',  ( -13.97534115310000047, 1452.817890303329932, 195.2694346246979933 ) ) ;
#9985=CARTESIAN_POINT ( 'NONE',  ( -4.780671213366310290, 1410.433596435060053, 269.6173310763380186 ) ) ;
#9987=CARTESIAN_POINT ( 'NONE',  ( 4.696240690070100143, 1417.218906874169988, 231.8673332382849992 ) ) ;
#9988=CARTESIAN_POINT ( 'NONE',  ( -18.20496907859999780, 1430.287838494730067, 193.4343735864979976 ) ) ;
#9990=ORIENTED_EDGE ( 'NONE', *, *, #76663, .F. ) ;
#9992=CARTESIAN_POINT ( 'NONE',  ( -23.72163544602249630, 1410.855579502579985, 210.2587994297539922 ) ) ;
#9993=CARTESIAN_POINT ( 'NONE',  ( -4.229370274619999925, 1423.902571003530056, 184.2263527321979950 ) ) ;
#9994=CARTESIAN_POINT ( 'NONE',  ( 3.686304469464770861, 1424.203457939092914, 183.9872173849159083 ) ) ;
#9995=CARTESIAN_POINT ( 'NONE',  ( 2.500020115319840031, 1419.382923540379807, 144.1035841389490031 ) ) ;
#9996=CARTESIAN_POINT ( 'NONE',  ( -19.67328662190290345, 1464.359412933360090, 193.5541274441619919 ) ) ;
#9997=CARTESIAN_POINT ( 'NONE',  ( -18.41394400640000129, 1420.837661492430016, 224.8930013675980035 ) ) ;
#9998=VECTOR ( 'NONE', #104191, 1000.000000000000114 ) ;
#9999=CARTESIAN_POINT ( 'NONE',  ( 38.77362862126869913, 1459.095958665629951, 269.1610570729100118 ) ) ;
#10000=CARTESIAN_POINT ( 'NONE',  ( -5.032517913996907843, 1466.392609142821584, 234.4269938085604394 ) ) ;
#10001=CARTESIAN_POINT ( 'NONE',  ( -11.44665353847253186, 1425.798163151176823, 139.1345268192609126 ) ) ;
#10005=CARTESIAN_POINT ( 'NONE',  ( 1.483850069390550086, 1475.343092926309737, 182.4989731883329966 ) ) ;
#10006=CARTESIAN_POINT ( 'NONE',  ( 23.58069158640000040, 1410.392965674430116, 208.0807130311279991 ) ) ;
#10009=CARTESIAN_POINT ( 'NONE',  ( 25.32246794855759831, 1452.028780111509832, 135.3106647663209969 ) ) ;
#10013=CARTESIAN_POINT ( 'NONE',  ( -18.63787277242401075, 1508.244465050728877, 229.7911781032966303 ) ) ;
#10014=CARTESIAN_POINT ( 'NONE',  ( 18.33790473009999999, 1409.718233535930040, 195.1838260118980202 ) ) ;
#10016=CARTESIAN_POINT ( 'NONE',  ( 3.374891144018687505, 1439.690136908176555, 184.4234125476535269 ) ) ;
#10018=CARTESIAN_POINT ( 'NONE',  ( -21.84936520677460337, 1429.838685647439434, 218.4389703241229199 ) ) ;
#10019=CARTESIAN_POINT ( 'NONE',  ( 8.774939133739998454, 1409.219488014130093, 228.7704650873980086 ) ) ;
#10027=CARTESIAN_POINT ( 'NONE',  ( -0.2712437013090800431, 1408.932510966370273, 231.9264321468249932 ) ) ;
#10033=CARTESIAN_POINT ( 'NONE',  ( -6.509745555140000306, 1455.357238135929947, 219.6133830849979915 ) ) ;
#10035=CARTESIAN_POINT ( 'NONE',  ( 11.86680595310000008, 1433.219746834359967, 150.3047385607980004 ) ) ;
#10036=CARTESIAN_POINT ( 'NONE',  ( 20.41675352909999930, 1440.913060387330006, 219.6133834379979817 ) ) ;
#10038=B_SPLINE_CURVE_WITH_KNOTS ( 'NONE', 3,
 ( #20130, #63820, #55959, #97934, #71130, #47013, #106347, #80602, #81676, #62173, #28544, #105251, #81138, #4982, #72225, #20665, #96299, #63281, #54866, #105818, #45370, #88453, #11741, #62743, #3368, #27988, #19579, #11206, #96862, #46471, #21758, #89543, #45910, #80046, #37494, #2814, #71698, #72760, #38581, #53781, #38048, #64368, #55411 ),
 .UNSPECIFIED., .F., .F.,
 ( 4, 3, 3, 3, 3, 3, 3, 3, 3, 3, 3, 3, 3, 3, 4 ),
 ( 0.7655572723410000169, 0.9910019214004439636, 1.224379696603769885, 1.462078613819520090, 1.704827352795679873, 1.793853281190000093, 2.038466587732339796, 2.281256468177419894, 2.316155491850000026, 2.583989317132500130, 2.855920919038569927, 3.139267318828499853, 3.387490792979999554, 3.680707183893040302, 3.835724788489999426 ),
 .UNSPECIFIED. ) ;
#10041=CARTESIAN_POINT ( 'NONE',  ( -12.25055778059999945, 1486.242977004730164, 184.4831925055979980 ) ) ;
#10043=CARTESIAN_POINT ( 'NONE',  ( -21.72141783274009796, 1509.710993503089867, 231.6292274468669916 ) ) ;
#10044=CARTESIAN_POINT ( 'NONE',  ( 24.89847827690000059, 1430.363150105230034, 209.6261949212619982 ) ) ;
#10053=EDGE_LOOP ( 'NONE', ( #8259, #3877, #19761, #84650 ) ) ;
#10054=CARTESIAN_POINT ( 'NONE',  ( -1.341974385850000173, 1416.832348306829999, 228.0804724305980073 ) ) ;
#10057=CARTESIAN_POINT ( 'NONE',  ( -5.487972707081399726, 1440.608688506979888, 154.7779097410979716 ) ) ;
#10059=ORIENTED_EDGE ( 'NONE', *, *, #8351, .T. ) ;
#10063=CARTESIAN_POINT ( 'NONE',  ( -15.66638209299999929, 1416.825421876430028, 219.1964221495979928 ) ) ;
#10064=CARTESIAN_POINT ( 'NONE',  ( -1.086003861333974196, 1508.993070980561242, 238.8005286751018446 ) ) ;
#10068=CARTESIAN_POINT ( 'NONE',  ( 14.76663485449640056, 1409.428722639259831, 206.8871449305759711 ) ) ;
#10071=CARTESIAN_POINT ( 'NONE',  ( -17.63837303440000426, 1411.935330354230018, 193.4048893071979762 ) ) ;
#10079=ORIENTED_EDGE ( 'NONE', *, *, #91961, .F. ) ;
#10083=EDGE_CURVE ( 'NONE', #59101, #68673, #63773, .T. ) ;
#10084=CARTESIAN_POINT ( 'NONE',  ( 35.06721089139576719, 1457.701433636751972, 269.5324293830444731 ) ) ;
#10085=CYLINDRICAL_SURFACE ( 'NONE', #48110, 1.999999999999994449 ) ;
#10086=CARTESIAN_POINT ( 'NONE',  ( -28.25086642335310216, 1508.135711581739997, 208.8579954535609886 ) ) ;
#10096=CARTESIAN_POINT ( 'NONE',  ( 14.00875066949999947, 1416.819760216229952, 196.3921940529979793 ) ) ;
#10099=B_SPLINE_CURVE_WITH_KNOTS ( 'NONE', 3,
 ( #81766, #31922, #21842, #66661 ),
 .UNSPECIFIED., .F., .F.,
 ( 4, 4 ),
 ( -21.94916620480000091, -5.186424823540001228 ),
 .UNSPECIFIED. ) ;
#10104=CARTESIAN_POINT ( 'NONE',  ( -27.16947874219999903, 1488.689296590230015, 207.4688266076479692 ) ) ;
#10105=CARTESIAN_POINT ( 'NONE',  ( -10.45732730569119795, 1425.117602760000182, 121.9097720391450110 ) ) ;
#10106=CARTESIAN_POINT ( 'NONE',  ( 16.57702714126169852, 1410.724566313010200, 191.7206609563160100 ) ) ;
#10109=CARTESIAN_POINT ( 'NONE',  ( 12.44492264844295448, 1509.471699171668433, 181.7748644473435604 ) ) ;
#10110=CARTESIAN_POINT ( 'NONE',  ( -22.11623627239999834, 1489.468502498230009, 207.6017525449580035 ) ) ;
#10111=CARTESIAN_POINT ( 'NONE',  ( -33.66409354169999801, 1434.352089750010236, 250.0355534200980401 ) ) ;
#10112=CARTESIAN_POINT ( 'NONE',  ( 17.56822049365750260, 1509.536650904990211, 232.8514770280130222 ) ) ;
#10113=CARTESIAN_POINT ( 'NONE',  ( 28.70934402868200408, 1509.343126748570285, 209.4988959437390292 ) ) ;
#10115=CARTESIAN_POINT ( 'NONE',  ( 33.12914009259999659, 1451.756166416729911, 134.7383383604980054 ) ) ;
#10117=CARTESIAN_POINT ( 'NONE',  ( 11.14207291371160125, 1397.935304532519922, 216.8346386145179849 ) ) ;
#10120=CARTESIAN_POINT ( 'NONE',  ( -18.47628410029999912, 1457.312873679730046, 229.4267097870979910 ) ) ;
#10121=ORIENTED_EDGE ( 'NONE', *, *, #96826, .T. ) ;
#10122=VERTEX_POINT ( 'NONE', #14658 ) ;
#10123=CARTESIAN_POINT ( 'NONE',  ( -29.23325473176074851, 1509.933901906174697, 211.7644991624144097 ) ) ;
#10125=B_SPLINE_CURVE_WITH_KNOTS ( 'NONE', 5,
 ( #46570, #80149, #37041, #38140, #20771, #71799, #44926, #3470, #47108, #63387, #97502, #54971, #54431, #89097, #12385, #53318, #79073, #63921, #80705, #62853, #37597, #105918, #4014, #95849, #36495, #106452, #11309, #71235, #29735, #53889 ),
 .UNSPECIFIED., .F., .F.,
 ( 6, 3, 3, 3, 3, 3, 3, 3, 3, 6 ),
 ( 0.000000000000000000, 0.007519188799632491732, 0.01525432589305721759, 0.03846436772750950334, 0.06167440956112346662, 0.1235555043535759567, 0.2624078012577487629, 0.4012600981619215967, 0.5405650403839840079, 1.000000000000000000 ),
 .UNSPECIFIED. ) ;
#10127=CARTESIAN_POINT ( 'NONE',  ( -1.069244773279999894, 1410.308942914629824, 185.3176740583979836 ) ) ;
#10128=CARTESIAN_POINT ( 'NONE',  ( 9.484196478038136036, 1446.608455646244693, 153.5742700972787986 ) ) ;
#10129=LINE ( 'NONE', #70078, #9998 ) ;
#10130=CARTESIAN_POINT ( 'NONE',  ( -9.474342455649999550, 1470.475897465230219, 232.9250315801980094 ) ) ;
#10131=CARTESIAN_POINT ( 'NONE',  ( -12.78776258890000150, 1416.851343894929869, 195.7518694485980006 ) ) ;
#10135=ORIENTED_EDGE ( 'NONE', *, *, #78317, .T. ) ;
#10139=CARTESIAN_POINT ( 'NONE',  ( 11.86259848306839970, 1432.091341794900018, 149.9768531085499887 ) ) ;
#10140=CARTESIAN_POINT ( 'NONE',  ( 13.18251122944204390, 1444.726075940572173, 187.2757804206736978 ) ) ;
#10142=CARTESIAN_POINT ( 'NONE',  ( -15.73091603027213914, 1506.446781340835969, 193.7509379680487314 ) ) ;
#10144=CARTESIAN_POINT ( 'NONE',  ( 6.924875051240000801, 1507.862635227430019, 235.4241313661979973 ) ) ;
#10146=CARTESIAN_POINT ( 'NONE',  ( -5.151887371179999953, 1423.035654755729865, 185.3911223247979763 ) ) ;
#10147=CARTESIAN_POINT ( 'NONE',  ( 4.814684546780449992, 1410.439504313829957, 269.6173903879380305 ) ) ;
#10152=CARTESIAN_POINT ( 'NONE',  ( 0.03022822327178078736, 1410.187553064696885, 233.2131390692366892 ) ) ;
#10155=CARTESIAN_POINT ( 'NONE',  ( 15.17327376946160022, 1507.614846715330032, 226.3720743403030156 ) ) ;
#10157=CARTESIAN_POINT ( 'NONE',  ( -5.360126306917530670, 1422.242609447140012, 144.1609271584179908 ) ) ;
#10158=VERTEX_POINT ( 'NONE', #92457 ) ;
#10159=CARTESIAN_POINT ( 'NONE',  ( 11.47403709129999960, 1414.639208232530109, 262.6648722416979922 ) ) ;
#10160=DIRECTION ( 'NONE',  ( 0.000000000000000000, 1.000000000000000000, 0.000000000000000000 ) ) ;
#10165=( BOUNDED_SURFACE ( )  B_SPLINE_SURFACE ( 3, 2, ( 
 ( #91144, #82748, #37996 ),
 ( #39074, #29581, #105764 ),
 ( #64318, #72710, #55914 ),
 ( #98439, #63235, #56454 ),
 ( #97881, #54812, #55361 ),
 ( #3869, #12231, #46421 ),
 ( #21156, #29049, #72179 ),
 ( #81628, #97341, #89494 ),
 ( #90032, #12788, #88939 ),
 ( #14421, #46966, #57019 ),
 ( #106833, #81087, #4404 ),
 ( #73251, #107390, #13866 ),
 ( #30687, #22812, #64874 ),
 ( #98981, #90589, #48051 ),
 ( #82188, #5488, #73816 ),
 ( #107945, #31237, #65420 ),
 ( #99527, #92797, #108500 ),
 ( #49164, #91694, #100100 ) ),
 .UNSPECIFIED., .F., .F., .F. ) 
 B_SPLINE_SURFACE_WITH_KNOTS ( ( 4, 2, 2, 2, 2, 2, 2, 2, 4 ),
 ( 3, 3 ),
 ( -1.056814893231837992E-05, 4.513480273177641422E-05, 0.0001008377543958712084, 0.0002122436577240607966, 0.0004350554643804399732, 0.0008806790776931983263, 0.001326302691005956571, 0.001549114497662335693, 0.001771926304318715032 ),
 ( 0.000000000000000000, 1.000000000000000000 ),
 .UNSPECIFIED. ) 
 GEOMETRIC_REPRESENTATION_ITEM ( )  RATIONAL_B_SPLINE_SURFACE ( (
 ( 1.000000000000000000, 0.8674263646877330425, 1.000000000000000000),
 ( 1.000000000000000000, 0.8678218641029733504, 1.000000000000000000),
 ( 1.000000000000000000, 0.8697758742242241992, 1.000000000000000000),
 ( 1.000000000000000000, 0.8728331949133366630, 1.000000000000000000),
 ( 1.000000000000000000, 0.8743688320447627893, 1.000000000000000000),
 ( 1.000000000000000000, 0.8789934887300921984, 1.000000000000000000),
 ( 1.000000000000000000, 0.8821003874863629912, 1.000000000000000000),
 ( 1.000000000000000000, 0.8914624349615335452, 1.000000000000000000),
 ( 1.000000000000000000, 0.8977612400248787816, 1.000000000000000000),
 ( 1.000000000000000000, 0.9165107280359201525, 1.000000000000000000),
 ( 1.000000000000000000, 0.9288478704676672582, 1.000000000000000000),
 ( 1.000000000000000000, 0.9506413689712427395, 1.000000000000000000),
 ( 1.000000000000000000, 0.9600128686476009365, 1.000000000000000000),
 ( 1.000000000000000000, 0.9692757131723997999, 1.000000000000000000),
 ( 1.000000000000000000, 0.9715763504693073482, 1.000000000000000000),
 ( 1.000000000000000000, 0.9742738933835981552, 1.000000000000000000),
 ( 1.000000000000000000, 0.9746552859465718033, 1.000000000000000000),
 ( 1.000000000000000000, 0.9740159740112075415, 1.000000000000000000) ) ) 
 REPRESENTATION_ITEM ( '' )  SURFACE ( )  );
#10169=CARTESIAN_POINT ( 'NONE',  ( -24.31100006580000183, 1442.893711221979856, 212.2583796852279931 ) ) ;
#10172=CARTESIAN_POINT ( 'NONE',  ( -10.50426069749999947, 1440.655587673750006, 187.1572747102979974 ) ) ;
#10174=CARTESIAN_POINT ( 'NONE',  ( 13.15712928874680010, 1428.815432648289971, 222.5930086189890176 ) ) ;
#10176=CARTESIAN_POINT ( 'NONE',  ( 7.345502919380000328, 1415.074004183030183, 230.9439570329979858 ) ) ;
#10178=CARTESIAN_POINT ( 'NONE',  ( -16.73813953200000171, 1460.714426248530117, 228.2661735262979903 ) ) ;
#10180=CARTESIAN_POINT ( 'NONE',  ( 31.73325210529999296, 1415.263605584930247, 267.4236301385980710 ) ) ;
#10182=CARTESIAN_POINT ( 'NONE',  ( 37.66849513895419932, 1445.052233489950140, 137.0436250799990034 ) ) ;
#10184=CARTESIAN_POINT ( 'NONE',  ( 25.82017203379999870, 1508.004933221630154, 200.5938135955979931 ) ) ;
#10185=CARTESIAN_POINT ( 'NONE',  ( -22.99624282800000330, 1433.297116904619998, 215.2097649112580200 ) ) ;
#10188=CARTESIAN_POINT ( 'NONE',  ( -1.433829655579999862, 1450.688199285750215, 182.8043069899979969 ) ) ;
#10191=B_SPLINE_CURVE_WITH_KNOTS ( 'NONE', 5,
 ( #48136, #107465, #11764, #47039, #29118, #90108, #5573, #73330, #97958, #89013, #81702, #30202, #13391, #47578, #81163, #4478, #30761, #3390, #31311, #56535, #38608 ),
 .UNSPECIFIED., .F., .F.,
 ( 6, 3, 3, 3, 3, 3, 6 ),
 ( 0.000000000000000000, 0.4999938077254366120, 0.6403281941878481431, 0.8201641551007432529, 0.9100821355580290817, 0.9550411257862527759, 1.000000000000000000 ),
 .UNSPECIFIED. ) ;
#10192=CARTESIAN_POINT ( 'NONE',  ( -13.11337116420000015, 1442.804475998300177, 187.4630894580980112 ) ) ;
#10195=FACE_OUTER_BOUND ( 'NONE', #61696, .T. ) ;
#10196=VERTEX_POINT ( 'NONE', #39870 ) ;
#10198=CARTESIAN_POINT ( 'NONE',  ( -14.09333513740220134, 1409.405210495020128, 204.1816249279730187 ) ) ;
#10200=CARTESIAN_POINT ( 'NONE',  ( -33.05470698740527524, 1442.773887286368563, 154.3540262795430067 ) ) ;
#10202=CARTESIAN_POINT ( 'NONE',  ( -42.11994550690000239, 1455.888674964030088, 268.8741266023980074 ) ) ;
#10205=CARTESIAN_POINT ( 'NONE',  ( -24.06692873656430010, 1444.368885470432588, 212.0869959726532272 ) ) ;
#10209=CARTESIAN_POINT ( 'NONE',  ( 13.00742463789999981, 1414.913060387329779, 218.5570036086780021 ) ) ;
#10210=CARTESIAN_POINT ( 'NONE',  ( -28.29378357199729876, 1508.482245365549943, 208.8393840306729885 ) ) ;
#10211=CARTESIAN_POINT ( 'NONE',  ( -27.24430363784859921, 1507.989586464290142, 211.0156678195309894 ) ) ;
#10213=CARTESIAN_POINT ( 'NONE',  ( -7.789308819770000447, 1507.432058219530063, 181.7020214070979875 ) ) ;
#10214=CARTESIAN_POINT ( 'NONE',  ( -23.00682135910000170, 1409.716476292929883, 208.3124398812599907 ) ) ;
#10215=CARTESIAN_POINT ( 'NONE',  ( 16.30669509790000049, 1415.087745006229852, 204.0605247263480067 ) ) ;
#10218=CARTESIAN_POINT ( 'NONE',  ( -11.93818408299999945, 1433.480074519959999, 149.8972116839979947 ) ) ;
#10222=CARTESIAN_POINT ( 'NONE',  ( -22.38213066169999976, 1410.189388595030096, 211.7294389034280186 ) ) ;
#10227=CARTESIAN_POINT ( 'NONE',  ( -23.58466550250000182, 1425.864548988530032, 211.0897696391780016 ) ) ;
#10232=CARTESIAN_POINT ( 'NONE',  ( -14.59646112059999901, 1484.617543311429927, 186.9027180520979812 ) ) ;
#10233=CARTESIAN_POINT ( 'NONE',  ( 1.591349661450000008, 1508.276900102130185, 237.0058671888980086 ) ) ;
#10235=CARTESIAN_POINT ( 'NONE',  ( 40.01268977396789950, 1445.988963729020043, 136.7986924672030113 ) ) ;
#10238=ORIENTED_EDGE ( 'NONE', *, *, #63890, .F. ) ;
#10239=ORIENTED_EDGE ( 'NONE', *, *, #48250, .F. ) ;
#10240=CARTESIAN_POINT ( 'NONE',  ( 11.84597236525540076, 1433.773622760579883, 150.7447557071740221 ) ) ;
#10245=CARTESIAN_POINT ( 'NONE',  ( 16.84159957015370068, 1450.438998685270235, 190.2947511461639749 ) ) ;
#10248=CARTESIAN_POINT ( 'NONE',  ( 7.252303098479999655, 1488.166944670630073, 183.5694544787980078 ) ) ;
#10250=CARTESIAN_POINT ( 'NONE',  ( 4.363122647530000009, 1423.854802298929826, 179.4243885131980107 ) ) ;
#10252=CARTESIAN_POINT ( 'NONE',  ( 14.32414760831999878, 1416.073666499230058, 196.9890948053629813 ) ) ;
#10256=CARTESIAN_POINT ( 'NONE',  ( 14.17148602175130101, 1435.193163544880008, 149.2585390295329830 ) ) ;
#10261=CARTESIAN_POINT ( 'NONE',  ( -2.763419390480000182, 1466.129840014930096, 235.1610046648980017 ) ) ;
#10268=CARTESIAN_POINT ( 'NONE',  ( 4.259522660623400014, 1446.576511802210007, 159.6066588128159935 ) ) ;
#10269=CARTESIAN_POINT ( 'NONE',  ( 0.5005539547930000221, 1508.988185698529833, 238.8806144467979777 ) ) ;
#10270=VERTEX_POINT ( 'NONE', #6802 ) ;
#10273=CARTESIAN_POINT ( 'NONE',  ( 31.61825852761390010, 1440.913060387330006, 255.2595036761919971 ) ) ;
#10274=CARTESIAN_POINT ( 'NONE',  ( -15.56111295170000020, 1509.395558335530040, 184.1751395816980050 ) ) ;
#10276=CARTESIAN_POINT ( 'NONE',  ( 25.24523437353879984, 1450.837001535949867, 137.6108059648960023 ) ) ;
#10277=CARTESIAN_POINT ( 'NONE',  ( -14.62683816560000061, 1410.356143933229987, 190.5625663710980007 ) ) ;
#10278=CARTESIAN_POINT ( 'NONE',  ( -24.37050012060000270, 1442.224872846740027, 212.1537385428579796 ) ) ;
#10280=CARTESIAN_POINT ( 'NONE',  ( 0.0002634086548581413153, 1396.454024644930314, 196.7541624207434552 ) ) ;
#10281=CARTESIAN_POINT ( 'NONE',  ( 25.98561784903089844, 1441.261220175989820, 138.2899391456000160 ) ) ;
#10282=CARTESIAN_POINT ( 'NONE',  ( -13.80523795290000066, 1434.979592755129943, 149.2726119245979817 ) ) ;
#10283=CARTESIAN_POINT ( 'NONE',  ( 17.95374924460000088, 1435.124687891739995, 145.3138471459980110 ) ) ;
#10290=CARTESIAN_POINT ( 'NONE',  ( -17.22592475670000312, 1443.913060387330006, 162.9227486557980171 ) ) ;
#10291=EDGE_CURVE ( 'NONE', #28591, #43475, #83402, .T. ) ;
#10297=ORIENTED_EDGE ( 'NONE', *, *, #49035, .F. ) ;
#10299=CARTESIAN_POINT ( 'NONE',  ( 14.70061896480000030, 1464.437658295830033, 244.5173669037980346 ) ) ;
#10302=CARTESIAN_POINT ( 'NONE',  ( -11.74015320060000001, 1428.979986575930070, 144.1938086916980239 ) ) ;
#10304=CARTESIAN_POINT ( 'NONE',  ( -5.389426750931309407, 1508.548281180689855, 236.7560892007110169 ) ) ;
#10305=CARTESIAN_POINT ( 'NONE',  ( -22.44033291929999763, 1451.339077370430005, 219.6664876968980025 ) ) ;
#10308=CARTESIAN_POINT ( 'NONE',  ( 17.70873813924769991, 1409.985199876030038, 222.7474336651429780 ) ) ;
#10309=CARTESIAN_POINT ( 'NONE',  ( 0.1710941751449999992, 1506.802866779329861, 186.9387561868979901 ) ) ;
#10314=CARTESIAN_POINT ( 'NONE',  ( 27.74496033939999862, 1507.996570538830156, 207.7306165369780047 ) ) ;
#10315=CARTESIAN_POINT ( 'NONE',  ( 13.17363969167560178, 1472.364508107560141, 270.4167824513199889 ) ) ;
#10316=CARTESIAN_POINT ( 'NONE',  ( 22.52609212299890018, 1509.699688857919909, 227.3081665486540146 ) ) ;
#10317=EDGE_CURVE ( 'NONE', #94490, #64525, #92348, .T. ) ;
#10321=CARTESIAN_POINT ( 'NONE',  ( 35.72414125057429857, 1450.114973065470167, 136.2375792952020106 ) ) ;
#10328=ORIENTED_EDGE ( 'NONE', *, *, #55141, .F. ) ;
#10329=CARTESIAN_POINT ( 'NONE',  ( -20.14739811709999984, 1412.328483943929996, 271.1218459616979999 ) ) ;
#10330=ADVANCED_FACE ( 'NONE', ( #91916 ), #30119, .F. ) ;
#10331=CARTESIAN_POINT ( 'NONE',  ( -0.8073792788704451384, 1450.884866113202406, 181.3631603842342486 ) ) ;
#10333=CARTESIAN_POINT ( 'NONE',  ( -0.4667605481589999772, 1416.135518339629925, 233.5066626509980097 ) ) ;
#10338=CARTESIAN_POINT ( 'NONE',  ( -18.63578313170000200, 1416.568813547830132, 208.5538819738139864 ) ) ;
#10339=CARTESIAN_POINT ( 'NONE',  ( 11.87158682754100170, 1432.747848164100105, 149.9813451862029865 ) ) ;
#10340=CARTESIAN_POINT ( 'NONE',  ( 26.16070222434640158, 1436.533894928910058, 136.8495626736880126 ) ) ;
#10341=CARTESIAN_POINT ( 'NONE',  ( -8.061180465434720332, 1396.194563012580147, 201.5581022159940119 ) ) ;
#10345=CARTESIAN_POINT ( 'NONE',  ( -17.19883865694049874, 1410.595981660250118, 225.9965367844259845 ) ) ;
#10346=CARTESIAN_POINT ( 'NONE',  ( 2.493947715939999643, 1442.756953654919926, 150.6345094620980092 ) ) ;
#10347=EDGE_LOOP ( 'NONE', ( #30085, #63176, #104924, #82385 ) ) ;
#10349=PLANE ( 'NONE',  #47502 ) ;
#10352=DIRECTION ( 'NONE',  ( 0.03234404824097146525, -0.9989938922171894831, -0.03106550910795196491 ) ) ;
#10353=CARTESIAN_POINT ( 'NONE',  ( 1.448679645196929933, 1507.129709964000085, 181.1126013477120011 ) ) ;
#10354=B_SPLINE_CURVE_WITH_KNOTS ( 'NONE', 5,
 ( #56953, #14364, #82694, #40132, #108445, #100030 ),
 .UNSPECIFIED., .F., .F.,
 ( 6, 6 ),
 ( -105.4335682549999973, -86.05908199089999755 ),
 .UNSPECIFIED. ) ;
#10356=CIRCLE ( 'NONE', #40808, 1.999999999999998224 ) ;
#10361=CARTESIAN_POINT ( 'NONE',  ( 2.500000876580000142, 1448.997560968779908, 182.3441048618979892 ) ) ;
#10363=CARTESIAN_POINT ( 'NONE',  ( -8.808667343012501760, 1463.337573556750840, 235.3868218242529906 ) ) ;
#10364=ORIENTED_EDGE ( 'NONE', *, *, #29516, .T. ) ;
#10366=CARTESIAN_POINT ( 'NONE',  ( -40.70526361830000184, 1444.199272583730135, 137.0833898022980009 ) ) ;
#10367=CARTESIAN_POINT ( 'NONE',  ( 1.442233445782429957, 1490.976481901869874, 236.0750500844659996 ) ) ;
#10368=CARTESIAN_POINT ( 'NONE',  ( -1.454166803559999943, 1473.250322698830132, 270.4288814092980147 ) ) ;
#10370=CARTESIAN_POINT ( 'NONE',  ( -0.5747759660569999873, 1486.512367523630019, 181.7356503477979857 ) ) ;
#10373=CARTESIAN_POINT ( 'NONE',  ( 22.53878436229999949, 1411.058442725530085, 206.1986151520480064 ) ) ;
#10375=CARTESIAN_POINT ( 'NONE',  ( -2.500000000000000000, 1448.758219214420023, 157.1656513902149754 ) ) ;
#10376=CARTESIAN_POINT ( 'NONE',  ( -13.04464049575494045, 1434.926819199586134, 149.8863372439509760 ) ) ;
#10377=CARTESIAN_POINT ( 'NONE',  ( 15.38805437926849784, 1409.450423087220088, 203.9135902043169892 ) ) ;
#10378=CARTESIAN_POINT ( 'NONE',  ( 5.717839861821480532E-05, 1405.749489006759859, 267.5370922816329653 ) ) ;
#10379=CARTESIAN_POINT ( 'NONE',  ( -13.85777447298269927, 1434.981442650969939, 148.6210011382069922 ) ) ;
#10381=CARTESIAN_POINT ( 'NONE',  ( 3.585180483099999815, 1424.862442824429991, 185.0085506464979801 ) ) ;
#10382=CARTESIAN_POINT ( 'NONE',  ( 13.42038842620000061, 1444.421388250450264, 187.7727034152979968 ) ) ;
#10384=AXIS2_PLACEMENT_3D ( 'NONE', #14433, #32892, #16081 ) ;
#10385=ORIENTED_EDGE ( 'NONE', *, *, #71431, .T. ) ;
#10386=EDGE_CURVE ( 'NONE', #44146, #86029, #84680, .T. ) ;
#10390=EDGE_CURVE ( 'NONE', #24504, #34701, #106666, .T. ) ;
#10393=B_SPLINE_SURFACE_WITH_KNOTS ( 'NONE', 3, 5, ( 
 ( #72844, #14008, #22952, #107529, #21292, #15104 ),
 ( #64457, #99661, #99113, #39217, #73393, #48753 ),
 ( #81765, #57710, #108074, #4535, #38669, #6169 ),
 ( #98572, #91282, #56590, #14563, #100237, #63905 ) ),
 .UNSPECIFIED., .F., .F., .F.,
 ( 4, 4 ),
 ( 6, 6 ),
 ( 5.479556543930000245, 5.505627295709999203 ),
 ( 0.000000000000000000, 1.000000000000000000 ),
 .UNSPECIFIED. ) ;
#10401=CARTESIAN_POINT ( 'NONE',  ( -28.07231162100000077, 1508.101920006030241, 207.7749232119980149 ) ) ;
#10407=CARTESIAN_POINT ( 'NONE',  ( -6.316132940400000173, 1409.300553759430159, 230.7650132070980078 ) ) ;
#10408=CARTESIAN_POINT ( 'NONE',  ( -7.322107218450000232, 1446.343164073429989, 185.2693503152979986 ) ) ;
#10410=CARTESIAN_POINT ( 'NONE',  ( -27.68994704303559828, 1508.175463917300021, 210.5782600342069770 ) ) ;
#10411=CARTESIAN_POINT ( 'NONE',  ( 0.000000000000000000, 1508.913060387330006, 224.7618459619980058 ) ) ;
#10414=CARTESIAN_POINT ( 'NONE',  ( -24.94579848589999926, 1435.368615134259926, 135.7553688025980136 ) ) ;
#10418=CARTESIAN_POINT ( 'NONE',  ( 0.006240583433823138071, 1508.657668050519987, 238.1872277698262224 ) ) ;
#10420=CARTESIAN_POINT ( 'NONE',  ( -11.60004869885203682, 1424.140773631476577, 136.0101406523738490 ) ) ;
#10423=ORIENTED_EDGE ( 'NONE', *, *, #56955, .T. ) ;
#10424=CARTESIAN_POINT ( 'NONE',  ( 2.500000000000000000, 1439.114301455650093, 157.7261946041980138 ) ) ;
#10425=CARTESIAN_POINT ( 'NONE',  ( -6.492126169470000541, 1412.832739453629983, 231.4048330429980069 ) ) ;
#10428=VERTEX_POINT ( 'NONE', #62775 ) ;
#10431=CARTESIAN_POINT ( 'NONE',  ( 11.76920103414339991, 1434.891807205950045, 151.2471915141129841 ) ) ;
#10432=CARTESIAN_POINT ( 'NONE',  ( 8.124014794800109129, 1488.402311747539898, 234.1398025081960270 ) ) ;
#10436=CARTESIAN_POINT ( 'NONE',  ( -0.07532719850957350638, 1420.449570258260110, 182.6937329275319826 ) ) ;
#10439=CARTESIAN_POINT ( 'NONE',  ( -3.185236608319999885, 1421.319945421930015, 185.4942751512979839 ) ) ;
#10440=CARTESIAN_POINT ( 'NONE',  ( 18.63864990469999938, 1509.044553701730138, 187.9652674623980033 ) ) ;
#10444=CARTESIAN_POINT ( 'NONE',  ( -19.88572122277579979, 1484.728771715989751, 191.0592865161910083 ) ) ;
#10445=ORIENTED_EDGE ( 'NONE', *, *, #95112, .T. ) ;
#10446=CARTESIAN_POINT ( 'NONE',  ( 4.015231150059999088, 1421.847071512329876, 183.7162519361979776 ) ) ;
#10447=ADVANCED_FACE ( 'NONE', ( #81711 ), #49884, .F. ) ;
#10452=CARTESIAN_POINT ( 'NONE',  ( -18.05542497264810109, 1416.825784014559986, 209.4840452940109969 ) ) ;
#10453=CARTESIAN_POINT ( 'NONE',  ( -4.293785995879999540, 1447.009251615389985, 154.3906955766980218 ) ) ;
#10454=CARTESIAN_POINT ( 'NONE',  ( -18.55308284270000030, 1424.846930163729894, 224.9900042346980058 ) ) ;
#10455=CARTESIAN_POINT ( 'NONE',  ( -14.59275605859999914, 1436.244805951940180, 149.8708530261979774 ) ) ;
#10456=CARTESIAN_POINT ( 'NONE',  ( -0.5919877880829009786, 1487.510302489449941, 230.8834977925120029 ) ) ;
#10458=CARTESIAN_POINT ( 'NONE',  ( 0.5679639878839999323, 1416.568813547830132, 190.4860628299979908 ) ) ;
#10459=CARTESIAN_POINT ( 'NONE',  ( -19.08015071520780737, 1440.747599611412397, 209.7861252745999252 ) ) ;
#10460=CARTESIAN_POINT ( 'NONE',  ( 0.5623041700042573643, 1416.835806650143240, 190.4756569920872664 ) ) ;
#10462=CARTESIAN_POINT ( 'NONE',  ( 1.135155432552129806, 1507.593744646030018, 186.1936170170519915 ) ) ;
#10465=CARTESIAN_POINT ( 'NONE',  ( -23.74108624850000027, 1436.296627321610003, 212.5883426267580205 ) ) ;
#10467=AXIS2_PLACEMENT_3D ( 'NONE', #91065, #31158, #65896 ) ;
#10468=CARTESIAN_POINT ( 'NONE',  ( -3.547964652322029178, 1426.008885103042758, 185.9028156952102506 ) ) ;
#10470=CARTESIAN_POINT ( 'NONE',  ( -13.70772824027479864, 1507.648153509909889, 184.2587339175119894 ) ) ;
#10473=ADVANCED_FACE ( 'NONE', ( #91231 ), #39067, .F. ) ;
#10480=DIRECTION ( 'NONE',  ( 0.000000000000000000, 0.000000000000000000, 1.000000000000000000 ) ) ;
#10482=DIRECTION ( 'NONE',  ( 0.03489949670250328678, 0.9993908270190956511, 0.000000000000000000 ) ) ;
#10484=CARTESIAN_POINT ( 'NONE',  ( 17.15874754026939897, 1507.620489270460212, 193.8380741321440155 ) ) ;
#10486=CARTESIAN_POINT ( 'NONE',  ( 20.21913194945920011, 1509.384053626160039, 230.0320258892189997 ) ) ;
#10489=CARTESIAN_POINT ( 'NONE',  ( 17.41906133238040155, 1508.769966748330035, 231.1703520980719873 ) ) ;
#10491=CARTESIAN_POINT ( 'NONE',  ( 13.01686712407386359, 1442.959643518457597, 169.4188180632390015 ) ) ;
#10492=CARTESIAN_POINT ( 'NONE',  ( 20.42904319129999635, 1470.816572149729836, 208.8910212311110115 ) ) ;
#10493=CARTESIAN_POINT ( 'NONE',  ( -6.526375087349999937, 1473.529235870629918, 262.4989463880980338 ) ) ;
#10497=DIRECTION ( 'NONE',  ( 0.7071067811860475283, 8.350994033320553495E-15, 0.7071067811870476172 ) ) ;
#10500=CARTESIAN_POINT ( 'NONE',  ( 4.738395335269999897, 1421.880050881929947, 185.2211201735979955 ) ) ;
#10501=CARTESIAN_POINT ( 'NONE',  ( -11.88948492470000140, 1437.278290821260043, 151.6406834257980165 ) ) ;
#10502=CARTESIAN_POINT ( 'NONE',  ( 11.88948418939999918, 1437.278291760409957, 151.6406840026980092 ) ) ;
#10504=CARTESIAN_POINT ( 'NONE',  ( 1.399926847669999974, 1507.072115598929940, 236.8180522793980174 ) ) ;
#10505=CARTESIAN_POINT ( 'NONE',  ( -16.18755144487676745, 1409.478342139989536, 193.2473228669673233 ) ) ;
#10509=CARTESIAN_POINT ( 'NONE',  ( -37.60287116660000351, 1456.179137436829706, 270.1614696094979990 ) ) ;
#10510=CARTESIAN_POINT ( 'NONE',  ( -23.70839420758922245, 1436.152046287332951, 211.9671219878686657 ) ) ;
#10511=CARTESIAN_POINT ( 'NONE',  ( 12.00000000000000000, 1443.913060387330006, 150.5878346084980137 ) ) ;
#10512=CARTESIAN_POINT ( 'NONE',  ( -14.17566286230000117, 1463.287831902929838, 223.4212262942980090 ) ) ;
#10514=CARTESIAN_POINT ( 'NONE',  ( 2.924457912680139771, 1409.899976016270102, 231.5199593976699930 ) ) ;
#10516=CARTESIAN_POINT ( 'NONE',  ( -6.236116630490000645, 1418.000551928829964, 232.4301535818979971 ) ) ;
#10519=CARTESIAN_POINT ( 'NONE',  ( -45.07081559816839444, 1434.497539603230052, 268.7802826201569815 ) ) ;
#10521=ORIENTED_EDGE ( 'NONE', *, *, #30249, .T. ) ;
#10523=ORIENTED_EDGE ( 'NONE', *, *, #70667, .F. ) ;
#10527=CARTESIAN_POINT ( 'NONE',  ( -21.33082462610000007, 1509.431344384229988, 190.3781974747980144 ) ) ;
#10528=CARTESIAN_POINT ( 'NONE',  ( -13.06548816099999932, 1410.400106175530027, 189.7504201498980194 ) ) ;
#10529=CARTESIAN_POINT ( 'NONE',  ( -18.64588652299999794, 1416.828040475229955, 208.5593769277110141 ) ) ;
#10530=B_SPLINE_SURFACE_WITH_KNOTS ( 'NONE', 5, 5, ( 
 ( #69326, #93386, #50850, #103434, #83889, #32929 ),
 ( #16653, #24517, #84979, #58707, #92839, #8273 ),
 ( #42438, #110748, #34039, #68230, #63154, #37361 ),
 ( #28964, #9942, #44114, #86646, #54187, #78813 ),
 ( #79920, #87779, #88864, #62035, #106214, #78249 ),
 ( #96721, #27854, #3233, #2682, #1563, #36807 ),
 ( #3785, #52516, #71561, #72098, #27297, #35695 ),
 ( #70998, #97253, #36252, #87208, #20529, #69884 ),
 ( #62606, #12148, #80469, #19995, #44672, #104000 ),
 ( #18325, #53071, #10500, #105680, #61478, #2128 ),
 ( #54735, #70440, #46340, #37917, #29495, #63689 ),
 ( #105116, #104559, #96158, #11059, #19435, #95605 ) ),
 .UNSPECIFIED., .F., .F., .F.,
 ( 6, 3, 3, 6 ),
 ( 6, 6 ),
 ( 5.632673649860000076, 8.026914679749999948, 9.819017978390000678, 13.16393005930000015 ),
 ( 0.000000000000000000, 2.000000000000000000 ),
 .UNSPECIFIED. ) ;
#10533=DIRECTION ( 'NONE',  ( 5.551115123126445838E-17, -0.7071067811865475727, -0.7071067811865475727 ) ) ;
#10537=ADVANCED_FACE ( 'NONE', ( #20570 ), #32875, .T. ) ;
#10540=EDGE_LOOP ( 'NONE', ( #38923, #76186, #77766, #108705 ) ) ;
#10541=CARTESIAN_POINT ( 'NONE',  ( -28.16679250621550068, 1415.942106301169815, 270.3408856473929518 ) ) ;
#10543=CARTESIAN_POINT ( 'NONE',  ( 10.83349776640000073, 1418.147168774629790, 229.8848599606979803 ) ) ;
#10545=EDGE_CURVE ( 'NONE', #66863, #24877, #71239, .T. ) ;
#10549=CARTESIAN_POINT ( 'NONE',  ( -22.84135781497329987, 1409.740462049710004, 209.6362336836220095 ) ) ;
#10550=FACE_OUTER_BOUND ( 'NONE', #65360, .T. ) ;
#10551=CARTESIAN_POINT ( 'NONE',  ( -9.910697518993066168, 1439.577035592592665, 153.0464723132166966 ) ) ;
#10552=B_SPLINE_CURVE_WITH_KNOTS ( 'NONE', 3,
 ( #40590, #68028, #23774, #66375, #24864, #99930, #59067, #93190, #16458, #50653, #14826, #57424, #100493, #91549, #8082, #102138, #90985, #48464, #108899, #82602, #57961, #5892, #92094, #27114, #2491, #51766, #53432, #35502, #85900, #273, #34399, #26543, #77515, #17565, #61298, #87579, #87006, #103814, #36069, #60169, #52331, #95964, #70254, #102674, #93724, #816, #9207, #104361, #19225, #43367, #1360, #36608 ),
 .UNSPECIFIED., .F., .F.,
 ( 4, 2, 2, 1, 1, 1, 1, 1, 2, 2, 2, 2, 1, 1, 1, 1, 1, 2, 2, 2, 2, 1, 1, 1, 1, 2, 2, 2, 1, 1, 1, 1, 2, 2, 4 ),
 ( 0.000000000000000000, 0.2499999999998676614, 0.3749999999998021583, 0.4374999999997692957, 0.4687499999997517541, 0.4843749999997438715, 0.4921874999997398747, 0.4960937499997377653, 0.4980468749997370437, 0.4999999999997362110, 0.6249999999996997957, 0.6874999999996812550, 0.7187499999996714850, 0.7343749999996661559, 0.7421874999996637134, 0.7460937499996643796, 0.7480468749996647126, 0.7490234374996664890, 0.7499999999996681543, 0.8124999999997845057, 0.8437499999998424594, 0.8593749999998731015, 0.8671874999998884226, 0.8710937499998943068, 0.8730468749998955280, 0.8740234374998968603, 0.8749999999998980815, 0.9062499999999307221, 0.9218749999999444888, 0.9296874999999530376, 0.9335937499999571454, 0.9355468749999610312, 0.9365234374999620304, 0.9374999999999629186, 1.000000000000000000 ),
 .UNSPECIFIED. ) ;
#10553=CARTESIAN_POINT ( 'NONE',  ( -0.01532161567281509901, 1408.960427760659968, 186.0999207095659926 ) ) ;
#10556=CARTESIAN_POINT ( 'NONE',  ( -18.76327566866549645, 1416.196255291290072, 207.5730052496820122 ) ) ;
#10557=CARTESIAN_POINT ( 'NONE',  ( -22.89689784409999973, 1430.784059188729998, 215.1258104306580208 ) ) ;
#10558=CARTESIAN_POINT ( 'NONE',  ( 35.81931705070430638, 1463.269900429220115, 267.9387327459060089 ) ) ;
#10559=CARTESIAN_POINT ( 'NONE',  ( -8.825868239193008336, 1465.145812743426859, 232.9019923126272715 ) ) ;
#10560=CARTESIAN_POINT ( 'NONE',  ( 9.218600481020001070, 1445.521936428739991, 184.5777863060980053 ) ) ;
#10563=CARTESIAN_POINT ( 'NONE',  ( 21.65343676871068723, 1411.029628520915139, 216.8370129969001425 ) ) ;
#10564=CARTESIAN_POINT ( 'NONE',  ( 1.506875757802919935, 1462.572888004679953, 183.0571693780200064 ) ) ;
#10565=CARTESIAN_POINT ( 'NONE',  ( 23.92908890809999889, 1410.712361784030008, 208.4166298941610194 ) ) ;
#10567=CARTESIAN_POINT ( 'NONE',  ( -3.827327205999999649, 1424.046157813729906, 127.2892455880980123 ) ) ;
#10569=CARTESIAN_POINT ( 'NONE',  ( 26.16029670472540047, 1451.268733793390084, 136.4243401975820120 ) ) ;
#10570=DIRECTION ( 'NONE',  ( 0.0002626049189776629507, -0.0002559000790209099187, -0.9999999327769008017 ) ) ;
#10572=ADVANCED_FACE ( 'NONE', ( #24430 ), #57528, .F. ) ;
#10574=CARTESIAN_POINT ( 'NONE',  ( 17.83376335750000052, 1409.535829129529930, 195.1640540924980201 ) ) ;
#10575=CARTESIAN_POINT ( 'NONE',  ( 17.11714625305219073, 1444.740067931810245, 162.7561045841208909 ) ) ;
#10576=CARTESIAN_POINT ( 'NONE',  ( 2.609822991816500348, 1439.645108688199571, 183.4245757125495118 ) ) ;
#10577=CARTESIAN_POINT ( 'NONE',  ( 0.8893907640070000120, 1417.383361611430018, 235.4581877438980086 ) ) ;
#10578=CARTESIAN_POINT ( 'NONE',  ( -18.59108776923753226, 1424.390149891285546, 224.8865353940923626 ) ) ;
#10579=CARTESIAN_POINT ( 'NONE',  ( 11.60004869885203682, 1425.894332500278097, 137.5113157688821275 ) ) ;
#10582=CARTESIAN_POINT ( 'NONE',  ( 27.85007276605439941, 1509.193792694948570, 207.4562352035727884 ) ) ;
#10585=ORIENTED_EDGE ( 'NONE', *, *, #11168, .F. ) ;
#10588=CARTESIAN_POINT ( 'NONE',  ( -0.4694225489305150489, 1409.462648608420068, 232.8560743051169766 ) ) ;
#10590=DIRECTION ( 'NONE',  ( 1.000000000000000000, 0.000000000000000000, 0.000000000000000000 ) ) ;
#10592=DIRECTION ( 'NONE',  ( 0.000000000000000000, 0.000000000000000000, 1.000000000000000000 ) ) ;
#10593=CARTESIAN_POINT ( 'NONE',  ( -19.80583356029999820, 1445.467019065099976, 219.6133833564979909 ) ) ;
#10596=CARTESIAN_POINT ( 'NONE',  ( -45.55748378925329689, 1443.471975657500025, 268.9766690249090288 ) ) ;
#10597=CARTESIAN_POINT ( 'NONE',  ( 25.75379067826139945, 1440.913060398739844, 220.5312563427889927 ) ) ;
#10600=EDGE_CURVE ( 'NONE', #85148, #102192, #36479, .T. ) ;
#10601=CARTESIAN_POINT ( 'NONE',  ( 22.62861454470000311, 1507.212883763329955, 209.7205631874760172 ) ) ;
#10603=CARTESIAN_POINT ( 'NONE',  ( -7.031825459540000267, 1486.383742291129920, 182.5071239263980090 ) ) ;
#10604=CARTESIAN_POINT ( 'NONE',  ( 7.991873292109088922, 1398.150424849050751, 198.8685539432230200 ) ) ;
#10605=CARTESIAN_POINT ( 'NONE',  ( -15.00563130453249983, 1509.437066463229939, 236.2075740539809772 ) ) ;
#10609=CARTESIAN_POINT ( 'NONE',  ( 25.25968088009999946, 1449.800564152120160, 211.7062984677579891 ) ) ;
#10613=CARTESIAN_POINT ( 'NONE',  ( 21.01360359149740020, 1507.224983811549919, 226.0477246056319984 ) ) ;
#10615=CARTESIAN_POINT ( 'NONE',  ( 5.617607972230620028, 1423.117395914830013, 104.0874243697959969 ) ) ;
#10617=CARTESIAN_POINT ( 'NONE',  ( 0.1625026641855710219, 1484.765001907559963, 181.8896783937200041 ) ) ;
#10619=ORIENTED_EDGE ( 'NONE', *, *, #17357, .F. ) ;
#10620=CARTESIAN_POINT ( 'NONE',  ( -12.91247410300000276, 1445.052233488288948, 177.4417055768979026 ) ) ;
#10627=ORIENTED_EDGE ( 'NONE', *, *, #96163, .F. ) ;
#10630=CARTESIAN_POINT ( 'NONE',  ( 11.54856215818386111, 1426.051318353786428, 138.9194232893295293 ) ) ;
#10631=CARTESIAN_POINT ( 'NONE',  ( 23.35503201018713426, 1410.253263171711296, 207.9904190973228140 ) ) ;
#10633=DIRECTION ( 'NONE',  ( -0.9995237709234254808, 0.03085824620771311644, -1.986952269380852068E-13 ) ) ;
#10634=CARTESIAN_POINT ( 'NONE',  ( 11.81689878039349928, 1409.325715576620041, 218.2705614814449859 ) ) ;
#10637=CARTESIAN_POINT ( 'NONE',  ( 2.933761696634608285, 1464.631290068389944, 236.6723688072773939 ) ) ;
#10639=ORIENTED_EDGE ( 'NONE', *, *, #86258, .F. ) ;
#10643=ORIENTED_EDGE ( 'NONE', *, *, #89035, .T. ) ;
#10647=CARTESIAN_POINT ( 'NONE',  ( 25.23579092139999958, 1509.794313625030100, 223.6174824585980048 ) ) ;
#10649=CARTESIAN_POINT ( 'NONE',  ( -11.48887253859999902, 1433.998994749410031, 151.3897975962979956 ) ) ;
#10650=CARTESIAN_POINT ( 'NONE',  ( 33.74597417575863290, 1459.080184772059056, 269.5147043096913535 ) ) ;
#10652=CARTESIAN_POINT ( 'NONE',  ( -28.28208339020000039, 1508.151294418729776, 209.1342425839550287 ) ) ;
#10657=CARTESIAN_POINT ( 'NONE',  ( -18.93704128152869970, 1430.332824596809814, 208.8580461249810014 ) ) ;
#10660=VECTOR ( 'NONE', #26822, 1000.000000000000000 ) ;
#10661=CARTESIAN_POINT ( 'NONE',  ( -12.97204092183419988, 1434.766546360639950, 149.2832816642720104 ) ) ;
#10662=B_SPLINE_SURFACE_WITH_KNOTS ( 'NONE', 5, 5, ( 
 ( #42590, #76743, #55, #68926, #60515, #9530, #43698, #77852, #63825 ),
 ( #88993, #46475, #106353, #44821, #78974, #27993, #105822, #79514, #19583 ),
 ( #11745, #35853, #88458, #71704, #95750, #104698, #2818, #1713, #70037 ),
 ( #45374, #53217, #2278, #53787, #87924, #38052, #104149, #96305, #12281 ),
 ( #62178, #29639, #62748, #97938, #80607, #11211, #36937, #87356, #71134 ),
 ( #21206, #27435, #105255, #20135, #61618, #28549, #29100, #86795, #72229 ) ),
 .UNSPECIFIED., .F., .F., .F.,
 ( 6, 6 ),
 ( 6, 3, 6 ),
 ( 0.000000000000000000, 8.627065936320001072 ),
 ( 0.000000000000000000, 1.000000000000000000, 2.000000000000000000 ),
 .UNSPECIFIED. ) ;
#10663=CARTESIAN_POINT ( 'NONE',  ( 0.000000000000000000, 1450.913060387330006, 198.0847581337980046 ) ) ;
#10666=B_SPLINE_CURVE_WITH_KNOTS ( 'NONE', 3,
 ( #94221, #51693, #59545, #41632, #109939, #93658, #16939, #747, #42736, #34329, #94788, #68507 ),
 .UNSPECIFIED., .F., .F.,
 ( 4, 2, 2, 2, 2, 4 ),
 ( -0.1123552069981540030, -0.09789079992753631221, -0.08345977618154098998, -0.05408602697413120164, -0.02844237633788339326, 0.000000000000000000 ),
 .UNSPECIFIED. ) ;
#10669=CARTESIAN_POINT ( 'NONE',  ( 43.50118997730000103, 1438.239417958949844, 263.8966302629980305 ) ) ;
#10670=CARTESIAN_POINT ( 'NONE',  ( -27.46043821989999856, 1488.693027618630140, 209.0953481391420041 ) ) ;
#10671=CARTESIAN_POINT ( 'NONE',  ( -11.06108549758080173, 1426.493804035829953, 95.13674927509649137 ) ) ;
#10672=CARTESIAN_POINT ( 'NONE',  ( 16.35901261092910275, 1409.492683085800081, 193.1285600932399973 ) ) ;
#10674=CARTESIAN_POINT ( 'NONE',  ( 2.782332782707229946, 1396.010221589069943, 198.4612922233270069 ) ) ;
#10676=AXIS2_PLACEMENT_3D ( 'NONE', #58441, #84173, #67408 ) ;
#10677=CARTESIAN_POINT ( 'NONE',  ( -26.19682245239999929, 1416.543456363630185, 259.6166969371979576 ) ) ;
#10679=CARTESIAN_POINT ( 'NONE',  ( 28.97445500250269745, 1509.604966148099948, 209.5493756428880090 ) ) ;
#10681=CARTESIAN_POINT ( 'NONE',  ( 30.22858968940000324, 1451.857573268230226, 134.8239104374980002 ) ) ;
#10683=CARTESIAN_POINT ( 'NONE',  ( 13.90997033016400053, 1397.713899063759982, 206.9547035159640131 ) ) ;
#10685=CARTESIAN_POINT ( 'NONE',  ( 37.88774006571860298, 1442.824633575369944, 137.1073183462559939 ) ) ;
#10686=ORIENTED_EDGE ( 'NONE', *, *, #72040, .F. ) ;
#10691=CARTESIAN_POINT ( 'NONE',  ( -1.363527627800000142, 1415.665897350729892, 185.3780671533980069 ) ) ;
#10692=CARTESIAN_POINT ( 'NONE',  ( 8.279338672908640007, 1446.667838523203045, 153.9572786840106176 ) ) ;
#10694=CARTESIAN_POINT ( 'NONE',  ( -5.653753708210000006, 1470.479446996229854, 234.4212017938980068 ) ) ;
#10695=CARTESIAN_POINT ( 'NONE',  ( 1.957738139717299930, 1421.112252580069935, 183.1490905797940059 ) ) ;
#10697=FACE_OUTER_BOUND ( 'NONE', #97105, .T. ) ;
#10698=CARTESIAN_POINT ( 'NONE',  ( 15.13403569980000007, 1507.625766696829942, 226.3980367026980218 ) ) ;
#10702=CARTESIAN_POINT ( 'NONE',  ( 11.86131399675660170, 1432.001727244180074, 149.9720548203619899 ) ) ;
#10705=CARTESIAN_POINT ( 'NONE',  ( 1.600048698852036821, 1411.254281879943164, 134.0999999980979851 ) ) ;
#10707=CARTESIAN_POINT ( 'NONE',  ( -15.56138138465544607, 1506.691119431732886, 193.2904356335322689 ) ) ;
#10711=CARTESIAN_POINT ( 'NONE',  ( -6.189336700450000173, 1423.191529671129956, 186.6229957612979717 ) ) ;
#10712=AXIS2_PLACEMENT_3D ( 'NONE', #46501, #12864, #106380 ) ;
#10713=CARTESIAN_POINT ( 'NONE',  ( 2.278116099415719908, 1409.246459464170130, 270.3712219384140099 ) ) ;
#10714=CARTESIAN_POINT ( 'NONE',  ( -7.052967567875161770, 1427.664849047028611, 137.0999999980979851 ) ) ;
#10722=CARTESIAN_POINT ( 'NONE',  ( 17.75620770209309995, 1415.752091378990144, 224.9496030967819991 ) ) ;
#10724=ORIENTED_EDGE ( 'NONE', *, *, #52290, .F. ) ;
#10725=CARTESIAN_POINT ( 'NONE',  ( 31.32742178679999512, 1440.913060387330006, 255.3819207742980097 ) ) ;
#10729=CARTESIAN_POINT ( 'NONE',  ( 38.19123335760763638, 1450.350430573902031, 134.7938291898653915 ) ) ;
#10731=CARTESIAN_POINT ( 'NONE',  ( 11.96188367727480006, 1407.497305617939901, 269.6154717270600258 ) ) ;
#10735=FACE_OUTER_BOUND ( 'NONE', #108441, .T. ) ;
#10740=CARTESIAN_POINT ( 'NONE',  ( 27.87567397839760375, 1509.925536542059945, 194.5356986537630064 ) ) ;
#10743=CARTESIAN_POINT ( 'NONE',  ( 14.99625699449999949, 1410.404882082729955, 227.4791858470979946 ) ) ;
#10748=CARTESIAN_POINT ( 'NONE',  ( 41.20202881409999662, 1425.323100257629903, 268.8974569184979941 ) ) ;
#10749=CARTESIAN_POINT ( 'NONE',  ( -18.72407526530000155, 1458.246115540929850, 227.3156487912980026 ) ) ;
#10751=CARTESIAN_POINT ( 'NONE',  ( 18.17633956390000094, 1435.132278384110123, 145.0981326318980109 ) ) ;
#10752=CARTESIAN_POINT ( 'NONE',  ( 19.87154596619999936, 1488.588627089529837, 190.3431199549980022 ) ) ;
#10753=CARTESIAN_POINT ( 'NONE',  ( -21.44806981200000351, 1428.950306416729973, 219.4680445577980095 ) ) ;
#10755=CARTESIAN_POINT ( 'NONE',  ( -17.66442964079999811, 1420.867159957530021, 226.1080994653979985 ) ) ;
#10757=CARTESIAN_POINT ( 'NONE',  ( -40.71506854697640421, 1443.618868117700003, 137.1015915340059905 ) ) ;
#10759=CARTESIAN_POINT ( 'NONE',  ( -4.363122647530000009, 1432.413060387330006, 146.1721969590979882 ) ) ;
#10761=CARTESIAN_POINT ( 'NONE',  ( -12.53380499110000024, 1442.773887285770115, 185.9733677063979940 ) ) ;
#10763=CARTESIAN_POINT ( 'NONE',  ( -3.326017048431102679E-16, 1419.995592097834106, 171.1876449949939456 ) ) ;
#10764=VERTEX_POINT ( 'NONE', #52433 ) ;
#10766=CARTESIAN_POINT ( 'NONE',  ( -13.41295867642740092, 1409.381451225490082, 215.7039827110959891 ) ) ;
#10767=CARTESIAN_POINT ( 'NONE',  ( -5.483194490039999813, 1439.280902438360044, 154.7474842100980084 ) ) ;
#10768=CARTESIAN_POINT ( 'NONE',  ( -33.98065672744881027, 1443.913060387328869, 154.9321739644268234 ) ) ;
#10769=CARTESIAN_POINT ( 'NONE',  ( -27.10895137460000015, 1469.515388080030107, 268.1710267444980218 ) ) ;
#10771=CARTESIAN_POINT ( 'NONE',  ( 0.4863421998530879642, 1418.702335047680208, 184.7127968358159933 ) ) ;
#10774=CARTESIAN_POINT ( 'NONE',  ( 17.89269544292019631, 1424.514345381910061, 226.2830465645759830 ) ) ;
#10775=CARTESIAN_POINT ( 'NONE',  ( 17.23902921200000193, 1416.518938591829965, 215.4040154682980130 ) ) ;
#10776=CARTESIAN_POINT ( 'NONE',  ( 15.59201085350000149, 1506.806593714529981, 224.7816022336980097 ) ) ;
#10780=CARTESIAN_POINT ( 'NONE',  ( 1.435281448510400182, 1482.857262105389964, 235.7275092897180002 ) ) ;
#10781=CARTESIAN_POINT ( 'NONE',  ( 14.11509896619999971, 1414.913060387329779, 199.7393156684579765 ) ) ;
#10783=CIRCLE ( 'NONE', #89427, 1.999999999999921174 ) ;
#10785=B_SPLINE_CURVE_WITH_KNOTS ( 'NONE', 5,
 ( #22243, #30110, #37983, #98425, #37433, #71631, #73237, #29035, #72165, #107379, #21697 ),
 .UNSPECIFIED., .F., .F.,
 ( 6, 5, 6 ),
 ( -167.7485006210000051, -75.51693185479999215, -75.51691072595589560 ),
 .UNSPECIFIED. ) ;
#10786=CARTESIAN_POINT ( 'NONE',  ( 22.99745501010000126, 1409.716149210629965, 209.9703408740099917 ) ) ;
#10788=CARTESIAN_POINT ( 'NONE',  ( 4.500000000000000000, 1448.210448412289907, 182.3842140122979743 ) ) ;
#10790=CARTESIAN_POINT ( 'NONE',  ( -16.26200603700000258, 1421.946001659629928, 227.1818636008979979 ) ) ;
#10791=CARTESIAN_POINT ( 'NONE',  ( 11.90005888108785115, 1434.918254481208578, 147.6452161523065172 ) ) ;
#10793=CARTESIAN_POINT ( 'NONE',  ( -0.5044665043120000192, 1413.022983338129961, 233.2877477755979783 ) ) ;
#10794=CARTESIAN_POINT ( 'NONE',  ( -27.01380866140000236, 1450.681584507220123, 136.4483241423979791 ) ) ;
#10797=B_SPLINE_CURVE_WITH_KNOTS ( 'NONE', 5,
 ( #108216, #47224, #81350, #83021, #31504, #64596, #23096, #65134, #99802 ),
 .UNSPECIFIED., .F., .F.,
 ( 6, 3, 6 ),
 ( 0.000000000000000000, 0.4258937504861698975, 1.000000000000000000 ),
 .UNSPECIFIED. ) ;
#10800=CARTESIAN_POINT ( 'NONE',  ( -16.69612950000000140, 1484.879939360330127, 188.0702094165980043 ) ) ;
#10805=ORIENTED_EDGE ( 'NONE', *, *, #35036, .T. ) ;
#10807=CARTESIAN_POINT ( 'NONE',  ( 11.59845407533470052, 1433.863182457509993, 151.1985623341290079 ) ) ;
#10813=CARTESIAN_POINT ( 'NONE',  ( 15.87725485892149990, 1417.455994837740036, 191.3130337353669859 ) ) ;
#10814=CARTESIAN_POINT ( 'NONE',  ( 0.1700419896689999988, 1508.143047484930094, 180.7157097131980095 ) ) ;
#10816=CARTESIAN_POINT ( 'NONE',  ( 1.002856167820000088, 1507.642691268429871, 181.0118679135980244 ) ) ;
#10818=CARTESIAN_POINT ( 'NONE',  ( -24.31736970558739941, 1444.784419045710138, 211.2645309320329829 ) ) ;
#10819=SURFACE_SIDE_STYLE ('',( #61795 ) ) ;
#10821=CARTESIAN_POINT ( 'NONE',  ( 38.53505231964519595, 1437.347470673020098, 134.0999999971709826 ) ) ;
#10822=CARTESIAN_POINT ( 'NONE',  ( 10.97017907350000065, 1432.399092116580050, 151.7699749429979761 ) ) ;
#10825=CARTESIAN_POINT ( 'NONE',  ( 13.81711443553279928, 1435.003621955109793, 148.8829541362160001 ) ) ;
#10827=VERTEX_POINT ( 'NONE', #42351 ) ;
#10833=CARTESIAN_POINT ( 'NONE',  ( -0.3328314641405109575, 1452.976685807730291, 183.2631399573310205 ) ) ;
#10834=CARTESIAN_POINT ( 'NONE',  ( 2.500000000000000000, 1439.615672362369878, 170.5246407131980106 ) ) ;
#10837=CARTESIAN_POINT ( 'NONE',  ( -18.52846729114558144, 1445.641343889673180, 214.4839088109478382 ) ) ;
#10839=CARTESIAN_POINT ( 'NONE',  ( 4.222051968967549307, 1446.225890581839849, 170.2166983236299700 ) ) ;
#10844=CARTESIAN_POINT ( 'NONE',  ( 26.08449786710409768, 1440.913060387330006, 242.4625039277019880 ) ) ;
#10846=CARTESIAN_POINT ( 'NONE',  ( -20.01067436350000150, 1507.877435269729858, 188.9709114762979993 ) ) ;
#10849=CARTESIAN_POINT ( 'NONE',  ( -14.94606559790000055, 1410.367200001129959, 190.7402031657980217 ) ) ;
#10851=CARTESIAN_POINT ( 'NONE',  ( -24.90010528310000026, 1441.007489118620015, 210.4306619436680137 ) ) ;
#10855=CARTESIAN_POINT ( 'NONE',  ( 26.75392368510250307, 1441.320991048120050, 137.5422836279790033 ) ) ;
#10856=CARTESIAN_POINT ( 'NONE',  ( -27.08505272378080164, 1438.263425979839894, 136.9491044588319824 ) ) ;
#10857=CARTESIAN_POINT ( 'NONE',  ( 18.91392684480000241, 1435.157588376100193, 144.3614089622979861 ) ) ;
#10858=CARTESIAN_POINT ( 'NONE',  ( 15.71587021594741884, 1409.995737203585577, 191.8203616610946085 ) ) ;
#10861=FACE_OUTER_BOUND ( 'NONE', #21519, .T. ) ;
#10864=CARTESIAN_POINT ( 'NONE',  ( 28.32265147949999928, 1509.673549455729926, 207.2611521497780132 ) ) ;
#10866=CARTESIAN_POINT ( 'NONE',  ( -18.16348015480000200, 1416.820969729830040, 209.0764828567799896 ) ) ;
#10872=CARTESIAN_POINT ( 'NONE',  ( 20.03573726229999963, 1460.150672172730083, 240.3194873227980111 ) ) ;
#10876=CARTESIAN_POINT ( 'NONE',  ( -7.324858259705050223, 1509.160117843870012, 237.2583435074130023 ) ) ;
#10877=CARTESIAN_POINT ( 'NONE',  ( -20.63308528640000006, 1455.489145095029926, 224.0314336810980080 ) ) ;
#10878=CARTESIAN_POINT ( 'NONE',  ( -21.65063745823909258, 1411.029531829768075, 201.4006313786291855 ) ) ;
#10879=CARTESIAN_POINT ( 'NONE',  ( 17.23552702700579786, 1409.586384505080105, 222.3856984215319983 ) ) ;
#10880=CARTESIAN_POINT ( 'NONE',  ( 0.2646381833610000345, 1434.810047171390124, 189.9884865742980082 ) ) ;
#10882=ORIENTED_EDGE ( 'NONE', *, *, #12497, .T. ) ;
#10884=CARTESIAN_POINT ( 'NONE',  ( 0.5523900547170000896, 1406.508913882830029, 269.4985896812980286 ) ) ;
#10885=CARTESIAN_POINT ( 'NONE',  ( 27.74968890970000146, 1508.601238174130003, 207.7069383892280143 ) ) ;
#10887=CARTESIAN_POINT ( 'NONE',  ( 44.13013282332929776, 1446.281291277249920, 270.2165820380340051 ) ) ;
#10888=CARTESIAN_POINT ( 'NONE',  ( 5.395424494550000283, 1433.568245638130065, 154.6346167951979851 ) ) ;
#10890=CARTESIAN_POINT ( 'NONE',  ( -36.83756290334599726, 1440.913060387389805, 254.3462983698770472 ) ) ;
#10891=CARTESIAN_POINT ( 'NONE',  ( 36.55810202059989678, 1449.776383268349946, 136.2665498954540055 ) ) ;
#10892=CARTESIAN_POINT ( 'NONE',  ( 0.8295539019444626572, 1450.884091712275449, 154.2427803864302405 ) ) ;
#10893=CARTESIAN_POINT ( 'NONE',  ( 2.303292329924660375, 1449.840026814039902, 154.2474790657759911 ) ) ;
#10898=CARTESIAN_POINT ( 'NONE',  ( 0.4960531524660349856, 1409.436441971110071, 185.2773250395759987 ) ) ;
#10902=CARTESIAN_POINT ( 'NONE',  ( -1.327697533569999866, 1475.746612594030012, 269.0450429478979686 ) ) ;
#10905=CARTESIAN_POINT ( 'NONE',  ( -3.779110701619425861, 1448.294363581284188, 185.0060619559291695 ) ) ;
#10907=CARTESIAN_POINT ( 'NONE',  ( -18.90690566160000330, 1416.819756528429934, 208.2173862770389690 ) ) ;
#10909=CARTESIAN_POINT ( 'NONE',  ( 26.41104128045460087, 1435.419835122459972, 135.2945573537490134 ) ) ;
#10910=CARTESIAN_POINT ( 'NONE',  ( -11.05338566285159807, 1396.299053120159897, 208.4942113865890292 ) ) ;
#10912=CARTESIAN_POINT ( 'NONE',  ( -15.20078488979999953, 1421.481067149630007, 227.2882089291979923 ) ) ;
#10913=CARTESIAN_POINT ( 'NONE',  ( -16.59151158838270135, 1409.592917334169897, 225.4533943397379971 ) ) ;
#10915=ORIENTED_EDGE ( 'NONE', *, *, #31975, .T. ) ;
#10917=CARTESIAN_POINT ( 'NONE',  ( 1.984522837200000112, 1409.916377421130164, 231.9929760013979774 ) ) ;
#10919=CARTESIAN_POINT ( 'NONE',  ( 10.22494416990000055, 1425.155393777929930, 108.0534255276979962 ) ) ;
#10933=CARTESIAN_POINT ( 'NONE',  ( -40.27309184310000489, 1443.612070458560083, 137.1163417766980217 ) ) ;
#10935=CARTESIAN_POINT ( 'NONE',  ( 0.06029893845285259901, 1482.863300304640006, 236.3492419568210039 ) ) ;
#10936=CARTESIAN_POINT ( 'NONE',  ( 6.553899686920000356, 1408.913060387329779, 225.8798606464979741 ) ) ;
#10938=CARTESIAN_POINT ( 'NONE',  ( -0.6009897688609999733, 1485.972025337430068, 182.1351461919979897 ) ) ;
#10945=CARTESIAN_POINT ( 'NONE',  ( 35.12833357477309448, 1435.886684291350093, 135.9061531807790004 ) ) ;
#10946=CARTESIAN_POINT ( 'NONE',  ( 32.00871303854333405, 1435.615229631456941, 135.1257567998584364 ) ) ;
#10947=CARTESIAN_POINT ( 'NONE',  ( 8.999538239140179030, 1407.274461440940058, 198.9439808189530083 ) ) ;
#10948=CARTESIAN_POINT ( 'NONE',  ( 5.721593877714729399E-05, 1405.775960253769881, 268.4837777154720015 ) ) ;
#10952=CARTESIAN_POINT ( 'NONE',  ( 12.89029109540000029, 1442.787888345740157, 187.7063189797979987 ) ) ;
#10963=CARTESIAN_POINT ( 'NONE',  ( 7.752198807150000981, 1416.823872462329973, 225.7667597232980086 ) ) ;
#10968=CARTESIAN_POINT ( 'NONE',  ( -5.984203303400000173, 1409.122033371430007, 229.9503900095979816 ) ) ;
#10969=CARTESIAN_POINT ( 'NONE',  ( -10.46909318259999999, 1447.037035936289840, 186.8418773576979959 ) ) ;
#10970=EDGE_LOOP ( 'NONE', ( #105669, #63673, #71568, #13766, #92751 ) ) ;
#10972=FACE_OUTER_BOUND ( 'NONE', #25113, .T. ) ;
#10973=CARTESIAN_POINT ( 'NONE',  ( 20.59705046560049624, 1507.771217143799959, 227.0402443945910136 ) ) ;
#10975=CARTESIAN_POINT ( 'NONE',  ( -25.09080907949999784, 1435.392650067190061, 135.9845614618979823 ) ) ;
#10979=CARTESIAN_POINT ( 'NONE',  ( 0.01526382458731936030, 1507.788721570215102, 237.5012585564631706 ) ) ;
#10981=CARTESIAN_POINT ( 'NONE',  ( 21.47298199986007816, 1411.021785953378640, 201.3753046382076377 ) ) ;
#10984=CARTESIAN_POINT ( 'NONE',  ( 2.500000000000000000, 1439.039897141910160, 157.7230890540980113 ) ) ;
#10985=CARTESIAN_POINT ( 'NONE',  ( -3.071779842299999785, 1420.448432582830037, 232.9517911341980039 ) ) ;
#10987=ORIENTED_EDGE ( 'NONE', *, *, #98959, .T. ) ;
#10991=EDGE_CURVE ( 'NONE', #96609, #110603, #39049, .T. ) ;
#10992=CARTESIAN_POINT ( 'NONE',  ( 18.44206918373069826, 1469.011769097089882, 228.2221280545410025 ) ) ;
#10994=CARTESIAN_POINT ( 'NONE',  ( -24.03031496624599583, 1509.069760856670200, 222.9704818946499927 ) ) ;
#10995=CARTESIAN_POINT ( 'NONE',  ( -0.8265242350169998975, 1408.941923249630008, 187.0792671732980068 ) ) ;
#10999=CARTESIAN_POINT ( 'NONE',  ( -2.566419091909999839, 1420.628703720230078, 185.8818997532980006 ) ) ;
#11000=CARTESIAN_POINT ( 'NONE',  ( 18.65451754129999529, 1507.632629717330019, 188.5326157632979971 ) ) ;
#11002=ORIENTED_EDGE ( 'NONE', *, *, #66601, .T. ) ;
#11003=CARTESIAN_POINT ( 'NONE',  ( -11.57735155928969917, 1414.971513442450032, 196.9567343561169821 ) ) ;
#11004=CARTESIAN_POINT ( 'NONE',  ( -20.06431043899999622, 1490.513422158030153, 190.0771971858980294 ) ) ;
#11007=CARTESIAN_POINT ( 'NONE',  ( 2.713698362399999731, 1421.382238371229960, 183.9342778676980004 ) ) ;
#11008=DIRECTION ( 'NONE',  ( -0.9995237703344608260, 0.03085826527909721340, -5.905782510576255506E-07 ) ) ;
#11011=CARTESIAN_POINT ( 'NONE',  ( -26.35750891854250000, 1508.044014828989930, 201.5443954048259911 ) ) ;
#11013=CARTESIAN_POINT ( 'NONE',  ( 18.04709463619999710, 1415.245980412329800, 210.4308792091779878 ) ) ;
#11014=CARTESIAN_POINT ( 'NONE',  ( -17.95904881909999773, 1424.699834624730101, 227.3705041876980033 ) ) ;
#11015=FACE_OUTER_BOUND ( 'NONE', #96976, .T. ) ;
#11017=CARTESIAN_POINT ( 'NONE',  ( 17.39646299289999831, 1418.986622976930221, 191.8562750549980080 ) ) ;
#11019=CARTESIAN_POINT ( 'NONE',  ( 0.5969155455355750206, 1501.813611154769887, 186.7307704303590015 ) ) ;
#11020=CARTESIAN_POINT ( 'NONE',  ( 27.39760735127830316, 1439.876886201499929, 137.1284513264700138 ) ) ;
#11022=CARTESIAN_POINT ( 'NONE',  ( 1.556517342736410070, 1415.020374539499926, 191.6346848232400077 ) ) ;
#11023=CARTESIAN_POINT ( 'NONE',  ( 26.35471571933159751, 1507.985750330240080, 216.6976075425179999 ) ) ;
#11026=CARTESIAN_POINT ( 'NONE',  ( -11.89516918277866964, 1433.269309810761570, 149.9552381126513865 ) ) ;
#11030=CARTESIAN_POINT ( 'NONE',  ( 13.22806383200000013, 1431.113060387329824, 222.3499097933980124 ) ) ;
#11031=B_SPLINE_CURVE_WITH_KNOTS ( 'NONE', 3,
 ( #50729, #77594, #42329, #43445, #49645, #84862, #85413, #900, #8712, #77049, #26053, #60248 ),
 .UNSPECIFIED., .F., .F.,
 ( 4, 2, 2, 2, 2, 4 ),
 ( -0.1123552056274609995, -0.09789079770775470368, -0.08345975727710699954, -0.05408602632130809357, -0.02844277166756620234, 0.000000000000000000 ),
 .UNSPECIFIED. ) ;
#11038=DIRECTION ( 'NONE',  ( 0.000000000000000000, -1.000000000000000000, 0.000000000000000000 ) ) ;
#11039=CARTESIAN_POINT ( 'NONE',  ( -15.95383389570000077, 1506.798305147730161, 224.6865364803979901 ) ) ;
#11041=CARTESIAN_POINT ( 'NONE',  ( 21.06390421310000249, 1509.318873927029927, 189.5956816894980079 ) ) ;
#11048=FACE_OUTER_BOUND ( 'NONE', #60712, .T. ) ;
#11050=CARTESIAN_POINT ( 'NONE',  ( 13.51610093809999924, 1443.913060387330006, 169.3501091259980171 ) ) ;
#11051=CARTESIAN_POINT ( 'NONE',  ( 18.16348015480000200, 1416.820969729830040, 209.1672090666169765 ) ) ;
#11052=CARTESIAN_POINT ( 'NONE',  ( -38.77640752969999483, 1448.325305151830207, 259.1404898689979746 ) ) ;
#11054=CARTESIAN_POINT ( 'NONE',  ( -11.29670609480000110, 1433.873747960979927, 151.5261222975980218 ) ) ;
#11058=CARTESIAN_POINT ( 'NONE',  ( 13.30361592369999890, 1409.377632892530073, 191.9462335214980158 ) ) ;
#11059=CARTESIAN_POINT ( 'NONE',  ( 4.132091976209999906, 1421.241915956429921, 185.3693088014979935 ) ) ;
#11060=CARTESIAN_POINT ( 'NONE',  ( -10.72974951780000019, 1437.118219917419992, 152.1700466790979931 ) ) ;
#11061=CARTESIAN_POINT ( 'NONE',  ( 10.13504311139999992, 1439.368087371720094, 152.9209920991980027 ) ) ;
#11064=CARTESIAN_POINT ( 'NONE',  ( 1.971095687570000088, 1464.814373034330174, 236.1963163484979873 ) ) ;
#11065=ORIENTED_EDGE ( 'NONE', *, *, #22765, .T. ) ;
#11066=CARTESIAN_POINT ( 'NONE',  ( -33.91369265678890343, 1437.010538859309918, 136.5611844326260211 ) ) ;
#11067=ADVANCED_FACE ( 'NONE', ( #17113 ), #92788, .T. ) ;
#11070=CARTESIAN_POINT ( 'NONE',  ( -37.36936258469999927, 1456.002134664930054, 270.0098740415979819 ) ) ;
#11072=CARTESIAN_POINT ( 'NONE',  ( 8.437694987149998527E-15, 1442.756953654919926, 155.7628527808980152 ) ) ;
#11075=VECTOR ( 'NONE', #47652, 1000.000000000000000 ) ;
#11076=CARTESIAN_POINT ( 'NONE',  ( 4.963802804109999300, 1497.713060387329961, 187.3310108713980071 ) ) ;
#11078=CARTESIAN_POINT ( 'NONE',  ( 2.838492387013249907, 1409.123886199480012, 230.7524214366010256 ) ) ;
#11079=CARTESIAN_POINT ( 'NONE',  ( 1.205197961869999945, 1507.636020686930124, 237.0931865834980101 ) ) ;
#11080=CARTESIAN_POINT ( 'NONE',  ( -12.47269130070000109, 1419.287450240530006, 228.5775552544979803 ) ) ;
#11084=CARTESIAN_POINT ( 'NONE',  ( -44.65796480198309837, 1433.806179381780112, 269.0022936558889910 ) ) ;
#11089=EDGE_CURVE ( 'NONE', #17927, #75668, #5774, .T. ) ;
#11093=CARTESIAN_POINT ( 'NONE',  ( 17.56004567126451477, 1410.529979399466811, 224.8086585292313373 ) ) ;
#11094=CARTESIAN_POINT ( 'NONE',  ( -12.30019964340000094, 1410.398530115529866, 189.3840444957980083 ) ) ;
#11097=CARTESIAN_POINT ( 'NONE',  ( -27.02719243892629919, 1451.200357981530033, 136.2769546900069884 ) ) ;
#11103=AXIS2_PLACEMENT_3D ( 'NONE', #56938, #47433, #98369 ) ;
#11104=CARTESIAN_POINT ( 'NONE',  ( 11.60004869885203682, 1423.972955187191246, 135.9380529689869661 ) ) ;
#11108=CARTESIAN_POINT ( 'NONE',  ( 5.511665417999469900E-05, 1508.970066526555001, 238.8757070596369942 ) ) ;
#11109=ORIENTED_EDGE ( 'NONE', *, *, #33043, .T. ) ;
#11110=CARTESIAN_POINT ( 'NONE',  ( -22.40264917047960225, 1414.570795220049831, 269.9085733495129489 ) ) ;
#11115=ORIENTED_EDGE ( 'NONE', *, *, #46758, .T. ) ;
#11116=VERTEX_POINT ( 'NONE', #88437 ) ;
#11118=CARTESIAN_POINT ( 'NONE',  ( 42.90684747031818347, 1452.569395717577436, 269.0510755419506950 ) ) ;
#11121=CARTESIAN_POINT ( 'NONE',  ( -0.03180497178026089888, 1409.232592949579839, 185.5579152414480291 ) ) ;
#11122=EDGE_CURVE ( 'NONE', #72755, #61631, #108424, .T. ) ;
#11123=CARTESIAN_POINT ( 'NONE',  ( -18.73709653282620025, 1416.134159090969888, 207.5726623008649767 ) ) ;
#11124=CARTESIAN_POINT ( 'NONE',  ( -18.80193033609999986, 1425.815728067429973, 224.6524251216980019 ) ) ;
#11125=CARTESIAN_POINT ( 'NONE',  ( 5.345145192925599531, 1476.109332684420224, 267.8539259984499949 ) ) ;
#11127=CARTESIAN_POINT ( 'NONE',  ( 5.514569887500000434, 1447.126989177859969, 184.6235071523979911 ) ) ;
#11129=ORIENTED_EDGE ( 'NONE', *, *, #81853, .T. ) ;
#11130=CARTESIAN_POINT ( 'NONE',  ( 23.96131741799887394, 1411.110629221238696, 210.1578133893788447 ) ) ;
#11131=CARTESIAN_POINT ( 'NONE',  ( 1.491499242636469935, 1470.574770574250124, 182.7072383254629813 ) ) ;
#11134=CARTESIAN_POINT ( 'NONE',  ( 24.82914352958970028, 1452.046038066890105, 135.7260749457049940 ) ) ;
#11135=CARTESIAN_POINT ( 'NONE',  ( -22.98253258309999936, 1410.218983115129959, 210.7724375874179827 ) ) ;
#11137=CARTESIAN_POINT ( 'NONE',  ( -18.68654022863783126, 1509.565608751230002, 231.3997216384849480 ) ) ;
#11138=CARTESIAN_POINT ( 'NONE',  ( 18.88590846800000023, 1410.068559083629907, 195.4829271619979920 ) ) ;
#11139=CARTESIAN_POINT ( 'NONE',  ( 22.60520531310000081, 1410.200391392630081, 207.0451948584779984 ) ) ;
#11140=CARTESIAN_POINT ( 'NONE',  ( 17.59268502629999631, 1410.455475180429858, 224.8086594958979845 ) ) ;
#11141=CARTESIAN_POINT ( 'NONE',  ( 1.853755023460000206, 1417.534146448229876, 234.9926947069979803 ) ) ;
#11142=CARTESIAN_POINT ( 'NONE',  ( -22.81609663431766322, 1432.397462965666591, 215.5375287057428864 ) ) ;
#11143=DIRECTION ( 'NONE',  ( 0.000000000000000000, 0.000000000000000000, 1.000000000000000000 ) ) ;
#11148=CARTESIAN_POINT ( 'NONE',  ( -11.03307619032269926, 1509.369276855707540, 181.1467085314911571 ) ) ;
#11150=CARTESIAN_POINT ( 'NONE',  ( -0.4197533444684409809, 1409.214796873330215, 232.6058533239929886 ) ) ;
#11155=CARTESIAN_POINT ( 'NONE',  ( -36.91771901113230570, 1449.587085128020135, 136.2865250079899795 ) ) ;
#11158=CARTESIAN_POINT ( 'NONE',  ( -9.562842729590000701, 1454.397736416729913, 219.6133831120980062 ) ) ;
#11159=CARTESIAN_POINT ( 'NONE',  ( -2.151425146572340186, 1458.408547725810195, 184.2393776212050227 ) ) ;
#11160=CARTESIAN_POINT ( 'NONE',  ( 11.85372112360000152, 1433.007143084950030, 150.3176596395979914 ) ) ;
#11161=CARTESIAN_POINT ( 'NONE',  ( -10.02643927592029982, 1473.539698929279893, 270.1204779540980212 ) ) ;
#11168=EDGE_CURVE ( 'NONE', #84761, #83948, #9721, .T. ) ;
#11169=CARTESIAN_POINT ( 'NONE',  ( -5.863845177379999996, 1486.251790869430124, 182.2701570709980103 ) ) ;
#11170=CARTESIAN_POINT ( 'NONE',  ( 6.114550669599164046, 1398.094264554022629, 197.6339483949746523 ) ) ;
#11173=CARTESIAN_POINT ( 'NONE',  ( 26.05067190899999829, 1469.243640230129813, 211.9776772231579969 ) ) ;
#11175=CARTESIAN_POINT ( 'NONE',  ( -18.11157307520000259, 1509.545530455829976, 231.7129770453979916 ) ) ;
#11178=CARTESIAN_POINT ( 'NONE',  ( 9.630115647840000292, 1408.206715791229954, 218.8876307819480189 ) ) ;
#11180=CARTESIAN_POINT ( 'NONE',  ( 0.1641804351734459932, 1483.764984357220101, 181.9326469513949860 ) ) ;
#11183=CARTESIAN_POINT ( 'NONE',  ( -28.84486411959998975, 1445.052233488288948, 176.6843673542979332 ) ) ;
#11186=CARTESIAN_POINT ( 'NONE',  ( -34.05830400111539547, 1451.723718204009856, 134.0999999980979851 ) ) ;
#11187=ORIENTED_EDGE ( 'NONE', *, *, #40476, .T. ) ;
#11193=CARTESIAN_POINT ( 'NONE',  ( -11.60004869885203682, 1426.786830457828273, 134.3786150874268799 ) ) ;
#11196=CARTESIAN_POINT ( 'NONE',  ( 13.63037056512779976, 1409.389043413630134, 215.2370763268489782 ) ) ;
#11199=CARTESIAN_POINT ( 'NONE',  ( -17.91710591500000049, 1430.610093325130038, 191.6993286258980049 ) ) ;
#11203=ORIENTED_EDGE ( 'NONE', *, *, #42023, .T. ) ;
#11206=CARTESIAN_POINT ( 'NONE',  ( -11.82816149695419838, 1415.492117401590122, 195.0961401479450217 ) ) ;
#11209=CARTESIAN_POINT ( 'NONE',  ( 30.32292150136714071, 1462.007245838464087, 269.4743000939319018 ) ) ;
#11211=CARTESIAN_POINT ( 'NONE',  ( 1.248675305699999960, 1397.026872654030058, 221.9424282998979834 ) ) ;
#11213=CARTESIAN_POINT ( 'NONE',  ( 18.34590456075850184, 1416.851343895820037, 209.3831232368769975 ) ) ;
#11214=CARTESIAN_POINT ( 'NONE',  ( 0.1921617888820000009, 1467.451472553630083, 182.6332811564979863 ) ) ;
#11216=CARTESIAN_POINT ( 'NONE',  ( -19.52793969879499869, 1443.814312415009908, 208.8557621776470228 ) ) ;
#11218=B_SPLINE_CURVE_WITH_KNOTS ( 'NONE', 3,
 ( #26367, #19622, #60563, #94682, #17955, #74335, #83259, #31745, #73779, #23341, #71739, #41260, #6554 ),
 .UNSPECIFIED., .F., .F.,
 ( 4, 3, 3, 3, 4 ),
 ( 12.29943287511600047, 12.57667482080269927, 12.78275953180000002, 13.14531714606529889, 13.22332100184470072 ),
 .UNSPECIFIED. ) ;
#11220=CARTESIAN_POINT ( 'NONE',  ( -12.92312651603950080, 1435.712930329199935, 150.6986646158220253 ) ) ;
#11221=CARTESIAN_POINT ( 'NONE',  ( 0.9041354861050000524, 1416.839648759230158, 190.2140800323980159 ) ) ;
#11226=CARTESIAN_POINT ( 'NONE',  ( 41.51802785006640306, 1444.090987553060131, 136.2824697322219833 ) ) ;
#11227=ORIENTED_EDGE ( 'NONE', *, *, #98140, .F. ) ;
#11228=CARTESIAN_POINT ( 'NONE',  ( 44.59183228759999906, 1432.587449243339961, 266.2372568909979691 ) ) ;
#11229=CARTESIAN_POINT ( 'NONE',  ( -25.96988284309999884, 1469.243118074230097, 205.9471369671879870 ) ) ;
#11230=CARTESIAN_POINT ( 'NONE',  ( -9.958863145267260464, 1425.240638064680070, 91.95675206801159618 ) ) ;
#11231=CARTESIAN_POINT ( 'NONE',  ( 13.53550618839999942, 1416.067629290630066, 196.4934937118979974 ) ) ;
#11233=FACE_OUTER_BOUND ( 'NONE', #12076, .T. ) ;
#11234=CARTESIAN_POINT ( 'NONE',  ( -22.11712025940000004, 1419.857860618830045, 248.4077083964980091 ) ) ;
#11236=CARTESIAN_POINT ( 'NONE',  ( 44.93136303390000563, 1440.913033067569813, 269.6838066906980202 ) ) ;
#11238=CARTESIAN_POINT ( 'NONE',  ( 32.73687873290000283, 1450.481804922550054, 136.2800402082980042 ) ) ;
#11239=EDGE_LOOP ( 'NONE', ( #34490, #27448, #16640, #89742 ) ) ;
#11242=EDGE_CURVE ( 'NONE', #99690, #97372, #64907, .T. ) ;
#11243=CARTESIAN_POINT ( 'NONE',  ( 8.749060160640000916, 1509.218584300429939, 237.3209794345979731 ) ) ;
#11245=ORIENTED_EDGE ( 'NONE', *, *, #7783, .T. ) ;
#11247=CARTESIAN_POINT ( 'NONE',  ( -24.08061883806700010, 1410.858032682979911, 208.7043793227939830 ) ) ;
#11248=ORIENTED_EDGE ( 'NONE', *, *, #84962, .T. ) ;
#11249=CARTESIAN_POINT ( 'NONE',  ( 0.2236527445229999911, 1424.317476911029871, 227.5167485599979784 ) ) ;
#11252=CARTESIAN_POINT ( 'NONE',  ( -11.98374141780000102, 1442.037920581979961, 187.4992083556979878 ) ) ;
#11253=CARTESIAN_POINT ( 'NONE',  ( -2.550769027769999919, 1470.484038555629922, 235.3001169919980100 ) ) ;
#11254=CARTESIAN_POINT ( 'NONE',  ( 0.2538829723067779764, 1420.503732877419907, 182.7635795570130028 ) ) ;
#11256=CARTESIAN_POINT ( 'NONE',  ( 45.84258480992210139, 1442.785980012289883, 266.4134452310810275 ) ) ;
#11262=CARTESIAN_POINT ( 'NONE',  ( 11.86387080397740057, 1432.180192431070054, 149.9801236115920062 ) ) ;
#11263=CARTESIAN_POINT ( 'NONE',  ( 13.16682460439568381, 1444.741529113969136, 187.2442499540229903 ) ) ;
#11265=CARTESIAN_POINT ( 'NONE',  ( -1.438891081339280120, 1452.191228260170192, 183.8587004481619829 ) ) ;
#11267=CARTESIAN_POINT ( 'NONE',  ( 7.116648072490000310, 1508.988559591530020, 236.4115320528979964 ) ) ;
#11270=CARTESIAN_POINT ( 'NONE',  ( 0.9761199062051429953, 1408.566078314740025, 270.4290152450159894 ) ) ;
#11275=CARTESIAN_POINT ( 'NONE',  ( 0.02963793501150268836, 1410.197113369034241, 233.2142573394254157 ) ) ;
#11277=CARTESIAN_POINT ( 'NONE',  ( 14.91819045380000119, 1434.994518313960043, 196.0939301745980003 ) ) ;
#11282=CARTESIAN_POINT ( 'NONE',  ( 3.444929437869999500, 1424.916853932230197, 224.8635561661979807 ) ) ;
#11290=CARTESIAN_POINT ( 'NONE',  ( -24.35304516410000275, 1443.448750497869923, 211.2141737005680113 ) ) ;
#11294=CARTESIAN_POINT ( 'NONE',  ( 5.369445160534993988, 1422.349658812444204, 139.4596679017404881 ) ) ;
#11295=CARTESIAN_POINT ( 'NONE',  ( 27.15098025384490299, 1509.861193510510248, 222.4858292230849770 ) ) ;
#11296=B_SPLINE_CURVE_WITH_KNOTS ( 'NONE', 3,
 ( #39732, #100186, #58196, #73898 ),
 .UNSPECIFIED., .F., .F.,
 ( 4, 4 ),
 ( 0.000000000000000000, 1.000000000000000000 ),
 .UNSPECIFIED. ) ;
#11298=CARTESIAN_POINT ( 'NONE',  ( -8.407921469289998839, 1475.513060387329915, 228.4380765505979980 ) ) ;
#11299=CARTESIAN_POINT ( 'NONE',  ( 13.58451889480000041, 1417.422108894029861, 228.5739723679979818 ) ) ;
#11301=CARTESIAN_POINT ( 'NONE',  ( -17.14943359400000134, 1460.897694268729992, 228.2718315504980069 ) ) ;
#11303=CARTESIAN_POINT ( 'NONE',  ( 45.70279908820000259, 1434.850533281740127, 267.6096423418979953 ) ) ;
#11304=CARTESIAN_POINT ( 'NONE',  ( -18.68376360200000263, 1410.488798158429972, 223.5328836508979862 ) ) ;
#11305=CARTESIAN_POINT ( 'NONE',  ( 22.16387887220000152, 1435.699526443600007, 142.3412916024980177 ) ) ;
#11306=CARTESIAN_POINT ( 'NONE',  ( 22.45934772189999862, 1508.010250242130269, 192.8395958341980077 ) ) ;
#11307=CARTESIAN_POINT ( 'NONE',  ( 29.34113783274351306, 1509.937680645843329, 206.7119583629535953 ) ) ;
#11309=CARTESIAN_POINT ( 'NONE',  ( -42.07524608051735271, 1455.849907682117873, 266.2935988973322310 ) ) ;
#11311=CARTESIAN_POINT ( 'NONE',  ( -40.26705548447760208, 1440.962086013470071, 136.8039402764729857 ) ) ;
#11312=LINE ( 'NONE', #27547, #99761 ) ;
#11314=CARTESIAN_POINT ( 'NONE',  ( -17.60627216660330063, 1410.895669502700230, 193.4350316886979897 ) ) ;
#11316=CARTESIAN_POINT ( 'NONE',  ( -32.75718327559999921, 1435.641353515060018, 135.5388831429980030 ) ) ;
#11317=CARTESIAN_POINT ( 'NONE',  ( -7.978005036616639956, 1456.316316171971948, 227.3102628134479630 ) ) ;
#11318=VERTEX_POINT ( 'NONE', #56495 ) ;
#11320=CARTESIAN_POINT ( 'NONE',  ( -9.846997683718040406, 1409.256925123650035, 220.3815847126709855 ) ) ;
#11323=CARTESIAN_POINT ( 'NONE',  ( -3.280536648517546894, 1420.304670650970138, 137.1408270732875110 ) ) ;
#11324=CARTESIAN_POINT ( 'NONE',  ( -26.80974433740000151, 1468.951693103129855, 269.2446796842979779 ) ) ;
#11326=CARTESIAN_POINT ( 'NONE',  ( 0.3958445684936310327, 1418.988079762759980, 184.6579903234699884 ) ) ;
#11329=B_SPLINE_SURFACE_WITH_KNOTS ( 'NONE', 5, 1, ( 
 ( #105232, #71676 ),
 ( #20108, #10057 ),
 ( #105795, #19554 ),
 ( #45890, #86767 ),
 ( #54301, #3348 ),
 ( #103562, #2250 ) ),
 .UNSPECIFIED., .F., .F., .F.,
 ( 6, 6 ),
 ( 2, 2 ),
 ( 65.12635869110000897, 66.80154955991109489 ),
 ( 0.6126808583520000351, 3.463904696680000228 ),
 .UNSPECIFIED. ) ;
#11331=DIRECTION ( 'NONE',  ( 0.000000000000000000, 1.000000000000000000, 0.000000000000000000 ) ) ;
#11332=CARTESIAN_POINT ( 'NONE',  ( 20.59437597599999847, 1507.765470465330054, 227.7647620796980164 ) ) ;
#11333=CARTESIAN_POINT ( 'NONE',  ( 14.13195592469999973, 1452.421092192730157, 222.7290593249980191 ) ) ;
#11334=CARTESIAN_POINT ( 'NONE',  ( 2.370970874524633398, 1427.002265528473799, 137.0999999980980135 ) ) ;
#11337=CARTESIAN_POINT ( 'NONE',  ( -24.06753813140000275, 1410.675710981530074, 208.6186337047089978 ) ) ;
#11339=CARTESIAN_POINT ( 'NONE',  ( -12.00387303569999986, 1415.296882282229944, 195.7718046162979704 ) ) ;
#11342=CARTESIAN_POINT ( 'NONE',  ( 22.72019863759999936, 1409.706467206729940, 211.0465802060780049 ) ) ;
#11345=CARTESIAN_POINT ( 'NONE',  ( -5.366470797799430592, 1426.055677132399978, 152.4431534743949896 ) ) ;
#11346=CARTESIAN_POINT ( 'NONE',  ( -11.86547436779999920, 1432.299056944690165, 150.3973009728979946 ) ) ;
#11352=B_SPLINE_CURVE_WITH_KNOTS ( 'NONE', 3,
 ( #90642, #30741, #73309, #88992, #12837, #81142, #47017, #89548, #74429, #13369, #12280, #47558, #100154, #64922, #91201, #48674, #23439, #4457, #72764, #30179, #107995, #73867, #99035, #21205, #106891, #63824, #6093, #22312, #31292, #64371, #97937, #5551, #82250, #13925, #65476, #99585, #40246, #48112, #39701, #46474, #57077, #80606, #3921, #38051, #4986, #72228, #106352, #98494, #29638, #55414, #21762, #90086, #81680, #39130, #67682, #68244, #110206, #77179, #41363, #110762, #482 ),
 .UNSPECIFIED., .F., .F.,
 ( 4, 3, 3, 3, 3, 3, 3, 3, 3, 3, 3, 3, 3, 3, 3, 3, 3, 3, 3, 3, 4 ),
 ( -166.9410549240000137, -166.6317463252630091, -165.1629312876659981, -163.7366513399680059, -162.3365470994540090, -160.9755933037990019, -159.6378003704959951, -158.3210010880789866, -157.0233722586470151, -156.3417070556260171, -154.7029146182070178, -153.0275451752820004, -151.3241472847070099, -149.5649634833510220, -147.7605963360979899, -145.9029318570200076, -143.9806754146449919, -141.9771156308089815, -139.8276503982599763, -137.3711187039190236, -134.5636539103869893 ),
 .UNSPECIFIED. ) ;
#11353=CARTESIAN_POINT ( 'NONE',  ( -23.14270888800000137, 1415.981602844629833, 211.1002275068279914 ) ) ;
#11355=EDGE_CURVE ( 'NONE', #9890, #758, #2800, .T. ) ;
#11357=CARTESIAN_POINT ( 'NONE',  ( -19.24890086970000169, 1426.049025734429961, 226.0195547209980305 ) ) ;
#11358=CARTESIAN_POINT ( 'NONE',  ( -19.02807259538449713, 1485.647960197060002, 189.5790945604939850 ) ) ;
#11363=EDGE_CURVE ( 'NONE', #25815, #4737, #69839, .T. ) ;
#11365=CARTESIAN_POINT ( 'NONE',  ( 28.87050041479999862, 1509.923266469329747, 215.0239930259780010 ) ) ;
#11366=EDGE_LOOP ( 'NONE', ( #32457, #79960, #104344, #85651 ) ) ;
#11369=CARTESIAN_POINT ( 'NONE',  ( 1.608351468689999786, 1426.598937817530214, 144.1938086916980239 ) ) ;
#11370=CARTESIAN_POINT ( 'NONE',  ( 22.30619483830000149, 1451.363309493629913, 221.4011829164979872 ) ) ;
#11371=CARTESIAN_POINT ( 'NONE',  ( -0.7176848839889999887, 1417.283279384530033, 235.8571367780980097 ) ) ;
#11372=CARTESIAN_POINT ( 'NONE',  ( -24.97479332202350122, 1451.884380675330021, 136.4887619541970025 ) ) ;
#11374=CARTESIAN_POINT ( 'NONE',  ( 13.47403807739999948, 1410.316254106229962, 228.2920107387979840 ) ) ;
#11376=CARTESIAN_POINT ( 'NONE',  ( 40.21460569533279994, 1439.107902997649944, 134.0999999981339954 ) ) ;
#11378=CARTESIAN_POINT ( 'NONE',  ( -0.5656601614563600000, 1424.194575819369902, 228.0927458373740251 ) ) ;
#11383=VERTEX_POINT ( 'NONE', #46455 ) ;
#11386=CARTESIAN_POINT ( 'NONE',  ( -1.835915931920000022, 1464.997577601130160, 237.8268836853979735 ) ) ;
#11387=CARTESIAN_POINT ( 'NONE',  ( 20.24763625415679513, 1450.973946380246161, 145.3523280452958488 ) ) ;
#11388=CARTESIAN_POINT ( 'NONE',  ( -3.043465616510000249, 1485.522934885530049, 182.9100814775980268 ) ) ;
#11390=ADVANCED_FACE ( 'NONE', ( #3903 ), #55397, .F. ) ;
#11392=CARTESIAN_POINT ( 'NONE',  ( -17.72975366969933830, 1447.779520654833505, 217.4447075265184139 ) ) ;
#11394=CARTESIAN_POINT ( 'NONE',  ( 4.275908414736929508, 1446.766556631309868, 157.1258821310249800 ) ) ;
#11395=EDGE_CURVE ( 'NONE', #22920, #8770, #79160, .T. ) ;
#11396=CARTESIAN_POINT ( 'NONE',  ( 0.9965953362400000737, 1508.939483211730021, 238.5777243435979926 ) ) ;
#11399=ORIENTED_EDGE ( 'NONE', *, *, #59162, .T. ) ;
#11400=CARTESIAN_POINT ( 'NONE',  ( 28.57350514777099804, 1440.913060387330006, 248.9574316567099856 ) ) ;
#11402=CARTESIAN_POINT ( 'NONE',  ( -14.35518106359999990, 1509.483853030530099, 182.9676315445979924 ) ) ;
#11403=ORIENTED_EDGE ( 'NONE', *, *, #26110, .T. ) ;
#11405=CARTESIAN_POINT ( 'NONE',  ( -14.68857900839999964, 1409.425996869029859, 192.2200297474979891 ) ) ;
#11407=CARTESIAN_POINT ( 'NONE',  ( -24.49620803319999851, 1440.956469628590185, 210.9946876184580162 ) ) ;
#11408=CARTESIAN_POINT ( 'NONE',  ( 0.04987450923691939819, 1450.914802043100053, 185.2444802929140053 ) ) ;
#11409=CARTESIAN_POINT ( 'NONE',  ( 22.39828147038580397, 1410.488771300080089, 206.2224881104899907 ) ) ;
#11411=CARTESIAN_POINT ( 'NONE',  ( 25.91590772989999891, 1441.261220175949802, 138.4451201509980365 ) ) ;
#11414=CARTESIAN_POINT ( 'NONE',  ( 10.13643151279999977, 1462.749890840729904, 234.3975521353980014 ) ) ;
#11417=CARTESIAN_POINT ( 'NONE',  ( 11.73709356406289928, 1426.695943121369965, 144.1748013758129900 ) ) ;
#11425=CARTESIAN_POINT ( 'NONE',  ( -0.7692391029760000665, 1415.628674266529742, 227.3871686175980074 ) ) ;
#11426=CARTESIAN_POINT ( 'NONE',  ( 17.31784991639999660, 1457.605539162629839, 225.7849821470979919 ) ) ;
#11429=CARTESIAN_POINT ( 'NONE',  ( 2.421990954390000006, 1414.535087205929813, 231.9310730028979890 ) ) ;
#11430=CARTESIAN_POINT ( 'NONE',  ( -18.84860651810000221, 1456.786630790930076, 228.5413354239980208 ) ) ;
#11431=CARTESIAN_POINT ( 'NONE',  ( -21.75307144610911791, 1411.033070506304966, 201.6242908587096565 ) ) ;
#11432=CARTESIAN_POINT ( 'NONE',  ( 19.24021961950000303, 1455.885573259829926, 225.9459216509980024 ) ) ;
#11435=ORIENTED_EDGE ( 'NONE', *, *, #56421, .T. ) ;
#11437=CARTESIAN_POINT ( 'NONE',  ( 1.312236371940000090, 1406.790645662230190, 269.6495478408979807 ) ) ;
#11439=CARTESIAN_POINT ( 'NONE',  ( 31.30797101508039759, 1465.106566905469890, 270.3267909516169993 ) ) ;
#11440=CARTESIAN_POINT ( 'NONE',  ( 2.477972021390000279, 1440.426960907559987, 157.8055583485979980 ) ) ;
#11441=CARTESIAN_POINT ( 'NONE',  ( 10.43902076892678288, 1423.422239459952834, 137.2931753684112550 ) ) ;
#11442=CARTESIAN_POINT ( 'NONE',  ( -39.96238005862740295, 1440.913060402280053, 259.2337657365459904 ) ) ;
#11443=CARTESIAN_POINT ( 'NONE',  ( -26.25855011770000047, 1449.905647651959953, 136.7332828859979941 ) ) ;
#11446=CARTESIAN_POINT ( 'NONE',  ( 1.747352932607996179, 1465.628108031464308, 235.0395402516389822 ) ) ;
#11448=CARTESIAN_POINT ( 'NONE',  ( 17.45961317077569674, 1413.562297865003075, 192.3730989426080669 ) ) ;
#11449=ORIENTED_EDGE ( 'NONE', *, *, #7124, .F. ) ;
#11450=CARTESIAN_POINT ( 'NONE',  ( -19.47651264659999626, 1426.266543402430216, 243.9198229517980110 ) ) ;
#11454=CARTESIAN_POINT ( 'NONE',  ( -0.8852285261829999641, 1475.753581647529927, 269.0453912508980352 ) ) ;
#11455=CARTESIAN_POINT ( 'NONE',  ( -4.272885081469669721, 1446.730020358119873, 157.5808617883949978 ) ) ;
#11456=CARTESIAN_POINT ( 'NONE',  ( -28.44347337880000381, 1509.158830949329968, 209.7035872210599905 ) ) ;
#11457=CARTESIAN_POINT ( 'NONE',  ( -2.774022723599062878, 1448.257693116544715, 184.1777864073213493 ) ) ;
#11461=CARTESIAN_POINT ( 'NONE',  ( -18.46483594369999892, 1415.628674276729953, 207.5691869113279893 ) ) ;
#11463=CARTESIAN_POINT ( 'NONE',  ( 26.57248659439540006, 1436.418273096599933, 136.7276480538729970 ) ) ;
#11464=( BOUNDED_SURFACE ( )  B_SPLINE_SURFACE ( 1, 2, ( 
 ( #87864, #70525, #36329, #36884, #27938, #62120, #46418, #28491, #104086 ),
 ( #18960, #45315, #2763, #37444, #103528, #78910, #61560, #80550, #35788 ) ),
 .UNSPECIFIED., .F., .T., .F. ) 
 B_SPLINE_SURFACE_WITH_KNOTS ( ( 2, 2 ),
 ( 3, 2, 2, 2, 3 ),
 ( -10000.00000000000000, 10000.00000000000000 ),
 ( 0.000000000000000000, 1.570796326794899889, 3.141592653589790007, 4.712388980384689674, 6.283185307179590673 ),
 .UNSPECIFIED. ) 
 GEOMETRIC_REPRESENTATION_ITEM ( )  RATIONAL_B_SPLINE_SURFACE ( (
 ( 1.000000000000000000, 0.7071067811865480168, 1.000000000000000000, 0.7071067811865480168, 1.000000000000000000, 0.7071067811865480168, 1.000000000000000000, 0.7071067811865480168, 1.000000000000000000),
 ( 1.000000000000000000, 0.7071067811865480168, 1.000000000000000000, 0.7071067811865480168, 1.000000000000000000, 0.7071067811865480168, 1.000000000000000000, 0.7071067811865480168, 1.000000000000000000) ) ) 
 REPRESENTATION_ITEM ( '' )  SURFACE ( )  );
#11465=CARTESIAN_POINT ( 'NONE',  ( -9.494076726826639501, 1396.244600852259964, 214.8009319264149894 ) ) ;
#11466=CARTESIAN_POINT ( 'NONE',  ( -15.08655487470000089, 1422.047410306030088, 227.7513007382979993 ) ) ;
#11468=CARTESIAN_POINT ( 'NONE',  ( 2.500000000000000000, 1443.913060387330006, 150.6726614421979775 ) ) ;
#11471=CARTESIAN_POINT ( 'NONE',  ( 2.643999269920000117, 1409.509886378629972, 231.4605033490980190 ) ) ;
#11472=CARTESIAN_POINT ( 'NONE',  ( -16.30638770610000066, 1484.820604609629981, 187.8396872195979768 ) ) ;
#11473=CARTESIAN_POINT ( 'NONE',  ( 10.83435298340000053, 1425.666604291029898, 103.4417286516979999 ) ) ;
#11475=FACE_OUTER_BOUND ( 'NONE', #88696, .T. ) ;
#11476=CARTESIAN_POINT ( 'NONE',  ( -12.37499353609999986, 1442.762691980110048, 151.6327898328030130 ) ) ;
#11480=CARTESIAN_POINT ( 'NONE',  ( 4.349085017430000200, 1508.966281798729824, 180.4853875712980198 ) ) ;
#11485=CARTESIAN_POINT ( 'NONE',  ( -11.45446813149230003, 1462.185551532946420, 233.9517320718034625 ) ) ;
#11488=ADVANCED_FACE ( 'NONE', ( #83880 ), #84440, .F. ) ;
#11490=CARTESIAN_POINT ( 'NONE',  ( -12.41103214550000011, 1409.346463180030014, 190.9867524833979928 ) ) ;
#11494=CARTESIAN_POINT ( 'NONE',  ( -2.783288780519999950, 1486.112700186630036, 181.9037838507979927 ) ) ;
#11498=CARTESIAN_POINT ( 'NONE',  ( -41.04864394093900160, 1445.151157643809938, 136.7380822686889985 ) ) ;
#11499=CARTESIAN_POINT ( 'NONE',  ( -2.500000000000000000, 1448.592472799309917, 159.2571715835509849 ) ) ;
#11500=CARTESIAN_POINT ( 'NONE',  ( -12.99570043321834589, 1434.780757546461246, 149.5535408288678241 ) ) ;
#11501=CARTESIAN_POINT ( 'NONE',  ( -28.11559569040000284, 1443.570698335159932, 137.5389433187979762 ) ) ;
#11502=CARTESIAN_POINT ( 'NONE',  ( -3.789557337974839957, 1406.612116051730027, 269.4941210699120120 ) ) ;
#11503=CARTESIAN_POINT ( 'NONE',  ( 40.27287714639999905, 1443.726400947989987, 137.1298442681979850 ) ) ;
#11504=VERTEX_POINT ( 'NONE', #67110 ) ;
#11508=VERTEX_POINT ( 'NONE', #93378 ) ;
#11520=CARTESIAN_POINT ( 'NONE',  ( -41.37929305821487702, 1435.466738718876059, 269.6357249460477306 ) ) ;
#11522=CARTESIAN_POINT ( 'NONE',  ( -5.081689812120000482, 1409.257665803229884, 231.2512572095979806 ) ) ;
#11523=CARTESIAN_POINT ( 'NONE',  ( -4.080430317250000272, 1447.666642389649951, 185.0612220870980025 ) ) ;
#11524=ORIENTED_EDGE ( 'NONE', *, *, #17257, .T. ) ;
#11525=CARTESIAN_POINT ( 'NONE',  ( -12.53380499169999851, 1445.052233488290085, 177.5748921271979839 ) ) ;
#11526=CARTESIAN_POINT ( 'NONE',  ( -26.09031900081160060, 1440.913060473340011, 222.3459699190599963 ) ) ;
#11529=CARTESIAN_POINT ( 'NONE',  ( 21.02608924029999926, 1456.853724928630072, 225.6706377209980303 ) ) ;
#11530=CARTESIAN_POINT ( 'NONE',  ( 39.81566866050809494, 1428.288687989800110, 270.1753679354689552 ) ) ;
#11533=VECTOR ( 'NONE', #14759, 1000.000000000000000 ) ;
#11534=CARTESIAN_POINT ( 'NONE',  ( 0.01782758894743981942, 1507.551620162875224, 237.4204223254480155 ) ) ;
#11536=CARTESIAN_POINT ( 'NONE',  ( 18.96076900870300008, 1410.937160519182044, 195.1859992452610300 ) ) ;
#11539=CARTESIAN_POINT ( 'NONE',  ( 2.500000000000000000, 1436.420121157869971, 157.6233376561979753 ) ) ;
#11540=CARTESIAN_POINT ( 'NONE',  ( -10.30053490859999954, 1417.902178291030168, 229.8560290380979723 ) ) ;
#11541=CARTESIAN_POINT ( 'NONE',  ( 5.940759646534202076, 1420.421523195163218, 137.0999999980978146 ) ) ;
#11545=CARTESIAN_POINT ( 'NONE',  ( 18.64722824082740260, 1478.712861779200011, 228.5761396551030202 ) ) ;
#11546=CARTESIAN_POINT ( 'NONE',  ( 19.08918182269999875, 1507.695925188030060, 188.5883432463980114 ) ) ;
#11549=CARTESIAN_POINT ( 'NONE',  ( 0.1036083437597169893, 1420.454746905719958, 182.6982413274450039 ) ) ;
#11552=CARTESIAN_POINT ( 'NONE',  ( 19.28393622879999825, 1507.737928638330004, 188.6540313642980209 ) ) ;
#11555=CARTESIAN_POINT ( 'NONE',  ( -12.84940689358420052, 1416.524489948229984, 196.3858981729360096 ) ) ;
#11556=CARTESIAN_POINT ( 'NONE',  ( -0.7339482261329999258, 1499.713796587029947, 181.0788772114979963 ) ) ;
#11559=DIRECTION ( 'NONE',  ( 0.000000000000000000, -5.238603995039999762E-10, -1.000000000000000000 ) ) ;
#11563=CARTESIAN_POINT ( 'NONE',  ( 16.31271465393231068, 1421.545148970794116, 227.2409568857196689 ) ) ;
#11564=LINE ( 'NONE', #48910, #42464 ) ;
#11566=CARTESIAN_POINT ( 'NONE',  ( -17.61522799909999648, 1423.733526167929767, 226.4046865996980102 ) ) ;
#11567=CARTESIAN_POINT ( 'NONE',  ( -15.45606833479999942, 1435.037147414750052, 147.9572051551980110 ) ) ;
#11568=CARTESIAN_POINT ( 'NONE',  ( 4.363122647530000009, 1409.354802298930053, 146.1721969590979882 ) ) ;
#11569=CARTESIAN_POINT ( 'NONE',  ( 16.57268409019999922, 1413.521687218830039, 191.5369357848979917 ) ) ;
#11570=CARTESIAN_POINT ( 'NONE',  ( 1.354644225578049976, 1409.895065699369752, 232.6225702936600044 ) ) ;
#11576=CARTESIAN_POINT ( 'NONE',  ( -24.23130831839999999, 1437.896962395750052, 211.0914046272980045 ) ) ;
#11578=CARTESIAN_POINT ( 'NONE',  ( -18.59400683710000024, 1508.850372359329867, 229.9901379698980008 ) ) ;
#11580=CARTESIAN_POINT ( 'NONE',  ( 18.71266994490000002, 1408.913060387329779, 210.0964815640089682 ) ) ;
#11581=B_SPLINE_SURFACE_WITH_KNOTS ( 'NONE', 5, 5, ( 
 ( #20254, #104827, #11873, #62304, #28113, #95324 ),
 ( #80177, #77966, #1274, #70165, #35413, #11332 ),
 ( #79645, #3493, #46045, #61748, #36520, #2402 ),
 ( #2947, #71824, #105944, #19136, #53340, #70713 ),
 ( #86364, #103719, #27021, #61210, #4038, #38166 ),
 ( #72347, #30310, #99704, #106476, #98616, #21879 ) ),
 .UNSPECIFIED., .F., .F., .F.,
 ( 6, 6 ),
 ( 6, 6 ),
 ( 4.813401939820000308, 5.109425210320000410 ),
 ( 0.000000000000000000, 2.000000000000000000 ),
 .UNSPECIFIED. ) ;
#11583=CARTESIAN_POINT ( 'NONE',  ( -14.10735888110919944, 1509.405700215120078, 183.4262508031069956 ) ) ;
#11590=CARTESIAN_POINT ( 'NONE',  ( 20.32974505740000026, 1508.870382120730028, 189.2250245169979905 ) ) ;
#11593=CARTESIAN_POINT ( 'NONE',  ( -0.6434364284315916560, 1417.244662098927847, 234.6835996158768864 ) ) ;
#11596=CARTESIAN_POINT ( 'NONE',  ( 12.70666910289999940, 1441.123310893239932, 188.6801198206979961 ) ) ;
#11597=CARTESIAN_POINT ( 'NONE',  ( 13.87302018090000111, 1509.389573182929780, 234.2955351351979800 ) ) ;
#11599=CARTESIAN_POINT ( 'NONE',  ( 41.15573334512143333, 1434.647116362632005, 269.6315103028593398 ) ) ;
#11600=CARTESIAN_POINT ( 'NONE',  ( -29.81189556660000051, 1458.385315375329810, 254.8364576145980038 ) ) ;
#11606=CARTESIAN_POINT ( 'NONE',  ( 6.453500081109999620, 1409.641075296729923, 187.1560900367980196 ) ) ;
#11609=CARTESIAN_POINT ( 'NONE',  ( -10.83341047090000053, 1434.513252305289825, 151.9041012880979906 ) ) ;
#11610=DIRECTION ( 'NONE',  ( 0.000000000000000000, 1.000000000000000000, 0.000000000000000000 ) ) ;
#11612=AXIS2_PLACEMENT_3D ( 'NONE', #51948, #93374, #84968 ) ;
#11613=CARTESIAN_POINT ( 'NONE',  ( -19.40246366119999877, 1452.235511427830033, 144.9801693602979640 ) ) ;
#11616=EDGE_LOOP ( 'NONE', ( #34097, #91233, #54486, #103055, #21866, #102196 ) ) ;
#11619=CARTESIAN_POINT ( 'NONE',  ( -29.18142758420000149, 1466.479558604430167, 269.9486951468979896 ) ) ;
#11620=CARTESIAN_POINT ( 'NONE',  ( -23.91170749936344464, 1435.927394111685089, 211.3044503123053914 ) ) ;
#11621=CARTESIAN_POINT ( 'NONE',  ( 11.94206337009999963, 1438.199233188169956, 150.9847479746979957 ) ) ;
#11622=CARTESIAN_POINT ( 'NONE',  ( -23.10442739037580040, 1411.095127590459924, 210.9251608898400150 ) ) ;
#11624=CARTESIAN_POINT ( 'NONE',  ( 18.48251015503148764, 1457.399406872058989, 229.7677033836061185 ) ) ;
#11627=CARTESIAN_POINT ( 'NONE',  ( -45.36516505088270179, 1434.423077423250106, 268.2311484050200079 ) ) ;
#11633=CARTESIAN_POINT ( 'NONE',  ( -20.86040077539999871, 1508.959081886430113, 190.3921826422979962 ) ) ;
#11634=CARTESIAN_POINT ( 'NONE',  ( -15.31473337059999906, 1410.405885239830013, 190.9489869040980068 ) ) ;
#11635=CARTESIAN_POINT ( 'NONE',  ( -24.89775034519999863, 1442.835538705840008, 210.5176537872779932 ) ) ;
#11637=CARTESIAN_POINT ( 'NONE',  ( 0.4834647446390000214, 1450.896177426419854, 181.9315483554979949 ) ) ;
#11638=CIRCLE ( 'NONE', #104594, 4.941741911590025182 ) ;
#11640=DIRECTION ( 'NONE',  ( 0.03489949670244908014, -0.9993908270190976495, 0.000000000000000000 ) ) ;
#11644=CARTESIAN_POINT ( 'NONE',  ( -9.792171405701560971, 1409.347304102430144, 270.4184784957810734 ) ) ;
#11646=CARTESIAN_POINT ( 'NONE',  ( 3.519941190947349696, 1417.854933870999957, 233.1899663063400112 ) ) ;
#11650=ORIENTED_EDGE ( 'NONE', *, *, #35181, .F. ) ;
#11651=CARTESIAN_POINT ( 'NONE',  ( 45.58093450282833459, 1442.609263607555022, 268.9762866484336996 ) ) ;
#11654=CARTESIAN_POINT ( 'NONE',  ( 3.628618679598039076, 1424.505256609078970, 184.4894892356298328 ) ) ;
#11655=CARTESIAN_POINT ( 'NONE',  ( -0.001500122192890200124, 1408.913112772820114, 186.4349499642330272 ) ) ;
#11657=CARTESIAN_POINT ( 'NONE',  ( -18.68599070930379824, 1416.029511582830082, 207.5720217176579752 ) ) ;
#11658=CARTESIAN_POINT ( 'NONE',  ( 2.500000000000000000, 1439.114301455650093, 157.7261946041980138 ) ) ;
#11659=CARTESIAN_POINT ( 'NONE',  ( -14.30536636630000125, 1420.164009348430000, 221.8419782042979875 ) ) ;
#11660=CARTESIAN_POINT ( 'NONE',  ( 12.60885230210000074, 1416.021639796329964, 222.8465216075979924 ) ) ;
#11661=CARTESIAN_POINT ( 'NONE',  ( 9.350144766380001471, 1445.503299043049992, 184.2959263576980220 ) ) ;
#11663=ORIENTED_EDGE ( 'NONE', *, *, #71431, .F. ) ;
#11665=CARTESIAN_POINT ( 'NONE',  ( 1.513134720104279962, 1459.713768463400129, 183.1823380342580094 ) ) ;
#11666=ORIENTED_EDGE ( 'NONE', *, *, #45955, .T. ) ;
#11667=CARTESIAN_POINT ( 'NONE',  ( 17.79624440539630470, 1458.182673695933318, 228.6901989447007679 ) ) ;
#11668=CARTESIAN_POINT ( 'NONE',  ( 24.26879693951600103, 1452.060463742079946, 136.4940726181909838 ) ) ;
#11669=CARTESIAN_POINT ( 'NONE',  ( 16.19492570339999915, 1409.478599654730033, 224.8086529783979870 ) ) ;
#11672=CARTESIAN_POINT ( 'NONE',  ( 21.49042858359999641, 1409.827641821229918, 203.4051265432880200 ) ) ;
#11673=CARTESIAN_POINT ( 'NONE',  ( 12.29654148988069373, 1445.052233488290085, 164.4841150006940325 ) ) ;
#11674=CARTESIAN_POINT ( 'NONE',  ( 3.356639108386120895, 1439.689563386633836, 184.4108225802596053 ) ) ;
#11676=CARTESIAN_POINT ( 'NONE',  ( 21.67251142306619016, 1453.432672215584944, 220.8666736850036614 ) ) ;
#11677=CARTESIAN_POINT ( 'NONE',  ( 2.500000000000000000, 1439.481493058779961, 163.2933130068350067 ) ) ;
#11683=CARTESIAN_POINT ( 'NONE',  ( -0.5147827871106269715, 1410.238466821279872, 233.1669068061830217 ) ) ;
#11685=FACE_OUTER_BOUND ( 'NONE', #17840, .T. ) ;
#11688=CARTESIAN_POINT ( 'NONE',  ( -40.06635116240170191, 1445.481206507490015, 136.8845248586889909 ) ) ;
#11692=CARTESIAN_POINT ( 'NONE',  ( 40.83414858899995892, 1456.643249355430044, 266.3275291775977962 ) ) ;
#11693=ADVANCED_FACE ( 'NONE', ( #25613 ), #59805, .F. ) ;
#11694=CARTESIAN_POINT ( 'NONE',  ( 11.87081876380000089, 1433.087150165419871, 150.2039343203979911 ) ) ;
#11695=CARTESIAN_POINT ( 'NONE',  ( -44.92381742691460289, 1442.155912586060140, 269.6913903957949969 ) ) ;
#11696=B_SPLINE_SURFACE_WITH_KNOTS ( 'NONE', 5, 4, ( 
 ( #107388, #37994, #64871, #97877, #89491 ),
 ( #81626, #23377, #90030, #39645, #82186 ),
 ( #106831, #100097, #5485, #30124, #22809 ),
 ( #98436, #29577, #98979, #22253, #46964 ),
 ( #73814, #38529, #81085, #21707, #55912 ),
 ( #107942, #57568, #21154, #31234, #40188 ) ),
 .UNSPECIFIED., .F., .F., .F.,
 ( 6, 6 ),
 ( 5, 5 ),
 ( -0.0001726411652746099863, 52.98902693510000006 ),
 ( 25.78146411700000229, 39.23969207129999859 ),
 .UNSPECIFIED. ) ;
#11697=CARTESIAN_POINT ( 'NONE',  ( -17.84692692827389848, 1410.032954271290237, 195.3924044303319931 ) ) ;
#11702=CARTESIAN_POINT ( 'NONE',  ( -2.343308028451718261, 1485.565572280186416, 182.6780017704854515 ) ) ;
#11703=CARTESIAN_POINT ( 'NONE',  ( 5.527464195969298721, 1398.076716713788755, 197.3337701784347473 ) ) ;
#11704=CARTESIAN_POINT ( 'NONE',  ( 1.921481516869999906, 1474.709560945429985, 234.8855729059979751 ) ) ;
#11705=CARTESIAN_POINT ( 'NONE',  ( 25.55495559159999885, 1449.803351295099901, 210.4363185493679964 ) ) ;
#11707=DIRECTION ( 'NONE',  ( -1.000000000000000000, -1.944759044220000059E-14, -3.085874980950000024E-15 ) ) ;
#11709=AXIS2_PLACEMENT_3D ( 'NONE', #89745, #23072, #5188 ) ;
#11711=CARTESIAN_POINT ( 'NONE',  ( 2.499937872101899661, 1420.083820293880080, 95.10876171418870229 ) ) ;
#11715=CARTESIAN_POINT ( 'NONE',  ( -6.259455327080631015, 1439.877182118289738, 154.4997780959237446 ) ) ;
#11717=CARTESIAN_POINT ( 'NONE',  ( -1.114904039080000020, 1451.704834585230174, 183.4401667605979753 ) ) ;
#11719=CARTESIAN_POINT ( 'NONE',  ( -20.01067139950000140, 1507.877425041529932, 188.9709217985979706 ) ) ;
#11723=VERTEX_POINT ( 'NONE', #15004 ) ;
#11729=ADVANCED_FACE ( 'NONE', ( #1009 ), #75827, .T. ) ;
#11733=CARTESIAN_POINT ( 'NONE',  ( 9.512845714357990090, 1409.245256277939916, 220.6667643274379884 ) ) ;
#11734=CARTESIAN_POINT ( 'NONE',  ( 18.12493657479999953, 1425.163099838030121, 224.8025639441979990 ) ) ;
#11741=CARTESIAN_POINT ( 'NONE',  ( -11.94473499059260213, 1415.666200591949973, 194.9815815898240032 ) ) ;
#11743=CARTESIAN_POINT ( 'NONE',  ( 29.85894071568812080, 1462.352465317911765, 269.4693070817808689 ) ) ;
#11745=CARTESIAN_POINT ( 'NONE',  ( 3.320518013340000074, 1396.029015431430025, 219.7196859380979959 ) ) ;
#11746=CARTESIAN_POINT ( 'NONE',  ( 1.363639811660000145, 1415.765555525229956, 232.8698637559979829 ) ) ;
#11747=CARTESIAN_POINT ( 'NONE',  ( -0.5186190627380000695, 1457.272028348329968, 183.0645885489979889 ) ) ;
#11753=CARTESIAN_POINT ( 'NONE',  ( 0.5624686996209999901, 1416.828044802929981, 190.4759595091980202 ) ) ;
#11759=CARTESIAN_POINT ( 'NONE',  ( 6.248994650120000216, 1409.477337451929998, 259.9484463607980160 ) ) ;
#11760=CARTESIAN_POINT ( 'NONE',  ( -23.81087019679999628, 1469.236087444030090, 199.7892800214279987 ) ) ;
#11761=CARTESIAN_POINT ( 'NONE',  ( -11.01664542227860011, 1426.516231295739999, 91.95526548305120684 ) ) ;
#11763=CARTESIAN_POINT ( 'NONE',  ( 14.38276615812612036, 1514.413060387330006, 235.4493228184091720 ) ) ;
#11764=CARTESIAN_POINT ( 'NONE',  ( -43.48931973434065412, 1430.236537677061960, 269.7109761710999010 ) ) ;
#11765=CARTESIAN_POINT ( 'NONE',  ( 2.451862795619999984E-09, 1414.987262868229891, 244.5742075744979900 ) ) ;
#11767=CARTESIAN_POINT ( 'NONE',  ( 4.291176059336820003, 1446.971469614359876, 154.7965853925720126 ) ) ;
#11768=CARTESIAN_POINT ( 'NONE',  ( -23.30842551276433738, 1409.842257829955088, 208.8031236852703785 ) ) ;
#11778=ORIENTED_EDGE ( 'NONE', *, *, #59297, .T. ) ;
#11779=CARTESIAN_POINT ( 'NONE',  ( 0.4959747488679999705, 1415.645648335029819, 184.8436836604979874 ) ) ;
#11781=EDGE_CURVE ( 'NONE', #99658, #46627, #107438, .T. ) ;
#11782=CARTESIAN_POINT ( 'NONE',  ( 0.4808923648170000398, 1450.896267255910061, 181.2821022293979922 ) ) ;
#11783=CARTESIAN_POINT ( 'NONE',  ( -4.734919033409999756, 1489.058994670830089, 235.5547056775980082 ) ) ;
#11787=FACE_OUTER_BOUND ( 'NONE', #16017, .T. ) ;
#11788=CARTESIAN_POINT ( 'NONE',  ( -13.15726448930059966, 1414.913060387399810, 219.9105443326110105 ) ) ;
#11789=CARTESIAN_POINT ( 'NONE',  ( 14.10003875770000015, 1474.744286201729892, 225.3785174790980079 ) ) ;
#11791=( BOUNDED_CURVE ( )  B_SPLINE_CURVE ( 3, ( #53001, #79298, #36734, #19917 ),
 .UNSPECIFIED., .F., .F. ) 
 B_SPLINE_CURVE_WITH_KNOTS ( ( 4, 4 ),
 ( 0.2461548770693000043, 0.5332284340196910000 ),
 .UNSPECIFIED. ) 
 CURVE ( )  GEOMETRIC_REPRESENTATION_ITEM ( )  RATIONAL_B_SPLINE_CURVE ( ( 1.000000000000000000, 0.9931441806372443004, 0.9931441806372443004, 1.000000000000000000 ) ) 
 REPRESENTATION_ITEM ( '' )  );
#11793=ORIENTED_EDGE ( 'NONE', *, *, #103442, .F. ) ;
#11794=CARTESIAN_POINT ( 'NONE',  ( 11.85058003275609906, 1431.258819511150023, 149.8778382379539948 ) ) ;
#11795=EDGE_CURVE ( 'NONE', #51888, #90510, #50240, .T. ) ;
#11798=ORIENTED_EDGE ( 'NONE', *, *, #57038, .T. ) ;
#11804=CARTESIAN_POINT ( 'NONE',  ( 17.43092393268590001, 1452.304359110679798, 145.9286196276850092 ) ) ;
#11805=CARTESIAN_POINT ( 'NONE',  ( 4.281468235900000252, 1408.076772451330044, 270.2892484966980078 ) ) ;
#11809=CARTESIAN_POINT ( 'NONE',  ( -21.02559120289207684, 1509.697962614031894, 230.2053966973059005 ) ) ;
#11812=CARTESIAN_POINT ( 'NONE',  ( 14.93446018370000061, 1453.159462792729983, 195.2131447753980069 ) ) ;
#11814=CARTESIAN_POINT ( 'NONE',  ( 17.84432149610639939, 1418.606169056330145, 225.0325621462739889 ) ) ;
#11816=ORIENTED_EDGE ( 'NONE', *, *, #24856, .T. ) ;
#11817=CARTESIAN_POINT ( 'NONE',  ( 40.73184307449999864, 1440.913060387330006, 268.3665355201979992 ) ) ;
#11828=CARTESIAN_POINT ( 'NONE',  ( -24.43616533349999997, 1442.711518362400284, 211.0968143008180107 ) ) ;
#11829=CARTESIAN_POINT ( 'NONE',  ( -11.73709356400000026, 1426.695943121429991, 144.1748013713979901 ) ) ;
#11830=CARTESIAN_POINT ( 'NONE',  ( 29.75012120190000076, 1509.993914123429931, 209.6841247587719863 ) ) ;
#11833=CARTESIAN_POINT ( 'NONE',  ( 19.20880922570000138, 1509.714298116030022, 184.5747400720979954 ) ) ;
#11836=CARTESIAN_POINT ( 'NONE',  ( 16.36321488700000160, 1415.089959694529853, 226.8952736679979978 ) ) ;
#11839=CARTESIAN_POINT ( 'NONE',  ( -15.72949124279999999, 1459.406586711229920, 229.6279973257979918 ) ) ;
#11841=CARTESIAN_POINT ( 'NONE',  ( 46.16776989860000668, 1440.913083889750169, 266.9714971360980371 ) ) ;
#11842=CARTESIAN_POINT ( 'NONE',  ( -17.64143905099999898, 1409.529113013930100, 222.5042051235980125 ) ) ;
#11843=CARTESIAN_POINT ( 'NONE',  ( 20.53228480110000120, 1435.642735894570023, 144.3848875112979897 ) ) ;
#11844=CARTESIAN_POINT ( 'NONE',  ( 20.37750482680000275, 1488.586794206330069, 191.0822492793979848 ) ) ;
#11845=EDGE_CURVE ( 'NONE', #68424, #53112, #13539, .T. ) ;
#11846=CARTESIAN_POINT ( 'NONE',  ( 5.383702537648559883, 1431.669030977889861, 154.5771441291960286 ) ) ;
#11848=CARTESIAN_POINT ( 'NONE',  ( -16.04920218319999847, 1423.363755928130104, 227.1130481936980061 ) ) ;
#11850=CARTESIAN_POINT ( 'NONE',  ( -40.03876954321400206, 1439.602033950459827, 136.4880915068820002 ) ) ;
#11851=CARTESIAN_POINT ( 'NONE',  ( -10.74459946700000046, 1409.109315431730010, 199.8441821536079885 ) ) ;
#11853=CARTESIAN_POINT ( 'NONE',  ( -17.05103801767675265, 1409.778322827861302, 193.4350317778312842 ) ) ;
#11855=CARTESIAN_POINT ( 'NONE',  ( 13.19909928449999903, 1434.900406568759763, 146.5971321357980059 ) ) ;
#11856=CARTESIAN_POINT ( 'NONE',  ( -32.76525568849999814, 1436.117894521449898, 136.3349802012980092 ) ) ;
#11857=CARTESIAN_POINT ( 'NONE',  ( -8.095121878198867194, 1456.266568741559013, 227.2460153072438516 ) ) ;
#11858=VERTEX_POINT ( 'NONE', #74142 ) ;
#11860=CARTESIAN_POINT ( 'NONE',  ( 8.742163716520650412E-12, 1408.913060387359792, 224.1216835645979870 ) ) ;
#11863=CARTESIAN_POINT ( 'NONE',  ( -5.506664947740000038, 1440.093543047909861, 154.7592479031980019 ) ) ;
#11865=CARTESIAN_POINT ( 'NONE',  ( -29.91790837370000133, 1467.081768096229780, 269.1810262515979844 ) ) ;
#11867=CARTESIAN_POINT ( 'NONE',  ( 0.1632388131350529792, 1420.111806197110127, 183.8575883265500295 ) ) ;
#11869=CARTESIAN_POINT ( 'NONE',  ( 2.500000000000039968, 1439.615672328189930, 182.7715275322960053 ) ) ;
#11872=CARTESIAN_POINT ( 'NONE',  ( 16.77431906226270186, 1423.634601885720031, 228.4330072057720145 ) ) ;
#11873=CARTESIAN_POINT ( 'NONE',  ( 21.32617020600000046, 1509.431680020230033, 227.8426432890980209 ) ) ;
#11874=CARTESIAN_POINT ( 'NONE',  ( 14.55718211070000123, 1474.164285818730150, 224.0619686816980050 ) ) ;
#11879=ORIENTED_EDGE ( 'NONE', *, *, #4250, .T. ) ;
#11883=CARTESIAN_POINT ( 'NONE',  ( -11.54717405559999932, 1415.048591087029763, 195.8252350565979896 ) ) ;
#11885=CARTESIAN_POINT ( 'NONE',  ( 23.93004698060000024, 1410.670645398829947, 210.2052696501280025 ) ) ;
#11888=CARTESIAN_POINT ( 'NONE',  ( -15.07724445960000104, 1422.393410174129940, 228.4053988666979933 ) ) ;
#11892=CARTESIAN_POINT ( 'NONE',  ( 0.3785032462900000394, 1486.990708827730032, 230.2501120783980184 ) ) ;
#11895=CARTESIAN_POINT ( 'NONE',  ( -0.6713814905552020207, 1419.496215425129776, 184.7333992447800313 ) ) ;
#11897=CARTESIAN_POINT ( 'NONE',  ( -18.78018960140000360, 1425.453421275130040, 226.8344281414980230 ) ) ;
#11898=CARTESIAN_POINT ( 'NONE',  ( -18.07364243031040019, 1485.804844989679850, 188.7995565196659982 ) ) ;
#11902=ORIENTED_EDGE ( 'NONE', *, *, #69473, .F. ) ;
#11904=CARTESIAN_POINT ( 'NONE',  ( 27.70972759929999896, 1508.058934375229910, 212.2396871123379753 ) ) ;
#11908=CARTESIAN_POINT ( 'NONE',  ( -2.075990293979999676E-15, 1427.305457135430061, 123.0297916884979941 ) ) ;
#11909=CARTESIAN_POINT ( 'NONE',  ( 15.73554083432909856, 1409.462555430399789, 192.8532499784679999 ) ) ;
#11910=DIRECTION ( 'NONE',  ( 0.000000000000000000, 2.176037128269999911E-14, 1.000000000000000000 ) ) ;
#11911=CARTESIAN_POINT ( 'NONE',  ( -24.75919491527180227, 1451.809128946330020, 137.0711371202310147 ) ) ;
#11913=CARTESIAN_POINT ( 'NONE',  ( 13.31824321100000041, 1409.378143688529917, 226.7832290943979956 ) ) ;
#11916=CARTESIAN_POINT ( 'NONE',  ( 41.14836836624020577, 1446.538313982190175, 134.0999999985649822 ) ) ;
#11920=ORIENTED_EDGE ( 'NONE', *, *, #107543, .F. ) ;
#11922=ORIENTED_EDGE ( 'NONE', *, *, #3615, .F. ) ;
#11933=CARTESIAN_POINT ( 'NONE',  ( 1.067730373280000089, 1508.997447140530085, 238.8264927836980007 ) ) ;
#11934=ORIENTED_EDGE ( 'NONE', *, *, #44989, .T. ) ;
#11936=EDGE_LOOP ( 'NONE', ( #10627, #53562, #79164, #6761, #60677 ) ) ;
#11937=CARTESIAN_POINT ( 'NONE',  ( 25.80232757302710311, 1440.913060387330006, 241.6272588468080187 ) ) ;
#11938=EDGE_CURVE ( 'NONE', #92390, #62647, #95890, .T. ) ;
#11942=CARTESIAN_POINT ( 'NONE',  ( -14.39047323610000184, 1409.582260767330126, 191.0429864508980131 ) ) ;
#11944=CARTESIAN_POINT ( 'NONE',  ( -24.41028537817162203, 1440.675387093458539, 212.0168806395822401 ) ) ;
#11946=CARTESIAN_POINT ( 'NONE',  ( 22.20862914986459558, 1410.187580636810026, 206.2522814213569973 ) ) ;
#11951=CARTESIAN_POINT ( 'NONE',  ( 15.71037775574616191, 1410.149708096691711, 191.7130642213688247 ) ) ;
#11956=CARTESIAN_POINT ( 'NONE',  ( 28.14152795669999918, 1508.624282194429952, 208.2673348377579998 ) ) ;
#11958=CARTESIAN_POINT ( 'NONE',  ( -19.03312856000000153, 1434.814457748080031, 208.9576311756670179 ) ) ;
#11962=DIRECTION ( 'NONE',  ( 0.4530882417530768813, -0.7475172582776776764, 0.4857252245479219410 ) ) ;
#11964=CARTESIAN_POINT ( 'NONE',  ( 10.53938673539999904, 1467.231892115330083, 248.5638781408979696 ) ) ;
#11965=EDGE_CURVE ( 'NONE', #45814, #48553, #41652, .T. ) ;
#11967=CARTESIAN_POINT ( 'NONE',  ( -26.24895334306360084, 1509.829694036420051, 222.2356625040769984 ) ) ;
#11968=CARTESIAN_POINT ( 'NONE',  ( -0.4986482637964069764, 1508.982360564700230, 238.8511999805219830 ) ) ;
#11970=CARTESIAN_POINT ( 'NONE',  ( -19.83396412799999808, 1455.741242482730058, 225.6883558546980169 ) ) ;
#11972=EDGE_CURVE ( 'NONE', #17632, #29227, #107089, .T. ) ;
#11973=CARTESIAN_POINT ( 'NONE',  ( -19.54838982620000110, 1444.804232268380019, 224.9727483068980121 ) ) ;
#11974=CARTESIAN_POINT ( 'NONE',  ( 2.500000000000000000, 1419.383841502129826, 144.0536014349980007 ) ) ;
#11975=CARTESIAN_POINT ( 'NONE',  ( 0.1695961737810000036, 1488.805759878529898, 187.7260248280979908 ) ) ;
#11979=CARTESIAN_POINT ( 'NONE',  ( 1.777827934399999865, 1405.774244366030189, 267.5358630757979768 ) ) ;
#11982=CARTESIAN_POINT ( 'NONE',  ( 40.88432421962840380, 1450.842314229549856, 269.8587844018130681 ) ) ;
#11983=CARTESIAN_POINT ( 'NONE',  ( -27.01382282590000017, 1451.969727051930022, 134.9184453750980026 ) ) ;
#11985=CARTESIAN_POINT ( 'NONE',  ( -45.44691271756050099, 1440.913060394409968, 265.9511583644469965 ) ) ;
#11991=PLANE ( 'NONE',  #64049 ) ;
#11993=CARTESIAN_POINT ( 'NONE',  ( -31.32742177469999945, 1440.913060387330006, 255.3819207742980097 ) ) ;
#11995=CARTESIAN_POINT ( 'NONE',  ( -0.1067711740600000014, 1475.319450600529990, 269.4986873274979757 ) ) ;
#11996=CARTESIAN_POINT ( 'NONE',  ( -4.259705254135069730, 1446.578490207630011, 159.5784562383719845 ) ) ;
#11997=CARTESIAN_POINT ( 'NONE',  ( -28.22027524449999802, 1509.158030585729875, 210.3012591173880139 ) ) ;
#11998=B_SPLINE_CURVE_WITH_KNOTS ( 'NONE', 3,
 ( #105087, #76701, #54160, #79894 ),
 .UNSPECIFIED., .F., .F.,
 ( 4, 4 ),
 ( 0.000000000000000000, 1.000000000000000000 ),
 .UNSPECIFIED. ) ;
#12000=CARTESIAN_POINT ( 'NONE',  ( -4.122335531849919299, 1448.298783337578470, 185.1042314757649194 ) ) ;
#12003=CARTESIAN_POINT ( 'NONE',  ( -17.58950218620000072, 1415.041103189330215, 207.8054830739180261 ) ) ;
#12004=CARTESIAN_POINT ( 'NONE',  ( 11.87252949456130047, 1432.818935466539870, 149.9811197374779965 ) ) ;
#12005=CARTESIAN_POINT ( 'NONE',  ( 26.79700173971789923, 1435.433286571610097, 135.3787855487989873 ) ) ;
#12006=CARTESIAN_POINT ( 'NONE',  ( -8.229377170839249800, 1396.200436570979946, 216.4989716017560113 ) ) ;
#12008=CARTESIAN_POINT ( 'NONE',  ( -14.77963593200000147, 1422.241748322230023, 229.4612819423979886 ) ) ;
#12012=CARTESIAN_POINT ( 'NONE',  ( 1.802301219090000073, 1409.910657985330090, 232.1755723407979985 ) ) ;
#12014=CARTESIAN_POINT ( 'NONE',  ( 11.56973989449999962, 1426.806448162329843, 132.2115754456980028 ) ) ;
#12022=CARTESIAN_POINT ( 'NONE',  ( 4.416389894569999086, 1509.047812932029956, 180.2178558522979870 ) ) ;
#12031=CARTESIAN_POINT ( 'NONE',  ( -18.57722710470001815, 1435.146103754618707, 144.7442513582978449 ) ) ;
#12034=CARTESIAN_POINT ( 'NONE',  ( -1.358753378944950185, 1412.017682228260128, 185.5325774167320105 ) ) ;
#12037=CARTESIAN_POINT ( 'NONE',  ( -41.45619614403190667, 1444.641645903369863, 136.4680537501220101 ) ) ;
#12039=CARTESIAN_POINT ( 'NONE',  ( -2.500000000000000000, 1448.231807117899962, 166.4374264918500046 ) ) ;
#12040=LINE ( 'NONE', #46222, #88414 ) ;
#12042=CARTESIAN_POINT ( 'NONE',  ( -2.286937354066500117, 1406.300447436870172, 269.2931096073519939 ) ) ;
#12043=CARTESIAN_POINT ( 'NONE',  ( 41.48252513910000516, 1444.135613576870128, 136.5500652558980050 ) ) ;
#12048=VERTEX_POINT ( 'NONE', #101786 ) ;
#12055=CARTESIAN_POINT ( 'NONE',  ( -14.44412179201740010, 1509.548839732050055, 182.8006781750410141 ) ) ;
#12057=CARTESIAN_POINT ( 'NONE',  ( 18.00081235489999898, 1415.932617989529945, 212.9990166833879925 ) ) ;
#12061=CARTESIAN_POINT ( 'NONE',  ( -4.219013252539999925, 1410.436621388929780, 232.1416577203980012 ) ) ;
#12062=CARTESIAN_POINT ( 'NONE',  ( -15.28420222189999933, 1497.713060387329961, 192.4536333146980098 ) ) ;
#12064=CARTESIAN_POINT ( 'NONE',  ( 1.705087066220000169, 1507.082462650630077, 236.5153987699980007 ) ) ;
#12067=CARTESIAN_POINT ( 'NONE',  ( -8.301987938657498844, 1512.913060387330006, 185.0111222839169898 ) ) ;
#12068=CARTESIAN_POINT ( 'NONE',  ( 28.88161794570000040, 1415.817973096529840, 270.2667682292980089 ) ) ;
#12072=CARTESIAN_POINT ( 'NONE',  ( 0.02043389301803385377, 1507.170882767263492, 237.3556640025030049 ) ) ;
#12076=EDGE_LOOP ( 'NONE', ( #7714, #56960, #63977, #55408 ) ) ;
#12077=CARTESIAN_POINT ( 'NONE',  ( 4.352598717569040154, 1420.338240732929989, 185.6900682800660149 ) ) ;
#12078=CARTESIAN_POINT ( 'NONE',  ( -4.415413580500000101, 1415.372779959029913, 232.3000245577979967 ) ) ;
#12084=CARTESIAN_POINT ( 'NONE',  ( -20.84038636311550263, 1509.309337355510024, 228.9357793634370069 ) ) ;
#12086=CARTESIAN_POINT ( 'NONE',  ( 0.1069017372639999991, 1409.419549215130019, 233.0164748551979983 ) ) ;
#12087=CARTESIAN_POINT ( 'NONE',  ( -0.06409245479768720111, 1420.448119606670161, 182.6888690408050024 ) ) ;
#12092=VECTOR ( 'NONE', #102025, 1000.000000000000000 ) ;
#12093=ORIENTED_EDGE ( 'NONE', *, *, #34433, .T. ) ;
#12099=( BOUNDED_CURVE ( )  B_SPLINE_CURVE ( 3, ( #65073, #32560, #91367, #22469 ),
 .UNSPECIFIED., .F., .F. ) 
 B_SPLINE_CURVE_WITH_KNOTS ( ( 4, 4 ),
 ( 1.535862050798705081, 1.553281469862595188 ),
 .UNSPECIFIED. ) 
 CURVE ( )  GEOMETRIC_REPRESENTATION_ITEM ( )  RATIONAL_B_SPLINE_CURVE ( ( 1.000000000000000000, 0.9999747138131391822, 0.9999747138131391822, 1.000000000000000000 ) ) 
 REPRESENTATION_ITEM ( '' )  );
#12104=CARTESIAN_POINT ( 'NONE',  ( 15.66605189140578247, 1421.055886089876594, 227.6080301534365731 ) ) ;
#12105=CARTESIAN_POINT ( 'NONE',  ( 5.557914828519999517, 1420.826195899929871, 186.0956685246979987 ) ) ;
#12106=CARTESIAN_POINT ( 'NONE',  ( -18.18255051909999764, 1424.952931054730016, 227.0171290564980211 ) ) ;
#12107=CARTESIAN_POINT ( 'NONE',  ( -17.78508617079999610, 1435.118679338369930, 145.5186544196980094 ) ) ;
#12110=CARTESIAN_POINT ( 'NONE',  ( 0.8764178805871419842, 1410.319213181679970, 233.0346325316370155 ) ) ;
#12113=ORIENTED_EDGE ( 'NONE', *, *, #32367, .T. ) ;
#12114=DIRECTION ( 'NONE',  ( -1.000000000000000000, 0.000000000000000000, 0.000000000000000000 ) ) ;
#12118=CARTESIAN_POINT ( 'NONE',  ( -11.92436196651230240, 1433.423664094866126, 149.9160749996637492 ) ) ;
#12122=CARTESIAN_POINT ( 'NONE',  ( 14.59882275880000080, 1475.513060387329915, 223.7206687199980308 ) ) ;
#12123=FACE_OUTER_BOUND ( 'NONE', #109175, .T. ) ;
#12124=CARTESIAN_POINT ( 'NONE',  ( -7.338592697498807382, 1507.281022697548451, 235.5381695832356854 ) ) ;
#12130=EDGE_CURVE ( 'NONE', #29403, #16786, #60291, .T. ) ;
#12131=CARTESIAN_POINT ( 'NONE',  ( 21.18965232119999698, 1508.901491395929952, 190.3943043406979996 ) ) ;
#12132=ORIENTED_EDGE ( 'NONE', *, *, #72671, .F. ) ;
#12139=CARTESIAN_POINT ( 'NONE',  ( 13.17455542446274741, 1443.091355729311545, 169.3947984149703814 ) ) ;
#12140=CARTESIAN_POINT ( 'NONE',  ( 40.92779976970093259, 1433.910425749881142, 269.6272358578021340 ) ) ;
#12141=CARTESIAN_POINT ( 'NONE',  ( -13.69364984400000118, 1462.915759927429917, 238.2645906006979999 ) ) ;
#12143=CONICAL_SURFACE ( 'NONE', #15702, 1.499999999999955369, 0.3430239404209998177 ) ;
#12144=CARTESIAN_POINT ( 'NONE',  ( -11.93818826309999892, 1433.480069981700126, 149.8971985194979766 ) ) ;
#12145=CARTESIAN_POINT ( 'NONE',  ( 26.88784107860000105, 1509.181461243030071, 204.0448338698880093 ) ) ;
#12146=CARTESIAN_POINT ( 'NONE',  ( -19.56601163170000390, 1485.666649664629858, 190.1001640202979956 ) ) ;
#12147=CARTESIAN_POINT ( 'NONE',  ( 5.996724739790000314, 1409.122470629630016, 188.2987590254980148 ) ) ;
#12148=CARTESIAN_POINT ( 'NONE',  ( 4.876253047089999626, 1422.291999688530041, 184.8458127703979983 ) ) ;
#12149=FACE_OUTER_BOUND ( 'NONE', #15169, .T. ) ;
#12151=DIRECTION ( 'NONE',  ( 0.03489949406805378795, 0.9993908271110926167, 3.148602398629828534E-12 ) ) ;
#12152=AXIS2_PLACEMENT_3D ( 'NONE', #59672, #27712, #78669 ) ;
#12154=CARTESIAN_POINT ( 'NONE',  ( -16.19493240869999795, 1409.478599888930148, 193.4350318414979881 ) ) ;
#12156=VERTEX_POINT ( 'NONE', #82399 ) ;
#12157=CARTESIAN_POINT ( 'NONE',  ( -11.85768019138030027, 1431.748854777190218, 149.9507373201959979 ) ) ;
#12160=CARTESIAN_POINT ( 'NONE',  ( -10.68754386630000042, 1471.687871048830175, 270.3681166667980165 ) ) ;
#12162=CARTESIAN_POINT ( 'NONE',  ( 6.464994551020000202, 1433.443311356699951, 154.6859263780980029 ) ) ;
#12163=CARTESIAN_POINT ( 'NONE',  ( -15.61596525200000229, 1495.917977012930123, 224.3506286668980181 ) ) ;
#12164=CARTESIAN_POINT ( 'NONE',  ( 0.2052324461623580010, 1452.314876516149980, 183.1678648498289874 ) ) ;
#12165=CARTESIAN_POINT ( 'NONE',  ( -14.19989568679999969, 1422.015600902929918, 228.9627754381980083 ) ) ;
#12168=CARTESIAN_POINT ( 'NONE',  ( -45.88106474657430311, 1437.104218600800095, 268.2135919139319640 ) ) ;
#12170=CARTESIAN_POINT ( 'NONE',  ( -3.541468562257029884, 1499.388879724870094, 181.3066299419379845 ) ) ;
#12172=ORIENTED_EDGE ( 'NONE', *, *, #30380, .F. ) ;
#12177=CARTESIAN_POINT ( 'NONE',  ( -13.31934106549999974, 1410.400658079930054, 189.8751199163980061 ) ) ;
#12178=CARTESIAN_POINT ( 'NONE',  ( -27.01940583621439984, 1450.860076101910181, 136.4173285475219757 ) ) ;
#12186=CARTESIAN_POINT ( 'NONE',  ( -19.24938132970260085, 1411.370636520449807, 270.3367931074290027 ) ) ;
#12187=CARTESIAN_POINT ( 'NONE',  ( 3.463848119014229621, 1417.013915635440071, 232.0800632347320231 ) ) ;
#12188=CARTESIAN_POINT ( 'NONE',  ( 0.02816689439180000351, 1396.454734805430007, 196.6641013465980166 ) ) ;
#12192=CARTESIAN_POINT ( 'NONE',  ( 44.85566571832070082, 1447.217473659629604, 268.9966131275909902 ) ) ;
#12194=CARTESIAN_POINT ( 'NONE',  ( -13.65886266334669941, 1436.196144125749925, 150.4235525661960082 ) ) ;
#12196=CARTESIAN_POINT ( 'NONE',  ( -0.008200652638768689967, 1408.924627079619995, 186.2841847630899963 ) ) ;
#12198=DIRECTION ( 'NONE',  ( -0.03489950311976935254, 0.9993908267949999091, 1.331239895961819999E-11 ) ) ;
#12199=CARTESIAN_POINT ( 'NONE',  ( -0.0001210645912511750048, 1475.561026843769923, 269.2948676583999941 ) ) ;
#12200=CARTESIAN_POINT ( 'NONE',  ( 11.50684714920000040, 1415.041103189330215, 222.4903113597979996 ) ) ;
#12201=CARTESIAN_POINT ( 'NONE',  ( 3.981544315609999884, 1446.451571810050154, 183.2730513936979833 ) ) ;
#12205=CARTESIAN_POINT ( 'NONE',  ( -23.52416583785102944, 1448.205401278070667, 215.6064549854269785 ) ) ;
#12207=CARTESIAN_POINT ( 'NONE',  ( 11.47315440600428715, 1454.673345936858368, 225.8564051334478506 ) ) ;
#12211=CARTESIAN_POINT ( 'NONE',  ( 19.58436876019999673, 1409.761450691529944, 197.7698869336979897 ) ) ;
#12212=CARTESIAN_POINT ( 'NONE',  ( 21.81076600339999771, 1409.674709119329918, 208.0390244633379950 ) ) ;
#12213=CARTESIAN_POINT ( 'NONE',  ( 17.00542863269999927, 1410.873424589829938, 226.2926139095980034 ) ) ;
#12217=CARTESIAN_POINT ( 'NONE',  ( 2.500000000000000000, 1439.419208462029928, 162.1010771267879704 ) ) ;
#12222=DIRECTION ( 'NONE',  ( 0.01393861123991820168, -0.01013782210637889994, 0.9998514588075779752 ) ) ;
#12225=CARTESIAN_POINT ( 'NONE',  ( -18.05542497264810109, 1416.825784014559986, 209.4840452940109969 ) ) ;
#12229=CARTESIAN_POINT ( 'NONE',  ( -38.47491875445290077, 1448.367029702490072, 136.4422118765199912 ) ) ;
#12231=CARTESIAN_POINT ( 'NONE',  ( 11.60004869885203682, 1425.261174633484188, 138.0376396451788139 ) ) ;
#12232=CARTESIAN_POINT ( 'NONE',  ( 11.73700276280139931, 1426.696010850159837, 144.1682878426319974 ) ) ;
#12233=CARTESIAN_POINT ( 'NONE',  ( -2.902293737380750027, 1471.341547563029962, 183.8916672433869905 ) ) ;
#12234=CARTESIAN_POINT ( 'NONE',  ( 11.06271855039999963, 1433.091631396069943, 151.7087564066980008 ) ) ;
#12236=CARTESIAN_POINT ( 'NONE',  ( -19.58397906120409715, 1471.164316944340044, 270.0578164987000491 ) ) ;
#12240=ORIENTED_EDGE ( 'NONE', *, *, #104640, .F. ) ;
#12241=FACE_OUTER_BOUND ( 'NONE', #56637, .T. ) ;
#12242=CARTESIAN_POINT ( 'NONE',  ( 12.37499353609999986, 1445.063428794549964, 150.7815459944920065 ) ) ;
#12244=CARTESIAN_POINT ( 'NONE',  ( 8.006052564334819266, 1398.150843778026456, 198.8796111588884230 ) ) ;
#12245=CARTESIAN_POINT ( 'NONE',  ( 1.907725587109999843, 1490.900299108929858, 235.6062317305980116 ) ) ;
#12246=AXIS2_PLACEMENT_3D ( 'NONE', #89299, #56253, #28850 ) ;
#12247=B_SPLINE_CURVE_WITH_KNOTS ( 'NONE', 5,
 ( #69512, #60556, #94677, #96338, #17390, #70072 ),
 .UNSPECIFIED., .F., .F.,
 ( 6, 6 ),
 ( 0.000000000000000000, 11.48858425020000240 ),
 .UNSPECIFIED. ) ;
#12248=CARTESIAN_POINT ( 'NONE',  ( -10.58047146200000022, 1509.111071725129932, 235.4109798456979945 ) ) ;
#12250=CARTESIAN_POINT ( 'NONE',  ( 20.34262379729999992, 1485.757879992529979, 225.3684058912980106 ) ) ;
#12251=CARTESIAN_POINT ( 'NONE',  ( 5.390423872767819979, 1422.474059485570024, 133.9852895348969923 ) ) ;
#12253=CARTESIAN_POINT ( 'NONE',  ( 2.379842363999999932, 1464.647331468930133, 236.2541381392979929 ) ) ;
#12254=CARTESIAN_POINT ( 'NONE',  ( -41.66021910349999757, 1443.875694946319754, 135.6929188412979954 ) ) ;
#12256=CARTESIAN_POINT ( 'NONE',  ( -1.271037680349999865, 1450.748653814689987, 181.7779247749980129 ) ) ;
#12260=VERTEX_POINT ( 'NONE', #74003 ) ;
#12268=CARTESIAN_POINT ( 'NONE',  ( 14.34763326340369893, 1409.414090780570177, 213.2724514398500162 ) ) ;
#12271=CARTESIAN_POINT ( 'NONE',  ( -18.87572180689999968, 1452.014070220629947, 191.8431515786979844 ) ) ;
#12273=CARTESIAN_POINT ( 'NONE',  ( 13.35741048202589809, 1443.913060387329324, 164.9741927960640453 ) ) ;
#12277=CARTESIAN_POINT ( 'NONE',  ( 18.22279825098010164, 1457.639640533290049, 229.9734878635680104 ) ) ;
#12279=CARTESIAN_POINT ( 'NONE',  ( 29.83693158363007569, 1462.368600761292100, 269.4690755030636637 ) ) ;
#12280=CARTESIAN_POINT ( 'NONE',  ( -20.51885332321579725, 1505.236437000949991, 190.4655934336639689 ) ) ;
#12281=CARTESIAN_POINT ( 'NONE',  ( 2.551411588599999725, 1397.989669479629811, 221.9716508525979748 ) ) ;
#12283=CARTESIAN_POINT ( 'NONE',  ( -1.459671184189999860, 1476.698137529930136, 182.8094855557980054 ) ) ;
#12285=CARTESIAN_POINT ( 'NONE',  ( -25.00976051679999657, 1436.598010167069788, 137.9330532114979917 ) ) ;
#12289=CARTESIAN_POINT ( 'NONE',  ( -12.84236090119540030, 1435.935773415550102, 150.8115148268369978 ) ) ;
#12292=CARTESIAN_POINT ( 'NONE',  ( -0.3621993323151809774, 1416.825784014559986, 191.0664209890499876 ) ) ;
#12294=CARTESIAN_POINT ( 'NONE',  ( 18.64588652299999794, 1416.828040475229955, 209.6843149956849857 ) ) ;
#12296=ORIENTED_EDGE ( 'NONE', *, *, #2389, .T. ) ;
#12298=CARTESIAN_POINT ( 'NONE',  ( 16.98088721830000125, 1414.156372837330082, 255.1565004954979941 ) ) ;
#12299=CARTESIAN_POINT ( 'NONE',  ( -25.61862525230000287, 1449.804154372189942, 208.1054677997580029 ) ) ;
#12300=CARTESIAN_POINT ( 'NONE',  ( -10.88730305954610067, 1426.101976979720121, 91.15062580800939429 ) ) ;
#12301=CARTESIAN_POINT ( 'NONE',  ( -16.60786730719999937, 1409.493019893330029, 195.7756164720979939 ) ) ;
#12302=EDGE_CURVE ( 'NONE', #8198, #76159, #47014, .T. ) ;
#12304=CARTESIAN_POINT ( 'NONE',  ( -1.011872109909999887E-09, 1411.425361493330001, 255.2684082166979920 ) ) ;
#12306=EDGE_CURVE ( 'NONE', #46444, #36359, #16663, .T. ) ;
#12308=CARTESIAN_POINT ( 'NONE',  ( 2.935146075021433543, 1447.712003106908014, 154.8057247725446643 ) ) ;
#12309=CARTESIAN_POINT ( 'NONE',  ( -23.01872370112488753, 1409.746765365450756, 208.8717086315775759 ) ) ;
#12313=CARTESIAN_POINT ( 'NONE',  ( 38.59236949370160374, 1443.548215515760148, 137.1678974980540033 ) ) ;
#12315=ORIENTED_EDGE ( 'NONE', *, *, #104866, .T. ) ;
#12316=CARTESIAN_POINT ( 'NONE',  ( -10.85852385830536448, 1424.794007418652882, 138.1924915167475660 ) ) ;
#12317=CARTESIAN_POINT ( 'NONE',  ( -23.01870917701389985, 1409.746761054060244, 208.8717042921039990 ) ) ;
#12319=CARTESIAN_POINT ( 'NONE',  ( -0.3052841619420000319, 1412.052214267130012, 184.9138573875980285 ) ) ;
#12320=AXIS2_PLACEMENT_3D ( 'NONE', #93297, #94388, #33944 ) ;
#12321=CARTESIAN_POINT ( 'NONE',  ( 10.27910644096741422, 1446.578925969647344, 153.2874156164771193 ) ) ;
#12322=CARTESIAN_POINT ( 'NONE',  ( -3.369831055830000199, 1489.060830314729856, 235.9240531713980147 ) ) ;
#12325=CARTESIAN_POINT ( 'NONE',  ( -11.61527099314350053, 1414.971349104630008, 221.0857754848229888 ) ) ;
#12326=CARTESIAN_POINT ( 'NONE',  ( 15.25222867979999819, 1496.677411259530118, 225.2158252260980191 ) ) ;
#12330=CARTESIAN_POINT ( 'NONE',  ( 11.86031229030020029, 1431.931911824779945, 149.9673457447429996 ) ) ;
#12333=VERTEX_POINT ( 'NONE', #84989 ) ;
#12339=CARTESIAN_POINT ( 'NONE',  ( 18.16558062136190088, 1452.278704333800079, 145.2414311030810268 ) ) ;
#12343=CARTESIAN_POINT ( 'NONE',  ( -10.96966273854589957, 1432.359729197300112, 151.7701366752919796 ) ) ;
#12344=CARTESIAN_POINT ( 'NONE',  ( 0.03526024722610697493, 1409.948177333189051, 233.1655130677910108 ) ) ;
#12349=CARTESIAN_POINT ( 'NONE',  ( -24.51492576923349986, 1509.184387879659880, 222.5504090698890138 ) ) ;
#12352=CARTESIAN_POINT ( 'NONE',  ( 28.02005514660000074, 1440.913060387330006, 248.0989693021979861 ) ) ;
#12357=CARTESIAN_POINT ( 'NONE',  ( -1.676215897828090107, 1450.511945644329899, 182.4451613505460159 ) ) ;
#12359=DIRECTION ( 'NONE',  ( 0.000000000000000000, 0.000000000000000000, 1.000000000000000000 ) ) ;
#12362=CARTESIAN_POINT ( 'NONE',  ( 10.11781796957937551, 1428.435797280887527, 137.0999999980966777 ) ) ;
#12363=CARTESIAN_POINT ( 'NONE',  ( -2.689480282155449764, 1439.963151421470002, 157.5730576003849990 ) ) ;
#12365=CARTESIAN_POINT ( 'NONE',  ( -1.013621472345935359, 1450.828806111348285, 154.2477477248477555 ) ) ;
#12367=ADVANCED_FACE ( 'NONE', ( #93944 ), #33805, .T. ) ;
#12370=CARTESIAN_POINT ( 'NONE',  ( 27.74304799147289913, 1509.894878401100186, 194.6056596535900098 ) ) ;
#12372=CARTESIAN_POINT ( 'NONE',  ( -4.762729318109999888, 1475.513060387329915, 229.9230423263979901 ) ) ;
#12373=CARTESIAN_POINT ( 'NONE',  ( 17.00050166700000176, 1419.772799493030107, 226.7240349780979898 ) ) ;
#12374=B_SPLINE_CURVE_WITH_KNOTS ( 'NONE', 5,
 ( #91410, #14687, #48876, #55076, #38240, #72422, #106553, #83538, #110403, #33682, #101423, #59473 ),
 .UNSPECIFIED., .F., .F.,
 ( 6, 3, 3, 6 ),
 ( 5.812632519320040103, 6.561021380799999747, 7.569428689259999565, 8.073627588195819271 ),
 .UNSPECIFIED. ) ;
#12378=CARTESIAN_POINT ( 'NONE',  ( 45.67177355289999241, 1440.913081031829961, 266.1885934315979512 ) ) ;
#12379=CARTESIAN_POINT ( 'NONE',  ( -17.84543917770000121, 1409.701167236529727, 223.9496858625980167 ) ) ;
#12380=CARTESIAN_POINT ( 'NONE',  ( 16.10667296019999739, 1435.057002741109955, 146.9490725771979953 ) ) ;
#12382=CARTESIAN_POINT ( 'NONE',  ( 21.81574974289999957, 1508.011787535030180, 191.7684141494979997 ) ) ;
#12383=CARTESIAN_POINT ( 'NONE',  ( -16.34132978743479825, 1409.483684619830001, 192.7109133032730028 ) ) ;
#12385=CARTESIAN_POINT ( 'NONE',  ( -6.179141267909999513, 1475.525926640629905, 266.9460417852980072 ) ) ;
#12387=CARTESIAN_POINT ( 'NONE',  ( -36.93201630645109645, 1436.283700798310065, 135.4717700503809965 ) ) ;
#12388=CARTESIAN_POINT ( 'NONE',  ( 0.2109277773507400033, 1456.827200395890031, 183.0892095144770053 ) ) ;
#12389=CARTESIAN_POINT ( 'NONE',  ( -9.197920992606320567, 1408.707683617470138, 199.0017040286450083 ) ) ;
#12393=CARTESIAN_POINT ( 'NONE',  ( 13.80599399779999992, 1434.979619872729927, 146.4346930199980079 ) ) ;
#12394=CARTESIAN_POINT ( 'NONE',  ( -28.14962045949999592, 1435.955305551769925, 136.4811531283980059 ) ) ;
#12395=CARTESIAN_POINT ( 'NONE',  ( 10.45867790589999835, 1442.264568908580031, 186.5135257037979670 ) ) ;
#12396=ORIENTED_EDGE ( 'NONE', *, *, #43476, .T. ) ;
#12398=CARTESIAN_POINT ( 'NONE',  ( -10.59587896540769947, 1409.283076634259942, 219.6744605712179919 ) ) ;
#12400=ADVANCED_FACE ( 'NONE', ( #52527 ), #58830, .F. ) ;
#12402=CARTESIAN_POINT ( 'NONE',  ( 15.96280133942260271, 1508.735390535940041, 232.0448960862960064 ) ) ;
#12403=CARTESIAN_POINT ( 'NONE',  ( -37.88641905019999712, 1461.898525134130068, 267.8844275163979773 ) ) ;
#12404=CARTESIAN_POINT ( 'NONE',  ( -15.52964687406499955, 1451.324136384999974, 222.4830579234560162 ) ) ;
#12405=CARTESIAN_POINT ( 'NONE',  ( 18.95884613770000016, 1416.837177098729853, 210.4637958795879911 ) ) ;
#12407=CARTESIAN_POINT ( 'NONE',  ( 2.652938167623881238, 1396.005703029557708, 216.7884906539198369 ) ) ;
#12412=CARTESIAN_POINT ( 'NONE',  ( -28.97445500416739961, 1509.604966152339784, 208.6943162784619972 ) ) ;
#12422=CARTESIAN_POINT ( 'NONE',  ( 22.82660133449999762, 1409.710182870830067, 210.6508517238679872 ) ) ;
#12426=CARTESIAN_POINT ( 'NONE',  ( -11.31243770530000070, 1433.012837821759831, 151.5204583838979886 ) ) ;
#12428=CARTESIAN_POINT ( 'NONE',  ( 27.95579582530499962, 1508.164266001930173, 207.9317693576919908 ) ) ;
#12431=CARTESIAN_POINT ( 'NONE',  ( -22.65374348950000183, 1411.052683204430195, 211.5465440029780098 ) ) ;
#12434=CARTESIAN_POINT ( 'NONE',  ( 13.41316562022890047, 1508.156439062169966, 233.1856428097420064 ) ) ;
#12435=ADVANCED_FACE ( 'NONE', ( #81556 ), #108429, .T. ) ;
#12436=CARTESIAN_POINT ( 'NONE',  ( -14.64177459002939941, 1485.585968447049936, 186.6436936439779686 ) ) ;
#12437=ORIENTED_EDGE ( 'NONE', *, *, #102136, .T. ) ;
#12439=AXIS2_PLACEMENT_3D ( 'NONE', #12899, #48177, #99095 ) ;
#12442=ORIENTED_EDGE ( 'NONE', *, *, #13778, .T. ) ;
#12444=CARTESIAN_POINT ( 'NONE',  ( 27.93978865640000109, 1508.083000434530049, 211.1815961025180286 ) ) ;
#12448=CARTESIAN_POINT ( 'NONE',  ( 1.527505831956530002, 1414.913527275050001, 192.0113405201620083 ) ) ;
#12449=CARTESIAN_POINT ( 'NONE',  ( 15.95479805056280043, 1420.121857128410056, 191.2307307053519878 ) ) ;
#12450=CARTESIAN_POINT ( 'NONE',  ( 1.005224880929999953, 1508.991333441630104, 179.4394713248979940 ) ) ;
#12453=ADVANCED_FACE ( 'NONE', ( #3799 ), #84376, .T. ) ;
#12455=CARTESIAN_POINT ( 'NONE',  ( -25.08193098539699761, 1451.798897095909979, 136.5882795326729990 ) ) ;
#12457=CARTESIAN_POINT ( 'NONE',  ( 12.14295705810000037, 1409.337101792229987, 227.8566549244980024 ) ) ;
#12460=CARTESIAN_POINT ( 'NONE',  ( 40.85417709044089918, 1440.196123996860024, 134.0999999980799657 ) ) ;
#12465=CARTESIAN_POINT ( 'NONE',  ( -17.29674189031538489, 1410.881757619984910, 225.9250326850611827 ) ) ;
#12469=EDGE_CURVE ( 'NONE', #33967, #61502, #79808, .T. ) ;
#12472=CARTESIAN_POINT ( 'NONE',  ( 7.871325772944452126, 1451.393740844790500, 152.9831421267123517 ) ) ;
#12473=FACE_OUTER_BOUND ( 'NONE', #61275, .T. ) ;
#12475=EDGE_CURVE ( 'NONE', #22102, #57273, #5547, .T. ) ;
#12476=CARTESIAN_POINT ( 'NONE',  ( -18.04424466527178694, 1447.053540243377711, 216.4274986648658796 ) ) ;
#12479=CARTESIAN_POINT ( 'NONE',  ( 8.506179033730001393, 1416.518532928429977, 193.0747662988979982 ) ) ;
#12485=CARTESIAN_POINT ( 'NONE',  ( 29.57591471954300033, 1440.913060387330006, 251.2017233884100165 ) ) ;
#12486=CARTESIAN_POINT ( 'NONE',  ( -19.00191528430000076, 1508.825455351729943, 187.6945225472979928 ) ) ;
#12487=ORIENTED_EDGE ( 'NONE', *, *, #109837, .T. ) ;
#12488=CARTESIAN_POINT ( 'NONE',  ( -0.1871068506425229983, 1450.906526472119822, 181.2442446829110168 ) ) ;
#12489=CARTESIAN_POINT ( 'NONE',  ( -15.12918126009999931, 1409.441383038730010, 192.4788841068979934 ) ) ;
#12490=DIRECTION ( 'NONE',  ( 0.000000000000000000, 0.000000000000000000, -1.000000000000000000 ) ) ;
#12491=ADVANCED_FACE ( 'NONE', ( #60241 ), #24834, .T. ) ;
#12492=CARTESIAN_POINT ( 'NONE',  ( -24.36542518180000272, 1440.980548595849996, 211.6891219858079864 ) ) ;
#12496=CARTESIAN_POINT ( 'NONE',  ( 26.93223535810000158, 1412.607180478629971, 266.6753325838979549 ) ) ;
#12497=EDGE_CURVE ( 'NONE', #3072, #35478, #25640, .T. ) ;
#12499=CARTESIAN_POINT ( 'NONE',  ( -13.41957906060000028, 1453.146242305830128, 193.5352814221980111 ) ) ;
#12500=CARTESIAN_POINT ( 'NONE',  ( 15.73570983720359884, 1409.462563483369877, 192.9527024472970140 ) ) ;
#12501=CARTESIAN_POINT ( 'NONE',  ( -23.76744983355909824, 1425.881514248650092, 210.9077260303419905 ) ) ;
#12502=AXIS2_PLACEMENT_3D ( 'NONE', #69862, #18853, #11038 ) ;
#12505=EDGE_CURVE ( 'NONE', #11318, #57273, #71030, .T. ) ;
#12508=CARTESIAN_POINT ( 'NONE',  ( 18.26221324211669739, 1446.581092866262679, 215.9872273256496840 ) ) ;
#12510=CARTESIAN_POINT ( 'NONE',  ( 2.127049456099050051, 1416.948096802419968, 220.8082361830769855 ) ) ;
#12511=CARTESIAN_POINT ( 'NONE',  ( -8.970355387749442855, 1421.589330327102971, 137.0999999980979851 ) ) ;
#12513=ORIENTED_EDGE ( 'NONE', *, *, #88460, .T. ) ;
#12516=CARTESIAN_POINT ( 'NONE',  ( 9.545816653570000199, 1464.920850548930048, 240.4008508649979774 ) ) ;
#12520=B_SPLINE_CURVE_WITH_KNOTS ( 'NONE', 3,
 ( #21328, #56626, #64494, #90199, #30853, #65028, #49329, #81253, #107566, #100273, #14601, #57194, #14041, #15139, #4568, #99146, #38702, #66150, #6205, #56072, #107014, #6750, #30302, #22424, #31404, #23553, #40356, #13483, #98610, #83455, #65585, #57745, #73979, #75088, #82913, #21873, #74537, #55534, #82373, #109238, #47673, #90762, #98056, #91319, #89659, #32522, #48232, #5672, #99698, #81802, #5102, #22989, #39257, #73432, #48791, #52090 ),
 .UNSPECIFIED., .F., .F.,
 ( 4, 2, 2, 2, 2, 2, 1, 1, 1, 1, 1, 1, 1, 1, 2, 2, 2, 2, 2, 2, 2, 2, 2, 1, 1, 2, 2, 1, 1, 2, 2, 2, 2, 4 ),
 ( 0.000000000000000000, 0.1249999999950490714, 0.2499999999900982539, 0.3749999999851474364, 0.4374999999826721386, 0.4687499999814371265, 0.4843749999808195095, 0.4921874999805105344, 0.4960937499803561579, 0.4980468749802758888, 0.4990234374802387518, 0.4995117187302201556, 0.4997558593552078876, 0.4998779296677017259, 0.4999389648239485617, 0.4999999999801953421, 0.5312499999787845262, 0.5624999999773735437, 0.5937499999759626723, 0.6249999999745516899, 0.6562499999731408185, 0.6874999999717298360, 0.6953124999714096477, 0.6992187499712494425, 0.6997070312212948506, 0.6999511718463149457, 0.7001953124713350407, 0.7011718749714233034, 0.7031249999716070453, 0.7187499999730988520, 0.7499999999760904590, 0.8124999999820647911, 0.8749999999880391233, 1.000000000000000000 ),
 .UNSPECIFIED. ) ;
#12522=CARTESIAN_POINT ( 'NONE',  ( -20.09300522639999897, 1457.445247091630108, 225.1158171901979870 ) ) ;
#12524=CARTESIAN_POINT ( 'NONE',  ( -1.639329852409999955, 1484.768299803630043, 182.6367947853979956 ) ) ;
#12528=CARTESIAN_POINT ( 'NONE',  ( 0.7655880511680001055, 1406.782360832429958, 269.6498828098979743 ) ) ;
#12531=CARTESIAN_POINT ( 'NONE',  ( 18.87687341284280151, 1468.931718062809978, 269.6477239524390370 ) ) ;
#12534=CARTESIAN_POINT ( 'NONE',  ( 0.000000000000000000, 1413.913060387330006, 209.1218459616979999 ) ) ;
#12539=CARTESIAN_POINT ( 'NONE',  ( 2.493007212856739763, 1449.246563104740062, 154.5202210656170223 ) ) ;
#12540=CARTESIAN_POINT ( 'NONE',  ( -13.73229811677040146, 1415.184612916749984, 220.6533628109979759 ) ) ;
#12541=DIRECTION ( 'NONE',  ( 0.000000000000000000, 1.000000000000000000, 0.000000000000000000 ) ) ;
#12543=CARTESIAN_POINT ( 'NONE',  ( -12.15345565450000009, 1413.272114130229966, 265.6112251771979800 ) ) ;
#12544=ADVANCED_FACE ( 'NONE', ( #65211 ), #101723, .F. ) ;
#12546=CARTESIAN_POINT ( 'NONE',  ( -0.2163474815539999929, 1476.109084357029815, 267.8540247851980212 ) ) ;
#12548=CARTESIAN_POINT ( 'NONE',  ( -10.81507089441019964, 1424.921187596680056, 144.1620444830689962 ) ) ;
#12549=CARTESIAN_POINT ( 'NONE',  ( -3.344594669770147188, 1448.284147565596413, 184.7768058458345308 ) ) ;
#12555=CARTESIAN_POINT ( 'NONE',  ( -10.58554379023919978, 1396.282715721989916, 212.3608612925139880 ) ) ;
#12557=CARTESIAN_POINT ( 'NONE',  ( -14.61089922049999856, 1422.243781465129814, 228.7538395214980085 ) ) ;
#12559=CARTESIAN_POINT ( 'NONE',  ( 19.57204117397504817, 1455.492560539847773, 225.8522660090905561 ) ) ;
#12562=CARTESIAN_POINT ( 'NONE',  ( 1.443308927659999963, 1409.130619246129982, 231.7887507488979963 ) ) ;
#12563=CARTESIAN_POINT ( 'NONE',  ( -11.76598820887720009, 1428.979787295000051, 145.3127948738930115 ) ) ;
#12564=CARTESIAN_POINT ( 'NONE',  ( 11.26090570969999938, 1425.591115143630077, 132.2030400731979967 ) ) ;
#12566=DIRECTION ( 'NONE',  ( -1.000000000000000000, -4.614530979569559207E-09, -3.922279168137524319E-10 ) ) ;
#12567=EDGE_CURVE ( 'NONE', #10827, #104308, #94988, .T. ) ;
#12568=CARTESIAN_POINT ( 'NONE',  ( -12.37499353609999986, 1445.063428794549964, 205.2217743980949933 ) ) ;
#12569=CIRCLE ( 'NONE', #76932, 4079.102027089948479 ) ;
#12572=CARTESIAN_POINT ( 'NONE',  ( -7.298550013359999866, 1430.724169039930075, 149.5003602673979799 ) ) ;
#12573=CARTESIAN_POINT ( 'NONE',  ( 7.288579114480000065, 1509.158655100730130, 180.9739811970979702 ) ) ;
#12580=CARTESIAN_POINT ( 'NONE',  ( -6.016809048099999835, 1396.654460031930057, 198.2004533729979983 ) ) ;
#12581=CARTESIAN_POINT ( 'NONE',  ( 1.165162292670530064, 1482.877340327559978, 235.9985051030799923 ) ) ;
#12583=CARTESIAN_POINT ( 'NONE',  ( 13.22806383159999832, 1431.113060387329824, 223.7296695649979767 ) ) ;
#12584=CARTESIAN_POINT ( 'NONE',  ( 0.1955981723673640149, 1414.913060387329779, 225.1861338915940109 ) ) ;
#12586=CARTESIAN_POINT ( 'NONE',  ( -1.363590407445679942, 1415.730364842510198, 185.3753152215819853 ) ) ;
#12588=CARTESIAN_POINT ( 'NONE',  ( 0.5133699756429999095, 1410.311097179130002, 185.0719926106980040 ) ) ;
#12593=CARTESIAN_POINT ( 'NONE',  ( 41.18767709054869641, 1440.809226716479998, 135.8247641852480001 ) ) ;
#12594=CARTESIAN_POINT ( 'NONE',  ( 7.862841600128040120, 1396.187636867450010, 216.8852634763560161 ) ) ;
#12596=CARTESIAN_POINT ( 'NONE',  ( 11.70410276859999854, 1427.698297935130086, 149.0273710990979907 ) ) ;
#12597=CARTESIAN_POINT ( 'NONE',  ( -18.89905695062199698, 1416.828039266840278, 207.5749027128360069 ) ) ;
#12598=ORIENTED_EDGE ( 'NONE', *, *, #92867, .F. ) ;
#12599=CARTESIAN_POINT ( 'NONE',  ( 4.098422289620000214, 1424.674502485429912, 185.1777122999980065 ) ) ;
#12601=ORIENTED_EDGE ( 'NONE', *, *, #34273, .F. ) ;
#12602=ORIENTED_EDGE ( 'NONE', *, *, #68472, .F. ) ;
#12603=EDGE_CURVE ( 'NONE', #74077, #8151, #5723, .T. ) ;
#12604=CARTESIAN_POINT ( 'NONE',  ( -17.36423504460000089, 1468.191340553330065, 228.4970079188980208 ) ) ;
#12605=CARTESIAN_POINT ( 'NONE',  ( -12.83453119069999993, 1463.115711949329807, 230.6691871800979925 ) ) ;
#12612=CARTESIAN_POINT ( 'NONE',  ( 2.576993404970000512, 1414.913060387329779, 225.2932022862979977 ) ) ;
#12616=B_SPLINE_SURFACE_WITH_KNOTS ( 'NONE', 5, 5, ( 
 ( #52956, #87090, #78697, #70330, #27734, #96041 ),
 ( #19312, #36691, #10945, #70885, #93001, #58322 ),
 ( #48836, #16277, #57787, #58871, #97696, #57239 ),
 ( #82958, #6252, #6793, #71987, #20968, #50479 ),
 ( #40954, #55171, #74578, #33099, #84603, #75131 ),
 ( #15182, #29378, #63579, #46771, #24132, #109281 ),
 ( #7894, #84056, #89297, #91370, #67289, #80902 ),
 ( #106101, #12593, #4198, #72510, #49370, #7355 ),
 ( #40401, #23598, #66739, #41517, #32563, #101380 ),
 ( #108714, #32005, #24673, #91907, #38330, #99747 ),
 ( #83498, #49921, #66193, #100842, #100313, #92445 ),
 ( #15720, #106638, #29929, #64120, #75676, #109820 ) ),
 .UNSPECIFIED., .F., .F., .F.,
 ( 6, 3, 3, 6 ),
 ( 6, 6 ),
 ( -8.488962093846350222E-06, 6.410372910170000438, 10.64487668199999959, 14.62797318289999993 ),
 ( -8.488962093846350222E-06, 1.479090568609999989 ),
 .UNSPECIFIED. ) ;
#12617=CARTESIAN_POINT ( 'NONE',  ( -42.06231988464593741, 1439.942263177195628, 269.6487542301402414 ) ) ;
#12618=CARTESIAN_POINT ( 'NONE',  ( -3.191350148519999763, 1410.401812535530098, 232.4693402741980037 ) ) ;
#12619=FACE_OUTER_BOUND ( 'NONE', #96138, .T. ) ;
#12620=ORIENTED_EDGE ( 'NONE', *, *, #67215, .F. ) ;
#12621=EDGE_CURVE ( 'NONE', #68839, #53112, #109661, .T. ) ;
#12623=CARTESIAN_POINT ( 'NONE',  ( 28.27621775960000150, 1508.136061369130175, 209.2246319227680260 ) ) ;
#12626=CARTESIAN_POINT ( 'NONE',  ( 44.13009079475659746, 1436.416161715979797, 270.2165924888440145 ) ) ;
#12627=ADVANCED_FACE ( 'NONE', ( #94240 ), #84757, .F. ) ;
#12631=CARTESIAN_POINT ( 'NONE',  ( 22.60265952820000024, 1409.702346025430188, 208.8284293190110077 ) ) ;
#12632=CARTESIAN_POINT ( 'NONE',  ( 0.004059509192577217401, 1508.830451557245169, 238.4590521952922018 ) ) ;
#12636=CARTESIAN_POINT ( 'NONE',  ( 27.01367402797299277, 1509.856398671217903, 221.2719421893247898 ) ) ;
#12637=CARTESIAN_POINT ( 'NONE',  ( -11.61299349109999923, 1417.902132930430071, 229.0839532085980181 ) ) ;
#12643=CARTESIAN_POINT ( 'NONE',  ( -20.97376010811069946, 1508.893464270799996, 228.1411980946349729 ) ) ;
#12650=CARTESIAN_POINT ( 'NONE',  ( 19.06981280680000168, 1509.578992924630029, 186.6663347137979940 ) ) ;
#12651=DIRECTION ( 'NONE',  ( 0.000000000000000000, 1.000000000000000000, -2.081668171172166620E-14 ) ) ;
#12656=CARTESIAN_POINT ( 'NONE',  ( 11.60004869885204748, 1426.730434226297575, 134.4361623791434397 ) ) ;
#12657=CARTESIAN_POINT ( 'NONE',  ( 9.930928656378739561, 1435.775907024141588, 152.5385279279675785 ) ) ;
#12660=CARTESIAN_POINT ( 'NONE',  ( -26.36538957056309940, 1508.144877758350049, 201.5400870493360230 ) ) ;
#12662=CARTESIAN_POINT ( 'NONE',  ( -2.704954423899999849, 1447.065239520570003, 170.5387359060979975 ) ) ;
#12663=CARTESIAN_POINT ( 'NONE',  ( -19.15459394270000004, 1425.147755204630130, 223.9734305455980063 ) ) ;
#12666=CARTESIAN_POINT ( 'NONE',  ( 17.95536526520000109, 1461.940388925729849, 190.0337052255979984 ) ) ;
#12678=CARTESIAN_POINT ( 'NONE',  ( -13.24668964730320297, 1444.655481269342545, 186.6492647222285370 ) ) ;
#12679=CARTESIAN_POINT ( 'NONE',  ( -16.81223226430000039, 1414.913060387329779, 207.5743821216680089 ) ) ;
#12685=CARTESIAN_POINT ( 'NONE',  ( 21.90604547420000259, 1509.617455791430075, 189.8984835829979829 ) ) ;
#12686=ORIENTED_EDGE ( 'NONE', *, *, #46138, .F. ) ;
#12693=CARTESIAN_POINT ( 'NONE',  ( 13.38997184703062260, 1443.386902099714234, 169.3691664011028593 ) ) ;
#12694=CARTESIAN_POINT ( 'NONE',  ( 16.15334260449234449, 1412.751362655629691, 269.3697234748176470 ) ) ;
#12695=CARTESIAN_POINT ( 'NONE',  ( -33.60183516099999679, 1440.913060390449800, 248.0844435644980024 ) ) ;
#12696=CARTESIAN_POINT ( 'NONE',  ( -20.18772548640000153, 1494.510936209429929, 190.7767133961980051 ) ) ;
#12697=CARTESIAN_POINT ( 'NONE',  ( -11.93562850120000007, 1433.536276356740018, 150.1881428924980071 ) ) ;
#12698=CARTESIAN_POINT ( 'NONE',  ( 26.15185231619999939, 1509.826303196630079, 197.3935024311979873 ) ) ;
#12699=CARTESIAN_POINT ( 'NONE',  ( 11.60004869885203682, 1426.786827912535728, 134.3786173235958472 ) ) ;
#12703=CARTESIAN_POINT ( 'NONE',  ( 5.268693351980000550, 1440.707873525929926, 154.8524945618979700 ) ) ;
#12709=ORIENTED_EDGE ( 'NONE', *, *, #12603, .T. ) ;
#12711=CARTESIAN_POINT ( 'NONE',  ( -11.86563452110919847, 1432.303449558290140, 149.9823120433860026 ) ) ;
#12713=CARTESIAN_POINT ( 'NONE',  ( -20.06107000609999957, 1468.329342173230089, 269.8982276395979625 ) ) ;
#12716=CIRCLE ( 'NONE', #14449, 1.999999999999998890 ) ;
#12718=ADVANCED_FACE ( 'NONE', ( #61789 ), #50795, .T. ) ;
#12720=EDGE_CURVE ( 'NONE', #25318, #19628, #54948, .T. ) ;
#12723=TOROIDAL_SURFACE ( 'NONE', #27037, 20.98341875039999849, 2.000000000000000000 ) ;
#12724=CARTESIAN_POINT ( 'NONE',  ( -15.68560381520000035, 1410.853898380629971, 226.7268320020979786 ) ) ;
#12726=CARTESIAN_POINT ( 'NONE',  ( -45.52611345104049434, 1436.768312834970175, 268.7663215527609850 ) ) ;
#12728=CARTESIAN_POINT ( 'NONE',  ( -3.542930565813509958, 1500.789291168119917, 181.2469841982909884 ) ) ;
#12729=ORIENTED_EDGE ( 'NONE', *, *, #97538, .T. ) ;
#12734=CARTESIAN_POINT ( 'NONE',  ( 16.37831395161595793, 1409.485003713481547, 224.8086535334813334 ) ) ;
#12735=CARTESIAN_POINT ( 'NONE',  ( -16.01768569949999943, 1425.422481232729979, 190.6310110230979831 ) ) ;
#12736=ADVANCED_FACE ( 'NONE', ( #64537 ), #22470, .T. ) ;
#12737=CARTESIAN_POINT ( 'NONE',  ( -16.20519014447769734, 1470.472166712469971, 228.6977888834950079 ) ) ;
#12743=VERTEX_POINT ( 'NONE', #107611 ) ;
#12745=CARTESIAN_POINT ( 'NONE',  ( -16.36542536654240010, 1412.568371408070107, 269.6441855290919989 ) ) ;
#12746=CARTESIAN_POINT ( 'NONE',  ( -32.74366472130000716, 1435.640891862840135, 135.1028903260980201 ) ) ;
#12751=CARTESIAN_POINT ( 'NONE',  ( 42.04271831246587254, 1454.216331209674536, 269.0746633548914133 ) ) ;
#12753=CARTESIAN_POINT ( 'NONE',  ( -2.500000000000000000, 1419.498728202598613, 138.4985336053808282 ) ) ;
#12754=CARTESIAN_POINT ( 'NONE',  ( -0.03619593704711999982, 1409.492594519410204, 185.3096333675919993 ) ) ;
#12758=CARTESIAN_POINT ( 'NONE',  ( -21.97938480444670262, 1506.433683733529961, 209.5040264213440082 ) ) ;
#12759=CARTESIAN_POINT ( 'NONE',  ( -20.96644920750000196, 1435.767435547340028, 221.3947938468980112 ) ) ;
#12760=CARTESIAN_POINT ( 'NONE',  ( 10.49648151684939990, 1474.485926324769935, 269.6275812235440412 ) ) ;
#12761=CARTESIAN_POINT ( 'NONE',  ( 12.62835224979999893, 1416.067629290630066, 222.6573521500980064 ) ) ;
#12763=( BOUNDED_CURVE ( )  B_SPLINE_CURVE ( 3, ( #39585, #82125, #5428, #81566 ),
 .UNSPECIFIED., .F., .F. ) 
 B_SPLINE_CURVE_WITH_KNOTS ( ( 4, 4 ),
 ( 4.245297863855720166, 5.179473289257879642 ),
 .UNSPECIFIED. ) 
 CURVE ( )  GEOMETRIC_REPRESENTATION_ITEM ( )  RATIONAL_B_SPLINE_CURVE ( ( 1.000000000000000000, 0.9285889602860022407, 0.9285889602860022407, 1.000000000000000000 ) ) 
 REPRESENTATION_ITEM ( '' )  );
#12766=ORIENTED_EDGE ( 'NONE', *, *, #72866, .F. ) ;
#12767=CARTESIAN_POINT ( 'NONE',  ( -42.60628464670860183, 1443.705283352449896, 135.6928033759050152 ) ) ;
#12768=CARTESIAN_POINT ( 'NONE',  ( -22.53754828600002469, 1451.487084850873543, 219.3519410532077529 ) ) ;
#12770=CARTESIAN_POINT ( 'NONE',  ( 2.483946272145344913, 1457.674397455789176, 228.7507860573133485 ) ) ;
#12772=CARTESIAN_POINT ( 'NONE',  ( 24.19930084177359930, 1452.068017472880001, 136.4480432603959912 ) ) ;
#12773=CARTESIAN_POINT ( 'NONE',  ( 13.72467564589999967, 1416.021639796329964, 196.5129936595979814 ) ) ;
#12775=CARTESIAN_POINT ( 'NONE',  ( 20.06637829199999956, 1410.535413374630252, 197.5507824890980260 ) ) ;
#12776=CARTESIAN_POINT ( 'NONE',  ( 13.26516604059999693, 1444.994950788470987, 176.9857848810979704 ) ) ;
#12777=CARTESIAN_POINT ( 'NONE',  ( 16.10810117269999964, 1409.475567675330012, 225.1222583912979758 ) ) ;
#12780=CARTESIAN_POINT ( 'NONE',  ( 2.500000000000000000, 1439.435444791209875, 162.3942721139659682 ) ) ;
#12782=ORIENTED_EDGE ( 'NONE', *, *, #72558, .T. ) ;
#12784=CARTESIAN_POINT ( 'NONE',  ( -4.161170142469999611, 1448.299083525829928, 185.1109003835979934 ) ) ;
#12786=CARTESIAN_POINT ( 'NONE',  ( -40.17892786689739637, 1444.958062479619912, 136.9709319305609938 ) ) ;
#12788=CARTESIAN_POINT ( 'NONE',  ( 11.60004869885213097, 1425.419067644911820, 138.1638145324133689 ) ) ;
#12790=CARTESIAN_POINT ( 'NONE',  ( 17.91230580668798211, 1423.874090688956358, 225.7940723398736793 ) ) ;
#12792=CARTESIAN_POINT ( 'NONE',  ( -41.54777830462669641, 1453.906998726859911, 269.7546269283009792 ) ) ;
#12793=CARTESIAN_POINT ( 'NONE',  ( 29.00640787322850045, 1440.913060387239966, 234.9866596484439754 ) ) ;
#12794=CARTESIAN_POINT ( 'NONE',  ( -20.79315288949999996, 1508.014485607329789, 228.0232908942979861 ) ) ;
#12797=CARTESIAN_POINT ( 'NONE',  ( -2.041421749081904657, 1485.165825109578918, 182.8125668038368303 ) ) ;
#12799=CARTESIAN_POINT ( 'NONE',  ( 1.719367447270000016, 1490.891747643629969, 235.7942165053979977 ) ) ;
#12801=CARTESIAN_POINT ( 'NONE',  ( -16.45186348020000011, 1509.487572119630158, 233.0276686348979922 ) ) ;
#12804=CARTESIAN_POINT ( 'NONE',  ( 7.121584085660000341, 1409.161751583630121, 222.2855843900980233 ) ) ;
#12805=FACE_OUTER_BOUND ( 'NONE', #10347, .T. ) ;
#12806=CARTESIAN_POINT ( 'NONE',  ( 2.033228060669999948, 1464.794380306530002, 236.1307052698979874 ) ) ;
#12808=ORIENTED_EDGE ( 'NONE', *, *, #30380, .T. ) ;
#12809=CARTESIAN_POINT ( 'NONE',  ( -1.298785104950000102, 1450.901045541719895, 182.8763096061979923 ) ) ;
#12813=CARTESIAN_POINT ( 'NONE',  ( -18.07834331186310095, 1415.943166310999914, 208.8325883090850255 ) ) ;
#12823=CARTESIAN_POINT ( 'NONE',  ( 2.300012252027449744, 1408.993378584980064, 194.3064046096619961 ) ) ;
#12824=CARTESIAN_POINT ( 'NONE',  ( 1.249000902699999922E-15, 1417.199650551829791, 167.6845966677979902 ) ) ;
#12826=CARTESIAN_POINT ( 'NONE',  ( -17.84189080239999825, 1437.050698146910008, 191.2181082141979971 ) ) ;
#12828=AXIS2_PLACEMENT_3D ( 'NONE', #107679, #83026, #58386 ) ;
#12829=CARTESIAN_POINT ( 'NONE',  ( -0.2129864720161060154, 1450.905624701759962, 126.7681033905349892 ) ) ;
#12833=CARTESIAN_POINT ( 'NONE',  ( 17.92115727113900192, 1457.712037597299968, 229.4665076238089796 ) ) ;
#12835=CARTESIAN_POINT ( 'NONE',  ( -11.25904675279999978, 1434.364368409959980, 151.5755386760980059 ) ) ;
#12836=CARTESIAN_POINT ( 'NONE',  ( -3.883342170835969822E-10, 1466.795683113560017, 244.3026181627860183 ) ) ;
#12837=CARTESIAN_POINT ( 'NONE',  ( -20.57999989205229951, 1507.217024252700185, 190.4080422748829733 ) ) ;
#12840=CARTESIAN_POINT ( 'NONE',  ( 0.2010921131289999941, 1462.358627342330010, 182.8518807857980164 ) ) ;
#12842=CARTESIAN_POINT ( 'NONE',  ( -25.16089740380983386, 1436.602010722529030, 137.5955485560597253 ) ) ;
#12845=CARTESIAN_POINT ( 'NONE',  ( 11.23207286718879949, 1433.984507984109769, 151.5867044815779821 ) ) ;
#12846=CARTESIAN_POINT ( 'NONE',  ( -13.57458050278340167, 1434.962060795229945, 148.8580072349309944 ) ) ;
#12849=FACE_OUTER_BOUND ( 'NONE', #49693, .T. ) ;
#12852=ADVANCED_FACE ( 'NONE', ( #81297 ), #77652, .F. ) ;
#12853=CARTESIAN_POINT ( 'NONE',  ( -4.322907466360000002E-09, 1413.741945241729809, 248.5896189551980058 ) ) ;
#12855=CARTESIAN_POINT ( 'NONE',  ( -11.02848032900000064, 1426.931206522629736, 92.75091704169790319 ) ) ;
#12856=CARTESIAN_POINT ( 'NONE',  ( 2.447291524873689738E-14, 1423.636407223090146, 230.6287594130560024 ) ) ;
#12858=CARTESIAN_POINT ( 'NONE',  ( -25.00557959500000038, 1439.269656963860143, 216.3898167378279993 ) ) ;
#12860=EDGE_CURVE ( 'NONE', #57270, #38397, #9499, .T. ) ;
#12861=CARTESIAN_POINT ( 'NONE',  ( 0.7590917812330791881, 1415.513639922078028, 233.2736437612532825 ) ) ;
#12862=CARTESIAN_POINT ( 'NONE',  ( 27.01382310970000233, 1451.969724731730139, 134.9184576876980088 ) ) ;
#12863=ORIENTED_EDGE ( 'NONE', *, *, #18575, .T. ) ;
#12864=DIRECTION ( 'NONE',  ( 0.7636030818040332457, 6.919574257186762174E-11, 0.6456859402676993209 ) ) ;
#12866=B_SPLINE_CURVE_WITH_KNOTS ( 'NONE', 3,
 ( #86796, #62179, #63287, #97401, #106354, #20670, #35854, #29640, #97939, #52659 ),
 .UNSPECIFIED., .F., .F.,
 ( 4, 3, 3, 4 ),
 ( -157.4421957110000108, -134.5125350903350068, -78.90080931318131263, -29.52656374274130258 ),
 .UNSPECIFIED. ) ;
#12868=ORIENTED_EDGE ( 'NONE', *, *, #33938, .T. ) ;
#12871=CARTESIAN_POINT ( 'NONE',  ( -22.70505693412289716, 1409.705930895240272, 208.9454396691020008 ) ) ;
#12875=CARTESIAN_POINT ( 'NONE',  ( 4.291176059336820003, 1446.971469614359876, 154.7965853925720126 ) ) ;
#12876=CARTESIAN_POINT ( 'NONE',  ( -0.6623973197610000252, 1470.488054031330194, 235.6950254979980173 ) ) ;
#12883=ORIENTED_EDGE ( 'NONE', *, *, #69252, .F. ) ;
#12886=CARTESIAN_POINT ( 'NONE',  ( 12.80669964242905223, 1442.848007414932908, 186.8680711929162328 ) ) ;
#12887=ORIENTED_EDGE ( 'NONE', *, *, #21584, .F. ) ;
#12891=CARTESIAN_POINT ( 'NONE',  ( 13.43167347780000043, 1509.382104760729817, 235.1752220498979966 ) ) ;
#12892=( BOUNDED_CURVE ( )  B_SPLINE_CURVE ( 3, ( #45209, #17180, #1543, #51373 ),
 .UNSPECIFIED., .F., .T. ) 
 B_SPLINE_CURVE_WITH_KNOTS ( ( 4, 4 ),
 ( 1.861138363454700073, 2.499452639686874811 ),
 .UNSPECIFIED. ) 
 CURVE ( )  GEOMETRIC_REPRESENTATION_ITEM ( )  RATIONAL_B_SPLINE_CURVE ( ( 1.000000000000000000, 0.9663334780259177359, 0.9663334780259177359, 1.000000000000000000 ) ) 
 REPRESENTATION_ITEM ( '' )  );
#12894=CARTESIAN_POINT ( 'NONE',  ( 13.66841340714169917, 1452.435748873430157, 148.7307978952950123 ) ) ;
#12898=CARTESIAN_POINT ( 'NONE',  ( -10.97167842400910054, 1432.478566107110055, 151.7700680134270215 ) ) ;
#12899=CARTESIAN_POINT ( 'NONE',  ( 0.000000000000000000, 1508.913060387330006, 224.7618459619980058 ) ) ;
#12900=CARTESIAN_POINT ( 'NONE',  ( -1.600048698852036821, 1411.254281879943164, 137.0999999980979851 ) ) ;
#12902=CARTESIAN_POINT ( 'NONE',  ( -24.12862833684370045, 1508.487934531239944, 222.3657772772859857 ) ) ;
#12904=ORIENTED_EDGE ( 'NONE', *, *, #84370, .T. ) ;
#12910=CARTESIAN_POINT ( 'NONE',  ( -4.146782895030730387, 1426.018316030089863, 186.1121555109529879 ) ) ;
#12912=CARTESIAN_POINT ( 'NONE',  ( -2.746125756363450243, 1440.068789215269817, 157.5210582709530058 ) ) ;
#12916=CARTESIAN_POINT ( 'NONE',  ( 12.93742170084699872, 1415.431750870129918, 196.9031077866209785 ) ) ;
#12918=B_SPLINE_CURVE_WITH_KNOTS ( 'NONE', 5,
 ( #9384, #110736, #43547, #35132, #69314, #103421, #60918, #18315, #52506, #86635, #28395, #62595, #11596, #89403, #63142 ),
 .UNSPECIFIED., .F., .F.,
 ( 6, 3, 3, 3, 6 ),
 ( 0.000000000000000000, 0.2487888922080676302, 0.5151303747020953283, 0.7162082858933614959, 1.000000000000000000 ),
 .UNSPECIFIED. ) ;
#12920=CARTESIAN_POINT ( 'NONE',  ( 14.98057229850000027, 1422.105921276430081, 228.0570637948979993 ) ) ;
#12923=CARTESIAN_POINT ( 'NONE',  ( 43.99407931230000202, 1429.912879050529909, 268.5626800188979928 ) ) ;
#12924=CARTESIAN_POINT ( 'NONE',  ( -18.23736806889999684, 1410.046425294630126, 223.9609750991980093 ) ) ;
#12925=CARTESIAN_POINT ( 'NONE',  ( 16.20369265950000326, 1435.886343892520017, 148.6899262114979763 ) ) ;
#12926=CARTESIAN_POINT ( 'NONE',  ( -1.341411944869999928, 1418.672989064230023, 228.1617829935980239 ) ) ;
#12927=CARTESIAN_POINT ( 'NONE',  ( 20.22895499020875576, 1427.701001985137054, 222.9553950507804814 ) ) ;
#12928=CARTESIAN_POINT ( 'NONE',  ( -17.73407118999999810, 1423.343216095430080, 226.1884512641980223 ) ) ;
#12930=CARTESIAN_POINT ( 'NONE',  ( -34.93809870825160147, 1435.719286479559969, 135.4750084030100084 ) ) ;
#12931=CARTESIAN_POINT ( 'NONE',  ( 0.2168213374743849786, 1453.534145733320202, 183.2304789241289882 ) ) ;
#12932=CARTESIAN_POINT ( 'NONE',  ( -8.967593744529999356, 1409.166218292129997, 220.9728305157979946 ) ) ;
#12933=CARTESIAN_POINT ( 'NONE',  ( -0.1387231356229999824, 1418.535612649829773, 184.6749245791980059 ) ) ;
#12935=CARTESIAN_POINT ( 'NONE',  ( -28.64126805841279833, 1509.753974595000273, 211.2596818611239939 ) ) ;
#12936=CARTESIAN_POINT ( 'NONE',  ( 12.91324334049999933, 1434.774337969269936, 147.6246349161979765 ) ) ;
#12937=CARTESIAN_POINT ( 'NONE',  ( 12.53380499169999851, 1445.052233488290085, 169.4755105685979970 ) ) ;
#12938=CARTESIAN_POINT ( 'NONE',  ( 7.146336540040000074, 1441.350815057550108, 185.4538290344979714 ) ) ;
#12941=CARTESIAN_POINT ( 'NONE',  ( 39.43202460889999372, 1438.613999458619901, 136.5563049865980076 ) ) ;
#12945=CARTESIAN_POINT ( 'NONE',  ( -46.27884720130000318, 1440.913036523590108, 267.5894368609980347 ) ) ;
#12946=CARTESIAN_POINT ( 'NONE',  ( -11.76640019110000068, 1437.123680669209989, 147.7210023317979903 ) ) ;
#12947=CARTESIAN_POINT ( 'NONE',  ( 19.76088122879999887, 1434.994518313850222, 210.4584719956679919 ) ) ;
#12948=CARTESIAN_POINT ( 'NONE',  ( -24.93044165159999892, 1508.532778223230025, 220.3720830472979912 ) ) ;
#12953=CARTESIAN_POINT ( 'NONE',  ( -27.77560365120000085, 1451.943158935029942, 134.8960326030979786 ) ) ;
#12961=CARTESIAN_POINT ( 'NONE',  ( 0.003812576784339999879, 1466.393772618229832, 235.6965108690979775 ) ) ;
#12962=CARTESIAN_POINT ( 'NONE',  ( 22.52035456810000014, 1409.863932199730016, 213.1945697568480114 ) ) ;
#12966=CARTESIAN_POINT ( 'NONE',  ( -11.77090792110000095, 1432.440105173310030, 150.8116828678980141 ) ) ;
#12968=CARTESIAN_POINT ( 'NONE',  ( 28.15873685633160051, 1508.155813927709914, 208.2598873620850100 ) ) ;
#12971=FACE_OUTER_BOUND ( 'NONE', #74099, .T. ) ;
#12974=CARTESIAN_POINT ( 'NONE',  ( -8.348176302887580391, 1484.298473836920039, 184.3911193790379741 ) ) ;
#12977=CARTESIAN_POINT ( 'NONE',  ( 18.83207817909999804, 1416.311719782429918, 210.6697760117079952 ) ) ;
#12979=VERTEX_POINT ( 'NONE', #45932 ) ;
#12980=ORIENTED_EDGE ( 'NONE', *, *, #97538, .F. ) ;
#12981=CARTESIAN_POINT ( 'NONE',  ( 28.09217170250000351, 1508.632189945129994, 210.4865295626480020 ) ) ;
#12985=CARTESIAN_POINT ( 'NONE',  ( 0.7625704858929999164, 1427.674934138829940, 112.4493539157979995 ) ) ;
#12988=CARTESIAN_POINT ( 'NONE',  ( -24.43329073687169739, 1451.996401077730070, 136.8824426089099973 ) ) ;
#12989=CARTESIAN_POINT ( 'NONE',  ( -10.81509838440000060, 1424.921163249430037, 144.1641696258980119 ) ) ;
#12990=CARTESIAN_POINT ( 'NONE',  ( 14.33852263799999882, 1409.413772630230142, 226.7380482434979854 ) ) ;
#12993=CARTESIAN_POINT ( 'NONE',  ( 39.63067020500510296, 1438.364472239110000, 134.0999999979140114 ) ) ;
#12996=CARTESIAN_POINT ( 'NONE',  ( -16.80365118935687363, 1410.870881529783446, 226.3880813221334449 ) ) ;
#12999=ORIENTED_EDGE ( 'NONE', *, *, #68110, .T. ) ;
#13000=CARTESIAN_POINT ( 'NONE',  ( 10.01592177394908134, 1410.637502406660360, 229.8105954444164354 ) ) ;
#13003=CARTESIAN_POINT ( 'NONE',  ( -3.092456351079999610, 1485.137949221930057, 183.1787329613979978 ) ) ;
#13004=CARTESIAN_POINT ( 'NONE',  ( -17.59211063817642895, 1448.069329004949168, 217.8528919356413667 ) ) ;
#13007=CARTESIAN_POINT ( 'NONE',  ( -1.115466430919999974, 1497.688001115629959, 231.6381069598980105 ) ) ;
#13008=CARTESIAN_POINT ( 'NONE',  ( 7.803088030789999685, 1414.971262582530017, 194.2636415098980081 ) ) ;
#13013=CARTESIAN_POINT ( 'NONE',  ( 11.33192160910000013, 1414.988015876829877, 222.3303154034980196 ) ) ;
#13014=CARTESIAN_POINT ( 'NONE',  ( 18.79931365210000038, 1467.189280536129900, 227.8818516051979941 ) ) ;
#13016=CARTESIAN_POINT ( 'NONE',  ( -0.2055871306533119947, 1452.986193894690132, 183.2455700887460068 ) ) ;
#13019=CARTESIAN_POINT ( 'NONE',  ( -24.34734233041475093, 1439.542451668733065, 212.0350045365903497 ) ) ;
#13022=CARTESIAN_POINT ( 'NONE',  ( 2.764799436670000166, 1406.050782495030035, 266.9581426506979938 ) ) ;
#13024=CARTESIAN_POINT ( 'NONE',  ( 25.50965763837719891, 1477.613428519450053, 206.2229539054640099 ) ) ;
#13025=EDGE_CURVE ( 'NONE', #102287, #55469, #29534, .T. ) ;
#13026=CARTESIAN_POINT ( 'NONE',  ( 15.73405928501899886, 1409.498448401794349, 192.5840719006893949 ) ) ;
#13028=DIRECTION ( 'NONE',  ( 0.3363363969979660806, 0.9417419115949053898, 0.000000000000000000 ) ) ;
#13032=CARTESIAN_POINT ( 'NONE',  ( -20.46400528210000047, 1470.815019615029996, 209.2097780812300130 ) ) ;
#13033=CARTESIAN_POINT ( 'NONE',  ( 18.42577555256999844, 1424.509265906519886, 223.4215472205989954 ) ) ;
#13037=CARTESIAN_POINT ( 'NONE',  ( 10.82580776920000076, 1458.182933819829941, 213.1729752121979971 ) ) ;
#13038=CARTESIAN_POINT ( 'NONE',  ( -11.84746402709999913, 1431.045614906520086, 149.8348319904980031 ) ) ;
#13043=CARTESIAN_POINT ( 'NONE',  ( -20.99010852809999861, 1470.085365941430155, 224.6554786799979979 ) ) ;
#13044=FACE_OUTER_BOUND ( 'NONE', #27093, .T. ) ;
#13046=VERTEX_POINT ( 'NONE', #47037 ) ;
#13048=CARTESIAN_POINT ( 'NONE',  ( 3.443661293909999976, 1405.813131581129937, 267.8489083852979888 ) ) ;
#13049=CARTESIAN_POINT ( 'NONE',  ( -4.653281936863520762, 1425.827070423550140, 186.2156739099499987 ) ) ;
#13050=EDGE_CURVE ( 'NONE', #7383, #102192, #44225, .T. ) ;
#13052=CARTESIAN_POINT ( 'NONE',  ( 23.23643549727285063, 1432.926938218388614, 215.5924835263426758 ) ) ;
#13053=EDGE_CURVE ( 'NONE', #42334, #96903, #20691, .T. ) ;
#13055=CARTESIAN_POINT ( 'NONE',  ( 11.60004869885203682, 1424.919899798115239, 136.4495436088716360 ) ) ;
#13056=ADVANCED_FACE ( 'NONE', ( #105838 ), #85664, .F. ) ;
#13058=CARTESIAN_POINT ( 'NONE',  ( -0.8745088286755380302, 1450.882521866100205, 155.0624047495070101 ) ) ;
#13059=CARTESIAN_POINT ( 'NONE',  ( -1.554659401664016727, 1451.069394390376146, 183.6377582331552674 ) ) ;
#13060=EDGE_CURVE ( 'NONE', #95045, #31004, #47900, .T. ) ;
#13061=CARTESIAN_POINT ( 'NONE',  ( -19.65651483509421382, 1486.193852463049325, 190.0039420846813982 ) ) ;
#13063=CARTESIAN_POINT ( 'NONE',  ( -13.54623986534339863, 1415.059973079209840, 220.4667060011670117 ) ) ;
#13065=CARTESIAN_POINT ( 'NONE',  ( -10.05164999069999965, 1426.487183120430245, 224.8635561966979708 ) ) ;
#13066=CARTESIAN_POINT ( 'NONE',  ( -26.90036304580700133, 1508.005472205750038, 211.7893878585630034 ) ) ;
#13068=CARTESIAN_POINT ( 'NONE',  ( -0.8789521870270000647, 1475.313312798630022, 269.4984183591980127 ) ) ;
#13073=CARTESIAN_POINT ( 'NONE',  ( -16.81223434880759982, 1414.913060387349788, 207.5743820648510223 ) ) ;
#13078=CARTESIAN_POINT ( 'NONE',  ( -11.06418126257080026, 1396.299430110810135, 209.4736323295360023 ) ) ;
#13081=CARTESIAN_POINT ( 'NONE',  ( -14.46398808510000045, 1422.169897544629976, 229.1124523973979876 ) ) ;
#13082=CARTESIAN_POINT ( 'NONE',  ( 19.61749532786501504, 1455.455351503277598, 225.9183519794877384 ) ) ;
#13084=CARTESIAN_POINT ( 'NONE',  ( -2.355634153848364942, 1410.373534213158564, 232.7087846842507588 ) ) ;
#13085=CARTESIAN_POINT ( 'NONE',  ( 2.671304308019999851, 1410.383647588429994, 231.6679768729979969 ) ) ;
#13088=CARTESIAN_POINT ( 'NONE',  ( 11.15439083589999925, 1426.467706535029947, 101.9064184266980106 ) ) ;
#13090=CARTESIAN_POINT ( 'NONE',  ( 11.74015320060000001, 1428.979986575930070, 144.1938086916980239 ) ) ;
#13091=EDGE_CURVE ( 'NONE', #35126, #33349, #26654, .T. ) ;
#13095=CARTESIAN_POINT ( 'NONE',  ( -9.609284535499998725, 1429.602790706330097, 148.1400166355980161 ) ) ;
#13096=CARTESIAN_POINT ( 'NONE',  ( 3.450834020359999865, 1508.929450314329870, 180.3008642914979873 ) ) ;
#13099=EDGE_CURVE ( 'NONE', #24662, #8790, #108574, .T. ) ;
#13103=ORIENTED_EDGE ( 'NONE', *, *, #53572, .T. ) ;
#13104=CARTESIAN_POINT ( 'NONE',  ( -10.56206167739999913, 1397.610775313830118, 200.9354534292479855 ) ) ;
#13105=CARTESIAN_POINT ( 'NONE',  ( 2.777171832513400052, 1409.013373976660205, 230.3099596325619984 ) ) ;
#13106=CARTESIAN_POINT ( 'NONE',  ( -1.326919707039999841, 1414.988017870030035, 226.4745228631980183 ) ) ;
#13107=CARTESIAN_POINT ( 'NONE',  ( -13.15002888018213056, 1444.757386539127083, 169.3984147371142512 ) ) ;
#13112=CARTESIAN_POINT ( 'NONE',  ( 12.12259107610000086, 1429.760645300329998, 188.8483479879979825 ) ) ;
#13114=CARTESIAN_POINT ( 'NONE',  ( -40.40395559827349814, 1447.793233377660044, 135.9869587023879944 ) ) ;
#13115=CARTESIAN_POINT ( 'NONE',  ( 11.01686548338170013, 1396.297777807429839, 210.2008554867939836 ) ) ;
#13117=CARTESIAN_POINT ( 'NONE',  ( 11.84480386869999968, 1430.772386585429786, 150.1926085328979923 ) ) ;
#13118=CARTESIAN_POINT ( 'NONE',  ( 40.26734871130000215, 1444.073094270329875, 137.1207092272979935 ) ) ;
#13120=CARTESIAN_POINT ( 'NONE',  ( 3.923287301289999807, 1424.011886354829812, 184.0527492022980027 ) ) ;
#13124=CARTESIAN_POINT ( 'NONE',  ( -18.50511553393410225, 1458.242655195800126, 227.6372299999850100 ) ) ;
#13125=CARTESIAN_POINT ( 'NONE',  ( -15.56902241549999921, 1459.426448572030040, 230.4822614389979947 ) ) ;
#13126=CARTESIAN_POINT ( 'NONE',  ( 3.663607833879999998, 1422.147183830330050, 212.8701394151179898 ) ) ;
#13127=CARTESIAN_POINT ( 'NONE',  ( 12.51099981750000012, 1416.825784017130218, 196.0986189373979869 ) ) ;
#13132=CARTESIAN_POINT ( 'NONE',  ( -2.970203372320949775, 1509.150402853229934, 179.1115872997399947 ) ) ;
#13134=CARTESIAN_POINT ( 'NONE',  ( 5.314269450500000325, 1416.216252248530054, 226.4136833372980107 ) ) ;
#13137=CARTESIAN_POINT ( 'NONE',  ( -20.67635594879999772, 1509.397142808630178, 229.5476599413979670 ) ) ;
#13138=CARTESIAN_POINT ( 'NONE',  ( -34.37676906152069023, 1423.369835011513487, 269.5228724793240076 ) ) ;
#13139=CARTESIAN_POINT ( 'NONE',  ( -0.7965761836729999823, 1409.108857835930166, 232.5344281013979924 ) ) ;
#13141=ORIENTED_EDGE ( 'NONE', *, *, #41774, .F. ) ;
#13142=CARTESIAN_POINT ( 'NONE',  ( 2.500000000000000000, 1419.365944793089966, 145.1180007323769985 ) ) ;
#13143=CARTESIAN_POINT ( 'NONE',  ( -29.89626096159269864, 1440.913060386809775, 238.0180708521619977 ) ) ;
#13147=CARTESIAN_POINT ( 'NONE',  ( 35.87497415728719830, 1421.176152893739982, 270.2893687456389671 ) ) ;
#13150=CARTESIAN_POINT ( 'NONE',  ( 22.75767681520000352, 1409.716280410829995, 208.6970310087830001 ) ) ;
#13156=CARTESIAN_POINT ( 'NONE',  ( -2.333469697930000031, 1420.450119961529936, 233.1581355964979707 ) ) ;
#13161=CARTESIAN_POINT ( 'NONE',  ( 18.89905520810000183, 1416.828042640230024, 210.6687957187479867 ) ) ;
#13162=CARTESIAN_POINT ( 'NONE',  ( 0.6621667027629999369, 1417.277712856329799, 235.8679543975979982 ) ) ;
#13163=CARTESIAN_POINT ( 'NONE',  ( -21.45144533046939728, 1509.599841436300039, 228.9220801472459925 ) ) ;
#13164=DIRECTION ( 'NONE',  ( 0.7087494536659948441, -1.509903313468208275E-11, 0.7054602837354869704 ) ) ;
#13166=DIRECTION ( 'NONE',  ( -0.001259577792888569910, -0.9990026034370939056, 0.04463419977654350251 ) ) ;
#13169=CARTESIAN_POINT ( 'NONE',  ( 18.24633262864339756, 1416.842625005220043, 209.2839319684169936 ) ) ;
#13170=DIRECTION ( 'NONE',  ( 0.03489949670246857150, -0.9993908270190969834, 0.000000000000000000 ) ) ;
#13178=ADVANCED_FACE ( 'NONE', ( #110225 ), #94621, .F. ) ;
#13183=CARTESIAN_POINT ( 'NONE',  ( -27.95267126734610130, 1509.877447535139936, 200.9175030071420167 ) ) ;
#13184=CARTESIAN_POINT ( 'NONE',  ( -2.500000000000000000, 1448.191388957439813, 168.9995349906980096 ) ) ;
#13185=CARTESIAN_POINT ( 'NONE',  ( -18.96805899230000136, 1425.896737524130003, 225.7257654465979897 ) ) ;
#13187=CARTESIAN_POINT ( 'NONE',  ( -5.319029970947924291, 1474.880592167660325, 269.6432403010445569 ) ) ;
#13189=CARTESIAN_POINT ( 'NONE',  ( 16.49310356919999876, 1438.571641227850023, 190.6611314653979719 ) ) ;
#13191=CARTESIAN_POINT ( 'NONE',  ( 28.82461957139999953, 1509.587741799730111, 209.3236985425249941 ) ) ;
#13195=CARTESIAN_POINT ( 'NONE',  ( -1.804213505890000180, 1410.351307731129964, 186.0507930254979954 ) ) ;
#13198=ADVANCED_FACE ( 'NONE', ( #36282 ), #55310, .T. ) ;
#13200=CARTESIAN_POINT ( 'NONE',  ( -0.9746356023110001043, 1408.913060387329779, 227.8345159065979715 ) ) ;
#13201=CARTESIAN_POINT ( 'NONE',  ( -18.66848659289999901, 1509.564978303230191, 231.0930269267980179 ) ) ;
#13202=CARTESIAN_POINT ( 'NONE',  ( -2.500000000000000000, 1425.944554418600092, 184.4763172118897785 ) ) ;
#13203=CARTESIAN_POINT ( 'NONE',  ( -13.38590766640819929, 1443.378323276218453, 187.0149398295905883 ) ) ;
#13204=CARTESIAN_POINT ( 'NONE',  ( -24.74784509953980205, 1438.337673821209819, 210.4711784212679788 ) ) ;
#13216=ORIENTED_EDGE ( 'NONE', *, *, #66097, .T. ) ;
#13218=CARTESIAN_POINT ( 'NONE',  ( 18.20034151899999841, 1415.948532224930204, 209.5286862425880088 ) ) ;
#13221=CARTESIAN_POINT ( 'NONE',  ( 16.03281798909471334, 1412.714820832511350, 269.3691768658688375 ) ) ;
#13222=CARTESIAN_POINT ( 'NONE',  ( -29.66529950549999839, 1450.991311267029914, 244.2516413496979908 ) ) ;
#13223=CARTESIAN_POINT ( 'NONE',  ( -20.47206495659999703, 1503.720923633429948, 190.5096218837979904 ) ) ;
#13224=EDGE_CURVE ( 'NONE', #84614, #80633, #51701, .T. ) ;
#13227=CARTESIAN_POINT ( 'NONE',  ( 11.68729876646599841, 1426.728740079569889, 140.6125123695689751 ) ) ;
#13229=CARTESIAN_POINT ( 'NONE',  ( -25.98834112620000170, 1441.634093611399976, 138.4860864867980297 ) ) ;
#13230=CARTESIAN_POINT ( 'NONE',  ( -24.39234959440000239, 1440.942615255600003, 211.3352088233380073 ) ) ;
#13236=CARTESIAN_POINT ( 'NONE',  ( 1.330142072575580153E-08, 1408.768101624430074, 261.3699198151659857 ) ) ;
#13239=CARTESIAN_POINT ( 'NONE',  ( -11.86071752599299955, 1431.960136582280029, 149.9694963188620136 ) ) ;
#13241=CARTESIAN_POINT ( 'NONE',  ( -25.90444642199999947, 1468.044424510629824, 270.1671806390979782 ) ) ;
#13242=CARTESIAN_POINT ( 'NONE',  ( -1.556886619979999997, 1415.063410501429871, 226.7642036972980009 ) ) ;
#13244=CARTESIAN_POINT ( 'NONE',  ( 35.25104840220150493, 1451.457745839210020, 135.5593480995689788 ) ) ;
#13245=CARTESIAN_POINT ( 'NONE',  ( 0.2091819028966719896, 1452.039107084460056, 183.0587606973180073 ) ) ;
#13247=CARTESIAN_POINT ( 'NONE',  ( 2.500000005229999989, 1448.233542442588032, 182.8968085845170037 ) ) ;
#13250=CARTESIAN_POINT ( 'NONE',  ( -27.47176941845090070, 1412.619294620689971, 267.2173682766330103 ) ) ;
#13252=CARTESIAN_POINT ( 'NONE',  ( -3.527569048119670203, 1486.518325592330029, 181.8541486797999767 ) ) ;
#13255=ORIENTED_EDGE ( 'NONE', *, *, #18621, .T. ) ;
#13259=CARTESIAN_POINT ( 'NONE',  ( -3.307305241536517393, 1441.238720758000682, 170.5343657646909321 ) ) ;
#13260=CARTESIAN_POINT ( 'NONE',  ( -17.30344447809999764, 1440.441197234099945, 190.6958610362979982 ) ) ;
#13262=CARTESIAN_POINT ( 'NONE',  ( -2.166650729859409097, 1450.000234473310456, 182.9036927443551690 ) ) ;
#13264=ORIENTED_EDGE ( 'NONE', *, *, #91628, .F. ) ;
#13265=CARTESIAN_POINT ( 'NONE',  ( 1.600048698852036821, 1402.754281879943164, 137.0999999980979851 ) ) ;
#13270=CARTESIAN_POINT ( 'NONE',  ( -42.11756425049719610, 1430.851161910550218, 270.3372090159310233 ) ) ;
#13271=CARTESIAN_POINT ( 'NONE',  ( 2.854350849340439922, 1416.619839790820151, 231.9963541232479827 ) ) ;
#13272=CARTESIAN_POINT ( 'NONE',  ( -2.546644429710000157, 1397.067797496830053, 196.4597125348979887 ) ) ;
#13276=CARTESIAN_POINT ( 'NONE',  ( 45.63713076155215731, 1440.913099924324115, 268.9747509450593839 ) ) ;
#13283=CARTESIAN_POINT ( 'NONE',  ( -20.19344737140000134, 1435.770039937179945, 222.9975873334980179 ) ) ;
#13285=CARTESIAN_POINT ( 'NONE',  ( 12.77587743780000018, 1416.568813547830132, 222.7009457741980327 ) ) ;
#13289=CARTESIAN_POINT ( 'NONE',  ( -36.37832868396120034, 1435.767865609909904, 135.3761632872109999 ) ) ;
#13290=CARTESIAN_POINT ( 'NONE',  ( -22.20861559396504603, 1452.332390273548299, 220.3331572959684195 ) ) ;
#13292=CARTESIAN_POINT ( 'NONE',  ( 2.786005956417805685, 1457.636688197868125, 228.7054548384536190 ) ) ;
#13293=EDGE_CURVE ( 'NONE', #38397, #3072, #38844, .T. ) ;
#13294=CARTESIAN_POINT ( 'NONE',  ( 14.30561690719999923, 1416.274718424630009, 196.7258643987979951 ) ) ;
#13295=DIRECTION ( 'NONE',  ( 0.004026485253168931785, 0.9999913661844075374, -0.001027118858027144602 ) ) ;
#13296=CARTESIAN_POINT ( 'NONE',  ( 20.92457307240000119, 1409.643762580330076, 205.0061534547180031 ) ) ;
#13300=CARTESIAN_POINT ( 'NONE',  ( 24.58073941009117291, 1443.411714615211622, 213.1237255199102378 ) ) ;
#13301=FACE_OUTER_BOUND ( 'NONE', #46050, .T. ) ;
#13305=CARTESIAN_POINT ( 'NONE',  ( 4.613723315850000479E-06, 1474.175172091230024, 270.1377426632980132 ) ) ;
#13308=CARTESIAN_POINT ( 'NONE',  ( -37.65379800284389944, 1449.104226875719860, 136.3438977234109757 ) ) ;
#13311=CARTESIAN_POINT ( 'NONE',  ( 18.01996314195137927, 1424.295345311109713, 225.2602986464550838 ) ) ;
#13314=CARTESIAN_POINT ( 'NONE',  ( -3.602921956033400071E-07, 1407.180382923570050, 222.1388580509179747 ) ) ;
#13315=CARTESIAN_POINT ( 'NONE',  ( 35.88934487943939899, 1440.913060387049882, 252.6421940191889632 ) ) ;
#13320=ORIENTED_EDGE ( 'NONE', *, *, #56827, .F. ) ;
#13323=EDGE_CURVE ( 'NONE', #108385, #69912, #9621, .T. ) ;
#13334=FACE_OUTER_BOUND ( 'NONE', #70550, .T. ) ;
#13336=CARTESIAN_POINT ( 'NONE',  ( 2.318246505679999903, 1464.667746032229843, 236.3197918910979922 ) ) ;
#13339=CARTESIAN_POINT ( 'NONE',  ( -0.5354439702209998764, 1451.096935658430084, 182.2556569121979919 ) ) ;
#13342=CARTESIAN_POINT ( 'NONE',  ( -17.65703761238349756, 1415.429375168339902, 208.7951508728979775 ) ) ;
#13346=B_SPLINE_CURVE_WITH_KNOTS ( 'NONE', 5,
 ( #40738, #66525, #92239, #49709, #83839, #110693, #33986, #7140, #102286, #25567, #75469, #109603 ),
 .UNSPECIFIED., .F., .F.,
 ( 6, 3, 3, 6 ),
 ( 0.000000000000000000, 0.3830643373806639218, 0.7943583785163387256, 1.000000000000000000 ),
 .UNSPECIFIED. ) ;
#13348=CARTESIAN_POINT ( 'NONE',  ( 36.10037600688230697, 1437.471261748140023, 136.5386461258349868 ) ) ;
#13352=CARTESIAN_POINT ( 'NONE',  ( 19.21355886149643055, 1509.590266407224817, 186.7400054175685113 ) ) ;
#13355=CARTESIAN_POINT ( 'NONE',  ( 18.80463711554499895, 1425.800691016006112, 225.6053601209239901 ) ) ;
#13358=CARTESIAN_POINT ( 'NONE',  ( -19.14657372330000129, 1478.162773027329877, 190.0467893125980083 ) ) ;
#13359=CARTESIAN_POINT ( 'NONE',  ( 11.30106291239999905, 1432.291791669059876, 151.5220416249979962 ) ) ;
#13360=CARTESIAN_POINT ( 'NONE',  ( -2.833916579333589869, 1449.814275768419975, 184.3649903733470126 ) ) ;
#13362=VERTEX_POINT ( 'NONE', #105933 ) ;
#13363=VECTOR ( 'NONE', #51012, 1000.000000000000000 ) ;
#13367=CARTESIAN_POINT ( 'NONE',  ( -11.68969520689999797, 1434.472878431520030, 151.2717061033980031 ) ) ;
#13369=CARTESIAN_POINT ( 'NONE',  ( -20.52883463880759862, 1505.559739956360090, 190.4562007501970129 ) ) ;
#13370=CARTESIAN_POINT ( 'NONE',  ( -24.71655169530576401, 1435.786948140999357, 137.7886807324425149 ) ) ;
#13375=CARTESIAN_POINT ( 'NONE',  ( -45.63478668459259779, 1440.473321573280145, 268.9749136988990017 ) ) ;
#13376=CARTESIAN_POINT ( 'NONE',  ( 14.01395624050939936, 1452.538953007629743, 222.8951477747749834 ) ) ;
#13379=CARTESIAN_POINT ( 'NONE',  ( 3.872712109488329890, 1407.067885255820102, 221.6343841272010025 ) ) ;
#13380=CARTESIAN_POINT ( 'NONE',  ( -13.66429424859150110, 1434.998729100779883, 149.0303311387329757 ) ) ;
#13382=B_SPLINE_SURFACE_WITH_KNOTS ( 'NONE', 5, 4, ( 
 ( #84587, #58304, #92426, #15701, #49904 ),
 ( #58854, #109262, #82938, #39843, #40937 ),
 ( #74006, #7878, #40384, #42047, #65613 ),
 ( #67270, #15162, #76198, #110344, #24112 ),
 ( #84039, #7337, #75660, #33617, #100296 ),
 ( #74561, #59419, #101362, #93531, #100825 ) ),
 .UNSPECIFIED., .F., .F., .F.,
 ( 6, 6 ),
 ( 5, 5 ),
 ( 0.000000000000000000, 111.1101480259999903 ),
 ( 25.81581217359999769, 39.03307591160000101 ),
 .UNSPECIFIED. ) ;
#13383=CARTESIAN_POINT ( 'NONE',  ( 6.440382586182271218, 1425.293263514254704, 226.4189292768371047 ) ) ;
#13386=CARTESIAN_POINT ( 'NONE',  ( 24.26836175920000116, 1418.067430823330142, 255.0044386299979919 ) ) ;
#13387=CARTESIAN_POINT ( 'NONE',  ( -27.85639448530000095, 1508.131721226830223, 206.6638992223579976 ) ) ;
#13389=CARTESIAN_POINT ( 'NONE',  ( -17.71298236049999986, 1410.454334518429960, 194.8352300936979873 ) ) ;
#13390=( BOUNDED_CURVE ( )  B_SPLINE_CURVE ( 3, ( #40800, #13926, #89549, #48113 ),
 .UNSPECIFIED., .F., .F. ) 
 B_SPLINE_CURVE_WITH_KNOTS ( ( 4, 4 ),
 ( 4.801238875923769633, 5.185567269779980393 ),
 .UNSPECIFIED. ) 
 CURVE ( )  GEOMETRIC_REPRESENTATION_ITEM ( )  RATIONAL_B_SPLINE_CURVE ( ( 1.000000000000000000, 0.9877288052443483624, 0.9877288052443483624, 1.000000000000000000 ) ) 
 REPRESENTATION_ITEM ( '' )  );
#13391=CARTESIAN_POINT ( 'NONE',  ( -8.718170062098048234, 1408.261133769854041, 270.1210666218138385 ) ) ;
#13392=CARTESIAN_POINT ( 'NONE',  ( -29.87496801789999878, 1438.990456365560021, 238.0574310508980318 ) ) ;
#13393=DIRECTION ( 'NONE',  ( -0.008080911954619110840, -0.2617474919842974757, -0.9651025589552190143 ) ) ;
#13394=CARTESIAN_POINT ( 'NONE',  ( -7.916648676117490346, 1452.636604923769937, 151.3511352965829815 ) ) ;
#13395=CARTESIAN_POINT ( 'NONE',  ( -18.89959501459999913, 1416.839692131129823, 207.5749782147480289 ) ) ;
#13399=CARTESIAN_POINT ( 'NONE',  ( -0.04627975075399999583, 1508.911444262829946, 238.5489451465980153 ) ) ;
#13400=ORIENTED_EDGE ( 'NONE', *, *, #84946, .F. ) ;
#13407=B_SPLINE_CURVE_WITH_KNOTS ( 'NONE', 5,
 ( #103031, #53223, #21096, #87362, #47437, #81561 ),
 .UNSPECIFIED., .F., .F.,
 ( 6, 6 ),
 ( 0.000000000000000000, 1.000000000000000000 ),
 .UNSPECIFIED. ) ;
#13408=CARTESIAN_POINT ( 'NONE',  ( -13.51912611120000030, 1489.054086407930072, 231.6518530692979994 ) ) ;
#13411=CARTESIAN_POINT ( 'NONE',  ( 46.27887280396929981, 1441.860040026859906, 267.5894435840550045 ) ) ;
#13412=CARTESIAN_POINT ( 'NONE',  ( -11.54244540313270129, 1414.913060387399810, 220.3473659478999878 ) ) ;
#13413=CARTESIAN_POINT ( 'NONE',  ( -0.06054275102980000156, 1420.434684236430030, 183.3377748591979923 ) ) ;
#13417=CARTESIAN_POINT ( 'NONE',  ( 13.45802170480480875, 1444.282616009370258, 187.8687362809869512 ) ) ;
#13424=CARTESIAN_POINT ( 'NONE',  ( 17.05418697632569902, 1452.317515055090098, 146.2608711844959828 ) ) ;
#13428=CARTESIAN_POINT ( 'NONE',  ( -10.98084453577630093, 1433.016921785290151, 151.7694248368179899 ) ) ;
#13429=CARTESIAN_POINT ( 'NONE',  ( 0.03447861350279703141, 1409.362621839177336, 232.8245751882662660 ) ) ;
#13433=CARTESIAN_POINT ( 'NONE',  ( -24.17892280350069711, 1508.624304443510027, 222.3905331272610226 ) ) ;
#13434=CARTESIAN_POINT ( 'NONE',  ( 11.29523459009999975, 1425.738185348830029, 112.3426556953979940 ) ) ;
#13435=ORIENTED_EDGE ( 'NONE', *, *, #35986, .F. ) ;
#13436=CARTESIAN_POINT ( 'NONE',  ( 2.984513020910000147, 1427.913060387330006, 209.1218459616979999 ) ) ;
#13437=CARTESIAN_POINT ( 'NONE',  ( -2.534203887357130203, 1421.318133204249989, 184.2270941939309807 ) ) ;
#13445=CARTESIAN_POINT ( 'NONE',  ( -2.461716435160000049, 1435.943783413959864, 150.4083956814980070 ) ) ;
#13447=CARTESIAN_POINT ( 'NONE',  ( -12.53380652166779896, 1445.052232296300190, 185.6742736269380032 ) ) ;
#13450=CARTESIAN_POINT ( 'NONE',  ( 13.01538513870689862, 1416.535698381769862, 196.3451722032600060 ) ) ;
#13454=CARTESIAN_POINT ( 'NONE',  ( 4.466626895270000119, 1422.096238294529940, 231.9296400908980047 ) ) ;
#13455=CARTESIAN_POINT ( 'NONE',  ( 0.03226293719758020068, 1410.297897419189894, 233.2219341505459909 ) ) ;
#13457=CARTESIAN_POINT ( 'NONE',  ( -18.56577482049999972, 1410.923936267830186, 223.7868423640980211 ) ) ;
#13459=CARTESIAN_POINT ( 'NONE',  ( -1.121218465919999963, 1416.837080256330182, 228.0853546198979984 ) ) ;
#13460=CARTESIAN_POINT ( 'NONE',  ( -4.219438644781110526, 1441.595895916910195, 183.5288106640859951 ) ) ;
#13461=CARTESIAN_POINT ( 'NONE',  ( 24.26322120380000058, 1437.059134594650232, 214.0566016570280112 ) ) ;
#13465=CARTESIAN_POINT ( 'NONE',  ( -40.51263981762689781, 1439.427258870550077, 135.2566580804950149 ) ) ;
#13466=CARTESIAN_POINT ( 'NONE',  ( -7.490735701819999370, 1414.913060387329779, 223.4518716291979956 ) ) ;
#13468=CARTESIAN_POINT ( 'NONE',  ( -6.425367583159999896, 1409.137439167629964, 223.2437179294980183 ) ) ;
#13469=CARTESIAN_POINT ( 'NONE',  ( -15.10946924899999999, 1415.087745006229852, 201.1701658454080075 ) ) ;
#13473=CARTESIAN_POINT ( 'NONE',  ( 12.06099931120000157, 1433.903617051039873, 149.0256926596979952 ) ) ;
#13474=CARTESIAN_POINT ( 'NONE',  ( -27.26054292650000122, 1435.602462706470078, 136.1497272824979916 ) ) ;
#13475=CARTESIAN_POINT ( 'NONE',  ( 9.098928921009999726, 1442.287229081999840, 185.1767890527980001 ) ) ;
#13476=ORIENTED_EDGE ( 'NONE', *, *, #95878, .T. ) ;
#13479=CARTESIAN_POINT ( 'NONE',  ( -11.93607054898440012, 1409.329877155629902, 218.1202972442949886 ) ) ;
#13483=CARTESIAN_POINT ( 'NONE',  ( 37.48449069387330468, 1421.396168078520759, 269.1919258218934488 ) ) ;
#13485=CARTESIAN_POINT ( 'NONE',  ( -10.81518761075750135, 1424.921099531289883, 144.1705495212430037 ) ) ;
#13490=CARTESIAN_POINT ( 'NONE',  ( -29.21489664634600203, 1509.775817166219895, 208.6508206576949931 ) ) ;
#13492=CARTESIAN_POINT ( 'NONE',  ( -16.78911523114979687, 1410.870482649229871, 226.4125133055940182 ) ) ;
#13501=CARTESIAN_POINT ( 'NONE',  ( -0.2485702761457760368, 1419.163708210889808, 184.5897658516240085 ) ) ;
#13502=CARTESIAN_POINT ( 'NONE',  ( 0.002025548741049999855, 1465.101603547730065, 237.0127861282980177 ) ) ;
#13503=CARTESIAN_POINT ( 'NONE',  ( 20.45064351119999912, 1410.549291213930019, 219.2538096947979795 ) ) ;
#13505=CARTESIAN_POINT ( 'NONE',  ( -1.795919047817160052, 1417.208812584569841, 185.7430934334929873 ) ) ;
#13507=CARTESIAN_POINT ( 'NONE',  ( -17.86706492440000105, 1424.552609962230008, 227.1966067826979838 ) ) ;
#13509=CARTESIAN_POINT ( 'NONE',  ( -11.61328182866063408, 1426.778534732830167, 135.3257729749631721 ) ) ;
#13510=CARTESIAN_POINT ( 'NONE',  ( 27.45153079662120277, 1488.737808995739897, 208.6597228503549957 ) ) ;
#13513=CARTESIAN_POINT ( 'NONE',  ( -24.02615488320000026, 1435.747509074109985, 211.0797796158580013 ) ) ;
#13516=CARTESIAN_POINT ( 'NONE',  ( -11.27431701509130058, 1484.787218902319864, 185.3755693123800086 ) ) ;
#13519=CARTESIAN_POINT ( 'NONE',  ( 14.20190145760000000, 1416.831305841230005, 196.5056575589980241 ) ) ;
#13521=ORIENTED_EDGE ( 'NONE', *, *, #12505, .F. ) ;
#13528=CARTESIAN_POINT ( 'NONE',  ( -10.79135257254849911, 1424.935556423300113, 142.6770767068849750 ) ) ;
#13529=CARTESIAN_POINT ( 'NONE',  ( 24.59498489902570029, 1440.913044926110160, 213.3385239659299941 ) ) ;
#13532=CARTESIAN_POINT ( 'NONE',  ( -24.22051753955809872, 1452.051472547239882, 136.7607190383920113 ) ) ;
#13533=CARTESIAN_POINT ( 'NONE',  ( -11.15489169059999952, 1425.160568487430055, 144.1681086605980227 ) ) ;
#13534=CARTESIAN_POINT ( 'NONE',  ( 12.32229772640000043, 1409.510185481929966, 228.2568190012979983 ) ) ;
#13536=SHAPE_DEFINITION_REPRESENTATION ( #2615, #49395 ) ;
#13537=CARTESIAN_POINT ( 'NONE',  ( 41.34669637366360462, 1445.942886885989992, 134.0999999985539830 ) ) ;
#13538=AXIS2_PLACEMENT_3D ( 'NONE', #100357, #98704, #23645 ) ;
#13539=( BOUNDED_CURVE ( )  B_SPLINE_CURVE ( 3, ( #66848, #100423, #33757, #92562 ),
 .UNSPECIFIED., .F., .F. ) 
 B_SPLINE_CURVE_WITH_KNOTS ( ( 4, 4 ),
 ( 4.731011162954751548, 4.740923033578477330 ),
 .UNSPECIFIED. ) 
 CURVE ( )  GEOMETRIC_REPRESENTATION_ITEM ( )  RATIONAL_B_SPLINE_CURVE ( ( 1.000000000000000000, 0.9999918129184852678, 0.9999918129184852678, 1.000000000000000000 ) ) 
 REPRESENTATION_ITEM ( '' )  );
#13540=CARTESIAN_POINT ( 'NONE',  ( -39.89415922108589996, 1441.413485003220103, 136.8703014936540114 ) ) ;
#13545=CARTESIAN_POINT ( 'NONE',  ( 13.44542361074219272, 1410.755498752201902, 228.3208216478837755 ) ) ;
#13553=CARTESIAN_POINT ( 'NONE',  ( 8.513185067469999368, 1416.823418193329871, 193.0629307024979937 ) ) ;
#13555=ORIENTED_EDGE ( 'NONE', *, *, #106659, .F. ) ;
#13559=CARTESIAN_POINT ( 'NONE',  ( 39.12848466419210069, 1440.913060387330006, 266.3488084145499784 ) ) ;
#13560=CARTESIAN_POINT ( 'NONE',  ( -0.001791162408697688979, 1451.698462366203557, 154.0731293207397812 ) ) ;
#13561=EDGE_LOOP ( 'NONE', ( #41763, #77920, #33546, #44076 ) ) ;
#13563=CARTESIAN_POINT ( 'NONE',  ( -16.05717579490000091, 1409.640429902829965, 192.0135573943979921 ) ) ;
#13564=DIRECTION ( 'NONE',  ( 0.000000000000000000, 1.000000000000000000, 0.000000000000000000 ) ) ;
#13565=B_SPLINE_CURVE_WITH_KNOTS ( 'NONE', 3,
 ( #81896, #5202, #39356, #73530, #56718, #90852, #82468, #5766, #83013, #6305, #108762, #32054, #66243, #33694, #76266, #7949, #75725, #67337, #102543, #136 ),
 .UNSPECIFIED., .F., .F.,
 ( 4, 2, 1, 2, 2, 2, 1, 1, 1, 2, 2, 4 ),
 ( 0.000000000000000000, 0.1249999999999671929, 0.1874999999999319433, 0.2187499999999147626, 0.2499999999998974987, 0.3749999999999085731, 0.4374999999999144018, 0.4687499999999174549, 0.4843749999999021894, 0.4921874999998945288, 0.4999999999998868683, 1.000000000000000000 ),
 .UNSPECIFIED. ) ;
#13569=CARTESIAN_POINT ( 'NONE',  ( -2.853750452219999900, 1508.244831386429951, 180.6847236935980163 ) ) ;
#13572=CARTESIAN_POINT ( 'NONE',  ( 11.91931064610000135, 1462.777662358629868, 231.7750175801980106 ) ) ;
#13573=CARTESIAN_POINT ( 'NONE',  ( -11.60004869885203505, 1422.719538780906987, 136.9994203799023751 ) ) ;
#13575=CARTESIAN_POINT ( 'NONE',  ( -22.70509189929999749, 1409.705932116229860, 208.9454376012710100 ) ) ;
#13578=CARTESIAN_POINT ( 'NONE',  ( 18.05155555704234160, 1447.068055369337799, 216.4740371628595028 ) ) ;
#13580=AXIS2_PLACEMENT_3D ( 'NONE', #79892, #88284, #70969 ) ;
#13586=CARTESIAN_POINT ( 'NONE',  ( 1.850459186030000239E-08, 1461.348673278630031, 221.5631610194979828 ) ) ;
#13587=CARTESIAN_POINT ( 'NONE',  ( -10.95393205669999936, 1431.218946973030143, 151.6850706372979971 ) ) ;
#13589=CARTESIAN_POINT ( 'NONE',  ( 2.188346568509999646, 1415.918919806530084, 232.1097023429979913 ) ) ;
#13591=CARTESIAN_POINT ( 'NONE',  ( 12.09590827429999926, 1445.294669298059944, 186.8687448601980066 ) ) ;
#13592=CARTESIAN_POINT ( 'NONE',  ( -24.98397261459999896, 1470.079709032829896, 213.5815951536679904 ) ) ;
#13593=CARTESIAN_POINT ( 'NONE',  ( -2.461141685384151234, 1421.750035621559618, 139.1420193482996410 ) ) ;
#13594=CARTESIAN_POINT ( 'NONE',  ( -2.296012628010000611, 1485.567333802330040, 182.6448570080980005 ) ) ;
#13597=CARTESIAN_POINT ( 'NONE',  ( 3.386199433509999857, 1406.870005270030106, 269.6463559134979846 ) ) ;
#13600=CIRCLE ( 'NONE', #76208, 1.999999999999921618 ) ;
#13602=CARTESIAN_POINT ( 'NONE',  ( 21.02260244975787629, 1428.161636300771761, 219.7400186835844522 ) ) ;
#13603=CARTESIAN_POINT ( 'NONE',  ( 18.70459388984919968, 1509.566239199539950, 186.5372755781170042 ) ) ;
#13604=CARTESIAN_POINT ( 'NONE',  ( 10.10004869885228196, 1422.222932908421399, 137.0999999980979567 ) ) ;
#13606=CARTESIAN_POINT ( 'NONE',  ( -2.499999999939920059, 1448.906648583599917, 155.3362572337090057 ) ) ;
#13608=CARTESIAN_POINT ( 'NONE',  ( 2.434526083211889791, 1449.527760230520016, 155.0642281637050246 ) ) ;
#13611=B_SPLINE_CURVE_WITH_KNOTS ( 'NONE', 3,
 ( #54951, #48194, #89077, #64456, #47092, #12363, #12912, #46551, #56589, #108633 ),
 .UNSPECIFIED., .F., .F.,
 ( 4, 2, 2, 2, 4 ),
 ( -0.1575290654450730021, -0.1192767518302590007, -0.08059141058286700687, -0.04144259288940019270, 0.000000000000000000 ),
 .UNSPECIFIED. ) ;
#13612=CARTESIAN_POINT ( 'NONE',  ( -5.052203702459999946, 1416.825952163429974, 255.3819207742980097 ) ) ;
#13613=CARTESIAN_POINT ( 'NONE',  ( -27.24294176985399929, 1507.989564505149929, 211.0449899648789938 ) ) ;
#13614=CARTESIAN_POINT ( 'NONE',  ( 2.707874995500000104, 1440.598919863020001, 162.2212737941979981 ) ) ;
#13615=CARTESIAN_POINT ( 'NONE',  ( -2.765183635730000145, 1475.775321107629907, 266.9581418145979796 ) ) ;
#13616=CARTESIAN_POINT ( 'NONE',  ( -4.225123281554489907, 1446.251028937339925, 166.4050594329440003 ) ) ;
#13622=B_SPLINE_CURVE_WITH_KNOTS ( 'NONE', 3,
 ( #100036, #23327, #49112, #98934 ),
 .UNSPECIFIED., .F., .F.,
 ( 4, 4 ),
 ( 0.000000000000000000, 1.000000000000000000 ),
 .UNSPECIFIED. ) ;
#13626=CARTESIAN_POINT ( 'NONE',  ( -18.88476838489999921, 1410.934753883030226, 196.4486472547980043 ) ) ;
#13628=CARTESIAN_POINT ( 'NONE',  ( -45.45115383179999924, 1437.791621493419825, 268.9798130223979911 ) ) ;
#13629=VERTEX_POINT ( 'NONE', #24626 ) ;
#13630=CARTESIAN_POINT ( 'NONE',  ( -23.64337456402409998, 1435.765682558080016, 212.0350035351450231 ) ) ;
#13632=CARTESIAN_POINT ( 'NONE',  ( -1.581688265954455330, 1426.946673137334528, 134.0999999980979851 ) ) ;
#13633=CARTESIAN_POINT ( 'NONE',  ( 11.70398732309999978, 1426.301175225830093, 141.8453807417980101 ) ) ;
#13636=CARTESIAN_POINT ( 'NONE',  ( 27.95267559299999860, 1445.173348664639889, 137.3670106792980050 ) ) ;
#13640=CARTESIAN_POINT ( 'NONE',  ( 7.316304300719999709, 1507.280216345330018, 182.6970440027980089 ) ) ;
#13645=ORIENTED_EDGE ( 'NONE', *, *, #100660, .T. ) ;
#13647=FACE_OUTER_BOUND ( 'NONE', #31595, .T. ) ;
#13648=CARTESIAN_POINT ( 'NONE',  ( -18.11398223329999979, 1409.545614585430030, 221.5743542847980052 ) ) ;
#13649=CARTESIAN_POINT ( 'NONE',  ( 2.017315236659999567, 1508.958728568330116, 238.2933174268979997 ) ) ;
#13650=CARTESIAN_POINT ( 'NONE',  ( -13.41779013147873556, 1444.382168163145707, 169.3666020351543580 ) ) ;
#13651=CARTESIAN_POINT ( 'NONE',  ( -26.37063482739999998, 1509.833943247529987, 196.6232252598979926 ) ) ;
#13654=CARTESIAN_POINT ( 'NONE',  ( 17.67011187210000145, 1416.263755027329807, 225.7720003271979863 ) ) ;
#13655=CARTESIAN_POINT ( 'NONE',  ( 3.391241998599999974, 1410.302160405929953, 185.8412960619979799 ) ) ;
#13657=CARTESIAN_POINT ( 'NONE',  ( -41.14067036663129784, 1444.183244330699836, 136.8991323217539957 ) ) ;
#13659=CARTESIAN_POINT ( 'NONE',  ( 11.05052638022029932, 1396.298953271829987, 208.4418276999739987 ) ) ;
#13660=CARTESIAN_POINT ( 'NONE',  ( 0.7186627752419999515, 1416.547221146729953, 190.3376467024980059 ) ) ;
#13661=CARTESIAN_POINT ( 'NONE',  ( 11.46948732749999955, 1425.744653023729825, 146.7325240263980106 ) ) ;
#13662=CARTESIAN_POINT ( 'NONE',  ( 8.118253553867917915, 1509.196863918152303, 180.9331809445035901 ) ) ;
#13668=DIRECTION ( 'NONE',  ( 0.03489949677361985775, 0.9993908270166123042, -2.608312631526985536E-10 ) ) ;
#13669=CARTESIAN_POINT ( 'NONE',  ( -15.19063573600000083, 1460.421792992729934, 229.0783609468980160 ) ) ;
#13670=CARTESIAN_POINT ( 'NONE',  ( -7.605711504302860249, 1407.218299713070110, 198.4634440487380118 ) ) ;
#13677=FACE_OUTER_BOUND ( 'NONE', #79414, .T. ) ;
#13680=ADVANCED_FACE ( 'NONE', ( #93504 ), #109236, .F. ) ;
#13683=ORIENTED_EDGE ( 'NONE', *, *, #1786, .T. ) ;
#13685=CARTESIAN_POINT ( 'NONE',  ( -20.65148373499999934, 1509.627424770630114, 230.2251059840980076 ) ) ;
#13687=CARTESIAN_POINT ( 'NONE',  ( -30.31662843376689764, 1419.814115720066638, 269.4742331920600691 ) ) ;
#13692=CARTESIAN_POINT ( 'NONE',  ( -0.006857176400948759853, 1451.190334390920043, 182.2890573962069993 ) ) ;
#13693=CARTESIAN_POINT ( 'NONE',  ( -28.26405544321290009, 1440.913060387430050, 232.2089891578019945 ) ) ;
#13696=CARTESIAN_POINT ( 'NONE',  ( 6.330344484264800009, 1409.538285424360083, 270.3701841699830197 ) ) ;
#13699=CARTESIAN_POINT ( 'NONE',  ( 22.79202929419999890, 1409.708931967830040, 208.9783749518630032 ) ) ;
#13700=CARTESIAN_POINT ( 'NONE',  ( -20.35720160430000192, 1509.285577334429945, 188.5733222705979983 ) ) ;
#13705=CARTESIAN_POINT ( 'NONE',  ( 22.51756156282889876, 1509.699390964210124, 227.9212218486820234 ) ) ;
#13708=CARTESIAN_POINT ( 'NONE',  ( 6.075340425011860113, 1422.570843986066166, 139.1419349980001812 ) ) ;
#13713=CARTESIAN_POINT ( 'NONE',  ( 1.533058233270000015, 1417.373139556630122, 235.5867829536979912 ) ) ;
#13715=CARTESIAN_POINT ( 'NONE',  ( -20.38982155428609744, 1508.363530249980158, 228.6178044578140032 ) ) ;
#13722=CARTESIAN_POINT ( 'NONE',  ( -22.53878221424140094, 1411.058442688259902, 212.0450776560099939 ) ) ;
#13727=ORIENTED_EDGE ( 'NONE', *, *, #47344, .T. ) ;
#13730=CARTESIAN_POINT ( 'NONE',  ( 23.99815499239999994, 1446.810867530319911, 216.6209177652979747 ) ) ;
#13731=CARTESIAN_POINT ( 'NONE',  ( 6.562075743890480872, 1439.579727447380037, 154.3677175799390398 ) ) ;
#13735=CARTESIAN_POINT ( 'NONE',  ( -27.75185986752750011, 1509.834791352900083, 200.9939385945500021 ) ) ;
#13736=CARTESIAN_POINT ( 'NONE',  ( -4.225063841879999949, 1446.249083902760276, 165.9135368162980058 ) ) ;
#13737=CARTESIAN_POINT ( 'NONE',  ( -19.90838456339999851, 1426.253534361829907, 222.6506651951980018 ) ) ;
#13738=CARTESIAN_POINT ( 'NONE',  ( -19.09679337948567834, 1472.008470696052427, 269.5331241273682394 ) ) ;
#13740=CARTESIAN_POINT ( 'NONE',  ( 16.69260089830000027, 1445.375861641200117, 190.4510651168980075 ) ) ;
#13742=CARTESIAN_POINT ( 'NONE',  ( -18.44765774540020331, 1436.509381524827404, 212.9697281596460243 ) ) ;
#13743=CARTESIAN_POINT ( 'NONE',  ( -34.90552475763031737, 1457.877490100739578, 269.5302477027990449 ) ) ;
#13745=LINE ( 'NONE', #71524, #19489 ) ;
#13747=CARTESIAN_POINT ( 'NONE',  ( -10.75110831211170925, 1424.962421341598429, 140.1405872077429535 ) ) ;
#13749=CARTESIAN_POINT ( 'NONE',  ( -4.963802804109999300, 1497.713060387329961, 230.9126810519979927 ) ) ;
#13750=CARTESIAN_POINT ( 'NONE',  ( 1.461527277530950020, 1494.461654286979865, 181.6651345972479703 ) ) ;
#13751=CARTESIAN_POINT ( 'NONE',  ( -0.1669645939030000026, 1417.346234731630148, 235.5731359111979941 ) ) ;
#13753=CARTESIAN_POINT ( 'NONE',  ( -13.41712910526564428, 1444.385627665757056, 186.9257196579762592 ) ) ;
#13755=CARTESIAN_POINT ( 'NONE',  ( -16.68599179819999989, 1461.099982565929849, 230.2790296985980092 ) ) ;
#13759=CARTESIAN_POINT ( 'NONE',  ( 24.18632888440000173, 1435.416476431710180, 137.3041773823979952 ) ) ;
#13761=FACE_OUTER_BOUND ( 'NONE', #62968, .T. ) ;
#13766=ORIENTED_EDGE ( 'NONE', *, *, #8063, .T. ) ;
#13769=CARTESIAN_POINT ( 'NONE',  ( 34.62851765911016599, 1423.653131627848325, 269.5264373704582113 ) ) ;
#13770=CARTESIAN_POINT ( 'NONE',  ( -30.53571888319999772, 1440.913060387119913, 240.1260121746980190 ) ) ;
#13771=CARTESIAN_POINT ( 'NONE',  ( -20.32871120239999740, 1505.119216028529991, 189.5393039330980116 ) ) ;
#13772=CARTESIAN_POINT ( 'NONE',  ( -11.67569575809999982, 1433.467371848380026, 150.9894905005979808 ) ) ;
#13774=CARTESIAN_POINT ( 'NONE',  ( 22.52609270479999992, 1509.699688878229836, 209.5602205471840023 ) ) ;
#13775=CARTESIAN_POINT ( 'NONE',  ( -19.21919559470000394, 1486.268158006530030, 189.5244098630979863 ) ) ;
#13776=AXIS2_PLACEMENT_3D ( 'NONE', #50255, #100081, #110682 ) ;
#13777=CARTESIAN_POINT ( 'NONE',  ( 26.41765092578760132, 1465.529458439430073, 209.4782902591080074 ) ) ;
#13778=EDGE_CURVE ( 'NONE', #22756, #88339, #100798, .T. ) ;
#13779=CARTESIAN_POINT ( 'NONE',  ( -14.94707557629999961, 1464.258769156330118, 228.3755978434980136 ) ) ;
#13781=LINE ( 'NONE', #98358, #26469 ) ;
#13784=CARTESIAN_POINT ( 'NONE',  ( -11.05535904383813772, 1509.424240718018382, 237.0105353482844350 ) ) ;
#13785=CARTESIAN_POINT ( 'NONE',  ( 1.580222541931140213E-08, 1407.992705438240137, 263.0165072346359807 ) ) ;
#13787=ORIENTED_EDGE ( 'NONE', *, *, #54464, .T. ) ;
#13788=CARTESIAN_POINT ( 'NONE',  ( -11.86521650604180067, 1432.274229656389934, 149.9820447970350017 ) ) ;
#13790=CARTESIAN_POINT ( 'NONE',  ( -25.76377174219999944, 1467.778888206429883, 270.2932678896979724 ) ) ;
#13791=CARTESIAN_POINT ( 'NONE',  ( 12.76760079159999961, 1508.356069781229962, 233.5455612081979950 ) ) ;
#13793=CARTESIAN_POINT ( 'NONE',  ( 35.95601944595329513, 1451.436210798189904, 134.6957181338510168 ) ) ;
#13797=CARTESIAN_POINT ( 'NONE',  ( 12.59722465782060929, 1416.835288274323830, 223.3994078652815745 ) ) ;
#13800=CARTESIAN_POINT ( 'NONE',  ( -33.58184217919399828, 1416.684724268960053, 268.5991851112240170 ) ) ;
#13806=CARTESIAN_POINT ( 'NONE',  ( 4.881181484400870296, 1423.435338320519350, 184.1811047220472517 ) ) ;
#13807=EDGE_CURVE ( 'NONE', #46504, #104636, #82961, .T. ) ;
#13809=CARTESIAN_POINT ( 'NONE',  ( -2.959283871624123652, 1440.912977528160809, 170.5323342040075545 ) ) ;
#13810=CARTESIAN_POINT ( 'NONE',  ( -16.90743626299999747, 1425.425775615030034, 191.1833389174979914 ) ) ;
#13812=CARTESIAN_POINT ( 'NONE',  ( -2.338681342886227643, 1449.681344963495803, 182.9863964398574865 ) ) ;
#13814=CARTESIAN_POINT ( 'NONE',  ( -26.33338208449999840, 1436.244409726509957, 136.6927053810979942 ) ) ;
#13815=EDGE_CURVE ( 'NONE', #38555, #69834, #64344, .T. ) ;
#13818=CARTESIAN_POINT ( 'NONE',  ( -35.15123146724445746, 1451.685553865498377, 134.6826639932257024 ) ) ;
#13822=CARTESIAN_POINT ( 'NONE',  ( -2.494988787169999611, 1396.538086358129931, 196.8133008506979991 ) ) ;
#13825=ORIENTED_EDGE ( 'NONE', *, *, #92728, .F. ) ;
#13829=CARTESIAN_POINT ( 'NONE',  ( -13.31006320136440024, 1436.110929636480023, 150.6000258946120312 ) ) ;
#13830=CARTESIAN_POINT ( 'NONE',  ( -0.03701251498699020120, 1409.597194001649996, 185.2367800943269742 ) ) ;
#13833=B_SPLINE_CURVE_WITH_KNOTS ( 'NONE', 3,
 ( #87361, #10657, #11216, #46479, #45380, #80611, #63830 ),
 .UNSPECIFIED., .F., .F.,
 ( 4, 3, 4 ),
 ( -157.6565403109999863, -100.4035695696150015, -30.32814665380000463 ),
 .UNSPECIFIED. ) ;
#13836=CARTESIAN_POINT ( 'NONE',  ( -19.49135957599999713, 1435.772693388610151, 224.3034628955980168 ) ) ;
#13839=CARTESIAN_POINT ( 'NONE',  ( 11.87714094419999888, 1445.674110516890096, 187.3195964094980184 ) ) ;
#13843=CARTESIAN_POINT ( 'NONE',  ( -12.81185530964340025, 1416.835419214280137, 196.2456592538570135 ) ) ;
#13845=CARTESIAN_POINT ( 'NONE',  ( 7.392443486661196772, 1456.543737492606169, 227.5801189955647885 ) ) ;
#13846=CARTESIAN_POINT ( 'NONE',  ( 24.11264749536519858, 1452.065943334660005, 136.7679447854590080 ) ) ;
#13847=CARTESIAN_POINT ( 'NONE',  ( 13.25967437329999932, 1414.983773852829927, 197.8194332346980104 ) ) ;
#13850=CARTESIAN_POINT ( 'NONE',  ( 18.78254047960000150, 1409.568961153929877, 198.1179043739980159 ) ) ;
#13853=ADVANCED_FACE ( 'NONE', ( #70917 ), #70360, .F. ) ;
#13854=CARTESIAN_POINT ( 'NONE',  ( -0.07181796816713301168, 1506.512156835258793, 187.0734039034420562 ) ) ;
#13855=CARTESIAN_POINT ( 'NONE',  ( 24.59034321158132030, 1443.280774260655335, 213.0723101612708206 ) ) ;
#13857=CARTESIAN_POINT ( 'NONE',  ( 2.500000000000000000, 1439.559074696859852, 165.1937459529769967 ) ) ;
#13859=ORIENTED_EDGE ( 'NONE', *, *, #107025, .T. ) ;
#13863=CARTESIAN_POINT ( 'NONE',  ( -2.500000000000000000, 1448.552414648389913, 183.1264116536979998 ) ) ;
#13864=CARTESIAN_POINT ( 'NONE',  ( 0.2699275208915274948, 1452.980711559484462, 183.2606270490059615 ) ) ;
#13866=CARTESIAN_POINT ( 'NONE',  ( 11.31084951485244439, 1425.493973826349475, 138.7225535732650883 ) ) ;
#13867=FACE_OUTER_BOUND ( 'NONE', #26592, .T. ) ;
#13868=CARTESIAN_POINT ( 'NONE',  ( -2.500000000000000000, 1429.342233201230101, 157.2075084771979903 ) ) ;
#13871=CARTESIAN_POINT ( 'NONE',  ( 30.29215768548720078, 1440.913060385460085, 239.2711865524379959 ) ) ;
#13876=B_SPLINE_CURVE_WITH_KNOTS ( 'NONE', 3,
 ( #71531, #83190, #92679, #75892, #99972, #109499, #82072 ),
 .UNSPECIFIED., .F., .F.,
 ( 4, 3, 4 ),
 ( 4.902660412303320943E-05, 0.0008424868313097026457, 0.002262927881332990609 ),
 .UNSPECIFIED. ) ;
#13877=CARTESIAN_POINT ( 'NONE',  ( 11.23388613411650638, 1442.762691980111640, 207.0699376370758955 ) ) ;
#13878=AXIS2_PLACEMENT_3D ( 'NONE', #77283, #75081, #92395 ) ;
#13880=CARTESIAN_POINT ( 'NONE',  ( -1.160688383098266607, 1409.478226354181515, 185.8299063934154276 ) ) ;
#13883=VECTOR ( 'NONE', #40248, 1000.000000000000114 ) ;
#13885=EDGE_CURVE ( 'NONE', #84300, #9928, #40971, .T. ) ;
#13892=CARTESIAN_POINT ( 'NONE',  ( 1.594477961910000019, 1465.161208926829886, 235.7125682595980152 ) ) ;
#13895=CARTESIAN_POINT ( 'NONE',  ( -0.4378289194489999869, 1452.327479224130002, 183.2409674511980029 ) ) ;
#13903=CARTESIAN_POINT ( 'NONE',  ( 35.00372651682169334, 1437.143722424219959, 136.5385674641080129 ) ) ;
#13911=DIRECTION ( 'NONE',  ( 0.000000000000000000, 1.000000000000000000, 0.000000000000000000 ) ) ;
#13912=CARTESIAN_POINT ( 'NONE',  ( 18.28980197170000110, 1425.401422957629848, 225.1796033777980028 ) ) ;
#13914=CARTESIAN_POINT ( 'NONE',  ( -18.58834951790000289, 1452.000874628230122, 191.0927309286979892 ) ) ;
#13916=LINE ( 'NONE', #74421, #46317 ) ;
#13918=ORIENTED_EDGE ( 'NONE', *, *, #25586, .T. ) ;
#13920=CARTESIAN_POINT ( 'NONE',  ( 18.98230138205870077, 1456.646672190919844, 228.3944069568109967 ) ) ;
#13921=CARTESIAN_POINT ( 'NONE',  ( -13.07625826729999829, 1434.964688253329996, 150.0206613299980063 ) ) ;
#13922=B_SPLINE_CURVE_WITH_KNOTS ( 'NONE', 5,
 ( #11265, #1211, #9581, #86297, #71186, #103080, #88515, #44315, #43210, #105308, #77359, #26381 ),
 .UNSPECIFIED., .F., .F.,
 ( 6, 3, 3, 6 ),
 ( 22.90453557749570024, 35.06371889219999360, 67.00219837880000284, 78.53166967965620415 ),
 .UNSPECIFIED. ) ;
#13925=CARTESIAN_POINT ( 'NONE',  ( -20.29633810112639836, 1498.028987413850246, 190.6747321216680007 ) ) ;
#13926=CARTESIAN_POINT ( 'NONE',  ( 6.447768684100981140, 1509.138221431309603, 237.9469272652861775 ) ) ;
#13935=CARTESIAN_POINT ( 'NONE',  ( -15.26161778761860077, 1417.220034897830146, 226.9233734088860217 ) ) ;
#13936=CARTESIAN_POINT ( 'NONE',  ( 1.303375595325469982, 1408.418417958420150, 222.6667617130129884 ) ) ;
#13937=CARTESIAN_POINT ( 'NONE',  ( -13.17087381283750069, 1434.856356709339934, 149.0413483970049811 ) ) ;
#13939=CARTESIAN_POINT ( 'NONE',  ( -1.132427485120000064E-14, 1421.588970873729977, 90.97065375769790307 ) ) ;
#13942=CARTESIAN_POINT ( 'NONE',  ( 36.81312681149999833, 1438.597774589839901, 254.5659337911980060 ) ) ;
#13943=CARTESIAN_POINT ( 'NONE',  ( -26.66930585420000099, 1508.126733771030104, 202.3624711673980130 ) ) ;
#13944=CARTESIAN_POINT ( 'NONE',  ( -2.534380535060000383, 1489.036591809629954, 181.6187424111979851 ) ) ;
#13945=CARTESIAN_POINT ( 'NONE',  ( 28.15443155984639745, 1509.896245780209938, 217.4026704617729990 ) ) ;
#13946=CARTESIAN_POINT ( 'NONE',  ( 1.454856650999370338, 1507.661996469931182, 181.0451578313067387 ) ) ;
#13947=CARTESIAN_POINT ( 'NONE',  ( -2.499803828369999546E-09, 1418.297051470129873, 231.7760247027979972 ) ) ;
#13948=CARTESIAN_POINT ( 'NONE',  ( -29.14950047876969563, 1509.937906416141459, 204.4881255053639109 ) ) ;
#13949=ADVANCED_FACE ( 'NONE', ( #83676 ), #40577, .F. ) ;
#13950=CARTESIAN_POINT ( 'NONE',  ( -15.09100122165660096, 1452.386071012250113, 147.7982250704480123 ) ) ;
#13951=CARTESIAN_POINT ( 'NONE',  ( -18.64618908219999938, 1416.835809767629826, 208.5595418432099848 ) ) ;
#13955=CARTESIAN_POINT ( 'NONE',  ( -0.04733364164779999689, 1508.924981715130116, 238.6962721304979880 ) ) ;
#13959=AXIS2_PLACEMENT_3D ( 'NONE', #98850, #90996, #59082 ) ;
#13960=CARTESIAN_POINT ( 'NONE',  ( 2.902343876856320115, 1466.632250330839952, 234.1422825383600070 ) ) ;
#13961=CARTESIAN_POINT ( 'NONE',  ( -24.05637053410000092, 1410.857966063630101, 209.5800563058490127 ) ) ;
#13963=ORIENTED_EDGE ( 'NONE', *, *, #31840, .T. ) ;
#13968=ADVANCED_FACE ( 'NONE', ( #40026 ), #51737, .F. ) ;
#13969=CARTESIAN_POINT ( 'NONE',  ( -6.824245157110000015, 1498.345970854529924, 235.3115248808979914 ) ) ;
#13970=CARTESIAN_POINT ( 'NONE',  ( 5.496544696010749576, 1440.579441483889923, 154.7743156854139954 ) ) ;
#13972=CARTESIAN_POINT ( 'NONE',  ( 45.23156575188859563, 1448.572260723799900, 267.6264533449969463 ) ) ;
#13973=CARTESIAN_POINT ( 'NONE',  ( -11.22084002886469989, 1414.913060387399810, 220.6193154192710040 ) ) ;
#13974=CARTESIAN_POINT ( 'NONE',  ( 0.08742462538030000563, 1420.450111770730018, 182.6858894113979943 ) ) ;
#13976=ORIENTED_EDGE ( 'NONE', *, *, #14442, .T. ) ;
#13977=CARTESIAN_POINT ( 'NONE',  ( -12.01638156518240130, 1440.881463477919851, 187.8051726210379968 ) ) ;
#13978=CARTESIAN_POINT ( 'NONE',  ( 13.24072114446620496, 1443.163570684924025, 187.6152391747091599 ) ) ;
#13981=DIRECTION ( 'NONE',  ( 0.03489949670246857150, 0.9993908270190969834, 0.000000000000000000 ) ) ;
#13984=CARTESIAN_POINT ( 'NONE',  ( 0.2432393513109950001, 1452.904566282009910, 152.5224177206319780 ) ) ;
#13985=CARTESIAN_POINT ( 'NONE',  ( 0.4721006504984889829, 1410.034462268999960, 269.8654312524320176 ) ) ;
#13986=ADVANCED_FACE ( 'NONE', ( #67461 ), #34389, .F. ) ;
#13988=CARTESIAN_POINT ( 'NONE',  ( 19.03616775833818409, 1456.571930367182176, 225.7629732080275176 ) ) ;
#13990=CARTESIAN_POINT ( 'NONE',  ( 0.03346608192457139336, 1410.062748283369501, 233.1925408425690875 ) ) ;
#13991=CARTESIAN_POINT ( 'NONE',  ( -13.53570968906610084, 1434.951797543509883, 148.7640763676990048 ) ) ;
#13997=CARTESIAN_POINT ( 'NONE',  ( 2.416798835000000256, 1426.601114010129777, 146.0361887655980127 ) ) ;
#13998=ORIENTED_EDGE ( 'NONE', *, *, #86486, .T. ) ;
#14000=CARTESIAN_POINT ( 'NONE',  ( 4.500000000000000000, 1439.615672362369878, 127.8666744532979891 ) ) ;
#14005=ORIENTED_EDGE ( 'NONE', *, *, #3506, .F. ) ;
#14008=CARTESIAN_POINT ( 'NONE',  ( -14.35483103309999819, 1416.837177090929799, 221.5788728750979999 ) ) ;
#14014=CARTESIAN_POINT ( 'NONE',  ( 9.464617871280001538, 1422.096644224830015, 230.5969590778979921 ) ) ;
#14017=CARTESIAN_POINT ( 'NONE',  ( 18.26532265589999682, 1415.628674266529742, 209.8910850646770143 ) ) ;
#14019=CARTESIAN_POINT ( 'NONE',  ( -0.5647852981080000445, 1422.358767625429891, 228.0117178583979864 ) ) ;
#14020=CARTESIAN_POINT ( 'NONE',  ( -25.74151704639999849, 1448.987115190519944, 137.5013012925980149 ) ) ;
#14025=CARTESIAN_POINT ( 'NONE',  ( -1.523411567629999963, 1416.219761280829971, 227.9399405097980207 ) ) ;
#14027=CARTESIAN_POINT ( 'NONE',  ( -13.49752382283059937, 1408.354313590640004, 207.9364978486700295 ) ) ;
#14028=CARTESIAN_POINT ( 'NONE',  ( -14.59411311879999928, 1414.913060387329779, 201.4749348725179914 ) ) ;
#14030=CARTESIAN_POINT ( 'NONE',  ( 13.80526003289999970, 1434.979593547039940, 149.1900205729979803 ) ) ;
#14031=CARTESIAN_POINT ( 'NONE',  ( -26.81574567050000013, 1435.910853872800089, 136.5210682332980241 ) ) ;
#14041=CARTESIAN_POINT ( 'NONE',  ( 31.03490941718551710, 1415.854366402851610, 269.3355724915077190 ) ) ;
#14043=CARTESIAN_POINT ( 'NONE',  ( -20.01067139950000140, 1507.877425041529932, 188.9709217985979706 ) ) ;
#14044=CARTESIAN_POINT ( 'NONE',  ( 21.39771952614790251, 1509.704955107219803, 188.4542851670070149 ) ) ;
#14045=CARTESIAN_POINT ( 'NONE',  ( 3.421433458210000111, 1428.746990730030120, 185.0224803175979957 ) ) ;
#14050=CARTESIAN_POINT ( 'NONE',  ( -29.15335221010520073, 1509.735908701399921, 208.6618227458789931 ) ) ;
#14051=CARTESIAN_POINT ( 'NONE',  ( -16.03581849651680002, 1409.473033727780148, 225.1836456777660089 ) ) ;
#14058=CARTESIAN_POINT ( 'NONE',  ( 2.446787376320000096, 1432.353341358199941, 150.2884730787980061 ) ) ;
#14060=CARTESIAN_POINT ( 'NONE',  ( -0.07455736060109920127, 1420.122296152110039, 183.7971148460100039 ) ) ;
#14061=CARTESIAN_POINT ( 'NONE',  ( 1.600823151459999982, 1464.924551132029819, 236.5189088668979878 ) ) ;
#14062=CARTESIAN_POINT ( 'NONE',  ( 22.37934482829999894, 1410.615956673830169, 215.1176883408980132 ) ) ;
#14063=CARTESIAN_POINT ( 'NONE',  ( -1.801360752315949831, 1412.633430038469896, 185.9483006541370003 ) ) ;
#14065=CARTESIAN_POINT ( 'NONE',  ( -17.58613261789999882, 1424.135132543530062, 227.0015458978980121 ) ) ;
#14066=DIRECTION ( 'NONE',  ( -9.520246157234046601E-08, 3.411689477181459810E-09, 0.9999999999999954481 ) ) ;
#14068=CARTESIAN_POINT ( 'NONE',  ( 25.80251995263579801, 1449.911705404210124, 208.7286070993190208 ) ) ;
#14074=AXIS2_PLACEMENT_3D ( 'NONE', #80508, #36840, #11640 ) ;
#14075=CARTESIAN_POINT ( 'NONE',  ( -17.67465541829999864, 1423.538376080030048, 226.2965632852980207 ) ) ;
#14077=CARTESIAN_POINT ( 'NONE',  ( 14.57021081669999951, 1474.586296236829867, 224.5225414627979887 ) ) ;
#14078=CARTESIAN_POINT ( 'NONE',  ( -4.221396571449520074, 1441.605459665790022, 169.0259831405610100 ) ) ;
#14084=CARTESIAN_POINT ( 'NONE',  ( 4.084250103052634806, 1507.178795293708163, 181.6747635981337510 ) ) ;
#14086=CARTESIAN_POINT ( 'NONE',  ( -11.64111738558995235, 1425.862200434439728, 144.4792545450150385 ) ) ;
#14087=CARTESIAN_POINT ( 'NONE',  ( 15.76856008000959974, 1410.855127137190038, 191.5168014226029811 ) ) ;
#14095=CARTESIAN_POINT ( 'NONE',  ( 35.14989576411770145, 1451.591923343930148, 134.0999999983660018 ) ) ;
#14096=CARTESIAN_POINT ( 'NONE',  ( -40.23150629975690151, 1442.858491698010084, 137.0288987757270149 ) ) ;
#14101=CARTESIAN_POINT ( 'NONE',  ( 15.03292567439081040, 1410.810032661595415, 227.4772455420474842 ) ) ;
#14103=CARTESIAN_POINT ( 'NONE',  ( -0.01304308391829999900, 1452.999749671330164, 183.2385070535979708 ) ) ;
#14104=CARTESIAN_POINT ( 'NONE',  ( -3.151745281339999760, 1484.261526075930078, 183.3481135453979789 ) ) ;
#14105=CARTESIAN_POINT ( 'NONE',  ( -2.500000000000000000, 1439.579545607999989, 165.8618564662860138 ) ) ;
#14107=CARTESIAN_POINT ( 'NONE',  ( -41.48252422893380498, 1444.135613197089924, 136.5500652606600056 ) ) ;
#14110=CARTESIAN_POINT ( 'NONE',  ( -9856.831406432045696, 2833.746317950422963, 1378.242121024269181 ) ) ;
#14112=FACE_OUTER_BOUND ( 'NONE', #90102, .T. ) ;
#14118=CARTESIAN_POINT ( 'NONE',  ( 38.27236334520110006, 1440.913060387330006, 265.3011690063839865 ) ) ;
#14120=CARTESIAN_POINT ( 'NONE',  ( -0.0002251272801281111791, 1452.162349662644374, 153.8758817369695464 ) ) ;
#14123=CARTESIAN_POINT ( 'NONE',  ( -0.1792353353211550149, 1451.688816654250104, 183.0380716929619780 ) ) ;
#14124=CARTESIAN_POINT ( 'NONE',  ( -16.66095200220000194, 1410.867389019930215, 191.7375190235979971 ) ) ;
#14127=CARTESIAN_POINT ( 'NONE',  ( -13.11134949370000058, 1419.893956787529987, 222.0035429825979918 ) ) ;
#14128=CARTESIAN_POINT ( 'NONE',  ( -20.17495577355367686, 1508.361608974187902, 228.9114165637121232 ) ) ;
#14129=CARTESIAN_POINT ( 'NONE',  ( -1.469541472189999975, 1508.190586172730036, 180.6206999101979989 ) ) ;
#14132=CARTESIAN_POINT ( 'NONE',  ( 15.64891445259999969, 1459.656115944430212, 231.4809545682979888 ) ) ;
#14133=FACE_OUTER_BOUND ( 'NONE', #71585, .T. ) ;
#14139=CIRCLE ( 'NONE', #76730, 26.43993992909998525 ) ;
#14141=CARTESIAN_POINT ( 'NONE',  ( -0.1362281291136649974, 1507.781361289090000, 180.7563895008119914 ) ) ;
#14146=EDGE_CURVE ( 'NONE', #64548, #98856, #1462, .T. ) ;
#14147=CARTESIAN_POINT ( 'NONE',  ( 4.283856666023710069, 1440.956247486469920, 155.9231014612180104 ) ) ;
#14151=B_SPLINE_CURVE_WITH_KNOTS ( 'NONE', 5,
 ( #51995, #86136, #104037, #93973, #1599, #35736 ),
 .UNSPECIFIED., .F., .F.,
 ( 6, 6 ),
 ( -14.36013212639999992, -6.500205904970000503 ),
 .UNSPECIFIED. ) ;
#14152=CARTESIAN_POINT ( 'NONE',  ( 7.894399719279999950, 1460.747930716730025, 221.5712129898979867 ) ) ;
#14153=CARTESIAN_POINT ( 'NONE',  ( -11.27444857399999911, 1430.307468795130035, 151.2292110278980033 ) ) ;
#14156=CARTESIAN_POINT ( 'NONE',  ( 6.384249653904870314, 1425.832381260119973, 153.2928915029530117 ) ) ;
#14157=CARTESIAN_POINT ( 'NONE',  ( -21.25167763996070036, 1489.809143648679992, 209.5009534265659852 ) ) ;
#14158=CARTESIAN_POINT ( 'NONE',  ( 12.50628814030000058, 1446.659047563680133, 188.2618572318980057 ) ) ;
#14159=CARTESIAN_POINT ( 'NONE',  ( -24.63752222140000114, 1457.439077831530085, 211.8173745106979879 ) ) ;
#14161=CARTESIAN_POINT ( 'NONE',  ( -1.518145821790000127, 1484.332293859730044, 182.5346457296979850 ) ) ;
#14165=CARTESIAN_POINT ( 'NONE',  ( 6.208817084409999687, 1406.025614260530119, 267.8376454021980066 ) ) ;
#14166=CARTESIAN_POINT ( 'NONE',  ( 0.4274135159440000109, 1409.096031525230046, 185.6227926432979984 ) ) ;
#14167=CARTESIAN_POINT ( 'NONE',  ( 18.09099147780000294, 1410.879528734529913, 193.6270419906979896 ) ) ;
#14168=CARTESIAN_POINT ( 'NONE',  ( 22.92656223559736262, 1432.082429570070190, 216.2522404191055614 ) ) ;
#14170=CARTESIAN_POINT ( 'NONE',  ( -1.466750842539999988, 1450.866641565780128, 183.4132864747979852 ) ) ;
#14172=CARTESIAN_POINT ( 'NONE',  ( -2.500094832422949942, 1448.919094719029999, 155.0643300295350002 ) ) ;
#14173=CARTESIAN_POINT ( 'NONE',  ( -1.635975655120868177, 1451.617099953195975, 184.0322519377451727 ) ) ;
#14174=CARTESIAN_POINT ( 'NONE',  ( 0.5697989934050000649, 1450.893162568020216, 155.6080914337979948 ) ) ;
#14175=CARTESIAN_POINT ( 'NONE',  ( -14.45145579027879990, 1416.702560754940123, 221.3854044765280094 ) ) ;
#14177=CARTESIAN_POINT ( 'NONE',  ( -1.221245327089999926E-15, 1427.913060387330006, 209.1218459616979999 ) ) ;
#14178=CARTESIAN_POINT ( 'NONE',  ( -27.01737277763200140, 1507.999902240279880, 211.4327103027169983 ) ) ;
#14179=B_SPLINE_CURVE_WITH_KNOTS ( 'NONE', 3,
 ( #87742, #11020, #62566, #65297 ),
 .UNSPECIFIED., .F., .F.,
 ( 4, 4 ),
 ( 7.312299096839999457, 15.60583060000000089 ),
 .UNSPECIFIED. ) ;
#14180=CARTESIAN_POINT ( 'NONE',  ( 3.137342596209999890, 1440.799554483159909, 158.1457359887980090 ) ) ;
#14181=CARTESIAN_POINT ( 'NONE',  ( -4.953282586809999444, 1475.369567567530112, 269.2856847212980256 ) ) ;
#14182=CARTESIAN_POINT ( 'NONE',  ( -10.86003582634030806, 1424.791813296290229, 138.1872773544496624 ) ) ;
#14184=CARTESIAN_POINT ( 'NONE',  ( 17.71073067720600136, 1414.282064044829895, 224.0326197095010059 ) ) ;
#14192=CARTESIAN_POINT ( 'NONE',  ( -21.90047919039999869, 1409.842284365829983, 203.3532602289579927 ) ) ;
#14194=CARTESIAN_POINT ( 'NONE',  ( -42.76956658369999786, 1430.336806088530011, 269.7319452664979735 ) ) ;
#14197=CARTESIAN_POINT ( 'NONE',  ( -4.294703086410359916, 1410.439188197537533, 232.1146548671422067 ) ) ;
#14201=CARTESIAN_POINT ( 'NONE',  ( 11.15477939360000015, 1425.160653555029967, 144.1599692641979971 ) ) ;
#14206=CARTESIAN_POINT ( 'NONE',  ( 28.03239352649999816, 1444.711964598699979, 137.4439080250980112 ) ) ;
#14209=DIRECTION ( 'NONE',  ( -1.000000000000000000, 0.000000000000000000, -1.989566177384290042E-13 ) ) ;
#14214=CARTESIAN_POINT ( 'NONE',  ( 20.46625007539810071, 1507.818601948450123, 228.4183590306939777 ) ) ;
#14217=ORIENTED_EDGE ( 'NONE', *, *, #26901, .T. ) ;
#14218=CARTESIAN_POINT ( 'NONE',  ( -11.92220220670000153, 1397.363550527129746, 203.3627882915380098 ) ) ;
#14219=CARTESIAN_POINT ( 'NONE',  ( -20.26547961730000225, 1410.542145032029794, 220.2212046400979943 ) ) ;
#14221=CARTESIAN_POINT ( 'NONE',  ( -12.70095137425357379, 1445.015557356070303, 169.4597653655617648 ) ) ;
#14225=CARTESIAN_POINT ( 'NONE',  ( -1.362564840747860107, 1414.935332577269946, 185.4090015132200051 ) ) ;
#14226=CARTESIAN_POINT ( 'NONE',  ( 3.798727053469999504, 1410.301227430230028, 185.9690677660979645 ) ) ;
#14227=CARTESIAN_POINT ( 'NONE',  ( -7.752197826429999772, 1416.823872462129884, 192.4769319036979880 ) ) ;
#14229=CARTESIAN_POINT ( 'NONE',  ( 10.95806849906840164, 1396.295724571469918, 207.5366794976360154 ) ) ;
#14230=CARTESIAN_POINT ( 'NONE',  ( 1.555569193349999990, 1415.296882296330068, 191.0414296403980075 ) ) ;
#14231=CARTESIAN_POINT ( 'NONE',  ( 10.93289368750000001, 1429.709397299530110, 151.3050649637980030 ) ) ;
#14233=ORIENTED_EDGE ( 'NONE', *, *, #96652, .F. ) ;
#14234=CARTESIAN_POINT ( 'NONE',  ( 13.34701713054489858, 1434.912624059160180, 148.9125970433090060 ) ) ;
#14238=DIRECTION ( 'NONE',  ( -0.7020890432300541661, 0.02451748950546728256, -0.7116669643060977712 ) ) ;
#14239=CARTESIAN_POINT ( 'NONE',  ( -13.76044198839999844, 1462.505312967929967, 230.0314476057980073 ) ) ;
#14240=AXIS2_PLACEMENT_3D ( 'NONE', #97532, #73991, #89129 ) ;
#14247=CARTESIAN_POINT ( 'NONE',  ( -11.73541398288529969, 1509.403454113690032, 181.4876751329869933 ) ) ;
#14254=CARTESIAN_POINT ( 'NONE',  ( -20.28559706309999910, 1508.605287556030135, 228.9894631997980241 ) ) ;
#14256=CARTESIAN_POINT ( 'NONE',  ( -5.503799114343967958, 1410.587718136319836, 269.3375590789236753 ) ) ;
#14257=CARTESIAN_POINT ( 'NONE',  ( -0.5979851740210000433, 1408.933942489730043, 231.6757385099979842 ) ) ;
#14258=CARTESIAN_POINT ( 'NONE',  ( -7.713339349770000020, 1475.513060387329915, 189.5179100386980053 ) ) ;
#14260=CARTESIAN_POINT ( 'NONE',  ( 2.500000000000000000, 1432.255994091859975, 157.4927853088979930 ) ) ;
#14261=CARTESIAN_POINT ( 'NONE',  ( -34.53043532563810203, 1440.913060389100110, 249.9798763198099891 ) ) ;
#14264=CARTESIAN_POINT ( 'NONE',  ( 13.52613638629999926, 1409.420097905330067, 270.2585879650980019 ) ) ;
#14266=CARTESIAN_POINT ( 'NONE',  ( 22.70509154759999859, 1409.705932507530179, 209.2982499274170323 ) ) ;
#14267=CARTESIAN_POINT ( 'NONE',  ( -20.27305603270000134, 1508.384852854430164, 189.2299609745979865 ) ) ;
#14271=CARTESIAN_POINT ( 'NONE',  ( 4.172462890132850433, 1421.447587853880123, 185.0121838783159944 ) ) ;
#14272=CARTESIAN_POINT ( 'NONE',  ( 0.4435038406939999511, 1418.672163285830038, 184.7048927289980043 ) ) ;
#14273=CARTESIAN_POINT ( 'NONE',  ( 10.98083629090000102, 1433.016921068679949, 151.7694307944979926 ) ) ;
#14277=CARTESIAN_POINT ( 'NONE',  ( 18.95839814150000180, 1416.827520077830059, 210.4638737380680027 ) ) ;
#14280=CARTESIAN_POINT ( 'NONE',  ( -1.347852712580000167, 1417.336052002229962, 235.7060345899980121 ) ) ;
#14282=CARTESIAN_POINT ( 'NONE',  ( -5.386815040730001058, 1432.449270638659982, 154.6099187821979797 ) ) ;
#14287=CARTESIAN_POINT ( 'NONE',  ( -25.76861165497327022, 1450.790415003483076, 136.9094829965818292 ) ) ;
#14291=CARTESIAN_POINT ( 'NONE',  ( -13.58235846979999906, 1416.828040475229955, 221.9087530951979659 ) ) ;
#14294=CARTESIAN_POINT ( 'NONE',  ( 1.600048698852036821, 1401.254281879943164, 135.5999999980979851 ) ) ;
#14295=CARTESIAN_POINT ( 'NONE',  ( 24.32016871089999910, 1444.936401044380091, 214.5085396922679877 ) ) ;
#14299=CARTESIAN_POINT ( 'NONE',  ( 15.61977316628497015, 1421.021825222467442, 227.6337086628678037 ) ) ;
#14301=CARTESIAN_POINT ( 'NONE',  ( -19.72693241579999679, 1426.900081331430101, 224.3685230545979721 ) ) ;
#14305=CARTESIAN_POINT ( 'NONE',  ( 0.2758982302775880302, 1410.303294781930163, 233.2202553833849663 ) ) ;
#14306=CARTESIAN_POINT ( 'NONE',  ( -29.82212560978975802, 1462.379445244557701, 269.4689213073284577 ) ) ;
#14308=CARTESIAN_POINT ( 'NONE',  ( -5.642160312090365615, 1406.970328519305667, 269.6422777563649333 ) ) ;
#14312=CARTESIAN_POINT ( 'NONE',  ( -0.2068382967480000001, 1416.433929650830123, 233.7159416108979997 ) ) ;
#14313=CARTESIAN_POINT ( 'NONE',  ( -13.11599568954357942, 1444.787961940224932, 186.4523988439049731 ) ) ;
#14315=CARTESIAN_POINT ( 'NONE',  ( 12.53380499169999851, 1442.773887286369927, 169.4755105685979970 ) ) ;
#14320=CARTESIAN_POINT ( 'NONE',  ( 24.97897394130000137, 1436.441733159510022, 137.9167456186980019 ) ) ;
#14322=DIRECTION ( 'NONE',  ( 0.000000000000000000, 0.000000000000000000, -1.000000000000000000 ) ) ;
#14323=ORIENTED_EDGE ( 'NONE', *, *, #72941, .F. ) ;
#14329=CARTESIAN_POINT ( 'NONE',  ( 18.16418870590809931, 1416.835419214280137, 209.1673351295509917 ) ) ;
#14331=CARTESIAN_POINT ( 'NONE',  ( 41.80252838952070249, 1437.000150592197542, 269.6437000537932818 ) ) ;
#14332=CARTESIAN_POINT ( 'NONE',  ( -9.325404508809999271, 1464.388849669230012, 238.2842606474980016 ) ) ;
#14333=CARTESIAN_POINT ( 'NONE',  ( -19.81987573899999688, 1494.487655362629766, 189.5802261639979918 ) ) ;
#14334=CARTESIAN_POINT ( 'NONE',  ( -11.74619720679999979, 1433.378107375729996, 150.8204405054979986 ) ) ;
#14337=CARTESIAN_POINT ( 'NONE',  ( -27.30723893600000096, 1439.410402289340254, 137.0765984299980005 ) ) ;
#14338=CARTESIAN_POINT ( 'NONE',  ( -12.78690713350000152, 1416.828040475229955, 195.5394874918979724 ) ) ;
#14339=DIRECTION ( 'NONE',  ( 0.000000000000000000, 1.000000000000000000, 0.000000000000000000 ) ) ;
#14340=CARTESIAN_POINT ( 'NONE',  ( -2.923263464371510079, 1409.521016840560151, 186.8216758237240072 ) ) ;
#14342=CARTESIAN_POINT ( 'NONE',  ( -11.06185805447235104, 1509.424462684860146, 237.0079586032242389 ) ) ;
#14343=CARTESIAN_POINT ( 'NONE',  ( 8.404157474328759975E-09, 1409.508817234440130, 259.7239082992959993 ) ) ;
#14345=ORIENTED_EDGE ( 'NONE', *, *, #92728, .T. ) ;
#14346=CARTESIAN_POINT ( 'NONE',  ( -11.85807509641779944, 1431.776270381120185, 149.9536850627220019 ) ) ;
#14348=CARTESIAN_POINT ( 'NONE',  ( -7.287608047049999982, 1471.338968442629948, 269.8696687364979994 ) ) ;
#14350=CARTESIAN_POINT ( 'NONE',  ( -1.110223024630000146E-16, 1433.447556881219953, 155.4376913957980264 ) ) ;
#14351=CARTESIAN_POINT ( 'NONE',  ( 34.59019106360999984, 1451.551308700359868, 135.5662212263999891 ) ) ;
#14358=CARTESIAN_POINT ( 'NONE',  ( -37.25277800141729756, 1420.473031640739919, 269.0086013173549873 ) ) ;
#14361=ORIENTED_EDGE ( 'NONE', *, *, #40545, .T. ) ;
#14364=CARTESIAN_POINT ( 'NONE',  ( -2.500000000000000000, 1428.666845053830002, 184.0221679455979995 ) ) ;
#14367=CARTESIAN_POINT ( 'NONE',  ( -14.25300571640000058, 1440.433557114710084, 188.8957244713979833 ) ) ;
#14369=CARTESIAN_POINT ( 'NONE',  ( -2.310656430857296328, 1449.746119739275400, 182.9714966330411698 ) ) ;
#14371=CARTESIAN_POINT ( 'NONE',  ( -26.37348269860000016, 1435.500559562420221, 135.8355299040979958 ) ) ;
#14375=DIRECTION ( 'NONE',  ( 0.000000000000000000, -1.000000000000000000, 0.000000000000000000 ) ) ;
#14377=CARTESIAN_POINT ( 'NONE',  ( 0.02192820754129999605, 1407.539782043129890, 196.0601747759980071 ) ) ;
#14379=DIRECTION ( 'NONE',  ( 0.4794255386041986200, 0.000000000000000000, 0.8775825618903752012 ) ) ;
#14382=ORIENTED_EDGE ( 'NONE', *, *, #25710, .T. ) ;
#14383=CARTESIAN_POINT ( 'NONE',  ( 0.2568979742649999398, 1452.981230334829888, 183.2590030997980080 ) ) ;
#14385=CARTESIAN_POINT ( 'NONE',  ( -14.59279134157089963, 1436.244781760590058, 149.8708244536879874 ) ) ;
#14387=CARTESIAN_POINT ( 'NONE',  ( -0.8179048554660000026, 1485.520952860329999, 181.9073606171980089 ) ) ;
#14390=CARTESIAN_POINT ( 'NONE',  ( 5.519893427111519202, 1440.499866072189889, 154.7645221071819890 ) ) ;
#14392=CARTESIAN_POINT ( 'NONE',  ( -3.887243918150000104E-16, 1418.913060387330006, 172.2701767054979882 ) ) ;
#14395=ORIENTED_EDGE ( 'NONE', *, *, #46699, .F. ) ;
#14396=CARTESIAN_POINT ( 'NONE',  ( -33.91369114127179785, 1435.681798693280143, 134.7398496782940072 ) ) ;
#14398=CARTESIAN_POINT ( 'NONE',  ( -24.02428866992241652, 1445.062781591384919, 212.2832923785209118 ) ) ;
#14399=ORIENTED_EDGE ( 'NONE', *, *, #83173, .T. ) ;
#14402=CARTESIAN_POINT ( 'NONE',  ( 12.83022075569469855, 1434.689919048429829, 149.3777740995939780 ) ) ;
#14403=CARTESIAN_POINT ( 'NONE',  ( 13.40958059889999987, 1414.996444526030018, 197.9133051477979848 ) ) ;
#14405=DIRECTION ( 'NONE',  ( -0.7067699325516847431, 0.03085807370037648573, 0.7067701477343176775 ) ) ;
#14409=CARTESIAN_POINT ( 'NONE',  ( 4.243484587782480055, 1441.412175538559950, 162.2162703121909999 ) ) ;
#14411=CARTESIAN_POINT ( 'NONE',  ( -15.73573827020000060, 1409.462564476230000, 225.2909780739980192 ) ) ;
#14417=CARTESIAN_POINT ( 'NONE',  ( -18.10358820054819873, 1416.830086716310007, 209.2067746984330086 ) ) ;
#14420=CARTESIAN_POINT ( 'NONE',  ( -0.04582397527460040088, 1508.911460179130017, 179.8421084519130204 ) ) ;
#14421=CARTESIAN_POINT ( 'NONE',  ( 11.60004869885203682, 1426.172749320205185, 138.0249698027471936 ) ) ;
#14422=CARTESIAN_POINT ( 'NONE',  ( -2.500000000000000000, 1419.382898089430000, 144.1038810569979773 ) ) ;
#14424=CARTESIAN_POINT ( 'NONE',  ( -3.527889728650740089E-07, 1407.083036151889928, 222.1289087389290273 ) ) ;
#14426=CARTESIAN_POINT ( 'NONE',  ( 28.28124823237279983, 1440.913060387279984, 232.2763879390959971 ) ) ;
#14430=ORIENTED_EDGE ( 'NONE', *, *, #3607, .T. ) ;
#14433=CARTESIAN_POINT ( 'NONE',  ( -47.22427986889969276, 1578.884133025160281, 191.3316845414530007 ) ) ;
#14436=CARTESIAN_POINT ( 'NONE',  ( 2.087781202739551034, 1508.813655593662361, 237.6275677725071773 ) ) ;
#14439=CARTESIAN_POINT ( 'NONE',  ( 0.000000000000000000, 1441.261220175949802, 126.8032249175980155 ) ) ;
#14442=EDGE_CURVE ( 'NONE', #11383, #24304, #33558, .T. ) ;
#14444=B_SPLINE_CURVE_WITH_KNOTS ( 'NONE', 5,
 ( #100965, #57360, #65744, #92032, #92570, #59000, #99307, #66856, #74149 ),
 .UNSPECIFIED., .F., .F.,
 ( 6, 3, 6 ),
 ( 0.000000000000000000, 0.5050532947838839437, 1.000000000000000000 ),
 .UNSPECIFIED. ) ;
#14446=CARTESIAN_POINT ( 'NONE',  ( -15.13403568919999920, 1507.625766668030110, 191.8456552481979998 ) ) ;
#14449=AXIS2_PLACEMENT_3D ( 'NONE', #41685, #68562, #33271 ) ;
#14450=EDGE_CURVE ( 'NONE', #52333, #69312, #68198, .T. ) ;
#14457=ORIENTED_EDGE ( 'NONE', *, *, #76813, .F. ) ;
#14458=EDGE_LOOP ( 'NONE', ( #57796, #95237, #45423, #19049 ) ) ;
#14462=CARTESIAN_POINT ( 'NONE',  ( -0.5623044073341159077, 1416.835806620478706, 227.7680351671496624 ) ) ;
#14464=EDGE_CURVE ( 'NONE', #31461, #79161, #63821, .T. ) ;
#14468=CARTESIAN_POINT ( 'NONE',  ( -22.52564151159999639, 1509.699673122230024, 190.3321270482979912 ) ) ;
#14469=CARTESIAN_POINT ( 'NONE',  ( 0.6562332730204689657, 1408.935976558159837, 194.1358227214440149 ) ) ;
#14470=CARTESIAN_POINT ( 'NONE',  ( 18.28844460585999698, 1425.323495367109899, 225.4768200461419951 ) ) ;
#14473=CARTESIAN_POINT ( 'NONE',  ( 11.86584296470000055, 1432.318021067500013, 149.9824182361979865 ) ) ;
#14474=CARTESIAN_POINT ( 'NONE',  ( -4.162009348731279701, 1449.631390586350108, 185.0510865354499970 ) ) ;
#14478=CARTESIAN_POINT ( 'NONE',  ( 19.75053106571979811, 1455.500286668259832, 226.5546858144080318 ) ) ;
#14479=CARTESIAN_POINT ( 'NONE',  ( 14.06572279189999897, 1410.763503171529919, 191.2785366137979963 ) ) ;
#14486=CARTESIAN_POINT ( 'NONE',  ( -1.211166369079999861, 1482.210497797730113, 182.3203058735979880 ) ) ;
#14488=CARTESIAN_POINT ( 'NONE',  ( -45.63009907890679528, 1440.261568459579848, 268.9750367124860304 ) ) ;
#14489=CARTESIAN_POINT ( 'NONE',  ( -20.64235243649999774, 1507.778435260330070, 191.4718973457979985 ) ) ;
#14490=EDGE_CURVE ( 'NONE', #87520, #16155, #52247, .T. ) ;
#14492=CARTESIAN_POINT ( 'NONE',  ( 6.294750265487480512, 1408.079328831549901, 220.7028845641339672 ) ) ;
#14497=ADVANCED_FACE ( 'NONE', ( #85751 ), #787, .T. ) ;
#14498=EDGE_LOOP ( 'NONE', ( #14430, #92431, #53703, #36932 ) ) ;
#14499=CARTESIAN_POINT ( 'NONE',  ( 22.11712025709999807, 1419.857860618529912, 248.4077083947979929 ) ) ;
#14500=CARTESIAN_POINT ( 'NONE',  ( -28.00748489060000068, 1508.132844953629956, 207.4252966237179976 ) ) ;
#14501=CARTESIAN_POINT ( 'NONE',  ( 0.4750796042289999743, 1494.209875447929790, 181.4895372315980069 ) ) ;
#14504=CARTESIAN_POINT ( 'NONE',  ( -25.73196798229999871, 1439.230040327810002, 220.8240077837979811 ) ) ;
#14505=FACE_OUTER_BOUND ( 'NONE', #31759, .T. ) ;
#14506=CARTESIAN_POINT ( 'NONE',  ( -19.88783023904650094, 1452.218562051830304, 143.3852592352909880 ) ) ;
#14507=CARTESIAN_POINT ( 'NONE',  ( 29.25355977910000149, 1451.030362765829977, 136.3073753608980212 ) ) ;
#14511=CARTESIAN_POINT ( 'NONE',  ( 15.74706555227250249, 1422.765470877109919, 229.4186969687229976 ) ) ;
#14514=ORIENTED_EDGE ( 'NONE', *, *, #31026, .T. ) ;
#14516=CARTESIAN_POINT ( 'NONE',  ( -24.11339479709999978, 1410.986675406829818, 209.4109128042719874 ) ) ;
#14521=CARTESIAN_POINT ( 'NONE',  ( -16.93884296450000093, 1507.634939588830093, 230.1482605005980133 ) ) ;
#14524=CARTESIAN_POINT ( 'NONE',  ( 43.30895383271469967, 1452.717412850039864, 266.4924207902549824 ) ) ;
#14525=CARTESIAN_POINT ( 'NONE',  ( -0.9591896699583389863, 1424.151861139469929, 228.3373416235070010 ) ) ;
#14531=CARTESIAN_POINT ( 'NONE',  ( -7.228663065755877248, 1519.913060387329779, 183.1074954935087646 ) ) ;
#14533=CARTESIAN_POINT ( 'NONE',  ( 12.92590733569883810, 1442.905621755283619, 187.0717105805051119 ) ) ;
#14544=CARTESIAN_POINT ( 'NONE',  ( 0.000000000000000000, 1440.913060387330006, 134.0999999980979851 ) ) ;
#14545=CARTESIAN_POINT ( 'NONE',  ( -16.73048837315040061, 1413.002407920880160, 191.6778219149559845 ) ) ;
#14546=DIRECTION ( 'NONE',  ( 0.03206686913393481247, -0.9990097415445143847, -0.03084237674223211378 ) ) ;
#14548=EDGE_CURVE ( 'NONE', #72755, #24414, #54393, .T. ) ;
#14550=CARTESIAN_POINT ( 'NONE',  ( -25.71573637233310095, 1509.811073689510067, 223.1001859706680079 ) ) ;
#14551=CARTESIAN_POINT ( 'NONE',  ( 11.81707110430000007, 1430.266231075130008, 147.2485970657980090 ) ) ;
#14552=ORIENTED_EDGE ( 'NONE', *, *, #4232, .F. ) ;
#14553=CARTESIAN_POINT ( 'NONE',  ( -0.1681681984989999989, 1420.473120458229914, 179.3023655596979893 ) ) ;
#14557=CARTESIAN_POINT ( 'NONE',  ( 2.382436964801011303, 1426.901689560120076, 137.0999999980980135 ) ) ;
#14561=CARTESIAN_POINT ( 'NONE',  ( -1.657615632539999773, 1440.444625599219989, 150.6406752848980091 ) ) ;
#14563=CARTESIAN_POINT ( 'NONE',  ( -14.00875083269999877, 1416.819760292330102, 221.8514977783980271 ) ) ;
#14564=CARTESIAN_POINT ( 'NONE',  ( 11.53532962319999911, 1433.771858699349877, 151.2647645120979973 ) ) ;
#14566=CARTESIAN_POINT ( 'NONE',  ( 0.6359931820546259607, 1450.890027228909958, 181.3124269289969845 ) ) ;
#14569=CARTESIAN_POINT ( 'NONE',  ( 11.76598840989999850, 1428.979790717830156, 145.3128034382980047 ) ) ;
#14571=CARTESIAN_POINT ( 'NONE',  ( 12.64400598149999944, 1419.760550675029890, 229.1492764728980092 ) ) ;
#14573=CARTESIAN_POINT ( 'NONE',  ( 8.623178418239669796, 1441.178012935769857, 153.8582158081470084 ) ) ;
#14574=CARTESIAN_POINT ( 'NONE',  ( -17.56312616970000207, 1409.691384886529931, 224.4360229823980148 ) ) ;
#14576=CARTESIAN_POINT ( 'NONE',  ( -0.7149693253490000400, 1422.352078937030001, 228.1616098511979942 ) ) ;
#14577=CARTESIAN_POINT ( 'NONE',  ( -25.87590796830000173, 1449.884901504650088, 136.9990172420979775 ) ) ;
#14579=CARTESIAN_POINT ( 'NONE',  ( 12.78701137800000076, 1416.830001031129996, 222.9175051919979751 ) ) ;
#14581=EDGE_CURVE ( 'NONE', #94751, #25667, #106950, .T. ) ;
#14583=CARTESIAN_POINT ( 'NONE',  ( -3.346430209710000270, 1414.913060387329779, 225.7371794378979928 ) ) ;
#14584=CARTESIAN_POINT ( 'NONE',  ( 0.2075961268654689940, 1458.701262879619890, 183.0088039633720030 ) ) ;
#14585=CARTESIAN_POINT ( 'NONE',  ( -5.629143959155359589, 1407.138657505239962, 221.3608015446720003 ) ) ;
#14586=EDGE_LOOP ( 'NONE', ( #51294, #61822, #95993, #26911 ) ) ;
#14587=CARTESIAN_POINT ( 'NONE',  ( -0.3973340087122340103, 1418.672806152889962, 184.7148007238050127 ) ) ;
#14588=ADVANCED_FACE ( 'NONE', ( #108056 ), #6150, .T. ) ;
#14589=CARTESIAN_POINT ( 'NONE',  ( -27.78452750130110260, 1508.000976266860107, 210.4681927182890036 ) ) ;
#14590=CARTESIAN_POINT ( 'NONE',  ( 11.87926624510000018, 1433.311557364369946, 149.0256386714980010 ) ) ;
#14596=CARTESIAN_POINT ( 'NONE',  ( 26.78807150899999812, 1436.761941354120154, 136.7824147662979897 ) ) ;
#14598=CARTESIAN_POINT ( 'NONE',  ( -0.3328314641405109575, 1452.976685807730291, 183.2631399573310205 ) ) ;
#14600=CARTESIAN_POINT ( 'NONE',  ( 14.96949722733650034, 1508.714436942260136, 232.5787688410800058 ) ) ;
#14601=CARTESIAN_POINT ( 'NONE',  ( 29.75796374405569367, 1414.999058895863755, 269.3609185650325912 ) ) ;
#14602=CARTESIAN_POINT ( 'NONE',  ( 21.99073835760000151, 1489.474306034229812, 209.8571700393559922 ) ) ;
#14604=CARTESIAN_POINT ( 'NONE',  ( 2.500000004270000353, 1431.428399487389925, 183.6496936308980139 ) ) ;
#14610=CARTESIAN_POINT ( 'NONE',  ( -27.26775544359999870, 1450.672803855060010, 136.4409915286979924 ) ) ;
#14611=ADVANCED_FACE ( 'NONE', ( #39766 ), #73926, .F. ) ;
#14612=EDGE_CURVE ( 'NONE', #55821, #101169, #98554, .T. ) ;
#14613=CARTESIAN_POINT ( 'NONE',  ( -16.62210571749790233, 1410.725220498880162, 226.5039651633489939 ) ) ;
#14615=ORIENTED_EDGE ( 'NONE', *, *, #7519, .F. ) ;
#14616=CARTESIAN_POINT ( 'NONE',  ( -12.17829449539999942, 1509.277426923929852, 182.3210652022980014 ) ) ;
#14618=CARTESIAN_POINT ( 'NONE',  ( 21.23228481039999949, 1508.977225803030024, 226.2585636259979935 ) ) ;
#14621=CARTESIAN_POINT ( 'NONE',  ( 1.236506327399999883, 1466.454922307530069, 235.1997163242980093 ) ) ;
#14622=CARTESIAN_POINT ( 'NONE',  ( 20.12362348629999786, 1409.615792804430157, 216.8331973927680281 ) ) ;
#14623=CARTESIAN_POINT ( 'NONE',  ( -1.979485596885299792, 1414.929432389800013, 186.0262034026189895 ) ) ;
#14624=CARTESIAN_POINT ( 'NONE',  ( -15.98001441509999943, 1422.636699047329785, 227.8263916563979876 ) ) ;
#14627=CARTESIAN_POINT ( 'NONE',  ( 27.33115299130880160, 1488.742645355629975, 208.2830191072760044 ) ) ;
#14629=CARTESIAN_POINT ( 'NONE',  ( 22.81443202775711754, 1509.728776510858552, 190.2493757223895727 ) ) ;
#14630=CARTESIAN_POINT ( 'NONE',  ( -0.9329003126829999992, 1416.492614553930025, 233.5735679209980162 ) ) ;
#14632=AXIS2_PLACEMENT_3D ( 'NONE', #63408, #80726, #72343 ) ;
#14634=CARTESIAN_POINT ( 'NONE',  ( -18.26675480510339966, 1424.840341062940070, 227.6848255537819909 ) ) ;
#14635=ORIENTED_EDGE ( 'NONE', *, *, #90472, .T. ) ;
#14636=ADVANCED_FACE ( 'NONE', ( #65536 ), #99642, .F. ) ;
#14638=CARTESIAN_POINT ( 'NONE',  ( -4.248370253443329858, 1441.364699328089955, 161.3861545258119747 ) ) ;
#14640=ORIENTED_EDGE ( 'NONE', *, *, #107504, .F. ) ;
#14641=ORIENTED_EDGE ( 'NONE', *, *, #65688, .F. ) ;
#14646=CARTESIAN_POINT ( 'NONE',  ( -11.16292084342922486, 1425.155877134990533, 144.6903838373057454 ) ) ;
#14647=CARTESIAN_POINT ( 'NONE',  ( 15.78629296034880092, 1410.112424319529964, 191.7210461700169901 ) ) ;
#14655=CARTESIAN_POINT ( 'NONE',  ( 38.02701353894249792, 1450.427746997079794, 134.0999999984749991 ) ) ;
#14658=CARTESIAN_POINT ( 'NONE',  ( -42.06231979437640689, 1440.913089571769888, 269.6487552725350270 ) ) ;
#14660=ORIENTED_EDGE ( 'NONE', *, *, #6976, .F. ) ;
#14665=CARTESIAN_POINT ( 'NONE',  ( -2.500000000000000000, 1439.588444403090080, 166.1975935960979882 ) ) ;
#14668=CARTESIAN_POINT ( 'NONE',  ( 12.53380745427929988, 1442.773887455719887, 186.4115735415020083 ) ) ;
#14669=CARTESIAN_POINT ( 'NONE',  ( 36.37832874669670247, 1451.642701154630004, 134.4205496038819945 ) ) ;
#14671=CARTESIAN_POINT ( 'NONE',  ( 25.59635045179999580, 1439.616312306700138, 138.2644159780979862 ) ) ;
#14672=CARTESIAN_POINT ( 'NONE',  ( 5.681577933589999851, 1414.971279908829956, 193.1266172032979966 ) ) ;
#14678=VERTEX_POINT ( 'NONE', #40306 ) ;
#14679=CARTESIAN_POINT ( 'NONE',  ( 40.65972102606890104, 1440.913060387330006, 268.1254238195359676 ) ) ;
#14680=CARTESIAN_POINT ( 'NONE',  ( -0.001314202166405476846, 1451.878195095055389, 154.0173218471571488 ) ) ;
#14681=EDGE_LOOP ( 'NONE', ( #77189, #60144, #51166, #24450, #29333 ) ) ;
#14682=CARTESIAN_POINT ( 'NONE',  ( -0.2068025458765339886, 1451.165312576740007, 182.5378010495940089 ) ) ;
#14686=CARTESIAN_POINT ( 'NONE',  ( -13.25650536310000049, 1429.127351718030013, 222.3136094715979993 ) ) ;
#14687=CARTESIAN_POINT ( 'NONE',  ( 12.95816640841469969, 1435.988574857560025, 150.7628740217149925 ) ) ;
#14688=CARTESIAN_POINT ( 'NONE',  ( -0.6813215632989999548, 1508.998955527629960, 179.3434203495980057 ) ) ;
#14689=CARTESIAN_POINT ( 'NONE',  ( -13.50155420119999938, 1434.968988600790226, 146.4346116559979976 ) ) ;
#14691=CARTESIAN_POINT ( 'NONE',  ( 14.97860510539999979, 1460.097680310830128, 231.5368076450980084 ) ) ;
#14692=CARTESIAN_POINT ( 'NONE',  ( -11.60004869885203682, 1422.222932908413441, 135.5999999980978714 ) ) ;
#14694=CARTESIAN_POINT ( 'NONE',  ( 0.5133626083067620582, 1410.311097044259895, 185.0719925509139898 ) ) ;
#14696=CARTESIAN_POINT ( 'NONE',  ( -22.71973404851811651, 1409.706432500549909, 209.0865126238462892 ) ) ;
#14697=CARTESIAN_POINT ( 'NONE',  ( -0.06152828947505290663, 1508.663433079589822, 180.0530326742579916 ) ) ;
#14701=CARTESIAN_POINT ( 'NONE',  ( -11.60004869885203682, 1425.267055893744555, 138.0405467508053050 ) ) ;
#14705=CARTESIAN_POINT ( 'NONE',  ( 22.61371014190000039, 1448.753361709010051, 213.3230883210279956 ) ) ;
#14706=EDGE_CURVE ( 'NONE', #67085, #103816, #42913, .T. ) ;
#14707=CARTESIAN_POINT ( 'NONE',  ( -11.28722548159999839, 1431.252270778690217, 151.4401771847979887 ) ) ;
#14708=CARTESIAN_POINT ( 'NONE',  ( 19.09768422228310314, 1456.930751240180143, 225.1426474012400263 ) ) ;
#14710=CARTESIAN_POINT ( 'NONE',  ( 27.01916870379659841, 1450.861785352695961, 136.4169503727333392 ) ) ;
#14713=CARTESIAN_POINT ( 'NONE',  ( -20.18632372599999769, 1482.730689116930080, 226.9986024029979887 ) ) ;
#14715=CARTESIAN_POINT ( 'NONE',  ( -2.041421758439999845, 1485.165825108230138, 182.8125668122980017 ) ) ;
#14718=CARTESIAN_POINT ( 'NONE',  ( 12.63282632850000020, 1407.538329530530063, 269.2355767699979765 ) ) ;
#14719=CARTESIAN_POINT ( 'NONE',  ( 38.62985698226480480, 1443.711942198199949, 137.1840658525169943 ) ) ;
#14721=DIRECTION ( 'NONE',  ( 1.000000000000000000, 0.000000000000000000, 0.000000000000000000 ) ) ;
#14722=DIRECTION ( 'NONE',  ( 0.4794255386042028388, 0.000000000000000000, 0.8775825618903727587 ) ) ;
#14723=( BOUNDED_CURVE ( )  B_SPLINE_CURVE ( 3, ( #84201, #56808, #100453, #99885 ),
 .UNSPECIFIED., .F., .F. ) 
 B_SPLINE_CURVE_WITH_KNOTS ( ( 4, 4 ),
 ( 1.168456980160074821, 1.504276012154933673 ),
 .UNSPECIFIED. ) 
 CURVE ( )  GEOMETRIC_REPRESENTATION_ITEM ( )  RATIONAL_B_SPLINE_CURVE ( ( 1.000000000000000000, 0.9906241907223192200, 0.9906241907223192200, 1.000000000000000000 ) ) 
 REPRESENTATION_ITEM ( '' )  );
#14724=CARTESIAN_POINT ( 'NONE',  ( 11.86716023049999968, 1432.353341358199941, 147.6509521729980179 ) ) ;
#14726=CARTESIAN_POINT ( 'NONE',  ( -2.431405112757329956, 1449.537433628249801, 154.7921730761810011 ) ) ;
#14728=CARTESIAN_POINT ( 'NONE',  ( -1.620797157046767856, 1450.704051676946619, 183.2587108462243748 ) ) ;
#14730=FACE_OUTER_BOUND ( 'NONE', #103844, .T. ) ;
#14731=CARTESIAN_POINT ( 'NONE',  ( -14.45556168306239897, 1416.765224586759814, 221.3896323238510035 ) ) ;
#14732=DIRECTION ( 'NONE',  ( 0.03489949670247471936, -0.9993908270190967613, 3.814740354449985581E-14 ) ) ;
#14733=CARTESIAN_POINT ( 'NONE',  ( -3.268607721189999982, 1425.981674306129889, 219.6133833292979887 ) ) ;
#14735=ADVANCED_FACE ( 'NONE', ( #87281 ), #95682, .F. ) ;
#14736=CARTESIAN_POINT ( 'NONE',  ( 2.704768305889999613, 1440.770142154440009, 166.9241121263980006 ) ) ;
#14737=CARTESIAN_POINT ( 'NONE',  ( -1.778075049280000153, 1476.051869520629907, 267.5358627141980037 ) ) ;
#14738=CARTESIAN_POINT ( 'NONE',  ( -11.28161544973855612, 1425.477714925698820, 138.6342417071923592 ) ) ;
#14740=CARTESIAN_POINT ( 'NONE',  ( 18.05970663803819676, 1417.701653607439994, 223.4092527363580132 ) ) ;
#14743=CIRCLE ( 'NONE', #57624, 2.000000000062579275 ) ;
#14745=EDGE_CURVE ( 'NONE', #75409, #91917, #62992, .T. ) ;
#14749=CARTESIAN_POINT ( 'NONE',  ( -0.4983014274912969666, 1395.930461456620151, 220.1163257280059895 ) ) ;
#14751=CARTESIAN_POINT ( 'NONE',  ( -43.43972853289999847, 1430.028892233129909, 269.0356351862979523 ) ) ;
#14755=CARTESIAN_POINT ( 'NONE',  ( -0.7913646410377903617, 1426.918876941764893, 134.0999999980979851 ) ) ;
#14756=CARTESIAN_POINT ( 'NONE',  ( 11.57203810419999890, 1425.906236901130114, 139.6353521643979718 ) ) ;
#14759=DIRECTION ( 'NONE',  ( 0.000000000000000000, 1.000000000000000000, 0.000000000000000000 ) ) ;
#14760=CARTESIAN_POINT ( 'NONE',  ( 39.49614528243539979, 1448.959577479020027, 136.3036146745320139 ) ) ;
#14763=CARTESIAN_POINT ( 'NONE',  ( -12.60062663947178407, 1398.286608578669757, 212.3194447688631499 ) ) ;
#14768=ADVANCED_FACE ( 'NONE', ( #45300 ), #61386, .F. ) ;
#14769=CARTESIAN_POINT ( 'NONE',  ( 21.02092206099549898, 1509.698195058749889, 230.2140218131270046 ) ) ;
#14771=VERTEX_POINT ( 'NONE', #20596 ) ;
#14773=CARTESIAN_POINT ( 'NONE',  ( 12.04367873614740070, 1433.833094619370058, 150.1136006245660042 ) ) ;
#14774=CARTESIAN_POINT ( 'NONE',  ( -12.05715834750000148, 1396.854116735730031, 212.7715747960579904 ) ) ;
#14775=CARTESIAN_POINT ( 'NONE',  ( -19.57217229339999776, 1409.761027581930193, 220.5029208888979895 ) ) ;
#14776=ORIENTED_EDGE ( 'NONE', *, *, #28893, .F. ) ;
#14777=CARTESIAN_POINT ( 'NONE',  ( -12.53380499174499896, 1445.052233488290085, 169.4755105688890069 ) ) ;
#14778=CARTESIAN_POINT ( 'NONE',  ( 20.81322922288373434, 1509.688917493156396, 230.4060755301925667 ) ) ;
#14780=DIRECTION ( 'NONE',  ( 0.03489949888733943212, -0.1170789740109212107, 0.9925092134695590040 ) ) ;
#14781=CARTESIAN_POINT ( 'NONE',  ( -13.70767992804610103, 1507.681782264339972, 184.2567517037919913 ) ) ;
#14782=EDGE_CURVE ( 'NONE', #24877, #79432, #101580, .T. ) ;
#14783=CARTESIAN_POINT ( 'NONE',  ( 2.434134029640000030, 1449.238291734089898, 183.8493297274980023 ) ) ;
#14784=CARTESIAN_POINT ( 'NONE',  ( -12.22918613309999891, 1416.219761279530076, 194.7382282326980203 ) ) ;
#14787=CARTESIAN_POINT ( 'NONE',  ( 10.81872853871839979, 1396.290858712909994, 206.7702252306009711 ) ) ;
#14788=CARTESIAN_POINT ( 'NONE',  ( -1.458875156116091532, 1414.913372219064286, 226.1171707424567785 ) ) ;
#14791=ORIENTED_EDGE ( 'NONE', *, *, #57648, .F. ) ;
#14792=CARTESIAN_POINT ( 'NONE',  ( 13.00929752435379960, 1434.785411124280017, 149.1497742818210099 ) ) ;
#14793=ORIENTED_EDGE ( 'NONE', *, *, #106659, .T. ) ;
#14796=CARTESIAN_POINT ( 'NONE',  ( -6.816513146730000194, 1465.924515906329816, 233.8132117517980078 ) ) ;
#14800=VERTEX_POINT ( 'NONE', #106819 ) ;
#14809=CARTESIAN_POINT ( 'NONE',  ( -29.83131695263168837, 1419.453406920455336, 269.4690164430861614 ) ) ;
#14810=CARTESIAN_POINT ( 'NONE',  ( -2.286415621570000223, 1410.371193408130011, 232.7320840571979943 ) ) ;
#14811=CARTESIAN_POINT ( 'NONE',  ( -0.8265315298756289453, 1415.089948427370018, 226.4875429796719857 ) ) ;
#14812=ORIENTED_EDGE ( 'NONE', *, *, #99379, .F. ) ;
#14813=CARTESIAN_POINT ( 'NONE',  ( 24.62909011900000067, 1439.532667989389893, 212.3621347402479955 ) ) ;
#14814=CARTESIAN_POINT ( 'NONE',  ( -34.94693337376789799, 1440.913060388619897, 250.8280191517029891 ) ) ;
#14816=CARTESIAN_POINT ( 'NONE',  ( -0.3779027989101099716, 1465.092193578540218, 236.9869935022780112 ) ) ;
#14817=CARTESIAN_POINT ( 'NONE',  ( 10.49062974637460144, 1411.164843042819939, 269.6264656941679618 ) ) ;
#14819=CARTESIAN_POINT ( 'NONE',  ( 23.51425668899999621, 1409.991808817929950, 208.7354357160110112 ) ) ;
#14820=CARTESIAN_POINT ( 'NONE',  ( -21.25388494759999958, 1509.593767402129970, 188.9414823285979992 ) ) ;
#14822=CARTESIAN_POINT ( 'NONE',  ( -11.60004869885203682, 1424.920234265779300, 136.4497806840202827 ) ) ;
#14824=CARTESIAN_POINT ( 'NONE',  ( -3.099034158239330150, 1447.528034658634169, 154.8291887632518922 ) ) ;
#14825=CARTESIAN_POINT ( 'NONE',  ( 0.1542088501289999858, 1419.787199956130053, 184.3756093272979797 ) ) ;
#14826=CARTESIAN_POINT ( 'NONE',  ( -11.61583318246324126, 1486.022327833872623, 184.5199211660089134 ) ) ;
#14830=CARTESIAN_POINT ( 'NONE',  ( 44.59191286470000648, 1449.238683939599923, 266.2373440796980049 ) ) ;
#14832=CARTESIAN_POINT ( 'NONE',  ( -5.334367723879999801, 1417.997726539230143, 234.5082296770980008 ) ) ;
#14833=CARTESIAN_POINT ( 'NONE',  ( -5.455799340109999562, 1438.116814643030011, 154.7280984898980307 ) ) ;
#14835=DIRECTION ( 'NONE',  ( -1.000000000000000000, 0.000000000000000000, -1.989566177384290042E-13 ) ) ;
#14839=CARTESIAN_POINT ( 'NONE',  ( -25.25200574389469921, 1450.804213008409988, 137.6134964715130025 ) ) ;
#14840=CARTESIAN_POINT ( 'NONE',  ( 10.36471150681333775, 1423.168727259207344, 137.2130303604900803 ) ) ;
#14844=CARTESIAN_POINT ( 'NONE',  ( 0.08825444290579999296, 1477.418261180029958, 229.8744888911979842 ) ) ;
#14846=CARTESIAN_POINT ( 'NONE',  ( 5.519893427111519202, 1440.499866072189889, 154.7645221071819890 ) ) ;
#14849=CARTESIAN_POINT ( 'NONE',  ( 12.93497730519910149, 1419.267168090624182, 228.9863995134908521 ) ) ;
#14850=CARTESIAN_POINT ( 'NONE',  ( 40.24868989356649962, 1444.402556327009961, 137.0644448199289798 ) ) ;
#14851=CARTESIAN_POINT ( 'NONE',  ( -20.17314850740000409, 1426.673360916329784, 222.1514211777979995 ) ) ;
#14854=EDGE_CURVE ( 'NONE', #86349, #107294, #10785, .T. ) ;
#14855=CARTESIAN_POINT ( 'NONE',  ( -17.16924453729999911, 1410.829424874530105, 226.1263841768980001 ) ) ;
#14857=CARTESIAN_POINT ( 'NONE',  ( -16.03274444936123899, 1469.111322135198634, 269.3691765490368653 ) ) ;
#14863=CARTESIAN_POINT ( 'NONE',  ( -0.2732116802759999574, 1417.283604781830036, 234.8460454422980206 ) ) ;
#14864=CARTESIAN_POINT ( 'NONE',  ( -13.44006708864586841, 1443.498725820041955, 187.0768896222344324 ) ) ;
#14867=CARTESIAN_POINT ( 'NONE',  ( -4.273773890143617749, 1416.013655775612051, 232.3752477624281312 ) ) ;
#14870=CARTESIAN_POINT ( 'NONE',  ( 17.33524322635545545, 1423.908641254848817, 228.7533431997620994 ) ) ;
#14871=CARTESIAN_POINT ( 'NONE',  ( -12.58564406202428998, 1442.782412299425005, 169.4702538016106814 ) ) ;
#14872=CARTESIAN_POINT ( 'NONE',  ( 18.11901460572769906, 1425.007341518409930, 225.3790264464149971 ) ) ;
#14874=CARTESIAN_POINT ( 'NONE',  ( -0.2193365489855410022, 1416.521607925270018, 191.0676367320770055 ) ) ;
#14875=CARTESIAN_POINT ( 'NONE',  ( -7.764017272732929520, 1409.184185844869944, 229.1854234326909818 ) ) ;
#14880=CARTESIAN_POINT ( 'NONE',  ( 13.13145645029999997, 1509.139720533629998, 233.9873431947980009 ) ) ;
#14882=CARTESIAN_POINT ( 'NONE',  ( -24.79040425310000018, 1444.204229992539922, 216.4501235802679844 ) ) ;
#14884=CARTESIAN_POINT ( 'NONE',  ( -11.66444761839999877, 1433.408000155229956, 150.9992530625980010 ) ) ;
#14886=CARTESIAN_POINT ( 'NONE',  ( 28.25086641300000068, 1508.135711190629991, 209.3856964555159834 ) ) ;
#14887=CARTESIAN_POINT ( 'NONE',  ( -26.05361808410000179, 1437.534443763920081, 137.0219046968979910 ) ) ;
#14888=CARTESIAN_POINT ( 'NONE',  ( -24.54165285250000039, 1438.756210186880026, 210.7135935008279830 ) ) ;
#14890=CARTESIAN_POINT ( 'NONE',  ( 1.228114143200000008, 1450.757138824929825, 181.5372585326979902 ) ) ;
#14893=CARTESIAN_POINT ( 'NONE',  ( 1.538781636355590080E-08, 1408.254370158240135, 262.4690811517129418 ) ) ;
#14895=ORIENTED_EDGE ( 'NONE', *, *, #73385, .F. ) ;
#14898=CARTESIAN_POINT ( 'NONE',  ( -3.409545297029999755, 1471.487073322530023, 269.6161692879980478 ) ) ;
#14902=CARTESIAN_POINT ( 'NONE',  ( 35.28300974739020290, 1451.608449428380027, 134.6903707226859979 ) ) ;
#14903=CARTESIAN_POINT ( 'NONE',  ( 18.91838588339999916, 1497.713060387329961, 197.2233373248979831 ) ) ;
#14904=LINE ( 'NONE', #91627, #103334 ) ;
#14908=CARTESIAN_POINT ( 'NONE',  ( -28.90140687091280114, 1413.853327124249972, 268.9772634007230181 ) ) ;
#14914=CARTESIAN_POINT ( 'NONE',  ( 16.68463225827361995, 1445.052233488289630, 162.0935120918203154 ) ) ;
#14918=CARTESIAN_POINT ( 'NONE',  ( -16.35848859230000230, 1455.453302215730218, 189.3475188266980069 ) ) ;
#14919=CARTESIAN_POINT ( 'NONE',  ( -1.835536242490369840, 1450.383119622699951, 182.7750508701979868 ) ) ;
#14921=CARTESIAN_POINT ( 'NONE',  ( -26.61235046579999874, 1435.626708122829996, 136.0714870250980084 ) ) ;
#14925=CARTESIAN_POINT ( 'NONE',  ( -27.50230175260729837, 1417.006653921450152, 270.1128687280570375 ) ) ;
#14927=CARTESIAN_POINT ( 'NONE',  ( -2.290042571849999931, 1395.993030436130084, 197.9397562440980209 ) ) ;
#14931=CARTESIAN_POINT ( 'NONE',  ( 0.2831897529540000069, 1451.162134428330091, 182.5531190971980209 ) ) ;
#14932=AXIS2_PLACEMENT_3D ( 'NONE', #97133, #20951, #54607 ) ;
#14933=CARTESIAN_POINT ( 'NONE',  ( 3.796654292859254376, 1425.671869022633928, 185.2437681722715581 ) ) ;
#14935=CARTESIAN_POINT ( 'NONE',  ( -24.59692435790000076, 1435.635346037049885, 137.3894803190979985 ) ) ;
#14936=CARTESIAN_POINT ( 'NONE',  ( -24.39471558800000039, 1441.818671265830062, 212.1017248396279911 ) ) ;
#14939=CARTESIAN_POINT ( 'NONE',  ( -2.120283308187459692, 1484.250716573789987, 183.0521180702210131 ) ) ;
#14944=CARTESIAN_POINT ( 'NONE',  ( -2.852604639739960035, 1451.959738234309953, 184.7483465814129886 ) ) ;
#14947=ORIENTED_EDGE ( 'NONE', *, *, #98035, .F. ) ;
#14948=CARTESIAN_POINT ( 'NONE',  ( -22.65254426311538083, 1509.725512665801261, 228.2121030422732701 ) ) ;
#14951=CARTESIAN_POINT ( 'NONE',  ( 13.57909981250000087, 1416.568813547830132, 196.3459685238979944 ) ) ;
#14954=CARTESIAN_POINT ( 'NONE',  ( -26.79413167943010166, 1436.761919080860025, 136.7821860765010058 ) ) ;
#14957=CARTESIAN_POINT ( 'NONE',  ( 23.34067364815647494, 1449.548550064944266, 217.2395114868710095 ) ) ;
#14958=CARTESIAN_POINT ( 'NONE',  ( -11.91321771470000002, 1435.943783413959864, 147.6429393588979906 ) ) ;
#14963=B_SPLINE_CURVE_WITH_KNOTS ( 'NONE', 5,
 ( #16259, #7877, #61088, #34189, #86798, #76746, #103029, #43155, #1163, #59418, #52661, #609 ),
 .UNSPECIFIED., .F., .F.,
 ( 6, 3, 3, 6 ),
 ( 0.000000000000000000, 0.3833332903980340434, 0.7666665807883968897, 1.000000000000000000 ),
 .UNSPECIFIED. ) ;
#14965=CARTESIAN_POINT ( 'NONE',  ( 2.409586283469999923, 1426.663880916129983, 144.1938086916980239 ) ) ;
#14971=CARTESIAN_POINT ( 'NONE',  ( 1.814287398422984365, 1416.723938728748408, 232.7280257503442158 ) ) ;
#14972=CARTESIAN_POINT ( 'NONE',  ( 17.08600013005979790, 1422.205976245335933, 226.7881206011809354 ) ) ;
#14975=CARTESIAN_POINT ( 'NONE',  ( 33.00780592730710339, 1440.913060383419861, 246.6091112861189742 ) ) ;
#14981=VERTEX_POINT ( 'NONE', #63220 ) ;
#14983=CARTESIAN_POINT ( 'NONE',  ( 16.19087789078229989, 1409.478458302130093, 193.2334102746530107 ) ) ;
#14984=CARTESIAN_POINT ( 'NONE',  ( -28.63451944679999883, 1509.912999839430086, 211.5264680655480163 ) ) ;
#14990=CARTESIAN_POINT ( 'NONE',  ( -15.52081487708860053, 1478.411708281340225, 223.8101585285860153 ) ) ;
#14991=DIRECTION ( 'NONE',  ( 0.5219928277095973179, -0.8520822723975763902, -0.03846152474253997089 ) ) ;
#14996=CARTESIAN_POINT ( 'NONE',  ( -1.273048297609999935, 1451.180663451930059, 183.3072205426980190 ) ) ;
#14999=ORIENTED_EDGE ( 'NONE', *, *, #15065, .T. ) ;
#15001=CARTESIAN_POINT ( 'NONE',  ( 1.188403172992487766, 1416.818673809778147, 190.1193007443792453 ) ) ;
#15004=CARTESIAN_POINT ( 'NONE',  ( 6.232532001850000114, 1407.162969929529936, 220.5304192662980256 ) ) ;
#15005=AXIS2_PLACEMENT_3D ( 'NONE', #84258, #83164, #32753 ) ;
#15010=CARTESIAN_POINT ( 'NONE',  ( 9.726491193908251375E-12, 1408.913060387299993, 194.1220083575990145 ) ) ;
#15011=CARTESIAN_POINT ( 'NONE',  ( 18.03150314649800023, 1424.669146068439886, 225.2932228502139935 ) ) ;
#15014=CARTESIAN_POINT ( 'NONE',  ( -2.500000055771189889, 1440.197962455250035, 166.9350719905560254 ) ) ;
#15015=AXIS2_PLACEMENT_3D ( 'NONE', #13755, #90479, #47396 ) ;
#15016=FACE_OUTER_BOUND ( 'NONE', #66767, .T. ) ;
#15018=( BOUNDED_SURFACE ( )  B_SPLINE_SURFACE ( 3, 2, ( 
 ( #14182, #82511, #99281 ),
 ( #40494, #107706, #30991 ),
 ( #107148, #14738, #74672 ),
 ( #108805, #56204, #66286 ) ),
 .UNSPECIFIED., .F., .F., .F. ) 
 B_SPLINE_SURFACE_WITH_KNOTS ( ( 4, 4 ),
 ( 3, 3 ),
 ( 0.008319848492105399312, 0.01047023456112128326 ),
 ( 0.6817855796338941898, 1.000000000000000000 ),
 .UNSPECIFIED. ) 
 GEOMETRIC_REPRESENTATION_ITEM ( )  RATIONAL_B_SPLINE_SURFACE ( (
 ( 0.8701819858983746991, 0.9047955706460268921, 1.000000000000000000),
 ( 0.8701112842800549085, 0.9047437203132890904, 1.000000000000000000),
 ( 0.8701364165503382431, 0.9047621515261470293, 1.000000000000000000),
 ( 0.8702549240939394526, 0.9048490612138414546, 1.000000000000000000) ) ) 
 REPRESENTATION_ITEM ( '' )  SURFACE ( )  );
#15019=CARTESIAN_POINT ( 'NONE',  ( -0.8090580814599999115, 1427.166763959530044, 147.9649995502979891 ) ) ;
#15020=CARTESIAN_POINT ( 'NONE',  ( 18.61241607401199616, 1457.060397574680110, 228.8782662039849924 ) ) ;
#15021=CARTESIAN_POINT ( 'NONE',  ( -12.94539156839999983, 1434.910719961430004, 150.0942592413979924 ) ) ;
#15026=CARTESIAN_POINT ( 'NONE',  ( -0.5542659975529999894, 1483.385152224330113, 181.9510117909979954 ) ) ;
#15028=CARTESIAN_POINT ( 'NONE',  ( -45.85454091276539401, 1440.913070276949838, 268.7563665289580399 ) ) ;
#15029=CARTESIAN_POINT ( 'NONE',  ( 13.62520701428609904, 1508.937755598840113, 233.7142831108280063 ) ) ;
#15031=EDGE_CURVE ( 'NONE', #13046, #93687, #48185, .T. ) ;
#15033=CARTESIAN_POINT ( 'NONE',  ( -23.28626003949876377, 1507.873436380149997, 195.0116325568262710 ) ) ;
#15035=CARTESIAN_POINT ( 'NONE',  ( 11.15268687969999917, 1425.700851675330114, 101.7515397216980091 ) ) ;
#15038=CARTESIAN_POINT ( 'NONE',  ( 17.30165530980000099, 1424.236263306130013, 225.6855429073979735 ) ) ;
#15039=FACE_OUTER_BOUND ( 'NONE', #60897, .T. ) ;
#15040=CARTESIAN_POINT ( 'NONE',  ( 0.5071369118009999566, 1469.874380101830184, 182.5356705811979907 ) ) ;
#15045=CARTESIAN_POINT ( 'NONE',  ( -8.163757246560001235, 1420.362486717730008, 225.2112877850979942 ) ) ;
#15046=CARTESIAN_POINT ( 'NONE',  ( -29.48232863870257603, 1509.960453018734142, 206.3162625148400764 ) ) ;
#15047=CARTESIAN_POINT ( 'NONE',  ( -6.943015404634899745, 1452.670604946809817, 151.6351347268530105 ) ) ;
#15050=CARTESIAN_POINT ( 'NONE',  ( -5.362275202304809696, 1424.093369006069906, 150.3042897941160163 ) ) ;
#15052=CARTESIAN_POINT ( 'NONE',  ( 15.63428379070249896, 1422.707660709189895, 229.1465903752480244 ) ) ;
#15057=CARTESIAN_POINT ( 'NONE',  ( -23.95203783885379778, 1410.422133454150071, 208.8949471922620091 ) ) ;
#15061=CARTESIAN_POINT ( 'NONE',  ( -1.395300564360000051, 1498.352961133030021, 236.7605676195980209 ) ) ;
#15063=EDGE_CURVE ( 'NONE', #52165, #69390, #24246, .T. ) ;
#15064=CARTESIAN_POINT ( 'NONE',  ( 41.51622458814379257, 1455.223082529530075, 269.0892613835300153 ) ) ;
#15065=EDGE_CURVE ( 'NONE', #22209, #3563, #39373, .T. ) ;
#15067=CARTESIAN_POINT ( 'NONE',  ( -0.2357814831160000291, 1418.572813431130044, 184.6863074503980044 ) ) ;
#15080=CARTESIAN_POINT ( 'NONE',  ( 3.725874866239260008, 1452.782949969990113, 152.2831223846509943 ) ) ;
#15082=CARTESIAN_POINT ( 'NONE',  ( 22.57032379820000045, 1409.701233462030132, 209.8663284536589799 ) ) ;
#15085=VECTOR ( 'NONE', #945, 1000.000000000000114 ) ;
#15086=CARTESIAN_POINT ( 'NONE',  ( 1.988761914397050079, 1408.982509483710146, 186.9246551635189917 ) ) ;
#15087=CARTESIAN_POINT ( 'NONE',  ( -13.01189509148379919, 1434.786097740819969, 149.1479131938150147 ) ) ;
#15088=CARTESIAN_POINT ( 'NONE',  ( -18.41706550949158938, 1424.167467087569776, 225.1579557749482774 ) ) ;
#15089=CARTESIAN_POINT ( 'NONE',  ( 3.307325631547500144, 1441.238735741373148, 170.5343657987176300 ) ) ;
#15091=CARTESIAN_POINT ( 'NONE',  ( 11.16223122930000144, 1428.970455832429934, 101.8807690336980016 ) ) ;
#15092=ORIENTED_EDGE ( 'NONE', *, *, #5003, .T. ) ;
#15093=CARTESIAN_POINT ( 'NONE',  ( 16.42420380379999756, 1507.212883763329955, 193.5443561786979956 ) ) ;
#15095=DIRECTION ( 'NONE',  ( 0.0008672850459984940506, -0.9990096763985240047, -0.04448498936456254937 ) ) ;
#15096=CARTESIAN_POINT ( 'NONE',  ( 19.34100150109859939, 1467.084855511749993, 225.9993250057500234 ) ) ;
#15103=CARTESIAN_POINT ( 'NONE',  ( -43.50000000000000000, 1445.861068816730040, 271.1218459616979999 ) ) ;
#15104=CARTESIAN_POINT ( 'NONE',  ( -13.58268883510000080, 1416.851343894929869, 221.9096085503980191 ) ) ;
#15105=CARTESIAN_POINT ( 'NONE',  ( 11.94146967429999862, 1433.521468468569992, 150.1184368365979935 ) ) ;
#15106=CARTESIAN_POINT ( 'NONE',  ( 10.04572263220000039, 1464.202968133530021, 255.3819207742980097 ) ) ;
#15109=EDGE_CURVE ( 'NONE', #44371, #79447, #40755, .T. ) ;
#15113=CARTESIAN_POINT ( 'NONE',  ( -14.63705847081953593, 1422.169902665600603, 229.4588690542234417 ) ) ;
#15114=CARTESIAN_POINT ( 'NONE',  ( -17.71284803180000011, 1486.217784300129779, 188.1321109405980110 ) ) ;
#15116=CARTESIAN_POINT ( 'NONE',  ( 18.58720762869999987, 1416.311719779230089, 209.7162280979700029 ) ) ;
#15123=CARTESIAN_POINT ( 'NONE',  ( -6.250808155840000602, 1416.216596894629902, 226.2958911897979988 ) ) ;
#15124=AXIS2_PLACEMENT_3D ( 'NONE', #100885, #41566, #39905 ) ;
#15125=CARTESIAN_POINT ( 'NONE',  ( 0.1699996708203529716, 1480.329832774919851, 182.0802225456559995 ) ) ;
#15126=CARTESIAN_POINT ( 'NONE',  ( 0.02192821825021479959, 1407.539782046369965, 222.1835171484239879 ) ) ;
#15129=CARTESIAN_POINT ( 'NONE',  ( 13.80567663220000085, 1434.979608490319833, 147.6248746541980097 ) ) ;
#15130=CARTESIAN_POINT ( 'NONE',  ( -39.77086281159900238, 1438.526156311480008, 134.0999999980039945 ) ) ;
#15138=B_SPLINE_CURVE_WITH_KNOTS ( 'NONE', 5,
 ( #69801, #105593, #37279, #20444, #63072, #79285, #97172, #78725, #103919, #54653, #61399, #46254 ),
 .UNSPECIFIED., .F., .F.,
 ( 6, 3, 3, 6 ),
 ( 0.000000000000000000, 0.2842603455368540866, 0.7006323907210947333, 1.000000000000000000 ),
 .UNSPECIFIED. ) ;
#15139=CARTESIAN_POINT ( 'NONE',  ( 31.52040524782195874, 1416.197860221249357, 269.3256485028547331 ) ) ;
#15146=ORIENTED_EDGE ( 'NONE', *, *, #8408, .F. ) ;
#15147=CARTESIAN_POINT ( 'NONE',  ( -29.80701629120000007, 1451.872188912029969, 134.8363203424979986 ) ) ;
#15148=CARTESIAN_POINT ( 'NONE',  ( -16.26157404866599876, 1409.582217294140037, 225.7367796582349797 ) ) ;
#15153=CARTESIAN_POINT ( 'NONE',  ( -19.30538610943497346, 1410.948714638366710, 222.3723562416497259 ) ) ;
#15155=CARTESIAN_POINT ( 'NONE',  ( -0.3961054703501400431, 1418.676517288780133, 184.7143626773449796 ) ) ;
#15156=CARTESIAN_POINT ( 'NONE',  ( 21.76795527650000039, 1409.673214137629884, 214.0268462324280279 ) ) ;
#15157=CARTESIAN_POINT ( 'NONE',  ( -2.919750075684910406, 1419.523100886769953, 186.2043985311460119 ) ) ;
#15158=CARTESIAN_POINT ( 'NONE',  ( -17.58914910740000082, 1423.039930255530180, 226.3751546217980035 ) ) ;
#15162=CARTESIAN_POINT ( 'NONE',  ( 3.871411596960000256, 1475.513060387329915, 229.5852438705979921 ) ) ;
#15167=CARTESIAN_POINT ( 'NONE',  ( -6.358070405449739226, 1484.270638837799879, 183.8946224230450355 ) ) ;
#15168=ADVANCED_FACE ( 'NONE', ( #71921 ), #42518, .T. ) ;
#15169=EDGE_LOOP ( 'NONE', ( #3415, #96183, #5041, #53963 ) ) ;
#15172=CARTESIAN_POINT ( 'NONE',  ( -4.221801104570530150, 1441.602310353549910, 168.2831674553420100 ) ) ;
#15174=ORIENTED_EDGE ( 'NONE', *, *, #99268, .T. ) ;
#15179=CARTESIAN_POINT ( 'NONE',  ( -11.73940163521978519, 1426.278578077852444, 144.3763880045744656 ) ) ;
#15180=CARTESIAN_POINT ( 'NONE',  ( 15.89852580928170056, 1409.468224213880148, 192.8813377015480057 ) ) ;
#15182=CARTESIAN_POINT ( 'NONE',  ( 40.26322191559909669, 1439.095366118250240, 135.2291069399360026 ) ) ;
#15184=B_SPLINE_SURFACE_WITH_KNOTS ( 'NONE', 5, 1, ( 
 ( #65739, #6914 ),
 ( #22030, #14206 ),
 ( #83615, #13636 ),
 ( #99304, #32673 ),
 ( #99858, #5265 ),
 ( #66851, #57356 ),
 ( #14760, #73597 ),
 ( #31012, #41070 ),
 ( #48947, #6372 ) ),
 .UNSPECIFIED., .F., .F., .F.,
 ( 6, 3, 6 ),
 ( 2, 2 ),
 ( 0.7097524320730000946, 4.064565667710000163, 10.06421383387139912 ),
 ( -13.48619596139999999, -1.265881781730000100 ),
 .UNSPECIFIED. ) ;
#15185=CARTESIAN_POINT ( 'NONE',  ( 33.92724808885991905, 1435.682287743722554, 135.5036907871966037 ) ) ;
#15189=CARTESIAN_POINT ( 'NONE',  ( 13.58268853708210067, 1416.851343896850040, 196.3340833727469885 ) ) ;
#15190=EDGE_LOOP ( 'NONE', ( #75577, #6786, #101326 ) ) ;
#15191=CARTESIAN_POINT ( 'NONE',  ( -18.41508126919999810, 1458.154041264329862, 227.7774065783979722 ) ) ;
#15194=CARTESIAN_POINT ( 'NONE',  ( 11.60004869885203682, 1426.043485606469631, 137.7524099801277657 ) ) ;
#15195=CARTESIAN_POINT ( 'NONE',  ( -1.757532416683340148, 1451.933574871519795, 184.1885909450070073 ) ) ;
#15197=CARTESIAN_POINT ( 'NONE',  ( -3.296302496939999660, 1485.523047861029909, 182.9415910454979723 ) ) ;
#15199=CARTESIAN_POINT ( 'NONE',  ( 18.22873622136830107, 1457.634151734390116, 229.9687917111629929 ) ) ;
#15200=CARTESIAN_POINT ( 'NONE',  ( -41.65674268029999894, 1443.992461967939789, 135.6790812281979868 ) ) ;
#15201=CARTESIAN_POINT ( 'NONE',  ( 40.71747595459699909, 1438.773003512770174, 135.6938347574059947 ) ) ;
#15202=CARTESIAN_POINT ( 'NONE',  ( 2.613239871555069538, 1421.346360341460013, 183.3165747233060188 ) ) ;
#15204=EDGE_CURVE ( 'NONE', #68277, #31171, #94683, .T. ) ;
#15205=CARTESIAN_POINT ( 'NONE',  ( 25.67574771179999971, 1437.591200499259912, 137.2873827178979695 ) ) ;
#15212=CARTESIAN_POINT ( 'NONE',  ( 42.06232107555830169, 1440.913060387330006, 269.6487541170399709 ) ) ;
#15214=CARTESIAN_POINT ( 'NONE',  ( -0.0002035089733392563926, 1452.237673957955622, 153.8261543310597688 ) ) ;
#15216=CARTESIAN_POINT ( 'NONE',  ( -14.20165756390000134, 1416.819756528530206, 221.7375112866980089 ) ) ;
#15217=CARTESIAN_POINT ( 'NONE',  ( -11.00562449240939955, 1432.347154516129876, 151.7431427700479958 ) ) ;
#15219=CARTESIAN_POINT ( 'NONE',  ( 24.08426297012860218, 1411.115209414830133, 209.6325633951909708 ) ) ;
#15220=CARTESIAN_POINT ( 'NONE',  ( 21.95096434148669928, 1409.939836231839990, 206.2919199104040331 ) ) ;
#15225=EDGE_CURVE ( 'NONE', #34381, #84728, #104817, .T. ) ;
#15226=CARTESIAN_POINT ( 'NONE',  ( 15.19576882900000037, 1461.839785508229852, 229.8993157890980115 ) ) ;
#15228=CARTESIAN_POINT ( 'NONE',  ( -4.641209657417020296, 1422.124063284806425, 184.6640048031023298 ) ) ;
#15229=B_SPLINE_SURFACE_WITH_KNOTS ( 'NONE', 5, 5, ( 
 ( #79021, #96350, #2322, #80650, #36432, #63869 ),
 ( #104747, #62224, #19627, #72266, #87968, #106400 ),
 ( #21251, #97984, #100200, #73910, #107490, #98538 ),
 ( #13974, #108038, #48162, #81727, #40845, #31333 ),
 ( #75018, #83390, #6132, #49264, #58212, #5035 ),
 ( #82299, #57677, #64964, #23484, #6688, #56558 ),
 ( #39180, #109168, #91791, #40289, #5597, #15067 ),
 ( #21806, #22913, #92338, #24015, #72810, #32454 ),
 ( #106941, #13413, #15610, #82841, #90686, #66630 ) ),
 .UNSPECIFIED., .F., .F., .F.,
 ( 6, 3, 6 ),
 ( 6, 6 ),
 ( 0.8628043814250000443, 1.314432051750000108, 1.883620747549999974 ),
 ( 0.000000000000000000, 2.000000000000000000 ),
 .UNSPECIFIED. ) ;
#15235=CARTESIAN_POINT ( 'NONE',  ( -0.0001187281342228439996, 1508.967929526819944, 179.3767679645770272 ) ) ;
#15239=CARTESIAN_POINT ( 'NONE',  ( -11.60004869885203682, 1426.044482836622592, 137.7673702721163238 ) ) ;
#15243=CARTESIAN_POINT ( 'NONE',  ( 21.19943833389999810, 1451.689670470829924, 217.4746504698680098 ) ) ;
#15244=CARTESIAN_POINT ( 'NONE',  ( -11.85178780869999926, 1431.281462211560211, 150.3047777764980140 ) ) ;
#15245=CARTESIAN_POINT ( 'NONE',  ( 19.02706862106219887, 1456.916313564460097, 225.6436289706080345 ) ) ;
#15247=CARTESIAN_POINT ( 'NONE',  ( 11.84030397337090079, 1430.235998727099741, 151.0624529839080026 ) ) ;
#15251=CARTESIAN_POINT ( 'NONE',  ( -19.32501916510000228, 1470.091136407030035, 227.3171351542980005 ) ) ;
#15254=ORIENTED_EDGE ( 'NONE', *, *, #3680, .T. ) ;
#15256=CARTESIAN_POINT ( 'NONE',  ( 3.773607150769999752, 1405.866055185730147, 267.5310499900980403 ) ) ;
#15258=CARTESIAN_POINT ( 'NONE',  ( -0.1764364529069999965, 1409.076774544030059, 185.6010313908980152 ) ) ;
#15259=CARTESIAN_POINT ( 'NONE',  ( 19.07614737060000110, 1410.874611392730003, 195.4187278566980126 ) ) ;
#15260=CARTESIAN_POINT ( 'NONE',  ( 21.16486544290946981, 1428.404148231732506, 219.5078859491472656 ) ) ;
#15261=CARTESIAN_POINT ( 'NONE',  ( 0.000000000000000000, 1502.413060387330006, 209.1218459616979999 ) ) ;
#15262=CARTESIAN_POINT ( 'NONE',  ( 26.35471571933159751, 1507.985750330240080, 216.6976075425179999 ) ) ;
#15263=B_SPLINE_CURVE_WITH_KNOTS ( 'NONE', 5,
 ( #96313, #38598, #72778, #29650, #97410, #63837, #71143, #88469, #87932, #96874, #104706, #20680, #72238, #97949, #89004 ),
 .UNSPECIFIED., .F., .F.,
 ( 6, 3, 3, 3, 6 ),
 ( -48.56910781718399761, -39.03858743909999873, -32.22913687700000196, -31.51384161189999844, -29.50806686130000145 ),
 .UNSPECIFIED. ) ;
#15264=CARTESIAN_POINT ( 'NONE',  ( -18.84860651825824363, 1456.786630790735671, 228.5413354237351768 ) ) ;
#15266=CARTESIAN_POINT ( 'NONE',  ( -12.79312897949999872, 1445.016120524290045, 186.3935252196979775 ) ) ;
#15267=CARTESIAN_POINT ( 'NONE',  ( 2.499999999889860103, 1448.906648695949798, 155.3362529649780015 ) ) ;
#15272=CARTESIAN_POINT ( 'NONE',  ( -27.15947446952620226, 1507.993364321890112, 211.1689828938959863 ) ) ;
#15274=CARTESIAN_POINT ( 'NONE',  ( -1.757373113509999918, 1475.295645524329984, 269.4976378123980112 ) ) ;
#15275=CARTESIAN_POINT ( 'NONE',  ( -4.229825888870420769, 1446.290640099090069, 165.0045831357620045 ) ) ;
#15277=CARTESIAN_POINT ( 'NONE',  ( 17.84759684480400210, 1410.895160446669934, 223.1913782762499920 ) ) ;
#15279=CARTESIAN_POINT ( 'NONE',  ( 13.58256589259447011, 1416.843574543525847, 196.3343232356145052 ) ) ;
#15281=CARTESIAN_POINT ( 'NONE',  ( -25.17436548464209878, 1470.080601114610090, 212.0235103180719705 ) ) ;
#15283=CARTESIAN_POINT ( 'NONE',  ( -2.884599899255949917E-09, 1473.199988346640112, 268.3915997654160037 ) ) ;
#15287=CARTESIAN_POINT ( 'NONE',  ( -15.06844210530799977, 1422.391250798362080, 229.4663103607340133 ) ) ;
#15289=CARTESIAN_POINT ( 'NONE',  ( -25.33241404900000049, 1413.251821757829930, 269.9969244510980388 ) ) ;
#15291=CARTESIAN_POINT ( 'NONE',  ( -4.556184579163090831, 1410.448051561546436, 232.0254849714374075 ) ) ;
#15296=CARTESIAN_POINT ( 'NONE',  ( 10.68407736780000050, 1425.006924162730229, 135.9205847407980059 ) ) ;
#15301=ADVANCED_FACE ( 'NONE', ( #83423 ), #10393, .F. ) ;
#15304=CARTESIAN_POINT ( 'NONE',  ( -11.79165762230000070, 1429.416862815430022, 146.4064176768980019 ) ) ;
#15310=ORIENTED_EDGE ( 'NONE', *, *, #67325, .F. ) ;
#15312=CARTESIAN_POINT ( 'NONE',  ( 11.86993521259999973, 1433.837969291950003, 150.7297411583980136 ) ) ;
#15313=CARTESIAN_POINT ( 'NONE',  ( -10.98139245720000012, 1398.238761414130067, 216.8837352115380099 ) ) ;
#15314=CARTESIAN_POINT ( 'NONE',  ( -19.88787437039999872, 1410.102804823130100, 220.6443014318979863 ) ) ;
#15316=CARTESIAN_POINT ( 'NONE',  ( -13.39960398253788476, 1444.421273251342882, 169.3685383806885056 ) ) ;
#15317=CARTESIAN_POINT ( 'NONE',  ( 22.10835456647167874, 1509.702725196560550, 228.7991371166729948 ) ) ;
#15320=CARTESIAN_POINT ( 'NONE',  ( -13.70766983986010068, 1507.659368579370266, 184.2581583972360022 ) ) ;
#15322=CARTESIAN_POINT ( 'NONE',  ( 13.43062830470000080, 1488.164680700029976, 186.5792399276980120 ) ) ;
#15325=CARTESIAN_POINT ( 'NONE',  ( 7.892725014381700710, 1396.188680504749982, 201.3838934717110192 ) ) ;
#15326=CARTESIAN_POINT ( 'NONE',  ( 1.556886619979999997, 1415.063410501330054, 191.4794882261979865 ) ) ;
#15327=CARTESIAN_POINT ( 'NONE',  ( 11.86596898630000041, 1432.335940955089882, 150.3973237302979840 ) ) ;
#15328=CARTESIAN_POINT ( 'NONE',  ( 8.170454128426975160, 1509.198649520710887, 180.9503965351503609 ) ) ;
#15330=CARTESIAN_POINT ( 'NONE',  ( 13.02655316196230117, 1434.814175597650092, 149.4409609364860216 ) ) ;
#15334=CARTESIAN_POINT ( 'NONE',  ( 12.97436564310944185, 1444.891968944272094, 169.4253161487108059 ) ) ;
#15335=CARTESIAN_POINT ( 'NONE',  ( -11.13796040809999965, 1464.110348585029897, 231.7316128992979998 ) ) ;
#15336=CARTESIAN_POINT ( 'NONE',  ( -13.02322702429999879, 1416.825784017130218, 196.6108461441979784 ) ) ;
#15339=ORIENTED_EDGE ( 'NONE', *, *, #95552, .F. ) ;
#15346=ORIENTED_EDGE ( 'NONE', *, *, #84679, .F. ) ;
#15350=CARTESIAN_POINT ( 'NONE',  ( -32.05312539274948591, 1421.205571191992931, 269.4939401719450416 ) ) ;
#15351=CARTESIAN_POINT ( 'NONE',  ( -2.933338486410000279, 1410.393077976529867, 232.5461313705979762 ) ) ;
#15352=EDGE_CURVE ( 'NONE', #42031, #24662, #76139, .T. ) ;
#15353=CARTESIAN_POINT ( 'NONE',  ( -2.499989269620250809, 1419.524750234567819, 137.1000002976804808 ) ) ;
#15354=VERTEX_POINT ( 'NONE', #93469 ) ;
#15355=CARTESIAN_POINT ( 'NONE',  ( 19.81803190540000159, 1427.321367310129972, 222.3183646145980106 ) ) ;
#15356=CARTESIAN_POINT ( 'NONE',  ( -29.09122759982509976, 1440.913060387109908, 235.2915179107689880 ) ) ;
#15358=DIRECTION ( 'NONE',  ( 0.1402804634180439824, -0.9901118076173108795, 0.000000000000000000 ) ) ;
#15359=EDGE_CURVE ( 'NONE', #22669, #101515, #74095, .T. ) ;
#15360=CARTESIAN_POINT ( 'NONE',  ( 14.82025145092669938, 1411.931168022049860, 269.8832746614870075 ) ) ;
#15363=CARTESIAN_POINT ( 'NONE',  ( 22.71803131159999722, 1409.706390560829959, 209.2188350014689888 ) ) ;
#15365=CARTESIAN_POINT ( 'NONE',  ( -20.54538654549999777, 1508.881852289130165, 189.3180432071980022 ) ) ;
#15367=CIRCLE ( 'NONE', #76132, 34.90184096762461508 ) ;
#15368=CARTESIAN_POINT ( 'NONE',  ( -4.363122647530000009, 1421.971318475729959, 179.5815723472979926 ) ) ;
#15370=CARTESIAN_POINT ( 'NONE',  ( 0.5000000000152821089, 1448.894380913990062, 155.6080914337030094 ) ) ;
#15373=CARTESIAN_POINT ( 'NONE',  ( 10.97941491499529931, 1432.933185717909964, 151.7695633904889974 ) ) ;
#15377=CARTESIAN_POINT ( 'NONE',  ( 14.25481165789999949, 1474.931993151730012, 267.1910255919980273 ) ) ;
#15379=CARTESIAN_POINT ( 'NONE',  ( -11.91935979259999989, 1420.493316629130049, 231.2800121289980098 ) ) ;
#15382=CARTESIAN_POINT ( 'NONE',  ( -23.83765245669999899, 1446.530553800920188, 215.3656821590780055 ) ) ;
#15386=DIRECTION ( 'NONE',  ( 0.1400401707400374951, -0.004890310883056902050, 0.9901337462376323950 ) ) ;
#15389=EDGE_CURVE ( 'NONE', #5604, #35589, #55453, .T. ) ;
#15391=CARTESIAN_POINT ( 'NONE',  ( 0.2316317416650000294, 1477.419807478629991, 229.8396568727980025 ) ) ;
#15393=CARTESIAN_POINT ( 'NONE',  ( 7.229617388605507955, 1438.908991744435752, 154.0610282733643999 ) ) ;
#15396=CARTESIAN_POINT ( 'NONE',  ( 26.14468651563449342, 1450.763943277846010, 136.6602026170544377 ) ) ;
#15397=DIRECTION ( 'NONE',  ( 0.000000000000000000, 0.000000000000000000, -1.000000000000000000 ) ) ;
#15398=CARTESIAN_POINT ( 'NONE',  ( 27.58302911533250068, 1435.460667994110054, 135.2629876134730011 ) ) ;
#15399=CARTESIAN_POINT ( 'NONE',  ( 38.58175818029209836, 1448.251245179850002, 136.4584366939950257 ) ) ;
#15400=CARTESIAN_POINT ( 'NONE',  ( -21.74327147740000044, 1430.168649232730104, 219.0066490272480166 ) ) ;
#15403=CARTESIAN_POINT ( 'NONE',  ( 8.768085951239999787, 1509.161958816129982, 181.7959786723980073 ) ) ;
#15405=CARTESIAN_POINT ( 'NONE',  ( -9.579969104820666104, 1470.643550730757852, 269.3463861652618334 ) ) ;
#15406=ORIENTED_EDGE ( 'NONE', *, *, #59018, .T. ) ;
#15408=CARTESIAN_POINT ( 'NONE',  ( 9.336110127025321503, 1506.539416727244770, 189.1210688587442803 ) ) ;
#15411=CARTESIAN_POINT ( 'NONE',  ( -0.02484813282310000329, 1416.432140399929949, 233.7186307104979903 ) ) ;
#15412=CARTESIAN_POINT ( 'NONE',  ( -28.28208339020000039, 1508.151294418729776, 209.1342425839550287 ) ) ;
#15415=CARTESIAN_POINT ( 'NONE',  ( -3.958671420333373714, 1415.944797298322328, 232.4758296456245716 ) ) ;
#15416=CARTESIAN_POINT ( 'NONE',  ( -7.776877434901703801, 1451.396943400985947, 153.0106348905935931 ) ) ;
#15417=CARTESIAN_POINT ( 'NONE',  ( 24.32116265780000219, 1435.530952642309785, 137.6072328918980077 ) ) ;
#15419=CARTESIAN_POINT ( 'NONE',  ( 11.87502392341400004, 1433.007271648830056, 149.9804723818110119 ) ) ;
#15420=ORIENTED_EDGE ( 'NONE', *, *, #59024, .F. ) ;
#15421=CARTESIAN_POINT ( 'NONE',  ( 1.377258800780170045, 1414.913060387399810, 192.4870635420249982 ) ) ;
#15423=VERTEX_POINT ( 'NONE', #45320 ) ;
#15425=CARTESIAN_POINT ( 'NONE',  ( 16.36863935783290103, 1414.913057862230062, 208.9007734745979974 ) ) ;
#15427=CARTESIAN_POINT ( 'NONE',  ( -11.62807272172398498, 1428.982488964479899, 136.1186897298418046 ) ) ;
#15428=CARTESIAN_POINT ( 'NONE',  ( -25.01541328220000082, 1442.557000325939953, 216.4497915791480125 ) ) ;
#15429=B_SPLINE_CURVE_WITH_KNOTS ( 'NONE', 5,
 ( #5542, #30172, #57625, #56507, #31838, #66024 ),
 .UNSPECIFIED., .F., .F.,
 ( 6, 6 ),
 ( 0.03026097244042860734, 1.000000000000000000 ),
 .UNSPECIFIED. ) ;
#15431=CARTESIAN_POINT ( 'NONE',  ( -11.81225577550000061, 1433.099404687269953, 150.5666296323979907 ) ) ;
#15433=CARTESIAN_POINT ( 'NONE',  ( -2.919621720534709919, 1419.522956690290130, 186.2043860719099939 ) ) ;
#15435=CARTESIAN_POINT ( 'NONE',  ( -24.38244995200000176, 1440.343059974619791, 211.3205732649580000 ) ) ;
#15439=CARTESIAN_POINT ( 'NONE',  ( -28.16265580408766667, 1510.008130024179991, 219.4883605467473160 ) ) ;
#15440=CIRCLE ( 'NONE', #56634, 24.00543915299668640 ) ;
#15441=CARTESIAN_POINT ( 'NONE',  ( -2.521777220032119811E-09, 1415.593833303999872, 242.3213147721250209 ) ) ;
#15444=CARTESIAN_POINT ( 'NONE',  ( -11.77777284958320081, 1427.343273226020074, 146.9184637112259963 ) ) ;
#15446=CARTESIAN_POINT ( 'NONE',  ( -4.235651747309999493, 1473.118544177530111, 270.4270856384979993 ) ) ;
#15447=CARTESIAN_POINT ( 'NONE',  ( 37.66849513895419932, 1445.052233489950140, 137.0436250799990034 ) ) ;
#15449=CARTESIAN_POINT ( 'NONE',  ( 39.65045748264740411, 1446.880369190260126, 136.6574868213660068 ) ) ;
#15451=CARTESIAN_POINT ( 'NONE',  ( 19.75084982879439721, 1455.504334177440114, 226.5702129464319796 ) ) ;
#15455=CARTESIAN_POINT ( 'NONE',  ( -33.44259286938519438, 1416.839468587309966, 266.5282928195520071 ) ) ;
#15459=EDGE_LOOP ( 'NONE', ( #678, #24417, #41589, #79926, #61967 ) ) ;
#15462=B_SPLINE_CURVE_WITH_KNOTS ( 'NONE', 3,
 ( #29225, #20802, #55001, #46597 ),
 .UNSPECIFIED., .F., .F.,
 ( 4, 4 ),
 ( -49.62857927099999955, -30.39441596882049978 ),
 .UNSPECIFIED. ) ;
#15467=CARTESIAN_POINT ( 'NONE',  ( -17.21868475540000176, 1485.486038110229856, 188.3681669011979807 ) ) ;
#15469=ORIENTED_EDGE ( 'NONE', *, *, #22282, .T. ) ;
#15470=CARTESIAN_POINT ( 'NONE',  ( -26.01569841849999776, 1436.364670503799744, 136.8463858237979878 ) ) ;
#15475=CARTESIAN_POINT ( 'NONE',  ( -43.01346508794090084, 1430.448015371199972, 270.1100027560920580 ) ) ;
#15477=CARTESIAN_POINT ( 'NONE',  ( -37.65047686723229958, 1442.773887284729881, 137.1096749952629921 ) ) ;
#15483=CARTESIAN_POINT ( 'NONE',  ( -24.81662394629999824, 1435.862065122790000, 137.5270316210979900 ) ) ;
#15484=CARTESIAN_POINT ( 'NONE',  ( -24.90625602310000275, 1442.467917342170267, 210.4928140592879799 ) ) ;
#15489=CARTESIAN_POINT ( 'NONE',  ( 3.672250414928510676, 1440.842333270420340, 156.5454195792117673 ) ) ;
#15492=DIRECTION ( 'NONE',  ( 0.000000000000000000, 0.000000000000000000, -1.000000000000000000 ) ) ;
#15493=CARTESIAN_POINT ( 'NONE',  ( -11.44291211132249941, 1428.994970299889928, 123.0295630242879952 ) ) ;
#15497=DIRECTION ( 'NONE',  ( 0.4604555384065119883, -0.2169306526911162492, 0.8607681389745879263 ) ) ;
#15498=CARTESIAN_POINT ( 'NONE',  ( 4.380088106299919737, 1459.297325631019930, 233.6318968629059896 ) ) ;
#15500=CARTESIAN_POINT ( 'NONE',  ( 23.96868460540000001, 1452.076057926130034, 136.6875046473980149 ) ) ;
#15503=CARTESIAN_POINT ( 'NONE',  ( 23.33267522454316278, 1449.572396795839040, 217.2601772566924581 ) ) ;
#15505=CARTESIAN_POINT ( 'NONE',  ( -12.00000000000000000, 1443.913060387330006, 147.5878346084980137 ) ) ;
#15510=ADVANCED_FACE ( 'NONE', ( #62124 ), #8541, .T. ) ;
#15512=CARTESIAN_POINT ( 'NONE',  ( 2.347483145930000070, 1420.008254648030061, 185.1099769671980084 ) ) ;
#15513=CARTESIAN_POINT ( 'NONE',  ( 1.458875156680665475, 1414.913372219064740, 192.1265211809087532 ) ) ;
#15514=EDGE_CURVE ( 'NONE', #67100, #69813, #30036, .T. ) ;
#15516=CARTESIAN_POINT ( 'NONE',  ( 11113.05219665069490, 50.13405481564041821, 8751.225064238969935 ) ) ;
#15518=CARTESIAN_POINT ( 'NONE',  ( 1.762089052713846193, 1416.154897214564016, 232.4884135401189269 ) ) ;
#15520=CARTESIAN_POINT ( 'NONE',  ( 17.67984484133276979, 1423.296779864863993, 226.2374533289532224 ) ) ;
#15523=CARTESIAN_POINT ( 'NONE',  ( 40.10692519302580195, 1440.913060364430066, 259.4359539563330372 ) ) ;
#15526=CARTESIAN_POINT ( 'NONE',  ( 13.07075197220000184, 1426.017600903129960, 222.5644795257979922 ) ) ;
#15529=CARTESIAN_POINT ( 'NONE',  ( -6.599309851546266259, 1506.776552836644441, 230.5385063488150479 ) ) ;
#15531=CARTESIAN_POINT ( 'NONE',  ( -28.32265151400000036, 1509.673549454329759, 210.9825397456980056 ) ) ;
#15534=CARTESIAN_POINT ( 'NONE',  ( 24.63413957469291304, 1509.887610572149470, 226.3134076709914382 ) ) ;
#15538=CARTESIAN_POINT ( 'NONE',  ( 24.24033398420000296, 1452.066569271830076, 137.1576855576979881 ) ) ;
#15545=CARTESIAN_POINT ( 'NONE',  ( -16.64778510051399962, 1409.494413853340120, 224.2640743094200104 ) ) ;
#15546=ORIENTED_EDGE ( 'NONE', *, *, #70127, .T. ) ;
#15549=CARTESIAN_POINT ( 'NONE',  ( 34.63223096084099950, 1437.077591941980018, 136.5438288522229868 ) ) ;
#15554=CARTESIAN_POINT ( 'NONE',  ( -7.628773549489999972, 1416.913060387330006, 201.4930723711279938 ) ) ;
#15558=CARTESIAN_POINT ( 'NONE',  ( 18.28913704150000186, 1425.363277320230054, 225.3253160533980122 ) ) ;
#15559=CARTESIAN_POINT ( 'NONE',  ( 4.401092417150000102, 1420.174153566729956, 185.7217845719979721 ) ) ;
#15561=CARTESIAN_POINT ( 'NONE',  ( -2.500000000000000000, 1439.625347662559989, 166.9460400830979836 ) ) ;
#15563=CARTESIAN_POINT ( 'NONE',  ( -3.179421471999289928, 1451.291958863610262, 184.8185991936910000 ) ) ;
#15565=FACE_OUTER_BOUND ( 'NONE', #75820, .T. ) ;
#15566=CARTESIAN_POINT ( 'NONE',  ( 15.71062681160000096, 1468.834934971430130, 189.3083005990980041 ) ) ;
#15567=CARTESIAN_POINT ( 'NONE',  ( -1.145689533615760081E-08, 1473.590260269789951, 262.5080731529990317 ) ) ;
#15571=CARTESIAN_POINT ( 'NONE',  ( -0.9017680944290000777, 1482.202343265330001, 182.1243025875980095 ) ) ;
#15577=CARTESIAN_POINT ( 'NONE',  ( 6.224176841430179685, 1407.473636843709983, 220.5349837105389668 ) ) ;
#15579=CARTESIAN_POINT ( 'NONE',  ( -2.453592884419999615E-14, 1422.045703177329870, 122.9811571859980006 ) ) ;
#15581=CARTESIAN_POINT ( 'NONE',  ( -27.01426103600620365, 1451.969699918799961, 134.9176446824099855 ) ) ;
#15583=CARTESIAN_POINT ( 'NONE',  ( 27.84455140360000058, 1437.266142704849926, 231.9094040490980149 ) ) ;
#15584=CARTESIAN_POINT ( 'NONE',  ( -3.465864926880000141, 1452.704890687129819, 183.2873751387980121 ) ) ;
#15587=CARTESIAN_POINT ( 'NONE',  ( -19.74442643839703138, 1455.875379727006475, 227.8590200339708929 ) ) ;
#15589=CARTESIAN_POINT ( 'NONE',  ( -13.44062186829930106, 1452.443703529229879, 148.8745159939319933 ) ) ;
#15592=CARTESIAN_POINT ( 'NONE',  ( -5.360343714066329923, 1422.242870833739971, 144.1500373561570143 ) ) ;
#15594=CARTESIAN_POINT ( 'NONE',  ( 13.40016148240000149, 1419.519095471729997, 228.7855739235980082 ) ) ;
#15595=CARTESIAN_POINT ( 'NONE',  ( -3.303457341579222550, 1448.967173816104150, 184.7286116801498395 ) ) ;
#15599=CARTESIAN_POINT ( 'NONE',  ( -23.70979485039999801, 1410.153424641430092, 209.4799370654980066 ) ) ;
#15603=CARTESIAN_POINT ( 'NONE',  ( -45.59505516556443183, 1438.873040481220869, 266.1907254621848438 ) ) ;
#15604=CARTESIAN_POINT ( 'NONE',  ( -2.491473724000000001, 1498.351190470029906, 236.5406736864979962 ) ) ;
#15605=CARTESIAN_POINT ( 'NONE',  ( -18.88570507609999893, 1415.855488934629875, 223.6420118195979967 ) ) ;
#15607=EDGE_CURVE ( 'NONE', #93915, #69834, #83378, .T. ) ;
#15608=CARTESIAN_POINT ( 'NONE',  ( 45.72295278579319699, 1446.162187926870047, 266.9864112351669974 ) ) ;
#15610=CARTESIAN_POINT ( 'NONE',  ( -0.02429775703179999635, 1420.196383118029871, 183.9091808095979843 ) ) ;
#15612=ORIENTED_EDGE ( 'NONE', *, *, #3058, .T. ) ;
#15613=CARTESIAN_POINT ( 'NONE',  ( -11.32027785699999889, 1433.946929803360035, 151.5080542412979980 ) ) ;
#15616=ORIENTED_EDGE ( 'NONE', *, *, #71049, .T. ) ;
#15618=CARTESIAN_POINT ( 'NONE',  ( 26.54187722018520290, 1451.986211319630002, 134.9387109740829942 ) ) ;
#15625=CARTESIAN_POINT ( 'NONE',  ( 1.948679763128840170, 1408.981109784140017, 186.9136448737170042 ) ) ;
#15626=CARTESIAN_POINT ( 'NONE',  ( 1.586289890350000009, 1417.233044477530029, 233.5609223597980133 ) ) ;
#15627=CARTESIAN_POINT ( 'NONE',  ( -18.58256518043385341, 1424.379116010960161, 224.8999308456852191 ) ) ;
#15628=CARTESIAN_POINT ( 'NONE',  ( 3.869327377972110682, 1441.524549520183427, 170.5363237134393160 ) ) ;
#15630=CARTESIAN_POINT ( 'NONE',  ( 2.446787376320000096, 1432.353341358199941, 150.2884730787980061 ) ) ;
#15632=CARTESIAN_POINT ( 'NONE',  ( 12.58433072604259984, 1415.426207913209964, 221.2617180145470002 ) ) ;
#15633=CARTESIAN_POINT ( 'NONE',  ( 11.54407487136669985, 1432.339775672029873, 151.1365564868350191 ) ) ;
#15634=CIRCLE ( 'NONE', #28227, 2.000010703461589490 ) ;
#15640=CARTESIAN_POINT ( 'NONE',  ( -1.633469776390000128, 1432.353341358199941, 150.3624711946980028 ) ) ;
#15643=CARTESIAN_POINT ( 'NONE',  ( 14.73695825029999895, 1462.639194746130215, 255.3819207682979595 ) ) ;
#15644=CARTESIAN_POINT ( 'NONE',  ( 12.37273845029059949, 1415.932840154009909, 196.2621238876739937 ) ) ;
#15645=CARTESIAN_POINT ( 'NONE',  ( 0.2550773510242848041, 1467.133396122514569, 235.6299148654997282 ) ) ;
#15648=CARTESIAN_POINT ( 'NONE',  ( -18.36047073010000119, 1486.213210630329968, 188.6962080947980098 ) ) ;
#15650=CARTESIAN_POINT ( 'NONE',  ( -17.39555449230000050, 1409.685578510729783, 224.7181607083980168 ) ) ;
#15652=CARTESIAN_POINT ( 'NONE',  ( 23.95220588820000174, 1410.918936072130236, 210.1545993587979808 ) ) ;
#15655=CARTESIAN_POINT ( 'NONE',  ( -3.340600809453960203E-09, 1406.914525921759832, 196.1218459609590070 ) ) ;
#15656=DIRECTION ( 'NONE',  ( -4.343610028670000616E-15, 1.498801083240000065E-15, -1.000000000000000000 ) ) ;
#15659=CARTESIAN_POINT ( 'NONE',  ( -3.877169465260000170, 1415.932617990029939, 227.1226588283979879 ) ) ;
#15661=CARTESIAN_POINT ( 'NONE',  ( 0.2055174958574400024, 1459.873963670999956, 182.9584848020919878 ) ) ;
#15663=ORIENTED_EDGE ( 'NONE', *, *, #66624, .T. ) ;
#15664=CARTESIAN_POINT ( 'NONE',  ( -20.24673233129999872, 1444.324653571829913, 162.1129423953979938 ) ) ;
#15665=CARTESIAN_POINT ( 'NONE',  ( -33.82146843645519851, 1444.740067931809335, 154.8031860135564273 ) ) ;
#15666=CARTESIAN_POINT ( 'NONE',  ( 13.50070407659999994, 1434.968958018969943, 149.9809230249979919 ) ) ;
#15667=CARTESIAN_POINT ( 'NONE',  ( -41.66155871503109864, 1443.633333536269902, 134.0999999981970063 ) ) ;
#15673=DIRECTION ( 'NONE',  ( 0.000000000000000000, 1.000000000000000000, 0.000000000000000000 ) ) ;
#15674=B_SPLINE_CURVE_WITH_KNOTS ( 'NONE', 3,
 ( #81278, #56099, #57770, #91349, #92986, #6229, #91889, #6773, #14629, #75115, #5698, #57222, #41501, #25214, #67814, #101928, #23018 ),
 .UNSPECIFIED., .F., .F.,
 ( 4, 2, 2, 1, 1, 1, 1, 1, 2, 2, 4 ),
 ( 0.000000000000000000, 0.2499999999998790412, 0.4999999999997580824, 0.6249999999997010169, 0.6874999999996719291, 0.7187499999996564970, 0.7343749999996487254, 0.7421874999996495026, 0.7460937499996537214, 0.7499999999996578293, 1.000000000000000000 ),
 .UNSPECIFIED. ) ;
#15676=CIRCLE ( 'NONE', #17531, 2.000000175757499665 ) ;
#15677=DIRECTION ( 'NONE',  ( 0.000000000000000000, -0.7041802892087485333, -0.7100212111549085714 ) ) ;
#15681=CARTESIAN_POINT ( 'NONE',  ( 12.74111629471100038, 1416.830086716310007, 196.2606222955850228 ) ) ;
#15684=CARTESIAN_POINT ( 'NONE',  ( -33.30821264389999925, 1450.888620760030108, 136.1896499959979678 ) ) ;
#15685=CARTESIAN_POINT ( 'NONE',  ( 16.68498601116327151, 1442.773887286369018, 162.0933193695679222 ) ) ;
#15686=CARTESIAN_POINT ( 'NONE',  ( 3.947090874974254149, 1427.113278099589934, 137.0999999980980704 ) ) ;
#15690=CARTESIAN_POINT ( 'NONE',  ( -18.08558846253097485, 1410.907777525342681, 224.6300668642674907 ) ) ;
#15692=CARTESIAN_POINT ( 'NONE',  ( -11.33192158569999819, 1414.988017870030035, 195.9133765299980041 ) ) ;
#15694=CARTESIAN_POINT ( 'NONE',  ( 2.500000000000000000, 1425.929641636930000, 126.8043280305979863 ) ) ;
#15696=ADVANCED_FACE ( 'NONE', ( #59770 ), #27377, .F. ) ;
#15697=CARTESIAN_POINT ( 'NONE',  ( -16.57130798100000035, 1422.287820404829972, 227.1266126762980093 ) ) ;
#15701=CARTESIAN_POINT ( 'NONE',  ( 9.668109322589998555, 1408.913060387329779, 224.6723891271980165 ) ) ;
#15702=AXIS2_PLACEMENT_3D ( 'NONE', #54032, #42975, #62996 ) ;
#15706=CARTESIAN_POINT ( 'NONE',  ( 2.705316712519999722, 1447.083576631230017, 165.9366036590980116 ) ) ;
#15709=CARTESIAN_POINT ( 'NONE',  ( -16.68599179819999989, 1461.099982565929849, 230.2790296985980092 ) ) ;
#15711=ORIENTED_EDGE ( 'NONE', *, *, #38378, .F. ) ;
#15717=CARTESIAN_POINT ( 'NONE',  ( 1.470421131539999982, 1428.420680932830237, 91.31218443469779800 ) ) ;
#15718=CARTESIAN_POINT ( 'NONE',  ( 15.87459988598749838, 1409.570044024510025, 192.3777976961339959 ) ) ;
#15720=CARTESIAN_POINT ( 'NONE',  ( 41.66134369672110438, 1443.796896187320044, 135.6885329911860083 ) ) ;
#15721=CARTESIAN_POINT ( 'NONE',  ( -13.01666274260000122, 1409.302079604029814, 262.4458674292980049 ) ) ;
#15723=CARTESIAN_POINT ( 'NONE',  ( 15.67195723210528691, 1461.477347166320897, 229.6037306798920383 ) ) ;
#15724=CARTESIAN_POINT ( 'NONE',  ( 39.75236484272360116, 1448.901857782450179, 134.0999999981239910 ) ) ;
#15725=CARTESIAN_POINT ( 'NONE',  ( 7.105427357599999217E-15, 1410.913060387329779, 146.1721969590979882 ) ) ;
#15726=ORIENTED_EDGE ( 'NONE', *, *, #52831, .F. ) ;
#15734=AXIS2_PLACEMENT_3D ( 'NONE', #58267, #50427, #92389 ) ;
#15738=CARTESIAN_POINT ( 'NONE',  ( 42.60628462810000627, 1443.705283505709758, 134.0999992373979808 ) ) ;
#15747=CARTESIAN_POINT ( 'NONE',  ( 11.76561647296150070, 1427.008901819209996, 146.1381330989469802 ) ) ;
#15749=VERTEX_POINT ( 'NONE', #79325 ) ;
#15751=EDGE_CURVE ( 'NONE', #93599, #94948, #52477, .T. ) ;
#15752=CARTESIAN_POINT ( 'NONE',  ( -11.07540131138789974, 1432.346177062760034, 151.6859278047610076 ) ) ;
#15755=CARTESIAN_POINT ( 'NONE',  ( -13.16128509840000049, 1426.050756123429892, 222.2185317868979837 ) ) ;
#15760=CARTESIAN_POINT ( 'NONE',  ( -16.63654591560000284, 1507.631725828329991, 224.7122666342980040 ) ) ;
#15761=CARTESIAN_POINT ( 'NONE',  ( 16.23843642359999606, 1460.007519691929929, 229.4167189755979734 ) ) ;
#15762=DIRECTION ( 'NONE',  ( 0.7067700363771036720, 0.03085824620770448445, 0.7067700363771035610 ) ) ;
#15763=PLANE ( 'NONE',  #15124 ) ;
#15766=VERTEX_POINT ( 'NONE', #2636 ) ;
#15767=DIRECTION ( 'NONE',  ( 0.000000000000000000, -1.000000000000000000, 0.000000000000000000 ) ) ;
#15774=CARTESIAN_POINT ( 'NONE',  ( 0.7130140427719999785, 1416.844618642330033, 190.3244982829980074 ) ) ;
#15775=CARTESIAN_POINT ( 'NONE',  ( -15.57416828428110023, 1507.336004463039899, 192.5523032500569798 ) ) ;
#15776=CARTESIAN_POINT ( 'NONE',  ( -11.21188824190000055, 1426.389936183530153, 148.4979915517980089 ) ) ;
#15779=CARTESIAN_POINT ( 'NONE',  ( 6.356853389496330387, 1423.329118960190044, 150.6733088057929990 ) ) ;
#15780=FACE_OUTER_BOUND ( 'NONE', #55730, .T. ) ;
#15781=CARTESIAN_POINT ( 'NONE',  ( 0.2730630983163809811, 1490.297625679229895, 187.5574216619969832 ) ) ;
#15782=EDGE_CURVE ( 'NONE', #65683, #52693, #45741, .T. ) ;
#15783=CARTESIAN_POINT ( 'NONE',  ( -19.34905394389999955, 1482.734125384130039, 228.2119762798980105 ) ) ;
#15785=CARTESIAN_POINT ( 'NONE',  ( -8.540055685515531181, 1393.051435267420175, 234.7075627498410029 ) ) ;
#15786=ORIENTED_EDGE ( 'NONE', *, *, #32901, .T. ) ;
#15789=CARTESIAN_POINT ( 'NONE',  ( 12.52700422740000086, 1408.033343574530136, 269.6003762864979763 ) ) ;
#15790=CARTESIAN_POINT ( 'NONE',  ( -0.0001187281342228439996, 1508.967929526819944, 179.3767679645770272 ) ) ;
#15791=CARTESIAN_POINT ( 'NONE',  ( 25.15310117689999814, 1469.151800109529859, 206.3831926792579736 ) ) ;
#15793=CARTESIAN_POINT ( 'NONE',  ( 3.938313870213109524, 1506.361927106564735, 230.7614585987053886 ) ) ;
#15795=FACE_OUTER_BOUND ( 'NONE', #17942, .T. ) ;
#15798=CARTESIAN_POINT ( 'NONE',  ( -13.37869130550000030, 1446.597787909739964, 188.1529836615980003 ) ) ;
#15799=CARTESIAN_POINT ( 'NONE',  ( -20.46339790889999932, 1475.513060387329915, 212.9932575586580015 ) ) ;
#15802=CARTESIAN_POINT ( 'NONE',  ( 1.464172579227420057, 1491.938057517099878, 181.7751837965830077 ) ) ;
#15803=CARTESIAN_POINT ( 'NONE',  ( -6.215408291180000155, 1427.423536210930024, 214.3676144197379756 ) ) ;
#15805=DIRECTION ( 'NONE',  ( 0.000000000000000000, 0.000000000000000000, 1.000000000000000000 ) ) ;
#15806=CARTESIAN_POINT ( 'NONE',  ( -3.427369262309999609, 1475.739996263529974, 266.9564229772980752 ) ) ;
#15809=CARTESIAN_POINT ( 'NONE',  ( -22.01225108839999933, 1509.713483275730141, 189.1785030504979943 ) ) ;
#15811=CARTESIAN_POINT ( 'NONE',  ( -3.527569048119670203, 1486.518325592330029, 181.8541486797999767 ) ) ;
#15814=CARTESIAN_POINT ( 'NONE',  ( -3.282394052629999948, 1438.199601172570055, 155.5836490844979778 ) ) ;
#15817=CARTESIAN_POINT ( 'NONE',  ( -14.28127427822060014, 1474.301216932419948, 223.9347614794640151 ) ) ;
#15818=ADVANCED_FACE ( 'NONE', ( #3192 ), #80174, .F. ) ;
#15819=CARTESIAN_POINT ( 'NONE',  ( -17.84692650809999748, 1410.032952996529957, 195.3924047753979778 ) ) ;
#15820=EDGE_CURVE ( 'NONE', #31171, #29814, #25269, .T. ) ;
#15825=ORIENTED_EDGE ( 'NONE', *, *, #64415, .F. ) ;
#15826=FACE_OUTER_BOUND ( 'NONE', #58034, .T. ) ;
#15831=CARTESIAN_POINT ( 'NONE',  ( 11.73701142390000030, 1426.696005485330033, 144.1689090389980095 ) ) ;
#15833=CARTESIAN_POINT ( 'NONE',  ( 11.70306882791220104, 1426.718062415309987, 141.7392483422370049 ) ) ;
#15837=EDGE_CURVE ( 'NONE', #101369, #35225, #43359, .T. ) ;
#15840=DIRECTION ( 'NONE',  ( 1.000000000000000000, 0.000000000000000000, 0.000000000000000000 ) ) ;
#15841=CARTESIAN_POINT ( 'NONE',  ( -12.84729496320930409, 1398.293704436309099, 206.6733356016319476 ) ) ;
#15843=DIRECTION ( 'NONE',  ( 0.000000000000000000, -0.4134839022732319513, 0.9105114291215131717 ) ) ;
#15847=ORIENTED_EDGE ( 'NONE', *, *, #86062, .T. ) ;
#15850=CARTESIAN_POINT ( 'NONE',  ( 11.99679312889339933, 1433.670206490089868, 149.8488618923190359 ) ) ;
#15851=CARTESIAN_POINT ( 'NONE',  ( -2.680633533590000006, 1397.680629565529898, 222.1367961445980086 ) ) ;
#15854=CARTESIAN_POINT ( 'NONE',  ( -26.80004305949999832, 1509.848938513930079, 198.9467878708979924 ) ) ;
#15858=CARTESIAN_POINT ( 'NONE',  ( 19.99034456412450211, 1507.818693454599952, 229.1208657279370016 ) ) ;
#15859=ADVANCED_FACE ( 'NONE', ( #89370 ), #76424, .F. ) ;
#15860=CARTESIAN_POINT ( 'NONE',  ( 2.856234944690000166, 1468.704783001229771, 183.0951156081980002 ) ) ;
#15861=CARTESIAN_POINT ( 'NONE',  ( -9.382530293249999431, 1414.913060387329779, 195.0067469954979913 ) ) ;
#15864=B_SPLINE_SURFACE_WITH_KNOTS ( 'NONE', 5, 5, ( 
 ( #80464, #64227, #22714, #88858, #63684, #46878 ),
 ( #107852, #22166, #89408, #46334, #37910, #30599 ),
 ( #91045, #63147, #31141, #56913, #72615, #97248 ),
 ( #72092, #14333, #82096, #97795, #21072, #12696 ),
 ( #64787, #55828, #38984, #73161, #4312, #106746 ),
 ( #20524, #48523, #98897, #47414, #81005, #13223 ),
 ( #3228, #4837, #13771, #37355, #71555, #56364 ),
 ( #90496, #47955, #105675, #58022, #49074, #93785 ),
 ( #74280, #15976, #108967, #32793, #40650, #110062 ) ),
 .UNSPECIFIED., .F., .F., .F.,
 ( 6, 3, 6 ),
 ( 6, 6 ),
 ( 134.5636516019999931, 157.0233722590000127, 167.1797832720000088 ),
 ( -2.775557561569999727E-17, 2.000000000000000000 ),
 .UNSPECIFIED. ) ;
#15867=CARTESIAN_POINT ( 'NONE',  ( 14.45750538832999865, 1416.828039266780024, 196.8520486936070029 ) ) ;
#15868=CARTESIAN_POINT ( 'NONE',  ( 11.57344360939999994, 1432.104224190049990, 151.1935562510979878 ) ) ;
#15869=CARTESIAN_POINT ( 'NONE',  ( 8.342231075979542609, 1509.204540318783074, 181.0076993523580313 ) ) ;
#15871=CARTESIAN_POINT ( 'NONE',  ( 13.22834362140159925, 1435.940882500919997, 150.6028531436949720 ) ) ;
#15872=ORIENTED_EDGE ( 'NONE', *, *, #70919, .F. ) ;
#15873=EDGE_CURVE ( 'NONE', #79125, #9730, #90121, .T. ) ;
#15875=CARTESIAN_POINT ( 'NONE',  ( 13.18758814857034167, 1444.720776282646966, 169.3929990596218431 ) ) ;
#15876=CARTESIAN_POINT ( 'NONE',  ( -12.55989168380000187, 1462.260622135130006, 231.0244227316980243 ) ) ;
#15885=CARTESIAN_POINT ( 'NONE',  ( 13.85929416875070075, 1410.325639211550197, 191.1496550842730073 ) ) ;
#15887=AXIS2_PLACEMENT_3D ( 'NONE', #57011, #37992, #40186 ) ;
#15888=B_SPLINE_CURVE_WITH_KNOTS ( 'NONE', 3,
 ( #89016, #97961, #2841, #72790, #3945, #96330, #36965, #19608, #12308, #71156, #97426, #105279, #62770, #11767 ),
 .UNSPECIFIED., .F., .F.,
 ( 4, 2, 2, 2, 2, 2, 4 ),
 ( 0.000000000000000000, 0.1249999999999999445, 0.2499999999999998890, 0.3749999999999998335, 0.4999999999999997780, 0.7499999999999998890, 1.000000000000000000 ),
 .UNSPECIFIED. ) ;
#15893=CARTESIAN_POINT ( 'NONE',  ( -18.85941459980000445, 1507.948893464629919, 229.7112672258979842 ) ) ;
#15894=CARTESIAN_POINT ( 'NONE',  ( -12.27459264500000025, 1410.274824613030205, 189.3792765279980017 ) ) ;
#15896=CARTESIAN_POINT ( 'NONE',  ( -0.5259141656838780543, 1414.913057855109855, 225.6201700896280045 ) ) ;
#15898=CARTESIAN_POINT ( 'NONE',  ( 24.55711019350000157, 1439.571810943109995, 212.6863966501479979 ) ) ;
#15901=CARTESIAN_POINT ( 'NONE',  ( 0.003700947952980240298, 1466.041018871260121, 235.8553854568179986 ) ) ;
#15903=CARTESIAN_POINT ( 'NONE',  ( 7.320732157969690235, 1410.234431376039993, 270.0738234895199525 ) ) ;
#15905=CARTESIAN_POINT ( 'NONE',  ( 24.11306831329999767, 1410.846617931330002, 209.3308953604909846 ) ) ;
#15906=EDGE_CURVE ( 'NONE', #109266, #94371, #68743, .T. ) ;
#15907=CARTESIAN_POINT ( 'NONE',  ( 24.07913373210075747, 1410.980207854583796, 209.6302519821946930 ) ) ;
#15911=CARTESIAN_POINT ( 'NONE',  ( -2.552678418909050340, 1448.464024222542548, 154.6753740974435232 ) ) ;
#15918=CARTESIAN_POINT ( 'NONE',  ( 6.814843616780000168, 1474.725755692929852, 264.8987716706979541 ) ) ;
#15928=CARTESIAN_POINT ( 'NONE',  ( 10.75213062065016345, 1424.456471968840106, 137.8384151154668018 ) ) ;
#15929=ORIENTED_EDGE ( 'NONE', *, *, #42540, .T. ) ;
#15933=CARTESIAN_POINT ( 'NONE',  ( 12.80114668729999927, 1422.763074512629828, 223.5079147161980018 ) ) ;
#15937=CARTESIAN_POINT ( 'NONE',  ( 0.000000000000000000, 1408.913060387329779, 226.8598803041980148 ) ) ;
#15938=CARTESIAN_POINT ( 'NONE',  ( 27.07064927763860140, 1436.337874274649948, 136.7243984374310060 ) ) ;
#15941=ADVANCED_FACE ( 'NONE', ( #95441 ), #63230, .F. ) ;
#15943=CARTESIAN_POINT ( 'NONE',  ( -23.63778291159999867, 1435.985561032100122, 212.2556568964579924 ) ) ;
#15944=CARTESIAN_POINT ( 'NONE',  ( -41.97830496582596282, 1454.330232234711730, 269.0763006382472895 ) ) ;
#15946=CARTESIAN_POINT ( 'NONE',  ( 12.20572978030000044, 1508.837378189130050, 184.1963009972980103 ) ) ;
#15948=CARTESIAN_POINT ( 'NONE',  ( -37.97313029066103240, 1453.984394254719291, 269.5760461896424545 ) ) ;
#15951=EDGE_CURVE ( 'NONE', #32742, #44146, #37986, .T. ) ;
#15952=CARTESIAN_POINT ( 'NONE',  ( -29.77764972417399747, 1414.913285559889800, 269.3620624046142780 ) ) ;
#15954=CARTESIAN_POINT ( 'NONE',  ( 14.38095606289810036, 1427.056691244839840, 190.6162741030670134 ) ) ;
#15956=CARTESIAN_POINT ( 'NONE',  ( 24.24036431055581886, 1452.066555927197214, 137.1576988608119336 ) ) ;
#15959=CARTESIAN_POINT ( 'NONE',  ( -1.186412362116890051, 1486.884137111580230, 199.7737105367970116 ) ) ;
#15960=CARTESIAN_POINT ( 'NONE',  ( -7.862669792100661859, 1451.394032558670915, 152.9856753053126965 ) ) ;
#15962=CARTESIAN_POINT ( 'NONE',  ( -18.02416168173120070, 1416.221314539589912, 209.1763259735849942 ) ) ;
#15963=CARTESIAN_POINT ( 'NONE',  ( 24.06727922369999817, 1435.337950089560081, 136.6674132985980066 ) ) ;
#15965=CARTESIAN_POINT ( 'NONE',  ( -13.13272715366738908, 1443.052901350239608, 169.4010147687362178 ) ) ;
#15967=CARTESIAN_POINT ( 'NONE',  ( 0.7266101759286229811, 1414.971717244350202, 192.1881877811019876 ) ) ;
#15969=CARTESIAN_POINT ( 'NONE',  ( -0.2331143941452460122, 1408.921200921389982, 231.7611568498559791 ) ) ;
#15972=CARTESIAN_POINT ( 'NONE',  ( 17.48265144437409901, 1415.426207913209964, 208.8075662200119780 ) ) ;
#15974=CARTESIAN_POINT ( 'NONE',  ( 41.23894881901300380, 1434.940505294187687, 269.6330775959622201 ) ) ;
#15975=CARTESIAN_POINT ( 'NONE',  ( -24.58004528950000278, 1449.381385745619809, 225.2788513490980051 ) ) ;
#15976=CARTESIAN_POINT ( 'NONE',  ( -20.23498361140000057, 1507.901949647030051, 189.1924027903980061 ) ) ;
#15977=CARTESIAN_POINT ( 'NONE',  ( -11.08092061109999982, 1433.166019614319794, 151.6958383069980130 ) ) ;
#15978=EDGE_CURVE ( 'NONE', #68958, #54399, #44516, .T. ) ;
#15980=CARTESIAN_POINT ( 'NONE',  ( -2.774956468634210083, 1419.962269928060323, 186.1082814807396630 ) ) ;
#15982=CARTESIAN_POINT ( 'NONE',  ( -24.40197519060000175, 1440.339844854569947, 212.0083896061380244 ) ) ;
#15984=CARTESIAN_POINT ( 'NONE',  ( -2.935740620858350081, 1409.954266029739983, 186.6342734442710025 ) ) ;
#15987=CARTESIAN_POINT ( 'NONE',  ( -20.87684431077013159, 1509.759617029159699, 230.6676771160481394 ) ) ;
#15991=CARTESIAN_POINT ( 'NONE',  ( -11.79841937739680091, 1428.159348747910144, 148.1013020209979913 ) ) ;
#15993=CARTESIAN_POINT ( 'NONE',  ( -6.470863364639999560, 1473.558147035430238, 270.2848116644980223 ) ) ;
#15994=CARTESIAN_POINT ( 'NONE',  ( 13.18025012471355240, 1434.856279462562952, 146.8601961898365005 ) ) ;
#15996=VECTOR ( 'NONE', #75789, 1000.000000000000227 ) ;
#15997=FACE_OUTER_BOUND ( 'NONE', #16008, .T. ) ;
#16000=CARTESIAN_POINT ( 'NONE',  ( -18.82191891289999930, 1431.113060387329824, 204.7612636155780024 ) ) ;
#16003=CARTESIAN_POINT ( 'NONE',  ( -8.335204523141790389, 1406.805845115979992, 269.2693966864819686 ) ) ;
#16004=CARTESIAN_POINT ( 'NONE',  ( -13.66554182117469907, 1436.203183890759874, 150.4225340564210001 ) ) ;
#16008=EDGE_LOOP ( 'NONE', ( #60789, #45996, #45820, #103863, #30593 ) ) ;
#16009=ORIENTED_EDGE ( 'NONE', *, *, #25237, .F. ) ;
#16015=CARTESIAN_POINT ( 'NONE',  ( -18.30299290700000014, 1485.488320381530002, 189.0823417877979864 ) ) ;
#16017=EDGE_LOOP ( 'NONE', ( #50211, #81905, #71994, #108858 ) ) ;
#16022=B_SPLINE_SURFACE_WITH_KNOTS ( 'NONE', 5, 5, ( 
 ( #56293, #73659, #13700, #5328, #74754, #107791 ),
 ( #108891, #32184, #99368, #48458, #23217, #66368 ),
 ( #57955, #57417, #22641, #56847, #14267, #74214 ),
 ( #91543, #14820, #92088, #15365, #8075, #16451 ),
 ( #101023, #102132, #94283, #75849, #43363, #9740 ),
 ( #102667, #101570, #59603, #50107, #93720, #77510 ),
 ( #109999, #17560, #51762, #34937, #34394, #68569 ),
 ( #42799, #50648, #33276, #52327, #76959, #110545 ),
 ( #18129, #69124, #33833, #43906, #109455, #85896 ) ),
 .UNSPECIFIED., .F., .F., .F.,
 ( 6, 3, 6 ),
 ( 6, 6 ),
 ( 6.548035129179999636, 9.290526163740000953, 11.10277561180000028 ),
 ( 0.000000000000000000, 2.000000000000000000 ),
 .UNSPECIFIED. ) ;
#16023=CARTESIAN_POINT ( 'NONE',  ( 1.455000209906389896, 1507.073729425429974, 236.7651043255590082 ) ) ;
#16029=ORIENTED_EDGE ( 'NONE', *, *, #91939, .F. ) ;
#16030=CARTESIAN_POINT ( 'NONE',  ( -25.82127556856010031, 1449.911323258540051, 209.1126152976609944 ) ) ;
#16031=CARTESIAN_POINT ( 'NONE',  ( 28.24200347700000080, 1508.135538548330260, 209.4469796410679976 ) ) ;
#16034=CARTESIAN_POINT ( 'NONE',  ( -13.21274905972310165, 1436.080685154540106, 150.6465363514350031 ) ) ;
#16035=CARTESIAN_POINT ( 'NONE',  ( -24.40357955099999998, 1441.574771106910021, 212.0768376842780185 ) ) ;
#16040=CARTESIAN_POINT ( 'NONE',  ( -14.29468279409999987, 1410.759725306329983, 226.8458938957979854 ) ) ;
#16041=CARTESIAN_POINT ( 'NONE',  ( 3.711480272509555256, 1440.856594891422901, 156.5043989337177379 ) ) ;
#16044=CARTESIAN_POINT ( 'NONE',  ( -2.155272317154649730, 1451.949265150150040, 184.4961430247039971 ) ) ;
#16046=CARTESIAN_POINT ( 'NONE',  ( -20.87663001988034139, 1455.029843775830841, 223.4912394292003341 ) ) ;
#16049=CARTESIAN_POINT ( 'NONE',  ( 12.76237656848210023, 1434.657230989279924, 149.5328040805229932 ) ) ;
#16050=CARTESIAN_POINT ( 'NONE',  ( -4.170414335751749135, 1441.567394449320091, 183.8415942696151433 ) ) ;
#16052=CARTESIAN_POINT ( 'NONE',  ( 24.77519968700000064, 1452.047894330230065, 135.6623939816980169 ) ) ;
#16055=CARTESIAN_POINT ( 'NONE',  ( 4.221769150835829265, 1441.602571462190099, 168.1843695343990248 ) ) ;
#16058=CARTESIAN_POINT ( 'NONE',  ( 36.40062690906153620, 1436.005110274238632, 135.0217588575150955 ) ) ;
#16061=ORIENTED_EDGE ( 'NONE', *, *, #10083, .T. ) ;
#16062=CARTESIAN_POINT ( 'NONE',  ( -18.25588481898620330, 1498.276152301830052, 229.4258147717129930 ) ) ;
#16064=CARTESIAN_POINT ( 'NONE',  ( 0.9538458998259999877, 1420.753719637230006, 182.9132178711979861 ) ) ;
#16066=DIRECTION ( 'NONE',  ( 1.000000000000000000, 0.000000000000000000, 0.000000000000000000 ) ) ;
#16067=CARTESIAN_POINT ( 'NONE',  ( -1232.316865285500171, 2833.596074015639715, -9639.481875266528732 ) ) ;
#16070=AXIS2_PLACEMENT_3D ( 'NONE', #37250, #78700, #2013 ) ;
#16071=CARTESIAN_POINT ( 'NONE',  ( 17.43505318546112193, 1422.809578927221992, 226.5206943312184933 ) ) ;
#16072=CARTESIAN_POINT ( 'NONE',  ( 18.25262555440377099, 1425.320047386311671, 224.8456491439040121 ) ) ;
#16073=CARTESIAN_POINT ( 'NONE',  ( -7.435066116149999793, 1441.600846913620217, 149.7516446007980164 ) ) ;
#16077=CARTESIAN_POINT ( 'NONE',  ( 13.12320631909999946, 1422.961664926129970, 221.9290738727979999 ) ) ;
#16081=DIRECTION ( 'NONE',  ( 0.6638413684297217454, -0.7475172610820757235, 0.02307773701440622716 ) ) ;
#16089=CARTESIAN_POINT ( 'NONE',  ( 10.91400993090000071, 1451.290521646029902, 152.3073314843979915 ) ) ;
#16093=EDGE_LOOP ( 'NONE', ( #60326, #78683, #47011, #27357, #68475 ) ) ;
#16096=AXIS2_PLACEMENT_3D ( 'NONE', #30900, #109822, #67291 ) ;
#16097=B_SPLINE_SURFACE_WITH_KNOTS ( 'NONE', 5, 5, ( 
 ( #67684, #72367, #64520, #6230, #65059, #47154, #65614, #110209, #50866 ),
 ( #99172, #22454, #47701, #14630, #5133, #23019, #57223, #101792, #16668 ),
 ( #63972, #91350, #48817, #21357, #38186, #82939, #84995, #29785, #55564 ),
 ( #89689, #81279, #4596, #38730, #72904, #107045, #30331, #21903, #95075 ),
 ( #27313, #1580, #43574, #18341, #76612, #87226, #35714, #69902, #60380 ),
 ( #44131, #36267, #78266, #51412, #61494, #86665, #68246, #52532, #18892 ),
 ( #85544, #95624, #104577, #9959, #1036, #42453, #77723, #35159, #86118 ),
 ( #110764, #104018, #78835, #17217, #10516, #53088, #34054, #60947, #94501 ),
 ( #44690, #2146, #69343, #102354, #9411, #70456, #27871, #62053, #103452 ),
 ( #26758, #96178, #19453, #25637, #59829, #93950, #8840, #17774, #8290 ),
 ( #43023, #77181, #53652, #484, #34607, #68793, #102893, #26192, #51976 ),
 ( #30059, #87796, #29515, #45247, #63706, #36822, #97272, #97816, #46355 ),
 ( #11080, #62623, #4335, #37378, #63170, #106768, #79934, #20546, #21095 ),
 ( #46903, #107329, #71012, #106230, #54750, #3251, #37935, #88880, #55298 ),
 ( #89972, #81026, #81560, #45801, #96740, #89429, #12165, #79384, #38466 ) ),
 .UNSPECIFIED., .F., .F., .F.,
 ( 6, 3, 3, 3, 6 ),
 ( 6, 3, 6 ),
 ( 20.95182776320000073, 25.72519398600000073, 33.50811105449999872, 41.29102812299999670, 53.47486354659999819 ),
 ( 0.000000000000000000, 1.000000000000000000, 2.000000000000000000 ),
 .UNSPECIFIED. ) ;
#16099=ADVANCED_FACE ( 'NONE', ( #76697 ), #34145, .F. ) ;
#16100=CARTESIAN_POINT ( 'NONE',  ( -16.97531057559999823, 1409.505851295029970, 223.7086794493979767 ) ) ;
#16102=EDGE_LOOP ( 'NONE', ( #24915, #86046, #66509, #57107, #75335, #29282 ) ) ;
#16104=CARTESIAN_POINT ( 'NONE',  ( 37.47794244721399792, 1438.218164175530092, 136.5783189908810016 ) ) ;
#16111=CARTESIAN_POINT ( 'NONE',  ( -11.65606946387948462, 1435.045539906245040, 151.3529213300715242 ) ) ;
#16112=CARTESIAN_POINT ( 'NONE',  ( 18.70459388984919968, 1509.566239199539950, 186.5372755781170042 ) ) ;
#16113=CARTESIAN_POINT ( 'NONE',  ( 0.1274748778641759950, 1507.111760713879903, 180.9260797659750040 ) ) ;
#16114=CARTESIAN_POINT ( 'NONE',  ( 1.431683340829999818, 1410.342262983229830, 185.2915050568979893 ) ) ;
#16115=CARTESIAN_POINT ( 'NONE',  ( 1.716045945209999868, 1509.007693206030126, 179.5167849949980052 ) ) ;
#16116=CARTESIAN_POINT ( 'NONE',  ( -11.86629850686009924, 1432.349867577580198, 149.9824227077560010 ) ) ;
#16117=CARTESIAN_POINT ( 'NONE',  ( -3.691951647117269530, 1441.076583034890064, 158.1234524560840100 ) ) ;
#16119=EDGE_CURVE ( 'NONE', #36240, #5765, #59564, .T. ) ;
#16120=CARTESIAN_POINT ( 'NONE',  ( 11.76598824432590185, 1428.979787898590075, 145.3127963841559733 ) ) ;
#16124=CARTESIAN_POINT ( 'NONE',  ( 18.99989700328560360, 1457.426100493899867, 226.6523199981070036 ) ) ;
#16125=CARTESIAN_POINT ( 'NONE',  ( 16.53426867370000153, 1488.224675751930135, 188.8661511851979640 ) ) ;
#16127=CARTESIAN_POINT ( 'NONE',  ( 20.52035477951934084, 1436.445808972336636, 144.8704347017549594 ) ) ;
#16133=CARTESIAN_POINT ( 'NONE',  ( -46.05541984167459901, 1438.448880790329895, 266.9752125373910303 ) ) ;
#16134=CARTESIAN_POINT ( 'NONE',  ( -2.695375846180000146, 1439.665988598389958, 184.6458907360980106 ) ) ;
#16141=ADVANCED_FACE ( 'NONE', ( #17308 ), #85635, .F. ) ;
#16144=CARTESIAN_POINT ( 'NONE',  ( -27.02103266032270312, 1451.952429640200080, 135.1697984406160344 ) ) ;
#16145=VERTEX_POINT ( 'NONE', #58803 ) ;
#16146=CARTESIAN_POINT ( 'NONE',  ( 24.09667807370000148, 1426.479303835230212, 238.1639188848979813 ) ) ;
#16149=EDGE_CURVE ( 'NONE', #36359, #2313, #45920, .T. ) ;
#16151=CARTESIAN_POINT ( 'NONE',  ( -3.625385342379999987, 1422.360590018430003, 211.7205299729980084 ) ) ;
#16153=CARTESIAN_POINT ( 'NONE',  ( 29.22958591724099975, 1509.933780020319773, 206.4713313096740137 ) ) ;
#16155=VERTEX_POINT ( 'NONE', #26851 ) ;
#16157=CARTESIAN_POINT ( 'NONE',  ( 16.32987610974730330, 1422.497371498959865, 227.4665333559439944 ) ) ;
#16161=CARTESIAN_POINT ( 'NONE',  ( -22.63974427064189854, 1409.703621529829888, 209.3606225731330142 ) ) ;
#16164=CARTESIAN_POINT ( 'NONE',  ( -9.110233712619999480, 1428.462521060929930, 112.4493539157979995 ) ) ;
#16165=CARTESIAN_POINT ( 'NONE',  ( -0.9772301425810001607, 1507.642725251929960, 237.2369517814979929 ) ) ;
#16167=CARTESIAN_POINT ( 'NONE',  ( 46.23666873409530353, 1442.813199615530038, 267.5908865687479761 ) ) ;
#16169=CARTESIAN_POINT ( 'NONE',  ( -15.97230738210199696, 1420.722887419069821, 227.0315163971459924 ) ) ;
#16171=EDGE_LOOP ( 'NONE', ( #474, #41390 ) ) ;
#16172=CARTESIAN_POINT ( 'NONE',  ( 19.00569199371070539, 1457.306189793003114, 226.5295724121195065 ) ) ;
#16175=DIRECTION ( 'NONE',  ( 0.5969061220947440294, -0.8023110876747339137, 0.000000000000000000 ) ) ;
#16178=CARTESIAN_POINT ( 'NONE',  ( 26.83111240151620080, 1451.219512166529967, 136.2764200117410098 ) ) ;
#16179=B_SPLINE_SURFACE_WITH_KNOTS ( 'NONE', 5, 5, ( 
 ( #35870, #37514, #19597, #29113, #69492, #28005, #19032, #63299, #11228, #62193, #71148, #36404 ),
 ( #27451, #36951, #17928, #61634, #45929, #96320, #105271, #95765, #53233, #87375, #10669, #44835 ),
 ( #52126, #79529, #53800, #28563, #70596, #104711, #86253, #62761, #35305, #96878, #103614, #20147 ),
 ( #54344, #11759, #9544, #43714, #77865, #29656, #80623, #64390, #97953, #40262, #31307, #73883 ),
 ( #4474, #54884, #81159, #12298, #13386, #82813, #99051, #64937, #22330, #55980, #13942, #5568 ),
 ( #48132, #90103, #63842, #81698, #55432, #65490, #72783, #38603, #39719, #106369, #108011, #89563 ),
 ( #12853, #21223, #47573, #82270, #14499, #20687, #106910, #47034, #5005, #22883, #73326, #89009 ),
 ( #30198, #72242, #3937, #99600, #98510, #21778, #39152, #57093, #107461, #91218, #30756, #48689 ),
 ( #6106, #74445, #56531, #108571, #46490, #90659, #31860, #97417, #38065, #49238, #75545, #58731 ),
 ( #67146, #110780, #92868, #6661, #49786, #16146, #74993, #83361, #8857, #40814, #50350, #59304 ),
 ( #101807, #51430, #17236, #68264, #76627, #93969, #85560, #8308, #109681, #15583, #66603, #43040 ),
 ( #102371, #32957, #109142, #84475, #15038, #92312, #77197, #67698, #500, #32424, #76085, #101244 ),
 ( #93418, #110223, #42469, #7762, #34071, #83919, #50882, #66048, #7223, #100171, #33497, #85014 ),
 ( #41381, #100707, #24543, #58184, #25099, #23456, #16685, #25654, #59845, #23988, #41929, #57650 ),
 ( #91762, #13126, #18355, #94517, #106650, #35176, #87242, #69920, #87812, #18907, #53669, #89856 ) ),
 .UNSPECIFIED., .F., .F., .F.,
 ( 6, 3, 3, 3, 6 ),
 ( 6, 3, 3, 6 ),
 ( 1.933760083099999916, 17.84603210599999912, 29.17820978809999843, 40.51038747020000130, 62.31975385239999810 ),
 ( 253.0908261109999842, 295.2726304679999885, 316.3635326440000313, 337.4544348200000172 ),
 .UNSPECIFIED. ) ;
#16185=CARTESIAN_POINT ( 'NONE',  ( 10.21005717583030048, 1409.269603440459832, 190.4196895962099916 ) ) ;
#16186=CARTESIAN_POINT ( 'NONE',  ( 2.250613398900000117, 1417.526871923430008, 235.1186440458980087 ) ) ;
#16190=CARTESIAN_POINT ( 'NONE',  ( 9.251407843868516778, 1419.243067687219764, 232.8166381639402118 ) ) ;
#16193=AXIS2_PLACEMENT_3D ( 'NONE', #110218, #51987, #9970 ) ;
#16200=CARTESIAN_POINT ( 'NONE',  ( 4.367411321880000158E-15, 1433.447543843880112, 150.4377610267980003 ) ) ;
#16201=CARTESIAN_POINT ( 'NONE',  ( -21.83810666687164570, 1509.467311522997079, 191.4893092206315259 ) ) ;
#16202=CARTESIAN_POINT ( 'NONE',  ( 11.91537912909999974, 1433.481023094019747, 150.2490204454979903 ) ) ;
#16205=VECTOR ( 'NONE', #52533, 1000.000000000000000 ) ;
#16206=CARTESIAN_POINT ( 'NONE',  ( -16.42371827013585062, 1409.486589267243062, 195.5290734195434936 ) ) ;
#16209=CARTESIAN_POINT ( 'NONE',  ( -15.58089241750000120, 1485.971873082329921, 186.8153789246979954 ) ) ;
#16211=CARTESIAN_POINT ( 'NONE',  ( 13.01309781538156507, 1398.298637390604881, 208.7135361888869625 ) ) ;
#16212=CARTESIAN_POINT ( 'NONE',  ( -18.02348485499999953, 1410.905797795330045, 224.7336264866979718 ) ) ;
#16213=CARTESIAN_POINT ( 'NONE',  ( 20.29535750659999849, 1430.346966363130150, 221.2589603778980063 ) ) ;
#16221=CARTESIAN_POINT ( 'NONE',  ( 0.1855511662499469971, 1471.274342563620166, 182.4691293643950019 ) ) ;
#16222=CARTESIAN_POINT ( 'NONE',  ( 0.06979890406090000221, 1408.910622955929966, 224.1218459632979716 ) ) ;
#16223=ORIENTED_EDGE ( 'NONE', *, *, #49063, .T. ) ;
#16224=CARTESIAN_POINT ( 'NONE',  ( -17.22592482065197927, 1443.913060387330233, 162.9227486220069920 ) ) ;
#16225=CIRCLE ( 'NONE', #225, 1.500000000000001332 ) ;
#16226=CARTESIAN_POINT ( 'NONE',  ( -16.65152936259426042, 1461.099982565929849, 228.2793266355078856 ) ) ;
#16228=CARTESIAN_POINT ( 'NONE',  ( -41.21983904267550258, 1446.341078050689703, 134.0999999985669717 ) ) ;
#16237=CARTESIAN_POINT ( 'NONE',  ( 22.95227133490000071, 1507.624369720630057, 210.2367868482679967 ) ) ;
#16238=CARTESIAN_POINT ( 'NONE',  ( -44.93136599389160324, 1440.913052653349951, 269.6838063022050278 ) ) ;
#16243=ORIENTED_EDGE ( 'NONE', *, *, #105682, .F. ) ;
#16244=CARTESIAN_POINT ( 'NONE',  ( -29.81974126589999941, 1451.871786491030207, 135.2695870736979771 ) ) ;
#16245=CARTESIAN_POINT ( 'NONE',  ( 13.31970894439976583, 1443.086052842850222, 169.4013815678758306 ) ) ;
#16250=DIRECTION ( 'NONE',  ( 0.7067700477513105817, -0.03085664260695931277, -0.7067700950157954631 ) ) ;
#16255=CARTESIAN_POINT ( 'NONE',  ( 13.64529111084437574, 1409.389564452892728, 192.7393524575074082 ) ) ;
#16256=CARTESIAN_POINT ( 'NONE',  ( 14.93435719577100329, 1430.577349657391323, 220.1736567016903052 ) ) ;
#16257=CARTESIAN_POINT ( 'NONE',  ( 1.711020842750000215, 1415.875572146229842, 232.5272861542979967 ) ) ;
#16259=CARTESIAN_POINT ( 'NONE',  ( -24.02854066789229748, 1507.902906607559999, 222.3115874531950169 ) ) ;
#16263=CARTESIAN_POINT ( 'NONE',  ( 2.499999999909999993, 1447.637843966240098, 170.5315787512979853 ) ) ;
#16270=CARTESIAN_POINT ( 'NONE',  ( -18.14245636085959745, 1424.695485258009057, 227.8876350735791618 ) ) ;
#16273=CARTESIAN_POINT ( 'NONE',  ( -24.89847827690000059, 1430.363150117730129, 208.6174969999159998 ) ) ;
#16274=CARTESIAN_POINT ( 'NONE',  ( -10.15536310392529984, 1425.168171719249813, 103.9028244493299979 ) ) ;
#16275=CARTESIAN_POINT ( 'NONE',  ( 15.78263224276630083, 1409.464194525379753, 192.9576963222289976 ) ) ;
#16277=CARTESIAN_POINT ( 'NONE',  ( 36.39711325428599764, 1436.006149706799988, 135.4589782244629816 ) ) ;
#16279=CARTESIAN_POINT ( 'NONE',  ( -39.71667698630000132, 1440.913060382720005, 259.0958797466979604 ) ) ;
#16284=VERTEX_POINT ( 'NONE', #20627 ) ;
#16286=CARTESIAN_POINT ( 'NONE',  ( -18.31479797789999964, 1458.692617178530099, 227.8150927488979960 ) ) ;
#16287=ORIENTED_EDGE ( 'NONE', *, *, #101450, .T. ) ;
#16290=CARTESIAN_POINT ( 'NONE',  ( -17.41346946009999996, 1410.020394389830017, 194.0661810129979870 ) ) ;
#16291=CIRCLE ( 'NONE', #39589, 1.999999999999939826 ) ;
#16296=CARTESIAN_POINT ( 'NONE',  ( 40.71747597329999735, 1448.637563247759999, 134.0999997049979982 ) ) ;
#16297=CARTESIAN_POINT ( 'NONE',  ( -11.60004869885203682, 1426.786830457828273, 134.3786150874268799 ) ) ;
#16305=CARTESIAN_POINT ( 'NONE',  ( 11.77337650133179991, 1427.210515917729936, 146.6415292692670107 ) ) ;
#16310=CARTESIAN_POINT ( 'NONE',  ( -13.25967437340000110, 1414.983773852929744, 220.4242586887980053 ) ) ;
#16311=CARTESIAN_POINT ( 'NONE',  ( -14.82726497260570042, 1470.530551423540146, 223.5668439764989728 ) ) ;
#16315=CARTESIAN_POINT ( 'NONE',  ( -13.01583361319999810, 1416.817366565030170, 221.9085595701980083 ) ) ;
#16320=CARTESIAN_POINT ( 'NONE',  ( 22.83994680308489933, 1417.789777542400088, 206.2015004188589842 ) ) ;
#16322=CARTESIAN_POINT ( 'NONE',  ( -1.738161548016574631, 1451.890872115781576, 184.1703666583102006 ) ) ;
#16324=CARTESIAN_POINT ( 'NONE',  ( -5.220193992062974964, 1506.416684590318710, 187.7825589291392134 ) ) ;
#16330=CARTESIAN_POINT ( 'NONE',  ( -2.912453515366174805, 1484.777513947625039, 183.2264124078621705 ) ) ;
#16332=CARTESIAN_POINT ( 'NONE',  ( -11.44770140791566782, 1425.800648919538389, 139.0556806801066898 ) ) ;
#16337=CARTESIAN_POINT ( 'NONE',  ( -11.77100579110000034, 1426.695143653130117, 146.7217168237980047 ) ) ;
#16339=B_SPLINE_CURVE_WITH_KNOTS ( 'NONE', 3,
 ( #62372, #70784, #88661, #104897, #28186, #107648, #108188, #65109, #81881, #66225, #91940, #40433, #99221, #56700, #73514, #90836, #99776, #108745, #15214, #74059, #98133, #39891, #22499, #14120, #48310, #107092, #91403, #21408, #6285, #75163, #56143, #23633, #74610, #49405, #64571, #100345, #14680, #82452, #83530, #57815, #55618, #6824, #31478, #5749, #64020, #65659, #23066, #13560, #57275 ),
 .UNSPECIFIED., .F., .F.,
 ( 4, 2, 2, 2, 1, 1, 2, 2, 2, 2, 1, 1, 1, 2, 2, 2, 2, 1, 1, 1, 1, 2, 2, 2, 2, 1, 1, 2, 2, 4 ),
 ( 0.000000000000000000, 0.2499999999899412129, 0.3749999999849299992, 0.4374999999824081831, 0.4687499999812275164, 0.4843749999805378459, 0.4921874999802942630, 0.4999999999800506245, 0.6249999999766993053, 0.6874999999750367463, 0.7187499999741949752, 0.7343749999738907741, 0.7421874999738452550, 0.7460937499738223844, 0.7499999999737995138, 0.8124999999729637379, 0.8437499999725540656, 0.8593749999723369060, 0.8671874999722284372, 0.8710937499721960187, 0.8730468749726765232, 0.8740234374729166644, 0.8749999999731568057, 0.9062499999781312710, 0.9218749999807583917, 0.9296874999823528940, 0.9335937499831684638, 0.9355468749835762488, 0.9374999999839840337, 1.000000000000000000 ),
 .UNSPECIFIED. ) ;
#16343=DIRECTION ( 'NONE',  ( 1.000000000000000000, 0.000000000000000000, 0.000000000000000000 ) ) ;
#16344=CARTESIAN_POINT ( 'NONE',  ( -21.65371239889999799, 1482.726465196330082, 224.5928689438979973 ) ) ;
#16347=ORIENTED_EDGE ( 'NONE', *, *, #96276, .F. ) ;
#16349=CARTESIAN_POINT ( 'NONE',  ( 21.73145256330000308, 1410.542624686630234, 269.3317000074980001 ) ) ;
#16352=CARTESIAN_POINT ( 'NONE',  ( 19.46859404899999646, 1449.731791413250221, 192.7299627095979986 ) ) ;
#16353=CARTESIAN_POINT ( 'NONE',  ( 9.033549554615403210, 1506.660407547515661, 229.3903933438921285 ) ) ;
#16355=CARTESIAN_POINT ( 'NONE',  ( -1.772878804569999911, 1450.437861259890042, 182.6449559054979659 ) ) ;
#16358=CARTESIAN_POINT ( 'NONE',  ( -13.59250350780000005, 1443.952310951140134, 187.6074426047979955 ) ) ;
#16359=CARTESIAN_POINT ( 'NONE',  ( -18.70730727500000157, 1431.113060387329824, 209.1218459618889938 ) ) ;
#16365=CARTESIAN_POINT ( 'NONE',  ( -22.59589169830000088, 1507.700907224229923, 190.9355248029980032 ) ) ;
#16366=VECTOR ( 'NONE', #26878, 1000.000000000000114 ) ;
#16367=CARTESIAN_POINT ( 'NONE',  ( -12.58443858789999936, 1474.054838308030185, 269.4439571418980108 ) ) ;
#16370=CARTESIAN_POINT ( 'NONE',  ( -24.05485985184647646, 1444.308342016315237, 212.3257452429839987 ) ) ;
#16373=CARTESIAN_POINT ( 'NONE',  ( -9.704564366399999642, 1443.913060387330006, 153.0477571643979786 ) ) ;
#16376=CARTESIAN_POINT ( 'NONE',  ( -46.15244900134240424, 1440.913028098642371, 268.2044261680690624 ) ) ;
#16377=CARTESIAN_POINT ( 'NONE',  ( -22.86371263479999882, 1409.875940094530051, 206.1192440645280044 ) ) ;
#16382=CARTESIAN_POINT ( 'NONE',  ( 1.633469776390000128, 1432.353341358199941, 150.3624711946980028 ) ) ;
#16385=CARTESIAN_POINT ( 'NONE',  ( -29.35128565762720143, 1441.653456051720013, 137.2693278004479964 ) ) ;
#16388=CARTESIAN_POINT ( 'NONE',  ( 11.69528020852439987, 1426.723312899609937, 141.1826440969780094 ) ) ;
#16389=CARTESIAN_POINT ( 'NONE',  ( -15.76859352898596356, 1409.463696381290220, 225.2884038137482037 ) ) ;
#16390=DIRECTION ( 'NONE',  ( -1.000000000000000000, 0.000000000000000000, 0.000000000000000000 ) ) ;
#16394=PLANE ( 'NONE',  #55363 ) ;
#16395=CARTESIAN_POINT ( 'NONE',  ( -13.01602554077795304, 1398.298692311873083, 208.8134195757005500 ) ) ;
#16396=CYLINDRICAL_SURFACE ( 'NONE', #81940, 29.99999999999999645 ) ;
#16400=CARTESIAN_POINT ( 'NONE',  ( 20.53373553494599690, 1507.794785362809989, 228.2241617207620266 ) ) ;
#16402=ORIENTED_EDGE ( 'NONE', *, *, #4413, .T. ) ;
#16404=CARTESIAN_POINT ( 'NONE',  ( 11.38192139399690106, 1434.162350676260075, 151.4680933403080019 ) ) ;
#16405=CARTESIAN_POINT ( 'NONE',  ( -6.969102451020000366, 1396.156426807830030, 218.5728573129879919 ) ) ;
#16410=CARTESIAN_POINT ( 'NONE',  ( 2.370970874524634286, 1427.002265528474027, 137.0999999980979851 ) ) ;
#16411=CARTESIAN_POINT ( 'NONE',  ( 17.55317606050000023, 1419.032763066429879, 226.2188323924980011 ) ) ;
#16412=CARTESIAN_POINT ( 'NONE',  ( 14.67020375005709987, 1498.108088576179853, 231.9734902996929975 ) ) ;
#16414=CARTESIAN_POINT ( 'NONE',  ( 1.204114676109999893, 1468.707964903529955, 182.7289636863979752 ) ) ;
#16419=CARTESIAN_POINT ( 'NONE',  ( 0.9518847404210000196, 1415.296882282229944, 191.1939211731979924 ) ) ;
#16420=CARTESIAN_POINT ( 'NONE',  ( 11.28896394650000090, 1431.382221484100000, 151.4573443959979784 ) ) ;
#16422=ORIENTED_EDGE ( 'NONE', *, *, #90884, .T. ) ;
#16423=CARTESIAN_POINT ( 'NONE',  ( 13.25659408744109946, 1435.807411741510123, 150.5347871980940226 ) ) ;
#16427=CARTESIAN_POINT ( 'NONE',  ( -18.91742159790479860, 1507.874522033449921, 229.7221451244979846 ) ) ;
#16428=CARTESIAN_POINT ( 'NONE',  ( -5.248956291309999855, 1464.339271744430107, 236.4982892100979939 ) ) ;
#16433=CARTESIAN_POINT ( 'NONE',  ( 2.500000000000000000, 1448.240804457780087, 166.0721002888749922 ) ) ;
#16437=ORIENTED_EDGE ( 'NONE', *, *, #46604, .F. ) ;
#16439=CARTESIAN_POINT ( 'NONE',  ( -19.94169788180000324, 1509.369061779629874, 230.2160215658979894 ) ) ;
#16440=CARTESIAN_POINT ( 'NONE',  ( -12.98407978699999887, 1410.739677414529979, 189.6949195340980054 ) ) ;
#16442=CARTESIAN_POINT ( 'NONE',  ( -0.1558546717220200273, 1414.913057860449953, 225.5221266254029899 ) ) ;
#16443=ORIENTED_EDGE ( 'NONE', *, *, #55659, .T. ) ;
#16444=CARTESIAN_POINT ( 'NONE',  ( 20.84789745129999972, 1428.606193423530158, 221.9193905426979825 ) ) ;
#16451=CARTESIAN_POINT ( 'NONE',  ( -20.34464802829999996, 1507.870840051529967, 189.3862473984979999 ) ) ;
#16458=CARTESIAN_POINT ( 'NONE',  ( -11.41379966406813296, 1486.020606230438489, 184.4293688767625667 ) ) ;
#16461=ORIENTED_EDGE ( 'NONE', *, *, #98671, .F. ) ;
#16464=CARTESIAN_POINT ( 'NONE',  ( 41.23308670169999601, 1446.065286249370047, 261.5842860979980173 ) ) ;
#16468=CARTESIAN_POINT ( 'NONE',  ( -17.58460349159999936, 1489.029732347030176, 229.1403505218980001 ) ) ;
#16477=VECTOR ( 'NONE', #51330, 1000.000000000000000 ) ;
#16478=CARTESIAN_POINT ( 'NONE',  ( 15.47624034080000222, 1495.631162584530102, 224.0604253471979916 ) ) ;
#16479=CARTESIAN_POINT ( 'NONE',  ( 13.06218954519999897, 1425.740256908130050, 222.9850514811979849 ) ) ;
#16483=CARTESIAN_POINT ( 'NONE',  ( 25.39696813641784701, 1450.809552082115033, 137.2718642792816297 ) ) ;
#16484=CARTESIAN_POINT ( 'NONE',  ( 2.921131820879320440, 1415.930151663460038, 231.8786077272699799 ) ) ;
#16485=CARTESIAN_POINT ( 'NONE',  ( 29.70034115211240078, 1436.430129212750217, 136.6408550299620117 ) ) ;
#16487=CARTESIAN_POINT ( 'NONE',  ( -4.161595075237580765, 1448.982995846620042, 185.0801961897900298 ) ) ;
#16489=CARTESIAN_POINT ( 'NONE',  ( 8.991745348219998490, 1509.227059053930134, 181.2342631838979798 ) ) ;
#16491=ADVANCED_FACE ( 'NONE', ( #107407 ), #30141, .F. ) ;
#16495=CARTESIAN_POINT ( 'NONE',  ( -42.04388406582121007, 1427.611912910882893, 269.0746004808472662 ) ) ;
#16498=CARTESIAN_POINT ( 'NONE',  ( 14.07564986092039838, 1417.487964905419858, 190.9160242924600084 ) ) ;
#16499=CARTESIAN_POINT ( 'NONE',  ( -0.3298027038899999930, 1417.349066637030091, 235.5653369626979838 ) ) ;
#16501=CARTESIAN_POINT ( 'NONE',  ( 25.16854151965715047, 1451.224510553128539, 137.5711253996577739 ) ) ;
#16505=CARTESIAN_POINT ( 'NONE',  ( 44.13011777698019955, 1440.913039006840108, 270.2165842967739877 ) ) ;
#16506=CARTESIAN_POINT ( 'NONE',  ( -20.87972035156535355, 1450.952513135669733, 144.6011053034232248 ) ) ;
#16507=CARTESIAN_POINT ( 'NONE',  ( 24.50330256149999997, 1435.537756670989893, 137.2482190513979958 ) ) ;
#16508=CARTESIAN_POINT ( 'NONE',  ( -13.14482159525874394, 1443.063907452323292, 169.3991812976872211 ) ) ;
#16516=CARTESIAN_POINT ( 'NONE',  ( 42.06232107555830169, 1440.913060387330006, 269.6487541170399709 ) ) ;
#16517=CARTESIAN_POINT ( 'NONE',  ( -12.01188880439999984, 1460.226730015830071, 225.2520635090980079 ) ) ;
#16519=CARTESIAN_POINT ( 'NONE',  ( -11.46138297819999963, 1433.011133141609889, 151.3008369595980014 ) ) ;
#16521=CARTESIAN_POINT ( 'NONE',  ( -2.911024527881161283, 1419.547881642413813, 186.2020241882692915 ) ) ;
#16523=CARTESIAN_POINT ( 'NONE',  ( -24.60027558000000170, 1439.385484703360135, 210.6880631153979664 ) ) ;
#16525=CARTESIAN_POINT ( 'NONE',  ( 2.175561048050000057, 1450.072456872719840, 182.0601473783979998 ) ) ;
#16527=CARTESIAN_POINT ( 'NONE',  ( -28.81191669830696611, 1510.030278085835562, 217.4830671067354899 ) ) ;
#16528=CARTESIAN_POINT ( 'NONE',  ( -2.798875629058170013E-09, 1414.961829792250001, 244.5380620272480030 ) ) ;
#16529=ORIENTED_EDGE ( 'NONE', *, *, #94649, .T. ) ;
#16531=CARTESIAN_POINT ( 'NONE',  ( -11.78013554155059950, 1427.423339285529892, 147.0626577189019883 ) ) ;
#16533=CARTESIAN_POINT ( 'NONE',  ( -4.188706515999999880, 1472.474584819730126, 270.3708462686980170 ) ) ;
#16536=CARTESIAN_POINT ( 'NONE',  ( 17.35500899530000041, 1519.913060387329779, 193.1522642759980215 ) ) ;
#16540=CARTESIAN_POINT ( 'NONE',  ( -15.05358279999999915, 1410.831827720429828, 226.7261506157979909 ) ) ;
#16541=CARTESIAN_POINT ( 'NONE',  ( -10.66017895455560094, 1406.634972685779985, 267.8057047216510114 ) ) ;
#16542=CARTESIAN_POINT ( 'NONE',  ( -14.48276039151240013, 1435.993670758189865, 149.8592331176449761 ) ) ;
#16543=ORIENTED_EDGE ( 'NONE', *, *, #68643, .F. ) ;
#16545=CARTESIAN_POINT ( 'NONE',  ( 14.41410989250000085, 1444.046959656890067, 189.7051000925980020 ) ) ;
#16547=EDGE_LOOP ( 'NONE', ( #65930, #18094, #116, #39249, #109308, #51984 ) ) ;
#16548=EDGE_CURVE ( 'NONE', #59443, #52693, #79238, .T. ) ;
#16549=CARTESIAN_POINT ( 'NONE',  ( 4.948917002315981861, 1423.300699232361467, 184.2784904492603744 ) ) ;
#16552=CARTESIAN_POINT ( 'NONE',  ( -6.487916422619999679, 1485.477811444930012, 183.8195409892980194 ) ) ;
#16553=FACE_OUTER_BOUND ( 'NONE', #41727, .T. ) ;
#16557=EDGE_CURVE ( 'NONE', #77352, #98841, #75282, .T. ) ;
#16558=CARTESIAN_POINT ( 'NONE',  ( -26.35475474280000086, 1507.985742568630030, 201.5462048709279941 ) ) ;
#16561=CARTESIAN_POINT ( 'NONE',  ( -1.299927615229999889, 1406.964219534829908, 196.1218459552979994 ) ) ;
#16566=CARTESIAN_POINT ( 'NONE',  ( 24.29269244049999799, 1508.123907550730110, 221.3514521437980136 ) ) ;
#16569=CARTESIAN_POINT ( 'NONE',  ( -12.96423123134679933, 1435.988822720060170, 150.7593588700239877 ) ) ;
#16573=B_SPLINE_CURVE_WITH_KNOTS ( 'NONE', 5,
 ( #89893, #56307, #62538, #3720, #63094, #89350, #64732, #4252, #19929 ),
 .UNSPECIFIED., .F., .F.,
 ( 6, 3, 6 ),
 ( 7.637039622810000594, 12.23404602909999994, 12.63071162247140045 ),
 .UNSPECIFIED. ) ;
#16574=CARTESIAN_POINT ( 'NONE',  ( 4.050793647536233166, 1440.940971268299108, 156.1560896747039067 ) ) ;
#16575=EDGE_CURVE ( 'NONE', #6139, #43805, #44993, .T. ) ;
#16577=EDGE_LOOP ( 'NONE', ( #905, #13727, #69289, #102941, #68421 ) ) ;
#16578=CARTESIAN_POINT ( 'NONE',  ( -42.60628463180169945, 1443.705283475299893, 134.4203400610479946 ) ) ;
#16579=CARTESIAN_POINT ( 'NONE',  ( -11.73563908010000034, 1425.610159190430068, 144.1657657165980027 ) ) ;
#16583=CARTESIAN_POINT ( 'NONE',  ( -21.75051292122820712, 1509.709027869026613, 229.3696503746045607 ) ) ;
#16584=CARTESIAN_POINT ( 'NONE',  ( -4.071011801012067721, 1440.982759184028509, 184.9244102487123200 ) ) ;
#16585=B_SPLINE_CURVE_WITH_KNOTS ( 'NONE', 3,
 ( #107583, #15155, #98624, #66710, #23569, #49346, #7331, #56090, #90216, #82930, #13501, #82390, #40928, #39276, #108126, #31420, #31978, #66168, #73450, #21890, #100818, #99715, #49898, #48807, #58297, #30319, #100289, #14060, #72892, #48247, #91882, #23008, #83472, #30869, #92419, #99161, #107033, #64507, #22441, #90777, #56643, #34182, #7872 ),
 .UNSPECIFIED., .F., .F.,
 ( 4, 3, 3, 3, 3, 3, 3, 3, 3, 3, 3, 3, 3, 3, 4 ),
 ( -2.000000000000000000, -1.991901403786979996, -1.843562329601740046, -1.687124659203469879, -1.535545284513649911, -1.380727046018200177, -1.226212339367769966, -1.070990695444660190, -0.9154280613754459672, -0.7599146134399699104, -0.6053024803659901032, -0.4517551365012870690, -0.2995620430569270187, -0.1489321397233329680, -3.117070652702835787E-07 ),
 .UNSPECIFIED. ) ;
#16593=CARTESIAN_POINT ( 'NONE',  ( 37.55019124142308584, 1436.545190195376108, 135.0428483764136445 ) ) ;
#16594=CARTESIAN_POINT ( 'NONE',  ( 20.01039973129999794, 1508.355603643830136, 189.0623068450979929 ) ) ;
#16595=CARTESIAN_POINT ( 'NONE',  ( -1.600048698852036821, 1411.254281879943164, 135.5999999980979851 ) ) ;
#16597=CARTESIAN_POINT ( 'NONE',  ( -12.78776258870000149, 1416.851343894929869, 195.5391574245979882 ) ) ;
#16598=CARTESIAN_POINT ( 'NONE',  ( -8.324962519149999840E-16, 1519.913060387329779, 209.1218459616979999 ) ) ;
#16599=ORIENTED_EDGE ( 'NONE', *, *, #45206, .F. ) ;
#16605=CARTESIAN_POINT ( 'NONE',  ( -8535.261851438322992, 2833.596074015641989, 11230.49242346659776 ) ) ;
#16611=CARTESIAN_POINT ( 'NONE',  ( -2.455820327400000114, 1434.541746329560056, 150.3615916412979914 ) ) ;
#16612=CARTESIAN_POINT ( 'NONE',  ( 39.54663510683320027, 1440.913060369859977, 258.6366483742290256 ) ) ;
#16615=CARTESIAN_POINT ( 'NONE',  ( 13.40566205799999899, 1429.098591196430107, 222.0107402513980333 ) ) ;
#16616=ORIENTED_EDGE ( 'NONE', *, *, #40642, .F. ) ;
#16619=EDGE_CURVE ( 'NONE', #48466, #59575, #29654, .T. ) ;
#16621=CARTESIAN_POINT ( 'NONE',  ( -24.41126182779999709, 1441.219864612629863, 212.0468573075179961 ) ) ;
#16622=CARTESIAN_POINT ( 'NONE',  ( 1.703662692062522188, 1410.351485318999721, 185.3575011929372636 ) ) ;
#16623=CARTESIAN_POINT ( 'NONE',  ( -3.612067548279275453, 1426.010407914519874, 185.9361413070191986 ) ) ;
#16624=EDGE_CURVE ( 'NONE', #14981, #45960, #55249, .T. ) ;
#16629=CARTESIAN_POINT ( 'NONE',  ( 10.80972683769999954, 1452.101161015629941, 151.9897701840980062 ) ) ;
#16635=CARTESIAN_POINT ( 'NONE',  ( 15.20184466319999927, 1507.442701412029919, 186.5339258382980177 ) ) ;
#16636=B_SPLINE_CURVE_WITH_KNOTS ( 'NONE', 5,
 ( #49910, #84044, #75665, #14077, #6237, #33088 ),
 .UNSPECIFIED., .F., .F.,
 ( 6, 6 ),
 ( -93.34500910270000418, -16.36816738400000304 ),
 .UNSPECIFIED. ) ;
#16640=ORIENTED_EDGE ( 'NONE', *, *, #4509, .F. ) ;
#16641=CARTESIAN_POINT ( 'NONE',  ( 18.20120699554579957, 1508.790952174090080, 230.6639428141660346 ) ) ;
#16646=B_SPLINE_CURVE_WITH_KNOTS ( 'NONE', 3,
 ( #93401, #42450, #66588, #75530, #84459, #102352, #100691, #8288, #32939, #58169, #7207, #24528, #92851, #8838, #6646, #16127, #59827, #84993, #16666 ),
 .UNSPECIFIED., .F., .F.,
 ( 4, 2, 2, 2, 1, 1, 1, 1, 1, 2, 2, 4 ),
 ( 0.000000000000000000, 0.2500000000002616796, 0.3750000000003925194, 0.4375000000004576339, 0.4687500000004921619, 0.4843750000005068723, 0.4921875000005165868, 0.4960937500005219158, 0.4980468750005243583, 0.4990234375005250245, 0.5000000000005256906, 1.000000000000000000 ),
 .UNSPECIFIED. ) ;
#16650=CARTESIAN_POINT ( 'NONE',  ( -11.21009720348472882, 1434.253606524949873, 151.6059541307748191 ) ) ;
#16651=CARTESIAN_POINT ( 'NONE',  ( -3.387218493868067171, 1485.678307060469024, 182.9053799028293383 ) ) ;
#16652=CARTESIAN_POINT ( 'NONE',  ( 4.382233832780000782, 1409.233371194429992, 186.7458337506980115 ) ) ;
#16653=CARTESIAN_POINT ( 'NONE',  ( 4.519805968770000071, 1423.798844936530031, 183.7327313443980188 ) ) ;
#16655=CARTESIAN_POINT ( 'NONE',  ( -2.500000010717490007, 1439.743081382919854, 158.2290103479810170 ) ) ;
#16656=CARTESIAN_POINT ( 'NONE',  ( 11.73563886785350086, 1425.610159375979947, 144.1657481682890136 ) ) ;
#16657=CARTESIAN_POINT ( 'NONE',  ( 0.5195835033840000561, 1465.018085799629944, 237.7479754663980032 ) ) ;
#16660=CARTESIAN_POINT ( 'NONE',  ( -1.116585105924089969E-07, 1397.914279478820163, 196.1218459578329885 ) ) ;
#16661=CARTESIAN_POINT ( 'NONE',  ( -26.36916569686470169, 1446.546730999289821, 137.7167333428670020 ) ) ;
#16663=LINE ( 'NONE', #84456, #41463 ) ;
#16665=CARTESIAN_POINT ( 'NONE',  ( -1.163550753797859917E-08, 1474.117094278439936, 263.5999159951250022 ) ) ;
#16666=CARTESIAN_POINT ( 'NONE',  ( 25.00977876991279913, 1436.598012848749931, 137.9330263815630246 ) ) ;
#16668=CARTESIAN_POINT ( 'NONE',  ( -1.347852712580000167, 1417.336052002229962, 235.7060345899980121 ) ) ;
#16673=CARTESIAN_POINT ( 'NONE',  ( -46.11540523431960281, 1439.221583252120126, 266.9731953717790134 ) ) ;
#16679=EDGE_CURVE ( 'NONE', #61380, #54399, #87363, .T. ) ;
#16683=CARTESIAN_POINT ( 'NONE',  ( -26.75564819202289968, 1450.885958589989968, 136.4275090895790186 ) ) ;
#16685=CARTESIAN_POINT ( 'NONE',  ( 21.16722375039999804, 1430.152617814430187, 217.2719924742480089 ) ) ;
#16688=CARTESIAN_POINT ( 'NONE',  ( 14.45760366715495593, 1416.831922878981004, 196.8518846270366396 ) ) ;
#16689=CARTESIAN_POINT ( 'NONE',  ( -7.240818526079999984, 1422.864346058830051, 211.7372259730379938 ) ) ;
#16691=EDGE_CURVE ( 'NONE', #45174, #13629, #91317, .T. ) ;
#16693=CARTESIAN_POINT ( 'NONE',  ( -17.40764085468179800, 1414.996442620800053, 207.5654756526599840 ) ) ;
#16695=CARTESIAN_POINT ( 'NONE',  ( -6.760649935883880524, 1408.923413865439898, 270.4241599285139728 ) ) ;
#16696=CARTESIAN_POINT ( 'NONE',  ( 4.766109705707320288, 1416.570715930979986, 231.5949414777570041 ) ) ;
#16703=CARTESIAN_POINT ( 'NONE',  ( -7.097634907420000694, 1427.571433844230114, 133.6118001900980232 ) ) ;
#16704=CARTESIAN_POINT ( 'NONE',  ( -19.47585981394729870, 1458.049649394619792, 193.7545121080359820 ) ) ;
#16705=CARTESIAN_POINT ( 'NONE',  ( -17.66551749759999979, 1410.882307517030085, 225.3279256837980142 ) ) ;
#16706=CARTESIAN_POINT ( 'NONE',  ( 33.13841419969649849, 1465.588173225519995, 268.0170166519210397 ) ) ;
#16711=CARTESIAN_POINT ( 'NONE',  ( 18.94699345070725016, 1457.564172839218827, 226.7977625303617515 ) ) ;
#16717=CARTESIAN_POINT ( 'NONE',  ( 27.03067664649999813, 1451.714498883330180, 135.7945611549980072 ) ) ;
#16724=CARTESIAN_POINT ( 'NONE',  ( 1.854665035029979814, 1408.977826717500193, 186.8880553776029956 ) ) ;
#16726=FACE_OUTER_BOUND ( 'NONE', #41781, .T. ) ;
#16730=VERTEX_POINT ( 'NONE', #2316 ) ;
#16731=CARTESIAN_POINT ( 'NONE',  ( 11.74432248201719986, 1415.089118586279938, 221.6914046880520175 ) ) ;
#16732=CARTESIAN_POINT ( 'NONE',  ( 11.19478300405899951, 1432.344513976420103, 151.5793324132870055 ) ) ;
#16739=CARTESIAN_POINT ( 'NONE',  ( -0.8167354255590000278, 1432.353341358199941, 150.3995506339979897 ) ) ;
#16740=DIRECTION ( 'NONE',  ( -0.9417419115949662300, -0.2378257470769920556, 0.2378257470769920556 ) ) ;
#16741=CARTESIAN_POINT ( 'NONE',  ( 11.23711414429999955, 1433.375750033149870, 151.5590630604979765 ) ) ;
#16742=CARTESIAN_POINT ( 'NONE',  ( 5.969073325650000150, 1453.512197679029896, 209.1218459616979999 ) ) ;
#16743=CARTESIAN_POINT ( 'NONE',  ( 12.87305953246699985, 1416.529254608160045, 196.3216546659990058 ) ) ;
#16750=CARTESIAN_POINT ( 'NONE',  ( 12.87601703102835593, 1398.294686622125255, 207.2957931138314507 ) ) ;
#16751=CARTESIAN_POINT ( 'NONE',  ( -27.67723492755769854, 1509.879570728590124, 222.2494832413370034 ) ) ;
#16752=EDGE_CURVE ( 'NONE', #73277, #33349, #10129, .T. ) ;
#16760=EDGE_CURVE ( 'NONE', #61195, #41530, #27473, .T. ) ;
#16763=CARTESIAN_POINT ( 'NONE',  ( 0.1717492930638790105, 1479.302881201929949, 182.1243356784760010 ) ) ;
#16764=CARTESIAN_POINT ( 'NONE',  ( -2.983724533230000198, 1408.833818059829809, 223.1998287106980001 ) ) ;
#16766=CARTESIAN_POINT ( 'NONE',  ( -13.59716640859999970, 1444.740067931808653, 176.5566119326980754 ) ) ;
#16767=DIRECTION ( 'NONE',  ( 0.000000000000000000, -0.9990482215818579093, 0.04361938736533144123 ) ) ;
#16768=CARTESIAN_POINT ( 'NONE',  ( 12.91279240200000089, 1434.774393157829991, 149.9807649658980040 ) ) ;
#16769=CARTESIAN_POINT ( 'NONE',  ( -40.71250048055519954, 1447.497876395859976, 134.0999999984609872 ) ) ;
#16773=CARTESIAN_POINT ( 'NONE',  ( -38.64592363268830155, 1443.862568456279860, 137.1880729353390223 ) ) ;
#16775=CARTESIAN_POINT ( 'NONE',  ( -16.64491379450000252, 1416.823872462229929, 216.8740446600579901 ) ) ;
#16776=DIRECTION ( 'NONE',  ( 0.000000000000000000, 1.000000000000000000, 0.000000000000000000 ) ) ;
#16778=CARTESIAN_POINT ( 'NONE',  ( -13.62020111877600215, 1443.814707039050063, 195.1253454527559938 ) ) ;
#16786=VERTEX_POINT ( 'NONE', #77890 ) ;
#16787=CARTESIAN_POINT ( 'NONE',  ( -29.82725620059999727, 1451.718533343729860, 135.7071959994979977 ) ) ;
#16789=ORIENTED_EDGE ( 'NONE', *, *, #62096, .T. ) ;
#16791=CARTESIAN_POINT ( 'NONE',  ( 22.59263393849999702, 1509.026251551730184, 224.5515445014980003 ) ) ;
#16794=CARTESIAN_POINT ( 'NONE',  ( 42.06232107018946920, 1441.883906795105304, 269.6487541092193396 ) ) ;
#16796=CARTESIAN_POINT ( 'NONE',  ( 14.95071165534215929, 1430.594940584589040, 220.1523712821232550 ) ) ;
#16799=LINE ( 'NONE', #77311, #109207 ) ;
#16804=CARTESIAN_POINT ( 'NONE',  ( 2.500000000000000000, 1448.685390747959900, 157.9322671792980088 ) ) ;
#16809=ORIENTED_EDGE ( 'NONE', *, *, #104233, .F. ) ;
#16813=ORIENTED_EDGE ( 'NONE', *, *, #102204, .F. ) ;
#16815=CARTESIAN_POINT ( 'NONE',  ( -19.06924802629999860, 1449.793579044900071, 193.8241538110980287 ) ) ;
#16816=CARTESIAN_POINT ( 'NONE',  ( -11.42633400283000000, 1426.449296649120015, 121.9050361278559933 ) ) ;
#16817=CARTESIAN_POINT ( 'NONE',  ( 17.30265999255270160, 1410.882230744779918, 192.3281541713860179 ) ) ;
#16819=CARTESIAN_POINT ( 'NONE',  ( 28.29401033920189334, 1510.012592320659451, 219.1028198056735050 ) ) ;
#16821=CARTESIAN_POINT ( 'NONE',  ( 16.87646696224889808, 1509.508879493530003, 233.2953025406949905 ) ) ;
#16822=CARTESIAN_POINT ( 'NONE',  ( 10.91472019480807099, 1464.331604664801262, 232.0109029648223498 ) ) ;
#16825=CARTESIAN_POINT ( 'NONE',  ( -36.67418371293260293, 1437.731587266990118, 136.5491800809179779 ) ) ;
#16826=ORIENTED_EDGE ( 'NONE', *, *, #62279, .F. ) ;
#16827=CARTESIAN_POINT ( 'NONE',  ( 6.518255528160000090, 1396.140682886129980, 199.2813087664480065 ) ) ;
#16829=CARTESIAN_POINT ( 'NONE',  ( -17.49295792170000041, 1458.163342941830024, 229.7618723593980121 ) ) ;
#16833=CARTESIAN_POINT ( 'NONE',  ( 16.27717394516742644, 1410.853839490788232, 226.7437855747935771 ) ) ;
#16841=CARTESIAN_POINT ( 'NONE',  ( -6.546422875089999316, 1461.189193418830200, 233.6698635447980053 ) ) ;
#16842=CARTESIAN_POINT ( 'NONE',  ( 19.25375188179999952, 1464.258769156330118, 224.0689215379980226 ) ) ;
#16844=CARTESIAN_POINT ( 'NONE',  ( 33.43619682799734250, 1442.831169986189025, 154.5918098732002477 ) ) ;
#16846=ORIENTED_EDGE ( 'NONE', *, *, #87030, .F. ) ;
#16853=CARTESIAN_POINT ( 'NONE',  ( -14.34604702270000054, 1416.547221147930031, 221.5678632711980072 ) ) ;
#16855=CARTESIAN_POINT ( 'NONE',  ( -12.94068535313328816, 1442.831169986190844, 169.4787936161724531 ) ) ;
#16856=CARTESIAN_POINT ( 'NONE',  ( 2.918143513847768445E-16, 1426.814114634534008, 137.0999999980979851 ) ) ;
#16858=CARTESIAN_POINT ( 'NONE',  ( -4.649632428550000363, 1420.176632528429991, 186.4708458343980055 ) ) ;
#16865=CARTESIAN_POINT ( 'NONE',  ( 18.22874257970000400, 1457.634144810630005, 229.9687939399979939 ) ) ;
#16867=CARTESIAN_POINT ( 'NONE',  ( -4.921467313154969325, 1423.360444961196208, 184.6901157546226671 ) ) ;
#16868=CARTESIAN_POINT ( 'NONE',  ( -5.690944892507480368, 1423.249492944180020, 98.05123491677301217 ) ) ;
#16870=CARTESIAN_POINT ( 'NONE',  ( 18.15379326206519650, 1424.500835680889850, 223.9151983833729957 ) ) ;
#16873=CARTESIAN_POINT ( 'NONE',  ( -2.911525634509525950, 1484.758356318058532, 183.2323580766349096 ) ) ;
#16875=VECTOR ( 'NONE', #97192, 1000.000000000000114 ) ;
#16878=CARTESIAN_POINT ( 'NONE',  ( 0.9116193683959998850, 1471.312091221629998, 187.8213723156979995 ) ) ;
#16880=EDGE_CURVE ( 'NONE', #74855, #52007, #11218, .T. ) ;
#16881=CARTESIAN_POINT ( 'NONE',  ( -10.90096434610000031, 1427.628183919430057, 150.0868075714980137 ) ) ;
#16882=CARTESIAN_POINT ( 'NONE',  ( 1.547463896846929865, 1414.913060387349788, 192.3096116128920130 ) ) ;
#16883=CARTESIAN_POINT ( 'NONE',  ( -7.472928504960000495, 1442.056855012459891, 184.7838669167980186 ) ) ;
#16884=CARTESIAN_POINT ( 'NONE',  ( 27.01620368378947035, 1451.969623355777230, 135.0020654903796640 ) ) ;
#16886=DIRECTION ( 'NONE',  ( 0.0002641870098999210353, 0.9990417697183311407, 0.04376611204218300993 ) ) ;
#16887=CARTESIAN_POINT ( 'NONE',  ( -20.21775582709999952, 1495.373515144229941, 227.9074475250980072 ) ) ;
#16889=CARTESIAN_POINT ( 'NONE',  ( -16.61577472324600180, 1459.965097909202086, 228.4923730740709971 ) ) ;
#16892=CARTESIAN_POINT ( 'NONE',  ( 21.91814464780000193, 1410.042932703930092, 267.0360865957980536 ) ) ;
#16894=CARTESIAN_POINT ( 'NONE',  ( 23.43244672160000164, 1469.150049903229956, 198.8857204875980074 ) ) ;
#16895=CARTESIAN_POINT ( 'NONE',  ( -0.2265857601506459928, 1508.856173191960124, 238.3683916615930229 ) ) ;
#16897=CARTESIAN_POINT ( 'NONE',  ( -1.331441941370000048, 1451.289091497329991, 183.6056191985979922 ) ) ;
#16901=CARTESIAN_POINT ( 'NONE',  ( -13.49844358240000020, 1443.565604340589971, 187.1529031832980081 ) ) ;
#16902=CARTESIAN_POINT ( 'NONE',  ( -22.58439900540000167, 1519.913060387329779, 209.1218459616979999 ) ) ;
#16903=LINE ( 'NONE', #43259, #26876 ) ;
#16905=ORIENTED_EDGE ( 'NONE', *, *, #62580, .T. ) ;
#16906=CARTESIAN_POINT ( 'NONE',  ( 1.462581545746759915, 1493.452708605139833, 181.7091337628779968 ) ) ;
#16907=CARTESIAN_POINT ( 'NONE',  ( -14.91623439969129983, 1409.433946770479906, 209.8509277100439760 ) ) ;
#16911=CARTESIAN_POINT ( 'NONE',  ( -21.98433884700000007, 1471.929809744629893, 267.6462616537980352 ) ) ;
#16914=CIRCLE ( 'NONE', #31254, 29.83173541461230727 ) ;
#16915=CARTESIAN_POINT ( 'NONE',  ( -24.61293950550089704, 1444.770188684140066, 210.8869336946189890 ) ) ;
#16919=CARTESIAN_POINT ( 'NONE',  ( -6.733046173459999117, 1443.913060387330006, 154.8821828340979891 ) ) ;
#16920=B_SPLINE_SURFACE_WITH_KNOTS ( 'NONE', 3, 5, ( 
 ( #21311, #55514, #28091, #70691, #89642, #79621 ),
 ( #81235, #4550, #38684, #72859, #106993, #104803 ),
 ( #62278, #96409, #6185, #7294, #14579, #49310 ),
 ( #56053, #66674, #99126, #82351, #83436, #23532 ) ),
 .UNSPECIFIED., .F., .F., .F.,
 ( 4, 4 ),
 ( 6, 6 ),
 ( 5.479555871690000579, 5.505626611740000342 ),
 ( 0.000000000000000000, 1.000000000000000000 ),
 .UNSPECIFIED. ) ;
#16924=CARTESIAN_POINT ( 'NONE',  ( -23.55015523019999790, 1410.657012870829931, 206.5846774848380107 ) ) ;
#16928=B_SPLINE_SURFACE_WITH_KNOTS ( 'NONE', 5, 5, ( 
 ( #34422, #843, #93749, #58538, #69150, #84269 ),
 ( #68053, #102700, #57988, #33303, #15938, #34968 ),
 ( #92122, #25445, #77538, #41719, #42829, #101054 ),
 ( #15398, #50142, #60192, #296, #75879, #102163 ),
 ( #94311, #25994, #17590, #51224, #92664, #49587 ),
 ( #7013, #59638, #83718, #24352, #7564, #76990 ),
 ( #41171, #59093, #75345, #23797, #16485, #110027 ),
 ( #66945, #109485, #93218, #84807, #32762, #51789 ),
 ( #67498, #101602, #24886, #50674, #76423, #8106 ),
 ( #85929, #42273, #110577, #33862, #17026, #85357 ),
 ( #68596, #8652, #9232, #43389, #65218, #38332 ),
 ( #20970, #80904, #63045, #72512, #71989, #99329 ) ),
 .UNSPECIFIED., .F., .F., .F.,
 ( 6, 3, 3, 6 ),
 ( 6, 6 ),
 ( 24.09973612510790275, 25.95605821120000201, 29.66855005029999859, 34.15088587921729868 ),
 ( 0.000000000000000000, 1.506138665727279946 ),
 .UNSPECIFIED. ) ;
#16929=CARTESIAN_POINT ( 'NONE',  ( 2.488082932330000219, 1441.600846913620217, 150.5962877614979902 ) ) ;
#16935=CARTESIAN_POINT ( 'NONE',  ( 11.70540788988509817, 1426.716494867529946, 141.9064542283970241 ) ) ;
#16939=CARTESIAN_POINT ( 'NONE',  ( -16.93613037863659798, 1507.562498015370011, 224.5799860225920099 ) ) ;
#16941=CARTESIAN_POINT ( 'NONE',  ( -8.104953377315247565, 1398.153764496908934, 219.2861827199897107 ) ) ;
#16942=CARTESIAN_POINT ( 'NONE',  ( -3.592552031026975179, 1440.810949641668003, 156.6291991093122249 ) ) ;
#16944=CARTESIAN_POINT ( 'NONE',  ( 1.622533072389999997, 1508.277906825730042, 236.9750079829979654 ) ) ;
#16946=ORIENTED_EDGE ( 'NONE', *, *, #93320, .T. ) ;
#16948=CARTESIAN_POINT ( 'NONE',  ( 11.73789100506060024, 1434.215254847310007, 151.1141485369599877 ) ) ;
#16955=DIRECTION ( 'NONE',  ( -1.000000000000000000, -8.646726228680001294E-15, 8.117787186050000125E-15 ) ) ;
#16956=CARTESIAN_POINT ( 'NONE',  ( -13.92066065641689931, 1508.898256883639988, 183.7940940037009909 ) ) ;
#16957=CARTESIAN_POINT ( 'NONE',  ( 18.84417403770989807, 1488.414032370149926, 228.9378882694660149 ) ) ;
#16958=CARTESIAN_POINT ( 'NONE',  ( 0.5822587378750000431, 1468.709556387730117, 182.6088673434980194 ) ) ;
#16960=CARTESIAN_POINT ( 'NONE',  ( -24.11922042919299614, 1444.793574266630003, 211.7007084662699867 ) ) ;
#16963=CARTESIAN_POINT ( 'NONE',  ( 14.13162141313959985, 1415.651572961190141, 197.1859206090720136 ) ) ;
#16965=CARTESIAN_POINT ( 'NONE',  ( 11.86651437599999959, 1432.376750741719889, 150.3970641568979829 ) ) ;
#16967=EDGE_LOOP ( 'NONE', ( #21388, #69655, #36508 ) ) ;
#16968=CARTESIAN_POINT ( 'NONE',  ( 13.74968914389999952, 1435.188641123959997, 149.5600858840979868 ) ) ;
#16971=CARTESIAN_POINT ( 'NONE',  ( 13.51157294017894017, 1444.017624626980023, 169.3518533014032243 ) ) ;
#16972=CARTESIAN_POINT ( 'NONE',  ( -11.45446824389999918, 1462.185551541130053, 233.9517322583979819 ) ) ;
#16976=CARTESIAN_POINT ( 'NONE',  ( -18.98174732980886859, 1443.401523302673013, 211.6634804359809152 ) ) ;
#16979=( BOUNDED_CURVE ( )  B_SPLINE_CURVE ( 3, ( #73205, #6546, #92200, #56409 ),
 .UNSPECIFIED., .F., .F. ) 
 B_SPLINE_CURVE_WITH_KNOTS ( ( 4, 4 ),
 ( 3.107150058479552168, 3.118904538992639086 ),
 .UNSPECIFIED. ) 
 CURVE ( )  GEOMETRIC_REPRESENTATION_ITEM ( )  RATIONAL_B_SPLINE_CURVE ( ( 1.000000000000000000, 0.9999884860487986415, 0.9999884860487986415, 1.000000000000000000 ) ) 
 REPRESENTATION_ITEM ( '' )  );
#16982=VERTEX_POINT ( 'NONE', #99486 ) ;
#16985=CARTESIAN_POINT ( 'NONE',  ( -9.049519031959999182, 1409.396208824930000, 188.6360524509980223 ) ) ;
#16987=FACE_OUTER_BOUND ( 'NONE', #9556, .T. ) ;
#16989=CARTESIAN_POINT ( 'NONE',  ( 19.98583999950000134, 1427.549906271330201, 222.6473461575979798 ) ) ;
#16997=EDGE_CURVE ( 'NONE', #83528, #10270, #20170, .T. ) ;
#17006=CARTESIAN_POINT ( 'NONE',  ( -1.026416548450000011E-08, 1474.725755678329961, 264.8987716733979596 ) ) ;
#17007=ADVANCED_FACE ( 'NONE', ( #83807 ), #29220, .T. ) ;
#17010=CARTESIAN_POINT ( 'NONE',  ( -5.589046920511240302, 1509.019018111649984, 237.4740947115990082 ) ) ;
#17011=CARTESIAN_POINT ( 'NONE',  ( -23.32672961829999991, 1448.440545525210155, 217.0581287948379838 ) ) ;
#17014=CARTESIAN_POINT ( 'NONE',  ( 19.75084982839999981, 1455.504334175230042, 226.5702129394979920 ) ) ;
#17017=EDGE_LOOP ( 'NONE', ( #12113, #53962, #87646, #64550 ) ) ;
#17020=CARTESIAN_POINT ( 'NONE',  ( 27.70707300099999770, 1508.597282344630003, 207.6634441784080138 ) ) ;
#17022=CARTESIAN_POINT ( 'NONE',  ( 13.00580119799999856, 1425.728651690429842, 223.4081755709979973 ) ) ;
#17023=CARTESIAN_POINT ( 'NONE',  ( -5.307053063608348609, 1425.580201077015545, 186.3543702352812659 ) ) ;
#17026=CARTESIAN_POINT ( 'NONE',  ( 32.65729098489229898, 1436.532483134479889, 136.5492245839050156 ) ) ;
#17027=DIRECTION ( 'NONE',  ( 1.000000000000000000, 0.000000000000000000, 0.000000000000000000 ) ) ;
#17028=CARTESIAN_POINT ( 'NONE',  ( -31.96358366148169949, 1465.307028659348589, 269.3165098066044152 ) ) ;
#17030=CARTESIAN_POINT ( 'NONE',  ( 11.99724100530000115, 1508.052968999630139, 184.6308883575979962 ) ) ;
#17037=CARTESIAN_POINT ( 'NONE',  ( 11.94171318090000078, 1433.614828344280113, 146.4341826372979938 ) ) ;
#17039=CARTESIAN_POINT ( 'NONE',  ( 16.05002729776590087, 1479.562477948200012, 188.9730107742090013 ) ) ;
#17040=CARTESIAN_POINT ( 'NONE',  ( 11.32679319035097443, 1425.526293419519106, 138.7440965005115743 ) ) ;
#17043=CARTESIAN_POINT ( 'NONE',  ( -28.27930516629999858, 1508.150008668130113, 209.2731387451690068 ) ) ;
#17047=CARTESIAN_POINT ( 'NONE',  ( 43.48864058788180387, 1440.913032444390183, 270.3367086676489635 ) ) ;
#17048=CARTESIAN_POINT ( 'NONE',  ( -38.61927355701700293, 1444.188087899089851, 137.1592452686400065 ) ) ;
#17049=CARTESIAN_POINT ( 'NONE',  ( -16.49832412793039893, 1414.913057855109855, 208.5959317959809880 ) ) ;
#17050=CARTESIAN_POINT ( 'NONE',  ( 24.84705735490000222, 1435.864857748740178, 137.4753733619980096 ) ) ;
#17051=CARTESIAN_POINT ( 'NONE',  ( -9.716620324715218970, 1396.252372248279926, 203.8292857818589994 ) ) ;
#17053=CARTESIAN_POINT ( 'NONE',  ( -0.08022770239056420394, 1416.524489948229984, 191.0302681666710214 ) ) ;
#17054=CARTESIAN_POINT ( 'NONE',  ( -4.781335570289999559, 1409.080028304630105, 230.4240303851980229 ) ) ;
#17060=CARTESIAN_POINT ( 'NONE',  ( -24.41186848150000444, 1440.913060429529878, 212.0284777737979880 ) ) ;
#17062=CARTESIAN_POINT ( 'NONE',  ( 4.191474726083669999, 1424.969438579149937, 185.2130605783640078 ) ) ;
#17064=CARTESIAN_POINT ( 'NONE',  ( -2.508314376045169158, 1421.038292245390949, 185.1991979782232249 ) ) ;
#17067=CARTESIAN_POINT ( 'NONE',  ( 8.768089064850000725, 1509.161960657329928, 181.7959779642980038 ) ) ;
#17070=CARTESIAN_POINT ( 'NONE',  ( -29.05308884557584648, 1510.038507275123038, 216.5997246920866530 ) ) ;
#17075=EDGE_CURVE ( 'NONE', #1945, #53899, #70875, .T. ) ;
#17079=CARTESIAN_POINT ( 'NONE',  ( -3.148011829640000148, 1473.184271403730008, 270.4279803161980453 ) ) ;
#17080=CARTESIAN_POINT ( 'NONE',  ( 11.87742785157381320, 1433.145466849493459, 147.6581215103447846 ) ) ;
#17082=CARTESIAN_POINT ( 'NONE',  ( 18.07642520410000131, 1475.513060387329915, 197.7809371531980105 ) ) ;
#17085=B_SPLINE_SURFACE_WITH_KNOTS ( 'NONE', 5, 5, ( 
 ( #60236, #52946, #346, #69763, #10366, #60807 ),
 ( #19865, #44539, #1426, #94355, #43435, #17635 ),
 ( #893, #54068, #79250, #87647, #78684, #35016 ),
 ( #28279, #85975, #27180, #96594, #36137, #70321 ),
 ( #103880, #27727, #61914, #103302, #34473, #18204 ),
 ( #95483, #69196, #77586, #18750, #36682, #10933 ) ),
 .UNSPECIFIED., .F., .F., .F.,
 ( 6, 6 ),
 ( 6, 6 ),
 ( 6.379848894300000239, 6.971437020549999808 ),
 ( 0.000000000000000000, 1.455467945630000148 ),
 .UNSPECIFIED. ) ;
#17090=CARTESIAN_POINT ( 'NONE',  ( -18.77802133838000032, 1408.856599020109797, 267.0889509827300117 ) ) ;
#17091=CARTESIAN_POINT ( 'NONE',  ( -14.19163021719490025, 1435.224332456559978, 149.3102015397809907 ) ) ;
#17094=CARTESIAN_POINT ( 'NONE',  ( 13.17178224790000129, 1444.791376412119916, 187.5900384370979737 ) ) ;
#17099=CARTESIAN_POINT ( 'NONE',  ( -18.90100382950000224, 1470.475492315429847, 190.2665493832980133 ) ) ;
#17103=AXIS2_PLACEMENT_3D ( 'NONE', #46052, #80185, #3500 ) ;
#17106=CARTESIAN_POINT ( 'NONE',  ( -28.21332310190000214, 1508.643929351929955, 208.4757879089329720 ) ) ;
#17107=CARTESIAN_POINT ( 'NONE',  ( -0.7293669130959999913, 1467.886321022529955, 230.1640753799979962 ) ) ;
#17110=AXIS2_PLACEMENT_3D ( 'NONE', #91809, #7263, #24583 ) ;
#17112=CARTESIAN_POINT ( 'NONE',  ( -3.985728878099999761, 1408.516724292330082, 196.0795530488979921 ) ) ;
#17113=FACE_OUTER_BOUND ( 'NONE', #32435, .T. ) ;
#17116=CARTESIAN_POINT ( 'NONE',  ( -24.86491373321030096, 1430.503315265359788, 209.8722520918030057 ) ) ;
#17117=CARTESIAN_POINT ( 'NONE',  ( 27.21299276530000100, 1488.689717874130110, 210.5521098509080105 ) ) ;
#17120=CARTESIAN_POINT ( 'NONE',  ( -23.87957571749999985, 1435.331403578989921, 136.9496437524980195 ) ) ;
#17123=CARTESIAN_POINT ( 'NONE',  ( -14.52771248069999999, 1418.016205493429879, 227.0709974350980076 ) ) ;
#17124=CARTESIAN_POINT ( 'NONE',  ( -12.98226561589999939, 1414.913060387329779, 219.9156672276980089 ) ) ;
#17127=FACE_OUTER_BOUND ( 'NONE', #23319, .T. ) ;
#17128=CARTESIAN_POINT ( 'NONE',  ( -5.961592730449999600, 1410.297059247229981, 231.5003550203979898 ) ) ;
#17130=ORIENTED_EDGE ( 'NONE', *, *, #18307, .T. ) ;
#17131=CARTESIAN_POINT ( 'NONE',  ( -13.15726396577390034, 1415.954755716080172, 220.1962943805110058 ) ) ;
#17133=CARTESIAN_POINT ( 'NONE',  ( 12.17555016557819947, 1435.314517998499923, 151.0473610424109836 ) ) ;
#17135=CARTESIAN_POINT ( 'NONE',  ( -4.089785825655819274, 1441.278398204691484, 184.5636933043436443 ) ) ;
#17136=CARTESIAN_POINT ( 'NONE',  ( -25.22529742364680061, 1509.794288727649928, 224.2186411218499984 ) ) ;
#17138=CARTESIAN_POINT ( 'NONE',  ( 44.21963038504740240, 1440.913060387359792, 267.5638318536060183 ) ) ;
#17139=DIRECTION ( 'NONE',  ( 0.4794255386041986200, 0.000000000000000000, 0.8775825618903752012 ) ) ;
#17140=CARTESIAN_POINT ( 'NONE',  ( 10.10004869885203682, 1423.143362674105219, 137.0999999980979851 ) ) ;
#17142=CARTESIAN_POINT ( 'NONE',  ( -2.917792487480000307, 1420.757440859130156, 185.9241331037979990 ) ) ;
#17146=CARTESIAN_POINT ( 'NONE',  ( -12.78690732010000097, 1416.828044802929981, 195.5394877781979801 ) ) ;
#17147=CARTESIAN_POINT ( 'NONE',  ( -11.60004869885203682, 1426.170950560207530, 138.0046165345982843 ) ) ;
#17150=CARTESIAN_POINT ( 'NONE',  ( 3.444734345749999704, 1421.426336298530032, 184.7111240843979942 ) ) ;
#17154=CARTESIAN_POINT ( 'NONE',  ( 9857.840209716168829, 50.13405481564039690, -1086.115145477200031 ) ) ;
#17157=CARTESIAN_POINT ( 'NONE',  ( 18.88088134670000073, 1416.274718424630009, 210.4721620632179793 ) ) ;
#17159=CARTESIAN_POINT ( 'NONE',  ( -4.926829097150000614, 1435.943783413959864, 150.1744789664979862 ) ) ;
#17160=CARTESIAN_POINT ( 'NONE',  ( 27.27137807743889653, 1446.453610523900124, 137.2094998867499953 ) ) ;
#17164=EDGE_LOOP ( 'NONE', ( #15726, #65572, #94800, #45351 ) ) ;
#17165=CARTESIAN_POINT ( 'NONE',  ( 1.547077000027379912, 1416.702560751770079, 190.2314781873849654 ) ) ;
#17167=CARTESIAN_POINT ( 'NONE',  ( 2.500000000000000000, 1440.913060387330006, 209.1218459616979999 ) ) ;
#17168=CARTESIAN_POINT ( 'NONE',  ( -24.41186848580399982, 1440.913060429360030, 212.0284777848129920 ) ) ;
#17170=ADVANCED_FACE ( 'NONE', ( #60277 ), #45312, .F. ) ;
#17180=CARTESIAN_POINT ( 'NONE',  ( 14.62022923471335467, 1410.806204316170351, 191.5183363024188168 ) ) ;
#17181=CARTESIAN_POINT ( 'NONE',  ( 24.34813363090000138, 1509.525084498130127, 194.8613372772980199 ) ) ;
#17182=ORIENTED_EDGE ( 'NONE', *, *, #78864, .T. ) ;
#17183=CARTESIAN_POINT ( 'NONE',  ( -18.42620122711428365, 1458.925670360632921, 227.7001417621163455 ) ) ;
#17185=CARTESIAN_POINT ( 'NONE',  ( -17.63065570870000087, 1409.528736451330133, 222.5595780730980096 ) ) ;
#17186=ORIENTED_EDGE ( 'NONE', *, *, #15389, .F. ) ;
#17187=EDGE_LOOP ( 'NONE', ( #91633, #104326, #88489, #74710 ) ) ;
#17188=CARTESIAN_POINT ( 'NONE',  ( 19.46142334528079942, 1509.259962660840074, 230.2314711598330064 ) ) ;
#17189=CARTESIAN_POINT ( 'NONE',  ( 18.80464302510000252, 1425.801049065629968, 225.6039134470979945 ) ) ;
#17190=CARTESIAN_POINT ( 'NONE',  ( 39.30684815028109824, 1440.174742933630114, 136.7448234688500008 ) ) ;
#17191=CARTESIAN_POINT ( 'NONE',  ( 18.10327300539999840, 1416.823634022829992, 209.0372315287800120 ) ) ;
#17198=CARTESIAN_POINT ( 'NONE',  ( 4.283818917599999665, 1409.998137916430096, 186.1439897097980065 ) ) ;
#17199=DIRECTION ( 'NONE',  ( -0.7636030817426309181, -3.014599818829910125E-11, -0.6456859403403150122 ) ) ;
#17200=CARTESIAN_POINT ( 'NONE',  ( 40.27297414431956923, 1443.653306489278748, 137.1208278072323878 ) ) ;
#17201=CARTESIAN_POINT ( 'NONE',  ( 8.002862298599998425, 1439.449515709130083, 153.7646872756980088 ) ) ;
#17202=CARTESIAN_POINT ( 'NONE',  ( -3.654169310603359921, 1441.538905863229957, 168.7225120603009714 ) ) ;
#17203=CARTESIAN_POINT ( 'NONE',  ( -24.63041513499999979, 1451.910759690930036, 137.3284483466979964 ) ) ;
#17204=CARTESIAN_POINT ( 'NONE',  ( 0.4781507175040000113, 1465.417316753030036, 236.2850646078979935 ) ) ;
#17206=EDGE_CURVE ( 'NONE', #93518, #54705, #53543, .T. ) ;
#17208=CARTESIAN_POINT ( 'NONE',  ( -44.28498751210000250, 1445.865707094600111, 269.9174198735980212 ) ) ;
#17209=CARTESIAN_POINT ( 'NONE',  ( -6.232532106187401055, 1407.162969929529936, 197.7132727037109987 ) ) ;
#17212=CARTESIAN_POINT ( 'NONE',  ( 16.40748204129999976, 1468.824047016830036, 189.6837539406980113 ) ) ;
#17214=CARTESIAN_POINT ( 'NONE',  ( -4.059787370426500287E-09, 1471.846784317870060, 258.6367045587240341 ) ) ;
#17217=CARTESIAN_POINT ( 'NONE',  ( -6.210268667529999398, 1417.485306226330067, 231.9805137463980031 ) ) ;
#17220=CARTESIAN_POINT ( 'NONE',  ( -0.6623775808828666900, 1485.388627107794946, 181.9464839905526219 ) ) ;
#17222=CARTESIAN_POINT ( 'NONE',  ( -46.08889470559520163, 1438.835070612000209, 266.9740849372739717 ) ) ;
#17223=CARTESIAN_POINT ( 'NONE',  ( 13.56161761879410044, 1508.782329442760101, 233.5620020540920052 ) ) ;
#17226=ORIENTED_EDGE ( 'NONE', *, *, #17075, .F. ) ;
#17228=CARTESIAN_POINT ( 'NONE',  ( -2.478759544509999913, 1435.233202498340006, 157.6046889441980170 ) ) ;
#17229=CARTESIAN_POINT ( 'NONE',  ( 19.26683521067225868, 1456.110280151028292, 225.0772932314519892 ) ) ;
#17232=B_SPLINE_SURFACE_WITH_KNOTS ( 'NONE', 5, 5, ( 
 ( #4200, #3673, #31035, #37801, #29380, #4734 ),
 ( #73058, #98794, #22056, #90381, #13660, #47849 ),
 ( #81983, #5291, #39449, #73622, #107752, #32699 ),
 ( #32147, #33792, #74174, #41658, #66335, #65765 ),
 ( #109965, #100451, #41096, #100989, #33243, #57382 ),
 ( #14230, #24285, #31588, #7496, #66879, #16419 ),
 ( #108303, #93150, #48419, #23734, #40546, #75275 ),
 ( #15326, #75814, #74720, #50612, #99883, #48974 ),
 ( #82562, #42210, #108853, #57922, #90944, #23181 ) ),
 .UNSPECIFIED., .F., .F., .F.,
 ( 6, 3, 6 ),
 ( 6, 6 ),
 ( 0.7655572723410000169, 2.316155491850000026, 3.835724788479999869 ),
 ( 0.000000000000000000, 1.000000000000000000 ),
 .UNSPECIFIED. ) ;
#17234=CARTESIAN_POINT ( 'NONE',  ( -26.79661678085199839, 1451.977403426660203, 134.9984873815419917 ) ) ;
#17235=ORIENTED_EDGE ( 'NONE', *, *, #65318, .F. ) ;
#17236=CARTESIAN_POINT ( 'NONE',  ( 8.713969742539999785, 1418.939459092229981, 231.9965623745979713 ) ) ;
#17240=CARTESIAN_POINT ( 'NONE',  ( -15.46685519719999924, 1426.081634757429811, 211.8324972136479971 ) ) ;
#17244=CARTESIAN_POINT ( 'NONE',  ( 5426.659192927022559, 54.07981494723836136, 8449.939230966730975 ) ) ;
#17246=CARTESIAN_POINT ( 'NONE',  ( -6.545930427259980533, 1410.746461301010186, 269.3398854477759983 ) ) ;
#17247=CARTESIAN_POINT ( 'NONE',  ( 4.082851105566869698, 1417.107827966569857, 231.9800176705820149 ) ) ;
#17248=CARTESIAN_POINT ( 'NONE',  ( -2.541329734699477427, 1448.915361678037016, 183.5773954481504688 ) ) ;
#17249=CARTESIAN_POINT ( 'NONE',  ( -2.500000000000000000, 1439.595905110280000, 166.5328619750869734 ) ) ;
#17250=VERTEX_POINT ( 'NONE', #45144 ) ;
#17251=ORIENTED_EDGE ( 'NONE', *, *, #102049, .T. ) ;
#17252=EDGE_CURVE ( 'NONE', #18109, #30631, #15138, .T. ) ;
#17253=CARTESIAN_POINT ( 'NONE',  ( -23.15985215759310023, 1409.837679178900089, 209.7045568244390097 ) ) ;
#17254=CARTESIAN_POINT ( 'NONE',  ( -1.354641933420439814, 1409.895065768689847, 185.6211235086560123 ) ) ;
#17256=CARTESIAN_POINT ( 'NONE',  ( -4.743041381730000339, 1427.184332118029943, 133.6118001900980232 ) ) ;
#17257=EDGE_CURVE ( 'NONE', #23409, #53095, #20495, .T. ) ;
#17258=CARTESIAN_POINT ( 'NONE',  ( -14.59279134157089963, 1436.244781760590058, 149.8708244536879874 ) ) ;
#17259=CARTESIAN_POINT ( 'NONE',  ( -17.69728439860000080, 1415.862141658330074, 225.6688577867979859 ) ) ;
#17260=CARTESIAN_POINT ( 'NONE',  ( 30.02970996041729990, 1467.470256667440026, 268.6852542625180149 ) ) ;
#17261=CARTESIAN_POINT ( 'NONE',  ( -3.031930836974722876, 1466.806735891728522, 235.0189408935569872 ) ) ;
#17264=EDGE_LOOP ( 'NONE', ( #7761, #27279, #24843, #55709 ) ) ;
#17265=CARTESIAN_POINT ( 'NONE',  ( -11.90119038212991498, 1433.600011632037877, 150.4754701663967467 ) ) ;
#17270=B_SPLINE_CURVE_WITH_KNOTS ( 'NONE', 3,
 ( #9756, #1370, #53445, #61310, #17576, #33849, #87591, #18691, #35512, #85344, #34955, #52888, #60182, #42816, #94870, #78627, #69705, #76977, #8640, #10308, #25429, #60747, #26553, #59625, #827, #61855, #44481, #68040, #87016, #43920, #9219, #10879, #284, #34410, #77526, #43377, #68582, #76409, #86463, #19236 ),
 .UNSPECIFIED., .F., .F.,
 ( 4, 3, 3, 3, 3, 3, 3, 3, 3, 3, 3, 3, 3, 4 ),
 ( -1.460858415939999988, -1.411203178505739952, -1.297247195856390034, -1.181596853130470137, -1.064890566428260188, -0.9466603196382510355, -0.8277066115153159931, -0.7083408824893170364, -0.5889085004284719815, -0.4643442267839680282, -0.3464089112407460203, -0.2295942582252259445, -0.1140863307625139544, 0.000000000000000000 ),
 .UNSPECIFIED. ) ;
#17271=CARTESIAN_POINT ( 'NONE',  ( 26.71914925442930056, 1451.974538300859876, 135.0890004682200072 ) ) ;
#17275=CARTESIAN_POINT ( 'NONE',  ( 18.49178363470000264, 1410.482338634230018, 194.3597946893979724 ) ) ;
#17277=CARTESIAN_POINT ( 'NONE',  ( 0.4554814033272580054, 1408.928966148389918, 186.5349708927100210 ) ) ;
#17279=CARTESIAN_POINT ( 'NONE',  ( -18.12762350887655316, 1423.809303112999032, 225.6003212586901157 ) ) ;
#17280=CARTESIAN_POINT ( 'NONE',  ( 15.94345596297699963, 1409.469818137940138, 225.2684692625209948 ) ) ;
#17281=LINE ( 'NONE', #85604, #10660 ) ;
#17283=CARTESIAN_POINT ( 'NONE',  ( 5.755110967747741668, 1418.244149184685966, 233.8060213123679887 ) ) ;
#17285=CARTESIAN_POINT ( 'NONE',  ( 12.77667375843740061, 1416.535698381769862, 222.1372311004039943 ) ) ;
#17286=DIRECTION ( 'NONE',  ( 0.000000000000000000, 1.000000000000000000, 0.000000000000000000 ) ) ;
#17290=EDGE_CURVE ( 'NONE', #5392, #49285, #70357, .T. ) ;
#17291=CARTESIAN_POINT ( 'NONE',  ( -34.62870020261659931, 1450.374171996330006, 136.2315969410039997 ) ) ;
#17292=CARTESIAN_POINT ( 'NONE',  ( -12.51099982459209947, 1416.825784013739849, 222.1450729932890056 ) ) ;
#17293=CARTESIAN_POINT ( 'NONE',  ( -28.05448518339999708, 1461.575973621429966, 265.6112251771979800 ) ) ;
#17295=CARTESIAN_POINT ( 'NONE',  ( 11.26092790689999923, 1433.522411100119825, 151.5416666487980137 ) ) ;
#17296=CARTESIAN_POINT ( 'NONE',  ( 28.02005515429999960, 1444.132107003350029, 248.0989693021979861 ) ) ;
#17297=CONICAL_SURFACE ( 'NONE', #85493, 24.00000000000002132, 0.3430239404209998177 ) ;
#17304=LINE ( 'NONE', #76147, #73573 ) ;
#17305=CARTESIAN_POINT ( 'NONE',  ( 2.145405888939999617, 1466.621345377330044, 234.3697071566979844 ) ) ;
#17306=CARTESIAN_POINT ( 'NONE',  ( 19.53984293219999913, 1410.902666560329862, 220.8234250620979822 ) ) ;
#17308=FACE_OUTER_BOUND ( 'NONE', #85713, .T. ) ;
#17309=CARTESIAN_POINT ( 'NONE',  ( -40.51263900100065030, 1439.427257612305539, 135.2566761075825923 ) ) ;
#17311=CARTESIAN_POINT ( 'NONE',  ( 13.91344329550000047, 1453.313060387329870, 223.0352892565979914 ) ) ;
#17316=CARTESIAN_POINT ( 'NONE',  ( 0.1686318752242309815, 1481.134048488709823, 182.0456757912619992 ) ) ;
#17319=CARTESIAN_POINT ( 'NONE',  ( -27.23063139319997816, 1444.324653571829003, 161.8596747266978753 ) ) ;
#17320=EDGE_CURVE ( 'NONE', #77609, #43746, #21586, .T. ) ;
#17321=FACE_OUTER_BOUND ( 'NONE', #80797, .T. ) ;
#17325=ORIENTED_EDGE ( 'NONE', *, *, #43617, .T. ) ;
#17328=CARTESIAN_POINT ( 'NONE',  ( -16.76079633530000024, 1415.087818611729972, 211.7983980607679939 ) ) ;
#17330=EDGE_CURVE ( 'NONE', #63715, #33885, #39139, .T. ) ;
#17340=ORIENTED_EDGE ( 'NONE', *, *, #93708, .F. ) ;
#17341=CARTESIAN_POINT ( 'NONE',  ( 13.14421740897469704, 1443.086052842850677, 164.8757063741590230 ) ) ;
#17343=ORIENTED_EDGE ( 'NONE', *, *, #921, .F. ) ;
#17345=CARTESIAN_POINT ( 'NONE',  ( 27.34567353230000109, 1509.867992349329825, 219.5431460416980087 ) ) ;
#17349=CARTESIAN_POINT ( 'NONE',  ( 0.5717981366250000086, 1450.893092756410169, 154.2461502948980012 ) ) ;
#17350=CARTESIAN_POINT ( 'NONE',  ( -11.60004869885204393, 1427.240389456164394, 134.3215321853161015 ) ) ;
#17351=CARTESIAN_POINT ( 'NONE',  ( 19.11061305480268402, 1438.203271981198668, 213.0090273355756381 ) ) ;
#17352=CARTESIAN_POINT ( 'NONE',  ( 2.489939931649999938, 1417.821760099730000, 233.9513212198979772 ) ) ;
#17357=EDGE_CURVE ( 'NONE', #44537, #80364, #60609, .T. ) ;
#17360=CARTESIAN_POINT ( 'NONE',  ( 4.239021759200000794, 1446.365493823910128, 162.7142476321979814 ) ) ;
#17362=CARTESIAN_POINT ( 'NONE',  ( 20.14111335559999816, 1472.214279811229972, 269.5303638422980157 ) ) ;
#17370=CARTESIAN_POINT ( 'NONE',  ( -23.43227205760000231, 1410.913138759029835, 206.1403821866979911 ) ) ;
#17371=CARTESIAN_POINT ( 'NONE',  ( -11.01180412374380069, 1426.052342128100008, 99.91299076298089687 ) ) ;
#17372=CARTESIAN_POINT ( 'NONE',  ( 17.03258580107809905, 1409.880850962159911, 192.7013530600950162 ) ) ;
#17374=CARTESIAN_POINT ( 'NONE',  ( 17.96796222303624191, 1509.660108813923898, 185.0969589919148461 ) ) ;
#17376=CARTESIAN_POINT ( 'NONE',  ( -20.04379692219999853, 1410.189666917429804, 264.7217003517980061 ) ) ;
#17377=CARTESIAN_POINT ( 'NONE',  ( 17.24816121598360041, 1509.523746382970103, 233.0580511170819875 ) ) ;
#17378=CARTESIAN_POINT ( 'NONE',  ( 17.28674646035066687, 1460.161652801043374, 228.5469262299488094 ) ) ;
#17381=CARTESIAN_POINT ( 'NONE',  ( -38.91668594174339546, 1439.604252461880151, 136.6912434827079892 ) ) ;
#17383=CARTESIAN_POINT ( 'NONE',  ( 12.22548255495519953, 1396.339983646510063, 207.2249384526400036 ) ) ;
#17386=CARTESIAN_POINT ( 'NONE',  ( -16.89883965940000365, 1458.595428821529822, 229.9355491509979856 ) ) ;
#17390=CARTESIAN_POINT ( 'NONE',  ( -2.416798835000000256, 1426.601114010129777, 146.0361887655980127 ) ) ;
#17391=CARTESIAN_POINT ( 'NONE',  ( 1.010302734856489960E-14, 1421.486528603629949, 147.6332008705779799 ) ) ;
#17393=CYLINDRICAL_SURFACE ( 'NONE', #4414, 2.000000000000002220 ) ;
#17394=ADVANCED_FACE ( 'NONE', ( #5879 ), #72173, .F. ) ;
#17397=CARTESIAN_POINT ( 'NONE',  ( -14.52593930399999955, 1470.476261423729966, 229.9537273268980186 ) ) ;
#17402=ORIENTED_EDGE ( 'NONE', *, *, #100810, .T. ) ;
#17405=ORIENTED_EDGE ( 'NONE', *, *, #28400, .T. ) ;
#17406=CARTESIAN_POINT ( 'NONE',  ( 10.79382126600000014, 1414.913060387329779, 222.1041115775979904 ) ) ;
#17409=CARTESIAN_POINT ( 'NONE',  ( -14.30561690719999923, 1416.274718424630009, 221.5178275245980046 ) ) ;
#17410=CARTESIAN_POINT ( 'NONE',  ( -12.53517974735311391, 1442.773887286368335, 169.5044317858154272 ) ) ;
#17413=CARTESIAN_POINT ( 'NONE',  ( -4.627424403969999211, 1421.862729080530244, 185.4837249234980163 ) ) ;
#17416=CARTESIAN_POINT ( 'NONE',  ( -10.04683427352762592, 1410.638564451745424, 188.4446185365461872 ) ) ;
#17418=CARTESIAN_POINT ( 'NONE',  ( -15.77309112549999881, 1462.582351688929975, 223.0144108837980070 ) ) ;
#17419=CARTESIAN_POINT ( 'NONE',  ( 17.31926483839999875, 1459.104205613330123, 228.6771837914980097 ) ) ;
#17420=CARTESIAN_POINT ( 'NONE',  ( -15.13342374508840038, 1507.606285602760181, 191.8462590464540085 ) ) ;
#17421=CARTESIAN_POINT ( 'NONE',  ( 15.31719370542390024, 1507.616838218729754, 226.2466523219209762 ) ) ;
#17423=CARTESIAN_POINT ( 'NONE',  ( -2.499950770261460065, 1420.115583131989979, 90.95036697406219162 ) ) ;
#17425=CARTESIAN_POINT ( 'NONE',  ( 18.03232038437150209, 1424.487826474579833, 224.4511121296560248 ) ) ;
#17427=CARTESIAN_POINT ( 'NONE',  ( -2.897197017797513485, 1484.284914968770636, 183.3151737225298916 ) ) ;
#17433=CARTESIAN_POINT ( 'NONE',  ( -12.78654151568484210, 1416.818673872114459, 195.1663110372768983 ) ) ;
#17434=CARTESIAN_POINT ( 'NONE',  ( -11.76003987410000029, 1426.815402127429934, 145.7846991655979991 ) ) ;
#17436=CARTESIAN_POINT ( 'NONE',  ( -4.121463778139999867, 1441.582014689759944, 184.1216907019980340 ) ) ;
#17437=CARTESIAN_POINT ( 'NONE',  ( 11.86610049529999955, 1432.336025054189804, 149.9824163679980131 ) ) ;
#17438=CARTESIAN_POINT ( 'NONE',  ( 1.716045945209999868, 1509.007693206030126, 179.5167849949980052 ) ) ;
#17440=CARTESIAN_POINT ( 'NONE',  ( 12.37239278490000061, 1410.398668474930219, 228.8262060006979937 ) ) ;
#17441=CARTESIAN_POINT ( 'NONE',  ( -23.68957226320000231, 1508.007654220830091, 223.0814278728979900 ) ) ;
#17444=CARTESIAN_POINT ( 'NONE',  ( -16.17890917207000001, 1459.145060716636181, 230.7168571672029884 ) ) ;
#17447=CARTESIAN_POINT ( 'NONE',  ( 18.29857331400000220, 1408.824872542730191, 266.8292035143980456 ) ) ;
#17449=CARTESIAN_POINT ( 'NONE',  ( 19.68669136100000117, 1449.730997079720055, 193.0903452006980103 ) ) ;
#17450=CARTESIAN_POINT ( 'NONE',  ( -0.2075483795266540032, 1507.637022368109911, 237.3602291488149945 ) ) ;
#17452=FACE_OUTER_BOUND ( 'NONE', #68604, .T. ) ;
#17455=CARTESIAN_POINT ( 'NONE',  ( -13.49821838159999920, 1443.540395460420086, 187.3682244081979889 ) ) ;
#17456=CARTESIAN_POINT ( 'NONE',  ( -19.76034656259999878, 1519.913060387329779, 221.5779544268979748 ) ) ;
#17458=CARTESIAN_POINT ( 'NONE',  ( -2.674172889476567061, 1457.854889596452495, 229.5525240896329819 ) ) ;
#17461=CARTESIAN_POINT ( 'NONE',  ( -14.92043776882830031, 1409.434093555360050, 208.4812704053670132 ) ) ;
#17462=CIRCLE ( 'NONE', #80082, 1.999994602261522036 ) ;
#17465=CARTESIAN_POINT ( 'NONE',  ( -18.10264220770000065, 1472.346832327329821, 269.5453876878980282 ) ) ;
#17466=B_SPLINE_CURVE_WITH_KNOTS ( 'NONE', 3,
 ( #58402, #7431, #39938, #74108 ),
 .UNSPECIFIED., .F., .F.,
 ( 4, 4 ),
 ( -21.04897729589999855, -13.79090555186670031 ),
 .UNSPECIFIED. ) ;
#17469=CARTESIAN_POINT ( 'NONE',  ( -24.29629205419795923, 1444.606322822562333, 211.3000715094191264 ) ) ;
#17472=CARTESIAN_POINT ( 'NONE',  ( 18.03020053570940107, 1424.665392966000127, 225.2865191207559690 ) ) ;
#17474=CARTESIAN_POINT ( 'NONE',  ( -6.620521211799999861, 1440.451554611820029, 154.8188655977980090 ) ) ;
#17479=CARTESIAN_POINT ( 'NONE',  ( -23.27028561550000063, 1410.220846923830095, 206.2737248513280122 ) ) ;
#17484=EDGE_CURVE ( 'NONE', #90113, #28026, #80613, .T. ) ;
#17489=CARTESIAN_POINT ( 'NONE',  ( -22.12673812610000112, 1409.685743109030000, 209.8966867356670036 ) ) ;
#17491=CARTESIAN_POINT ( 'NONE',  ( 11.71754611134989865, 1426.708450837530108, 142.7745908721059891 ) ) ;
#17495=CARTESIAN_POINT ( 'NONE',  ( -0.02428268839107049909, 1420.196391110329841, 183.9091636877150222 ) ) ;
#17498=CARTESIAN_POINT ( 'NONE',  ( -0.9520131522009163128, 1397.942409892914839, 222.1218459635456099 ) ) ;
#17499=CARTESIAN_POINT ( 'NONE',  ( -3.484680539907339281, 1440.761655002041607, 156.7439059081135042 ) ) ;
#17501=CARTESIAN_POINT ( 'NONE',  ( 1.399923991030000092, 1507.072109554030021, 236.8180446778980013 ) ) ;
#17508=CARTESIAN_POINT ( 'NONE',  ( 11.94196968702019923, 1433.494760352820094, 149.8932996039710019 ) ) ;
#17510=ORIENTED_EDGE ( 'NONE', *, *, #110394, .F. ) ;
#17512=CARTESIAN_POINT ( 'NONE',  ( -22.97499040840000006, 1509.490920569430045, 193.4133551238979862 ) ) ;
#17515=CARTESIAN_POINT ( 'NONE',  ( 2.368833328420000051, 1427.018531676430030, 133.6118001900980232 ) ) ;
#17516=CARTESIAN_POINT ( 'NONE',  ( 13.05116814624009969, 1498.106535309839956, 232.7503740319400265 ) ) ;
#17517=CARTESIAN_POINT ( 'NONE',  ( 7.424385365560000061, 1507.634762273629804, 182.7152872762979996 ) ) ;
#17519=CARTESIAN_POINT ( 'NONE',  ( 15.94344812639999631, 1409.469817864229981, 225.2684562213980257 ) ) ;
#17521=CARTESIAN_POINT ( 'NONE',  ( 4.809053151022830264, 1396.080996231650033, 199.1914258291379838 ) ) ;
#17522=CARTESIAN_POINT ( 'NONE',  ( 14.27868134601139971, 1415.948038442740199, 197.0356935349670096 ) ) ;
#17523=CARTESIAN_POINT ( 'NONE',  ( 11.56039809610000013, 1431.104951558719904, 151.0881388422979796 ) ) ;
#17525=ORIENTED_EDGE ( 'NONE', *, *, #28225, .T. ) ;
#17526=CARTESIAN_POINT ( 'NONE',  ( 13.76767358908210070, 1435.930931524279913, 150.2736258322640026 ) ) ;
#17529=CARTESIAN_POINT ( 'NONE',  ( 13.01250632543007235, 1444.867273317868239, 169.4194736224069686 ) ) ;
#17530=CARTESIAN_POINT ( 'NONE',  ( -1.528923355689999930, 1467.018653446829831, 235.3777442162979980 ) ) ;
#17531=AXIS2_PLACEMENT_3D ( 'NONE', #98076, #97537, #55008 ) ;
#17536=EDGE_CURVE ( 'NONE', #88847, #76760, #43648, .T. ) ;
#17544=CARTESIAN_POINT ( 'NONE',  ( 22.79168776688370102, 1440.913060387330006, 230.8904766920060183 ) ) ;
#17546=ORIENTED_EDGE ( 'NONE', *, *, #102850, .F. ) ;
#17547=CARTESIAN_POINT ( 'NONE',  ( -11.49135376729999969, 1409.816935674130036, 189.2372629410979812 ) ) ;
#17551=CARTESIAN_POINT ( 'NONE',  ( 24.58510744930000058, 1439.552595424130232, 212.5220241814980113 ) ) ;
#17552=DIRECTION ( 'NONE',  ( 0.000000000000000000, -0.7071067811865474617, -0.7071067811865474617 ) ) ;
#17555=DIRECTION ( 'NONE',  ( -0.8564730265368828421, -0.5161917810414575758, 0.000000000000000000 ) ) ;
#17556=CARTESIAN_POINT ( 'NONE',  ( 10.81506866283119983, 1424.921186100899831, 144.1620444812269852 ) ) ;
#17557=AXIS2_PLACEMENT_3D ( 'NONE', #91880, #67805, #16250 ) ;
#17560=CARTESIAN_POINT ( 'NONE',  ( -21.80461142280000075, 1509.640046815429741, 189.9822974792980119 ) ) ;
#17565=CARTESIAN_POINT ( 'NONE',  ( -17.17023220410861128, 1486.131980952480262, 187.8222342393189876 ) ) ;
#17568=VERTEX_POINT ( 'NONE', #70793 ) ;
#17570=CARTESIAN_POINT ( 'NONE',  ( 32.03901053310000435, 1451.703008376129901, 250.0966427451979825 ) ) ;
#17571=CARTESIAN_POINT ( 'NONE',  ( 2.923658500830763174, 1451.704853250206725, 183.8662944852202656 ) ) ;
#17572=CARTESIAN_POINT ( 'NONE',  ( -11.76598840989999850, 1428.979790717830156, 145.3128034382980047 ) ) ;
#17573=CARTESIAN_POINT ( 'NONE',  ( -7.229470473417760168, 1509.092253499190065, 236.9801883832320186 ) ) ;
#17576=CARTESIAN_POINT ( 'NONE',  ( 17.99263301768839796, 1410.773178293809906, 222.9786793883430107 ) ) ;
#17580=EDGE_LOOP ( 'NONE', ( #53232, #59934, #70429, #16599 ) ) ;
#17583=CARTESIAN_POINT ( 'NONE',  ( 29.19056935439999734, 1509.932417531129886, 206.4260805152879925 ) ) ;
#17584=B_SPLINE_CURVE_WITH_KNOTS ( 'NONE', 5,
 ( #11378, #45550, #79690, #2995, #37116, #71316 ),
 .UNSPECIFIED., .F., .F.,
 ( 6, 6 ),
 ( -17.01656662094779904, -6.621488669319999687 ),
 .UNSPECIFIED. ) ;
#17585=B_SPLINE_CURVE_WITH_KNOTS ( 'NONE', 3,
 ( #88229, #12617, #27759, #46796, #28872, #79834, #53538, #11520, #87684, #69794, #45696, #45139, #79280, #3140, #105587, #97168, #30513, #108329, #55750, #90408, #81451, #74741, #108879, #23206, #56277, #89869, #98267, #83128, #4224, #56833, #64148, #40570, #23757, #39475, #49544, #4757, #38901, #6425, #32171, #73083, #107223, #82011, #38356, #13138, #31612, #5875, #15350, #29955, #73645, #13687, #72535, #57406, #65789, #99910, #91531, #82584, #5316, #64702, #98819, #106665, #21538, #14809, #22081, #65242, #47322, #66356, #40018, #48995, #22628, #100475, #57944, #92076, #74197, #47873, #107776, #31061, #99354, #48446, #90967, #14256, #109988, #93707 ),
 .UNSPECIFIED., .F., .F.,
 ( 4, 2, 2, 1, 1, 1, 1, 2, 2, 2, 2, 1, 1, 1, 1, 1, 1, 2, 2, 2, 2, 2, 1, 1, 1, 1, 1, 1, 2, 2, 2, 2, 2, 2, 2, 1, 1, 1, 1, 1, 2, 2, 2, 2, 2, 1, 1, 1, 1, 1, 2, 2, 2, 4 ),
 ( 0.000000000000000000, 0.06249999999689971608, 0.09374999999534959494, 0.1093749999945813761, 0.1171874999941906192, 0.1210937499939952339, 0.1230468749938975065, 0.1240234374938485873, 0.1249999999937996542, 0.1874999999902269010, 0.2187499999884405799, 0.2343749999875474055, 0.2421874999870951839, 0.2460937499868637024, 0.2480468749867425493, 0.2490234374866871769, 0.2495117187366648337, 0.2497558593616537037, 0.2499999999866426015, 0.3124999999868266487, 0.3437499999869187972, 0.3593749999869604861, 0.3671874999869813583, 0.3710937499869957357, 0.3730468749870029521, 0.3740234374870101686, 0.3745117187370138323, 0.3747558593620157197, 0.3748779296745202716, 0.3749999999870247680, 0.4062499999879649049, 0.4374999999889049862, 0.4687499999898450675, 0.4843749999903206871, 0.4921874999905507253, 0.4960937499906657999, 0.4980468749907230319, 0.4990234374907395187, 0.4995117187407349668, 0.4997558593657326909, 0.4998779296782312476, 0.4999999999907298598, 0.6249999999927761118, 0.6874999999937994044, 0.7187499999943091078, 0.7343749999945639040, 0.7421874999946894702, 0.7460937499947539742, 0.7480468749947879470, 0.7490234374948067098, 0.7495117187448160356, 0.7499999999948252505, 0.8749999999974127363, 1.000000000000000000 ),
 .UNSPECIFIED. ) ;
#17586=CARTESIAN_POINT ( 'NONE',  ( 24.51094252870000290, 1443.736757004859783, 213.5018118478279803 ) ) ;
#17589=CARTESIAN_POINT ( 'NONE',  ( -20.01067139950000140, 1507.877425041529932, 188.9709217985979706 ) ) ;
#17590=CARTESIAN_POINT ( 'NONE',  ( 28.39357473329010162, 1435.648819368660043, 136.1155384844830110 ) ) ;
#17591=CARTESIAN_POINT ( 'NONE',  ( 35.47922246755190656, 1450.191545858459904, 136.2330231413669708 ) ) ;
#17592=CARTESIAN_POINT ( 'NONE',  ( 3.199222159840339634E-15, 1458.117154428349977, 230.2906725803670156 ) ) ;
#17599=CARTESIAN_POINT ( 'NONE',  ( 3.418717339140886935, 1426.008825658123897, 185.1440916679583211 ) ) ;
#17601=DIRECTION ( 'NONE',  ( -0.06436433998257497235, -0.7055452152167080992, -0.7057359145058558214 ) ) ;
#17602=CARTESIAN_POINT ( 'NONE',  ( -0.4362016210640000113, 1416.994873689529868, 234.1618458712980271 ) ) ;
#17605=CARTESIAN_POINT ( 'NONE',  ( -28.49020455409999997, 1509.161987687429928, 209.1271010973100033 ) ) ;
#17608=CARTESIAN_POINT ( 'NONE',  ( -12.49434536646978700, 1419.335010250987580, 228.5375418321167444 ) ) ;
#17609=CARTESIAN_POINT ( 'NONE',  ( -21.04449625164730620, 1450.946923703476841, 144.4076044022301062 ) ) ;
#17611=CARTESIAN_POINT ( 'NONE',  ( 24.42260775900000169, 1435.425039144950233, 136.9350572207980008 ) ) ;
#17612=CARTESIAN_POINT ( 'NONE',  ( -8.592347709929391897, 1396.213111781930138, 202.1620628003519755 ) ) ;
#17615=CARTESIAN_POINT ( 'NONE',  ( 5.001772368710000194, 1443.913060387330006, 150.4106346902979965 ) ) ;
#17616=ORIENTED_EDGE ( 'NONE', *, *, #51379, .F. ) ;
#17617=EDGE_LOOP ( 'NONE', ( #4364, #82032, #102768, #3410 ) ) ;
#17620=CARTESIAN_POINT ( 'NONE',  ( 11.01624074439999923, 1426.516487655429955, 91.92649746769789942 ) ) ;
#17622=CARTESIAN_POINT ( 'NONE',  ( -10.98083652350000072, 1433.016921829010016, 151.7694308519979813 ) ) ;
#17623=CARTESIAN_POINT ( 'NONE',  ( -2.529134858577002376, 1420.903940735018068, 185.4090734218341936 ) ) ;
#17627=CARTESIAN_POINT ( 'NONE',  ( 7.976840964510000020, 1508.678916850730047, 182.3492935605979994 ) ) ;
#17628=CARTESIAN_POINT ( 'NONE',  ( 3.451567150219999824, 1449.151155894430076, 184.0761302567979953 ) ) ;
#17631=CARTESIAN_POINT ( 'NONE',  ( -4.469061752933077614, 1464.606722936262031, 237.1332386249960678 ) ) ;
#17632=VERTEX_POINT ( 'NONE', #95402 ) ;
#17635=CARTESIAN_POINT ( 'NONE',  ( -40.26734664479999282, 1444.073158352789960, 137.1206983653979989 ) ) ;
#17636=CIRCLE ( 'NONE', #48048, 1.999235054590136507 ) ;
#17638=CARTESIAN_POINT ( 'NONE',  ( -1.469869910310000138, 1473.882853011830093, 270.2923612834979963 ) ) ;
#17641=CARTESIAN_POINT ( 'NONE',  ( -2.048334170740000015, 1486.024116770630144, 181.9733265186980020 ) ) ;
#17645=CARTESIAN_POINT ( 'NONE',  ( 12.27023112330000032, 1416.839692136459917, 223.5796784318309847 ) ) ;
#17647=CARTESIAN_POINT ( 'NONE',  ( -22.59376922909999763, 1497.713060387329961, 208.1432028049030123 ) ) ;
#17649=CARTESIAN_POINT ( 'NONE',  ( 9.029008260723980328, 1407.892909937350169, 198.8844728701529903 ) ) ;
#17650=CARTESIAN_POINT ( 'NONE',  ( -10.65237148710020065, 1406.670964572119829, 267.4893520522770132 ) ) ;
#17651=CARTESIAN_POINT ( 'NONE',  ( -14.38141623268059988, 1435.876664363790042, 149.8601871492290059 ) ) ;
#17653=CARTESIAN_POINT ( 'NONE',  ( -11.76966145709999978, 1432.350018154589861, 150.8118972717979887 ) ) ;
#17654=CARTESIAN_POINT ( 'NONE',  ( 13.85488084099999995, 1444.703314923880043, 189.1754263215979961 ) ) ;
#17657=CARTESIAN_POINT ( 'NONE',  ( 4.966635725421030934, 1423.255510328363698, 184.3056371891483138 ) ) ;
#17659=CIRCLE ( 'NONE', #80288, 1.999999999999967581 ) ;
#17661=CARTESIAN_POINT ( 'NONE',  ( -12.53056552249999989, 1470.463356747030048, 186.5986695887980034 ) ) ;
#17664=CARTESIAN_POINT ( 'NONE',  ( 9.257694918409999474, 1414.913060387329779, 222.9570521072979830 ) ) ;
#17666=B_SPLINE_CURVE_WITH_KNOTS ( 'NONE', 5,
 ( #77398, #700, #35387, #93614, #52755, #77940, #94737, #8515, #103121 ),
 .UNSPECIFIED., .F., .F.,
 ( 6, 3, 6 ),
 ( 0.000000000000000000, 0.4999964934256276861, 1.000000000000000000 ),
 .UNSPECIFIED. ) ;
#17667=CARTESIAN_POINT ( 'NONE',  ( -29.63837353179999923, 1509.975889270829839, 207.4461348473880093 ) ) ;
#17668=CARTESIAN_POINT ( 'NONE',  ( -4.649632279085039954, 1420.176633138330089, 186.4708453798239987 ) ) ;
#17671=CARTESIAN_POINT ( 'NONE',  ( 2.789446250490000126E-08, 1406.911841291630253, 196.1218459601980157 ) ) ;
#17673=CARTESIAN_POINT ( 'NONE',  ( -4.058567207959999479, 1447.362832675280060, 184.9425281217980057 ) ) ;
#17674=EDGE_LOOP ( 'NONE', ( #87517, #86696, #16813, #46362 ) ) ;
#17676=CARTESIAN_POINT ( 'NONE',  ( 26.42702185389999769, 1508.126183422229815, 216.5535634561180132 ) ) ;
#17677=CARTESIAN_POINT ( 'NONE',  ( 20.23159575734240079, 1487.448372438290107, 225.6309448190939975 ) ) ;
#17678=CARTESIAN_POINT ( 'NONE',  ( -25.92882744109999749, 1435.924328612949921, 136.6037266722979950 ) ) ;
#17683=CARTESIAN_POINT ( 'NONE',  ( 2.500000000000000000, 1438.463317487690119, 157.6994634259980046 ) ) ;
#17690=CARTESIAN_POINT ( 'NONE',  ( 12.22638525410440025, 1434.267039502970192, 150.2713860696590018 ) ) ;
#17691=B_SPLINE_SURFACE_WITH_KNOTS ( 'NONE', 5, 5, ( 
 ( #45067, #27688, #53461, #54030, #87606, #10893, #4152, #78643, #79210 ),
 ( #29330, #62994, #28237, #55667, #89243, #62425, #45622, #12539, #1958 ),
 ( #46172, #88158, #79761, #3068, #46718, #80849, #38279, #97102, #20368 ),
 ( #72462, #98186, #21457, #39942, #41035, #6338, #13608, #38826, #47796 ),
 ( #108798, #30983, #64619, #23679, #32091, #22000, #65158, #73005, #15267 ),
 ( #14174, #49459, #48359, #66820, #89790, #57863, #81932, #56194, #90329 ) ),
 .UNSPECIFIED., .F., .F., .F.,
 ( 6, 6 ),
 ( 6, 3, 6 ),
 ( 9.945329370599239382, 12.20377897060000016 ),
 ( 0.000000000000000000, 1.000000000000000000, 2.000000000000000000 ),
 .UNSPECIFIED. ) ;
#17692=CARTESIAN_POINT ( 'NONE',  ( 18.08821306226149872, 1459.310247305569874, 227.9716307757270215 ) ) ;
#17693=CARTESIAN_POINT ( 'NONE',  ( -24.27332534947139919, 1509.087562220649943, 222.4402390272340142 ) ) ;
#17694=CARTESIAN_POINT ( 'NONE',  ( -2.923521586279999696, 1410.394928897130058, 186.6127580804979971 ) ) ;
#17696=CARTESIAN_POINT ( 'NONE',  ( 4.236872543330679974, 1441.473390915530217, 163.4512186758819894 ) ) ;
#17697=B_SPLINE_CURVE_WITH_KNOTS ( 'NONE', 5,
 ( #105876, #31348, #50384, #59885, #23497, #84512 ),
 .UNSPECIFIED., .F., .F.,
 ( 6, 6 ),
 ( 0.000000000000000000, 0.03026097244042860734 ),
 .UNSPECIFIED. ) ;
#17699=CARTESIAN_POINT ( 'NONE',  ( -3.969564362200000307, 1421.142701091429899, 186.0775239138980055 ) ) ;
#17700=CARTESIAN_POINT ( 'NONE',  ( 20.18532048049999972, 1508.602711282329892, 189.1193814760979990 ) ) ;
#17702=ORIENTED_EDGE ( 'NONE', *, *, #49035, .T. ) ;
#17703=CARTESIAN_POINT ( 'NONE',  ( -12.61566556969999908, 1416.819759739430083, 194.9201884166980108 ) ) ;
#17706=ORIENTED_EDGE ( 'NONE', *, *, #12497, .F. ) ;
#17708=CARTESIAN_POINT ( 'NONE',  ( 4.132092042950000099, 1421.241915939129967, 185.3693087620980009 ) ) ;
#17715=CARTESIAN_POINT ( 'NONE',  ( 17.54299231450000107, 1415.063410489729904, 210.2814835228880099 ) ) ;
#17716=CARTESIAN_POINT ( 'NONE',  ( 19.48178958320507093, 1507.796605003039531, 229.4922759112947972 ) ) ;
#17717=CARTESIAN_POINT ( 'NONE',  ( -8.881784196999999612E-15, 1443.913060387330006, 126.8032249175980155 ) ) ;
#17719=CARTESIAN_POINT ( 'NONE',  ( 38.46602011401969889, 1440.913060379879880, 257.0153466912190083 ) ) ;
#17724=CARTESIAN_POINT ( 'NONE',  ( 14.24685689828609902, 1473.184890486440054, 194.3436051322440221 ) ) ;
#17725=CARTESIAN_POINT ( 'NONE',  ( 25.36184121639999844, 1469.165572951930244, 206.9791411554380147 ) ) ;
#17726=CARTESIAN_POINT ( 'NONE',  ( -24.41225618889999893, 1441.001746037479961, 212.0330686186080129 ) ) ;
#17727=CARTESIAN_POINT ( 'NONE',  ( 4.547831559409852176, 1410.447768422028275, 186.2153058587292094 ) ) ;
#17730=CARTESIAN_POINT ( 'NONE',  ( -11.82552473729999853, 1507.579552363830089, 183.2239286378979841 ) ) ;
#17731=CARTESIAN_POINT ( 'NONE',  ( -22.81224805166159797, 1509.788088251490080, 188.7721076916159859 ) ) ;
#17733=CARTESIAN_POINT ( 'NONE',  ( 13.10647016826960076, 1414.913527292460003, 198.0560097828689834 ) ) ;
#17736=CARTESIAN_POINT ( 'NONE',  ( -26.87217695997193800, 1508.240762366635636, 212.0141957947051026 ) ) ;
#17738=CARTESIAN_POINT ( 'NONE',  ( 0.000000000000000000, 1450.913060387330006, 187.0476703040980055 ) ) ;
#17740=CARTESIAN_POINT ( 'NONE',  ( -18.09679206583593469, 1459.548717300706812, 227.9697539532586461 ) ) ;
#17743=CARTESIAN_POINT ( 'NONE',  ( -0.5172272512948579148, 1416.765894075033202, 233.9543648737588626 ) ) ;
#17744=EDGE_LOOP ( 'NONE', ( #6242, #12513, #77862, #2726, #40777, #12296, #51252, #49927, #75500, #10643, #99614, #33415 ) ) ;
#17746=CARTESIAN_POINT ( 'NONE',  ( 19.43393205732160212, 1509.529646666910139, 230.8600434984439858 ) ) ;
#17748=CARTESIAN_POINT ( 'NONE',  ( 40.22348776513499757, 1442.812490084199908, 137.0237541975089925 ) ) ;
#17749=CARTESIAN_POINT ( 'NONE',  ( 9.580271555476294054, 1411.182622053547220, 269.3463862739754404 ) ) ;
#17750=CARTESIAN_POINT ( 'NONE',  ( -20.04379992670000377, 1471.636457544530003, 264.7217083835980134 ) ) ;
#17753=CARTESIAN_POINT ( 'NONE',  ( -11.72537676174745513, 1435.130261367574121, 151.3178099432534225 ) ) ;
#17754=CARTESIAN_POINT ( 'NONE',  ( -19.85061890739999768, 1484.702845893429867, 190.8243287402979718 ) ) ;
#17755=CARTESIAN_POINT ( 'NONE',  ( 1.129978713339999885, 1408.952520113529999, 186.6978219804979915 ) ) ;
#17757=CARTESIAN_POINT ( 'NONE',  ( -11.70596046909999899, 1435.783534794500156, 151.4055864423979756 ) ) ;
#17758=CARTESIAN_POINT ( 'NONE',  ( 11.53918857109999863, 1434.258397247200037, 151.3471602487979908 ) ) ;
#17760=CARTESIAN_POINT ( 'NONE',  ( -23.02752199190000226, 1452.108921600530039, 139.9703293178979777 ) ) ;
#17761=CARTESIAN_POINT ( 'NONE',  ( 1.283858640530000095, 1464.947442259230002, 237.5396736328980296 ) ) ;
#17765=CARTESIAN_POINT ( 'NONE',  ( -44.93136296710000011, 1440.913060597359845, 269.6838063816980480 ) ) ;
#17766=CARTESIAN_POINT ( 'NONE',  ( -4.311053961940764623, 1407.085547473677934, 196.6635586998287977 ) ) ;
#17767=CARTESIAN_POINT ( 'NONE',  ( 17.59268578599999699, 1410.455475235630047, 224.1775087684979724 ) ) ;
#17771=CARTESIAN_POINT ( 'NONE',  ( 2.927313424399410113, 1410.174542261320084, 231.6044306003970235 ) ) ;
#17772=CARTESIAN_POINT ( 'NONE',  ( -0.9667867126420001123, 1415.996778984329922, 227.8322076899980004 ) ) ;
#17774=CARTESIAN_POINT ( 'NONE',  ( -8.587497642409999798, 1419.088922007130122, 232.7581010276980180 ) ) ;
#17778=B_SPLINE_CURVE_WITH_KNOTS ( 'NONE', 5,
 ( #95100, #17803, #60975, #35188, #9988, #18366 ),
 .UNSPECIFIED., .F., .F.,
 ( 6, 6 ),
 ( -167.7881597310000075, -30.40382300159998863 ),
 .UNSPECIFIED. ) ;
#17780=CARTESIAN_POINT ( 'NONE',  ( -46.00060696795689807, 1439.228690553249862, 266.6786537750060120 ) ) ;
#17781=CARTESIAN_POINT ( 'NONE',  ( -2.499999999940000439, 1436.903610872740273, 184.2102826205979795 ) ) ;
#17786=CARTESIAN_POINT ( 'NONE',  ( -5.411782914500000707, 1435.306182108309940, 154.6725736572979883 ) ) ;
#17787=CARTESIAN_POINT ( 'NONE',  ( 19.27955013568295328, 1456.451286679076929, 224.7795789275638185 ) ) ;
#17790=CARTESIAN_POINT ( 'NONE',  ( -26.88878276533139910, 1451.048910818290096, 136.3593413721419836 ) ) ;
#17792=CARTESIAN_POINT ( 'NONE',  ( -16.68455607539956986, 1409.595982907923371, 225.3198891662985375 ) ) ;
#17794=CARTESIAN_POINT ( 'NONE',  ( 15.10313800449999988, 1488.809466529130077, 194.0858732079979916 ) ) ;
#17795=CARTESIAN_POINT ( 'NONE',  ( 11.60004869885203682, 1423.462004151896508, 135.7646869108323244 ) ) ;
#17799=ORIENTED_EDGE ( 'NONE', *, *, #36340, .F. ) ;
#17800=CARTESIAN_POINT ( 'NONE',  ( -1.200210185686839903, 1410.247648972750085, 269.6150193402980335 ) ) ;
#17802=CARTESIAN_POINT ( 'NONE',  ( 10.94784056215000057, 1419.904943497329896, 232.1968281718800142 ) ) ;
#17803=CARTESIAN_POINT ( 'NONE',  ( -19.99769045190000227, 1488.355546399329796, 191.5584535652979810 ) ) ;
#17804=CARTESIAN_POINT ( 'NONE',  ( -2.500000000000000000, 1439.435444884669778, 162.3942738332719955 ) ) ;
#17805=ORIENTED_EDGE ( 'NONE', *, *, #80504, .F. ) ;
#17807=CARTESIAN_POINT ( 'NONE',  ( -23.32570769421149848, 1410.008417559419968, 209.9356539553859875 ) ) ;
#17808=EDGE_CURVE ( 'NONE', #29004, #105413, #107172, .T. ) ;
#17809=CARTESIAN_POINT ( 'NONE',  ( -0.2759417911574060245, 1410.303294818389986, 185.0234033110549774 ) ) ;
#17811=CIRCLE ( 'NONE', #14240, 1.000000000000000000 ) ;
#17812=DIRECTION ( 'NONE',  ( 0.03489949670250328678, 0.9993908270190956511, 0.000000000000000000 ) ) ;
#17813=CARTESIAN_POINT ( 'NONE',  ( -18.85961944716780181, 1416.512142023939987, 207.5743260399690087 ) ) ;
#17814=CARTESIAN_POINT ( 'NONE',  ( -22.08220418359999826, 1420.825048654430020, 216.4967283580180037 ) ) ;
#17815=CARTESIAN_POINT ( 'NONE',  ( 29.68528746673739960, 1466.931583989530054, 269.3634784496489942 ) ) ;
#17817=CARTESIAN_POINT ( 'NONE',  ( -16.87601176900255595, 1421.848452965002934, 226.8668675059429631 ) ) ;
#17820=CARTESIAN_POINT ( 'NONE',  ( 18.94390663599199343, 1457.575929578803880, 226.8085174276290275 ) ) ;
#17821=CARTESIAN_POINT ( 'NONE',  ( 1.495889316277259962, 1468.096849455099800, 182.8155357973550110 ) ) ;
#17822=CARTESIAN_POINT ( 'NONE',  ( 22.85539255169999606, 1409.737614192629962, 208.6607040618730196 ) ) ;
#17825=CARTESIAN_POINT ( 'NONE',  ( 26.47933087948679898, 1450.735437991490016, 136.5163285050169861 ) ) ;
#17829=CARTESIAN_POINT ( 'NONE',  ( 17.60733967200000194, 1409.692916845429863, 193.8802571657980138 ) ) ;
#17832=CARTESIAN_POINT ( 'NONE',  ( 27.23063139319997816, 1444.324653571829003, 161.8596747266978753 ) ) ;
#17833=CARTESIAN_POINT ( 'NONE',  ( 2.554988275568651712, 1439.637233825041221, 183.2488012791049812 ) ) ;
#17834=CARTESIAN_POINT ( 'NONE',  ( 1.950421698860000053, 1417.553803591129963, 234.0318042942980128 ) ) ;
#17835=CARTESIAN_POINT ( 'NONE',  ( -22.38744152929581333, 1431.163389416910832, 216.9216883821636941 ) ) ;
#17839=CARTESIAN_POINT ( 'NONE',  ( 16.90742456150000095, 1444.994950788469851, 162.4348202098979925 ) ) ;
#17840=EDGE_LOOP ( 'NONE', ( #31950, #102446, #19374, #60827 ) ) ;
#17841=CARTESIAN_POINT ( 'NONE',  ( 11.84669589606929918, 1415.088506334920112, 221.4079050929989876 ) ) ;
#17843=CARTESIAN_POINT ( 'NONE',  ( -0.3445723587089969953, 1409.016293610590083, 232.2535758655419897 ) ) ;
#17846=EDGE_CURVE ( 'NONE', #22768, #103324, #12374, .T. ) ;
#17850=CARTESIAN_POINT ( 'NONE',  ( -26.42714720800000094, 1440.913060387330006, 243.9198229517980110 ) ) ;
#17852=CARTESIAN_POINT ( 'NONE',  ( -21.95218091425238782, 1509.537469399167094, 191.3967133988915919 ) ) ;
#17854=CARTESIAN_POINT ( 'NONE',  ( 11.88531770350000016, 1433.194006408179803, 149.9681147489979764 ) ) ;
#17855=CARTESIAN_POINT ( 'NONE',  ( 9.019386504720001696, 1461.887471368730075, 248.0989693021979861 ) ) ;
#17856=B_SPLINE_SURFACE_WITH_KNOTS ( 'NONE', 5, 5, ( 
 ( #23445, #24535, #16134, #50341, #84466, #1041 ),
 ( #36827, #17781, #36270, #18345, #9417, #104581 ),
 ( #52536, #104022, #18897, #70460, #35163, #53656 ),
 ( #26198, #27876, #94507, #53092, #68799, #43579 ),
 ( #62057, #78270, #102900, #9965, #60386, #71017 ),
 ( #95079, #87801, #77728, #34613, #61498, #87231 ) ),
 .UNSPECIFIED., .F., .F., .F.,
 ( 6, 6 ),
 ( 6, 6 ),
 ( 86.05908199089999755, 105.4335682549999973 ),
 ( 0.000000000000000000, 2.000000000000000000 ),
 .UNSPECIFIED. ) ;
#17857=CARTESIAN_POINT ( 'NONE',  ( 11.22084002889469900, 1414.913060387399810, 197.6243765041139966 ) ) ;
#17863=EDGE_CURVE ( 'NONE', #53899, #20182, #65740, .T. ) ;
#17864=CARTESIAN_POINT ( 'NONE',  ( 22.57319362359999815, 1409.701316935530031, 208.7927549349429910 ) ) ;
#17865=CARTESIAN_POINT ( 'NONE',  ( 10.12919404300857451, 1398.213353175035536, 200.9395953525430230 ) ) ;
#17866=CARTESIAN_POINT ( 'NONE',  ( -27.81315569556840117, 1509.884315111430169, 222.3141242500419992 ) ) ;
#17870=CARTESIAN_POINT ( 'NONE',  ( -8.482731032629999390, 1508.704755829329770, 235.6989776125980143 ) ) ;
#17876=CARTESIAN_POINT ( 'NONE',  ( 0.1601303935690119862, 1486.188272806359919, 181.8285171723719884 ) ) ;
#17879=FACE_OUTER_BOUND ( 'NONE', #82163, .T. ) ;
#17881=CARTESIAN_POINT ( 'NONE',  ( 12.91284616039999911, 1434.774386575559902, 149.6994772678979757 ) ) ;
#17884=ORIENTED_EDGE ( 'NONE', *, *, #6296, .F. ) ;
#17885=CARTESIAN_POINT ( 'NONE',  ( -38.64637139473789773, 1443.913060387190171, 137.1864063576500143 ) ) ;
#17886=EDGE_CURVE ( 'NONE', #44597, #1439, #99235, .T. ) ;
#17888=CARTESIAN_POINT ( 'NONE',  ( -13.24264662000000037, 1414.971439108430104, 220.7226513867979918 ) ) ;
#17889=CARTESIAN_POINT ( 'NONE',  ( 11.58492313561834131, 1426.183940868015270, 138.6952717246431064 ) ) ;
#17892=CARTESIAN_POINT ( 'NONE',  ( -1.353902514868472462, 1408.960339704959324, 187.6075962084191531 ) ) ;
#17893=CARTESIAN_POINT ( 'NONE',  ( 2.833799216370230134, 1466.651268623249734, 236.4511971046459848 ) ) ;
#17894=B_SPLINE_CURVE_WITH_KNOTS ( 'NONE', 3,
 ( #48324, #90849, #99236, #84100 ),
 .UNSPECIFIED., .F., .F.,
 ( 4, 4 ),
 ( 0.000000000000000000, 1.000000000000000000 ),
 .UNSPECIFIED. ) ;
#17898=CARTESIAN_POINT ( 'NONE',  ( -16.72903711220000034, 1412.957917587729980, 191.6790723950980180 ) ) ;
#17900=ORIENTED_EDGE ( 'NONE', *, *, #93344, .T. ) ;
#17902=CARTESIAN_POINT ( 'NONE',  ( -15.76858003950689913, 1409.463696000809932, 225.2883378276359849 ) ) ;
#17911=CARTESIAN_POINT ( 'NONE',  ( 41.28234918735198278, 1446.727361558453140, 269.6338958528504008 ) ) ;
#17913=CARTESIAN_POINT ( 'NONE',  ( 17.73602759646932370, 1434.477616020383493, 215.8487880863369810 ) ) ;
#17916=CARTESIAN_POINT ( 'NONE',  ( -12.01638156518240130, 1440.881463477919851, 187.8051726210379968 ) ) ;
#17920=CARTESIAN_POINT ( 'NONE',  ( 2.710413740429999940, 1447.398501226639837, 159.5173025968979914 ) ) ;
#17921=CARTESIAN_POINT ( 'NONE',  ( -2.500000000000000000, 1435.233731004240099, 157.5834550647980166 ) ) ;
#17922=CARTESIAN_POINT ( 'NONE',  ( 14.20165754500000155, 1416.819759739430083, 196.5061803919979866 ) ) ;
#17926=CARTESIAN_POINT ( 'NONE',  ( -33.92723093277399471, 1436.576986543423800, 136.5095885520893546 ) ) ;
#17927=VERTEX_POINT ( 'NONE', #68986 ) ;
#17928=CARTESIAN_POINT ( 'NONE',  ( 13.60516184949999996, 1408.134943172929979, 264.8398108144980370 ) ) ;
#17929=CARTESIAN_POINT ( 'NONE',  ( -24.42679094869999901, 1430.357408120730270, 206.6252289346280122 ) ) ;
#17930=CARTESIAN_POINT ( 'NONE',  ( -11.42728233630000112, 1426.866742535030198, 121.9076973341980050 ) ) ;
#17931=CARTESIAN_POINT ( 'NONE',  ( 16.36894064783199809, 1409.509743440080001, 192.9694638889519922 ) ) ;
#17934=CARTESIAN_POINT ( 'NONE',  ( 28.92450383220691990, 1510.034133629718781, 217.1252577293115280 ) ) ;
#17937=FACE_OUTER_BOUND ( 'NONE', #8058, .T. ) ;
#17941=CARTESIAN_POINT ( 'NONE',  ( -35.33152177045790410, 1437.220631632869981, 136.5361142770269964 ) ) ;
#17942=EDGE_LOOP ( 'NONE', ( #6695, #77884, #38620, #29366, #110625 ) ) ;
#17943=CARTESIAN_POINT ( 'NONE',  ( 9.694919637589999084, 1396.311071599129946, 201.2694852162679808 ) ) ;
#17945=CARTESIAN_POINT ( 'NONE',  ( -18.12928259929999797, 1459.009197536229976, 227.9558348735980076 ) ) ;
#17946=EDGE_LOOP ( 'NONE', ( #63319, #37943, #104856, #88261 ) ) ;
#17948=CARTESIAN_POINT ( 'NONE',  ( -29.22959469711409852, 1509.933780326070064, 211.7723416727030212 ) ) ;
#17949=CARTESIAN_POINT ( 'NONE',  ( -11.73563908010000034, 1425.610159190430068, 144.1657657165980027 ) ) ;
#17955=CARTESIAN_POINT ( 'NONE',  ( -11.87174114537739911, 1432.759493913710003, 149.9813063557689929 ) ) ;
#17956=CARTESIAN_POINT ( 'NONE',  ( -15.62061836090000000, 1461.188395550129826, 228.5769436422980050 ) ) ;
#17962=ORIENTED_EDGE ( 'NONE', *, *, #97292, .T. ) ;
#17966=CARTESIAN_POINT ( 'NONE',  ( 11.81696617721230069, 1429.121889755289885, 148.9598804145299766 ) ) ;
#17968=CARTESIAN_POINT ( 'NONE',  ( 20.60060554280000034, 1507.884458093629974, 227.6638854010979856 ) ) ;
#17969=ORIENTED_EDGE ( 'NONE', *, *, #104187, .F. ) ;
#17970=CARTESIAN_POINT ( 'NONE',  ( 7.709069255566407541, 1423.240024452770740, 139.1418590084687423 ) ) ;
#17971=CARTESIAN_POINT ( 'NONE',  ( -1.635875587731045355, 1484.273925081808557, 182.6549239315091029 ) ) ;
#17972=CARTESIAN_POINT ( 'NONE',  ( 7.245928414539999807, 1509.166093783229826, 236.9901212716980012 ) ) ;
#17975=CARTESIAN_POINT ( 'NONE',  ( -5.127859024660000209, 1422.417124035330062, 185.6440635277980107 ) ) ;
#17977=CARTESIAN_POINT ( 'NONE',  ( 4.259181585509999479, 1408.384021400730035, 270.3898288651980124 ) ) ;
#17982=CARTESIAN_POINT ( 'NONE',  ( 23.86274566002959929, 1440.678159878850011, 206.2105284970400021 ) ) ;
#17984=CARTESIAN_POINT ( 'NONE',  ( 15.50242774170000004, 1471.316885392330050, 194.6525715419979861 ) ) ;
#17987=CARTESIAN_POINT ( 'NONE',  ( 17.93107151423210155, 1421.416072919849967, 225.1143211638089952 ) ) ;
#17988=CARTESIAN_POINT ( 'NONE',  ( -4.566658896609312457, 1506.397480193153115, 187.6488660611327361 ) ) ;
#17991=CARTESIAN_POINT ( 'NONE',  ( -4.363122647530000009, 1409.354802298927325, 137.0999999980979851 ) ) ;
#17992=EDGE_CURVE ( 'NONE', #50150, #32822, #43759, .T. ) ;
#17993=CARTESIAN_POINT ( 'NONE',  ( -2.913496927302146933, 1484.798880128765177, 183.2196020003875390 ) ) ;
#17994=CARTESIAN_POINT ( 'NONE',  ( -16.95309613902585255, 1410.872492358897262, 191.9186258755552217 ) ) ;
#18002=CARTESIAN_POINT ( 'NONE',  ( -11.25881761529999991, 1429.196009723030102, 150.7919537440980093 ) ) ;
#18006=B_SPLINE_CURVE_WITH_KNOTS ( 'NONE', 3,
 ( #12292, #19025, #53228, #28559, #44831, #62757, #36400 ),
 .UNSPECIFIED., .F., .F.,
 ( 4, 3, 4 ),
 ( -157.7844419379999863, -101.5361819250880018, -30.93609007885059725 ),
 .UNSPECIFIED. ) ;
#18009=CARTESIAN_POINT ( 'NONE',  ( 14.34346040870000216, 1410.403127989829954, 227.8390325281980040 ) ) ;
#18012=CARTESIAN_POINT ( 'NONE',  ( -16.17783063698000134, 1459.145687810399977, 230.7168772285679950 ) ) ;
#18014=CARTESIAN_POINT ( 'NONE',  ( 30.19617742020000151, 1414.287258031230067, 267.1521104148980044 ) ) ;
#18016=CARTESIAN_POINT ( 'NONE',  ( 22.93100030269999934, 1430.293864573130122, 203.3539861534579813 ) ) ;
#18019=CARTESIAN_POINT ( 'NONE',  ( -20.92707481170000250, 1427.944386893930186, 220.6468670353979746 ) ) ;
#18020=CARTESIAN_POINT ( 'NONE',  ( 18.42577555256999844, 1424.509265906519886, 223.4215472205989954 ) ) ;
#18022=DIRECTION ( 'NONE',  ( -0.02578658883684968942, 0.9994800766169525952, 0.01935531663212984241 ) ) ;
#18023=CARTESIAN_POINT ( 'NONE',  ( -6.972733166630000312, 1409.156553594930301, 196.2309095765980089 ) ) ;
#18024=CARTESIAN_POINT ( 'NONE',  ( -18.89907699009999931, 1416.828040557830036, 207.5749716938179859 ) ) ;
#18025=CARTESIAN_POINT ( 'NONE',  ( -13.44162146400000069, 1443.167077655089997, 187.7002249684979915 ) ) ;
#18028=CARTESIAN_POINT ( 'NONE',  ( 4.363122647530000009, 1421.971318475729959, 172.2701767054979882 ) ) ;
#18032=CARTESIAN_POINT ( 'NONE',  ( -14.30375442816609954, 1409.412558498570206, 204.8191087406950146 ) ) ;
#18034=LINE ( 'NONE', #103138, #65255 ) ;
#18035=CARTESIAN_POINT ( 'NONE',  ( -18.40068035370000032, 1473.290853966130044, 267.7101340507979899 ) ) ;
#18036=CARTESIAN_POINT ( 'NONE',  ( 0.1762907655658970119, 1420.387354559859887, 183.3288319911129918 ) ) ;
#18037=EDGE_CURVE ( 'NONE', #3400, #99658, #62112, .T. ) ;
#18038=CARTESIAN_POINT ( 'NONE',  ( 18.04484862309950088, 1421.101146633960070, 223.7483925777569880 ) ) ;
#18043=CARTESIAN_POINT ( 'NONE',  ( 11.94908641555320017, 1415.673583082879986, 223.2663781018690088 ) ) ;
#18047=CARTESIAN_POINT ( 'NONE',  ( -23.36195796790000401, 1409.893412594229858, 207.9384553132279905 ) ) ;
#18053=CARTESIAN_POINT ( 'NONE',  ( 2.451271202390000070, 1433.447543843880112, 150.3250444719979839 ) ) ;
#18057=LINE ( 'NONE', #55013, #37185 ) ;
#18058=VECTOR ( 'NONE', #51221, 1000.000000000000000 ) ;
#18064=CARTESIAN_POINT ( 'NONE',  ( -0.6104152826046118641, 1418.823154379500011, 184.7568847501300127 ) ) ;
#18067=CARTESIAN_POINT ( 'NONE',  ( -9.382268578863946829, 1398.191384707091629, 218.1279820238655418 ) ) ;
#18068=CYLINDRICAL_SURFACE ( 'NONE', #3336, 12.50000000000001066 ) ;
#18070=CARTESIAN_POINT ( 'NONE',  ( 1.913188568150000046, 1508.750155563429871, 237.3579719449979848 ) ) ;
#18072=CARTESIAN_POINT ( 'NONE',  ( 38.05425021522230367, 1450.256561828500026, 135.6620645644130150 ) ) ;
#18074=ORIENTED_EDGE ( 'NONE', *, *, #15389, .T. ) ;
#18075=ORIENTED_EDGE ( 'NONE', *, *, #80371, .T. ) ;
#18076=CARTESIAN_POINT ( 'NONE',  ( 11.82056980545410063, 1433.695608034110137, 150.7613404324029887 ) ) ;
#18077=CARTESIAN_POINT ( 'NONE',  ( 28.10198114769999833, 1509.875926101730101, 215.6436498675279836 ) ) ;
#18083=CARTESIAN_POINT ( 'NONE',  ( 2.329729395510000245, 1427.373795049630189, 123.0297916884979941 ) ) ;
#18084=CARTESIAN_POINT ( 'NONE',  ( 17.93739292209999903, 1507.814075490329969, 230.5553894001980098 ) ) ;
#18086=CARTESIAN_POINT ( 'NONE',  ( 3.848404275880000114, 1507.638435329329923, 181.6079968732980205 ) ) ;
#18088=CARTESIAN_POINT ( 'NONE',  ( 15.26168084529999902, 1409.446010026229715, 225.6870430949980175 ) ) ;
#18090=CARTESIAN_POINT ( 'NONE',  ( 13.98791200557839964, 1415.441076448340027, 197.3320725003540019 ) ) ;
#18092=AXIS2_PLACEMENT_3D ( 'NONE', #49588, #8653, #17027 ) ;
#18094=ORIENTED_EDGE ( 'NONE', *, *, #30262, .T. ) ;
#18095=CARTESIAN_POINT ( 'NONE',  ( 13.47042191939980071, 1434.942646400420017, 148.9306420637369968 ) ) ;
#18100=CARTESIAN_POINT ( 'NONE',  ( -1.753158309049999808, 1464.912754134729994, 237.4770670691980001 ) ) ;
#18101=CARTESIAN_POINT ( 'NONE',  ( -9.972378110560478959, 1407.313660260299912, 200.5612547303060182 ) ) ;
#18104=AXIS2_PLACEMENT_3D ( 'NONE', #15959, #25466, #68074 ) ;
#18106=CARTESIAN_POINT ( 'NONE',  ( 13.04207810306199988, 1409.368499790489750, 192.3005055522939983 ) ) ;
#18107=CARTESIAN_POINT ( 'NONE',  ( 4.249254207745330802, 1446.470040732190000, 161.2344365711890077 ) ) ;
#18109=VERTEX_POINT ( 'NONE', #99091 ) ;
#18112=CARTESIAN_POINT ( 'NONE',  ( 20.92687816970969550, 1440.913060387330006, 221.9350866778629836 ) ) ;
#18114=CARTESIAN_POINT ( 'NONE',  ( -19.75079221190000212, 1509.023212918529907, 229.8582975788980036 ) ) ;
#18116=CARTESIAN_POINT ( 'NONE',  ( 26.41530183785989649, 1448.997685820419974, 136.8834598208839850 ) ) ;
#18117=CARTESIAN_POINT ( 'NONE',  ( -11.05974434320000022, 1410.673379371429974, 188.8342600372980087 ) ) ;
#18118=CARTESIAN_POINT ( 'NONE',  ( -24.65398899419999879, 1442.417487969639978, 210.7516708981580109 ) ) ;
#18119=CARTESIAN_POINT ( 'NONE',  ( -11.27186228789999944, 1414.983771850430003, 195.8113390693980023 ) ) ;
#18120=ORIENTED_EDGE ( 'NONE', *, *, #63971, .T. ) ;
#18122=CARTESIAN_POINT ( 'NONE',  ( 0.3382504354559999760, 1405.989871386730101, 266.9611136494980315 ) ) ;
#18126=CARTESIAN_POINT ( 'NONE',  ( -2.011314089155299634, 1484.247616858960100, 182.9841112829520000 ) ) ;
#18129=CARTESIAN_POINT ( 'NONE',  ( -22.52564151159999639, 1509.699673122230024, 190.3321270483980072 ) ) ;
#18130=CARTESIAN_POINT ( 'NONE',  ( 29.24528532949999970, 1509.871747146429925, 208.3253336781129974 ) ) ;
#18137=CARTESIAN_POINT ( 'NONE',  ( 33.60183515679999999, 1443.049082915059898, 248.0844435633979970 ) ) ;
#18140=CARTESIAN_POINT ( 'NONE',  ( -29.03287634025529940, 1509.926910769670030, 213.4187435708539908 ) ) ;
#18141=CARTESIAN_POINT ( 'NONE',  ( -8.482879236748889440, 1508.704785055359935, 235.6989384136039973 ) ) ;
#18142=EDGE_CURVE ( 'NONE', #68439, #46649, #17697, .T. ) ;
#18143=CARTESIAN_POINT ( 'NONE',  ( -21.75818116419999981, 1452.902822741230011, 221.5405819497979678 ) ) ;
#18144=EDGE_CURVE ( 'NONE', #8717, #33774, #88554, .T. ) ;
#18145=VECTOR ( 'NONE', #100803, 1000.000000000000227 ) ;
#18146=CARTESIAN_POINT ( 'NONE',  ( 11.86563475029999992, 1432.300009996690051, 149.9825381228980063 ) ) ;
#18147=CARTESIAN_POINT ( 'NONE',  ( 19.02030571170000073, 1456.697257245530182, 226.2527947047979922 ) ) ;
#18152=CARTESIAN_POINT ( 'NONE',  ( 0.3370331515910000020, 1406.265758353229785, 269.2946826180980224 ) ) ;
#18153=CARTESIAN_POINT ( 'NONE',  ( 27.85007275959999617, 1509.193792694529975, 207.4562351974080059 ) ) ;
#18155=FACE_OUTER_BOUND ( 'NONE', #105281, .T. ) ;
#18156=FACE_OUTER_BOUND ( 'NONE', #53531, .T. ) ;
#18157=CARTESIAN_POINT ( 'NONE',  ( -39.38489486480609969, 1449.784184279609917, 136.1650281365439810 ) ) ;
#18159=VECTOR ( 'NONE', #100408, 1000.000000000000000 ) ;
#18160=CARTESIAN_POINT ( 'NONE',  ( -38.33208885764259577, 1440.913060391839963, 256.8080927262569730 ) ) ;
#18161=CARTESIAN_POINT ( 'NONE',  ( 35.23055949741119974, 1450.257496671300032, 136.2304356426660092 ) ) ;
#18168=CARTESIAN_POINT ( 'NONE',  ( 2.623518071850000410, 1448.928635941619859, 183.1137651247979932 ) ) ;
#18169=CARTESIAN_POINT ( 'NONE',  ( 13.19906462199999986, 1434.900406958499843, 146.7591386227980195 ) ) ;
#18171=CARTESIAN_POINT ( 'NONE',  ( 16.47530569442600168, 1492.985912492669968, 188.5532949614449763 ) ) ;
#18172=CARTESIAN_POINT ( 'NONE',  ( -0.2907244602440000603, 1416.115749421129976, 233.5373085857980016 ) ) ;
#18174=CARTESIAN_POINT ( 'NONE',  ( -28.13497786889999830, 1508.084884472430076, 209.9324264222260013 ) ) ;
#18179=CARTESIAN_POINT ( 'NONE',  ( -12.61894528015529282, 1419.411281935211719, 228.4589828776151705 ) ) ;
#18180=CARTESIAN_POINT ( 'NONE',  ( -17.38235991649999690, 1414.983773854429955, 207.6803066081180020 ) ) ;
#18182=CARTESIAN_POINT ( 'NONE',  ( 25.11052302270000069, 1436.446855038549984, 137.6568901633980317 ) ) ;
#18183=CARTESIAN_POINT ( 'NONE',  ( -8.417397172205490108, 1396.207002374369949, 201.9581881603329805 ) ) ;
#18184=ADVANCED_FACE ( 'NONE', ( #25690 ), #21149, .F. ) ;
#18186=CARTESIAN_POINT ( 'NONE',  ( -17.27480999623900004, 1410.739465257400070, 225.9386244916770181 ) ) ;
#18192=CARTESIAN_POINT ( 'NONE',  ( 10.89837308280000094, 1426.095306331829761, 91.92372727469789595 ) ) ;
#18194=CARTESIAN_POINT ( 'NONE',  ( 4.152837535936280133, 1424.659374145959873, 185.0051014476340185 ) ) ;
#18195=CARTESIAN_POINT ( 'NONE',  ( -2.870322881153364758, 1419.668002344334354, 186.1847472751339012 ) ) ;
#18198=CARTESIAN_POINT ( 'NONE',  ( 8.309206006240000164, 1507.619018865230146, 183.0708158541980026 ) ) ;
#18204=CARTESIAN_POINT ( 'NONE',  ( -40.27288003839999675, 1443.726530270089825, 137.1298452635979856 ) ) ;
#18206=CARTESIAN_POINT ( 'NONE',  ( -2.920683203049999872E-09, 1474.175172929029941, 270.1377426661979939 ) ) ;
#18208=CARTESIAN_POINT ( 'NONE',  ( -1.319906717929999918, 1486.022175928729894, 181.9654110648980065 ) ) ;
#18211=CARTESIAN_POINT ( 'NONE',  ( 22.33897491209999941, 1410.187224165629914, 206.2328829822479861 ) ) ;
#18212=CARTESIAN_POINT ( 'NONE',  ( -2.500000000000000000, 1448.769782533650186, 157.0284636696169969 ) ) ;
#18214=CARTESIAN_POINT ( 'NONE',  ( 14.75735370008069935, 1409.369483614819956, 204.1261042358389943 ) ) ;
#18215=CARTESIAN_POINT ( 'NONE',  ( -8.399159049882628736, 1406.308215514319727, 267.5079637899610248 ) ) ;
#18216=CARTESIAN_POINT ( 'NONE',  ( -13.76076751202730009, 1434.979366489430049, 148.7044419327400249 ) ) ;
#18218=CARTESIAN_POINT ( 'NONE',  ( 3.566815704669999754, 1424.381564880729911, 184.5429952954980024 ) ) ;
#18219=CARTESIAN_POINT ( 'NONE',  ( 13.14468279130000106, 1445.308786585929965, 188.3807251759980090 ) ) ;
#18227=B_SPLINE_CURVE_WITH_KNOTS ( 'NONE', 3,
 ( #90990, #108355, #33286, #7546 ),
 .UNSPECIFIED., .F., .F.,
 ( 4, 4 ),
 ( 0.000000000000000000, 1.000000000000000000 ),
 .UNSPECIFIED. ) ;
#18228=ORIENTED_EDGE ( 'NONE', *, *, #105425, .F. ) ;
#18229=CARTESIAN_POINT ( 'NONE',  ( 2.500000000000000000, 1426.966631815929986, 170.4008037693979816 ) ) ;
#18232=AXIS2_PLACEMENT_3D ( 'NONE', #689, #76832, #95287 ) ;
#18233=CARTESIAN_POINT ( 'NONE',  ( -28.70528459879999872, 1509.871474410030032, 205.0464017625179736 ) ) ;
#18234=CARTESIAN_POINT ( 'NONE',  ( -1.330926000679999888, 1457.942373938230048, 229.8940546109979834 ) ) ;
#18238=CARTESIAN_POINT ( 'NONE',  ( -12.66869256729999904, 1410.724518653430096, 227.9982876970979930 ) ) ;
#18239=CARTESIAN_POINT ( 'NONE',  ( -12.03594993039999927, 1445.662098499869899, 187.0019535905980206 ) ) ;
#18241=CARTESIAN_POINT ( 'NONE',  ( -26.57998359160610136, 1469.327412759369736, 208.7761463849559789 ) ) ;
#18242=CARTESIAN_POINT ( 'NONE',  ( 28.02912970369999712, 1508.133041384130138, 210.7019033844679825 ) ) ;
#18244=CARTESIAN_POINT ( 'NONE',  ( -25.70525537839999686, 1436.337899435129884, 137.0032570942979930 ) ) ;
#18246=VECTOR ( 'NONE', #2620, 1000.000000000000000 ) ;
#18248=CARTESIAN_POINT ( 'NONE',  ( -14.16989796110000022, 1420.440730658529901, 227.4201728071980142 ) ) ;
#18250=CARTESIAN_POINT ( 'NONE',  ( -11.60004869885203682, 1422.941213646836331, 135.6422426701566053 ) ) ;
#18253=CARTESIAN_POINT ( 'NONE',  ( 2.500000000000000000, 1432.575364831350271, 157.5016493498980026 ) ) ;
#18254=CARTESIAN_POINT ( 'NONE',  ( -3.088334884859999629, 1412.839240486330027, 232.6088388287980138 ) ) ;
#18260=CARTESIAN_POINT ( 'NONE',  ( 12.44825556113039866, 1434.827193400389888, 150.5385283147030009 ) ) ;
#18262=CARTESIAN_POINT ( 'NONE',  ( 15.04655486393220087, 1478.705643649750073, 230.8080699388220012 ) ) ;
#18263=CARTESIAN_POINT ( 'NONE',  ( -23.54197198179479855, 1507.885248531370053, 223.3642489706239758 ) ) ;
#18264=CYLINDRICAL_SURFACE ( 'NONE', #102975, 8.000000000000000000 ) ;
#18265=B_SPLINE_CURVE_WITH_KNOTS ( 'NONE', 3,
 ( #4894, #13276, #81589, #71042, #96771, #72143, #28455, #104608, #54774, #20575, #105728, #4366, #21674, #87829, #79961, #55326, #20040, #62649, #53688, #88362, #3834, #2728, #11651, #54236, #106260, #98402, #70489, #105164, #88906, #80517, #19485, #36850, #62084, #12192, #27901, #29013, #37962, #45828, #47468, #63197, #46385, #29547, #63733, #89458, #96210, #11118, #71607, #46933, #38494, #3278, #55880, #97843, #79416, #37408, #21121, #12751, #81051, #72672, #106797, #30087, #90001, #64281, #45278, #73213, #56975, #5450, #23343, #107905, #39610, #57534, #83808, #49676, #109571, #32842, #98947, #108464 ),
 .UNSPECIFIED., .F., .F.,
 ( 4, 2, 2, 2, 1, 1, 1, 1, 2, 2, 2, 1, 1, 2, 2, 2, 2, 2, 2, 1, 1, 1, 1, 1, 1, 2, 2, 2, 2, 2, 1, 1, 1, 1, 1, 2, 2, 2, 2, 2, 1, 2, 2, 2, 2, 2, 4 ),
 ( 0.000000000000000000, 0.007812499999216796637, 0.01171874999882519669, 0.01367187499863343862, 0.01464843749853756219, 0.01513671874849285663, 0.01538085937346737354, 0.01550292968595155113, 0.01556396484219058768, 0.01562499999842962423, 0.02343749999855148508, 0.02734374999860635438, 0.02929687499863947026, 0.03027343749865050657, 0.03124999999866154288, 0.04687499999895392011, 0.05468749999910008097, 0.06249999999924624183, 0.09374999999981868670, 0.1093750000000989486, 0.1171875000002390588, 0.1210937500003148592, 0.1230468750003584633, 0.1240234375003802514, 0.1245117187503911454, 0.1247558593753966549, 0.1250000000004021505, 0.1875000000015698276, 0.2187500000021481705, 0.2343750000024373004, 0.2421875000025818792, 0.2460937500026541547, 0.2480468750026902647, 0.2490234375027044478, 0.2495117187527077784, 0.2497558593777093605, 0.2500000000027109426, 0.3750000000022902791, 0.4375000000020838886, 0.4687500000019808599, 0.4843750000019327873, 0.4921875000019087509, 0.5000000000018847146, 0.6250000000014135360, 0.7500000000009424683, 0.8750000000004711787, 1.000000000000000000 ),
 .UNSPECIFIED. ) ;
#18266=CARTESIAN_POINT ( 'NONE',  ( -0.4960403072899999821, 1409.436440935729934, 232.9663690048980129 ) ) ;
#18269=CARTESIAN_POINT ( 'NONE',  ( -4.270561097189999877, 1421.938260751330063, 185.0877191730979803 ) ) ;
#18270=CARTESIAN_POINT ( 'NONE',  ( 20.07277491569999839, 1508.598349460030022, 188.9934802953980011 ) ) ;
#18273=CARTESIAN_POINT ( 'NONE',  ( -12.57878310069559902, 1415.943166310999914, 196.1339907655800232 ) ) ;
#18274=CARTESIAN_POINT ( 'NONE',  ( -6.328709615500000218, 1508.913060324029857, 180.8323534384980178 ) ) ;
#18275=VERTEX_POINT ( 'NONE', #20594 ) ;
#18276=CARTESIAN_POINT ( 'NONE',  ( 3.238878936319999902, 1420.340958668729854, 185.3443125121980017 ) ) ;
#18277=EDGE_CURVE ( 'NONE', #64966, #93939, #42408, .T. ) ;
#18279=DIRECTION ( 'NONE',  ( 0.000000000000000000, 0.000000000000000000, -1.000000000000000000 ) ) ;
#18283=CARTESIAN_POINT ( 'NONE',  ( -3.138402261229999990, 1447.047508080440139, 157.7990927532979981 ) ) ;
#18284=CARTESIAN_POINT ( 'NONE',  ( -18.54535832700000242, 1425.392845097829877, 225.7569259269980080 ) ) ;
#18286=EDGE_CURVE ( 'NONE', #30631, #92476, #47100, .T. ) ;
#18287=FACE_OUTER_BOUND ( 'NONE', #106865, .T. ) ;
#18288=CARTESIAN_POINT ( 'NONE',  ( 18.16298593710000020, 1438.550562606130143, 191.5625238810979738 ) ) ;
#18290=CARTESIAN_POINT ( 'NONE',  ( 0.5678390018416790141, 1428.477637517579979, 189.9617647321709910 ) ) ;
#18293=CARTESIAN_POINT ( 'NONE',  ( 1.514738106409309948, 1507.606285602550088, 186.2052147526660235 ) ) ;
#18295=CARTESIAN_POINT ( 'NONE',  ( -24.42829869279999855, 1436.527038349410077, 210.7116707911179958 ) ) ;
#18296=CARTESIAN_POINT ( 'NONE',  ( 7.511829633256015271, 1410.548442039797692, 187.3987484226458946 ) ) ;
#18301=CARTESIAN_POINT ( 'NONE',  ( 13.08238251380000072, 1414.913528139129994, 198.0397827309980130 ) ) ;
#18303=CARTESIAN_POINT ( 'NONE',  ( 3.588016447739999837, 1452.642150377629832, 153.4169808353979931 ) ) ;
#18304=( BOUNDED_CURVE ( )  B_SPLINE_CURVE ( 3, ( #47177, #87535, #70216, #88091 ),
 .UNSPECIFIED., .F., .F. ) 
 B_SPLINE_CURVE_WITH_KNOTS ( ( 4, 4 ),
 ( 4.427184739196824204, 4.808362416880929580 ),
 .UNSPECIFIED. ) 
 CURVE ( )  GEOMETRIC_REPRESENTATION_ITEM ( )  RATIONAL_B_SPLINE_CURVE ( ( 1.000000000000000000, 0.9879285716166186226, 0.9879285716166186226, 1.000000000000000000 ) ) 
 REPRESENTATION_ITEM ( '' )  );
#18307=EDGE_CURVE ( 'NONE', #43746, #101156, #81772, .T. ) ;
#18308=CARTESIAN_POINT ( 'NONE',  ( 23.34540950859999953, 1507.878524956530100, 194.4697486434980078 ) ) ;
#18309=ORIENTED_EDGE ( 'NONE', *, *, #78222, .T. ) ;
#18310=CARTESIAN_POINT ( 'NONE',  ( -1.414439329499999953, 1414.913528139129994, 226.2086894112979962 ) ) ;
#18315=CARTESIAN_POINT ( 'NONE',  ( 14.41410989250000085, 1444.046959656890067, 189.7051000925980020 ) ) ;
#18316=CARTESIAN_POINT ( 'NONE',  ( -0.3821804589910179906, 1506.433683733660018, 187.1424611576989889 ) ) ;
#18318=CARTESIAN_POINT ( 'NONE',  ( 15.04404422727308344, 1412.425273560396590, 269.3648504014765876 ) ) ;
#18319=CARTESIAN_POINT ( 'NONE',  ( -6.248994634959999850, 1472.348783256330080, 259.9484462021979994 ) ) ;
#18322=CARTESIAN_POINT ( 'NONE',  ( -12.19020004887032727, 1435.566796327880638, 151.0976163169758877 ) ) ;
#18323=CARTESIAN_POINT ( 'NONE',  ( -19.80101799410000041, 1484.918799879129892, 190.6212978484980169 ) ) ;
#18324=CARTESIAN_POINT ( 'NONE',  ( 1.122881213689999935, 1410.331791442129997, 185.2157289252980092 ) ) ;
#18325=CARTESIAN_POINT ( 'NONE',  ( 4.770564261300000553, 1422.188385567129899, 184.2239224491979996 ) ) ;
#18326=CARTESIAN_POINT ( 'NONE',  ( -10.13504282470000106, 1439.368087670590057, 152.9209922797979857 ) ) ;
#18329=CARTESIAN_POINT ( 'NONE',  ( -3.141354938490000137, 1451.554175194630261, 154.1120778672979839 ) ) ;
#18331=ORIENTED_EDGE ( 'NONE', *, *, #26356, .T. ) ;
#18334=CARTESIAN_POINT ( 'NONE',  ( -43.48864995209999762, 1440.913074447990084, 270.3367068800979496 ) ) ;
#18335=CARTESIAN_POINT ( 'NONE',  ( 2.566893074593609807E-08, 1406.911841303630126, 196.1218459607310081 ) ) ;
#18336=CARTESIAN_POINT ( 'NONE',  ( 17.98939575750000230, 1410.465183456229852, 222.9682893216979949 ) ) ;
#18337=CARTESIAN_POINT ( 'NONE',  ( -14.38570825430000077, 1474.169743061429926, 223.8345247943979928 ) ) ;
#18338=CARTESIAN_POINT ( 'NONE',  ( 0.9766393796380001824, 1453.313060387329870, 188.4686263754979905 ) ) ;
#18339=CARTESIAN_POINT ( 'NONE',  ( 2.915910696398010149, 1409.692218141939975, 231.4126881937029907 ) ) ;
#18341=CARTESIAN_POINT ( 'NONE',  ( -2.995672382979999604, 1416.748940793229849, 233.0563413717979984 ) ) ;
#18344=CARTESIAN_POINT ( 'NONE',  ( -45.63195895436749794, 1439.443261914909954, 266.1896113851490213 ) ) ;
#18345=CARTESIAN_POINT ( 'NONE',  ( -3.087032477589999768, 1436.949765671180103, 185.2347600039979909 ) ) ;
#18350=PLANE ( 'NONE',  #16193 ) ;
#18355=CARTESIAN_POINT ( 'NONE',  ( 7.313756596019999279, 1422.662435718929828, 212.8858276506779816 ) ) ;
#18358=CARTESIAN_POINT ( 'NONE',  ( 11.60004869885203682, 1422.586145265931236, 135.5999999980982125 ) ) ;
#18359=CARTESIAN_POINT ( 'NONE',  ( -11.59119438181595818, 1426.213969660457678, 138.6120005729653144 ) ) ;
#18363=CARTESIAN_POINT ( 'NONE',  ( -4.332897253567730367, 1408.387299629059953, 270.3897631605610172 ) ) ;
#18365=CARTESIAN_POINT ( 'NONE',  ( 10.63881130030000044, 1418.746488869330051, 230.0613383181980112 ) ) ;
#18366=CARTESIAN_POINT ( 'NONE',  ( -17.60627563539920004, 1410.895669414250051, 194.0661810348550205 ) ) ;
#18369=VERTEX_POINT ( 'NONE', #84917 ) ;
#18370=CARTESIAN_POINT ( 'NONE',  ( -22.59787312113130042, 1409.702172917540111, 209.4225048435710050 ) ) ;
#18371=CARTESIAN_POINT ( 'NONE',  ( -4.216177480479998962, 1424.161827809529996, 185.4694233363979947 ) ) ;
#18372=CARTESIAN_POINT ( 'NONE',  ( 3.683511325231741740, 1425.182533976880450, 185.0553125120289906 ) ) ;
#18373=CARTESIAN_POINT ( 'NONE',  ( -0.005607894164331979868, 1408.917889387629884, 186.3448695751470154 ) ) ;
#18374=CARTESIAN_POINT ( 'NONE',  ( -20.53032749330389706, 1436.446110082554924, 144.8592029257055458 ) ) ;
#18375=CARTESIAN_POINT ( 'NONE',  ( -18.51512065000000007, 1415.857213627029978, 224.3066119029979859 ) ) ;
#18376=CARTESIAN_POINT ( 'NONE',  ( 36.87367878740020188, 1461.868311835329905, 266.6849271820060494 ) ) ;
#18377=CARTESIAN_POINT ( 'NONE',  ( -8.890585777435378034, 1465.118968690018619, 232.8711024472996201 ) ) ;
#18378=CARTESIAN_POINT ( 'NONE',  ( -16.84468799194050703, 1421.803329214568066, 226.8795727158544366 ) ) ;
#18381=CARTESIAN_POINT ( 'NONE',  ( 23.82822416500561502, 1411.105482365838270, 210.7039567702046554 ) ) ;
#18382=CARTESIAN_POINT ( 'NONE',  ( 1.475113315915349999, 1481.918977469239962, 182.2120507298820087 ) ) ;
#18383=CARTESIAN_POINT ( 'NONE',  ( 23.86654294979999946, 1410.978130439630149, 208.1633478644210129 ) ) ;
#18384=VERTEX_POINT ( 'NONE', #6023 ) ;
#18386=CARTESIAN_POINT ( 'NONE',  ( 25.88275927131619980, 1451.560184493740053, 136.3203580496130201 ) ) ;
#18387=CARTESIAN_POINT ( 'NONE',  ( 15.94345596297699963, 1409.469818137940138, 225.2684692625209948 ) ) ;
#18390=CARTESIAN_POINT ( 'NONE',  ( 16.34466203799999917, 1409.483828562729968, 193.4811910679979974 ) ) ;
#18391=CARTESIAN_POINT ( 'NONE',  ( 20.77846844200000120, 1444.740067931809790, 176.2781434906979996 ) ) ;
#18392=CARTESIAN_POINT ( 'NONE',  ( 2.713487254142998850, 1439.656254381911822, 183.6712819054291970 ) ) ;
#18393=CARTESIAN_POINT ( 'NONE',  ( -2.714091174029999877E-10, 1417.262443616730025, 235.9145977375980010 ) ) ;
#18395=CARTESIAN_POINT ( 'NONE',  ( 4.165142600520000293, 1409.058510372029787, 229.9895894434979766 ) ) ;
#18403=CARTESIAN_POINT ( 'NONE',  ( -0.3209257366447499926, 1408.978166690620128, 232.1464160328119988 ) ) ;
#18407=CARTESIAN_POINT ( 'NONE',  ( -24.08292308869999943, 1450.076351704500212, 243.9198229383979992 ) ) ;
#18409=CARTESIAN_POINT ( 'NONE',  ( 11.90133581370000115, 1433.308793707279847, 149.9471025605980117 ) ) ;
#18410=CARTESIAN_POINT ( 'NONE',  ( 9.145222436810001909, 1453.522154064530014, 214.3676144197979738 ) ) ;
#18411=CARTESIAN_POINT ( 'NONE',  ( 25.26688801316450039, 1440.913060399130018, 217.7010804864050044 ) ) ;
#18415=CARTESIAN_POINT ( 'NONE',  ( -9.574504100549999563, 1485.990341757929855, 183.6379974207980013 ) ) ;
#18417=CARTESIAN_POINT ( 'NONE',  ( 0.04628635179088989859, 1508.911441867209987, 238.5489216072199952 ) ) ;
#18418=CARTESIAN_POINT ( 'NONE',  ( 25.41997721730000137, 1449.801887500550038, 211.0416158964779925 ) ) ;
#18420=CARTESIAN_POINT ( 'NONE',  ( 25.68555131787286783, 1436.646045936909786, 137.1303311310317952 ) ) ;
#18425=CARTESIAN_POINT ( 'NONE',  ( 0.1639172357618859655, 1483.921440558410040, 181.9259246723260048 ) ) ;
#18428=CARTESIAN_POINT ( 'NONE',  ( -12.53380499169999851, 1445.052233488290085, 169.4755105685979970 ) ) ;
#18430=CARTESIAN_POINT ( 'NONE',  ( -28.77730029287999969, 1509.917985857419808, 212.2396942430650029 ) ) ;
#18431=CARTESIAN_POINT ( 'NONE',  ( -38.87405678782049989, 1449.786581495279961, 134.0999999981590065 ) ) ;
#18432=ORIENTED_EDGE ( 'NONE', *, *, #8351, .F. ) ;
#18435=CARTESIAN_POINT ( 'NONE',  ( 18.18137293399999876, 1507.546748832030062, 186.5307135875980009 ) ) ;
#18437=CARTESIAN_POINT ( 'NONE',  ( -13.95470550870000004, 1415.426952351230057, 221.1148131923979747 ) ) ;
#18439=CARTESIAN_POINT ( 'NONE',  ( 23.17538675820700789, 1409.994297229576887, 208.1793956993277845 ) ) ;
#18443=CARTESIAN_POINT ( 'NONE',  ( 11.39880752746310044, 1409.311115508779949, 218.7955269592959837 ) ) ;
#18444=CARTESIAN_POINT ( 'NONE',  ( 10.10004869885234058, 1422.222932908421171, 137.0999999980978430 ) ) ;
#18446=CARTESIAN_POINT ( 'NONE',  ( -17.60602154420000076, 1410.887439192729971, 193.4352696968979899 ) ) ;
#18451=ORIENTED_EDGE ( 'NONE', *, *, #74444, .T. ) ;
#18452=CARTESIAN_POINT ( 'NONE',  ( -8.313145311751080513, 1507.316772571419961, 235.1568484389069909 ) ) ;
#18453=EDGE_LOOP ( 'NONE', ( #24161, #73903, #53390, #13103 ) ) ;
#18454=B_SPLINE_CURVE_WITH_KNOTS ( 'NONE', 5,
 ( #53177, #53754, #45339, #20101, #54293, #4425 ),
 .UNSPECIFIED., .F., .F.,
 ( 6, 6 ),
 ( 0.000000000000000000, 1.000000000000000000 ),
 .UNSPECIFIED. ) ;
#18458=B_SPLINE_CURVE_WITH_KNOTS ( 'NONE', 3,
 ( #14839, #66388, #21575, #47359, #40604, #14287, #4259, #74774, #98851, #23786, #90997, #73113, #57975 ),
 .UNSPECIFIED., .F., .F.,
 ( 4, 2, 2, 1, 2, 2, 4 ),
 ( 0.000000000000000000, 0.2500000000000711098, 0.3750000000001102451, 0.4375000000001359468, 0.4687500000001467715, 0.5000000000001576517, 1.000000000000000000 ),
 .UNSPECIFIED. ) ;
#18459=CARTESIAN_POINT ( 'NONE',  ( 30.19399729140642563, 1462.104126541301866, 269.4728972154693452 ) ) ;
#18461=CARTESIAN_POINT ( 'NONE',  ( 17.99196544828748046, 1435.000034824831118, 215.3568569466342240 ) ) ;
#18462=CARTESIAN_POINT ( 'NONE',  ( 1.534959661399999842, 1416.490978422929857, 232.7302165538980034 ) ) ;
#18467=B_SPLINE_CURVE_WITH_KNOTS ( 'NONE', 3,
 ( #63748, #19504, #53138, #104624, #18943, #80537 ),
 .UNSPECIFIED., .F., .F.,
 ( 4, 2, 4 ),
 ( 0.000000000000000000, 0.5000000000000000000, 1.000000000000000000 ),
 .UNSPECIFIED. ) ;
#18468=CARTESIAN_POINT ( 'NONE',  ( -16.17567356680000046, 1459.146941997929844, 230.7169173512979796 ) ) ;
#18471=DIRECTION ( 'NONE',  ( 0.1041548977914050628, 0.000000000000000000, 0.9945610877497982338 ) ) ;
#18475=CARTESIAN_POINT ( 'NONE',  ( 40.26396420611710170, 1444.186530323160014, 137.1012295353969819 ) ) ;
#18479=CARTESIAN_POINT ( 'NONE',  ( -24.66781776999999920, 1430.359786449429976, 207.5926804364680152 ) ) ;
#18480=CARTESIAN_POINT ( 'NONE',  ( -11.50950220968000082, 1425.948128105500018, 135.2567894809000109 ) ) ;
#18481=CARTESIAN_POINT ( 'NONE',  ( 17.29966500927950079, 1410.740263436930263, 192.3341061383550255 ) ) ;
#18482=EDGE_CURVE ( 'NONE', #36240, #97581, #45726, .T. ) ;
#18484=CARTESIAN_POINT ( 'NONE',  ( 28.15304776960663347, 1510.007776421887002, 219.4938112226830640 ) ) ;
#18486=CARTESIAN_POINT ( 'NONE',  ( -11.55307676520000015, 1412.346723819529871, 255.2309104534979838 ) ) ;
#18488=EDGE_CURVE ( 'NONE', #60010, #75798, #87102, .T. ) ;
#18489=CARTESIAN_POINT ( 'NONE',  ( 28.37476903720190080, 1508.765197038709857, 209.4266949452929794 ) ) ;
#18492=CARTESIAN_POINT ( 'NONE',  ( -23.91153816693510592, 1410.421621729604794, 208.6572396396597355 ) ) ;
#18494=CARTESIAN_POINT ( 'NONE',  ( 11.09436156092809966, 1397.627175189450099, 216.7935160369219716 ) ) ;
#18496=CARTESIAN_POINT ( 'NONE',  ( -18.04322080909999926, 1457.691026831229919, 229.4369243693979854 ) ) ;
#18501=ORIENTED_EDGE ( 'NONE', *, *, #17206, .F. ) ;
#18502=CARTESIAN_POINT ( 'NONE',  ( -0.3187450556299999960, 1417.474787828929948, 184.6859738898979799 ) ) ;
#18503=CARTESIAN_POINT ( 'NONE',  ( 10.54091203686897416, 1446.571174882411242, 153.1861154149677589 ) ) ;
#18505=CARTESIAN_POINT ( 'NONE',  ( -0.7274293653769999812, 1461.199170862730170, 235.2852282102980155 ) ) ;
#18509=EDGE_CURVE ( 'NONE', #60035, #51052, #71117, .T. ) ;
#18513=ORIENTED_EDGE ( 'NONE', *, *, #62702, .T. ) ;
#18514=CARTESIAN_POINT ( 'NONE',  ( 11.85851152176929979, 1431.806602705250043, 149.9566501966939995 ) ) ;
#18519=CARTESIAN_POINT ( 'NONE',  ( 8.897726803999999490, 1507.634723498030098, 234.8284024826979817 ) ) ;
#18520=EDGE_CURVE ( 'NONE', #16786, #48269, #8426, .T. ) ;
#18522=CARTESIAN_POINT ( 'NONE',  ( -5.138143496799999710, 1421.871349575429804, 186.0645463248980036 ) ) ;
#18523=CARTESIAN_POINT ( 'NONE',  ( 1.454159971469330070, 1408.575797871499844, 270.4288814118980326 ) ) ;
#18533=CARTESIAN_POINT ( 'NONE',  ( 15.41004394052340132, 1507.593738228510119, 226.1372084082059928 ) ) ;
#18534=CARTESIAN_POINT ( 'NONE',  ( 17.98982283035719831, 1423.319075982959930, 225.1697406702290323 ) ) ;
#18537=CARTESIAN_POINT ( 'NONE',  ( 7.993605777300000598E-15, 1410.951844103529993, 268.3665355202980436 ) ) ;
#18540=B_SPLINE_SURFACE_WITH_KNOTS ( 'NONE', 5, 5, ( 
 ( #42510, #77781, #67186, #94014, #15626, #17834, #49832, #43079, #83962 ),
 ( #7804, #51469, #85056, #34112, #59345, #7262, #67739, #8346, #76670 ),
 ( #77239, #68302, #85601, #68850, #102952, #75591, #58775, #92913, #16186 ),
 ( #101287, #41971, #76123, #26253, #101848, #93454, #44186, #11141, #78327 ),
 ( #38383, #90436, #22105, #62109, #82035, #104073, #64730, #19510, #13713 ),
 ( #107246, #29979, #73106, #44748, #56305, #107801, #2204, #10577, #38926 ),
 ( #53715, #47899, #104630, #39499, #52592, #81476, #64171, #70515, #13162 ),
 ( #1639, #45301, #5340, #73674, #95131, #47349, #61005, #69959, #35777 ),
 ( #79441, #30539, #78898, #18949, #98844, #27368, #72559, #106688, #18393 ) ),
 .UNSPECIFIED., .F., .F., .F.,
 ( 6, 3, 6 ),
 ( 6, 3, 6 ),
 ( 19.36767300329999841, 21.57900985360000234, 24.75070551640000005 ),
 ( 0.000000000000000000, 1.000000000000000000, 2.000000000000000000 ),
 .UNSPECIFIED. ) ;
#18545=ORIENTED_EDGE ( 'NONE', *, *, #14450, .T. ) ;
#18547=CARTESIAN_POINT ( 'NONE',  ( -24.31663498039999638, 1442.649881727339789, 211.4598683180379908 ) ) ;
#18549=CARTESIAN_POINT ( 'NONE',  ( -14.45783243223209880, 1416.839692136300073, 221.3920770721769884 ) ) ;
#18550=CARTESIAN_POINT ( 'NONE',  ( 27.01381218759999925, 1450.681579806120226, 136.4483250053980044 ) ) ;
#18551=CARTESIAN_POINT ( 'NONE',  ( 14.10736255014890084, 1509.405700343320177, 234.8174336805699909 ) ) ;
#18553=CARTESIAN_POINT ( 'NONE',  ( 13.21074212996050079, 1428.906843343100036, 222.3308662938179907 ) ) ;
#18555=CARTESIAN_POINT ( 'NONE',  ( 4.407100737270000401, 1415.074620172329787, 231.6221103901980030 ) ) ;
#18557=CARTESIAN_POINT ( 'NONE',  ( -17.03425942710000029, 1460.964640061230057, 228.2738983644979953 ) ) ;
#18559=CARTESIAN_POINT ( 'NONE',  ( 26.91412824380000046, 1412.677791826929933, 269.0204588372980083 ) ) ;
#18560=CARTESIAN_POINT ( 'NONE',  ( 23.94500711619999933, 1436.145502024209918, 139.9316946685979701 ) ) ;
#18561=CARTESIAN_POINT ( 'NONE',  ( 19.05531048790000170, 1469.162939635429893, 190.6018527114979975 ) ) ;
#18562=CARTESIAN_POINT ( 'NONE',  ( -23.65757480440000293, 1436.093104310619992, 212.3677326929179969 ) ) ;
#18564=DIRECTION ( 'NONE',  ( 0.000000000000000000, 0.000000000000000000, -1.000000000000000000 ) ) ;
#18565=CARTESIAN_POINT ( 'NONE',  ( -1.740983587059999893, 1450.463600072650024, 182.5789179400979947 ) ) ;
#18566=CARTESIAN_POINT ( 'NONE',  ( -13.86092847646930082, 1410.765486861110048, 227.1170286572800023 ) ) ;
#18568=CARTESIAN_POINT ( 'NONE',  ( -12.65017221549999960, 1441.023539904969994, 188.0792847196979949 ) ) ;
#18570=CARTESIAN_POINT ( 'NONE',  ( -31.76432722529999708, 1435.606706419230022, 135.1329931210979964 ) ) ;
#18572=ORIENTED_EDGE ( 'NONE', *, *, #43940, .T. ) ;
#18574=CARTESIAN_POINT ( 'NONE',  ( -13.02096109902269916, 1409.367762368420017, 201.7918158736540022 ) ) ;
#18575=EDGE_CURVE ( 'NONE', #758, #85844, #84360, .T. ) ;
#18576=CARTESIAN_POINT ( 'NONE',  ( -5.468515302949999324, 1438.698907413310053, 154.7381877631979989 ) ) ;
#18578=CARTESIAN_POINT ( 'NONE',  ( -37.75040342469999644, 1461.765090176830199, 268.4864265932980061 ) ) ;
#18581=ADVANCED_FACE ( 'NONE', ( #37170 ), #44474, .F. ) ;
#18582=CARTESIAN_POINT ( 'NONE',  ( 17.81563488885300117, 1417.676982138360017, 224.3990780826929949 ) ) ;
#18586=CARTESIAN_POINT ( 'NONE',  ( 16.73038498189999856, 1415.425582719929707, 215.1584419701680133 ) ) ;
#18587=CARTESIAN_POINT ( 'NONE',  ( -3.240637488290000423, 1434.541222282480021, 155.4779008716980115 ) ) ;
#18590=CARTESIAN_POINT ( 'NONE',  ( -7.888904176470000529, 1508.843978788529967, 181.1771252059980100 ) ) ;
#18591=CARTESIAN_POINT ( 'NONE',  ( -23.14291596900000059, 1409.885718316829752, 207.0974899646379868 ) ) ;
#18592=CARTESIAN_POINT ( 'NONE',  ( 14.44608937009999927, 1416.522662136229883, 196.8582539822980095 ) ) ;
#18596=DIRECTION ( 'NONE',  ( 0.000000000000000000, 0.000000000000000000, 1.000000000000000000 ) ) ;
#18600=CARTESIAN_POINT ( 'NONE',  ( -22.77810859050000047, 1410.208903787329973, 210.9686725571380066 ) ) ;
#18602=CARTESIAN_POINT ( 'NONE',  ( -0.1059456692259999888, 1414.379792559529960, 233.4365792652980076 ) ) ;
#18605=CARTESIAN_POINT ( 'NONE',  ( -23.43225536839999990, 1425.871618787629814, 211.3010252580280053 ) ) ;
#18607=CARTESIAN_POINT ( 'NONE',  ( -1.483050551783430038, 1420.942730047339865, 183.9156232671229816 ) ) ;
#18609=CARTESIAN_POINT ( 'NONE',  ( -7.991989199987382442, 1398.150427817915897, 219.3750528887007647 ) ) ;
#18610=CARTESIAN_POINT ( 'NONE',  ( -17.38301961261850082, 1485.251990578760115, 188.4777382281349958 ) ) ;
#18611=CARTESIAN_POINT ( 'NONE',  ( 2.744339645710000219, 1509.008894839529830, 238.2322746441979859 ) ) ;
#18613=CARTESIAN_POINT ( 'NONE',  ( 38.88053497846389917, 1448.078305046199830, 136.4777416074680048 ) ) ;
#18616=ORIENTED_EDGE ( 'NONE', *, *, #21255, .F. ) ;
#18617=CARTESIAN_POINT ( 'NONE',  ( 11.74365990218139899, 1433.750782862119877, 150.9400914570229872 ) ) ;
#18619=VERTEX_POINT ( 'NONE', #59748 ) ;
#18620=DIRECTION ( 'NONE',  ( -0.007750486606685237645, 0.0002706418309149287806, 0.9999699279030140886 ) ) ;
#18621=EDGE_CURVE ( 'NONE', #106344, #91492, #32204, .T. ) ;
#18626=CARTESIAN_POINT ( 'NONE',  ( 6.629188914260000232, 1428.588785140030041, 91.31218443469779800 ) ) ;
#18630=CARTESIAN_POINT ( 'NONE',  ( 5.636002709010000444, 1488.168530458630130, 183.0004181446979885 ) ) ;
#18632=CARTESIAN_POINT ( 'NONE',  ( 15.35953408680000010, 1409.616044574130228, 226.6522495080980093 ) ) ;
#18633=B_SPLINE_SURFACE_WITH_KNOTS ( 'NONE', 5, 5, ( 
 ( #72987, #4671, #38810, #13591, #107124, #30415, #32071, #72447, #98722 ),
 ( #65692, #56733, #21982, #83563, #6320, #56174, #22533, #48901, #90313 ),
 ( #39926, #47779, #90870, #81914, #74094, #91436, #40468, #14158, #48344 ),
 ( #74643, #66262, #82483, #57847, #91974, #49441, #38262, #2017, #9290 ),
 ( #35033, #17094, #51855, #59703, #18219, #69212, #36153, #78704, #102234 ),
 ( #10382, #9834, #26629, #8719, #77601, #93282, #42336, #34489, #68664 ),
 ( #110640, #94373, #59163, #69779, #51286, #17654, #52964, #18767, #8167 ),
 ( #1441, #52415, #103321, #102764, #85420, #101664, #24953, #87097, #16545 ),
 ( #26060, #85992, #33925, #78138, #60255, #68121, #25511, #93815, #42898 ),
 ( #43453, #77056, #50736, #60825, #363, #907, #94950, #84869, #86541 ),
 ( #44555, #76488, #44003, #35587, #103897, #27196, #61379, #95498, #96048 ),
 ( #36698, #97703, #10952, #105569, #28855, #27741, #19319, #45681, #96611 ),
 ( #81428, #2576, #28295, #4205, #61932, #3678, #19880, #20425, #62491 ),
 ( #37806, #4739, #47304, #70892, #29936, #89849, #89304, #106108, #88212 ),
 ( #53520, #45124, #3126, #37254, #63586, #79266, #63050, #87663, #38337 ) ),
 .UNSPECIFIED., .F., .F., .F.,
 ( 6, 3, 3, 3, 6 ),
 ( 6, 3, 6 ),
 ( 3.366324640010000202, 5.876786115260000720, 8.564366035440000857, 10.59338889530000039, 13.45705438670000120 ),
 ( 0.000000000000000000, 1.000000000000000000, 2.000000000000000000 ),
 .UNSPECIFIED. ) ;
#18635=CARTESIAN_POINT ( 'NONE',  ( 36.12226356638380054, 1436.069430018940011, 134.0999999971620014 ) ) ;
#18639=CARTESIAN_POINT ( 'NONE',  ( 13.85944100054009986, 1434.989460371399900, 148.7312857378809952 ) ) ;
#18641=ORIENTED_EDGE ( 'NONE', *, *, #26073, .F. ) ;
#18643=ORIENTED_EDGE ( 'NONE', *, *, #49995, .F. ) ;
#18644=EDGE_CURVE ( 'NONE', #29004, #57276, #10797, .T. ) ;
#18646=CARTESIAN_POINT ( 'NONE',  ( -0.8516783078649999839, 1465.062050906930153, 236.8964322150979740 ) ) ;
#18651=CARTESIAN_POINT ( 'NONE',  ( -18.74243217561350505, 1444.811426355574213, 213.3821054765419376 ) ) ;
#18653=CARTESIAN_POINT ( 'NONE',  ( 4.269062038300520001, 1446.683782444980125, 158.1563956602039980 ) ) ;
#18654=CARTESIAN_POINT ( 'NONE',  ( -0.02849522097719999966, 1508.320473262429914, 237.7718752957979973 ) ) ;
#18658=CARTESIAN_POINT ( 'NONE',  ( 25.01214927662029908, 1440.913060387330006, 239.1462821668919787 ) ) ;
#18661=CARTESIAN_POINT ( 'NONE',  ( 26.84712632248179887, 1449.046460843219847, 136.7362323706379925 ) ) ;
#18662=CARTESIAN_POINT ( 'NONE',  ( -13.92641980429999826, 1410.772210879729982, 190.1674550056980024 ) ) ;
#18663=DIRECTION ( 'NONE',  ( 1.989694733329999956E-13, 6.948167114160000380E-15, -1.000000000000000000 ) ) ;
#18666=CARTESIAN_POINT ( 'NONE',  ( -12.41422776365670799, 1434.346862065572623, 147.3431289795544785 ) ) ;
#18667=ADVANCED_FACE ( 'NONE', ( #98715 ), #66252, .F. ) ;
#18672=EDGE_CURVE ( 'NONE', #44714, #29814, #90862, .T. ) ;
#18673=B_SPLINE_SURFACE_WITH_KNOTS ( 'NONE', 4, 5, ( 
 ( #20675, #103748, #76340, #27590, #25357, #17501 ),
 ( #33770, #34882, #27050, #54875, #104301, #34335 ),
 ( #18611, #43846, #18070, #10233, #51698, #44410 ),
 ( #103171, #752, #61775, #67966, #52264, #59550 ),
 ( #1298, #95899, #211, #16944, #8022, #78550 ) ),
 .UNSPECIFIED., .F., .F., .F.,
 ( 5, 5 ),
 ( 6, 6 ),
 ( 4.939581942080000232, 5.112719791149999971 ),
 ( 0.000000000000000000, 2.000000000000000000 ),
 .UNSPECIFIED. ) ;
#18677=CARTESIAN_POINT ( 'NONE',  ( 29.28654147530000174, 1509.872632245929935, 208.8940174685830016 ) ) ;
#18679=CARTESIAN_POINT ( 'NONE',  ( 13.98887932740000117, 1409.902971935330015, 191.4712550325980089 ) ) ;
#18683=CARTESIAN_POINT ( 'NONE',  ( 26.02371791099999854, 1449.849912737939803, 231.9820475135979905 ) ) ;
#18684=CARTESIAN_POINT ( 'NONE',  ( 2.886380516782709904, 1451.746737126376729, 183.8547243489458083 ) ) ;
#18685=CARTESIAN_POINT ( 'NONE',  ( -27.55179926645890021, 1509.875190418580132, 219.2242857432399887 ) ) ;
#18686=CARTESIAN_POINT ( 'NONE',  ( -2.551512840923239711, 1507.143442698440140, 236.9472663481859911 ) ) ;
#18687=CARTESIAN_POINT ( 'NONE',  ( -18.55872592980000135, 1457.839997766830038, 227.5285588847980023 ) ) ;
#18689=B_SPLINE_CURVE_WITH_KNOTS ( 'NONE', 3,
 ( #20494, #46308, #80437, #72067, #92674, #42282, #91021, #40627, #59104, #32230, #8116, #110039, #100528, #6476, #7024, #66410, #74797, #108941, #101611, #16495, #5930, #40076, #83187, #76433, #58548, #68062, #108388, #66956, #57999, #102176, #50152, #101066, #33313, #15952, #23807, #84281, #99968, #56890, #67507, #14308, #24896, #92133 ),
 .UNSPECIFIED., .F., .F.,
 ( 4, 2, 2, 2, 2, 2, 1, 1, 1, 1, 1, 2, 2, 2, 2, 2, 1, 1, 1, 2, 2, 2, 2, 2, 4 ),
 ( 0.000000000000000000, 0.06249999999974691078, 0.1249999999994938216, 0.1874999999992407185, 0.2187499999991080746, 0.2343749999990482891, 0.2421874999990115684, 0.2460937499989931943, 0.2480468749989771515, 0.2490234374989692134, 0.2495117187489654109, 0.2497558593739636346, 0.2499999999989618304, 0.3749999999990640820, 0.4374999999991111554, 0.4687499999991348032, 0.4843749999991467381, 0.4921874999991526778, 0.4960937499991557864, 0.4980468749991602828, 0.4999999999991647792, 0.6249999999993736122, 0.7499999999995823341, 0.8749999999997911670, 1.000000000000000000 ),
 .UNSPECIFIED. ) ;
#18690=CARTESIAN_POINT ( 'NONE',  ( 10.96878214529999873, 1432.307818762199986, 151.7701606857980039 ) ) ;
#18691=CARTESIAN_POINT ( 'NONE',  ( 17.96820147240839916, 1410.603916924019813, 222.9561480445759969 ) ) ;
#18692=DIRECTION ( 'NONE',  ( 0.000000000000000000, 0.000000000000000000, 1.000000000000000000 ) ) ;
#18696=CARTESIAN_POINT ( 'NONE',  ( 0.1067562447540000015, 1406.506670174130022, 269.4986873273979882 ) ) ;
#18698=CARTESIAN_POINT ( 'NONE',  ( 27.94676410629999808, 1509.200065888029940, 207.5540313486380057 ) ) ;
#18700=CARTESIAN_POINT ( 'NONE',  ( 6.588862402215439396, 1473.264983703350026, 270.4290835591440327 ) ) ;
#18705=CARTESIAN_POINT ( 'NONE',  ( -26.21059033610000100, 1446.264569515290077, 137.9459526830979996 ) ) ;
#18706=CARTESIAN_POINT ( 'NONE',  ( 2.424607408659378738, 1449.446473553185797, 154.4675859022806321 ) ) ;
#18712=ORIENTED_EDGE ( 'NONE', *, *, #65604, .F. ) ;
#18717=CARTESIAN_POINT ( 'NONE',  ( -0.3323210813560000254, 1416.988076901430077, 234.1774585115979903 ) ) ;
#18723=CARTESIAN_POINT ( 'NONE',  ( 26.13227424183079961, 1436.228979033299993, 136.7358178123800201 ) ) ;
#18725=CARTESIAN_POINT ( 'NONE',  ( -13.42559421921827756, 1443.464041502655164, 169.3656302353889771 ) ) ;
#18727=B_SPLINE_CURVE_WITH_KNOTS ( 'NONE', 3,
 ( #46343, #28967, #82106, #72623, #38992, #80472, #55286, #5404, #54738, #97256 ),
 .UNSPECIFIED., .F., .F.,
 ( 4, 2, 2, 2, 4 ),
 ( -0.1172112179306550039, -0.1055921015938769969, -0.09159876550525229699, -0.04939298262307730003, -2.270117807623428519E-08 ),
 .UNSPECIFIED. ) ;
#18728=ADVANCED_FACE ( 'NONE', ( #85209 ), #28306, .T. ) ;
#18730=CARTESIAN_POINT ( 'NONE',  ( 2.461716435160000049, 1435.943783413959864, 150.4083956814980070 ) ) ;
#18735=CARTESIAN_POINT ( 'NONE',  ( -9.499897081856666148, 1447.499268979973067, 186.3975894871608432 ) ) ;
#18736=CARTESIAN_POINT ( 'NONE',  ( 9.970730613730001579, 1425.233768695029994, 92.69245245969780456 ) ) ;
#18737=DIRECTION ( 'NONE',  ( 1.000000000000000000, 3.155441816300000491E-15, -4.343610028670000616E-15 ) ) ;
#18740=CARTESIAN_POINT ( 'NONE',  ( 4.147542412012739987, 1424.336585509140150, 184.6878609135509919 ) ) ;
#18747=CARTESIAN_POINT ( 'NONE',  ( -1.450401175619670857, 1465.036285778872980, 237.9109514038669886 ) ) ;
#18749=ORIENTED_EDGE ( 'NONE', *, *, #52842, .F. ) ;
#18750=CARTESIAN_POINT ( 'NONE',  ( -41.15112044609999487, 1443.645550130990159, 136.9181562709980255 ) ) ;
#18751=CARTESIAN_POINT ( 'NONE',  ( 0.8193110093525590720, 1474.780960361229745, 235.8603769791739921 ) ) ;
#18752=DIRECTION ( 'NONE',  ( -1.987538202299999878E-13, 0.000000000000000000, 1.000000000000000000 ) ) ;
#18757=CARTESIAN_POINT ( 'NONE',  ( 10.80134480061129842, 1446.564900598669965, 153.0805715986590201 ) ) ;
#18758=CARTESIAN_POINT ( 'NONE',  ( -35.06783964556029787, 1451.227222927539970, 135.9148696056909955 ) ) ;
#18759=CARTESIAN_POINT ( 'NONE',  ( -2.500000000000000000, 1448.271846337009947, 165.0527805226990097 ) ) ;
#18760=CARTESIAN_POINT ( 'NONE',  ( 5.343479918049999888, 1396.099658817830004, 218.7752541424879951 ) ) ;
#18761=CARTESIAN_POINT ( 'NONE',  ( 6.845616174217879824, 1409.091719448260164, 195.7806122793810175 ) ) ;
#18762=CARTESIAN_POINT ( 'NONE',  ( -0.7759870753352450246, 1405.716808862310018, 267.8539888477289992 ) ) ;
#18765=VERTEX_POINT ( 'NONE', #36472 ) ;
#18767=CARTESIAN_POINT ( 'NONE',  ( 14.11608679399999922, 1444.853469894119826, 189.4447253316980095 ) ) ;
#18771=CARTESIAN_POINT ( 'NONE',  ( -11.60004869885204215, 1426.273944179774844, 138.2686100621498326 ) ) ;
#18776=ADVANCED_FACE ( 'NONE', ( #96945 ), #4216, .F. ) ;
#18781=CARTESIAN_POINT ( 'NONE',  ( -27.92468909959999834, 1509.154588341429871, 205.8536344554680113 ) ) ;
#18782=B_SPLINE_SURFACE_WITH_KNOTS ( 'NONE', 5, 5, ( 
 ( #7993, #77417, #722, #69041, #26443, #60638 ),
 ( #104272, #106472, #89118, #63947, #12948, #46041 ),
 ( #88586, #53336, #29757, #79090, #45499, #70161 ),
 ( #95866, #4034, #71819, #2943, #104823, #27560 ),
 ( #105940, #28109, #62874, #87484, #61744, #98060 ),
 ( #89662, #20793, #54995, #38162, #37617, #29218 ) ),
 .UNSPECIFIED., .F., .F., .F.,
 ( 6, 6 ),
 ( 6, 6 ),
 ( 42.64499113449999612, 56.13383365260000346 ),
 ( 0.000000000000000000, 2.000000000000000000 ),
 .UNSPECIFIED. ) ;
#18784=CARTESIAN_POINT ( 'NONE',  ( 40.26396420611710170, 1444.186530323160014, 137.1012295353969819 ) ) ;
#18786=CARTESIAN_POINT ( 'NONE',  ( 20.50000000000000000, 1443.913060387330006, 169.0968414572980123 ) ) ;
#18787=CARTESIAN_POINT ( 'NONE',  ( -4.226789392379999732, 1409.996198396630007, 232.1190139888980184 ) ) ;
#18788=CARTESIAN_POINT ( 'NONE',  ( -5.757247049150000073, 1446.202579340599868, 184.3601040033979928 ) ) ;
#18789=ORIENTED_EDGE ( 'NONE', *, *, #18520, .T. ) ;
#18791=CARTESIAN_POINT ( 'NONE',  ( -13.96141271054625399, 1435.007883397890055, 148.7887677015099257 ) ) ;
#18793=CARTESIAN_POINT ( 'NONE',  ( 19.15622051997149811, 1456.936057672450261, 224.8950397092459923 ) ) ;
#18795=CARTESIAN_POINT ( 'NONE',  ( -24.64665313769999955, 1435.432891414579899, 136.6581518711979868 ) ) ;
#18796=EDGE_CURVE ( 'NONE', #5392, #38044, #109745, .T. ) ;
#18799=CARTESIAN_POINT ( 'NONE',  ( -12.87561223598270033, 1428.667272998819954, 222.5140706137790119 ) ) ;
#18802=CARTESIAN_POINT ( 'NONE',  ( 22.11164323276918608, 1411.043578901620094, 203.7708757951590428 ) ) ;
#18806=CARTESIAN_POINT ( 'NONE',  ( 2.500000000000000000, 1437.759198978020095, 157.6719144024980039 ) ) ;
#18807=CARTESIAN_POINT ( 'NONE',  ( -1.746867988079999989, 1410.306430355730072, 232.8692363036980169 ) ) ;
#18812=CARTESIAN_POINT ( 'NONE',  ( 12.11785592040000026, 1434.486425630220083, 150.7184365762979894 ) ) ;
#18813=CARTESIAN_POINT ( 'NONE',  ( 16.09934221701070101, 1488.408557597590061, 230.7030962951629931 ) ) ;
#18815=CARTESIAN_POINT ( 'NONE',  ( -24.09814616333339998, 1444.255785637029931, 212.5772553280679915 ) ) ;
#18818=CARTESIAN_POINT ( 'NONE',  ( 0.003115715631340339620, 1420.443923427290201, 182.6727572773859833 ) ) ;
#18820=CARTESIAN_POINT ( 'NONE',  ( -4.463702575220000135, 1420.728434228329888, 186.4092242875980219 ) ) ;
#18821=CARTESIAN_POINT ( 'NONE',  ( 19.05944848800000102, 1508.258419250929819, 188.5048453100980055 ) ) ;
#18827=CARTESIAN_POINT ( 'NONE',  ( 3.666229469220000148, 1421.722428054930106, 183.6097529654979894 ) ) ;
#18832=CARTESIAN_POINT ( 'NONE',  ( -15.94347048536829803, 1409.469818645040050, 192.9752432267480060 ) ) ;
#18833=CARTESIAN_POINT ( 'NONE',  ( 17.58950218620000072, 1415.041103189330215, 210.4382088494780021 ) ) ;
#18834=CARTESIAN_POINT ( 'NONE',  ( -19.04437315719999901, 1425.784752839030034, 226.3805134473980161 ) ) ;
#18835=CARTESIAN_POINT ( 'NONE',  ( -15.10045379129999965, 1436.261357401330088, 149.5558351856980153 ) ) ;
#18839=CARTESIAN_POINT ( 'NONE',  ( -9.854212473397289784, 1509.383236553660026, 180.6764149878760009 ) ) ;
#18842=CARTESIAN_POINT ( 'NONE',  ( 1.555973022161739827, 1415.219159636500081, 191.2001064328639757 ) ) ;
#18846=CARTESIAN_POINT ( 'NONE',  ( -3.639483821036900046, 1426.011012282639740, 185.9494021309836569 ) ) ;
#18853=DIRECTION ( 'NONE',  ( -0.7071067811860475283, 0.000000000000000000, -0.7071067811870476172 ) ) ;
#18858=CARTESIAN_POINT ( 'NONE',  ( 17.25022834990030063, 1507.614846683550240, 193.9485721999670034 ) ) ;
#18861=VERTEX_POINT ( 'NONE', #17292 ) ;
#18863=CARTESIAN_POINT ( 'NONE',  ( 19.72894155641759895, 1509.632479176759944, 231.2927645791820055 ) ) ;
#18865=CARTESIAN_POINT ( 'NONE',  ( 12.93207668273189981, 1442.909017868442334, 169.4317201798534711 ) ) ;
#18867=CARTESIAN_POINT ( 'NONE',  ( -43.50118975519999509, 1443.586702812149952, 263.8966299882980024 ) ) ;
#18870=CARTESIAN_POINT ( 'NONE',  ( 24.90812900910000138, 1507.935970732329906, 197.8880224007980075 ) ) ;
#18872=CARTESIAN_POINT ( 'NONE',  ( 8.355631587939999605, 1410.577119414130038, 187.7490234216979843 ) ) ;
#18874=CARTESIAN_POINT ( 'NONE',  ( -7.765022151240000170, 1439.035228022859883, 153.8379896386979908 ) ) ;
#18875=CARTESIAN_POINT ( 'NONE',  ( 10.92774547339999991, 1436.036448765360092, 151.9134061906980264 ) ) ;
#18877=CARTESIAN_POINT ( 'NONE',  ( -8.983165774390000635, 1452.599361326030248, 151.2716590506979912 ) ) ;
#18879=ORIENTED_EDGE ( 'NONE', *, *, #101526, .T. ) ;
#18883=CARTESIAN_POINT ( 'NONE',  ( -40.67651829279999731, 1454.550461609130025, 270.1403828920980459 ) ) ;
#18885=CARTESIAN_POINT ( 'NONE',  ( 17.57263885140000070, 1409.691669004730102, 222.6387591511980020 ) ) ;
#18886=CARTESIAN_POINT ( 'NONE',  ( -14.60169229409999936, 1463.277005629129917, 223.3429056284980163 ) ) ;
#18889=EDGE_CURVE ( 'NONE', #36972, #45161, #69727, .T. ) ;
#18890=CARTESIAN_POINT ( 'NONE',  ( 2.925549591967640417, 1409.954410087670112, 231.5402738976679871 ) ) ;
#18892=CARTESIAN_POINT ( 'NONE',  ( -4.619855912889999416, 1417.833749415829971, 234.7627619328980018 ) ) ;
#18894=CARTESIAN_POINT ( 'NONE',  ( -1.311131513420452421, 1484.544387571488642, 182.3338937980581420 ) ) ;
#18896=CARTESIAN_POINT ( 'NONE',  ( -45.24356817553269394, 1434.454005103070131, 268.5215513401200269 ) ) ;
#18897=CARTESIAN_POINT ( 'NONE',  ( -2.694874838370000081, 1434.191529021039969, 184.8910710316980044 ) ) ;
#18900=VERTEX_POINT ( 'NONE', #23514 ) ;
#18906=ORIENTED_EDGE ( 'NONE', *, *, #22964, .T. ) ;
#18907=CARTESIAN_POINT ( 'NONE',  ( 24.33278372090000019, 1437.669624983799849, 213.0855618553079864 ) ) ;
#18909=CARTESIAN_POINT ( 'NONE',  ( 14.69112492350000032, 1470.808655613429892, 194.6682620091980027 ) ) ;
#18915=CARTESIAN_POINT ( 'NONE',  ( -28.49266032979539887, 1415.418434190969947, 270.1377136304399755 ) ) ;
#18917=CARTESIAN_POINT ( 'NONE',  ( 8.821431567077510749, 1419.123291530620008, 231.9106426862639978 ) ) ;
#18920=ORIENTED_EDGE ( 'NONE', *, *, #80622, .T. ) ;
#18921=ORIENTED_EDGE ( 'NONE', *, *, #14581, .T. ) ;
#18923=CARTESIAN_POINT ( 'NONE',  ( -0.5926620228766540377, 1409.870422386290102, 185.1089675646719854 ) ) ;
#18924=CARTESIAN_POINT ( 'NONE',  ( 3.712429952897377650, 1424.143221639157218, 183.8426287002268964 ) ) ;
#18925=CARTESIAN_POINT ( 'NONE',  ( -0.02711300940577089993, 1409.107386744810128, 185.7397112177479812 ) ) ;
#18927=CARTESIAN_POINT ( 'NONE',  ( -20.51079079204400202, 1491.138387813179861, 192.7050494188490006 ) ) ;
#18928=CARTESIAN_POINT ( 'NONE',  ( -22.98680169079999658, 1425.805257318429994, 213.5345393129279898 ) ) ;
#18930=CARTESIAN_POINT ( 'NONE',  ( 28.46682226171239805, 1468.433058268769855, 268.7218470584510328 ) ) ;
#18932=CARTESIAN_POINT ( 'NONE',  ( -4.819546534003323224, 1466.444145834148230, 234.4964832952103677 ) ) ;
#18933=CARTESIAN_POINT ( 'NONE',  ( -17.36107116584603105, 1422.621875767651090, 226.5805576276689521 ) ) ;
#18938=CARTESIAN_POINT ( 'NONE',  ( 1.511551524885510034, 1460.417055334569795, 183.1515410192469915 ) ) ;
#18939=CARTESIAN_POINT ( 'NONE',  ( 23.81211169210000378, 1410.396487169730108, 208.4716996890240068 ) ) ;
#18942=CARTESIAN_POINT ( 'NONE',  ( 24.38835192978790189, 1452.061422661730148, 136.1897709901290057 ) ) ;
#18943=CARTESIAN_POINT ( 'NONE',  ( 11.08292358395013721, 1424.905641017491462, 138.1229852948969494 ) ) ;
#18946=CARTESIAN_POINT ( 'NONE',  ( 18.50440636980000164, 1410.921881894329772, 194.3442019313980040 ) ) ;
#18948=CARTESIAN_POINT ( 'NONE',  ( 2.898851852405722962, 1439.669638370619850, 183.9687869958605404 ) ) ;
#18949=CARTESIAN_POINT ( 'NONE',  ( -0.02483722075589999898, 1416.432140559029904, 233.7186305100979951 ) ) ;
#18950=CARTESIAN_POINT ( 'NONE',  ( -20.51844432163499832, 1427.241484048884786, 221.4774438843884639 ) ) ;
#18951=CARTESIAN_POINT ( 'NONE',  ( 0.3619638413112999387, 1452.022047269289942, 183.1176328467209942 ) ) ;
#18952=CARTESIAN_POINT ( 'NONE',  ( -0.002537736600710310125, 1508.960873149719873, 179.4060637200210238 ) ) ;
#18955=CARTESIAN_POINT ( 'NONE',  ( 27.31124572860469968, 1446.324645400339932, 137.1901751446029891 ) ) ;
#18959=CARTESIAN_POINT ( 'NONE',  ( -0.4878771540074440249, 1409.607344574789977, 232.9569252667809849 ) ) ;
#18960=CARTESIAN_POINT ( 'NONE',  ( 9816.840209715130186, 50.13405481578730161, 1424.308828391600173 ) ) ;
#18961=( BOUNDED_CURVE ( )  B_SPLINE_CURVE ( 3, ( #32126, #66311, #100428, #61090 ),
 .UNSPECIFIED., .F., .F. ) 
 B_SPLINE_CURVE_WITH_KNOTS ( ( 4, 4 ),
 ( 4.246412475983603940, 5.177358128112214963 ),
 .UNSPECIFIED. ) 
 CURVE ( )  GEOMETRIC_REPRESENTATION_ITEM ( )  RATIONAL_B_SPLINE_CURVE ( ( 1.000000000000000000, 0.9290729598085936125, 0.9290729598085936125, 1.000000000000000000 ) ) 
 REPRESENTATION_ITEM ( '' )  );
#18964=CARTESIAN_POINT ( 'NONE',  ( 1.043609643150000005E-14, 1456.909266842430043, 224.8635561844979804 ) ) ;
#18965=CARTESIAN_POINT ( 'NONE',  ( 36.73763096499994418, 1461.736697325623254, 266.4403429611982119 ) ) ;
#18967=CARTESIAN_POINT ( 'NONE',  ( 13.84930592310000108, 1450.388901282120059, 209.1218459616979999 ) ) ;
#18973=CARTESIAN_POINT ( 'NONE',  ( 8.235306720422707727, 1398.157613047823361, 199.0622384067150108 ) ) ;
#18974=CARTESIAN_POINT ( 'NONE',  ( 0.04570590800825859862, 1508.911464302090053, 238.4015887634199942 ) ) ;
#18975=CARTESIAN_POINT ( 'NONE',  ( 22.70805115470000146, 1469.235391016429958, 220.6124962964979943 ) ) ;
#18977=CARTESIAN_POINT ( 'NONE',  ( -36.93911630280124569, 1436.285477273010429, 135.0345624054817790 ) ) ;
#18985=CARTESIAN_POINT ( 'NONE',  ( -1.121465818060000119, 1416.819759814730105, 228.0845569899979921 ) ) ;
#18987=CARTESIAN_POINT ( 'NONE',  ( -27.33784579440922613, 1509.867718998758846, 219.6686939752406147 ) ) ;
#18988=CARTESIAN_POINT ( 'NONE',  ( -34.34692909063059574, 1451.701922534410187, 134.0999999981429767 ) ) ;
#18989=ORIENTED_EDGE ( 'NONE', *, *, #57733, .F. ) ;
#18993=CARTESIAN_POINT ( 'NONE',  ( -16.02395347670000447, 1414.971262582530017, 214.1105671929480252 ) ) ;
#18995=DIRECTION ( 'NONE',  ( -0.0003696129300649848913, 0.001489947244085779296, -0.9999988217210517005 ) ) ;
#18998=CARTESIAN_POINT ( 'NONE',  ( 13.92362594963720035, 1409.399284119610229, 203.7196187947509998 ) ) ;
#19001=CARTESIAN_POINT ( 'NONE',  ( -17.83186546889999846, 1421.470479459229864, 192.3242510227980233 ) ) ;
#19009=CARTESIAN_POINT ( 'NONE',  ( 25.61065848249999988, 1508.555233516829958, 218.7406679075980094 ) ) ;
#19011=CARTESIAN_POINT ( 'NONE',  ( -11.97796580090000162, 1433.627075391659901, 150.2895221116980053 ) ) ;
#19012=CARTESIAN_POINT ( 'NONE',  ( 29.43805146511517279, 1509.956782691962644, 212.2118635277215901 ) ) ;
#19013=DIRECTION ( 'NONE',  ( 0.7074300732573276518, 0.02470400251971152997, -0.7063514732133275853 ) ) ;
#19014=CARTESIAN_POINT ( 'NONE',  ( -27.93158978740000009, 1508.017348977630036, 210.2982006691480024 ) ) ;
#19017=CARTESIAN_POINT ( 'NONE',  ( -0.5328017128810000891, 1467.450758361530006, 182.6307715436979890 ) ) ;
#19019=DIRECTION ( 'NONE',  ( 0.000000000000000000, 0.000000000000000000, -1.000000000000000000 ) ) ;
#19021=CARTESIAN_POINT ( 'NONE',  ( 2.500000000000000000, 1448.210448409899982, 182.3842139592889851 ) ) ;
#19023=CARTESIAN_POINT ( 'NONE',  ( -12.99004886546730120, 1434.775507592019949, 149.1620289331810056 ) ) ;
#19024=CARTESIAN_POINT ( 'NONE',  ( -2.500000000000000000, 1432.593627935599898, 157.5021872924980073 ) ) ;
#19025=CARTESIAN_POINT ( 'NONE',  ( -0.3657622740145609619, 1430.070695917230069, 190.4861624611909861 ) ) ;
#19032=CARTESIAN_POINT ( 'NONE',  ( 39.02581916309999599, 1422.344273220830019, 266.4771548496979676 ) ) ;
#19033=CARTESIAN_POINT ( 'NONE',  ( -25.92853884490000027, 1469.242862528429896, 205.7879372785779992 ) ) ;
#19034=CARTESIAN_POINT ( 'NONE',  ( -10.03650023711350059, 1425.202651915989918, 96.73419986872309551 ) ) ;
#19035=CARTESIAN_POINT ( 'NONE',  ( 16.44149578104170217, 1409.512336796159843, 193.0768534555940050 ) ) ;
#19037=CARTESIAN_POINT ( 'NONE',  ( -20.50343491230000126, 1453.154616238729886, 208.2124688364239944 ) ) ;
#19038=CARTESIAN_POINT ( 'NONE',  ( -30.53571888280000124, 1438.952188671489921, 240.1260121775979997 ) ) ;
#19040=CARTESIAN_POINT ( 'NONE',  ( 28.30911832997569988, 1508.554176139660058, 209.4091768886380294 ) ) ;
#19041=EDGE_CURVE ( 'NONE', #59250, #36202, #54904, .T. ) ;
#19043=CARTESIAN_POINT ( 'NONE',  ( 30.80316601989999725, 1450.549250348119813, 136.3368496048979921 ) ) ;
#19044=EDGE_LOOP ( 'NONE', ( #29142, #88899, #101538, #84657 ) ) ;
#19045=CARTESIAN_POINT ( 'NONE',  ( 9.185964335410000459, 1396.233841330429868, 201.6855590868979675 ) ) ;
#19047=CARTESIAN_POINT ( 'NONE',  ( -17.47006112300000069, 1460.511276975630153, 228.2420954910980129 ) ) ;
#19049=ORIENTED_EDGE ( 'NONE', *, *, #84679, .T. ) ;
#19053=CARTESIAN_POINT ( 'NONE',  ( -0.3142596228660000102, 1415.641189163630088, 184.7630716501980146 ) ) ;
#19054=CARTESIAN_POINT ( 'NONE',  ( 8.950554794200915154, 1446.632273707716877, 153.7528715246174329 ) ) ;
#19055=CARTESIAN_POINT ( 'NONE',  ( -0.1822331536658439999, 1415.403647183765997, 233.4419826045449611 ) ) ;
#19056=CARTESIAN_POINT ( 'NONE',  ( -7.167074599660000267, 1461.188551261529938, 233.4299114769979724 ) ) ;
#19057=DIRECTION ( 'NONE',  ( -0.9995237720558002303, 0.03085820952913055637, 3.241389442709986064E-08 ) ) ;
#19060=CARTESIAN_POINT ( 'NONE',  ( 14.23687710369999948, 1463.789345363929897, 224.3885670368980243 ) ) ;
#19061=ORIENTED_EDGE ( 'NONE', *, *, #10390, .F. ) ;
#19065=CARTESIAN_POINT ( 'NONE',  ( 11.82848250736780038, 1429.808088084610063, 149.3741360895739660 ) ) ;
#19066=B_SPLINE_CURVE_WITH_KNOTS ( 'NONE', 3,
 ( #50998, #41495, #103024, #68368, #77306, #8416 ),
 .UNSPECIFIED., .F., .F.,
 ( 4, 2, 4 ),
 ( -0.1558933150621664987, -0.07794925273348111971, -6.503526063517117706E-07 ),
 .UNSPECIFIED. ) ;
#19067=CARTESIAN_POINT ( 'NONE',  ( 13.11038924667559336, 1444.793296087265162, 187.1321005147183882 ) ) ;
#19069=CARTESIAN_POINT ( 'NONE',  ( -15.62937150226415994, 1506.527232289704898, 193.5520135464122973 ) ) ;
#19070=CARTESIAN_POINT ( 'NONE',  ( -13.51702042466202158, 1443.913060387330461, 169.3754641244113373 ) ) ;
#19071=CARTESIAN_POINT ( 'NONE',  ( 2.883855425570000186, 1507.998768052829973, 236.1595088610979758 ) ) ;
#19073=CARTESIAN_POINT ( 'NONE',  ( -5.638178009059999773, 1424.929087014930019, 186.4582126495980106 ) ) ;
#19074=CARTESIAN_POINT ( 'NONE',  ( 0.9815367246191329942, 1408.241645913789853, 270.3924816116769989 ) ) ;
#19080=CARTESIAN_POINT ( 'NONE',  ( -17.46895492501760216, 1435.758675877850010, 191.0377360153560176 ) ) ;
#19083=B_SPLINE_CURVE_WITH_KNOTS ( 'NONE', 3,
 ( #29983, #48474, #40048, #64734, #98848, #74230 ),
 .UNSPECIFIED., .F., .F.,
 ( 4, 2, 4 ),
 ( 0.000000000000000000, 0.1289624413956479976, 0.2573965581621350251 ),
 .UNSPECIFIED. ) ;
#19087=CARTESIAN_POINT ( 'NONE',  ( 1.199040866600000048E-14, 1420.418457356630142, 243.9198229339980060 ) ) ;
#19088=CARTESIAN_POINT ( 'NONE',  ( 13.34704934129999998, 1434.912633013909954, 148.9126644935979868 ) ) ;
#19089=AXIS2_PLACEMENT_3D ( 'NONE', #86222, #10633, #85661 ) ;
#19097=CARTESIAN_POINT ( 'NONE',  ( -2.500574544111449971, 1448.942056179399970, 154.5733147259969940 ) ) ;
#19100=CARTESIAN_POINT ( 'NONE',  ( -7.291666587149999934, 1441.356683820160015, 185.8290540692979960 ) ) ;
#19101=CARTESIAN_POINT ( 'NONE',  ( 30.96823826980000050, 1510.122676044730042, 207.2974432662780089 ) ) ;
#19103=CARTESIAN_POINT ( 'NONE',  ( -7.612906430609999830, 1431.113060387329824, 226.5499313142980213 ) ) ;
#19104=CARTESIAN_POINT ( 'NONE',  ( 16.51790355380000008, 1415.090637380430053, 226.7996615004980185 ) ) ;
#19108=CARTESIAN_POINT ( 'NONE',  ( 41.61237968540000054, 1425.046497863630066, 267.7539489489980156 ) ) ;
#19111=CARTESIAN_POINT ( 'NONE',  ( 15.39963790060000015, 1435.849252446450009, 149.2652977341979863 ) ) ;
#19112=CARTESIAN_POINT ( 'NONE',  ( 26.00771452189999877, 1488.579595437629905, 206.3082675595479998 ) ) ;
#19113=CARTESIAN_POINT ( 'NONE',  ( 20.19282076750571875, 1506.569407721386142, 218.0946391673573999 ) ) ;
#19117=CARTESIAN_POINT ( 'NONE',  ( -40.27244786589999848, 1443.155312786579998, 137.0624732611979937 ) ) ;
#19118=CARTESIAN_POINT ( 'NONE',  ( -20.00077709783896296, 1506.539416727680191, 199.7857358250231812 ) ) ;
#19119=FACE_OUTER_BOUND ( 'NONE', #84798, .T. ) ;
#19120=CARTESIAN_POINT ( 'NONE',  ( -14.29155582609999975, 1442.454908126789860, 188.8169266407979876 ) ) ;
#19124=CARTESIAN_POINT ( 'NONE',  ( -33.15527080879999744, 1435.815762631380039, 135.9678225143980228 ) ) ;
#19127=CARTESIAN_POINT ( 'NONE',  ( -13.73196314922649819, 1409.392591107120097, 203.2471964003619860 ) ) ;
#19128=CARTESIAN_POINT ( 'NONE',  ( -5.519888651039999594, 1440.499828209809948, 154.7645161259980000 ) ) ;
#19130=CARTESIAN_POINT ( 'NONE',  ( -46.02998506200000151, 1446.027519629539938, 268.4959083590979958 ) ) ;
#19131=CARTESIAN_POINT ( 'NONE',  ( -13.53916864874639892, 1429.119333790580185, 222.2883575635510169 ) ) ;
#19132=CARTESIAN_POINT ( 'NONE',  ( 0.2192322612154889994, 1419.698823279740054, 184.2916502271359889 ) ) ;
#19135=CARTESIAN_POINT ( 'NONE',  ( 17.84384396026800346, 1424.152973260369890, 226.0594126201679899 ) ) ;
#19136=CARTESIAN_POINT ( 'NONE',  ( 20.86062014670000409, 1508.959785424030088, 227.7205171458979862 ) ) ;
#19137=CARTESIAN_POINT ( 'NONE',  ( 14.71289468370000009, 1474.176701919529933, 223.5077687996979989 ) ) ;
#19141=DIRECTION ( 'NONE',  ( 0.003573437736329575058, 0.9999913661844080925, 0.002120872317184724874 ) ) ;
#19142=CARTESIAN_POINT ( 'NONE',  ( 16.09868664480000078, 1415.425582719929707, 201.5601952599979825 ) ) ;
#19145=CARTESIAN_POINT ( 'NONE',  ( 23.41884693540000129, 1409.895416813330030, 210.0743532913309934 ) ) ;
#19148=CARTESIAN_POINT ( 'NONE',  ( -5.359938512223240359, 1422.303815611070149, 145.5146526691499673 ) ) ;
#19159=CARTESIAN_POINT ( 'NONE',  ( -14.11689929294730028, 1484.918870904669802, 186.6450022189229969 ) ) ;
#19166=CARTESIAN_POINT ( 'NONE',  ( 11.94269759412389931, 1433.497490334299755, 149.9951721422179958 ) ) ;
#19172=CARTESIAN_POINT ( 'NONE',  ( 11.59417695439999996, 1428.981093279630159, 133.6118001900980232 ) ) ;
#19173=CARTESIAN_POINT ( 'NONE',  ( 11.98890328080000067, 1442.756953654919926, 147.5994355510979688 ) ) ;
#19174=CARTESIAN_POINT ( 'NONE',  ( -24.07333629580420009, 1452.056479083659951, 137.0861003737580006 ) ) ;
#19176=CARTESIAN_POINT ( 'NONE',  ( 16.40118808329999922, 1409.652464304430168, 226.0181115163979939 ) ) ;
#19177=EDGE_CURVE ( 'NONE', #93667, #85148, #86937, .T. ) ;
#19180=CARTESIAN_POINT ( 'NONE',  ( 13.64809019993819916, 1415.124054205840139, 197.6749129713249999 ) ) ;
#19182=DIRECTION ( 'NONE',  ( -0.03489951250832355745, 0.9993908264671441666, -5.513386024302311512E-10 ) ) ;
#19184=CARTESIAN_POINT ( 'NONE',  ( 14.24850174863960106, 1435.298499589599942, 149.3936294197170014 ) ) ;
#19190=CARTESIAN_POINT ( 'NONE',  ( -0.5359129219849999570, 1465.001496343030112, 237.3400905133979961 ) ) ;
#19191=CARTESIAN_POINT ( 'NONE',  ( 7.885142363431777213, 1451.393272216873129, 152.9790937285441714 ) ) ;
#19196=CARTESIAN_POINT ( 'NONE',  ( -16.68699431115342335, 1449.695428686811283, 220.1589770093310676 ) ) ;
#19200=ORIENTED_EDGE ( 'NONE', *, *, #71307, .T. ) ;
#19203=CARTESIAN_POINT ( 'NONE',  ( 28.38347306510890178, 1440.913060387330006, 248.5147831249649926 ) ) ;
#19204=CARTESIAN_POINT ( 'NONE',  ( -19.49656203970000234, 1509.532970918229921, 187.1097474216979890 ) ) ;
#19206=CARTESIAN_POINT ( 'NONE',  ( 26.18878121679949800, 1448.069869514440143, 137.2982896685190042 ) ) ;
#19207=CARTESIAN_POINT ( 'NONE',  ( -14.04658979979999955, 1410.336061500830056, 190.2513870978979753 ) ) ;
#19209=CARTESIAN_POINT ( 'NONE',  ( -24.36525012050000072, 1441.101273928379896, 211.6948751338080115 ) ) ;
#19210=FACE_OUTER_BOUND ( 'NONE', #22478, .T. ) ;
#19213=CARTESIAN_POINT ( 'NONE',  ( -11.87905392670000104, 1433.311775745339901, 149.9804763677979906 ) ) ;
#19215=EDGE_CURVE ( 'NONE', #9928, #99690, #67463, .T. ) ;
#19216=CARTESIAN_POINT ( 'NONE',  ( 2.902343019699999971, 1466.632250434329762, 234.1422827139980143 ) ) ;
#19218=AXIS2_PLACEMENT_3D ( 'NONE', #15937, #32218, #66398 ) ;
#19221=LINE ( 'NONE', #55085, #98253 ) ;
#19224=CARTESIAN_POINT ( 'NONE',  ( -18.89028803260000089, 1434.820761660239896, 209.2076715186949798 ) ) ;
#19225=CARTESIAN_POINT ( 'NONE',  ( -18.14293122912915734, 1486.179943799410239, 188.5917708767873933 ) ) ;
#19229=CARTESIAN_POINT ( 'NONE',  ( 26.01655159059999889, 1446.111954671009926, 225.7845402501980061 ) ) ;
#19230=CARTESIAN_POINT ( 'NONE',  ( -18.92249268369999982, 1456.941604937630018, 229.2980728310979828 ) ) ;
#19231=CARTESIAN_POINT ( 'NONE',  ( -29.11400471147480218, 1509.929743834820101, 212.8719597320529999 ) ) ;
#19232=CARTESIAN_POINT ( 'NONE',  ( -6.887159582019999782, 1508.131488034229960, 235.9161536093979805 ) ) ;
#19233=CARTESIAN_POINT ( 'NONE',  ( -22.76393692040000261, 1450.407194713350009, 220.5314342330980253 ) ) ;
#19235=CARTESIAN_POINT ( 'NONE',  ( -21.10174429543511110, 1411.010612129340643, 200.2662915755269637 ) ) ;
#19236=CARTESIAN_POINT ( 'NONE',  ( 16.87240902346729854, 1409.502257893559772, 222.1138755377239988 ) ) ;
#19237=CARTESIAN_POINT ( 'NONE',  ( -0.2282788349709999887, 1452.819461535030086, 189.4800008897979922 ) ) ;
#19239=ORIENTED_EDGE ( 'NONE', *, *, #49642, .T. ) ;
#19241=CARTESIAN_POINT ( 'NONE',  ( 1.740066313259999932E-09, 1405.749477561730146, 267.5371647992980115 ) ) ;
#19243=AXIS2_PLACEMENT_3D ( 'NONE', #100957, #40513, #74691 ) ;
#19246=CARTESIAN_POINT ( 'NONE',  ( 40.26004082231700210, 1457.179229772390045, 269.7776957246979919 ) ) ;
#19248=CARTESIAN_POINT ( 'NONE',  ( 2.478372249629999580, 1438.462791060409927, 157.7210847686980060 ) ) ;
#19249=CARTESIAN_POINT ( 'NONE',  ( -28.03239352689999819, 1444.711964596309826, 137.4439080254979899 ) ) ;
#19251=CARTESIAN_POINT ( 'NONE',  ( -39.40535375317039524, 1440.913060398519974, 258.4323147971229560 ) ) ;
#19252=CARTESIAN_POINT ( 'NONE',  ( 36.67521471636259633, 1449.719261606250029, 136.2722729094319902 ) ) ;
#19258=ADVANCED_FACE ( 'NONE', ( #71644 ), #10165, .T. ) ;
#19262=CARTESIAN_POINT ( 'NONE',  ( -3.813082683120000433E-15, 1426.500992774829911, 146.0666368882980066 ) ) ;
#19264=CARTESIAN_POINT ( 'NONE',  ( -1.290300528639490629, 1450.731663515321770, 181.8236001353477036 ) ) ;
#19266=CARTESIAN_POINT ( 'NONE',  ( -1.334703446960000095, 1476.095835883030077, 267.8533186384979672 ) ) ;
#19269=LINE ( 'NONE', #70847, #44144 ) ;
#19270=CARTESIAN_POINT ( 'NONE',  ( -3.841073510662149637, 1448.295370182304396, 185.0282369137797218 ) ) ;
#19272=CARTESIAN_POINT ( 'NONE',  ( -18.06884258770000073, 1415.263254653229978, 207.6880149420679800 ) ) ;
#19274=CARTESIAN_POINT ( 'NONE',  ( 26.16433611993790009, 1436.692690809629994, 136.8774806592069808 ) ) ;
#19276=CARTESIAN_POINT ( 'NONE',  ( -10.63692245770969969, 1396.284509905209916, 206.0546994452240028 ) ) ;
#19279=CARTESIAN_POINT ( 'NONE',  ( -17.06997858521869915, 1410.142247367640039, 225.8741214327440048 ) ) ;
#19286=CARTESIAN_POINT ( 'NONE',  ( 10.71319734329999918, 1425.353252437830179, 115.7252223364979926 ) ) ;
#19290=CARTESIAN_POINT ( 'NONE',  ( 4.303869558802829509, 1423.888414498320117, 183.7752672280500121 ) ) ;
#19291=VECTOR ( 'NONE', #20810, 1000.000000000000000 ) ;
#19296=FACE_OUTER_BOUND ( 'NONE', #60235, .T. ) ;
#19297=CARTESIAN_POINT ( 'NONE',  ( 2.594674246779999915, 1449.291015053200226, 183.0785327561979727 ) ) ;
#19298=EDGE_CURVE ( 'NONE', #56404, #12156, #74374, .T. ) ;
#19301=ORIENTED_EDGE ( 'NONE', *, *, #81620, .T. ) ;
#19303=CARTESIAN_POINT ( 'NONE',  ( -12.65017221549999960, 1441.023539904969994, 188.0792847196979949 ) ) ;
#19304=CARTESIAN_POINT ( 'NONE',  ( -0.3160898611105850131, 1482.866385869289843, 236.2848248989660078 ) ) ;
#19305=CARTESIAN_POINT ( 'NONE',  ( -2.316392100889999917, 1473.548945576829965, 270.3918176930980053 ) ) ;
#19310=CARTESIAN_POINT ( 'NONE',  ( 12.34231650081810194, 1419.113258958060214, 223.6504151099339879 ) ) ;
#19312=CARTESIAN_POINT ( 'NONE',  ( 35.14729760223570310, 1435.724875811340098, 135.0317109007289957 ) ) ;
#19313=CARTESIAN_POINT ( 'NONE',  ( 6.451603462551370072, 1396.138355344729916, 218.0852709918889900 ) ) ;
#19314=CARTESIAN_POINT ( 'NONE',  ( 14.94931177939999856, 1409.376221040630071, 212.2047251789079780 ) ) ;
#19315=CARTESIAN_POINT ( 'NONE',  ( -0.7754702341989130332, 1405.749502388330029, 267.5370916581230176 ) ) ;
#19316=CARTESIAN_POINT ( 'NONE',  ( 41.49088685270000099, 1443.869556898650217, 136.5795280473980142 ) ) ;
#19318=CARTESIAN_POINT ( 'NONE',  ( -10.96966797059999799, 1432.360037085170234, 151.7701368415980028 ) ) ;
#19319=CARTESIAN_POINT ( 'NONE',  ( 12.93995891640000018, 1441.798025058569920, 188.7551818563979964 ) ) ;
#19321=AXIS2_PLACEMENT_3D ( 'NONE', #48039, #82179, #73242 ) ;
#19329=ORIENTED_EDGE ( 'NONE', *, *, #104250, .T. ) ;
#19339=B_SPLINE_CURVE_WITH_KNOTS ( 'NONE', 3,
 ( #34048, #93396, #8832, #16661, #35706, #9405, #68787, #27307, #102887, #67678 ),
 .UNSPECIFIED., .F., .F.,
 ( 4, 2, 2, 2, 4 ),
 ( 2.159480829822040206E-09, 0.05040947966427840321, 0.1104028076245519990, 0.1513866672460139895, 0.2227566989315760138 ),
 .UNSPECIFIED. ) ;
#19340=CARTESIAN_POINT ( 'NONE',  ( -11.42986879550000090, 1410.682064136229883, 228.8161090984979751 ) ) ;
#19341=CARTESIAN_POINT ( 'NONE',  ( -4.084527001869999729, 1446.441115836090148, 184.0652579870979935 ) ) ;
#19342=ORIENTED_EDGE ( 'NONE', *, *, #7012, .F. ) ;
#19343=CARTESIAN_POINT ( 'NONE',  ( -13.80541478530910027, 1434.979604282769969, 148.5370187744020143 ) ) ;
#19344=CARTESIAN_POINT ( 'NONE',  ( 10.73506988043325627, 1424.972993549859893, 139.1354236083641922 ) ) ;
#19346=CARTESIAN_POINT ( 'NONE',  ( 16.77792727996295596, 1423.636664231082932, 228.4337725396501355 ) ) ;
#19348=CARTESIAN_POINT ( 'NONE',  ( -25.74205574149999975, 1436.650732699449918, 137.0790728707980008 ) ) ;
#19352=CARTESIAN_POINT ( 'NONE',  ( 0.01485783991055205852, 1507.825067223495580, 237.5163643644461899 ) ) ;
#19354=CARTESIAN_POINT ( 'NONE',  ( 19.84840157878679534, 1410.966943121492704, 197.0192273420008178 ) ) ;
#19356=ORIENTED_EDGE ( 'NONE', *, *, #13091, .T. ) ;
#19357=CARTESIAN_POINT ( 'NONE',  ( 2.500000000000000000, 1437.040203032260024, 157.6453869839979802 ) ) ;
#19358=CARTESIAN_POINT ( 'NONE',  ( -1.898512081650000072, 1415.378575369830060, 233.0498031619979997 ) ) ;
#19364=CARTESIAN_POINT ( 'NONE',  ( 17.55481076435209786, 1469.009107921980103, 228.8208540407819669 ) ) ;
#19365=CARTESIAN_POINT ( 'NONE',  ( -24.92784963018079836, 1509.784682262980141, 224.7537335476830265 ) ) ;
#19369=CARTESIAN_POINT ( 'NONE',  ( 0.1432641814004909919, 1420.464960711380172, 182.7250166793000119 ) ) ;
#19371=CARTESIAN_POINT ( 'NONE',  ( -4.117405581809999937, 1420.599289921329955, 186.3488710820979861 ) ) ;
#19372=CARTESIAN_POINT ( 'NONE',  ( 19.26331593919999818, 1508.281539294829827, 188.5704572384980224 ) ) ;
#19373=CARTESIAN_POINT ( 'NONE',  ( 7.000000000000000000, 1418.913060387330006, 172.2701767054979882 ) ) ;
#19374=ORIENTED_EDGE ( 'NONE', *, *, #86306, .F. ) ;
#19375=CARTESIAN_POINT ( 'NONE',  ( -11.74432248202560025, 1415.089118586289942, 196.5522872353360242 ) ) ;
#19376=CARTESIAN_POINT ( 'NONE',  ( -6.106019680640000225, 1485.913060386929828, 181.8019572232980181 ) ) ;
#19378=CARTESIAN_POINT ( 'NONE',  ( 4.071927273580000062, 1420.049653579930009, 185.6171871639980111 ) ) ;
#19380=CARTESIAN_POINT ( 'NONE',  ( 9.978198430534376939, 1435.712339636959996, 152.5066790191562518 ) ) ;
#19385=CARTESIAN_POINT ( 'NONE',  ( -3.701619934510000043, 1446.913858801710148, 156.0868339982980046 ) ) ;
#19386=FACE_OUTER_BOUND ( 'NONE', #69178, .T. ) ;
#19388=CARTESIAN_POINT ( 'NONE',  ( -17.44469085659999763, 1435.922852757180181, 147.7537887305979893 ) ) ;
#19389=CARTESIAN_POINT ( 'NONE',  ( 33.93392841120000014, 1451.575795592029863, 135.5855060888980006 ) ) ;
#19390=CARTESIAN_POINT ( 'NONE',  ( 16.09124803980000351, 1410.842148622430159, 191.5172216204979918 ) ) ;
#19393=CARTESIAN_POINT ( 'NONE',  ( 10.86679789090769965, 1425.928602444132594, 148.0726311711557628 ) ) ;
#19395=CARTESIAN_POINT ( 'NONE',  ( 0.8261703649055629484, 1507.439225835989873, 186.3102742836619825 ) ) ;
#19396=CARTESIAN_POINT ( 'NONE',  ( 23.44331756030000236, 1430.465020642029913, 206.4626199018280204 ) ) ;
#19397=EDGE_CURVE ( 'NONE', #22237, #35341, #56200, .T. ) ;
#19398=CARTESIAN_POINT ( 'NONE',  ( -23.66389183400000107, 1436.227554635920114, 212.2198923620080109 ) ) ;
#19401=CARTESIAN_POINT ( 'NONE',  ( -18.51267907639999777, 1508.236097876829945, 229.7333076606979887 ) ) ;
#19405=CARTESIAN_POINT ( 'NONE',  ( -18.94135955378079572, 1509.705011416190018, 185.2601256149999926 ) ) ;
#19406=VECTOR ( 'NONE', #44843, 1000.000000000000227 ) ;
#19408=EDGE_CURVE ( 'NONE', #69834, #10158, #24258, .T. ) ;
#19416=DIRECTION ( 'NONE',  ( 0.000000000000000000, 0.000000000000000000, -1.000000000000000000 ) ) ;
#19418=CARTESIAN_POINT ( 'NONE',  ( -17.75078229062794222, 1460.106445376706233, 228.1476975191470444 ) ) ;
#19421=EDGE_LOOP ( 'NONE', ( #67561, #45683, #51082, #21617 ) ) ;
#19422=VERTEX_POINT ( 'NONE', #68052 ) ;
#19423=CARTESIAN_POINT ( 'NONE',  ( 17.36569701797450094, 1415.089948427370018, 209.9483774915429990 ) ) ;
#19424=CARTESIAN_POINT ( 'NONE',  ( 13.46763530789999841, 1509.145555155530019, 233.8319897144979791 ) ) ;
#19426=CARTESIAN_POINT ( 'NONE',  ( -24.09814616333339998, 1444.255785637029931, 212.5772553280679915 ) ) ;
#19427=CARTESIAN_POINT ( 'NONE',  ( -36.92073947260000466, 1453.101237517530080, 259.2254642747980142 ) ) ;
#19428=EDGE_CURVE ( 'NONE', #75409, #10270, #29621, .T. ) ;
#19430=CARTESIAN_POINT ( 'NONE',  ( -11.21270966080000164, 1433.906859537220043, 151.6012850642980254 ) ) ;
#19431=CARTESIAN_POINT ( 'NONE',  ( 26.61730932929999938, 1507.998999673229946, 204.1002567748479919 ) ) ;
#19432=LINE ( 'NONE', #69324, #67491 ) ;
#19434=CARTESIAN_POINT ( 'NONE',  ( 8.290629166600000488, 1409.704288481229923, 187.9461355818979769 ) ) ;
#19435=CARTESIAN_POINT ( 'NONE',  ( 4.234467102410000017, 1420.712403739130195, 185.6414432377980006 ) ) ;
#19436=CARTESIAN_POINT ( 'NONE',  ( -11.55343452480000010, 1436.871189028030130, 151.7006538029980049 ) ) ;
#19437=ADVANCED_FACE ( 'NONE', ( #22680 ), #108928, .T. ) ;
#19438=CARTESIAN_POINT ( 'NONE',  ( 9.548319690719999642, 1438.548742142269930, 152.9855552813980069 ) ) ;
#19443=CARTESIAN_POINT ( 'NONE',  ( -2.404122373123565914, 1426.711430350427463, 142.7750368341233695 ) ) ;
#19444=B_SPLINE_CURVE_WITH_KNOTS ( 'NONE', 5,
 ( #21039, #10458, #79330, #53594, #46303, #55242, #35656, #96117, #72060 ),
 .UNSPECIFIED., .F., .F.,
 ( 6, 3, 6 ),
 ( 0.000000000000000000, 0.5050532947658213923, 1.000000000000000000 ),
 .UNSPECIFIED. ) ;
#19446=CARTESIAN_POINT ( 'NONE',  ( -44.29556206470000035, 1444.183390959899953, 270.0939713427979996 ) ) ;
#19448=CARTESIAN_POINT ( 'NONE',  ( 17.37499703619999636, 1409.684548388429903, 222.9025586185979932 ) ) ;
#19451=CARTESIAN_POINT ( 'NONE',  ( 2.909553342395870157, 1409.594673830890088, 231.3464090763989986 ) ) ;
#19452=CARTESIAN_POINT ( 'NONE',  ( 1.272733413219999887, 1507.906795984730024, 237.1822243490979929 ) ) ;
#19453=CARTESIAN_POINT ( 'NONE',  ( -8.212003350069998930, 1417.874967654629927, 230.9629104793979764 ) ) ;
#19454=CARTESIAN_POINT ( 'NONE',  ( -1.268441606857695803, 1484.597036441479304, 182.2979883374861458 ) ) ;
#19456=CARTESIAN_POINT ( 'NONE',  ( -45.90003289832019817, 1437.099605401870122, 266.9804752891529915 ) ) ;
#19458=ORIENTED_EDGE ( 'NONE', *, *, #59272, .T. ) ;
#19459=CARTESIAN_POINT ( 'NONE',  ( 26.60254240749708643, 1435.426458660660273, 135.2844112663541694 ) ) ;
#19465=CARTESIAN_POINT ( 'NONE',  ( -5.779044620229999651, 1425.409882702530012, 186.4185359615979962 ) ) ;
#19470=DIRECTION ( 'NONE',  ( -1.000000000000000000, 0.000000000000000000, 0.000000000000000000 ) ) ;
#19478=CARTESIAN_POINT ( 'NONE',  ( -13.53287548934629925, 1409.390853263720146, 270.2591806110339689 ) ) ;
#19480=CARTESIAN_POINT ( 'NONE',  ( 3.564372338642340043, 1417.932634516880171, 233.5387638921010023 ) ) ;
#19483=VERTEX_POINT ( 'NONE', #50140 ) ;
#19485=CARTESIAN_POINT ( 'NONE',  ( 45.24071116116442681, 1445.446384637186156, 268.9857686712747977 ) ) ;
#19488=CARTESIAN_POINT ( 'NONE',  ( -0.02885268102940060156, 1409.146038359130216, 185.6769965299799878 ) ) ;
#19489=VECTOR ( 'NONE', #47385, 1000.000000000000000 ) ;
#19491=CARTESIAN_POINT ( 'NONE',  ( -21.91250632251765396, 1506.380977040318612, 210.8063876161204462 ) ) ;
#19492=CARTESIAN_POINT ( 'NONE',  ( -21.02025974500000061, 1430.787304677930024, 220.7233419882979888 ) ) ;
#19494=CARTESIAN_POINT ( 'NONE',  ( -0.0001236924928765489894, 1475.983344053139945, 267.2347465760000205 ) ) ;
#19498=ORIENTED_EDGE ( 'NONE', *, *, #91922, .T. ) ;
#19500=CARTESIAN_POINT ( 'NONE',  ( 1.505303296824910042, 1463.321697279820000, 183.0243996004219866 ) ) ;
#19501=ORIENTED_EDGE ( 'NONE', *, *, #21990, .F. ) ;
#19503=CARTESIAN_POINT ( 'NONE',  ( 24.12978840347330234, 1452.070425774049909, 136.4015957713419880 ) ) ;
#19504=CARTESIAN_POINT ( 'NONE',  ( 11.60004869885209899, 1425.673082948501360, 137.6482176788198615 ) ) ;
#19507=CARTESIAN_POINT ( 'NONE',  ( 17.23433708029999778, 1409.514896698529810, 194.1039298879979924 ) ) ;
#19509=CARTESIAN_POINT ( 'NONE',  ( 17.06941266450000327, 1409.674943318129863, 224.8086569787979840 ) ) ;
#19510=CARTESIAN_POINT ( 'NONE',  ( 1.383512846939999985, 1417.442430893029950, 235.2784810073979997 ) ) ;
#19512=CARTESIAN_POINT ( 'NONE',  ( 0.9375664774988570205, 1452.266183237480163, 183.3265372543810088 ) ) ;
#19516=CARTESIAN_POINT ( 'NONE',  ( 27.59078576489319801, 1447.301049566279971, 137.0121621487540153 ) ) ;
#19522=CARTESIAN_POINT ( 'NONE',  ( -37.24878679391060388, 1449.386611531670042, 136.3094430657310170 ) ) ;
#19524=CARTESIAN_POINT ( 'NONE',  ( -17.26713005039999871, 1453.798585005629775, 234.3916895853979838 ) ) ;
#19525=CARTESIAN_POINT ( 'NONE',  ( 32.87679566159992817, 1465.269378838331249, 266.5399014024979465 ) ) ;
#19527=EDGE_CURVE ( 'NONE', #79125, #108385, #80056, .T. ) ;
#19528=CARTESIAN_POINT ( 'NONE',  ( -19.86748946169999996, 1471.981010699629906, 269.5245921433980243 ) ) ;
#19529=CARTESIAN_POINT ( 'NONE',  ( 25.13768435607400065, 1440.913060398800098, 216.9184046046830190 ) ) ;
#19532=VERTEX_POINT ( 'NONE', #41717 ) ;
#19533=CYLINDRICAL_SURFACE ( 'NONE', #44817, 2.000000000000001776 ) ;
#19534=CARTESIAN_POINT ( 'NONE',  ( 21.31355172050000135, 1471.299568759730164, 210.6477759654979991 ) ) ;
#19535=CARTESIAN_POINT ( 'NONE',  ( -12.27011089310000003, 1486.375363512730246, 184.4446487454979717 ) ) ;
#19536=B_SPLINE_CURVE_WITH_KNOTS ( 'NONE', 3,
 ( #57045, #27277, #94462, #59793, #9921, #52498, #95037, #70421, #87758, #42985 ),
 .UNSPECIFIED., .F., .F.,
 ( 4, 2, 2, 2, 4 ),
 ( 0.000000000000000000, 0.2500000000000000000, 0.5000000000000000000, 0.7500000000000000000, 1.000000000000000000 ),
 .UNSPECIFIED. ) ;
#19537=CARTESIAN_POINT ( 'NONE',  ( 3.461063783934097859, 1398.015735858593189, 196.5635239469207249 ) ) ;
#19538=CARTESIAN_POINT ( 'NONE',  ( 1.726858845490000016, 1482.796399391929981, 235.4332745692979927 ) ) ;
#19540=CARTESIAN_POINT ( 'NONE',  ( 25.96988284260000057, 1469.243118069030061, 212.2965549575379782 ) ) ;
#19543=CARTESIAN_POINT ( 'NONE',  ( -17.74011923890000020, 1509.475909753130054, 231.2409737833980046 ) ) ;
#19546=CARTESIAN_POINT ( 'NONE',  ( 18.64618896912524448, 1416.835806650408813, 209.6841501312022160 ) ) ;
#19547=CARTESIAN_POINT ( 'NONE',  ( -28.15442856212169787, 1509.896234822020006, 200.8410265843269826 ) ) ;
#19551=CARTESIAN_POINT ( 'NONE',  ( -28.46619500829999794, 1445.052233488290085, 168.7181723459979992 ) ) ;
#19552=AXIS2_PLACEMENT_3D ( 'NONE', #15554, #58154, #92284 ) ;
#19554=CARTESIAN_POINT ( 'NONE',  ( -5.457743909444250363, 1440.715679462449998, 154.7912908061040014 ) ) ;
#19556=EDGE_LOOP ( 'NONE', ( #97666, #32705, #9030, #84849 ) ) ;
#19561=CARTESIAN_POINT ( 'NONE',  ( -8.311471914476035394, 1509.203303456682079, 237.2547473838516794 ) ) ;
#19562=DIRECTION ( 'NONE',  ( 0.9950083946325752882, 0.09971571435232254310, -0.003882128528443905269 ) ) ;
#19565=CARTESIAN_POINT ( 'NONE',  ( 12.02250444982000133, 1409.332895484829805, 218.0033144737150224 ) ) ;
#19566=CARTESIAN_POINT ( 'NONE',  ( 5.314807373273278124, 1420.217340012715113, 137.0999999980982125 ) ) ;
#19568=EDGE_CURVE ( 'NONE', #74353, #74738, #22852, .T. ) ;
#19570=CARTESIAN_POINT ( 'NONE',  ( -17.63667811080000192, 1430.609996739030066, 191.3996239150980045 ) ) ;
#19572=ORIENTED_EDGE ( 'NONE', *, *, #79699, .F. ) ;
#19579=CARTESIAN_POINT ( 'NONE',  ( -11.86597105770560034, 1415.542389211330146, 195.0589158601300142 ) ) ;
#19581=CARTESIAN_POINT ( 'NONE',  ( -11.52394156360000110, 1434.100698262960123, 151.3697489037979835 ) ) ;
#19582=CARTESIAN_POINT ( 'NONE',  ( 28.36448145873015036, 1509.903571177603226, 216.7772950919570292 ) ) ;
#19583=CARTESIAN_POINT ( 'NONE',  ( 5.077070885040000370, 1398.064298510030085, 221.1616505512979813 ) ) ;
#19586=CARTESIAN_POINT ( 'NONE',  ( -1.187216277370000128, 1457.285143779230111, 183.3846202966979888 ) ) ;
#19590=CARTESIAN_POINT ( 'NONE',  ( -12.99817078242380042, 1434.787734094880079, 149.3751819043959870 ) ) ;
#19591=B_SPLINE_SURFACE_WITH_KNOTS ( 'NONE', 5, 5, ( 
 ( #44955, #71834, #46606, #2410, #46055, #95881 ),
 ( #80740, #105953, #36527, #96439, #70723, #21345 ),
 ( #4048, #19717, #20809, #96999, #104835, #55007 ),
 ( #38175, #29771, #29231, #72355, #27573, #106486 ),
 ( #28122, #47142, #63960, #105391, #80188, #81268 ),
 ( #28682, #62315, #53920, #98075, #88055, #11339 ),
 ( #2958, #55551, #45512, #20262, #89677, #79653 ),
 ( #37075, #62889, #54462, #88600, #11883, #75107 ),
 ( #109255, #5689, #57211, #65602, #15692, #47690 ) ),
 .UNSPECIFIED., .F., .F., .F.,
 ( 6, 3, 6 ),
 ( 6, 6 ),
 ( 0.7655572723410000169, 2.316155491850000026, 3.835724788489999870 ),
 ( 0.000000000000000000, 1.000000000000000000 ),
 .UNSPECIFIED. ) ;
#19592=FACE_OUTER_BOUND ( 'NONE', #19632, .T. ) ;
#19596=ORIENTED_EDGE ( 'NONE', *, *, #63723, .F. ) ;
#19597=CARTESIAN_POINT ( 'NONE',  ( 14.25478695230000170, 1406.894174824430138, 267.1909361702979595 ) ) ;
#19598=CARTESIAN_POINT ( 'NONE',  ( -27.21299276520000276, 1488.689717875729912, 207.6915820717080123 ) ) ;
#19599=B_SPLINE_CURVE_WITH_KNOTS ( 'NONE', 5,
 ( #96194, #2164, #46784, #69359, #53104, #47310, #1051, #17792, #78854, #51992, #86133, #104033 ),
 .UNSPECIFIED., .F., .F.,
 ( 6, 3, 3, 6 ),
 ( 0.000000000000000000, 0.3237431521556269343, 0.7745810507185086902, 1.000000000000000000 ),
 .UNSPECIFIED. ) ;
#19600=CARTESIAN_POINT ( 'NONE',  ( -11.02774336400820054, 1426.509921592220053, 92.74671990447460246 ) ) ;
#19601=CARTESIAN_POINT ( 'NONE',  ( 3.378657952879999992E-14, 1414.110153932129833, 261.8343058782979824 ) ) ;
#19603=CARTESIAN_POINT ( 'NONE',  ( -21.36149126229999951, 1471.309244717429920, 207.7943419303680344 ) ) ;
#19605=CARTESIAN_POINT ( 'NONE',  ( -38.77640472460000609, 1433.500816082299934, 259.1404853845979801 ) ) ;
#19607=CARTESIAN_POINT ( 'NONE',  ( 29.75012120190000076, 1509.993914123429931, 209.6841247587719863 ) ) ;
#19608=CARTESIAN_POINT ( 'NONE',  ( 2.864408029580055803, 1447.807653760355834, 154.7916318795152506 ) ) ;
#19609=CARTESIAN_POINT ( 'NONE',  ( 33.14188703010000125, 1450.895165025899814, 136.1944683724980223 ) ) ;
#19611=CARTESIAN_POINT ( 'NONE',  ( -5.386577890436130112, 1432.378605031630059, 154.6079252277549756 ) ) ;
#19614=CARTESIAN_POINT ( 'NONE',  ( 38.48250450508500364, 1443.291876352919871, 137.1415221903349959 ) ) ;
#19615=VERTEX_POINT ( 'NONE', #70275 ) ;
#19620=CARTESIAN_POINT ( 'NONE',  ( -1.072088845450000161, 1412.065175156030136, 185.2438394658980201 ) ) ;
#19622=CARTESIAN_POINT ( 'NONE',  ( -11.87414320589479999, 1432.940728692309904, 149.9807111271900055 ) ) ;
#19623=CARTESIAN_POINT ( 'NONE',  ( -1.174483211909999936, 1470.486737867530110, 235.5973338944980071 ) ) ;
#19625=CARTESIAN_POINT ( 'NONE',  ( 46.27886946470769658, 1440.912966750240003, 267.5894436979959892 ) ) ;
#19627=CARTESIAN_POINT ( 'NONE',  ( 0.03533291443150000238, 1420.203121373229806, 183.8975548986979902 ) ) ;
#19628=VERTEX_POINT ( 'NONE', #85356 ) ;
#19629=( BOUNDED_CURVE ( )  B_SPLINE_CURVE ( 3, ( #88253, #45722, #3169, #63093 ),
 .UNSPECIFIED., .F., .F. ) 
 B_SPLINE_CURVE_WITH_KNOTS ( ( 4, 4 ),
 ( 4.245054931713185375, 5.179005799894629725 ),
 .UNSPECIFIED. ) 
 CURVE ( )  GEOMETRIC_REPRESENTATION_ITEM ( )  RATIONAL_B_SPLINE_CURVE ( ( 1.000000000000000000, 0.9286226616644226439, 0.9286226616644226439, 1.000000000000000000 ) ) 
 REPRESENTATION_ITEM ( '' )  );
#19632=EDGE_LOOP ( 'NONE', ( #96817, #50831, #31606, #8728 ) ) ;
#19633=CARTESIAN_POINT ( 'NONE',  ( 11.85901083361419950, 1431.841316764000112, 149.9599341808090003 ) ) ;
#19634=CARTESIAN_POINT ( 'NONE',  ( 12.78853242329685891, 1444.985736185042470, 186.5280363921234539 ) ) ;
#19638=DIRECTION ( 'NONE',  ( -1.000000000000000000, -5.823966869780000474E-19, 4.137698748469999823E-18 ) ) ;
#19640=CARTESIAN_POINT ( 'NONE',  ( 15.79557044279290068, 1452.361466912919923, 147.2817071249239973 ) ) ;
#19642=CARTESIAN_POINT ( 'NONE',  ( 2.339366202910509784, 1407.692004809400260, 270.1366117308560320 ) ) ;
#19645=CARTESIAN_POINT ( 'NONE',  ( 11.60004869885203682, 1422.222932908421853, 135.5999999980979851 ) ) ;
#19649=CARTESIAN_POINT ( 'NONE',  ( 14.35483055539999953, 1416.837177098629809, 196.6648191809980233 ) ) ;
#19651=CARTESIAN_POINT ( 'NONE',  ( 17.66473809693500030, 1412.789316240470043, 224.8635844683609832 ) ) ;
#19654=CARTESIAN_POINT ( 'NONE',  ( 32.79207797800000179, 1428.560640288129889, 262.6648722463980334 ) ) ;
#19662=EDGE_LOOP ( 'NONE', ( #37097, #66539, #66617, #16543, #9816, #104895, #107372 ) ) ;
#19664=CARTESIAN_POINT ( 'NONE',  ( -24.81337094160000234, 1443.616293363810200, 210.6361221007779818 ) ) ;
#19665=CARTESIAN_POINT ( 'NONE',  ( -1.843570366231615631, 1450.382637347590162, 154.3039494713565603 ) ) ;
#19668=CARTESIAN_POINT ( 'NONE',  ( -11.95688248459999947, 1441.464442770860160, 187.7513092272979804 ) ) ;
#19669=CARTESIAN_POINT ( 'NONE',  ( 6.436778620621919522, 1509.137837650079973, 179.8165091018489932 ) ) ;
#19671=CARTESIAN_POINT ( 'NONE',  ( 12.20256845149948610, 1434.091510794637998, 149.6914622690949273 ) ) ;
#19672=CARTESIAN_POINT ( 'NONE',  ( 11.80820258149999979, 1417.418794541129955, 229.4144358672980104 ) ) ;
#19674=CARTESIAN_POINT ( 'NONE',  ( -16.91862346270000117, 1461.030957408330096, 228.2759457765980073 ) ) ;
#19677=CARTESIAN_POINT ( 'NONE',  ( 45.48702313900000149, 1436.948642006169848, 266.1936685609980486 ) ) ;
#19678=CARTESIAN_POINT ( 'NONE',  ( -18.49972780619999924, 1410.921726043829949, 223.9058259105980255 ) ) ;
#19680=CARTESIAN_POINT ( 'NONE',  ( 18.04150427010000257, 1436.361837209869918, 147.3508937178980034 ) ) ;
#19681=CARTESIAN_POINT ( 'NONE',  ( 26.64435021830000139, 1508.005964801830032, 204.3334252420080190 ) ) ;
#19682=CARTESIAN_POINT ( 'NONE',  ( 5.374504625227119803, 1429.015749531610027, 154.0247573729420196 ) ) ;
#19685=FACE_OUTER_BOUND ( 'NONE', #30382, .T. ) ;
#19687=CARTESIAN_POINT ( 'NONE',  ( -38.35651281120340172, 1437.646912403469969, 136.3196577860490208 ) ) ;
#19688=DIRECTION ( 'NONE',  ( -0.001339522651315419892, 0.9999644786255611484, 0.008321488218843280452 ) ) ;
#19689=CARTESIAN_POINT ( 'NONE',  ( -18.18905553120000107, 1416.520322350429979, 205.1726131530880082 ) ) ;
#19691=CARTESIAN_POINT ( 'NONE',  ( -11.98663175510000123, 1441.172953348979945, 187.7782422411980008 ) ) ;
#19694=CARTESIAN_POINT ( 'NONE',  ( -33.93529342339999744, 1435.841716433050124, 135.9421945811979811 ) ) ;
#19695=CARTESIAN_POINT ( 'NONE',  ( 21.02608924029999926, 1456.853724928630072, 225.6706377209980303 ) ) ;
#19698=CARTESIAN_POINT ( 'NONE',  ( -6.394947566795919691, 1409.136376877240082, 222.6614285949029863 ) ) ;
#19702=CARTESIAN_POINT ( 'NONE',  ( -45.88374573399999434, 1446.003351892490173, 266.4124074795980164 ) ) ;
#19703=CARTESIAN_POINT ( 'NONE',  ( -13.08223627748380125, 1428.818921846599778, 222.3767532333990005 ) ) ;
#19709=CARTESIAN_POINT ( 'NONE',  ( 16.04707966210000336, 1416.518532928429977, 217.6280249965379880 ) ) ;
#19710=CARTESIAN_POINT ( 'NONE',  ( -11.86590139589999815, 1432.348266868109931, 151.0567667964980103 ) ) ;
#19711=CARTESIAN_POINT ( 'NONE',  ( -2.253566441613126910E-10, 1426.918876941764893, 137.0999999980980135 ) ) ;
#19714=CARTESIAN_POINT ( 'NONE',  ( 5.327762952207462099, 1422.321577162126232, 138.7600416031628754 ) ) ;
#19716=CARTESIAN_POINT ( 'NONE',  ( 15.32781700640000011, 1414.971279908829956, 201.8289935246679931 ) ) ;
#19717=CARTESIAN_POINT ( 'NONE',  ( -12.39598156289999942, 1416.274718424630009, 194.8162290544979953 ) ) ;
#19719=CARTESIAN_POINT ( 'NONE',  ( 0.1559730049430000098, 1467.142443652729980, 235.6419144452979992 ) ) ;
#19720=CARTESIAN_POINT ( 'NONE',  ( 23.52564803090000112, 1410.656144928030244, 211.7451932072379748 ) ) ;
#19721=B_SPLINE_SURFACE_WITH_KNOTS ( 'NONE', 4, 5, ( 
 ( #75765, #15277, #57336, #83591, #109913, #64629 ),
 ( #98749, #65169, #6890, #22559, #14184, #91462 ),
 ( #41046, #14740, #76311, #25882, #86914, #18582 ),
 ( #52777, #43816, #18038, #101481, #86359, #67934 ),
 ( #110462, #27016, #93635, #61206, #102584, #94762 ) ),
 .UNSPECIFIED., .F., .F., .F.,
 ( 5, 5 ),
 ( 6, 6 ),
 ( 30.35883180189999919, 49.62971790979390363 ),
 ( -0.001138638393163039862, 2.001138639208579928 ),
 .UNSPECIFIED. ) ;
#19722=CARTESIAN_POINT ( 'NONE',  ( -12.07610166159999920, 1433.870589910030048, 149.7869025145980117 ) ) ;
#19725=CARTESIAN_POINT ( 'NONE',  ( -11.86735416189999803, 1432.439689909539993, 150.3969688813980099 ) ) ;
#19727=CARTESIAN_POINT ( 'NONE',  ( -0.1180586146000000003, 1410.296227586130044, 233.2638028148980140 ) ) ;
#19729=AXIS2_PLACEMENT_3D ( 'NONE', #15709, #109269, #23586 ) ;
#19734=CARTESIAN_POINT ( 'NONE',  ( -19.98479248519999985, 1427.060832424730052, 224.6412401930980138 ) ) ;
#19735=CARTESIAN_POINT ( 'NONE',  ( -18.69214414528729762, 1485.716420687259870, 189.3114983721589795 ) ) ;
#19746=CARTESIAN_POINT ( 'NONE',  ( -15.72888735940112070, 1409.636818260307336, 226.0013290851642580 ) ) ;
#19747=CARTESIAN_POINT ( 'NONE',  ( 13.89716773895519886, 1452.853908481549979, 223.9136441993209985 ) ) ;
#19749=CARTESIAN_POINT ( 'NONE',  ( -24.89146661867219734, 1451.594294999959857, 137.4462232438879994 ) ) ;
#19751=CARTESIAN_POINT ( 'NONE',  ( 9.199108954039999730, 1410.609401603230026, 230.1463904532980109 ) ) ;
#19752=( LENGTH_UNIT ( ) NAMED_UNIT ( * ) SI_UNIT ( .MILLI., .METRE. ) );
#19754=CARTESIAN_POINT ( 'NONE',  ( 41.66188030070000536, 1443.705283505699754, 134.0999999982089719 ) ) ;
#19756=CARTESIAN_POINT ( 'NONE',  ( 9828.720208560080209, 54.28084071072819938, -1083.674256113199817 ) ) ;
#19757=VERTEX_POINT ( 'NONE', #15199 ) ;
#19758=CARTESIAN_POINT ( 'NONE',  ( 14.48646706370279880, 1435.954295751229893, 149.8410885043270184 ) ) ;
#19760=ORIENTED_EDGE ( 'NONE', *, *, #55052, .T. ) ;
#19761=ORIENTED_EDGE ( 'NONE', *, *, #60018, .F. ) ;
#19762=ORIENTED_EDGE ( 'NONE', *, *, #2284, .T. ) ;
#19764=CARTESIAN_POINT ( 'NONE',  ( -0.7051069384629999881, 1465.998960783829943, 235.7578936505979925 ) ) ;
#19766=CARTESIAN_POINT ( 'NONE',  ( 21.25084690298298895, 1450.939921383146611, 144.1607677896775783 ) ) ;
#19769=CARTESIAN_POINT ( 'NONE',  ( -17.47882303318302277, 1448.297325624284440, 218.1748229397720706 ) ) ;
#19770=CARTESIAN_POINT ( 'NONE',  ( 13.30361758462239941, 1409.377634028029888, 191.9462312207510308 ) ) ;
#19772=CARTESIAN_POINT ( 'NONE',  ( 0.3083299013670000033, 1507.389591484829907, 237.3685675047980226 ) ) ;
#19775=VERTEX_POINT ( 'NONE', #66759 ) ;
#19776=CARTESIAN_POINT ( 'NONE',  ( 25.13830754042900040, 1440.913060387330006, 239.5563470660360110 ) ) ;
#19779=ORIENTED_EDGE ( 'NONE', *, *, #20513, .F. ) ;
#19780=CARTESIAN_POINT ( 'NONE',  ( 25.74039302815520003, 1448.986371477839839, 137.5027126072619978 ) ) ;
#19781=CARTESIAN_POINT ( 'NONE',  ( -13.86209743629999913, 1409.397135496529927, 191.7555771504979987 ) ) ;
#19783=CARTESIAN_POINT ( 'NONE',  ( -24.41225618889999893, 1441.001746037479961, 212.0330686186080129 ) ) ;
#19785=CARTESIAN_POINT ( 'NONE',  ( -2.370970874524632510, 1427.002265528473799, 134.0999999980979851 ) ) ;
#19787=CARTESIAN_POINT ( 'NONE',  ( -12.02581300470458459, 1433.744446891241296, 147.5729342865741955 ) ) ;
#19788=CARTESIAN_POINT ( 'NONE',  ( -13.80542637100000114, 1434.979599513729909, 148.5642174889979970 ) ) ;
#19790=CARTESIAN_POINT ( 'NONE',  ( 9.952255756299999589, 1464.084013546329970, 232.4863585809980009 ) ) ;
#19795=CARTESIAN_POINT ( 'NONE',  ( 29.03008455810000044, 1509.878129441930014, 207.4556142791579987 ) ) ;
#19800=EDGE_LOOP ( 'NONE', ( #33268, #50720, #16616, #22231 ) ) ;
#19801=DIRECTION ( 'NONE',  ( 0.000000000000000000, 0.000000000000000000, -1.000000000000000000 ) ) ;
#19802=CARTESIAN_POINT ( 'NONE',  ( 21.00608537309999946, 1461.014378765330093, 244.4374624723980105 ) ) ;
#19805=CARTESIAN_POINT ( 'NONE',  ( 2.922318616430000127, 1413.151494948330082, 231.7542961375979758 ) ) ;
#19806=CARTESIAN_POINT ( 'NONE',  ( -19.13038500899999761, 1456.668630468730044, 226.8508188085980066 ) ) ;
#19807=CARTESIAN_POINT ( 'NONE',  ( -23.50967715347146125, 1411.094363712649283, 206.3755992539118438 ) ) ;
#19808=CARTESIAN_POINT ( 'NONE',  ( 2.500000000000000000, 1427.007219668030075, 156.3926178584979994 ) ) ;
#19811=EDGE_LOOP ( 'NONE', ( #58670, #36134, #91787, #94910 ) ) ;
#19813=CARTESIAN_POINT ( 'NONE',  ( 0.8788299526799999706, 1406.512806268830218, 269.4984184344980349 ) ) ;
#19815=CARTESIAN_POINT ( 'NONE',  ( 19.56475689569279908, 1470.874168187639725, 270.3418681666850034 ) ) ;
#19817=CARTESIAN_POINT ( 'NONE',  ( 5.500900010980000587, 1439.900099495260065, 154.7565255832979858 ) ) ;
#19819=CARTESIAN_POINT ( 'NONE',  ( -42.50114641298220164, 1440.913060410849994, 262.5787053766010217 ) ) ;
#19820=CARTESIAN_POINT ( 'NONE',  ( -27.28014783120000075, 1449.116319034829985, 136.7094420238979922 ) ) ;
#19827=ORIENTED_EDGE ( 'NONE', *, *, #74664, .F. ) ;
#19828=CARTESIAN_POINT ( 'NONE',  ( -40.73184307449999864, 1440.913060387330006, 268.3665355201979992 ) ) ;
#19832=CARTESIAN_POINT ( 'NONE',  ( -0.3381555172680000276, 1475.759016768630090, 269.0456609237979819 ) ) ;
#19833=CARTESIAN_POINT ( 'NONE',  ( -29.29916111349999852, 1451.889927077430229, 134.8511816846980196 ) ) ;
#19834=CARTESIAN_POINT ( 'NONE',  ( -29.22958589629999793, 1509.933780018729749, 211.7723606568879688 ) ) ;
#19835=CARTESIAN_POINT ( 'NONE',  ( -3.029999059705268394, 1448.271449514276583, 184.4966768164291864 ) ) ;
#19838=CARTESIAN_POINT ( 'NONE',  ( -17.97556616420000353, 1415.263254644529979, 208.0573017206880024 ) ) ;
#19840=CARTESIAN_POINT ( 'NONE',  ( 26.44714126616960215, 1435.441704364029874, 135.5654590955990102 ) ) ;
#19841=CARTESIAN_POINT ( 'NONE',  ( -3.345866853802129892, 1396.029900632619956, 219.6261091127090310 ) ) ;
#19842=AXIS2_PLACEMENT_3D ( 'NONE', #35258, #26862, #78371 ) ;
#19843=CARTESIAN_POINT ( 'NONE',  ( -14.79386498719999921, 1422.246529131229863, 228.4005900637979778 ) ) ;
#19844=CARTESIAN_POINT ( 'NONE',  ( -16.75463603240659793, 1409.872673125029905, 225.8937886272380240 ) ) ;
#19845=CARTESIAN_POINT ( 'NONE',  ( 22.39540279318442373, 1509.695125022787124, 227.2040457527074011 ) ) ;
#19848=CARTESIAN_POINT ( 'NONE',  ( 1.881594583719999880, 1409.481719934030025, 231.8401253045980184 ) ) ;
#19849=CARTESIAN_POINT ( 'NONE',  ( -11.84242364297029937, 1431.324255904990196, 147.6543138676789795 ) ) ;
#19850=CARTESIAN_POINT ( 'NONE',  ( 11.48762818220000170, 1426.845523664929942, 126.2888625367979927 ) ) ;
#19854=B_SPLINE_CURVE_WITH_KNOTS ( 'NONE', 5,
 ( #47291, #97141, #88197, #80346, #87649, #12031, #55164, #63571, #81414, #4726, #38870, #45111 ),
 .UNSPECIFIED., .F., .F.,
 ( 6, 3, 3, 6 ),
 ( 0.000000000000000000, 0.4310012308516226187, 0.8100023263410623953, 1.000000000000000000 ),
 .UNSPECIFIED. ) ;
#19857=FACE_OUTER_BOUND ( 'NONE', #25186, .T. ) ;
#19858=CARTESIAN_POINT ( 'NONE',  ( 4.080976423390000107, 1507.461518311630016, 181.6612281710979744 ) ) ;
#19864=ORIENTED_EDGE ( 'NONE', *, *, #6520, .T. ) ;
#19865=CARTESIAN_POINT ( 'NONE',  ( -41.65810620650000828, 1443.954352776429914, 135.6863023723980177 ) ) ;
#19866=CARTESIAN_POINT ( 'NONE',  ( 0.8514805750585270339, 1499.044650913519945, 236.8919523093149735 ) ) ;
#19867=CARTESIAN_POINT ( 'NONE',  ( 7.326859461719999800, 1453.313060387329870, 227.7771414719979930 ) ) ;
#19870=CARTESIAN_POINT ( 'NONE',  ( -2.773580850399999687, 1486.025199416829764, 182.0239507221979807 ) ) ;
#19872=CARTESIAN_POINT ( 'NONE',  ( -35.15123143180689880, 1451.685553933709798, 134.6826492062959915 ) ) ;
#19873=CARTESIAN_POINT ( 'NONE',  ( -2.500000000000000000, 1448.396495418279983, 162.2933047224009897 ) ) ;
#19874=CARTESIAN_POINT ( 'NONE',  ( 8.910237381932139655, 1396.224212735589845, 215.6676506388549797 ) ) ;
#19875=CARTESIAN_POINT ( 'NONE',  ( 6.242063231577089866, 1407.474368659629818, 197.0547293822570225 ) ) ;
#19876=CARTESIAN_POINT ( 'NONE',  ( -2.304782706912239743, 1405.786085933429831, 267.5351694450670266 ) ) ;
#19879=CARTESIAN_POINT ( 'NONE',  ( -11.30106291509999927, 1432.291791638479936, 151.5220416229979890 ) ) ;
#19880=CARTESIAN_POINT ( 'NONE',  ( 12.56537301320000033, 1441.599614738780019, 188.5161398251980245 ) ) ;
#19894=CARTESIAN_POINT ( 'NONE',  ( 11.30589650210000130, 1414.913060387329779, 221.8290180415980046 ) ) ;
#19896=CARTESIAN_POINT ( 'NONE',  ( -19.08445480129999794, 1440.913060387330006, 209.8212738029720299 ) ) ;
#19898=CARTESIAN_POINT ( 'NONE',  ( 11.58906603030466620, 1433.009685293574421, 151.1019960182966031 ) ) ;
#19900=FACE_OUTER_BOUND ( 'NONE', #89504, .T. ) ;
#19901=CARTESIAN_POINT ( 'NONE',  ( -8.350981080969999581, 1410.576960734530076, 230.4971537514980184 ) ) ;
#19902=CARTESIAN_POINT ( 'NONE',  ( -4.115442145179999400, 1447.984267398149996, 185.1172023007979988 ) ) ;
#19904=CARTESIAN_POINT ( 'NONE',  ( 5.731937518187070424, 1432.353341358199941, 149.9895731140795760 ) ) ;
#19905=CARTESIAN_POINT ( 'NONE',  ( -25.74005402952169774, 1440.913060490129965, 220.4485507050690103 ) ) ;
#19909=CARTESIAN_POINT ( 'NONE',  ( 41.30101714413999048, 1432.598592530589940, 269.8654501280279874 ) ) ;
#19912=CARTESIAN_POINT ( 'NONE',  ( 0.01069039238330171844, 1508.209830008338031, 237.7339634020152914 ) ) ;
#19914=CARTESIAN_POINT ( 'NONE',  ( 19.65563895711393982, 1410.960466841314201, 196.5957095808309703 ) ) ;
#19917=CARTESIAN_POINT ( 'NONE',  ( 8.991744574390811096, 1509.227061438039982, 181.2342617849590169 ) ) ;
#19918=CARTESIAN_POINT ( 'NONE',  ( -0.7927729341670000096, 1417.918636335230076, 233.4281342940980153 ) ) ;
#19921=VERTEX_POINT ( 'NONE', #106182 ) ;
#19924=CARTESIAN_POINT ( 'NONE',  ( 18.89959501459999913, 1416.839692131129823, 210.6687137086479993 ) ) ;
#19925=CARTESIAN_POINT ( 'NONE',  ( 6.264020380922289633, 1478.700514275750038, 234.1616571566459868 ) ) ;
#19926=EDGE_CURVE ( 'NONE', #89812, #68458, #7987, .T. ) ;
#19928=CARTESIAN_POINT ( 'NONE',  ( -20.17493600595490122, 1508.361572245040179, 228.9114206119960215 ) ) ;
#19929=CARTESIAN_POINT ( 'NONE',  ( -24.89939545272470056, 1440.978110083920001, 210.4300214511639808 ) ) ;
#19935=CARTESIAN_POINT ( 'NONE',  ( 19.01903744140000185, 1509.560719669929995, 186.9589011645979895 ) ) ;
#19939=LINE ( 'NONE', #53020, #105270 ) ;
#19942=CARTESIAN_POINT ( 'NONE',  ( 0.08972463244040000674, 1506.809279360230221, 231.1592509372979976 ) ) ;
#19943=( BOUNDED_CURVE ( )  B_SPLINE_CURVE ( 3, ( #59787, #9369, #2099, #51364 ),
 .UNSPECIFIED., .F., .F. ) 
 B_SPLINE_CURVE_WITH_KNOTS ( ( 4, 4 ),
 ( 3.148814872228629991, 3.786951980637359938 ),
 .UNSPECIFIED. ) 
 CURVE ( )  GEOMETRIC_REPRESENTATION_ITEM ( )  RATIONAL_B_SPLINE_CURVE ( ( 1.000000000000000000, 0.9663520053108367591, 0.9663520053108367591, 1.000000000000000000 ) ) 
 REPRESENTATION_ITEM ( '' )  );
#19946=UNCERTAINTY_MEASURE_WITH_UNIT (LENGTH_MEASURE( 1.000000000000000082E-05 ), #22879, 'distance_accuracy_value', 'NONE');
#19950=CARTESIAN_POINT ( 'NONE',  ( 18.26532265589999682, 1415.628674266529742, 209.8910850646770143 ) ) ;
#19951=CARTESIAN_POINT ( 'NONE',  ( -18.66276826640000053, 1424.482644047330041, 224.7741685936979934 ) ) ;
#19952=CARTESIAN_POINT ( 'NONE',  ( -14.94677667230000040, 1435.443163586859782, 149.2760775765979986 ) ) ;
#19954=CARTESIAN_POINT ( 'NONE',  ( 16.94262738639999810, 1413.517289013830123, 191.7422180533980054 ) ) ;
#19955=CARTESIAN_POINT ( 'NONE',  ( 0.8067250493409530154, 1409.444751007370314, 232.8393309433039917 ) ) ;
#19956=CARTESIAN_POINT ( 'NONE',  ( -12.18907324829999972, 1509.462877414930063, 181.5959492063950051 ) ) ;
#19959=CARTESIAN_POINT ( 'NONE',  ( 1.554318670623859866, 1415.441076448390049, 190.8942697646920124 ) ) ;
#19960=CARTESIAN_POINT ( 'NONE',  ( 27.59579075839436868, 1509.876726636794046, 217.1913360364012817 ) ) ;
#19961=CARTESIAN_POINT ( 'NONE',  ( -23.98687813229999932, 1436.754506703620109, 211.2894088040379756 ) ) ;
#19965=CARTESIAN_POINT ( 'NONE',  ( 11.38620825595340946, 1434.628468754609457, 151.4994770517398308 ) ) ;
#19968=CARTESIAN_POINT ( 'NONE',  ( -22.37852245395630035, 1509.694535611759875, 189.1625215705749952 ) ) ;
#19976=CARTESIAN_POINT ( 'NONE',  ( 21.00523825079999796, 1507.839072599329711, 190.5229776796980161 ) ) ;
#19979=CARTESIAN_POINT ( 'NONE',  ( 20.59987592950000135, 1509.677367935830262, 230.5839143914980127 ) ) ;
#19981=ORIENTED_EDGE ( 'NONE', *, *, #53056, .T. ) ;
#19983=CARTESIAN_POINT ( 'NONE',  ( 13.36714629989999814, 1508.095002141429859, 233.0794843863980077 ) ) ;
#19984=CARTESIAN_POINT ( 'NONE',  ( 12.53380499174499896, 1442.773887286369927, 169.4755105688890069 ) ) ;
#19985=CARTESIAN_POINT ( 'NONE',  ( 38.89760815976732289, 1429.358032043940739, 269.5912097956908724 ) ) ;
#19986=CARTESIAN_POINT ( 'NONE',  ( -28.68962070750000137, 1467.163296334329971, 264.4914082303979512 ) ) ;
#19988=CARTESIAN_POINT ( 'NONE',  ( -11.93097190810000008, 1433.475858514520041, 150.1043676198979995 ) ) ;
#19991=FACE_OUTER_BOUND ( 'NONE', #13561, .T. ) ;
#19992=CARTESIAN_POINT ( 'NONE',  ( -19.08494480400000270, 1485.680871126130114, 189.6157807285979970 ) ) ;
#19993=CARTESIAN_POINT ( 'NONE',  ( 9.483367929919999995, 1409.244226892830056, 189.9488811312979806 ) ) ;
#19995=CARTESIAN_POINT ( 'NONE',  ( 5.213606989689999693, 1421.909598794630028, 185.7541303422979979 ) ) ;
#19996=CARTESIAN_POINT ( 'NONE',  ( -6.267127244280000120, 1440.453902086580001, 154.5142011235980135 ) ) ;
#19998=CARTESIAN_POINT ( 'NONE',  ( -3.703129828913089838, 1440.893638029549948, 155.9280501976939775 ) ) ;
#19999=CARTESIAN_POINT ( 'NONE',  ( -15.18192270269999966, 1451.950609855530047, 149.7661401774980163 ) ) ;
#20001=ORIENTED_EDGE ( 'NONE', *, *, #34948, .F. ) ;
#20002=ORIENTED_EDGE ( 'NONE', *, *, #79699, .T. ) ;
#20005=CARTESIAN_POINT ( 'NONE',  ( -15.38665937919999926, 1471.938829346429884, 270.2482212355980096 ) ) ;
#20007=CARTESIAN_POINT ( 'NONE',  ( 11.91388749740000108, 1435.945967586000052, 151.0354243678980026 ) ) ;
#20008=CARTESIAN_POINT ( 'NONE',  ( -13.94201645220000074, 1463.289818900630053, 223.5921370626980149 ) ) ;
#20011=CARTESIAN_POINT ( 'NONE',  ( 4.762729318109999888, 1475.513060387329915, 188.3206495969979812 ) ) ;
#20013=CARTESIAN_POINT ( 'NONE',  ( -1.274375367929762914, 1484.589685195701577, 182.3028901116345253 ) ) ;
#20015=CARTESIAN_POINT ( 'NONE',  ( -44.13844595298070317, 1430.668308869690009, 268.2729030389940021 ) ) ;
#20022=CARTESIAN_POINT ( 'NONE',  ( -5.992819232552545117, 1414.913060387329779, 198.1520639380683235 ) ) ;
#20033=CARTESIAN_POINT ( 'NONE',  ( -18.55309621579120360, 1413.291055372490064, 269.6533643345190399 ) ) ;
#20035=CARTESIAN_POINT ( 'NONE',  ( 3.481980791854309754, 1416.697837385949924, 231.9089666833169758 ) ) ;
#20039=EDGE_LOOP ( 'NONE', ( #26630, #34925, #11934, #12808, #92188, #34177, #97302, #75125, #15146, #30926, #90562, #106909 ) ) ;
#20040=CARTESIAN_POINT ( 'NONE',  ( 45.61322772378891699, 1442.028537087034465, 268.9754013588537873 ) ) ;
#20046=CARTESIAN_POINT ( 'NONE',  ( -0.5697963391879999895, 1450.893162800530263, 181.2886238165980046 ) ) ;
#20047=CARTESIAN_POINT ( 'NONE',  ( -22.71012388409999971, 1435.763556584229946, 216.7363462006779855 ) ) ;
#20048=B_SPLINE_CURVE_WITH_KNOTS ( 'NONE', 5,
 ( #93220, #17592, #60194, #94313, #25447, #103257, #60762, #85359, #76992, #94885, #110579, #50676 ),
 .UNSPECIFIED., .F., .F.,
 ( 6, 3, 3, 6 ),
 ( -13.24352795601230071, -6.990622299139999996, 15.67373306499999686, 31.20981123833860238 ),
 .UNSPECIFIED. ) ;
#20049=CARTESIAN_POINT ( 'NONE',  ( -13.58268883559999907, 1416.851343902430017, 221.9096085507979979 ) ) ;
#20050=CARTESIAN_POINT ( 'NONE',  ( 11.41983032809999976, 1415.048591094029916, 222.6307558755980267 ) ) ;
#20051=CARTESIAN_POINT ( 'NONE',  ( 3.931911409020000026, 1448.296755876420093, 184.2998929499980250 ) ) ;
#20053=EDGE_LOOP ( 'NONE', ( #42781, #74531, #52598, #61912 ) ) ;
#20055=CARTESIAN_POINT ( 'NONE',  ( 1.475476450778450133, 1481.613566490490030, 182.2253701186220098 ) ) ;
#20058=CARTESIAN_POINT ( 'NONE',  ( 26.46213131619590087, 1451.086884292710010, 136.4161995186190097 ) ) ;
#20059=CARTESIAN_POINT ( 'NONE',  ( 14.19373553490000006, 1416.535385209630022, 196.5182439381979975 ) ) ;
#20062=CARTESIAN_POINT ( 'NONE',  ( 19.69576296570000196, 1409.600851585830014, 200.3825397104079968 ) ) ;
#20063=CARTESIAN_POINT ( 'NONE',  ( 22.43804736130000066, 1409.696614266430061, 208.0348436616479830 ) ) ;
#20064=CARTESIAN_POINT ( 'NONE',  ( 2.842270354763221984, 1439.666206437147821, 183.8926537781620141 ) ) ;
#20066=EDGE_CURVE ( 'NONE', #9014, #10764, #44109, .T. ) ;
#20067=CARTESIAN_POINT ( 'NONE',  ( 21.57000220118974454, 1453.624679045193488, 221.0567102288825367 ) ) ;
#20072=ORIENTED_EDGE ( 'NONE', *, *, #40161, .T. ) ;
#20076=DIRECTION ( 'NONE',  ( -4.654054919228650096E-15, -0.5877852522921409584, 0.8090169943751888137 ) ) ;
#20077=CARTESIAN_POINT ( 'NONE',  ( -39.91414502121379826, 1445.986949094549800, 136.8025261772779686 ) ) ;
#20078=B_SPLINE_CURVE_WITH_KNOTS ( 'NONE', 5,
 ( #34721, #96856, #60501, #86782, #10637, #103013 ),
 .UNSPECIFIED., .F., .F.,
 ( 6, 6 ),
 ( 0.000000000000000000, 1.000000000000000000 ),
 .UNSPECIFIED. ) ;
#20080=CARTESIAN_POINT ( 'NONE',  ( -19.00000000000000000, 1442.955095612160221, 209.1218459616979999 ) ) ;
#20083=CARTESIAN_POINT ( 'NONE',  ( 11.87551015580000069, 1433.043990029219913, 149.9802084965980100 ) ) ;
#20084=CARTESIAN_POINT ( 'NONE',  ( -2.417977538859999775, 1475.011631035330083, 269.6427107995980350 ) ) ;
#20089=DIRECTION ( 'NONE',  ( 1.000000000000000000, 0.000000000000000000, 0.000000000000000000 ) ) ;
#20090=CARTESIAN_POINT ( 'NONE',  ( 24.69315803756887462, 1435.858927457940808, 137.7793366136709494 ) ) ;
#20094=CARTESIAN_POINT ( 'NONE',  ( 2.623998188089999850, 1507.107345730630186, 235.9745089064979879 ) ) ;
#20096=CARTESIAN_POINT ( 'NONE',  ( 25.10029913760000042, 1449.799429875570013, 212.3150031425680027 ) ) ;
#20098=CARTESIAN_POINT ( 'NONE',  ( -10.69913757989999858, 1509.229551463630060, 235.6719099616980202 ) ) ;
#20101=CARTESIAN_POINT ( 'NONE',  ( 1.381905419950689495, 1417.049098607537871, 233.2953553763333616 ) ) ;
#20103=CARTESIAN_POINT ( 'NONE',  ( 0.1622922531163999982, 1484.890809331159971, 181.8842724489669820 ) ) ;
#20105=ORIENTED_EDGE ( 'NONE', *, *, #5277, .F. ) ;
#20106=CARTESIAN_POINT ( 'NONE',  ( -0.5624689348119998877, 1416.828044896230040, 227.7677326544980190 ) ) ;
#20108=CARTESIAN_POINT ( 'NONE',  ( -3.028500014641959837, 1440.533662533890038, 157.2362906761999852 ) ) ;
#20109=CARTESIAN_POINT ( 'NONE',  ( 1.556099495224211315, 1414.941240495253624, 191.9077315098595875 ) ) ;
#20113=B_SPLINE_CURVE_WITH_KNOTS ( 'NONE', 3,
 ( #102962, #76130, #92361, #83969, #52046, #16732, #50395, #84523, #50938, #86182, #102419, #7812, #15633, #41433, #101294, #43638, #25700, #33548, #94022, #77790, #75600, #85063, #41980, #43087, #42519, #51480, #76677, #1099 ),
 .UNSPECIFIED., .F., .F.,
 ( 4, 3, 3, 3, 3, 3, 3, 3, 3, 4 ),
 ( -1.114100599709999972, -0.9686742879261339700, -0.7108175189242720293, -0.4506292099621960201, -0.1893289210266050349, 0.07294244172766051193, 0.3351108158645359492, 0.5965830097836279933, 0.8568147313408711607, 1.114100599709999972 ),
 .UNSPECIFIED. ) ;
#20116=CARTESIAN_POINT ( 'NONE',  ( -3.917424962222913365, 1509.064125152231099, 238.3939863888493562 ) ) ;
#20118=EDGE_CURVE ( 'NONE', #62647, #19615, #18689, .T. ) ;
#20120=CARTESIAN_POINT ( 'NONE',  ( 20.71993696733170154, 1509.684823427714718, 187.7542232460070579 ) ) ;
#20121=CARTESIAN_POINT ( 'NONE',  ( 14.13940509691999914, 1409.406819292400087, 213.9383516266399852 ) ) ;
#20122=B_SPLINE_CURVE_WITH_KNOTS ( 'NONE', 5,
 ( #109482, #74784, #101050, #68050, #102159, #8649, #41715, #17023, #108924 ),
 .UNSPECIFIED., .F., .F.,
 ( 6, 3, 6 ),
 ( 0.000000000000000000, 0.5477639817078383544, 1.000000000000000000 ),
 .UNSPECIFIED. ) ;
#20128=ORIENTED_EDGE ( 'NONE', *, *, #4509, .T. ) ;
#20130=CARTESIAN_POINT ( 'NONE',  ( -12.26979726809049964, 1416.828039266780024, 194.6643405733680083 ) ) ;
#20133=CARTESIAN_POINT ( 'NONE',  ( 10.93744292050253897, 1470.445254532535955, 269.3493099203677730 ) ) ;
#20135=CARTESIAN_POINT ( 'NONE',  ( -0.01233344495960000085, 1396.097901039330281, 221.0480490741980191 ) ) ;
#20137=CARTESIAN_POINT ( 'NONE',  ( -19.19787601965154167, 1486.265670089333526, 189.5055532990568850 ) ) ;
#20139=CARTESIAN_POINT ( 'NONE',  ( 12.71038982811789886, 1507.471771741610155, 233.3404631503599944 ) ) ;
#20141=FACE_OUTER_BOUND ( 'NONE', #22803, .T. ) ;
#20142=CARTESIAN_POINT ( 'NONE',  ( 0.7130988073230000168, 1416.837309283630020, 190.3247695230979843 ) ) ;
#20143=CARTESIAN_POINT ( 'NONE',  ( -66.50000000000000000, 1457.239227002485222, 134.0999999980979851 ) ) ;
#20147=CARTESIAN_POINT ( 'NONE',  ( 41.56052307400000245, 1440.913060319270016, 261.5689801501980014 ) ) ;
#20148=CARTESIAN_POINT ( 'NONE',  ( -25.57225985890000075, 1469.240968291730042, 204.5212093847880226 ) ) ;
#20149=CARTESIAN_POINT ( 'NONE',  ( -2.548197114149999720, 1502.019144614829884, 181.0685241395979688 ) ) ;
#20150=CARTESIAN_POINT ( 'NONE',  ( 2.383381429599379737E-14, 1423.968400963209888, 229.1191372934970047 ) ) ;
#20151=CARTESIAN_POINT ( 'NONE',  ( -22.78790659570000088, 1507.631725798030175, 208.3821237218529916 ) ) ;
#20152=CARTESIAN_POINT ( 'NONE',  ( -34.48978217409999303, 1438.727114829129960, 250.0021841814979950 ) ) ;
#20156=CARTESIAN_POINT ( 'NONE',  ( 4.026786250540000722, 1418.591992575429913, 166.2922546441980103 ) ) ;
#20158=CARTESIAN_POINT ( 'NONE',  ( -5.374434774777560264, 1429.031894749750109, 154.0908929508950109 ) ) ;
#20160=EDGE_CURVE ( 'NONE', #87156, #89942, #60180, .T. ) ;
#20161=CARTESIAN_POINT ( 'NONE',  ( 8.877295140909998494, 1509.263243838729977, 237.7422070772980192 ) ) ;
#20164=CARTESIAN_POINT ( 'NONE',  ( -10.16547411475398732, 1422.464089038557177, 137.0999999980979851 ) ) ;
#20165=CARTESIAN_POINT ( 'NONE',  ( -24.09952038931490037, 1410.987018411419967, 208.6999156859300228 ) ) ;
#20168=CARTESIAN_POINT ( 'NONE',  ( -1.368191959960000093, 1419.344527984530032, 185.2221190034979941 ) ) ;
#20170=LINE ( 'NONE', #37537, #24302 ) ;
#20171=EDGE_CURVE ( 'NONE', #48999, #76557, #29408, .T. ) ;
#20172=CARTESIAN_POINT ( 'NONE',  ( -2.880886796239999548, 1470.483478263630104, 235.2207609509979989 ) ) ;
#20179=VERTEX_POINT ( 'NONE', #68606 ) ;
#20180=CARTESIAN_POINT ( 'NONE',  ( 11.85876122931039944, 1431.823958861970141, 149.9583335947500302 ) ) ;
#20181=CARTESIAN_POINT ( 'NONE',  ( 13.26498293510852200, 1444.636724116999403, 187.4437205532745168 ) ) ;
#20182=VERTEX_POINT ( 'NONE', #38150 ) ;
#20184=CARTESIAN_POINT ( 'NONE',  ( -4.500000000000000000, 1425.929641636930000, 184.1455913746980002 ) ) ;
#20186=CARTESIAN_POINT ( 'NONE',  ( -19.62228242832910396, 1409.598285588889894, 200.2165691342799789 ) ) ;
#20188=CARTESIAN_POINT ( 'NONE',  ( 18.52343394138449995, 1452.266207820500085, 144.8864230035439959 ) ) ;
#20189=CARTESIAN_POINT ( 'NONE',  ( 0.9478853872383249390, 1410.244833127959964, 269.6149691266229524 ) ) ;
#20196=CARTESIAN_POINT ( 'NONE',  ( 15.14114459860000039, 1453.154616238230119, 195.2667548292980086 ) ) ;
#20199=ADVANCED_FACE ( 'NONE', ( #26573 ), #104274, .T. ) ;
#20202=CARTESIAN_POINT ( 'NONE',  ( 8.881784196999999612E-15, 1412.362567936729874, 265.6112251771979800 ) ) ;
#20203=CARTESIAN_POINT ( 'NONE',  ( 18.63535449682491674, 1508.532394786521081, 188.3246405780103601 ) ) ;
#20205=CARTESIAN_POINT ( 'NONE',  ( -1.784652446394692227, 1450.428767247505903, 182.6692972897738230 ) ) ;
#20208=CARTESIAN_POINT ( 'NONE',  ( 30.04560769488690042, 1414.784964249760151, 269.9543914837240095 ) ) ;
#20211=CARTESIAN_POINT ( 'NONE',  ( 17.39559655639999747, 1414.988015881329829, 210.6209832631780046 ) ) ;
#20212=CARTESIAN_POINT ( 'NONE',  ( -24.28688219629999878, 1442.594724193030061, 211.8376374323679840 ) ) ;
#20213=CARTESIAN_POINT ( 'NONE',  ( -11.43741207009999883, 1425.481177415629872, 144.1677667564979970 ) ) ;
#20216=CARTESIAN_POINT ( 'NONE',  ( -10.73123306599999971, 1442.518496289960012, 185.8422046897979953 ) ) ;
#20217=CARTESIAN_POINT ( 'NONE',  ( 19.03563175159720089, 1509.617364368859853, 184.8006368254200140 ) ) ;
#20220=CARTESIAN_POINT ( 'NONE',  ( 2.906835402620000064, 1412.735488669030019, 231.7379915122980094 ) ) ;
#20222=CARTESIAN_POINT ( 'NONE',  ( -16.44430638549999912, 1460.459436675330153, 228.3413476960980120 ) ) ;
#20224=CARTESIAN_POINT ( 'NONE',  ( 35.66139618599999750, 1418.936225598229839, 269.0502396691979925 ) ) ;
#20225=CARTESIAN_POINT ( 'NONE',  ( -18.29129824860000042, 1410.914753684329753, 224.2736566455979812 ) ) ;
#20226=CARTESIAN_POINT ( 'NONE',  ( 20.01829564719999865, 1436.428735692270038, 145.4425850063980192 ) ) ;
#20227=CARTESIAN_POINT ( 'NONE',  ( 24.99297300310000125, 1508.005497761829929, 198.0964541023980132 ) ) ;
#20228=CARTESIAN_POINT ( 'NONE',  ( -16.87994269677939840, 1410.001063948119963, 192.1186093866529916 ) ) ;
#20230=CARTESIAN_POINT ( 'NONE',  ( -17.21795144880000095, 1423.339050169130132, 226.8104169026979946 ) ) ;
#20233=CARTESIAN_POINT ( 'NONE',  ( -7.689951449758970270, 1408.132615477319860, 198.3001377377659935 ) ) ;
#20235=CARTESIAN_POINT ( 'NONE',  ( -17.41472613699927408, 1410.192975592430230, 193.4350317396312562 ) ) ;
#20239=CARTESIAN_POINT ( 'NONE',  ( 22.86388141640000171, 1443.913060387330006, 134.0999999980979851 ) ) ;
#20240=ORIENTED_EDGE ( 'NONE', *, *, #81620, .F. ) ;
#20243=CARTESIAN_POINT ( 'NONE',  ( -16.90742456150000095, 1444.994950788469851, 162.4348202098979925 ) ) ;
#20245=CARTESIAN_POINT ( 'NONE',  ( -4.434413035407485992, 1421.449507706801796, 137.6342364636123534 ) ) ;
#20246=CARTESIAN_POINT ( 'NONE',  ( -31.40725736689999792, 1466.080781296829855, 269.1484934035979677 ) ) ;
#20248=CARTESIAN_POINT ( 'NONE',  ( 0.2538829723067779764, 1420.503732877419907, 182.7635795570130028 ) ) ;
#20254=CARTESIAN_POINT ( 'NONE',  ( 22.51756452349999904, 1509.699391067530087, 227.9212136326980271 ) ) ;
#20255=CARTESIAN_POINT ( 'NONE',  ( -9.421550853199999409, 1433.443826258700028, 153.1575888881980063 ) ) ;
#20259=CARTESIAN_POINT ( 'NONE',  ( -5.740872018370000163, 1508.767882438629840, 180.7041383050980130 ) ) ;
#20262=CARTESIAN_POINT ( 'NONE',  ( -11.70751967709999875, 1415.128105756529976, 195.6471422008980028 ) ) ;
#20264=CARTESIAN_POINT ( 'NONE',  ( 22.70034758849999790, 1409.705773992930062, 211.1194685625279988 ) ) ;
#20265=CARTESIAN_POINT ( 'NONE',  ( -12.24435440740000125, 1434.149509971349971, 149.6614242918979869 ) ) ;
#20267=CARTESIAN_POINT ( 'NONE',  ( -5.360263152496679950, 1422.240933723030139, 144.3253770615330041 ) ) ;
#20268=CARTESIAN_POINT ( 'NONE',  ( -10.97839346949999850, 1432.873346371779917, 151.7696626658980108 ) ) ;
#20270=CARTESIAN_POINT ( 'NONE',  ( 1.456985595923120158, 1417.743458194299819, 225.5366272655959676 ) ) ;
#20276=CARTESIAN_POINT ( 'NONE',  ( 13.37672536222529907, 1507.734881312529978, 233.0720187032129900 ) ) ;
#20277=CARTESIAN_POINT ( 'NONE',  ( -16.81674069857199783, 1486.117794611840054, 187.5515125930209877 ) ) ;
#20279=CARTESIAN_POINT ( 'NONE',  ( 18.73327636269999985, 1416.067629296030191, 210.6711993623479771 ) ) ;
#20283=CARTESIAN_POINT ( 'NONE',  ( 29.75011777459999962, 1509.993906964230064, 209.6841330031659822 ) ) ;
#20286=CARTESIAN_POINT ( 'NONE',  ( 1.547463840030000037, 1414.913060387329779, 192.3096136973980208 ) ) ;
#20287=CARTESIAN_POINT ( 'NONE',  ( 15.83156775414370010, 1415.884059795909934, 191.3615640054380265 ) ) ;
#20288=CARTESIAN_POINT ( 'NONE',  ( 0.4986428671280000446, 1508.154336060129936, 180.7475829099980160 ) ) ;
#20292=CARTESIAN_POINT ( 'NONE',  ( -25.28519595180179991, 1451.584664909089952, 136.7789216481089909 ) ) ;
#20293=CARTESIAN_POINT ( 'NONE',  ( 4.500000000000000000, 1418.913060387330006, 172.2701767054979882 ) ) ;
#20294=CARTESIAN_POINT ( 'NONE',  ( 7.055136800019999654, 1409.159431195129855, 229.7764860247980039 ) ) ;
#20298=CARTESIAN_POINT ( 'NONE',  ( 41.21983904255579745, 1446.341078051059867, 134.0999999985669717 ) ) ;
#20305=VERTEX_POINT ( 'NONE', #9504 ) ;
#20309=CARTESIAN_POINT ( 'NONE',  ( 8.479372880465721352, 1451.373121564088933, 152.7985077061053119 ) ) ;
#20314=CARTESIAN_POINT ( 'NONE',  ( 4.282754796476449854, 1446.855225404319981, 156.0904130296160019 ) ) ;
#20315=EDGE_CURVE ( 'NONE', #60804, #61195, #76711, .T. ) ;
#20316=CARTESIAN_POINT ( 'NONE',  ( 0.3083741877719999858, 1507.133244740429973, 237.3561682571980214 ) ) ;
#20320=CARTESIAN_POINT ( 'NONE',  ( 26.37664415071539992, 1440.913060387330006, 243.3089104971339793 ) ) ;
#20321=CARTESIAN_POINT ( 'NONE',  ( -19.21279374710000099, 1509.245052335930040, 187.4406862720980200 ) ) ;
#20322=ORIENTED_EDGE ( 'NONE', *, *, #3633, .T. ) ;
#20325=CARTESIAN_POINT ( 'NONE',  ( -13.35894093149999939, 1409.546307774629895, 190.4983039755979917 ) ) ;
#20327=B_SPLINE_CURVE_WITH_KNOTS ( 'NONE', 3,
 ( #60004, #42634, #94124, #67854 ),
 .UNSPECIFIED., .F., .F.,
 ( 4, 4 ),
 ( 0.6833227323573606293, 1.000000000000000000 ),
 .UNSPECIFIED. ) ;
#20328=CARTESIAN_POINT ( 'NONE',  ( -24.40370832145195479, 1440.437192627858167, 212.0119382815727249 ) ) ;
#20332=CARTESIAN_POINT ( 'NONE',  ( -1.676215897828090107, 1450.511945644329899, 182.4451613505460159 ) ) ;
#20333=CARTESIAN_POINT ( 'NONE',  ( -12.06083241689999852, 1433.903765800100018, 149.9805303096979969 ) ) ;
#20335=CARTESIAN_POINT ( 'NONE',  ( 6.415419946120000105, 1464.066614333030202, 235.9991510476980068 ) ) ;
#20339=CARTESIAN_POINT ( 'NONE',  ( -2.664535259099599458E-15, 1405.913060387330006, 209.1218459616979999 ) ) ;
#20340=CARTESIAN_POINT ( 'NONE',  ( 29.52080212560000305, 1509.954550774029940, 207.1882801656479955 ) ) ;
#20342=FACE_OUTER_BOUND ( 'NONE', #65945, .T. ) ;
#20348=CARTESIAN_POINT ( 'NONE',  ( 31.18244400220000045, 1447.044067090409953, 244.2061907871979827 ) ) ;
#20353=CARTESIAN_POINT ( 'NONE',  ( 11.77480454480000027, 1432.721964424879843, 150.8108404446980160 ) ) ;
#20354=CARTESIAN_POINT ( 'NONE',  ( 2.500000000000000000, 1421.615752562629950, 151.7766360386979727 ) ) ;
#20359=CARTESIAN_POINT ( 'NONE',  ( 1.333623352150000052, 1405.763012363830057, 267.5364538210980072 ) ) ;
#20361=CARTESIAN_POINT ( 'NONE',  ( 31.49563175233199885, 1465.375308357740096, 270.2507308408049767 ) ) ;
#20362=CARTESIAN_POINT ( 'NONE',  ( 2.478879819430000353, 1433.496472462500151, 157.5502782321979964 ) ) ;
#20364=CARTESIAN_POINT ( 'NONE',  ( -44.78652650876009744, 1440.913060399449932, 265.2360415858299802 ) ) ;
#20368=CARTESIAN_POINT ( 'NONE',  ( 2.500290409796250390, 1448.931711166909963, 154.7923209379179923 ) ) ;
#20371=ORIENTED_EDGE ( 'NONE', *, *, #11845, .F. ) ;
#20372=CARTESIAN_POINT ( 'NONE',  ( -28.02005516190000023, 1440.913060387330006, 248.0989693021979861 ) ) ;
#20373=CIRCLE ( 'NONE', #14932, 1.638701816490922836 ) ;
#20375=CARTESIAN_POINT ( 'NONE',  ( -0.1071916394719999999, 1475.561145520229957, 269.2947192205979832 ) ) ;
#20376=CARTESIAN_POINT ( 'NONE',  ( -4.269401038497079526, 1446.687744141539952, 158.1052691740970033 ) ) ;
#20377=CARTESIAN_POINT ( 'NONE',  ( -28.31864945599999928, 1509.156311078129875, 210.0890843349349950 ) ) ;
#20380=B_SPLINE_CURVE_WITH_KNOTS ( 'NONE', 5,
 ( #14634, #65062, #56103, #90232, #48820, #22457, #56658, #14075, #48264 ),
 .UNSPECIFIED., .F., .F.,
 ( 6, 3, 6 ),
 ( 0.000000000000000000, 0.5000000000000000000, 1.000000000000000000 ),
 .UNSPECIFIED. ) ;
#20383=CARTESIAN_POINT ( 'NONE',  ( -18.78419925920000111, 1416.547221146729953, 208.4031831864560047 ) ) ;
#20384=DIRECTION ( 'NONE',  ( 0.000000000000000000, 0.000000000000000000, 1.000000000000000000 ) ) ;
#20385=CARTESIAN_POINT ( 'NONE',  ( 26.45852657916749706, 1436.406839490560060, 136.7425343492149921 ) ) ;
#20386=CARTESIAN_POINT ( 'NONE',  ( -11.05566370613560068, 1396.299132671179905, 209.7399892603730223 ) ) ;
#20388=CARTESIAN_POINT ( 'NONE',  ( -16.09035704788109911, 1409.474929536219861, 225.2671591083089879 ) ) ;
#20390=ORIENTED_EDGE ( 'NONE', *, *, #34494, .F. ) ;
#20391=CARTESIAN_POINT ( 'NONE',  ( -21.33073281829999956, 1509.431426448229786, 190.3502236029979997 ) ) ;
#20392=CARTESIAN_POINT ( 'NONE',  ( 2.073856897040000202, 1408.985481066030161, 230.8023040625980116 ) ) ;
#20393=CARTESIAN_POINT ( 'NONE',  ( -11.81707100502839936, 1430.266226932280006, 147.2485954771549928 ) ) ;
#20394=CARTESIAN_POINT ( 'NONE',  ( 11.23902904340000042, 1426.879266721829936, 108.0467253156979979 ) ) ;
#20396=CARTESIAN_POINT ( 'NONE',  ( -4.649632279085039954, 1420.176633138330089, 186.4708453798239987 ) ) ;
#20397=CARTESIAN_POINT ( 'NONE',  ( 4.222917386638090242, 1423.993296039239794, 184.1168122550120074 ) ) ;
#20401=CARTESIAN_POINT ( 'NONE',  ( 5.579395061470000527, 1508.557821581529879, 181.5499561553979788 ) ) ;
#20405=CARTESIAN_POINT ( 'NONE',  ( 15.68557540059999766, 1410.853897593529837, 191.5168599455980143 ) ) ;
#20408=CARTESIAN_POINT ( 'NONE',  ( -12.97256852330023058, 1446.865977941818528, 187.9439244580588024 ) ) ;
#20409=CARTESIAN_POINT ( 'NONE',  ( 0.09108844601094030768, 1499.038884509760010, 237.0407834095410067 ) ) ;
#20413=CARTESIAN_POINT ( 'NONE',  ( -1.364118118321220097, 1416.140226195509968, 185.3579479993269672 ) ) ;
#20414=CARTESIAN_POINT ( 'NONE',  ( 0.8591459077770000619, 1410.309640869729947, 185.1536886007980058 ) ) ;
#20415=CARTESIAN_POINT ( 'NONE',  ( 13.15468524849227094, 1428.736268150490105, 222.9360349510320702 ) ) ;
#20416=CARTESIAN_POINT ( 'NONE',  ( -39.40612923876570051, 1447.975168223910032, 136.4769383534059841 ) ) ;
#20418=CARTESIAN_POINT ( 'NONE',  ( -2.500000000000000000, 1448.480947779509961, 160.8719867021480070 ) ) ;
#20421=CARTESIAN_POINT ( 'NONE',  ( -5.299937475575299928, 1406.728889454019964, 269.4890040361959791 ) ) ;
#20425=CARTESIAN_POINT ( 'NONE',  ( 12.62483932640000006, 1441.362374013529916, 188.6153039823980180 ) ) ;
#20427=EDGE_LOOP ( 'NONE', ( #1339, #39124, #47589, #105102 ) ) ;
#20429=CARTESIAN_POINT ( 'NONE',  ( -13.46389150100000087, 1461.194501461529853, 230.8146161405980195 ) ) ;
#20433=CARTESIAN_POINT ( 'NONE',  ( 2.500000000000000000, 1448.416731250589919, 161.9264764492260156 ) ) ;
#20436=CARTESIAN_POINT ( 'NONE',  ( 2.857576036340000236, 1416.519106787530063, 226.9547723584980190 ) ) ;
#20441=CARTESIAN_POINT ( 'NONE',  ( -4.079938673100000024, 1409.222872079729996, 231.6014056192980206 ) ) ;
#20443=ORIENTED_EDGE ( 'NONE', *, *, #21057, .F. ) ;
#20444=CARTESIAN_POINT ( 'NONE',  ( 32.73687869649999982, 1451.769863600429971, 134.7502305315980209 ) ) ;
#20445=CARTESIAN_POINT ( 'NONE',  ( 10.88633642001528479, 1425.077222887074640, 139.1358730495393559 ) ) ;
#20449=CARTESIAN_POINT ( 'NONE',  ( 20.61505026639999727, 1412.093511550830044, 270.3833838262979725 ) ) ;
#20453=CARTESIAN_POINT ( 'NONE',  ( 0.02024940985663903001, 1507.190131585810150, 237.3571517750307294 ) ) ;
#20455=CARTESIAN_POINT ( 'NONE',  ( 20.45512642757772781, 1410.987358542064840, 198.4416328032433512 ) ) ;
#20458=CARTESIAN_POINT ( 'NONE',  ( 4.315674504236409526, 1420.473761226789975, 185.6540625970839926 ) ) ;
#20459=CARTESIAN_POINT ( 'NONE',  ( -0.5925149063449999254, 1420.455671712929870, 233.5810819935980192 ) ) ;
#20464=CARTESIAN_POINT ( 'NONE',  ( -20.61688129168850026, 1509.299807670030077, 229.2235502797169886 ) ) ;
#20466=CARTESIAN_POINT ( 'NONE',  ( 0.08524399098180000800, 1408.910083407030015, 232.2087777920980045 ) ) ;
#20470=CARTESIAN_POINT ( 'NONE',  ( 19.27290132190000094, 1509.486203139530062, 187.3727875556980109 ) ) ;
#20471=DIRECTION ( 'NONE',  ( -1.000000000000000000, 0.000000000000000000, 0.000000000000000000 ) ) ;
#20473=CARTESIAN_POINT ( 'NONE',  ( -13.01305160751540058, 1416.520646088689773, 196.6194545781839906 ) ) ;
#20477=CARTESIAN_POINT ( 'NONE',  ( -0.2739174590469999893, 1497.001329539429889, 230.9798146536980141 ) ) ;
#20478=DIRECTION ( 'NONE',  ( 1.000000000000000000, 0.000000000000000000, 0.000000000000000000 ) ) ;
#20479=DIRECTION ( 'NONE',  ( 0.000000000000000000, 1.000000000000000000, 0.000000000000000000 ) ) ;
#20480=CIRCLE ( 'NONE', #17110, 262.4356363184970746 ) ;
#20482=CARTESIAN_POINT ( 'NONE',  ( 15.77707647795940638, 1421.138165674653692, 227.5460774834178608 ) ) ;
#20483=CARTESIAN_POINT ( 'NONE',  ( 6.032762746330000425, 1424.401310572229931, 186.1143022581979949 ) ) ;
#20484=CARTESIAN_POINT ( 'NONE',  ( -17.73405907629999589, 1423.343206274430031, 226.1884625415979997 ) ) ;
#20485=CARTESIAN_POINT ( 'NONE',  ( -19.18996605219999907, 1435.312409617389903, 145.3494678388979935 ) ) ;
#20486=CARTESIAN_POINT ( 'NONE',  ( 33.92643312500000263, 1450.868062273570104, 136.1711485282980050 ) ) ;
#20488=CARTESIAN_POINT ( 'NONE',  ( 0.5924570975656898719, 1409.870418501489894, 233.1347249525960024 ) ) ;
#20489=CARTESIAN_POINT ( 'NONE',  ( -17.77930361275660331, 1434.665529742419039, 215.4045010112904492 ) ) ;
#20493=DIRECTION ( 'NONE',  ( -0.7074300732097413835, -0.02470400246699151064, -0.7063514732628303205 ) ) ;
#20494=CARTESIAN_POINT ( 'NONE',  ( -45.63712966311000230, 1440.913059426480004, 268.9747523979869470 ) ) ;
#20495=B_SPLINE_CURVE_WITH_KNOTS ( 'NONE', 5,
 ( #3699, #36173, #2040, #106131, #62512, #95520, #88783, #37827, #18791, #29404, #63607, #19343 ),
 .UNSPECIFIED., .F., .F.,
 ( 6, 3, 3, 6 ),
 ( 0.000000000000000000, 0.3100030845520760359, 0.7700076031013588507, 1.000000000000000000 ),
 .UNSPECIFIED. ) ;
#20496=CARTESIAN_POINT ( 'NONE',  ( -11.93337329947367742, 1433.461403735681188, 149.9038200615264600 ) ) ;
#20499=CARTESIAN_POINT ( 'NONE',  ( 0.1595995995380000143, 1486.508831850330125, 181.8147405652979671 ) ) ;
#20500=CARTESIAN_POINT ( 'NONE',  ( 11.72456630055093996, 1435.127050470847053, 151.3186841771734237 ) ) ;
#20507=ADVANCED_FACE ( 'NONE', ( #110310 ), #11329, .T. ) ;
#20511=EDGE_LOOP ( 'NONE', ( #76229, #82432, #44434, #110269 ) ) ;
#20513=EDGE_CURVE ( 'NONE', #28929, #84627, #70179, .T. ) ;
#20516=EDGE_LOOP ( 'NONE', ( #50993, #44850, #11403, #41817, #40261 ) ) ;
#20518=CARTESIAN_POINT ( 'NONE',  ( 24.59711297958679665, 1435.768809675110106, 207.7339403979270003 ) ) ;
#20520=CARTESIAN_POINT ( 'NONE',  ( 12.94625993752471338, 1442.917207449076159, 169.4295987738932183 ) ) ;
#20521=CARTESIAN_POINT ( 'NONE',  ( 34.96930673469186246, 1424.017833468233675, 269.5310884720407216 ) ) ;
#20522=CARTESIAN_POINT ( 'NONE',  ( -33.60183515930000198, 1443.049082916849784, 248.0844435638979917 ) ) ;
#20524=CARTESIAN_POINT ( 'NONE',  ( -19.88118183330000122, 1503.697998832129997, 189.0919093254979941 ) ) ;
#20525=CARTESIAN_POINT ( 'NONE',  ( -11.22394236169999893, 1433.945146393620007, 151.5926485512979980 ) ) ;
#20526=CARTESIAN_POINT ( 'NONE',  ( 25.89800611569999944, 1509.146170259929931, 199.8184420921580227 ) ) ;
#20527=CARTESIAN_POINT ( 'NONE',  ( 11.68656446679660021, 1426.729241074910078, 140.5600695502919848 ) ) ;
#20528=CARTESIAN_POINT ( 'NONE',  ( 5.846862684000000421, 1409.284248634629876, 187.2876011129980043 ) ) ;
#20529=CARTESIAN_POINT ( 'NONE',  ( 5.871102057859999945, 1422.424335551330159, 186.1421875806979926 ) ) ;
#20535=CARTESIAN_POINT ( 'NONE',  ( -6.341639189019999456, 1451.866620239630265, 153.5781910428979984 ) ) ;
#20536=CARTESIAN_POINT ( 'NONE',  ( 2.689344590370000176, 1464.716346886629935, 236.9361822375979898 ) ) ;
#20537=ORIENTED_EDGE ( 'NONE', *, *, #36883, .T. ) ;
#20539=CARTESIAN_POINT ( 'NONE',  ( -11.86317285837269964, 1432.131441266870070, 149.9785579755850051 ) ) ;
#20541=CARTESIAN_POINT ( 'NONE',  ( -20.37632776330000084, 1469.127044835530114, 270.3601821493979855 ) ) ;
#20542=CARTESIAN_POINT ( 'NONE',  ( -24.02424858472472380, 1435.845097858818235, 211.1058378785815535 ) ) ;
#20543=CARTESIAN_POINT ( 'NONE',  ( 17.83435814839999978, 1410.458698069130151, 223.1757618168979889 ) ) ;
#20544=CARTESIAN_POINT ( 'NONE',  ( -11.87563350447849864, 1433.006677213540115, 147.6591432354780125 ) ) ;
#20545=CARTESIAN_POINT ( 'NONE',  ( 8.010413950200000244, 1453.313060387329870, 190.7496879910979715 ) ) ;
#20546=CARTESIAN_POINT ( 'NONE',  ( -12.65888505820000098, 1420.995398902329953, 230.4350877688980006 ) ) ;
#20547=EDGE_CURVE ( 'NONE', #33885, #64548, #68122, .T. ) ;
#20550=CARTESIAN_POINT ( 'NONE',  ( -45.50346263270189695, 1435.593246726289863, 268.5130472730970155 ) ) ;
#20551=EDGE_LOOP ( 'NONE', ( #26086, #84484, #53668, #37345, #99065 ) ) ;
#20552=CARTESIAN_POINT ( 'NONE',  ( -3.546551875093320039, 1504.287448871370088, 181.0979340408339908 ) ) ;
#20557=CARTESIAN_POINT ( 'NONE',  ( 17.41472478055370132, 1410.192973118622604, 224.8086574190646729 ) ) ;
#20558=CARTESIAN_POINT ( 'NONE',  ( -14.69625711549999991, 1410.404083825129874, 190.5984733045979738 ) ) ;
#20564=EDGE_CURVE ( 'NONE', #74353, #54755, #31987, .T. ) ;
#20565=CARTESIAN_POINT ( 'NONE',  ( 18.46438756856120023, 1509.557851009430124, 186.5303332237980101 ) ) ;
#20568=ORIENTED_EDGE ( 'NONE', *, *, #101731, .F. ) ;
#20569=CARTESIAN_POINT ( 'NONE',  ( -25.88986846590829671, 1416.384201605210137, 269.9259352108049939 ) ) ;
#20570=FACE_OUTER_BOUND ( 'NONE', #56993, .T. ) ;
#20571=CARTESIAN_POINT ( 'NONE',  ( 0.001991242090180000025, 1395.912990851529912, 197.8078701673980220 ) ) ;
#20575=CARTESIAN_POINT ( 'NONE',  ( 45.62473919765866981, 1441.709900562783332, 268.9750890229884135 ) ) ;
#20577=CARTESIAN_POINT ( 'NONE',  ( 3.689298841057521372, 1424.196346644569076, 183.9704267610078148 ) ) ;
#20580=CARTESIAN_POINT ( 'NONE',  ( 5.387463376540000404, 1432.539377501929948, 154.6119119043980277 ) ) ;
#20581=CARTESIAN_POINT ( 'NONE',  ( 10.58535985277509894, 1474.990920022710043, 269.2679215465090010 ) ) ;
#20582=CARTESIAN_POINT ( 'NONE',  ( 12.18103061950000132, 1415.553739809529816, 223.0375094449979940 ) ) ;
#20583=CARTESIAN_POINT ( 'NONE',  ( 4.049067852170000315, 1446.316878933369935, 182.9871537193980089 ) ) ;
#20584=( BOUNDED_CURVE ( )  B_SPLINE_CURVE ( 3, ( #59310, #50355, #41934, #34077 ),
 .UNSPECIFIED., .F., .F. ) 
 B_SPLINE_CURVE_WITH_KNOTS ( ( 4, 4 ),
 ( 1.570796326794965614, 4.212388980384758952 ),
 .UNSPECIFIED. ) 
 CURVE ( )  GEOMETRIC_REPRESENTATION_ITEM ( )  RATIONAL_B_SPLINE_CURVE ( ( 1.000000000000000000, 0.4982693061696819581, 0.4982693061696819581, 1.000000000000000000 ) ) 
 REPRESENTATION_ITEM ( '' )  );
#20587=DIRECTION ( 'NONE',  ( -5.164946217006259634E-18, 0.000000000000000000, -1.000000000000000000 ) ) ;
#20588=CARTESIAN_POINT ( 'NONE',  ( -23.83238225862761794, 1446.589712416024213, 213.8438450975477281 ) ) ;
#20589=ORIENTED_EDGE ( 'NONE', *, *, #90309, .T. ) ;
#20590=CARTESIAN_POINT ( 'NONE',  ( 10.56643885385577875, 1455.157788284585422, 226.2919240970107353 ) ) ;
#20591=CARTESIAN_POINT ( 'NONE',  ( 23.99734131323389974, 1452.069796923729882, 137.0529556418699997 ) ) ;
#20593=CARTESIAN_POINT ( 'NONE',  ( -2.923521517025829741, 1410.394928878200062, 186.6127595807840009 ) ) ;
#20594=CARTESIAN_POINT ( 'NONE',  ( -5.389719915088219793, 1440.971386074470047, 154.8246291213590098 ) ) ;
#20596=CARTESIAN_POINT ( 'NONE',  ( -3.827327205999999649, 1416.243718512830128, 162.3415388335980083 ) ) ;
#20600=CARTESIAN_POINT ( 'NONE',  ( 2.500000000000000000, 1439.615921250379870, 167.6891701647670061 ) ) ;
#20604=ORIENTED_EDGE ( 'NONE', *, *, #21307, .F. ) ;
#20606=CARTESIAN_POINT ( 'NONE',  ( 0.08276195847810161044, 1408.915950497909762, 187.0495686484979956 ) ) ;
#20607=CARTESIAN_POINT ( 'NONE',  ( -13.15726448721240160, 1416.851343896870048, 221.9096085506390068 ) ) ;
#20608=FACE_OUTER_BOUND ( 'NONE', #83788, .T. ) ;
#20610=CARTESIAN_POINT ( 'NONE',  ( -40.20457429252190451, 1444.781942773269975, 137.0004547941439910 ) ) ;
#20614=CARTESIAN_POINT ( 'NONE',  ( 11.07166356589999978, 1433.243716658159883, 151.7035676110980091 ) ) ;
#20615=FACE_OUTER_BOUND ( 'NONE', #89195, .T. ) ;
#20616=B_SPLINE_SURFACE_WITH_KNOTS ( 'NONE', 5, 5, ( 
 ( #105648, #79336, #46309, #11576, #63123, #2094 ),
 ( #45195, #80438, #70408, #70967, #60900, #52488 ),
 ( #45753, #105083, #86616, #27824, #3753, #37885 ),
 ( #72069, #28371, #35663, #19961, #54156, #18295 ),
 ( #44080, #78219, #28933, #1529, #62004, #103970 ),
 ( #10465, #19398, #53602, #87746, #3204, #82068 ) ),
 .UNSPECIFIED., .F., .F., .F.,
 ( 6, 6 ),
 ( 6, 6 ),
 ( 40.35130054919999765, 45.55451570600000366 ),
 ( 0.000000000000000000, 2.000000000060000005 ),
 .UNSPECIFIED. ) ;
#20619=CYLINDRICAL_SURFACE ( 'NONE', #22383, 10.00000000000000000 ) ;
#20621=DIRECTION ( 'NONE',  ( -1.000000000000000000, 0.000000000000000000, 0.000000000000000000 ) ) ;
#20625=CARTESIAN_POINT ( 'NONE',  ( 2.362637160190000252, 1507.103770644730048, 236.0496999084980132 ) ) ;
#20627=CARTESIAN_POINT ( 'NONE',  ( -0.6774325393469999845, 1465.095555782530027, 238.0673157071979915 ) ) ;
#20628=CARTESIAN_POINT ( 'NONE',  ( -13.71017305750000048, 1507.516664216029994, 232.5217224164979939 ) ) ;
#20632=CARTESIAN_POINT ( 'NONE',  ( 20.97834595694860127, 1506.096755889989936, 226.0120427145139956 ) ) ;
#20633=FACE_OUTER_BOUND ( 'NONE', #50596, .T. ) ;
#20635=CARTESIAN_POINT ( 'NONE',  ( 2.811694866999999931, 1464.674002741930053, 236.8041412282979934 ) ) ;
#20636=EDGE_CURVE ( 'NONE', #67105, #4207, #4061, .T. ) ;
#20637=DIRECTION ( 'NONE',  ( 0.000000000000000000, 0.000000000000000000, 1.000000000000000000 ) ) ;
#20638=EDGE_LOOP ( 'NONE', ( #98822, #30640, #40640, #76929, #54409, #57394, #7481, #79123, #57738, #48593 ) ) ;
#20639=CARTESIAN_POINT ( 'NONE',  ( -1.378953279320000114, 1450.758537438610119, 182.6902919710979916 ) ) ;
#20648=CARTESIAN_POINT ( 'NONE',  ( 12.27023112330000032, 1416.839692136459917, 223.5796784318309847 ) ) ;
#20649=CARTESIAN_POINT ( 'NONE',  ( 11.87973986201449961, 1433.324300360609868, 147.6568050212700030 ) ) ;
#20651=EDGE_CURVE ( 'NONE', #91418, #24977, #77411, .T. ) ;
#20654=CARTESIAN_POINT ( 'NONE',  ( 14.93347384300719938, 1409.434548785099878, 209.2195559055120100 ) ) ;
#20655=CARTESIAN_POINT ( 'NONE',  ( 18.02454965899999806, 1424.443906294430008, 224.7645392682979946 ) ) ;
#20657=CARTESIAN_POINT ( 'NONE',  ( -18.43186383950000007, 1440.792975980310075, 191.7737155625979995 ) ) ;
#20658=CARTESIAN_POINT ( 'NONE',  ( 10.96917002130000007, 1432.328099426499875, 151.7701195723979879 ) ) ;
#20659=EDGE_CURVE ( 'NONE', #18765, #75001, #37159, .T. ) ;
#20665=CARTESIAN_POINT ( 'NONE',  ( -12.10884181134970028, 1416.007771869970156, 194.8210225066299870 ) ) ;
#20667=CARTESIAN_POINT ( 'NONE',  ( 20.74483292822688441, 1467.449581717848332, 269.3942764596831125 ) ) ;
#20669=CARTESIAN_POINT ( 'NONE',  ( 0.1955981723673640149, 1414.913060387329779, 225.1861338915940109 ) ) ;
#20670=CARTESIAN_POINT ( 'NONE',  ( 20.76266746499769766, 1464.825020750889962, 209.7053101748109896 ) ) ;
#20672=CARTESIAN_POINT ( 'NONE',  ( -1.455133652010000000, 1471.168344426330123, 183.0463840045979964 ) ) ;
#20674=CARTESIAN_POINT ( 'NONE',  ( -26.57701928479934850, 1436.737487800338386, 136.7979441010809296 ) ) ;
#20675=CARTESIAN_POINT ( 'NONE',  ( 2.688588257229999723, 1509.006947958130013, 238.2844991894980069 ) ) ;
#20680=CARTESIAN_POINT ( 'NONE',  ( 16.65035232609999838, 1409.494503502829957, 193.9825473880979985 ) ) ;
#20682=DIRECTION ( 'NONE',  ( 0.7074300732946419146, 0.02470400257053509060, -0.7063514731741787900 ) ) ;
#20687=CARTESIAN_POINT ( 'NONE',  ( 27.17992431440000090, 1424.801532951130184, 248.2870168903980073 ) ) ;
#20688=CARTESIAN_POINT ( 'NONE',  ( -26.35247771899999947, 1469.246089667830120, 207.6027827722479913 ) ) ;
#20689=CARTESIAN_POINT ( 'NONE',  ( -11.09501388980000058, 1426.902722246829853, 97.52861334269789495 ) ) ;
#20691=LINE ( 'NONE', #11763, #75450 ) ;
#20693=CARTESIAN_POINT ( 'NONE',  ( -29.81189463440000154, 1423.440805878429956, 254.8364553539980193 ) ) ;
#20694=CARTESIAN_POINT ( 'NONE',  ( 19.82628316702480120, 1509.637547285240089, 231.2121791950689840 ) ) ;
#20696=CARTESIAN_POINT ( 'NONE',  ( 31.79025968199999852, 1451.649844149130104, 135.6495218311980011 ) ) ;
#20698=CARTESIAN_POINT ( 'NONE',  ( 3.774231707645040235, 1397.713543333530197, 196.1008760955799914 ) ) ;
#20700=CARTESIAN_POINT ( 'NONE',  ( 38.60856580501570079, 1443.613625263020140, 137.1750438873210101 ) ) ;
#20704=CARTESIAN_POINT ( 'NONE',  ( -24.08426373734519998, 1411.115196246010100, 208.6111089511020111 ) ) ;
#20705=ORIENTED_EDGE ( 'NONE', *, *, #105925, .T. ) ;
#20706=CARTESIAN_POINT ( 'NONE',  ( -0.3097659845029999692, 1413.830979672630065, 184.8391456572979905 ) ) ;
#20709=CARTESIAN_POINT ( 'NONE',  ( -0.8321976068670000615, 1470.487602970729995, 235.6631316893979999 ) ) ;
#20713=VECTOR ( 'NONE', #84535, 1000.000000000000000 ) ;
#20715=CARTESIAN_POINT ( 'NONE',  ( -12.30902781859879980, 1415.426561690370136, 221.5637004564220263 ) ) ;
#20720=ORIENTED_EDGE ( 'NONE', *, *, #84518, .T. ) ;
#20721=CARTESIAN_POINT ( 'NONE',  ( 11.85926072867510150, 1431.858703157390210, 149.9614524602589825 ) ) ;
#20723=VERTEX_POINT ( 'NONE', #28392 ) ;
#20730=CARTESIAN_POINT ( 'NONE',  ( 19.55518754910140089, 1452.230178190589868, 143.7793110295839938 ) ) ;
#20735=CARTESIAN_POINT ( 'NONE',  ( 0.03381540887034163723, 1410.042656433180582, 233.1880969024354897 ) ) ;
#20737=CARTESIAN_POINT ( 'NONE',  ( 16.83556426100000181, 1507.627022993330229, 193.5811530782980014 ) ) ;
#20739=EDGE_CURVE ( 'NONE', #65067, #45960, #84142, .T. ) ;
#20740=CARTESIAN_POINT ( 'NONE',  ( -24.71826599937909918, 1509.391144592290175, 222.6450861662429759 ) ) ;
#20742=ORIENTED_EDGE ( 'NONE', *, *, #28541, .T. ) ;
#20743=CARTESIAN_POINT ( 'NONE',  ( 24.08292308420000083, 1431.749769074620190, 243.9198229428980085 ) ) ;
#20744=CARTESIAN_POINT ( 'NONE',  ( 41.66193277014346563, 1443.744876556161444, 136.1277638562497998 ) ) ;
#20748=CARTESIAN_POINT ( 'NONE',  ( 0.0001732888907949209931, 1456.398128790439841, 144.1938086916980239 ) ) ;
#20749=CARTESIAN_POINT ( 'NONE',  ( -4.155669664704369382, 1439.704322410719897, 185.4969487652249995 ) ) ;
#20751=CARTESIAN_POINT ( 'NONE',  ( 17.08684344950000167, 1414.913528139129994, 210.5362852913079905 ) ) ;
#20752=CARTESIAN_POINT ( 'NONE',  ( -24.18145766900000027, 1443.722874644100102, 211.6519070434079879 ) ) ;
#20756=CARTESIAN_POINT ( 'NONE',  ( -9.295420174100000210, 1442.315068272750068, 184.6978245454979799 ) ) ;
#20757=CARTESIAN_POINT ( 'NONE',  ( 16.98869690429640045, 1509.546007420790147, 233.7379480452109988 ) ) ;
#20760=CARTESIAN_POINT ( 'NONE',  ( -12.29727565780000020, 1497.713060387329961, 227.1658498148980243 ) ) ;
#20761=CARTESIAN_POINT ( 'NONE',  ( 12.44046721790000021, 1412.739136509929949, 228.9069206073980070 ) ) ;
#20765=CARTESIAN_POINT ( 'NONE',  ( 46.15243926309999978, 1440.913083839520141, 268.2044236978980507 ) ) ;
#20766=CARTESIAN_POINT ( 'NONE',  ( -18.27903283859999917, 1410.475184850630058, 224.2578147637979953 ) ) ;
#20767=CARTESIAN_POINT ( 'NONE',  ( 18.91392684480000241, 1435.157588376100193, 144.3614089622979861 ) ) ;
#20768=CARTESIAN_POINT ( 'NONE',  ( 19.88385004780000287, 1469.159394736730064, 191.8385097409980062 ) ) ;
#20770=CARTESIAN_POINT ( 'NONE',  ( -16.64306880943670208, 1409.659795607699834, 192.3834754672400038 ) ) ;
#20771=CARTESIAN_POINT ( 'NONE',  ( -0.5566428566430000613, 1475.834717975330022, 266.9610393015980208 ) ) ;
#20773=CARTESIAN_POINT ( 'NONE',  ( -34.91933993935739977, 1435.878760628219879, 135.9122342505640120 ) ) ;
#20774=CARTESIAN_POINT ( 'NONE',  ( 0.2141777920064759921, 1455.006893489930007, 183.1673017730030040 ) ) ;
#20775=CARTESIAN_POINT ( 'NONE',  ( -12.39163543625050146, 1408.824655388370047, 216.1170731771779856 ) ) ;
#20780=CARTESIAN_POINT ( 'NONE',  ( 11.94161923459999919, 1433.614922939690132, 146.9203179002980164 ) ) ;
#20781=CARTESIAN_POINT ( 'NONE',  ( -27.23873616999999925, 1436.777316193260049, 136.7688712040979908 ) ) ;
#20785=CARTESIAN_POINT ( 'NONE',  ( 39.25629876709999877, 1437.713110276969928, 136.4562061956980017 ) ) ;
#20787=CARTESIAN_POINT ( 'NONE',  ( -1.598721155459999993E-13, 1416.913060387330006, 219.9105610086979823 ) ) ;
#20789=CARTESIAN_POINT ( 'NONE',  ( -15.24410741409210068, 1496.414356836550041, 193.0361994402150003 ) ) ;
#20790=CARTESIAN_POINT ( 'NONE',  ( -31.26311019219999565, 1465.876731228030167, 269.3319192047979982 ) ) ;
#20792=CARTESIAN_POINT ( 'NONE',  ( 18.89959452430000297, 1416.839692140529905, 210.6687134580079999 ) ) ;
#20793=CARTESIAN_POINT ( 'NONE',  ( -28.18475952270000207, 1509.897293877830180, 212.1715675502779845 ) ) ;
#20798=CARTESIAN_POINT ( 'NONE',  ( 14.58371298189999976, 1474.172472513229877, 223.7721885321980153 ) ) ;
#20800=CIRCLE ( 'NONE', #97710, 2.000003390274323500 ) ;
#20801=B_SPLINE_CURVE_WITH_KNOTS ( 'NONE', 3,
 ( #46305, #28928, #21597, #63118, #88278, #89377 ),
 .UNSPECIFIED., .F., .F.,
 ( 4, 2, 4 ),
 ( -0.03349458847672189682, -0.01726308003882509948, -1.826968507034898437E-10 ),
 .UNSPECIFIED. ) ;
#20802=CARTESIAN_POINT ( 'NONE',  ( 17.88592295531849885, 1419.953674261470042, 224.4724256833490017 ) ) ;
#20806=CARTESIAN_POINT ( 'NONE',  ( -13.70491633070000148, 1508.146349234029913, 184.2330007275980108 ) ) ;
#20809=CARTESIAN_POINT ( 'NONE',  ( -12.54563646380000108, 1416.254459047329874, 194.9661771226980136 ) ) ;
#20810=DIRECTION ( 'NONE',  ( -1.000000000000000000, 0.000000000000000000, 0.000000000000000000 ) ) ;
#20811=CARTESIAN_POINT ( 'NONE',  ( 23.89076625480000260, 1410.242936702429915, 209.5801481993979962 ) ) ;
#20812=CARTESIAN_POINT ( 'NONE',  ( -11.99985923319999870, 1433.681662988860126, 149.8469377335979971 ) ) ;
#20814=CARTESIAN_POINT ( 'NONE',  ( -15.52116303490000071, 1422.636867011229924, 228.4575560400980123 ) ) ;
#20815=CARTESIAN_POINT ( 'NONE',  ( -11.77285519380000167, 1432.580890241690213, 150.8112885044980089 ) ) ;
#20816=CARTESIAN_POINT ( 'NONE',  ( -11.70591916684050027, 1426.716063593939907, 141.9425537506020021 ) ) ;
#20821=EDGE_CURVE ( 'NONE', #7200, #61381, #85523, .T. ) ;
#20822=CARTESIAN_POINT ( 'NONE',  ( -28.15442856212169787, 1509.896234822020006, 200.8410265843269826 ) ) ;
#20824=B_SPLINE_CURVE_WITH_KNOTS ( 'NONE', 5,
 ( #85525, #1559, #25618, #60925, #93383, #41889, #50847, #1014, #9391 ),
 .UNSPECIFIED., .F., .F.,
 ( 6, 3, 6 ),
 ( 0.000000000000000000, 0.5000000000000000000, 1.000000000000000000 ),
 .UNSPECIFIED. ) ;
#20827=CARTESIAN_POINT ( 'NONE',  ( -16.69587879669180097, 1485.679718023270198, 187.8645734870310093 ) ) ;
#20830=CARTESIAN_POINT ( 'NONE',  ( -4.265900750095979355, 1441.170003579950162, 158.5225822146180121 ) ) ;
#20834=CARTESIAN_POINT ( 'NONE',  ( 29.36446925850000156, 1509.951008955230009, 212.6618214604380057 ) ) ;
#20835=EDGE_LOOP ( 'NONE', ( #95356, #68801, #77211, #38473, #17226 ) ) ;
#20838=FACE_OUTER_BOUND ( 'NONE', #57123, .T. ) ;
#20839=CARTESIAN_POINT ( 'NONE',  ( 1.476968277879999958, 1508.190462730230138, 180.8898692100979986 ) ) ;
#20840=CARTESIAN_POINT ( 'NONE',  ( 11.88140585900000090, 1433.447543843229823, 147.6490162021979984 ) ) ;
#20841=CARTESIAN_POINT ( 'NONE',  ( -25.81326821525899717, 1450.788444190880000, 136.8507296241930078 ) ) ;
#20843=CARTESIAN_POINT ( 'NONE',  ( 2.760778140020000215, 1409.009468884330090, 230.1977480460979848 ) ) ;
#20846=CARTESIAN_POINT ( 'NONE',  ( 38.86831401555139820, 1437.615293293499690, 134.0999999973729757 ) ) ;
#20852=ORIENTED_EDGE ( 'NONE', *, *, #19527, .T. ) ;
#20857=CARTESIAN_POINT ( 'NONE',  ( 11.19501794742983058, 1451.281070894506001, 151.7798007822887882 ) ) ;
#20860=VECTOR ( 'NONE', #24631, 1000.000000000000000 ) ;
#20861=DIRECTION ( 'NONE',  ( 0.000000000000000000, -1.000000000000000000, 0.000000000000000000 ) ) ;
#20864=CARTESIAN_POINT ( 'NONE',  ( -0.7373154782470000557, 1497.695374981930172, 231.4735153508979977 ) ) ;
#20870=CARTESIAN_POINT ( 'NONE',  ( 26.99384459419149707, 1440.913060387330006, 245.0106952250010011 ) ) ;
#20874=CARTESIAN_POINT ( 'NONE',  ( -15.94346743280000034, 1409.469818538429990, 192.9752478756980167 ) ) ;
#20875=CARTESIAN_POINT ( 'NONE',  ( -23.42267282419999930, 1430.824224223030114, 212.0368849767579889 ) ) ;
#20876=CARTESIAN_POINT ( 'NONE',  ( -24.67251852870000306, 1441.156518004890131, 210.6924577872079851 ) ) ;
#20877=CARTESIAN_POINT ( 'NONE',  ( -1.058602696091491602, 1414.913060387330006, 225.4991512363474726 ) ) ;
#20880=CARTESIAN_POINT ( 'NONE',  ( -3.567500082150000029, 1508.690877485930059, 180.4371975227980158 ) ) ;
#20881=CARTESIAN_POINT ( 'NONE',  ( -27.67757344910459949, 1441.322428384430168, 137.2891306214100098 ) ) ;
#20883=CARTESIAN_POINT ( 'NONE',  ( 7.819645599040000228, 1463.567355340829863, 234.8427059997979995 ) ) ;
#20888=CARTESIAN_POINT ( 'NONE',  ( 19.30664356132462700, 1442.871878066172258, 213.0659908379712704 ) ) ;
#20890=CARTESIAN_POINT ( 'NONE',  ( -19.64184507200000240, 1452.819461536229937, 209.3501247966860035 ) ) ;
#20895=CARTESIAN_POINT ( 'NONE',  ( 4.387875208460000565, 1463.596605969929897, 232.0486588174979943 ) ) ;
#20898=CARTESIAN_POINT ( 'NONE',  ( 2.189642700659999885, 1414.529581730530026, 232.0476498270979846 ) ) ;
#20900=CARTESIAN_POINT ( 'NONE',  ( -24.24300079589999868, 1470.078714870129943, 216.9670906892179971 ) ) ;
#20901=CARTESIAN_POINT ( 'NONE',  ( 2.500000000000000000, 1432.320537255040108, 157.4939813259980212 ) ) ;
#20907=CARTESIAN_POINT ( 'NONE',  ( 0.7745009778729999850, 1406.071044366729893, 269.0454658058980044 ) ) ;
#20909=CARTESIAN_POINT ( 'NONE',  ( 44.93138632836440394, 1446.458187732969918, 269.6837875076539603 ) ) ;
#20911=CARTESIAN_POINT ( 'NONE',  ( 11.60004869885203682, 1422.586092030433520, 135.6000000024070573 ) ) ;
#20912=EDGE_CURVE ( 'NONE', #49524, #95045, #83934, .T. ) ;
#20914=CARTESIAN_POINT ( 'NONE',  ( -1.971747436821430055, 1450.333125910620083, 155.0636771872389943 ) ) ;
#20915=CARTESIAN_POINT ( 'NONE',  ( 4.219439013950669448, 1441.595895969210005, 182.7715284958480026 ) ) ;
#20918=CIRCLE ( 'NONE', #97893, 1.999999999999967359 ) ;
#20919=CARTESIAN_POINT ( 'NONE',  ( -13.98791200573939975, 1415.441076448560125, 220.9116194232070143 ) ) ;
#20920=DIRECTION ( 'NONE',  ( 1.000000000000000000, 0.000000000000000000, 0.000000000000000000 ) ) ;
#20922=CARTESIAN_POINT ( 'NONE',  ( -17.87874069189999915, 1415.075539390429867, 265.6112251771979800 ) ) ;
#20924=CARTESIAN_POINT ( 'NONE',  ( -0.8893057567669999663, 1476.070256768630088, 267.5368301733980161 ) ) ;
#20925=CARTESIAN_POINT ( 'NONE',  ( -16.66101146819999812, 1410.867390116229899, 191.7375337716979971 ) ) ;
#20929=AXIS2_PLACEMENT_3D ( 'NONE', #5536, #30167, #63807 ) ;
#20934=CARTESIAN_POINT ( 'NONE',  ( -5.043610348250129327, 1396.089187143350046, 218.9331246055930080 ) ) ;
#20936=CARTESIAN_POINT ( 'NONE',  ( -15.64557667610000102, 1421.345166096630010, 227.1284468425980094 ) ) ;
#20937=CARTESIAN_POINT ( 'NONE',  ( -45.63153662610000083, 1440.326745910319914, 268.9749020108980062 ) ) ;
#20938=EDGE_LOOP ( 'NONE', ( #97808, #48348, #76472, #102548 ) ) ;
#20941=CARTESIAN_POINT ( 'NONE',  ( -14.59646112059999901, 1484.617543311429927, 186.9027180520979812 ) ) ;
#20942=CARTESIAN_POINT ( 'NONE',  ( 11.51723948480000104, 1426.416094619729847, 128.4916607458980309 ) ) ;
#20944=CARTESIAN_POINT ( 'NONE',  ( 5.402232622379999017E-16, 1413.913060387330006, 209.1218459616979999 ) ) ;
#20948=CIRCLE ( 'NONE', #87073, 31.41749213351482695 ) ;
#20949=CARTESIAN_POINT ( 'NONE',  ( -4.897375497219999652, 1432.353341358199941, 150.0655110971979980 ) ) ;
#20951=DIRECTION ( 'NONE',  ( 0.000000000000000000, 1.000000000000000000, 0.000000000000000000 ) ) ;
#20953=ADVANCED_FACE ( 'NONE', ( #88176 ), #81082, .F. ) ;
#20958=CARTESIAN_POINT ( 'NONE',  ( -5.343479920809999228, 1396.099658817930049, 199.4684377758579785 ) ) ;
#20959=CARTESIAN_POINT ( 'NONE',  ( -14.33393486070000122, 1409.413612422530150, 192.0174323315980018 ) ) ;
#20960=CARTESIAN_POINT ( 'NONE',  ( 6.940379574320000522, 1431.113060387329824, 226.8285010592979916 ) ) ;
#20963=CARTESIAN_POINT ( 'NONE',  ( -1.366316002913839922, 1417.860790559529960, 185.2850244214669999 ) ) ;
#20966=CARTESIAN_POINT ( 'NONE',  ( -40.24076440061289617, 1444.613910935890090, 137.0282073429019931 ) ) ;
#20968=CARTESIAN_POINT ( 'NONE',  ( 37.07887392490540179, 1437.327007662029928, 136.4872220464899897 ) ) ;
#20969=CARTESIAN_POINT ( 'NONE',  ( 6.014260514953510217, 1396.123082992429772, 218.3773295970819959 ) ) ;
#20970=CARTESIAN_POINT ( 'NONE',  ( 33.91375829818579746, 1435.681794709440055, 135.0664790576290102 ) ) ;
#20971=CARTESIAN_POINT ( 'NONE',  ( -1.514297760018489925, 1406.518541415770187, 269.4982389579009805 ) ) ;
#20977=EDGE_LOOP ( 'NONE', ( #101128, #48979, #45262, #56260 ) ) ;
#20979=CARTESIAN_POINT ( 'NONE',  ( -13.73081170289999875, 1460.732406911229873, 231.6108505850980066 ) ) ;
#20984=CARTESIAN_POINT ( 'NONE',  ( -5.947813039672949387, 1509.175827024919954, 179.7301802773710051 ) ) ;
#20987=CARTESIAN_POINT ( 'NONE',  ( 2.525974529359999998, 1414.913060387329779, 224.9911480561979999 ) ) ;
#20989=CARTESIAN_POINT ( 'NONE',  ( -28.25086440149999945, 1508.135696992230123, 208.8579908607459856 ) ) ;
#20991=CARTESIAN_POINT ( 'NONE',  ( -4.934427622899999477, 1409.085374397729993, 230.8376437965980301 ) ) ;
#20992=CARTESIAN_POINT ( 'NONE',  ( -11.34090880850000005, 1475.513060387329915, 191.0454207575980092 ) ) ;
#20994=DIRECTION ( 'NONE',  ( 0.000000000000000000, 0.000000000000000000, -1.000000000000000000 ) ) ;
#20995=CARTESIAN_POINT ( 'NONE',  ( 1.719367447207400090, 1490.891747713500081, 235.7942165085109991 ) ) ;
#20998=CARTESIAN_POINT ( 'NONE',  ( 17.04824238339829634, 1423.676546790900147, 228.9394188427949928 ) ) ;
#20999=CARTESIAN_POINT ( 'NONE',  ( 20.84494148150000115, 1411.509465946430055, 270.2130226657980074 ) ) ;
#21003=CARTESIAN_POINT ( 'NONE',  ( 23.61592788680000154, 1410.127845046630227, 208.5598851522910024 ) ) ;
#21004=CARTESIAN_POINT ( 'NONE',  ( 0.02005075328566424328, 1507.220604446680682, 237.3599021426030049 ) ) ;
#21009=CARTESIAN_POINT ( 'NONE',  ( 4.308397161744589532, 1421.939254178800184, 184.0347638950579778 ) ) ;
#21010=CARTESIAN_POINT ( 'NONE',  ( -1.314354605479999938, 1420.453030399730096, 233.4140791911979989 ) ) ;
#21014=CARTESIAN_POINT ( 'NONE',  ( -10.81518740880000173, 1424.921099675630103, 144.1705347734979910 ) ) ;
#21015=CARTESIAN_POINT ( 'NONE',  ( -20.81060428327939960, 1508.370615559120097, 228.0279630968090032 ) ) ;
#21018=CARTESIAN_POINT ( 'NONE',  ( -0.03430450970949740219, 1420.445176861049958, 182.6785821352689823 ) ) ;
#21021=CARTESIAN_POINT ( 'NONE',  ( 18.63787275289999812, 1508.244465050629969, 188.4525138200980052 ) ) ;
#21026=DIRECTION ( 'NONE',  ( 9.970439643713600747E-17, 0.7071067811865474617, 0.7071067811865474617 ) ) ;
#21029=CARTESIAN_POINT ( 'NONE',  ( 9.952822627054100479, 1435.746504192841257, 152.5237976836565679 ) ) ;
#21033=CARTESIAN_POINT ( 'NONE',  ( 16.42688314034032260, 1421.633920429433374, 227.1747839813914140 ) ) ;
#21034=CARTESIAN_POINT ( 'NONE',  ( -4.220927954649999592, 1446.217199771449941, 167.4561887392980282 ) ) ;
#21035=CARTESIAN_POINT ( 'NONE',  ( -20.26420847629999855, 1427.565864917729868, 222.2644582469980037 ) ) ;
#21036=CARTESIAN_POINT ( 'NONE',  ( -15.23375471800000014, 1435.180443442269961, 148.6429311973979850 ) ) ;
#21038=CARTESIAN_POINT ( 'NONE',  ( 16.93884269750000016, 1507.634939773729911, 188.0954309116980028 ) ) ;
#21039=CARTESIAN_POINT ( 'NONE',  ( 0.5624690339869999889, 1416.828040475229955, 190.4759594386979984 ) ) ;
#21043=CARTESIAN_POINT ( 'NONE',  ( -19.34729233231120205, 1486.470064436709890, 189.5887045964369975 ) ) ;
#21046=CARTESIAN_POINT ( 'NONE',  ( 11.81135191919999983, 1436.410413307749877, 147.6956600043980075 ) ) ;
#21050=FACE_OUTER_BOUND ( 'NONE', #3545, .T. ) ;
#21052=CARTESIAN_POINT ( 'NONE',  ( 20.80119636470000088, 1475.513060387329915, 213.8845752798079900 ) ) ;
#21057=EDGE_CURVE ( 'NONE', #25318, #47913, #49254, .T. ) ;
#21059=CARTESIAN_POINT ( 'NONE',  ( -6.896890933126118993E-05, 1408.913065613199933, 231.7784170915439859 ) ) ;
#21060=CARTESIAN_POINT ( 'NONE',  ( 22.24498329749999925, 1508.411266897830046, 192.4020607342980043 ) ) ;
#21064=ADVANCED_FACE ( 'NONE', ( #79783 ), #102418, .F. ) ;
#21065=ORIENTED_EDGE ( 'NONE', *, *, #93835, .T. ) ;
#21066=ORIENTED_EDGE ( 'NONE', *, *, #53596, .T. ) ;
#21068=FACE_OUTER_BOUND ( 'NONE', #7180, .T. ) ;
#21070=CARTESIAN_POINT ( 'NONE',  ( 29.59289186111734793, 1419.279954201788541, 269.4665317194949239 ) ) ;
#21071=CARTESIAN_POINT ( 'NONE',  ( 1.874402367650000219E-09, 1463.532726170529941, 231.7907868339979984 ) ) ;
#21072=CARTESIAN_POINT ( 'NONE',  ( -20.18744379279999990, 1494.501811925929815, 190.4612313790980238 ) ) ;
#21074=CARTESIAN_POINT ( 'NONE',  ( -11.92399326099999968, 1433.494514533970005, 150.2018804083979830 ) ) ;
#21075=CARTESIAN_POINT ( 'NONE',  ( 27.34966551919999844, 1509.645409999729964, 203.9598639501480193 ) ) ;
#21076=CARTESIAN_POINT ( 'NONE',  ( -18.96987419410000086, 1486.105584072130114, 189.3878642699980048 ) ) ;
#21083=CARTESIAN_POINT ( 'NONE',  ( -13.18094245060510517, 1509.496846870918034, 236.0820355107387627 ) ) ;
#21084=CARTESIAN_POINT ( 'NONE',  ( 1.582871032461760074E-08, 1407.860659628199983, 263.2896717771570252 ) ) ;
#21085=ORIENTED_EDGE ( 'NONE', *, *, #22808, .F. ) ;
#21088=AXIS2_PLACEMENT_3D ( 'NONE', #53109, #87246, #47865 ) ;
#21090=CARTESIAN_POINT ( 'NONE',  ( -29.04152419889999948, 1466.259437530530022, 270.1335450958980005 ) ) ;
#21091=CARTESIAN_POINT ( 'NONE',  ( -23.93572934907803784, 1435.909525931274629, 211.2608146398322333 ) ) ;
#21095=CARTESIAN_POINT ( 'NONE',  ( -12.81872062859999950, 1420.998869512129886, 230.6915806954980042 ) ) ;
#21096=CARTESIAN_POINT ( 'NONE',  ( 20.86040077215431410, 1508.959081887785487, 227.6602567278162041 ) ) ;
#21097=CARTESIAN_POINT ( 'NONE',  ( -1.185300654861193514, 1484.701227333132692, 182.2327694872268182 ) ) ;
#21099=CARTESIAN_POINT ( 'NONE',  ( -45.70040227590190085, 1436.740216172639975, 268.5066267783719809 ) ) ;
#21100=ORIENTED_EDGE ( 'NONE', *, *, #41168, .F. ) ;
#21101=CARTESIAN_POINT ( 'NONE',  ( -3.532157406807699740, 1490.686494827730030, 181.6769642933810189 ) ) ;
#21103=EDGE_LOOP ( 'NONE', ( #23897, #57997, #56545, #2625 ) ) ;
#21106=VECTOR ( 'NONE', #574, 1000.000000000000114 ) ;
#21107=CARTESIAN_POINT ( 'NONE',  ( -21.92450687779999896, 1509.678681038230025, 190.3751805934979870 ) ) ;
#21108=DIRECTION ( 'NONE',  ( -0.2857341017153708362, -0.9583089392864680978, -7.447054303646096154E-07 ) ) ;
#21109=CARTESIAN_POINT ( 'NONE',  ( -16.45911293875139592, 1470.466665006630137, 228.6107017031530120 ) ) ;
#21110=ORIENTED_EDGE ( 'NONE', *, *, #55628, .F. ) ;
#21112=CARTESIAN_POINT ( 'NONE',  ( 18.46505084572267563, 1509.557874171173125, 187.1463136620376702 ) ) ;
#21115=CARTESIAN_POINT ( 'NONE',  ( -8.488567187765550415, 1409.798321788380008, 270.3692809364429763 ) ) ;
#21116=CARTESIAN_POINT ( 'NONE',  ( -33.91369110859999836, 1435.681798638700002, 135.0664268289980043 ) ) ;
#21121=CARTESIAN_POINT ( 'NONE',  ( 42.04647649369601936, 1454.209662175047924, 269.0745616169903656 ) ) ;
#21123=CARTESIAN_POINT ( 'NONE',  ( -13.87677329403120119, 1436.230442017350015, 150.3050677568869844 ) ) ;
#21124=CARTESIAN_POINT ( 'NONE',  ( -0.03489894090345890126, 1409.380919406509975, 185.4002601856399792 ) ) ;
#21125=LINE ( 'NONE', #3283, #80554 ) ;
#21126=CARTESIAN_POINT ( 'NONE',  ( -18.72553219700000326, 1435.775956364280091, 225.5898836715979883 ) ) ;
#21127=CARTESIAN_POINT ( 'NONE',  ( 15.79272951203170017, 1474.038596115399969, 268.9599971491709880 ) ) ;
#21128=CARTESIAN_POINT ( 'NONE',  ( -1.500739301586951013, 1467.017219971860868, 235.3803771181077593 ) ) ;
#21129=CARTESIAN_POINT ( 'NONE',  ( 7.158636770289999340, 1447.499260772210164, 185.4013549890980244 ) ) ;
#21132=CARTESIAN_POINT ( 'NONE',  ( -38.81202642568430150, 1450.612734564189850, 135.0584858587309895 ) ) ;
#21133=CARTESIAN_POINT ( 'NONE',  ( -12.93261306534080113, 1416.826860677879949, 196.5036138660090046 ) ) ;
#21137=CARTESIAN_POINT ( 'NONE',  ( 14.23393746390000025, 1416.021639799829927, 196.8145123778979837 ) ) ;
#21139=CARTESIAN_POINT ( 'NONE',  ( 19.18632316300000085, 1409.583061558729923, 197.9438956507979981 ) ) ;
#21140=CARTESIAN_POINT ( 'NONE',  ( 22.74352444629999681, 1409.874439160429802, 207.7226808069280253 ) ) ;
#21141=CARTESIAN_POINT ( 'NONE',  ( -23.61227025210000008, 1435.322036687620084, 137.2858276859979867 ) ) ;
#21142=CARTESIAN_POINT ( 'NONE',  ( -24.45428651019999933, 1432.411055651390143, 210.5059752880879955 ) ) ;
#21143=CARTESIAN_POINT ( 'NONE',  ( 0.3740290774567820442, 1452.976564944560096, 183.2744728122640083 ) ) ;
#21149=B_SPLINE_SURFACE_WITH_KNOTS ( 'NONE', 5, 5, ( 
 ( #100217, #82856, #6145, #74486, #44184, #27365 ),
 ( #18390, #104627, #96230, #103511, #2750, #53141 ),
 ( #60438, #62106, #87279, #43628, #36315, #78324 ),
 ( #45298, #51466, #27924, #94556, #36870, #79438 ),
 ( #8898, #19507, #17829, #102949, #537, #53712 ),
 ( #77776, #26814, #70512, #9463, #87850, #1636 ),
 ( #52588, #1088, #71064, #35773, #35214, #69400 ),
 ( #61002, #62671, #95128, #28478, #17275, #18946 ),
 ( #26250, #10574, #86721, #86170, #85598, #43076 ),
 ( #69956, #68845, #10014, #61547, #44745, #104070 ),
 ( #105186, #77236, #95678, #11138, #78895, #2201 ),
 ( #34661, #52034, #72163, #3854, #106817, #98968 ),
 ( #72694, #88382, #22242, #29033, #71629, #79981 ),
 ( #37981, #46406, #106280, #4916, #88925, #39055 ),
 ( #13850, #21139, #12211, #48034, #12775, #80539 ),
 ( #29566, #63750, #31222, #97864, #107929, #96792 ),
 ( #20062, #105749, #98423, #55346, #54793, #54256 ),
 ( #107378, #38515, #37431, #89480, #30108, #90019 ),
 ( #21695, #82172, #11672, #46952, #56440, #81072 ),
 ( #13296, #4387, #64303, #55901, #47489, #81612 ),
 ( #30673, #90571, #45848, #5472, #73235, #3300 ) ),
 .UNSPECIFIED., .F., .F., .F.,
 ( 6, 3, 3, 3, 3, 3, 6 ),
 ( 6, 6 ),
 ( 29.50806686130000145, 31.51384161189999844, 32.22913687700000196, 33.93149951750000071, 35.63386215799999945, 39.03858743909999873, 48.56910801690000312 ),
 ( 0.000000000000000000, 1.468540379180000022 ),
 .UNSPECIFIED. ) ;
#21152=DIRECTION ( 'NONE',  ( 0.000000000000000000, 0.000000000000000000, -1.000000000000000000 ) ) ;
#21154=CARTESIAN_POINT ( 'NONE',  ( -5.553848058839999879, 1423.191816860230119, 91.03168606369779070 ) ) ;
#21155=CARTESIAN_POINT ( 'NONE',  ( -40.14605221587299155, 1445.134064018490108, 136.9416851659559882 ) ) ;
#21156=CARTESIAN_POINT ( 'NONE',  ( 11.60004869885203682, 1425.984133098859502, 137.6624196891229133 ) ) ;
#21157=CARTESIAN_POINT ( 'NONE',  ( 2.108904356780865186, 1417.396421507168725, 233.2477812154150172 ) ) ;
#21158=CARTESIAN_POINT ( 'NONE',  ( -1.929425373146870015, 1464.862440756950264, 183.7962778897980058 ) ) ;
#21160=CARTESIAN_POINT ( 'NONE',  ( -10.16997697100000053, 1474.408914113430001, 269.6186555620979561 ) ) ;
#21161=CARTESIAN_POINT ( 'NONE',  ( 29.33985996377240113, 1440.913060386940060, 236.1580507230389969 ) ) ;
#21164=ORIENTED_EDGE ( 'NONE', *, *, #109564, .T. ) ;
#21167=CARTESIAN_POINT ( 'NONE',  ( 1.834068947563254337, 1397.968134176382819, 196.2250787140935699 ) ) ;
#21168=CARTESIAN_POINT ( 'NONE',  ( 2.894887617429999782, 1490.918242441229950, 235.2239209075980000 ) ) ;
#21169=AXIS2_PLACEMENT_3D ( 'NONE', #86669, #27317, #95628 ) ;
#21171=CARTESIAN_POINT ( 'NONE',  ( -12.44137076039999990, 1509.176489603729806, 234.5038223836979796 ) ) ;
#21174=CARTESIAN_POINT ( 'NONE',  ( 2.499942005323459782, 1419.859829899919987, 115.5959393205330059 ) ) ;
#21175=CARTESIAN_POINT ( 'NONE',  ( 2.684660662710000256, 1464.593469353430010, 236.4393482303979965 ) ) ;
#21178=CARTESIAN_POINT ( 'NONE',  ( -1.406481360810000192, 1450.686779281020108, 182.3753173715980154 ) ) ;
#21185=VERTEX_POINT ( 'NONE', #25339 ) ;
#21189=CARTESIAN_POINT ( 'NONE',  ( -11.60004869885204215, 1426.273944179774844, 138.2686100621498326 ) ) ;
#21192=CARTESIAN_POINT ( 'NONE',  ( 4.580542335331530879, 1409.073016450339992, 194.8569092263689981 ) ) ;
#21197=B_SPLINE_CURVE_WITH_KNOTS ( 'NONE', 3,
 ( #69602, #95325, #37069, #96991, #52782, #86918, #10210, #56633, #99706, #72885, #82921, #23561, #30312, #38709, #65593, #39825, #47680, #48799, #21880, #66160, #80731, #91327, #6213, #5681, #12412, #108677, #81260, #14050, #13490, #107574, #64501, #106477, #40364, #100281, #89124, #38167, #30860 ),
 .UNSPECIFIED., .F., .F.,
 ( 4, 3, 3, 3, 3, 3, 3, 3, 3, 3, 3, 3, 4 ),
 ( -1.999999848858570184, -1.897891335478260055, -1.728761196501279906, -1.557452151978439892, -1.384905003028850112, -1.210695231704240094, -1.035838572815900083, -0.8607549783656509579, -0.6858798835383781434, -0.5121999524719260677, -0.3398111961833858441, -0.1690102497754839561, -5.802412736954920547E-06 ),
 .UNSPECIFIED. ) ;
#21198=CARTESIAN_POINT ( 'NONE',  ( -2.560277166941169913, 1449.672157588639948, 183.8693981670420214 ) ) ;
#21200=VERTEX_POINT ( 'NONE', #48381 ) ;
#21205=CARTESIAN_POINT ( 'NONE',  ( -20.39295167552050003, 1501.158379912629925, 190.5839871636399891 ) ) ;
#21206=CARTESIAN_POINT ( 'NONE',  ( -5.393559028770000581E-12, 1395.913060387330006, 220.1216245191979795 ) ) ;
#21208=CARTESIAN_POINT ( 'NONE',  ( -1.184997839870000069, 1455.069883079229839, 183.4791223000979983 ) ) ;
#21210=CARTESIAN_POINT ( 'NONE',  ( -26.34474851411561147, 1436.712219889005382, 136.8403030806463505 ) ) ;
#21214=CARTESIAN_POINT ( 'NONE',  ( 11.59211330538789930, 1433.842074355000022, 151.2028293458270127 ) ) ;
#21216=CARTESIAN_POINT ( 'NONE',  ( -13.13217473943669944, 1436.055352265540023, 150.6849122874139937 ) ) ;
#21221=ORIENTED_EDGE ( 'NONE', *, *, #9062, .F. ) ;
#21222=AXIS2_PLACEMENT_3D ( 'NONE', #16598, #102825, #84927 ) ;
#21223=CARTESIAN_POINT ( 'NONE',  ( 5.301749018989998952, 1413.741945239130018, 248.5896189552980218 ) ) ;
#21224=CARTESIAN_POINT ( 'NONE',  ( -24.64286055450000035, 1488.680273902429917, 199.5172922023679973 ) ) ;
#21225=CARTESIAN_POINT ( 'NONE',  ( -10.41164713266690001, 1425.393357077480005, 96.73048425825258789 ) ) ;
#21226=CARTESIAN_POINT ( 'NONE',  ( 2.956412232989999457E-14, 1420.418457356630142, 243.9198229339980060 ) ) ;
#21228=CARTESIAN_POINT ( 'NONE',  ( 18.72196290327717705, 1507.117986391379645, 196.2613482712523592 ) ) ;
#21229=CARTESIAN_POINT ( 'NONE',  ( 1.630039620769999944E-09, 1416.130848190830193, 240.4142140047979694 ) ) ;
#21231=CARTESIAN_POINT ( 'NONE',  ( 0.8007374150823964865, 1415.525414496541998, 233.2555237395259269 ) ) ;
#21232=CARTESIAN_POINT ( 'NONE',  ( 29.25358229339999738, 1451.890933296829871, 135.2860531028979949 ) ) ;
#21233=VERTEX_POINT ( 'NONE', #25894 ) ;
#21234=CARTESIAN_POINT ( 'NONE',  ( -0.06016863597635770111, 1397.283821687630052, 196.1836521277020040 ) ) ;
#21240=CARTESIAN_POINT ( 'NONE',  ( -24.10461029974740299, 1411.115259933990046, 208.6981664729640045 ) ) ;
#21241=ORIENTED_EDGE ( 'NONE', *, *, #5496, .T. ) ;
#21244=CARTESIAN_POINT ( 'NONE',  ( -7.416235415360000083, 1489.056178334129982, 234.6541755130980107 ) ) ;
#21248=CARTESIAN_POINT ( 'NONE',  ( 46.02990061730259441, 1440.912967656690171, 268.4960838911439964 ) ) ;
#21251=CARTESIAN_POINT ( 'NONE',  ( 0.1168360841530000083, 1420.456612005029911, 182.7029863163980110 ) ) ;
#21255=EDGE_CURVE ( 'NONE', #49156, #5142, #67606, .T. ) ;
#21256=CARTESIAN_POINT ( 'NONE',  ( 13.05663714242001028, 1442.990000998531968, 187.2968644710537660 ) ) ;
#21261=DIRECTION ( 'NONE',  ( -0.7071067811865475727, 0.000000000000000000, 0.7071067811865475727 ) ) ;
#21262=CARTESIAN_POINT ( 'NONE',  ( -18.33789049558490092, 1409.553433634309840, 198.1058259467170046 ) ) ;
#21266=DIRECTION ( 'NONE',  ( -0.1115146105487929418, 0.9937625046796735306, 0.0007588984999193657075 ) ) ;
#21270=CARTESIAN_POINT ( 'NONE',  ( 3.827327205999999649, 1409.546157813730133, 146.1721969590979882 ) ) ;
#21271=CARTESIAN_POINT ( 'NONE',  ( 0.03003581927826226919, 1409.173052036745048, 232.6080437499834943 ) ) ;
#21273=CARTESIAN_POINT ( 'NONE',  ( -19.06723915664710134, 1485.490521620860136, 189.6150037022410118 ) ) ;
#21276=CARTESIAN_POINT ( 'NONE',  ( -25.07152577354069933, 1509.629181063510032, 222.8076647697269834 ) ) ;
#21279=ORIENTED_EDGE ( 'NONE', *, *, #77433, .T. ) ;
#21280=CARTESIAN_POINT ( 'NONE',  ( 23.42675388089999799, 1438.250513043230058, 234.3916895697979612 ) ) ;
#21283=B_SPLINE_SURFACE_WITH_KNOTS ( 'NONE', 5, 5, ( 
 ( #45782, #3230, #44669, #37357, #103997, #3781 ),
 ( #27294, #97797, #21075, #12145, #71558, #19431 ),
 ( #89410, #28961, #63150, #78810, #80466, #97250 ),
 ( #37913, #104556, #53068, #20526, #87205, #29491 ),
 ( #63686, #12698, #35691, #95602, #69881, #18870 ),
 ( #53632, #2125, #70437, #27851, #45226, #62032 ) ),
 .UNSPECIFIED., .F., .F., .F.,
 ( 6, 6 ),
 ( 6, 6 ),
 ( 57.19174229819999766, 70.68201800039999227 ),
 ( 0.000000000000000000, 2.000000000000000000 ),
 .UNSPECIFIED. ) ;
#21288=ORIENTED_EDGE ( 'NONE', *, *, #66459, .T. ) ;
#21292=CARTESIAN_POINT ( 'NONE',  ( -13.79590941699999895, 1416.844618638129987, 221.9094009297979824 ) ) ;
#21298=CARTESIAN_POINT ( 'NONE',  ( -13.46280551501950029, 1426.665735440540175, 222.2126077582630046 ) ) ;
#21299=EDGE_CURVE ( 'NONE', #82900, #83651, #56091, .T. ) ;
#21300=CARTESIAN_POINT ( 'NONE',  ( 12.71163532969999821, 1422.101025195029933, 229.2301305095980126 ) ) ;
#21301=CARTESIAN_POINT ( 'NONE',  ( -0.5697989934050000649, 1450.893162568020216, 169.5117309619979835 ) ) ;
#21303=CARTESIAN_POINT ( 'NONE',  ( 41.54683551029999222, 1425.087414133530046, 267.1293096718979427 ) ) ;
#21304=CARTESIAN_POINT ( 'NONE',  ( -18.40570622650000132, 1410.918580325929952, 224.0732781207979940 ) ) ;
#21305=CARTESIAN_POINT ( 'NONE',  ( 17.03727604480000224, 1436.327040906540105, 148.1886016197979927 ) ) ;
#21307=EDGE_CURVE ( 'NONE', #47741, #104308, #15676, .T. ) ;
#21309=CARTESIAN_POINT ( 'NONE',  ( -17.00536272201560095, 1410.873511664369744, 191.9510081054149850 ) ) ;
#21311=CARTESIAN_POINT ( 'NONE',  ( 12.27023112300000030, 1416.839692131129823, 223.5796784315980119 ) ) ;
#21312=CARTESIAN_POINT ( 'NONE',  ( 13.15726396704670087, 1415.954755714380099, 198.0473975409559841 ) ) ;
#21313=CARTESIAN_POINT ( 'NONE',  ( -37.80877602953309946, 1438.319709222639858, 136.5786655222570118 ) ) ;
#21314=CARTESIAN_POINT ( 'NONE',  ( 0.2166443802809689678, 1453.632411855340024, 183.2262637060080124 ) ) ;
#21315=CARTESIAN_POINT ( 'NONE',  ( -13.68698573120000006, 1409.391020461129983, 216.8549264454580054 ) ) ;
#21316=CARTESIAN_POINT ( 'NONE',  ( -12.95840179510000034, 1416.218047894730262, 196.6656609298980243 ) ) ;
#21319=CARTESIAN_POINT ( 'NONE',  ( 12.06118834549999974, 1433.903448631609990, 147.9454112030979900 ) ) ;
#21320=CARTESIAN_POINT ( 'NONE',  ( -38.70428745504600698, 1437.478004126309997, 134.0999999972650016 ) ) ;
#21321=CARTESIAN_POINT ( 'NONE',  ( 11.79755445260000002, 1442.026836458709795, 187.8249092859979896 ) ) ;
#21324=CARTESIAN_POINT ( 'NONE',  ( 39.60771322839999442, 1439.514900260280001, 136.6564050689979979 ) ) ;
#21327=CARTESIAN_POINT ( 'NONE',  ( -13.86457764730300113, 1451.730262176210090, 194.4398952447820079 ) ) ;
#21328=CARTESIAN_POINT ( 'NONE',  ( 1.090037377353519974E-11, 1406.777728848529932, 269.6500679732980075 ) ) ;
#21335=B_SPLINE_CURVE_WITH_KNOTS ( 'NONE', 3,
 ( #76656, #101834, #102398, #25681, #43066, #8334, #67727, #100734, #67174, #24018, #77226, #83394, #110806, #25128, #101273, #6692, #59874, #83949, #34098, #58760, #7249, #34652, #42498, #59331, #92341, #24570, #41411, #68836, #40848, #68291, #26240, #93442, #60429, #94547, #84501, #51457, #75578, #109171, #17820, #75021, #66633, #16711, #32458, #85044, #109710, #32985, #16172, #50375, #7791, #77767, #35763, #36307 ),
 .UNSPECIFIED., .F., .F.,
 ( 4, 2, 2, 1, 1, 2, 2, 2, 1, 1, 1, 2, 2, 2, 2, 1, 1, 1, 2, 2, 2, 2, 1, 1, 1, 2, 2, 1, 1, 1, 2, 2, 4 ),
 ( 0.000000000000000000, 0.06249999999992944533, 0.09374999999989959421, 0.1093749999999656525, 0.1171875000000026784, 0.1210937500000212053, 0.1250000000000397182, 0.1875000000002257361, 0.2187500000004227174, 0.2343750000005219991, 0.2421875000006816214, 0.2460937500006476764, 0.2500000000006137313, 0.3750000000008417711, 0.4375000000009564016, 0.4687500000009153234, 0.4843750000008948398, 0.4921875000008845702, 0.4960937500008881229, 0.5000000000008917311, 0.6250000000009093837, 0.6875000000008434364, 0.7187500000009037215, 0.7343750000010336176, 0.7421875000011902701, 0.7460937500011635137, 0.7500000000011366463, 0.8125000000007555068, 0.8437500000004857226, 0.8593750000003508305, 0.8671875000002831069, 0.8750000000002154943, 1.000000000000000000 ),
 .UNSPECIFIED. ) ;
#21337=FACE_OUTER_BOUND ( 'NONE', #17187, .T. ) ;
#21340=EDGE_LOOP ( 'NONE', ( #55957, #39106, #83633 ) ) ;
#21342=CARTESIAN_POINT ( 'NONE',  ( 1.442193076691909992, 1490.929412776270055, 236.0730353711790031 ) ) ;
#21345=CARTESIAN_POINT ( 'NONE',  ( -12.77587743780000018, 1416.568813547830132, 195.5427461491979955 ) ) ;
#21348=CARTESIAN_POINT ( 'NONE',  ( 21.69405894630000020, 1409.835083189130046, 215.3959610885380016 ) ) ;
#21349=CARTESIAN_POINT ( 'NONE',  ( -2.922656181083440163, 1412.660035859490108, 186.5114004217930130 ) ) ;
#21351=CARTESIAN_POINT ( 'NONE',  ( -5.360299083833290013, 1422.241314829860130, 144.2409028308489667 ) ) ;
#21354=CARTESIAN_POINT ( 'NONE',  ( 24.86506402033909779, 1430.503309461649906, 208.3719473011869923 ) ) ;
#21357=CARTESIAN_POINT ( 'NONE',  ( -1.383935618409999790, 1416.536379228330134, 233.4680935172980014 ) ) ;
#21359=ADVANCED_FACE ( 'NONE', ( #55553 ), #86361, .F. ) ;
#21361=CARTESIAN_POINT ( 'NONE',  ( -4.338088841202789148, 1484.259041794070072, 183.5077872766069902 ) ) ;
#21364=CARTESIAN_POINT ( 'NONE',  ( 18.08041632129999954, 1415.296882296330068, 210.6774151550479814 ) ) ;
#21368=CARTESIAN_POINT ( 'NONE',  ( 29.02287039530000001, 1509.869659243430078, 211.4398731524179880 ) ) ;
#21370=CARTESIAN_POINT ( 'NONE',  ( -24.89939545272470056, 1440.978110083920001, 210.4300214511639808 ) ) ;
#21371=CARTESIAN_POINT ( 'NONE',  ( 1.547463840030000037, 1414.913060387329779, 192.3096136973980208 ) ) ;
#21372=CARTESIAN_POINT ( 'NONE',  ( 15.81261799660090084, 1415.231763502519925, 191.3817023155100117 ) ) ;
#21373=CARTESIAN_POINT ( 'NONE',  ( 0.4819869456859999790, 1507.639374880330024, 180.9399793378979950 ) ) ;
#21376=EDGE_CURVE ( 'NONE', #18619, #90692, #75269, .T. ) ;
#21377=CARTESIAN_POINT ( 'NONE',  ( -25.25219063472429681, 1451.151841954119845, 137.3646034387350028 ) ) ;
#21379=CARTESIAN_POINT ( 'NONE',  ( 2.825023431620000025, 1409.011712379730170, 230.6343984061979882 ) ) ;
#21382=CARTESIAN_POINT ( 'NONE',  ( 39.89055406515740287, 1448.739173192549970, 134.0999999981559938 ) ) ;
#21388=ORIENTED_EDGE ( 'NONE', *, *, #20659, .T. ) ;
#21394=CARTESIAN_POINT ( 'NONE',  ( -3.004397273099999932, 1485.815138895830160, 182.5519705833980026 ) ) ;
#21396=CARTESIAN_POINT ( 'NONE',  ( -17.53521452141892922, 1448.184789224442511, 218.0158466994055857 ) ) ;
#21399=EDGE_CURVE ( 'NONE', #7904, #45774, #49702, .T. ) ;
#21406=CARTESIAN_POINT ( 'NONE',  ( 40.21729846317249724, 1440.913060387330006, 267.6250173488770088 ) ) ;
#21408=CARTESIAN_POINT ( 'NONE',  ( -0.0005665943966642099589, 1451.957582760023797, 153.9843603111906134 ) ) ;
#21412=CARTESIAN_POINT ( 'NONE',  ( -16.40120703590000062, 1409.652464985630104, 192.2255933302979827 ) ) ;
#21413=CARTESIAN_POINT ( 'NONE',  ( -24.35246777550132435, 1439.602140306827550, 212.0316767823215685 ) ) ;
#21416=CARTESIAN_POINT ( 'NONE',  ( 14.57089808959999999, 1407.761835850630177, 266.8771382033980331 ) ) ;
#21418=CARTESIAN_POINT ( 'NONE',  ( 26.21319982379560187, 1493.418275869099944, 206.2276069840760044 ) ) ;
#21419=CARTESIAN_POINT ( 'NONE',  ( 10.17186614039999881, 1464.738249403130112, 232.3595462222980075 ) ) ;
#21422=B_SPLINE_SURFACE_WITH_KNOTS ( 'NONE', 5, 5, ( 
 ( #11583, #27270, #71535, #28378, #61454, #26144 ),
 ( #94452, #62579, #36228, #104533, #27829, #19405 ),
 ( #19968, #2654, #53609, #54162, #17731, #86074 ),
 ( #44214, #86753, #51499, #76695, #35807, #102981 ),
 ( #69989, #78357, #1116, #1666, #53170, #7 ),
 ( #43106, #101874, #50957, #8932, #103546, #85632 ),
 ( #34143, #104104, #95158, #60469, #27393, #26280 ),
 ( #16751, #17866, #87312, #67762, #68327, #102435 ),
 ( #25719, #77265, #94586, #10043, #34690, #77807 ),
 ( #26849, #10605, #44776, #78927, #8373, #564 ),
 ( #35245, #61037, #85084, #59370, #61575, #95708 ),
 ( #18974, #18417, #52065, #33570, #25167, #68880 ) ),
 .UNSPECIFIED., .F., .F., .F.,
 ( 6, 3, 3, 6 ),
 ( 6, 6 ),
 ( 30.85152358798220007, 67.48111802349998811, 89.44935581500000410, 144.2305269969999983 ),
 ( -1.869926188701470044E-05, 0.4689188517720000449 ),
 .UNSPECIFIED. ) ;
#21426=CARTESIAN_POINT ( 'NONE',  ( -0.1361220240859130071, 1507.783361145109893, 180.7555731139599970 ) ) ;
#21427=CARTESIAN_POINT ( 'NONE',  ( 18.42528818938584223, 1446.189480375194762, 215.6021398651423340 ) ) ;
#21431=EDGE_LOOP ( 'NONE', ( #31891, #38636, #12729, #104321 ) ) ;
#21432=DIRECTION ( 'NONE',  ( 0.000000000000000000, 0.000000000000000000, -1.000000000000000000 ) ) ;
#21434=CARTESIAN_POINT ( 'NONE',  ( 19.46363819460000144, 1452.609789409330006, 213.2823703743680142 ) ) ;
#21435=CARTESIAN_POINT ( 'NONE',  ( -11.76946808870000005, 1432.335038318230090, 150.8120985755979859 ) ) ;
#21437=CARTESIAN_POINT ( 'NONE',  ( 1.804219641780000050, 1410.346235427530019, 232.1926713004979774 ) ) ;
#21441=CARTESIAN_POINT ( 'NONE',  ( -21.86656088110000340, 1470.082911937230165, 223.0158589924980106 ) ) ;
#21442=CARTESIAN_POINT ( 'NONE',  ( 2.500000000000000000, 1428.988705744230174, 157.0781314899979861 ) ) ;
#21444=EDGE_LOOP ( 'NONE', ( #61942, #4749, #60805, #21812 ) ) ;
#21446=CARTESIAN_POINT ( 'NONE',  ( 2.744127903880000385, 1406.565768444329933, 269.4960847736980440 ) ) ;
#21449=CARTESIAN_POINT ( 'NONE',  ( 20.32238055547781741, 1427.042525162981065, 220.8319574201998421 ) ) ;
#21450=CARTESIAN_POINT ( 'NONE',  ( -23.84533141485470153, 1452.080363065020038, 136.9869391916130041 ) ) ;
#21451=CARTESIAN_POINT ( 'NONE',  ( 10.85844884284743550, 1424.793770695752301, 138.1921923629704168 ) ) ;
#21455=CARTESIAN_POINT ( 'NONE',  ( -2.493007233162190417, 1449.246563095040074, 154.5202250740130125 ) ) ;
#21456=CARTESIAN_POINT ( 'NONE',  ( -1.589953117590154230, 1450.801901463933291, 183.3727437628812709 ) ) ;
#21457=CARTESIAN_POINT ( 'NONE',  ( 1.177008278681779929, 1450.813907473600011, 155.0627464472840131 ) ) ;
#21458=CARTESIAN_POINT ( 'NONE',  ( -14.14453214052680075, 1415.673583083550056, 221.0709323776389965 ) ) ;
#21461=CARTESIAN_POINT ( 'NONE',  ( -19.46212512329999811, 1433.716220832530098, 224.8635562271979893 ) ) ;
#21462=B_SPLINE_CURVE_WITH_KNOTS ( 'NONE', 3,
 ( #47342, #81469, #29423, #12077, #107239, #20458, #3712, #105606, #38919, #90983, #4773, #29973, #64165, #39492, #71485, #56851, #63622, #73100, #72552, #55770, #89340, #14271, #80943, #30531, #106144, #46270, #73663, #64722, #98838, #22098, #97738, #56297, #89885, #21560, #37294, #72029, #21009, #55211, #88795, #46813 ),
 .UNSPECIFIED., .F., .F.,
 ( 4, 3, 3, 3, 3, 3, 3, 3, 3, 3, 3, 3, 3, 4 ),
 ( -1.999999742213449894, -1.877659734187909990, -1.724846248608389976, -1.569855302308919898, -1.413640332142279910, -1.255656791337570022, -1.096905799826189964, -0.9377556084170080020, -0.7786028042479620215, -0.6202726927077200081, -0.4629805089094820580, -0.3070336845188419428, -0.1526574299706571214, 0.000000000000000000 ),
 .UNSPECIFIED. ) ;
#21464=CARTESIAN_POINT ( 'NONE',  ( 11.02052227349364522, 1425.209676012653290, 138.6340692233841310 ) ) ;
#21465=CARTESIAN_POINT ( 'NONE',  ( 3.670783216920000314, 1441.353588345389880, 162.1787147853980002 ) ) ;
#21466=CARTESIAN_POINT ( 'NONE',  ( -0.3357575137870000281, 1475.318672749230018, 269.4986534752979992 ) ) ;
#21467=CARTESIAN_POINT ( 'NONE',  ( -4.285659226341840267, 1446.893803312319960, 155.6485943791360000 ) ) ;
#21468=CARTESIAN_POINT ( 'NONE',  ( -7.659352831203849910, 1423.043222450190115, 144.1531583550990092 ) ) ;
#21469=CARTESIAN_POINT ( 'NONE',  ( -3.430286617134524096, 1448.286537935908427, 184.8322057208431488 ) ) ;
#21475=CARTESIAN_POINT ( 'NONE',  ( -10.50081440230080077, 1396.279756906559896, 212.6139382770819850 ) ) ;
#21476=CARTESIAN_POINT ( 'NONE',  ( -14.49383190680000055, 1422.099016295730053, 229.4564906703980114 ) ) ;
#21477=CARTESIAN_POINT ( 'NONE',  ( -44.38044571260000026, 1435.204496188100165, 269.7015000828980078 ) ) ;
#21482=CARTESIAN_POINT ( 'NONE',  ( 11.02832889669999972, 1425.240829266930177, 135.9184656016980171 ) ) ;
#21484=CARTESIAN_POINT ( 'NONE',  ( 0.000000000000000000, 1408.913060387329779, 209.1218459616979999 ) ) ;
#21491=CARTESIAN_POINT ( 'NONE',  ( 4.084250106429999860, 1507.178795002029801, 181.6747636120979905 ) ) ;
#21492=DIRECTION ( 'NONE',  ( 0.0002625959325066309024, 0.0002558942237557529668, 0.9999999327807589378 ) ) ;
#21498=CARTESIAN_POINT ( 'NONE',  ( -10.29370527480000064, 1396.272524496429924, 204.1694594168680226 ) ) ;
#21499=FACE_OUTER_BOUND ( 'NONE', #101550, .T. ) ;
#21501=CARTESIAN_POINT ( 'NONE',  ( -13.07809777927165662, 1444.819332124669927, 169.4094072714121637 ) ) ;
#21502=CARTESIAN_POINT ( 'NONE',  ( 3.871411596960000256, 1475.513060387329915, 229.5852438705979921 ) ) ;
#21505=CARTESIAN_POINT ( 'NONE',  ( 16.66093705349999965, 1410.867258618529831, 226.5061971588980043 ) ) ;
#21511=CARTESIAN_POINT ( 'NONE',  ( -37.55262814633019275, 1450.862648038850011, 134.7342395472079772 ) ) ;
#21512=CARTESIAN_POINT ( 'NONE',  ( 10.68392919824940002, 1396.286151416399889, 212.0224123608280138 ) ) ;
#21513=CARTESIAN_POINT ( 'NONE',  ( -27.58075063647599734, 1440.826346164419874, 137.2340152947450065 ) ) ;
#21514=CARTESIAN_POINT ( 'NONE',  ( 10.92291495829999981, 1429.022423092130111, 151.0007450078979900 ) ) ;
#21515=FACE_OUTER_BOUND ( 'NONE', #66390, .T. ) ;
#21517=CARTESIAN_POINT ( 'NONE',  ( 12.89603720985889979, 1434.724810852120072, 149.2205511288100013 ) ) ;
#21519=EDGE_LOOP ( 'NONE', ( #93690, #54666, #7514, #43563 ) ) ;
#21521=CARTESIAN_POINT ( 'NONE',  ( -18.71221083172660116, 1488.018745540989812, 229.0186356013300042 ) ) ;
#21523=CARTESIAN_POINT ( 'NONE',  ( -15.26434951740000123, 1488.814055421730018, 194.3933819335980218 ) ) ;
#21524=DIRECTION ( 'NONE',  ( -1.971756091734232514E-14, 0.9876883405951697448, 0.1564344650400280867 ) ) ;
#21531=CARTESIAN_POINT ( 'NONE',  ( 16.25813024210000179, 1415.087797054229895, 214.9303854824879920 ) ) ;
#21537=B_SPLINE_SURFACE_WITH_KNOTS ( 'NONE', 5, 5, ( 
 ( #107591, #65056, #29780, #40382, #81826, #82936 ),
 ( #82400, #55015, #39841, #21354, #5129, #63968 ),
 ( #47151, #89686, #14068, #89142, #64517, #80748 ),
 ( #74004, #90785, #47698, #5696, #48257, #98083 ),
 ( #99169, #56097, #13510, #14627, #108136, #72363 ),
 ( #4057, #57220, #30328, #12968, #12428, #81276 ) ),
 .UNSPECIFIED., .F., .F., .F.,
 ( 6, 6 ),
 ( 6, 6 ),
 ( 30.58270283670000111, 167.9870597316549947 ),
 ( -0.001304527548221219926, 2.000000001660000137 ),
 .UNSPECIFIED. ) ;
#21538=CARTESIAN_POINT ( 'NONE',  ( -29.83016982462270050, 1419.452566825586246, 269.4690044093881056 ) ) ;
#21541=CARTESIAN_POINT ( 'NONE',  ( -3.294994957250000134, 1408.913060387329779, 191.6318278015979786 ) ) ;
#21544=CARTESIAN_POINT ( 'NONE',  ( -32.50007362375909992, 1440.913060389729935, 245.3806128234339781 ) ) ;
#21545=CARTESIAN_POINT ( 'NONE',  ( 20.41738288953820302, 1497.614343818499947, 226.1907077604399774 ) ) ;
#21548=CARTESIAN_POINT ( 'NONE',  ( 19.98018488065979881, 1413.700872769210036, 269.6585487226739701 ) ) ;
#21549=VECTOR ( 'NONE', #63589, 1000.000000000000000 ) ;
#21552=B_SPLINE_CURVE_WITH_KNOTS ( 'NONE', 3,
 ( #68406, #6806, #15194, #49385 ),
 .UNSPECIFIED., .F., .F.,
 ( 4, 4 ),
 ( 0.000000000000000000, 0.0008471112791177455191 ),
 .UNSPECIFIED. ) ;
#21554=CARTESIAN_POINT ( 'NONE',  ( 23.66726145979999885, 1411.111568590429897, 207.8869370808679946 ) ) ;
#21558=( BOUNDED_CURVE ( )  B_SPLINE_CURVE ( 3, ( #77063, #101127, #58609, #68132 ),
 .UNSPECIFIED., .F., .F. ) 
 B_SPLINE_CURVE_WITH_KNOTS ( ( 4, 4 ),
 ( 4.700155481640241106, 5.195524193123958412 ),
 .UNSPECIFIED. ) 
 CURVE ( )  GEOMETRIC_REPRESENTATION_ITEM ( )  RATIONAL_B_SPLINE_CURVE ( ( 1.000000000000000000, 0.9796551486682428811, 0.9796551486682428811, 1.000000000000000000 ) ) 
 REPRESENTATION_ITEM ( '' )  );
#21560=CARTESIAN_POINT ( 'NONE',  ( 4.261788892647819793, 1421.884621400550031, 184.2422145791730088 ) ) ;
#21561=CARTESIAN_POINT ( 'NONE',  ( -4.154905845549999199, 1420.446155431829993, 232.6175161300979823 ) ) ;
#21565=CARTESIAN_POINT ( 'NONE',  ( 18.79734781009999978, 1416.844618635330107, 209.8348600162860009 ) ) ;
#21568=CARTESIAN_POINT ( 'NONE',  ( -20.58241196329150213, 1507.840856726199945, 228.3121576391399685 ) ) ;
#21571=DIRECTION ( 'NONE',  ( 1.988618688120850357E-13, 0.03085824620771311644, -0.9995237709234254808 ) ) ;
#21575=CARTESIAN_POINT ( 'NONE',  ( -25.42178969536794142, 1450.805819428513587, 137.2829917403189484 ) ) ;
#21580=CARTESIAN_POINT ( 'NONE',  ( -13.58245605311162763, 1416.835806623488907, 221.9090835327766627 ) ) ;
#21582=FACE_OUTER_BOUND ( 'NONE', #102790, .T. ) ;
#21583=CARTESIAN_POINT ( 'NONE',  ( 10.64609503708443050, 1434.773768202574502, 152.0346824635861935 ) ) ;
#21584=EDGE_CURVE ( 'NONE', #6924, #22249, #54632, .T. ) ;
#21586=( BOUNDED_CURVE ( )  B_SPLINE_CURVE ( 3, ( #96070, #28321, #19904, #88234 ),
 .UNSPECIFIED., .F., .T. ) 
 B_SPLINE_CURVE_WITH_KNOTS ( ( 4, 4 ),
 ( 1.102258161761371813, 1.468409620127669957 ),
 .UNSPECIFIED. ) 
 CURVE ( )  GEOMETRIC_REPRESENTATION_ITEM ( )  RATIONAL_B_SPLINE_CURVE ( ( 1.000000000000000000, 0.9888589290277138844, 0.9888589290277138844, 1.000000000000000000 ) ) 
 REPRESENTATION_ITEM ( '' )  );
#21588=CARTESIAN_POINT ( 'NONE',  ( -27.55471748229280138, 1509.768035665449815, 201.0693058872570020 ) ) ;
#21591=CARTESIAN_POINT ( 'NONE',  ( -18.69805756450000089, 1425.031978227930040, 224.7610688237980128 ) ) ;
#21594=CARTESIAN_POINT ( 'NONE',  ( 19.08482065080000112, 1478.519531283130164, 189.9637900503979893 ) ) ;
#21596=CARTESIAN_POINT ( 'NONE',  ( -17.31582335683077645, 1433.702428048472257, 216.7375878835501339 ) ) ;
#21597=CARTESIAN_POINT ( 'NONE',  ( -0.09453244570555620341, 1457.861743394589894, 229.1248241851770047 ) ) ;
#21598=ORIENTED_EDGE ( 'NONE', *, *, #49371, .F. ) ;
#21603=DIRECTION ( 'NONE',  ( -0.2130860312228880504, 0.04225590415439329367, 0.9761192457183565097 ) ) ;
#21604=CARTESIAN_POINT ( 'NONE',  ( -18.64061453619999753, 1509.327891199630130, 230.4796374886979891 ) ) ;
#21606=CARTESIAN_POINT ( 'NONE',  ( -13.48891322911904922, 1444.164948460842197, 187.0585711215786091 ) ) ;
#21607=CARTESIAN_POINT ( 'NONE',  ( -17.40764061960000220, 1414.996442553730049, 207.5654756531779697 ) ) ;
#21617=ORIENTED_EDGE ( 'NONE', *, *, #50118, .F. ) ;
#21621=CARTESIAN_POINT ( 'NONE',  ( 37.67883452730400506, 1427.401834259486805, 269.5711273142176765 ) ) ;
#21622=CARTESIAN_POINT ( 'NONE',  ( -27.17992432010000314, 1457.024587825630078, 248.2870168934979915 ) ) ;
#21624=CARTESIAN_POINT ( 'NONE',  ( -11.93743581870000092, 1433.478165980000085, 150.0011823557980222 ) ) ;
#21625=DIRECTION ( 'NONE',  ( 1.989737444810000148E-13, 6.825857443600000379E-15, -1.000000000000000000 ) ) ;
#21626=CARTESIAN_POINT ( 'NONE',  ( 11.67392614361510006, 1426.737874814250063, 139.6575252623269989 ) ) ;
#21628=CARTESIAN_POINT ( 'NONE',  ( -26.48225558509999900, 1437.467569122950181, 136.8764125097979729 ) ) ;
#21630=CARTESIAN_POINT ( 'NONE',  ( 17.02668221408760019, 1422.112876149069962, 226.8213126862850118 ) ) ;
#21632=AXIS2_PLACEMENT_3D ( 'NONE', #110085, #42890, #42328 ) ;
#21634=CARTESIAN_POINT ( 'NONE',  ( -18.80593852474190797, 1509.688961265932903, 232.5129852480815487 ) ) ;
#21635=CARTESIAN_POINT ( 'NONE',  ( 5.455728723259139821E-10, 1411.010528177349897, 256.1339838009660070 ) ) ;
#21636=ORIENTED_EDGE ( 'NONE', *, *, #15782, .T. ) ;
#21640=CARTESIAN_POINT ( 'NONE',  ( -33.87346585150000067, 1461.272374640529961, 270.3444747636979741 ) ) ;
#21642=CARTESIAN_POINT ( 'NONE',  ( -9.992007221630000153E-16, 1432.353292893639946, 155.3998094795979910 ) ) ;
#21643=CARTESIAN_POINT ( 'NONE',  ( 34.60209068530420495, 1451.703683649660206, 135.1317529420850292 ) ) ;
#21644=CARTESIAN_POINT ( 'NONE',  ( 0.2153768123770790077, 1452.918741419729940, 183.2557861667889938 ) ) ;
#21646=CARTESIAN_POINT ( 'NONE',  ( 3.931910744533549718, 1448.296755838050103, 184.2998928686550073 ) ) ;
#21649=CARTESIAN_POINT ( 'NONE',  ( -39.91655809679639333, 1422.699949167599925, 267.8112314109329759 ) ) ;
#21651=CARTESIAN_POINT ( 'NONE',  ( -3.530576738627919653, 1489.241048346600110, 181.7384218624920038 ) ) ;
#21652=ORIENTED_EDGE ( 'NONE', *, *, #30125, .F. ) ;
#21658=CARTESIAN_POINT ( 'NONE',  ( -12.33247831520000126, 1440.430499810650190, 187.9573111595979924 ) ) ;
#21659=CARTESIAN_POINT ( 'NONE',  ( -17.92792478850000037, 1415.296882282229944, 208.1699612212720183 ) ) ;
#21660=ORIENTED_EDGE ( 'NONE', *, *, #103789, .F. ) ;
#21661=CARTESIAN_POINT ( 'NONE',  ( -26.34468263449999981, 1436.394472913030086, 136.7595242481980051 ) ) ;
#21666=CARTESIAN_POINT ( 'NONE',  ( 1.177525951771697388, 1508.992568668472586, 238.7712217697011852 ) ) ;
#21668=CARTESIAN_POINT ( 'NONE',  ( -43.48935866962139585, 1430.236520443860172, 269.7109362569590303 ) ) ;
#21669=CARTESIAN_POINT ( 'NONE',  ( -0.7772817352909999755, 1427.305457135430061, 123.0297916884979941 ) ) ;
#21670=CARTESIAN_POINT ( 'NONE',  ( -5.343479798080000620, 1396.099658813630185, 199.4684377197879996 ) ) ;
#21674=CARTESIAN_POINT ( 'NONE',  ( 45.62303547458256503, 1441.762580339629494, 268.9751351163830577 ) ) ;
#21676=CARTESIAN_POINT ( 'NONE',  ( -14.18979468069059990, 1436.254652937099763, 150.1235830601330008 ) ) ;
#21679=CARTESIAN_POINT ( 'NONE',  ( -21.40977040799994668, 1506.404057888697707, 214.0392949286786859 ) ) ;
#21680=CARTESIAN_POINT ( 'NONE',  ( -18.58859720539999927, 1430.796697030029918, 225.4129132132979692 ) ) ;
#21682=CARTESIAN_POINT ( 'NONE',  ( 10.65073847843230048, 1475.392797246900045, 267.2046423057439597 ) ) ;
#21683=CARTESIAN_POINT ( 'NONE',  ( 12.65530650809999891, 1416.254459046630018, 223.0920568362980134 ) ) ;
#21687=CARTESIAN_POINT ( 'NONE',  ( -36.37832866295150325, 1435.767865547330075, 135.6928026007940105 ) ) ;
#21690=CARTESIAN_POINT ( 'NONE',  ( 3.727901463303194163, 1457.491499694037429, 228.5408078901032525 ) ) ;
#21691=CARTESIAN_POINT ( 'NONE',  ( 25.25202363594589983, 1450.803879461809856, 137.6136435803179836 ) ) ;
#21693=CARTESIAN_POINT ( 'NONE',  ( 2.689344463419570452, 1464.716346866380036, 236.9361821190090041 ) ) ;
#21695=CARTESIAN_POINT ( 'NONE',  ( 20.63995201750000064, 1409.633823394030060, 203.6085390534680073 ) ) ;
#21696=CARTESIAN_POINT ( 'NONE',  ( -3.873467979927594396, 1446.300338454377652, 170.5362326176377508 ) ) ;
#21697=CARTESIAN_POINT ( 'NONE',  ( -24.89775034519999863, 1442.835538705840008, 210.5176537872779932 ) ) ;
#21700=CARTESIAN_POINT ( 'NONE',  ( 24.11105221579398616, 1446.721418104631312, 214.9938192866167697 ) ) ;
#21701=CARTESIAN_POINT ( 'NONE',  ( 2.500000000000000000, 1439.495310474650068, 163.5954646090490030 ) ) ;
#21703=ORIENTED_EDGE ( 'NONE', *, *, #42673, .T. ) ;
#21707=CARTESIAN_POINT ( 'NONE',  ( -2.809892567274479891, 1422.122748121970062, 101.6305808166549980 ) ) ;
#21708=CARTESIAN_POINT ( 'NONE',  ( -38.94952215260590123, 1447.803421510810040, 136.5227995632060072 ) ) ;
#21711=CARTESIAN_POINT ( 'NONE',  ( 1.982459036158376930, 1417.212962208210001, 233.0589578014529479 ) ) ;
#21712=CARTESIAN_POINT ( 'NONE',  ( -2.500000000000000000, 1422.798905948130141, 153.2868469301980099 ) ) ;
#21714=CARTESIAN_POINT ( 'NONE',  ( -4.829762623019999701, 1474.871956953530116, 269.6371214077980198 ) ) ;
#21715=CARTESIAN_POINT ( 'NONE',  ( 30.42008586110589974, 1440.913060385229983, 239.6619397494469865 ) ) ;
#21721=CARTESIAN_POINT ( 'NONE',  ( -19.07182359474698075, 1485.494300952754202, 189.6180619917788590 ) ) ;
#21723=CARTESIAN_POINT ( 'NONE',  ( -1.355725730386620587, 1410.152070539702208, 185.6110041341284216 ) ) ;
#21724=CARTESIAN_POINT ( 'NONE',  ( 2.892637806539999801, 1499.013587024830031, 235.5840335634979965 ) ) ;
#21729=CARTESIAN_POINT ( 'NONE',  ( -12.45702678070000147, 1416.837177098230086, 194.7670154063979737 ) ) ;
#21730=CARTESIAN_POINT ( 'NONE',  ( -11.90000415720300175, 1434.913060496859998, 147.6452464505769910 ) ) ;
#21731=CARTESIAN_POINT ( 'NONE',  ( 2.623456343980000049, 1464.614364364229914, 236.5050914573980094 ) ) ;
#21732=CARTESIAN_POINT ( 'NONE',  ( -11.14671771210699980, 1434.019356486030119, 151.6529807626459956 ) ) ;
#21733=ORIENTED_EDGE ( 'NONE', *, *, #89320, .F. ) ;
#21734=CARTESIAN_POINT ( 'NONE',  ( -0.3166280363130000164, 1452.331784132529947, 183.2228567541980055 ) ) ;
#21739=ORIENTED_EDGE ( 'NONE', *, *, #38495, .F. ) ;
#21741=ORIENTED_EDGE ( 'NONE', *, *, #89320, .T. ) ;
#21746=LINE ( 'NONE', #55948, #53564 ) ;
#21748=CARTESIAN_POINT ( 'NONE',  ( 11.27697011000779881, 1409.306860861120185, 199.3051403546259905 ) ) ;
#21749=CARTESIAN_POINT ( 'NONE',  ( 2.745142294599053567, 1419.769955103634175, 137.0999999980979567 ) ) ;
#21751=CARTESIAN_POINT ( 'NONE',  ( 18.70459388984919968, 1509.566239199539950, 186.5372755781170042 ) ) ;
#21752=CARTESIAN_POINT ( 'NONE',  ( 11.57603212340000098, 1432.304338796609954, 151.1967213793979852 ) ) ;
#21754=DIRECTION ( 'NONE',  ( 0.8644545129124839855, 0.5024715467361959842, 0.01551579278589970169 ) ) ;
#21758=CARTESIAN_POINT ( 'NONE',  ( -11.70773956410279837, 1415.348334734199852, 195.2149244325059954 ) ) ;
#21760=CARTESIAN_POINT ( 'NONE',  ( -12.91587818989999903, 1435.175565185170171, 150.4504693756979918 ) ) ;
#21762=CARTESIAN_POINT ( 'NONE',  ( -20.06702669026240216, 1490.601403728770038, 190.8896936984549768 ) ) ;
#21767=CARTESIAN_POINT ( 'NONE',  ( -46.02767451640849572, 1440.466588444049876, 268.4960630891500273 ) ) ;
#21768=CARTESIAN_POINT ( 'NONE',  ( -20.73258660329999614, 1507.783934695429934, 191.7300198070979889 ) ) ;
#21771=CARTESIAN_POINT ( 'NONE',  ( 5.257336836053539741, 1408.563318105239887, 221.6654867046719914 ) ) ;
#21772=CARTESIAN_POINT ( 'NONE',  ( -13.84829814514429991, 1435.980421560989953, 150.2434240975769910 ) ) ;
#21774=CARTESIAN_POINT ( 'NONE',  ( 1.121268454170000206, 1416.831305841230005, 190.1585927629979835 ) ) ;
#21778=CARTESIAN_POINT ( 'NONE',  ( 25.82475784460000057, 1425.523015328830070, 244.3435519239979783 ) ) ;
#21779=CARTESIAN_POINT ( 'NONE',  ( -28.30919303690000177, 1508.136605795629976, 209.2395761310839930 ) ) ;
#21780=CARTESIAN_POINT ( 'NONE',  ( -1.528188101399999832, 1489.032157980530201, 181.5697705370980088 ) ) ;
#21781=CARTESIAN_POINT ( 'NONE',  ( 13.58235846979999906, 1416.828040475229955, 196.3349388281980055 ) ) ;
#21782=B_SPLINE_CURVE_WITH_KNOTS ( 'NONE', 3,
 ( #5986, #22753, #58059, #40689 ),
 .UNSPECIFIED., .F., .F.,
 ( 4, 4 ),
 ( -0.005718497747916959605, -1.599190933582878005E-07 ),
 .UNSPECIFIED. ) ;
#21783=CARTESIAN_POINT ( 'NONE',  ( 1.448679645196929933, 1507.129709964000085, 181.1126013477120011 ) ) ;
#21784=CARTESIAN_POINT ( 'NONE',  ( -11.09767598430000035, 1423.160780147529977, 216.2628275680980039 ) ) ;
#21787=CARTESIAN_POINT ( 'NONE',  ( 27.42695666749999717, 1450.667309086389878, 136.4365165660979926 ) ) ;
#21789=CARTESIAN_POINT ( 'NONE',  ( -2.500000000000000000, 1432.183427936470025, 157.4912586936979721 ) ) ;
#21791=CARTESIAN_POINT ( 'NONE',  ( 2.958832406229999989, 1509.097160381630147, 238.9948613597979943 ) ) ;
#21801=CARTESIAN_POINT ( 'NONE',  ( -4.356169890730000382, 1470.481192091330058, 234.8232070940980236 ) ) ;
#21804=CARTESIAN_POINT ( 'NONE',  ( 11.15483420530000025, 1425.160608745730087, 144.1639996081979973 ) ) ;
#21805=CARTESIAN_POINT ( 'NONE',  ( -13.01538513870579905, 1416.535698381769862, 221.8985197201349990 ) ) ;
#21806=CARTESIAN_POINT ( 'NONE',  ( -0.1377404852739999852, 1420.462255397929766, 182.7340595799979894 ) ) ;
#21811=CARTESIAN_POINT ( 'NONE',  ( 13.39209664583887260, 1443.386748700186445, 187.8724463653802275 ) ) ;
#21812=ORIENTED_EDGE ( 'NONE', *, *, #56592, .F. ) ;
#21813=ORIENTED_EDGE ( 'NONE', *, *, #10991, .T. ) ;
#21822=CARTESIAN_POINT ( 'NONE',  ( -20.06202041079472664, 1509.646782119672707, 231.0063366968753940 ) ) ;
#21823=DIRECTION ( 'NONE',  ( -0.9993908270190798859, -0.03489949670295298956, 0.000000000000000000 ) ) ;
#21825=CARTESIAN_POINT ( 'NONE',  ( 16.63654589489999935, 1507.631725798030175, 193.5314252907980119 ) ) ;
#21827=CARTESIAN_POINT ( 'NONE',  ( -24.56184656835360158, 1509.239445071429827, 222.5723712071969942 ) ) ;
#21828=CARTESIAN_POINT ( 'NONE',  ( 11.00428676220000135, 1425.778354413130046, 91.15517427569778874 ) ) ;
#21830=CARTESIAN_POINT ( 'NONE',  ( 6.509745603069999831, 1426.468882613529786, 219.6133830848980040 ) ) ;
#21837=VERTEX_POINT ( 'NONE', #85400 ) ;
#21839=B_SPLINE_CURVE_WITH_KNOTS ( 'NONE', 5,
 ( #7558, #66393, #49580, #41712, #108370, #59087 ),
 .UNSPECIFIED., .F., .F.,
 ( 6, 6 ),
 ( 0.000000000000000000, 1.000000000000000000 ),
 .UNSPECIFIED. ) ;
#21840=CARTESIAN_POINT ( 'NONE',  ( -1.665548205979999974, 1442.756953654919926, 150.7199974615980125 ) ) ;
#21842=CARTESIAN_POINT ( 'NONE',  ( -12.75406323559999855, 1424.720109696429972, 222.3910987067980045 ) ) ;
#21847=CARTESIAN_POINT ( 'NONE',  ( 16.22122407919999887, 1419.769442695729822, 227.2112992638979847 ) ) ;
#21851=CARTESIAN_POINT ( 'NONE',  ( -18.65369358539999922, 1410.060631937529934, 223.2007661954980051 ) ) ;
#21852=CARTESIAN_POINT ( 'NONE',  ( 1.549824244036819954, 1416.029511582939904, 190.4358552523449930 ) ) ;
#21853=CARTESIAN_POINT ( 'NONE',  ( -1.341950169440000007, 1416.837177099130031, 228.0806925301980073 ) ) ;
#21854=LINE ( 'NONE', #30282, #11075 ) ;
#21857=CARTESIAN_POINT ( 'NONE',  ( 4.222531898828509433, 1446.229786520979815, 170.5365406785500113 ) ) ;
#21858=CARTESIAN_POINT ( 'NONE',  ( 0.2089863181176309925, 1457.918365060180122, 183.0423947760509975 ) ) ;
#21859=CARTESIAN_POINT ( 'NONE',  ( -8.161124881772790829, 1407.550611316829873, 219.8408402379180018 ) ) ;
#21860=CARTESIAN_POINT ( 'NONE',  ( -18.11157280723839946, 1509.545530446499924, 231.7129765844609892 ) ) ;
#21862=CARTESIAN_POINT ( 'NONE',  ( -28.95760783391549964, 1509.892758078639872, 211.5366180273940131 ) ) ;
#21863=CARTESIAN_POINT ( 'NONE',  ( 11.87938290520000173, 1433.311437408509846, 148.5014532950980026 ) ) ;
#21864=CARTESIAN_POINT ( 'NONE',  ( -27.25231198120000187, 1435.447456822929780, 135.7102113810979915 ) ) ;
#21865=CARTESIAN_POINT ( 'NONE',  ( 7.124127264130000192, 1440.776731797129742, 185.7078817695979751 ) ) ;
#21866=ORIENTED_EDGE ( 'NONE', *, *, #15906, .T. ) ;
#21869=CARTESIAN_POINT ( 'NONE',  ( -3.536556481637670224, 1409.036559661029969, 223.6857672521330187 ) ) ;
#21871=CARTESIAN_POINT ( 'NONE',  ( -1.438891081339280120, 1452.191228260170192, 183.8587004481619829 ) ) ;
#21873=CARTESIAN_POINT ( 'NONE',  ( 40.47987261475308429, 1425.122386052929869, 269.1161687812102059 ) ) ;
#21879=CARTESIAN_POINT ( 'NONE',  ( 20.59684415220000275, 1507.762623718730083, 227.6602567104980039 ) ) ;
#21880=CARTESIAN_POINT ( 'NONE',  ( -28.66375040065220148, 1509.283859623159969, 208.7539660915670083 ) ) ;
#21881=CARTESIAN_POINT ( 'NONE',  ( -3.549608351769999892, 1507.276797637930031, 180.9704965309979912 ) ) ;
#21886=CARTESIAN_POINT ( 'NONE',  ( 40.26903804221177552, 1443.994134351532466, 137.1270700188907483 ) ) ;
#21888=( BOUNDED_SURFACE ( )  B_SPLINE_SURFACE ( 1, 2, ( 
 ( #70763, #104874, #19756 ),
 ( #28164, #96476, #53958 ) ),
 .UNSPECIFIED., .F., .F., .F. ) 
 B_SPLINE_SURFACE_WITH_KNOTS ( ( 2, 2 ),
 ( 3, 3 ),
 ( -10000.00000000000000, 10000.00000000000000 ),
 ( 5.178100005969419328, 6.283185307179590673 ),
 .UNSPECIFIED. ) 
 GEOMETRIC_REPRESENTATION_ITEM ( )  RATIONAL_B_SPLINE_SURFACE ( (
 ( 0.8778166915507200629, 0.7939440108092760129, 1.000000000000000000),
 ( 0.8778166915507200629, 0.7939440108092760129, 1.000000000000000000) ) ) 
 REPRESENTATION_ITEM ( '' )  SURFACE ( )  );
#21890=CARTESIAN_POINT ( 'NONE',  ( -0.1204520906467640012, 1419.725873375750098, 184.2476600981560182 ) ) ;
#21893=CARTESIAN_POINT ( 'NONE',  ( 21.21836729700000390, 1410.149259758630023, 217.3752858609580016 ) ) ;
#21894=CARTESIAN_POINT ( 'NONE',  ( -2.193561875386760285, 1410.361078172129965, 186.3822773651310172 ) ) ;
#21895=EDGE_CURVE ( 'NONE', #6969, #16284, #66721, .T. ) ;
#21897=CARTESIAN_POINT ( 'NONE',  ( -16.47684141300000249, 1422.522700970730057, 227.3110121918980155 ) ) ;
#21899=CARTESIAN_POINT ( 'NONE',  ( -11.60004869885203682, 1426.786830457828273, 134.3786150874268799 ) ) ;
#21903=CARTESIAN_POINT ( 'NONE',  ( -2.165008118169999829, 1417.511146367829951, 235.1473874566980271 ) ) ;
#21906=CARTESIAN_POINT ( 'NONE',  ( -10.60916564155689912, 1486.014526782129906, 184.0550009821979813 ) ) ;
#21911=ORIENTED_EDGE ( 'NONE', *, *, #52966, .F. ) ;
#21917=CARTESIAN_POINT ( 'NONE',  ( -15.69847554260145728, 1410.486759826540947, 226.6795578664016375 ) ) ;
#21918=CARTESIAN_POINT ( 'NONE',  ( 15.71155388851390100, 1410.111410872460056, 191.7201049767249685 ) ) ;
#21920=EDGE_CURVE ( 'NONE', #94174, #101515, #10356, .T. ) ;
#21921=CARTESIAN_POINT ( 'NONE',  ( -25.31040623107189802, 1451.150865907959997, 137.2672303054409895 ) ) ;
#21923=CARTESIAN_POINT ( 'NONE',  ( 13.47022716080000215, 1410.756447827730199, 228.3151136380979835 ) ) ;
#21927=CARTESIAN_POINT ( 'NONE',  ( 41.66188030070000536, 1443.681299837730194, 134.0999999982049928 ) ) ;
#21928=FACE_OUTER_BOUND ( 'NONE', #52967, .T. ) ;
#21929=CARTESIAN_POINT ( 'NONE',  ( 14.22286847238659924, 1435.189194894129969, 149.2182491042620143 ) ) ;
#21934=CARTESIAN_POINT ( 'NONE',  ( 9.130068049997401403, 1410.607079801739701, 230.1289593719837967 ) ) ;
#21938=CARTESIAN_POINT ( 'NONE',  ( -26.92695807870000380, 1508.008395488129963, 203.1594552079080245 ) ) ;
#21943=CARTESIAN_POINT ( 'NONE',  ( 10.58917204930000011, 1416.519106787730152, 194.4914516038979855 ) ) ;
#21945=ORIENTED_EDGE ( 'NONE', *, *, #55537, .F. ) ;
#21949=CARTESIAN_POINT ( 'NONE',  ( 35.01374679072880269, 1440.913060387330006, 260.8650110618089570 ) ) ;
#21950=CARTESIAN_POINT ( 'NONE',  ( 19.56640942089999768, 1477.362144060529999, 227.5239896928979988 ) ) ;
#21952=CARTESIAN_POINT ( 'NONE',  ( -0.03276332933436820055, 1451.172142415660119, 182.5300517626539829 ) ) ;
#21953=CARTESIAN_POINT ( 'NONE',  ( -15.50892216750000152, 1410.826985104829873, 191.0414747596979907 ) ) ;
#21957=CARTESIAN_POINT ( 'NONE',  ( 22.24622733321460188, 1410.233794050260030, 206.2464451110010089 ) ) ;
#21959=CARTESIAN_POINT ( 'NONE',  ( 1.328042612950000034, 1406.002643151530037, 266.9604903208979749 ) ) ;
#21962=CARTESIAN_POINT ( 'NONE',  ( 16.16575468819999983, 1459.553750540530018, 229.8409642424979893 ) ) ;
#21963=CARTESIAN_POINT ( 'NONE',  ( 0.2456417414777120334, 1457.830897802899926, 228.9878416128509855 ) ) ;
#21968=CARTESIAN_POINT ( 'NONE',  ( -0.1573922665717430169, 1507.260657537599855, 180.8910309565839896 ) ) ;
#21971=CARTESIAN_POINT ( 'NONE',  ( 18.66848652210000026, 1509.564978301430074, 187.1506650077980112 ) ) ;
#21976=CARTESIAN_POINT ( 'NONE',  ( 25.89198661420000036, 1440.913060407119929, 221.6500998374979758 ) ) ;
#21977=CARTESIAN_POINT ( 'NONE',  ( -11.56980561469999991, 1431.824675720370124, 151.1783349937979892 ) ) ;
#21980=CARTESIAN_POINT ( 'NONE',  ( -0.3885940661755200032, 1508.683165393880245, 238.1397126418920038 ) ) ;
#21982=CARTESIAN_POINT ( 'NONE',  ( 12.40989122010000045, 1445.169290119350080, 186.8528423751979801 ) ) ;
#21984=CARTESIAN_POINT ( 'NONE',  ( -20.97306094379999664, 1457.442401685129880, 223.5384559969980103 ) ) ;
#21985=CARTESIAN_POINT ( 'NONE',  ( 5.366743882629579687, 1426.154185019739998, 152.4687380856059917 ) ) ;
#21986=FACE_OUTER_BOUND ( 'NONE', #25533, .T. ) ;
#21989=CARTESIAN_POINT ( 'NONE',  ( 2.094456431300000254, 1406.299313630030156, 269.2930948147979962 ) ) ;
#21990=EDGE_CURVE ( 'NONE', #63851, #22743, #45303, .T. ) ;
#21993=CARTESIAN_POINT ( 'NONE',  ( 23.71260330876479827, 1434.455778039984807, 214.5166046885597098 ) ) ;
#21995=CARTESIAN_POINT ( 'NONE',  ( 11.60004869885203682, 1423.633693347439475, 135.8154946617876249 ) ) ;
#21998=CARTESIAN_POINT ( 'NONE',  ( -0.5697989934050000649, 1450.893162568020216, 155.6080925171979743 ) ) ;
#21999=CARTESIAN_POINT ( 'NONE',  ( -1.554371093571602636, 1451.096106140563052, 183.6610704733489285 ) ) ;
#22000=CARTESIAN_POINT ( 'NONE',  ( 2.318887788901189850, 1449.808491804770028, 155.3361369919100241 ) ) ;
#22001=CARTESIAN_POINT ( 'NONE',  ( -13.59781064528760020, 1415.089996090609930, 220.5183280911249994 ) ) ;
#22003=CARTESIAN_POINT ( 'NONE',  ( -32.79207798510000771, 1428.560640286930038, 262.6648722511980054 ) ) ;
#22005=CARTESIAN_POINT ( 'NONE',  ( 3.654458881370000078, 1441.526081356940040, 166.9096120827979917 ) ) ;
#22006=CARTESIAN_POINT ( 'NONE',  ( -2.111022820160000091, 1476.015127867530055, 268.4819080596980143 ) ) ;
#22007=CARTESIAN_POINT ( 'NONE',  ( 9.767576865416099707, 1416.948096802409964, 215.8813206395359998 ) ) ;
#22010=CARTESIAN_POINT ( 'NONE',  ( -2.500000000000000000, 1448.210448412289907, 183.1418046154980175 ) ) ;
#22018=CARTESIAN_POINT ( 'NONE',  ( -2.054592539991249911, 1395.984808339839901, 219.9445789274560070 ) ) ;
#22021=CARTESIAN_POINT ( 'NONE',  ( -44.83996340390000057, 1438.826799026090157, 269.6929264061980120 ) ) ;
#22030=CARTESIAN_POINT ( 'NONE',  ( 40.24526342089999531, 1444.639349322710132, 137.0236526114979938 ) ) ;
#22035=CARTESIAN_POINT ( 'NONE',  ( 5.949633633660000420, 1509.124405061829975, 180.2787687912980061 ) ) ;
#22039=EDGE_CURVE ( 'NONE', #32788, #71548, #106907, .T. ) ;
#22043=CARTESIAN_POINT ( 'NONE',  ( -11.33516131130000026, 1396.308892942629882, 207.6268627275279925 ) ) ;
#22044=CARTESIAN_POINT ( 'NONE',  ( -21.35664706530000245, 1409.658850939629929, 213.3192769937880087 ) ) ;
#22046=CARTESIAN_POINT ( 'NONE',  ( -13.17594539069787274, 1444.732583810137385, 169.3946485105632291 ) ) ;
#22051=CARTESIAN_POINT ( 'NONE',  ( 1.298837812259999946, 1410.307958403729799, 185.2609176365979806 ) ) ;
#22052=CARTESIAN_POINT ( 'NONE',  ( -7.090791903819999575, 1414.913060387329779, 194.3735294399980091 ) ) ;
#22053=CARTESIAN_POINT ( 'NONE',  ( -41.14894028195599418, 1446.681896710060073, 135.2730459677599981 ) ) ;
#22055=CARTESIAN_POINT ( 'NONE',  ( 10.14935679994219875, 1396.267483737839939, 213.5348577357469821 ) ) ;
#22056=CARTESIAN_POINT ( 'NONE',  ( 1.124394188919999982, 1416.535385209630022, 190.1732668564980031 ) ) ;
#22057=CARTESIAN_POINT ( 'NONE',  ( 11.20517263770000049, 1426.030335666529936, 148.0940953015980028 ) ) ;
#22058=CARTESIAN_POINT ( 'NONE',  ( 8.680232473730548293, 1509.216213366276406, 181.1240079135133954 ) ) ;
#22059=ORIENTED_EDGE ( 'NONE', *, *, #93344, .F. ) ;
#22061=ORIENTED_EDGE ( 'NONE', *, *, #28887, .T. ) ;
#22062=EDGE_CURVE ( 'NONE', #108306, #93939, #71226, .T. ) ;
#22064=CARTESIAN_POINT ( 'NONE',  ( -19.00773967308149892, 1468.169424052289969, 227.6346832009180048 ) ) ;
#22074=CARTESIAN_POINT ( 'NONE',  ( 2.500000000000059952, 1448.812655445319933, 156.5234696244650081 ) ) ;
#22076=CARTESIAN_POINT ( 'NONE',  ( 16.97980319039999841, 1414.913060387329779, 210.1126989473540050 ) ) ;
#22078=VERTEX_POINT ( 'NONE', #12294 ) ;
#22081=CARTESIAN_POINT ( 'NONE',  ( -27.65802006675362890, 1417.861769239410251, 269.4462164507287980 ) ) ;
#22085=CARTESIAN_POINT ( 'NONE',  ( -0.01247695416628590015, 1452.307842348659960, 183.1512626530130206 ) ) ;
#22086=CARTESIAN_POINT ( 'NONE',  ( -32.66611254161259836, 1440.913060389849988, 245.7919302191029942 ) ) ;
#22088=CARTESIAN_POINT ( 'NONE',  ( -0.06005238713462270062, 1466.393664084419925, 235.6964261762240085 ) ) ;
#22089=CARTESIAN_POINT ( 'NONE',  ( 29.04137415450000148, 1415.566708622129909, 270.1335617710980159 ) ) ;
#22092=CARTESIAN_POINT ( 'NONE',  ( 23.72329886969999890, 1410.130063465129979, 208.9290854598660019 ) ) ;
#22098=CARTESIAN_POINT ( 'NONE',  ( 4.213210515277539869, 1421.777857766699981, 184.5142607373319947 ) ) ;
#22102=VERTEX_POINT ( 'NONE', #55430 ) ;
#22104=DIRECTION ( 'NONE',  ( -0.03248864917721539652, 0.9989961268278857442, 0.03084195612347889401 ) ) ;
#22105=CARTESIAN_POINT ( 'NONE',  ( 0.7357070794679999581, 1416.194395688229861, 233.4110786845979817 ) ) ;
#22111=EDGE_CURVE ( 'NONE', #56812, #46627, #58571, .T. ) ;
#22114=DIRECTION ( 'NONE',  ( 0.03489949677589983257, 0.9993908270165325902, 3.539110176465913504E-10 ) ) ;
#22118=CARTESIAN_POINT ( 'NONE',  ( 27.79064039367209915, 1508.605033446070138, 207.7520403700050053 ) ) ;
#22119=ORIENTED_EDGE ( 'NONE', *, *, #18509, .T. ) ;
#22121=AXIS2_PLACEMENT_3D ( 'NONE', #27604, #11910, #36556 ) ;
#22126=CARTESIAN_POINT ( 'NONE',  ( 16.31593820514824245, 1421.547646607773231, 227.2390930618354332 ) ) ;
#22128=DIRECTION ( 'NONE',  ( 0.000000000000000000, 0.000000000000000000, 1.000000000000000000 ) ) ;
#22129=CARTESIAN_POINT ( 'NONE',  ( -19.63203962769999933, 1425.837002826029902, 223.1478923402980001 ) ) ;
#22130=CARTESIAN_POINT ( 'NONE',  ( -31.87156127897992164, 1465.374349214318727, 269.3184216098884463 ) ) ;
#22132=CARTESIAN_POINT ( 'NONE',  ( 16.88838891829999866, 1438.560075112930235, 190.6614884790980113 ) ) ;
#22134=CARTESIAN_POINT ( 'NONE',  ( 29.78452510889999871, 1510.001069734030125, 209.1390482955230254 ) ) ;
#22135=CARTESIAN_POINT ( 'NONE',  ( -10.92505087063870661, 1470.396171842393642, 269.3500471555659033 ) ) ;
#22136=ORIENTED_EDGE ( 'NONE', *, *, #5717, .T. ) ;
#22138=ADVANCED_FACE ( 'NONE', ( #89561 ), #97274, .T. ) ;
#22140=CARTESIAN_POINT ( 'NONE',  ( 11.52810963750000006, 1441.751267666019885, 147.8533156590980013 ) ) ;
#22142=CARTESIAN_POINT ( 'NONE',  ( -11.73230603450000054, 1475.513060387329915, 226.3291547820980156 ) ) ;
#22145=CARTESIAN_POINT ( 'NONE',  ( -13.38968634609168973, 1444.443546846214304, 186.8783483159165257 ) ) ;
#22149=CARTESIAN_POINT ( 'NONE',  ( -14.20882318218850671, 1410.783320127021625, 226.8601890847973550 ) ) ;
#22151=CARTESIAN_POINT ( 'NONE',  ( 23.71772659069999989, 1435.325744483010112, 137.0491500660980080 ) ) ;
#22153=CARTESIAN_POINT ( 'NONE',  ( 21.45381977619999958, 1509.599256739130169, 189.3186887596979773 ) ) ;
#22156=EDGE_CURVE ( 'NONE', #3437, #31004, #9193, .T. ) ;
#22158=ORIENTED_EDGE ( 'NONE', *, *, #23342, .F. ) ;
#22162=CARTESIAN_POINT ( 'NONE',  ( 16.13326284106888409, 1412.745257486696573, 269.3696321425749147 ) ) ;
#22163=CARTESIAN_POINT ( 'NONE',  ( -29.79081509809999773, 1446.796541104080234, 240.1465591067980085 ) ) ;
#22165=B_SPLINE_CURVE_WITH_KNOTS ( 'NONE', 3,
 ( #101377, #5714, #32002, #100310, #24128, #73477 ),
 .UNSPECIFIED., .F., .F.,
 ( 4, 2, 4 ),
 ( -0.2778631991162420212, -0.1390217994342580199, -1.348645189525043975E-06 ),
 .UNSPECIFIED. ) ;
#22166=CARTESIAN_POINT ( 'NONE',  ( -19.61843700589999884, 1487.979149483630181, 189.7675855031980063 ) ) ;
#22167=CARTESIAN_POINT ( 'NONE',  ( -11.27542400379999954, 1433.368079989050102, 151.5215836857980207 ) ) ;
#22168=ADVANCED_FACE ( 'NONE', ( #61449 ), #74303, .T. ) ;
#22170=CARTESIAN_POINT ( 'NONE',  ( 11.66274484067749917, 1426.745571914170114, 138.8594401931470088 ) ) ;
#22171=LINE ( 'NONE', #90500, #66151 ) ;
#22173=CARTESIAN_POINT ( 'NONE',  ( -24.36390206349999943, 1440.635616014810012, 211.6747593621879844 ) ) ;
#22177=B_SPLINE_CURVE_WITH_KNOTS ( 'NONE', 5,
 ( #85212, #8503, #60603, #70124, #26983, #18549 ),
 .UNSPECIFIED., .F., .F.,
 ( 6, 6 ),
 ( -48.27399248280480037, -29.43575841650000058 ),
 .UNSPECIFIED. ) ;
#22179=CARTESIAN_POINT ( 'NONE',  ( 1.632486301776860348E-07, 1509.047264794319972, 239.1218459617020073 ) ) ;
#22180=CARTESIAN_POINT ( 'NONE',  ( 2.013013938216309949E-10, 1411.227950868479866, 255.5841367965100517 ) ) ;
#22181=VERTEX_POINT ( 'NONE', #62042 ) ;
#22182=ORIENTED_EDGE ( 'NONE', *, *, #94887, .T. ) ;
#22185=CARTESIAN_POINT ( 'NONE',  ( -19.91919522000000242, 1467.971789498529915, 269.3862225696980204 ) ) ;
#22187=CARTESIAN_POINT ( 'NONE',  ( 11.86590139589999815, 1432.348266868109931, 151.0567667964980103 ) ) ;
#22188=CARTESIAN_POINT ( 'NONE',  ( 2.500000000000000000, 1425.929641634319978, 183.3886485707629959 ) ) ;
#22189=CARTESIAN_POINT ( 'NONE',  ( 0.2130409879942949947, 1451.905578552620000, 182.9902910394959861 ) ) ;
#22190=DIRECTION ( 'NONE',  ( 0.000000000000000000, 0.000000000000000000, -1.000000000000000000 ) ) ;
#22194=CARTESIAN_POINT ( 'NONE',  ( -24.16313269558360233, 1410.872200102120132, 267.2902278704040100 ) ) ;
#22196=CARTESIAN_POINT ( 'NONE',  ( -3.538842271800570316, 1496.895311935370046, 181.4128009767959782 ) ) ;
#22199=ORIENTED_EDGE ( 'NONE', *, *, #67080, .T. ) ;
#22203=EDGE_CURVE ( 'NONE', #96481, #110373, #74642, .T. ) ;
#22206=CARTESIAN_POINT ( 'NONE',  ( -15.54206776589999883, 1455.451630440330064, 188.8651685368980395 ) ) ;
#22207=CARTESIAN_POINT ( 'NONE',  ( -16.16160143211049771, 1461.177280122519960, 228.3234948423969968 ) ) ;
#22208=B_SPLINE_SURFACE_WITH_KNOTS ( 'NONE', 5, 5, ( 
 ( #59114, #93239, #33881, #16505, #17047, #34443, #68619, #102721, #26015 ),
 ( #50163, #84291, #89331, #12626, #4233, #29964, #64713, #3703, #106674 ),
 ( #62517, #70920, #80935, #45149, #28326, #54658, #37833, #19909, #105035 ),
 ( #88238, #96639, #28881, #72018, #54109, #11530, #98829, #45705, #106135 ),
 ( #79843, #29411, #2600, #13147, #63076, #36725, #107231, #30521, #98275 ),
 ( #105598, #22089, #12068, #88787, #46805, #89877, #4766, #3152, #47331 ),
 ( #37284, #46260, #81460, #63612, #73092, #64157, #38366, #79290, #97728 ),
 ( #80387, #20999, #71476, #20449, #72543, #55203, #56287, #21548, #55760 ),
 ( #90416, #97176, #38909, #99920, #41687, #66364, #15360, #40028, #24317 ),
 ( #50104, #14264, #84229, #58500, #90976, #103086, #108338, #73655, #7530 ),
 ( #5883, #100484, #26386, #108888, #32731, #68985, #39483, #14817, #101019 ),
 ( #65798, #92628, #83678, #23765, #107786, #40579, #666, #49552, #92085 ),
 ( #83138, #41128, #6977, #5324, #31070, #15903, #75308, #57414, #49004 ),
 ( #32181, #77365, #34797, #60581, #13696, #65251, #99364, #22638, #6433 ),
 ( #74208, #57952, #47882, #109452, #66911, #82020, #56843, #74751, #48454 ),
 ( #23214, #82593, #31622, #91540, #2335, #86855, #53845, #10147, #61147 ),
 ( #45432, #11805, #17977, #94702, #36447, #52172, #70645, #43758, #104210 ),
 ( #53278, #69538, #77910, #28606, #35914, #44320, #70097, #2880, #78464 ),
 ( #28047, #62237, #87982, #79576, #3427, #87417, #36999, #71191, #1216 ),
 ( #19642, #86303, #35351, #27497, #10713, #103659, #9587, #1778, #26957 ),
 ( #61684, #44884, #95262, #18523, #37559, #52720, #79034, #104762, #95807 ),
 ( #96363, #105875, #19074, #11270, #105313, #62806, #96922, #20189, #54387 ),
 ( #88520, #45974, #80108, #71759, #29156, #56018, #13985, #29698, #56569 ),
 ( #99090, #99638, #90142, #81739, #108612, #90699, #107507, #5609, #54926 ) ),
 .UNSPECIFIED., .F., .F., .F.,
 ( 6, 3, 3, 3, 3, 3, 3, 6 ),
 ( 6, 3, 6 ),
 ( 24.02057840196890126, 75.98747947549999537, 109.6124278280000084, 126.4746888579999933, 132.7969126290000190, 135.9580245150000053, 139.1191364009999916, 143.3302516649309837 ),
 ( 0.000000000000000000, 1.000000000000000000, 2.000029560931110062 ),
 .UNSPECIFIED. ) ;
#22209=VERTEX_POINT ( 'NONE', #11066 ) ;
#22210=CARTESIAN_POINT ( 'NONE',  ( -26.79414277889999951, 1435.433175433119914, 135.2874649707979984 ) ) ;
#22213=CARTESIAN_POINT ( 'NONE',  ( 3.211131771843309668, 1415.841837342140252, 233.8555552817769865 ) ) ;
#22214=CARTESIAN_POINT ( 'NONE',  ( 2.688586027246119947, 1509.006950727750109, 238.2845013960090057 ) ) ;
#22215=CARTESIAN_POINT ( 'NONE',  ( -43.48865910597699980, 1440.913050606110119, 270.3367101327119713 ) ) ;
#22216=DIRECTION ( 'NONE',  ( 0.000000000000000000, -0.9990482215818579093, -0.04361938736533144123 ) ) ;
#22217=CARTESIAN_POINT ( 'NONE',  ( 0.06016749670950000128, 1397.283812747630009, 196.1836558358980085 ) ) ;
#22219=EDGE_LOOP ( 'NONE', ( #81813, #29835, #2504, #92599 ) ) ;
#22223=CARTESIAN_POINT ( 'NONE',  ( -2.500000000000000000, 1419.443562236106345, 141.2948928672179818 ) ) ;
#22224=CARTESIAN_POINT ( 'NONE',  ( -1.075916898909999864, 1485.885486078329905, 181.8684512949980103 ) ) ;
#22228=CARTESIAN_POINT ( 'NONE',  ( -14.61523087940000032, 1430.144796240230107, 222.1530162304980252 ) ) ;
#22229=CARTESIAN_POINT ( 'NONE',  ( 12.78667948450000047, 1416.822690122329959, 222.9174005869979851 ) ) ;
#22231=ORIENTED_EDGE ( 'NONE', *, *, #83503, .F. ) ;
#22233=EDGE_LOOP ( 'NONE', ( #5978, #14457, #87661, #5729, #47441 ) ) ;
#22237=VERTEX_POINT ( 'NONE', #86654 ) ;
#22239=CARTESIAN_POINT ( 'NONE',  ( 23.92107583702020079, 1452.077735920189980, 137.0198744514089810 ) ) ;
#22240=CARTESIAN_POINT ( 'NONE',  ( 13.53550618839999942, 1416.067629290630066, 196.4934937118979974 ) ) ;
#22242=CARTESIAN_POINT ( 'NONE',  ( 18.92936377790000080, 1409.738736466630144, 196.3471921528980033 ) ) ;
#22243=CARTESIAN_POINT ( 'NONE',  ( -27.68254001883949655, 1507.989615300039986, 210.5775529569929745 ) ) ;
#22246=CARTESIAN_POINT ( 'NONE',  ( -8.881784196999999612E-15, 1446.564900598709983, 126.8032249175980155 ) ) ;
#22247=CARTESIAN_POINT ( 'NONE',  ( 2.500000000000000000, 1439.361286091369948, 161.1256395968530057 ) ) ;
#22249=VERTEX_POINT ( 'NONE', #45236 ) ;
#22251=CARTESIAN_POINT ( 'NONE',  ( -29.18142758420000149, 1466.479558604430167, 269.9486951468979896 ) ) ;
#22252=CARTESIAN_POINT ( 'NONE',  ( -2.500000000000000000, 1448.894380913990062, 183.1110194797979887 ) ) ;
#22253=CARTESIAN_POINT ( 'NONE',  ( -2.885915196579980080, 1421.960918650529948, 112.2554875371340017 ) ) ;
#22257=CARTESIAN_POINT ( 'NONE',  ( -1.918070871662279853, 1477.784538725520179, 183.2207360801660059 ) ) ;
#22260=CARTESIAN_POINT ( 'NONE',  ( 27.70013467925890183, 1440.913060387809992, 229.9159422604259930 ) ) ;
#22263=ORIENTED_EDGE ( 'NONE', *, *, #102772, .T. ) ;
#22272=AXIS2_PLACEMENT_3D ( 'NONE', #81641, #56471, #109083 ) ;
#22273=CARTESIAN_POINT ( 'NONE',  ( 15.10324330609999954, 1409.440477264029823, 192.5109551743979921 ) ) ;
#22277=CARTESIAN_POINT ( 'NONE',  ( -15.54069288340000021, 1507.627022993330229, 192.2862817006979981 ) ) ;
#22279=CARTESIAN_POINT ( 'NONE',  ( 1.476596736730000137, 1465.998869369329896, 235.0546012516979886 ) ) ;
#22281=CARTESIAN_POINT ( 'NONE',  ( -0.5361601820109999084, 1452.003350861930130, 183.1486451269979909 ) ) ;
#22282=EDGE_CURVE ( 'NONE', #22747, #74953, #98128, .T. ) ;
#22292=CARTESIAN_POINT ( 'NONE',  ( 34.51169404606030611, 1437.059671538590237, 136.5459531931829815 ) ) ;
#22294=CARTESIAN_POINT ( 'NONE',  ( -11.60004869885204215, 1426.371424667298925, 136.9558864814476919 ) ) ;
#22298=CARTESIAN_POINT ( 'NONE',  ( 8.233640524757710466, 1409.200585450159906, 196.6252762661590054 ) ) ;
#22299=CARTESIAN_POINT ( 'NONE',  ( 18.02093605269999799, 1424.326858638329895, 225.1991111336980111 ) ) ;
#22301=CARTESIAN_POINT ( 'NONE',  ( -19.07203922379999739, 1485.640791703330024, 189.6106623856980207 ) ) ;
#22304=CARTESIAN_POINT ( 'NONE',  ( -2.499989904720139933, 1448.906960178189820, 183.3908600069959789 ) ) ;
#22305=ORIENTED_EDGE ( 'NONE', *, *, #62285, .F. ) ;
#22307=CONICAL_SURFACE ( 'NONE', #38399, 1.000000000000009104, 0.7853981633970000820 ) ;
#22309=CARTESIAN_POINT ( 'NONE',  ( 17.96600282473259824, 1457.758676852030021, 228.7894647061090154 ) ) ;
#22310=CARTESIAN_POINT ( 'NONE',  ( -12.65205114049999935, 1435.423691554170091, 150.7971429281979852 ) ) ;
#22311=CARTESIAN_POINT ( 'NONE',  ( 3.320959845659019973E-10, 1465.220663907560038, 238.5330492740649788 ) ) ;
#22312=CARTESIAN_POINT ( 'NONE',  ( -20.36866774749589837, 1500.371803671309863, 190.6068050527740070 ) ) ;
#22318=CARTESIAN_POINT ( 'NONE',  ( -46.15243863885639541, 1440.913067582900112, 268.2044766056350227 ) ) ;
#22319=CARTESIAN_POINT ( 'NONE',  ( -19.39897567239999887, 1468.962688716530010, 192.4463568245979843 ) ) ;
#22322=CARTESIAN_POINT ( 'NONE',  ( 1.344050583552389933, 1408.775600028340023, 223.1975148624649989 ) ) ;
#22323=CARTESIAN_POINT ( 'NONE',  ( -13.47209471068070030, 1435.515832415140039, 150.2099290526579694 ) ) ;
#22325=B_SPLINE_SURFACE_WITH_KNOTS ( 'NONE', 5, 5, ( 
 ( #4158, #108248, #72467, #40492, #47802, #99279 ),
 ( #30439, #38832, #74670, #23127, #98192, #31538 ),
 ( #106597, #74119, #14736, #57332, #22005, #47253 ),
 ( #73572, #32097, #108803, #48924, #82508, #83052 ),
 ( #81377, #107704, #13614, #29882, #21465, #90334 ),
 ( #56202, #5807, #4692, #66284, #65714, #30989 ),
 ( #65164, #56759, #55674, #14180, #57869, #38285 ),
 ( #73010, #91457, #81937, #6345, #39947, #64073 ),
 ( #99835, #100400, #107146, #64624, #89795, #23684 ) ),
 .UNSPECIFIED., .F., .F., .F.,
 ( 6, 3, 6 ),
 ( 6, 6 ),
 ( 50.07766623440000586, 62.52389936639999490, 69.76872775750000244 ),
 ( 0.000000000000000000, 2.000000000000000000 ),
 .UNSPECIFIED. ) ;
#22327=CARTESIAN_POINT ( 'NONE',  ( 4.221337299212926553, 1424.740940193975348, 226.9639360934303056 ) ) ;
#22330=CARTESIAN_POINT ( 'NONE',  ( 35.93744661969999754, 1433.966419429300004, 254.6052924894979697 ) ) ;
#22331=CARTESIAN_POINT ( 'NONE',  ( -27.53546928409999950, 1508.129852613929870, 205.2718258483980094 ) ) ;
#22334=EDGE_CURVE ( 'NONE', #105623, #109427, #34559, .T. ) ;
#22335=CARTESIAN_POINT ( 'NONE',  ( 1.447786046769359292, 1507.396806431331242, 181.1008358461068610 ) ) ;
#22336=CARTESIAN_POINT ( 'NONE',  ( -8.692320600269997755, 1418.992648084129996, 231.7739325360979876 ) ) ;
#22338=CARTESIAN_POINT ( 'NONE',  ( -17.43240527195019851, 1452.304307381109993, 145.9273250573520215 ) ) ;
#22339=CARTESIAN_POINT ( 'NONE',  ( 28.27346568420000139, 1451.774185556130078, 135.7527207400979989 ) ) ;
#22343=CARTESIAN_POINT ( 'NONE',  ( 15.87012503028160282, 1422.606634508830211, 228.1220680369120259 ) ) ;
#22345=ORIENTED_EDGE ( 'NONE', *, *, #24808, .F. ) ;
#22347=CARTESIAN_POINT ( 'NONE',  ( -22.82106830618239712, 1409.719725320740054, 209.4798526508069756 ) ) ;
#22351=CARTESIAN_POINT ( 'NONE',  ( -24.46348847106868618, 1436.579504986744041, 139.1503910763263718 ) ) ;
#22354=CARTESIAN_POINT ( 'NONE',  ( 46.02601385349320395, 1443.739552433979952, 268.2087485089310235 ) ) ;
#22355=B_SPLINE_CURVE_WITH_KNOTS ( 'NONE', 5,
 ( #59148, #37791, #79804, #106631, #72502, #71979, #11490, #54070, #106092, #20959, #37238, #70877, #61916, #55163, #28839, #62475, #87083, #71437 ),
 .UNSPECIFIED., .F., .F.,
 ( 6, 3, 3, 3, 3, 6 ),
 ( 10.40199318109999993, 19.90315615969999996, 26.66638367519999875, 26.99360131220000270, 28.03535140669999848, 29.40431913829999999 ),
 .UNSPECIFIED. ) ;
#22357=CARTESIAN_POINT ( 'NONE',  ( -13.15726442299999910, 1416.543503932829935, 221.9001046233979935 ) ) ;
#22361=CARTESIAN_POINT ( 'NONE',  ( 13.51222313460685776, 1443.793701217813350, 188.0482377676655119 ) ) ;
#22367=CARTESIAN_POINT ( 'NONE',  ( 7.191291722693810229, 1452.661934946750080, 151.5666603189569912 ) ) ;
#22368=B_SPLINE_CURVE_WITH_KNOTS ( 'NONE', 3,
 ( #12699, #89953, #46883, #98900, #81008, #4315, #45783, #22170, #21626, #64791, #88312, #20527, #13227, #47417, #81539, #4840, #36805, #30603, #56368, #201, #77441, #39558, #16388, #31144, #75782, #102601, #42732, #110480, #34324, #76891, #15833, #50583, #16935, #8013, #42180, #26463, #8560, #84166, #94782, #109935, #25347, #17491, #84713, #93653, #60658, #33758, #33213, #94216, #47959, #9127, #51689, #68503, #76330, #67955, #25902, #43293, #742, #67402, #102065, #41628, #59540, #60100, #51137, #85263, #24788, #58990, #82100 ),
 .UNSPECIFIED., .F., .F.,
 ( 4, 3, 3, 3, 3, 3, 3, 3, 3, 3, 3, 3, 3, 3, 3, 3, 3, 3, 3, 3, 3, 3, 4 ),
 ( 75.70921875734188689, 77.32181385522589778, 80.91190279622159665, 84.29463333639999689, 84.51613493880849148, 84.74302641768430533, 84.97629439946371122, 85.21717448936620087, 85.47327895300539069, 85.74291095813249797, 86.03175759668660305, 86.35217251418519879, 86.77738762425410357, 87.13887373325040642, 87.44388152653429813, 87.72348157678361247, 87.98689693641620124, 88.23857955550479915, 88.48405268548279423, 88.71622240253540781, 88.94338408580298960, 89.16444926645201008, 89.22047207541669422 ),
 .UNSPECIFIED. ) ;
#22372=CARTESIAN_POINT ( 'NONE',  ( -10.97588638302280017, 1432.726111932770209, 151.7698415246060222 ) ) ;
#22373=CARTESIAN_POINT ( 'NONE',  ( 0.02589805802711389951, 1409.083993410460153, 232.4593697285492340 ) ) ;
#22374=DIRECTION ( 'NONE',  ( 1.098156484365624113E-07, 0.8818472373848361689, 0.4715352053842007951 ) ) ;
#22378=CARTESIAN_POINT ( 'NONE',  ( 11.74015320060000001, 1428.979986575930070, 144.1938086916980239 ) ) ;
#22380=CARTESIAN_POINT ( 'NONE',  ( 20.41675352909999930, 1440.913060387330006, 219.6133834379979817 ) ) ;
#22383=AXIS2_PLACEMENT_3D ( 'NONE', #81635, #55370, #64881 ) ;
#22388=CARTESIAN_POINT ( 'NONE',  ( 16.81223226430000039, 1414.913060387329779, 210.6693098017280192 ) ) ;
#22389=CARTESIAN_POINT ( 'NONE',  ( -1.669693912109999845, 1443.913060387330006, 150.7596247526980164 ) ) ;
#22391=CARTESIAN_POINT ( 'NONE',  ( -12.78776258895079998, 1416.851343896850040, 195.5391574246120001 ) ) ;
#22392=CARTESIAN_POINT ( 'NONE',  ( 12.85916294179999930, 1469.933320803330162, 268.3665355202980436 ) ) ;
#22393=CARTESIAN_POINT ( 'NONE',  ( 1.228114002177200126, 1450.757138880049979, 181.5372592238319953 ) ) ;
#22397=CARTESIAN_POINT ( 'NONE',  ( 17.08931884779999777, 1422.113171145530032, 226.7814393765980014 ) ) ;
#22398=CARTESIAN_POINT ( 'NONE',  ( 1.188224663175142970, 1410.329429681951297, 232.8079325243718642 ) ) ;
#22400=CARTESIAN_POINT ( 'NONE',  ( -16.19082880930000101, 1409.478456588029985, 225.0103237202980040 ) ) ;
#22401=CARTESIAN_POINT ( 'NONE',  ( -0.4986843622567649348, 1508.982343520079894, 238.8510830230749775 ) ) ;
#22402=CARTESIAN_POINT ( 'NONE',  ( -1.340352705809999989, 1422.344613506229962, 228.3239229121980145 ) ) ;
#22403=CARTESIAN_POINT ( 'NONE',  ( -27.12584415899999968, 1450.023914463320125, 136.5580354838980099 ) ) ;
#22405=CARTESIAN_POINT ( 'NONE',  ( 7.016443067423660379E-06, 1406.952554981560070, 196.1216945173329975 ) ) ;
#22407=CARTESIAN_POINT ( 'NONE',  ( -5.386185223340929973, 1432.347042777500064, 154.6076275972019971 ) ) ;
#22408=CARTESIAN_POINT ( 'NONE',  ( -8.403208055529999498, 1415.931391677329884, 224.9948233075980113 ) ) ;
#22409=CARTESIAN_POINT ( 'NONE',  ( 0.2079255321337470097, 1458.515647613060082, 183.0167680703569886 ) ) ;
#22410=CARTESIAN_POINT ( 'NONE',  ( -9.949544832400000871, 1409.260506149029879, 198.1586515674979978 ) ) ;
#22411=CARTESIAN_POINT ( 'NONE',  ( -0.3212355716730000421, 1418.619114157530021, 184.6997714626980098 ) ) ;
#22412=CARTESIAN_POINT ( 'NONE',  ( -7.701966621347670738, 1441.125018359749902, 154.1230950350289959 ) ) ;
#22413=CARTESIAN_POINT ( 'NONE',  ( 11.94142139689999915, 1433.615122234779847, 147.9453765516980184 ) ) ;
#22414=CARTESIAN_POINT ( 'NONE',  ( -27.69668320559999941, 1436.360686759009923, 136.6994006594979965 ) ) ;
#22421=B_SPLINE_CURVE_WITH_KNOTS ( 'NONE', 3,
 ( #69853, #110717, #26704, #987, #77136, #1530, #60901, #102305, #441, #34008, #95026, #18296, #35112, #102848, #52489, #60332, #94448, #17727, #51929, #25592, #103971, #9367, #68202, #77674, #50818, #27268, #61451, #68745, #95575, #26141, #50288, #67637, #84417, #7702, #41861, #16622, #84949, #76014 ),
 .UNSPECIFIED., .F., .F.,
 ( 4, 2, 2, 1, 1, 1, 1, 2, 2, 2, 1, 1, 1, 1, 2, 2, 2, 2, 2, 2, 2, 2, 4 ),
 ( 0.000000000000000000, 0.2499999999998901989, 0.3749999999998352984, 0.4374999999998089306, 0.4687499999997937761, 0.4843749999997875033, 0.4921874999997847278, 0.4960937499997840616, 0.4999999999997833955, 0.6249999999998385736, 0.6874999999998663291, 0.7187499999998795408, 0.7343749999998852029, 0.7421874999998882005, 0.7460937499998898659, 0.7499999999998916422, 0.8124999999999265032, 0.8437499999999439337, 0.8593749999999512612, 0.8671874999999549249, 0.8710937499999568123, 0.8749999999999585887, 1.000000000000000000 ),
 .UNSPECIFIED. ) ;
#22424=CARTESIAN_POINT ( 'NONE',  ( 33.05090165468867980, 1417.318103022701280, 269.2938148436854249 ) ) ;
#22425=CARTESIAN_POINT ( 'NONE',  ( 21.31406882950000181, 1471.311257372230102, 210.6477718704180120 ) ) ;
#22427=CARTESIAN_POINT ( 'NONE',  ( 2.500000011050000026, 1436.902470912989884, 183.4044075271980034 ) ) ;
#22430=CARTESIAN_POINT ( 'NONE',  ( -24.89775034519999863, 1442.835538705840008, 210.5176537872779932 ) ) ;
#22431=CARTESIAN_POINT ( 'NONE',  ( -27.78835558220000124, 1451.082283293030059, 136.3521884964980018 ) ) ;
#22432=CARTESIAN_POINT ( 'NONE',  ( -16.57709675719999964, 1409.867837143930046, 226.0335794272980081 ) ) ;
#22435=ORIENTED_EDGE ( 'NONE', *, *, #67787, .T. ) ;
#22439=CARTESIAN_POINT ( 'NONE',  ( 18.53418652026280000, 1507.620785850910124, 188.5293807599879869 ) ) ;
#22441=CARTESIAN_POINT ( 'NONE',  ( -0.1213678470291219974, 1420.435499575030235, 183.0499996374540217 ) ) ;
#22442=CARTESIAN_POINT ( 'NONE',  ( 0.4118372133359999854, 1466.367795784230111, 235.6625353782980028 ) ) ;
#22444=CARTESIAN_POINT ( 'NONE',  ( 21.69352049569999963, 1409.670614816029911, 212.9121036625780050 ) ) ;
#22445=B_SPLINE_SURFACE_WITH_KNOTS ( 'NONE', 3, 1, ( 
 ( #83097, #65759 ),
 ( #31581, #90937 ),
 ( #6933, #74714 ),
 ( #16410, #50604 ) ),
 .UNSPECIFIED., .F., .F., .F.,
 ( 4, 4 ),
 ( 2, 2 ),
 ( 0.000000000000000000, 1.000000000000000000 ),
 ( 0.000000000000000000, 1.000000000000000000 ),
 .UNSPECIFIED. ) ;
#22446=CARTESIAN_POINT ( 'NONE',  ( 0.4512475842468137710, 1450.897302474460503, 181.2782477060373481 ) ) ;
#22454=CARTESIAN_POINT ( 'NONE',  ( -0.9341545002969999789, 1415.826342224429936, 233.3075236840979869 ) ) ;
#22457=CARTESIAN_POINT ( 'NONE',  ( -17.64168070010000022, 1423.919165630929911, 226.5634843356980070 ) ) ;
#22458=ORIENTED_EDGE ( 'NONE', *, *, #88472, .T. ) ;
#22460=CARTESIAN_POINT ( 'NONE',  ( -4.229761814456889368, 1441.533620886849803, 164.9558944606160082 ) ) ;
#22463=ORIENTED_EDGE ( 'NONE', *, *, #7202, .F. ) ;
#22469=CARTESIAN_POINT ( 'NONE',  ( -20.59684415639999955, 1507.762623716630060, 190.3921826403979765 ) ) ;
#22470=CYLINDRICAL_SURFACE ( 'NONE', #59380, 1.436538049339995737 ) ;
#22472=CARTESIAN_POINT ( 'NONE',  ( -24.96771051035950251, 1452.035975450660089, 135.7298172057880095 ) ) ;
#22473=CARTESIAN_POINT ( 'NONE',  ( -11.43735029920000024, 1425.481221014229959, 144.1633320290980009 ) ) ;
#22477=CARTESIAN_POINT ( 'NONE',  ( -40.06284621443700189, 1441.966320483619938, 136.9295851911570026 ) ) ;
#22478=EDGE_LOOP ( 'NONE', ( #29320, #92473, #55179 ) ) ;
#22483=CARTESIAN_POINT ( 'NONE',  ( 14.13769145736555899, 1410.779407556687829, 227.9671458598623701 ) ) ;
#22485=CARTESIAN_POINT ( 'NONE',  ( 0.3000392389890000344, 1450.902582786230141, 181.2594265962979705 ) ) ;
#22486=CARTESIAN_POINT ( 'NONE',  ( -3.343564312049999820, 1485.815321652630018, 182.5922648735979692 ) ) ;
#22487=CARTESIAN_POINT ( 'NONE',  ( -2.500000000000000000, 1439.361286679139994, 161.1256493471019837 ) ) ;
#22491=CARTESIAN_POINT ( 'NONE',  ( -0.9156123448460000702, 1507.627023022429967, 232.0153169555979957 ) ) ;
#22492=CARTESIAN_POINT ( 'NONE',  ( -10.32735784461773498, 1519.913060387329779, 184.1749888460368538 ) ) ;
#22498=CARTESIAN_POINT ( 'NONE',  ( 11.04992432786889900, 1414.913526854310021, 222.2523931539879811 ) ) ;
#22499=CARTESIAN_POINT ( 'NONE',  ( -0.0002245325643044376212, 1452.164049364258972, 153.8748112245245636 ) ) ;
#22501=CARTESIAN_POINT ( 'NONE',  ( -0.2499161997042609884, 1451.685132841090081, 183.0451107522330005 ) ) ;
#22502=CARTESIAN_POINT ( 'NONE',  ( -16.48822391639999907, 1410.861292066530041, 191.6305835189980087 ) ) ;
#22505=CARTESIAN_POINT ( 'NONE',  ( -12.71293088880000077, 1419.901838804629733, 222.1500227018980240 ) ) ;
#22507=CARTESIAN_POINT ( 'NONE',  ( -1.429922479960000103, 1509.031031462129704, 179.3412831849980194 ) ) ;
#22510=CARTESIAN_POINT ( 'NONE',  ( 17.66572951889999743, 1459.830952528330045, 228.2832691448980142 ) ) ;
#22511=CARTESIAN_POINT ( 'NONE',  ( -11.60004869885203682, 1425.704216035731406, 137.2038747579310893 ) ) ;
#22514=CARTESIAN_POINT ( 'NONE',  ( -22.71284877100005772, 1409.706192817229748, 209.1573958980538634 ) ) ;
#22515=CARTESIAN_POINT ( 'NONE',  ( -0.09497152921324419905, 1508.365128300149991, 180.3902598306100060 ) ) ;
#22519=ADVANCED_FACE ( 'NONE', ( #26043 ), #2001, .T. ) ;
#22527=CARTESIAN_POINT ( 'NONE',  ( -11.74544487829999895, 1430.504254567329781, 150.5476776824980334 ) ) ;
#22528=LINE ( 'NONE', #91970, #77254 ) ;
#22529=ADVANCED_FACE ( 'NONE', ( #45664 ), #17085, .T. ) ;
#22533=CARTESIAN_POINT ( 'NONE',  ( 12.09505026880000145, 1446.483279760800087, 187.9542664695979681 ) ) ;
#22534=CARTESIAN_POINT ( 'NONE',  ( -19.83923968069999688, 1457.446133080529989, 225.5370320128979813 ) ) ;
#22536=CARTESIAN_POINT ( 'NONE',  ( -1.674135989289999848, 1484.258142909130129, 182.6938733975980256 ) ) ;
#22537=ORIENTED_EDGE ( 'NONE', *, *, #32170, .F. ) ;
#22539=CARTESIAN_POINT ( 'NONE',  ( 3.414736771379999869, 1406.358550222729946, 269.2903006555980028 ) ) ;
#22542=AXIS2_PLACEMENT_3D ( 'NONE', #56279, #88781, #46798 ) ;
#22543=CARTESIAN_POINT ( 'NONE',  ( 24.15782421630898114, 1436.331097753197355, 213.4530830919744062 ) ) ;
#22548=CARTESIAN_POINT ( 'NONE',  ( -2.500000000000000000, 1448.894380904760055, 155.6080925163979884 ) ) ;
#22549=CARTESIAN_POINT ( 'NONE',  ( -1.589333880778387442, 1451.431681818979996, 183.9171754951539981 ) ) ;
#22550=CARTESIAN_POINT ( 'NONE',  ( 12.94448954231350868, 1511.163060387329779, 232.8165751327380519 ) ) ;
#22555=CARTESIAN_POINT ( 'NONE',  ( -21.13431252044160047, 1409.651086843229905, 211.8287216663260040 ) ) ;
#22556=CARTESIAN_POINT ( 'NONE',  ( -7.073260216319999572, 1475.574671051529776, 267.2142456188980191 ) ) ;
#22557=CARTESIAN_POINT ( 'NONE',  ( -4.247024088876750092, 1446.448240483110112, 161.6103351768979906 ) ) ;
#22558=CARTESIAN_POINT ( 'NONE',  ( -6.522631655713630572, 1422.592458550150013, 144.1528597353479881 ) ) ;
#22559=CARTESIAN_POINT ( 'NONE',  ( 17.75177446265830028, 1414.289121907220078, 223.7769287431660246 ) ) ;
#22566=CARTESIAN_POINT ( 'NONE',  ( -22.69629448799999949, 1411.065802167830043, 203.8940129321279926 ) ) ;
#22567=CARTESIAN_POINT ( 'NONE',  ( -15.65146756583599874, 1421.348246145913890, 227.1285423004100039 ) ) ;
#22568=CARTESIAN_POINT ( 'NONE',  ( 19.46330959930472204, 1455.604926216044305, 225.6731016573391457 ) ) ;
#22569=ORIENTED_EDGE ( 'NONE', *, *, #27503, .F. ) ;
#22570=EDGE_CURVE ( 'NONE', #43475, #18765, #9275, .T. ) ;
#22581=CARTESIAN_POINT ( 'NONE',  ( -6.232532191338900240, 1398.098440470949981, 197.7132727547819968 ) ) ;
#22586=CARTESIAN_POINT ( 'NONE',  ( 21.37693747720000204, 1440.913060387330006, 224.8635562088979896 ) ) ;
#22588=ORIENTED_EDGE ( 'NONE', *, *, #61063, .T. ) ;
#22589=B_SPLINE_CURVE_WITH_KNOTS ( 'NONE', 3,
 ( #53875, #10174, #1240, #77933, #18553, #79606, #53305, #78491 ),
 .UNSPECIFIED., .F., .F.,
 ( 4, 2, 2, 4 ),
 ( -0.07674005832873599664, -0.05880084693797370254, -0.03415900950112209927, -1.075081518253639956E-08 ),
 .UNSPECIFIED. ) ;
#22591=CARTESIAN_POINT ( 'NONE',  ( -8.482826003179999574, 1397.255022998529967, 199.1539838373379894 ) ) ;
#22592=CARTESIAN_POINT ( 'NONE',  ( -22.53878036859999767, 1411.058442714630019, 212.0450777197879972 ) ) ;
#22594=CARTESIAN_POINT ( 'NONE',  ( -12.89659922727121177, 1444.936763667012883, 169.4369277064754726 ) ) ;
#22595=CARTESIAN_POINT ( 'NONE',  ( -24.68679851519999957, 1508.521770562530037, 197.5360056163980005 ) ) ;
#22598=CARTESIAN_POINT ( 'NONE',  ( -1.356522590142140050, 1410.335674017130032, 185.6037846924129724 ) ) ;
#22599=CARTESIAN_POINT ( 'NONE',  ( 5.358763871729999906, 1429.765654666730143, 185.6049313592980070 ) ) ;
#22600=CARTESIAN_POINT ( 'NONE',  ( -12.26986021650000147, 1416.828040557830036, 194.6643751810979950 ) ) ;
#22601=DIRECTION ( 'NONE',  ( 0.1402804634180424004, 0.9901118076173111016, 0.000000000000000000 ) ) ;
#22602=CARTESIAN_POINT ( 'NONE',  ( 10.61042346008030179, 1396.283584539540016, 212.2790510548149996 ) ) ;
#22603=CARTESIAN_POINT ( 'NONE',  ( 14.37881581500380079, 1416.259629948840029, 196.9329869028040036 ) ) ;
#22604=CARTESIAN_POINT ( 'NONE',  ( 11.73075292130000058, 1429.442647445629973, 150.1417213462979987 ) ) ;
#22605=CARTESIAN_POINT ( 'NONE',  ( 8.127041000494140022, 1509.197164375159218, 180.9360732693761804 ) ) ;
#22608=CARTESIAN_POINT ( 'NONE',  ( 2.151265163027241911, 1450.023995276909773, 182.0536789941844802 ) ) ;
#22621=CARTESIAN_POINT ( 'NONE',  ( -2.966095081577469816, 1509.131301283620132, 179.1608205533310070 ) ) ;
#22623=B_SPLINE_CURVE_WITH_KNOTS ( 'NONE', 5,
 ( #71597, #104597, #97834, #106251, #21112, #20565 ),
 .UNSPECIFIED., .F., .F.,
 ( 6, 6 ),
 ( 0.000000000000000000, 1.000000000000000000 ),
 .UNSPECIFIED. ) ;
#22625=VERTEX_POINT ( 'NONE', #88195 ) ;
#22627=CARTESIAN_POINT ( 'NONE',  ( -19.86733818529999951, 1508.094164518030084, 229.2433209336980156 ) ) ;
#22628=CARTESIAN_POINT ( 'NONE',  ( -17.58753714432851822, 1413.209790116180329, 269.3766082286189203 ) ) ;
#22629=CARTESIAN_POINT ( 'NONE',  ( -2.179564447600000232, 1409.156885224530015, 232.1843940729979749 ) ) ;
#22630=CARTESIAN_POINT ( 'NONE',  ( -3.820317395759999561E-10, 1453.313060387329870, 189.4452657542980205 ) ) ;
#22632=CARTESIAN_POINT ( 'NONE',  ( 2.500000000000000000, 1427.007219668030075, 156.3926178584979994 ) ) ;
#22633=CARTESIAN_POINT ( 'NONE',  ( -29.42918164984530094, 1440.913060386839788, 236.4667028220079885 ) ) ;
#22634=B_SPLINE_CURVE_WITH_KNOTS ( 'NONE', 5,
 ( #58203, #76102, #26230, #60420, #59865, #25672, #42490, #15603, #110797, #49807, #100725, #58748, #7240, #34089, #41400, #68282, #8876, #102390, #109700, #50367, #93990, #3282, #63201, #104053, #97308, #88365, #44727, #77759, #71045, #35196, #1068, #69382, #78878, #103490, #2183, #37411, #29016, #2731, #60983 ),
 .UNSPECIFIED., .F., .F.,
 ( 6, 3, 3, 3, 3, 3, 3, 3, 3, 3, 3, 3, 6 ),
 ( 0.000000000000000000, 0.01986406830872220960, 0.03714071196419825582, 0.05441735561967429857, 0.08897064292978833222, 0.1583566291595912279, 0.2277426153893942207, 0.5076826711937041381, 0.6470691381323538938, 0.7864556050751944083, 0.8932279473768452993, 0.9466141185318610596, 1.000000000000000000 ),
 .UNSPECIFIED. ) ;
#22637=DIRECTION ( 'NONE',  ( 0.000000000000000000, 0.000000000000000000, -1.000000000000000000 ) ) ;
#22638=CARTESIAN_POINT ( 'NONE',  ( 6.215215835796609412, 1410.569368109790048, 269.6190100981399951 ) ) ;
#22640=CARTESIAN_POINT ( 'NONE',  ( 24.11333318339999821, 1410.980709295929955, 209.4832115230679790 ) ) ;
#22641=CARTESIAN_POINT ( 'NONE',  ( -20.70700216050000009, 1509.300535355729835, 188.9489426423980092 ) ) ;
#22644=EDGE_CURVE ( 'NONE', #61380, #110254, #37153, .T. ) ;
#22646=ADVANCED_FACE ( 'NONE', ( #13647 ), #38320, .T. ) ;
#22648=CARTESIAN_POINT ( 'NONE',  ( 0.1896301300600000128, 1420.480785433730034, 182.7505287346979799 ) ) ;
#22649=CARTESIAN_POINT ( 'NONE',  ( 9.459682105082901415, 1424.144415159054688, 137.0999999983294231 ) ) ;
#22658=ADVANCED_FACE ( 'NONE', ( #72499 ), #101110, .T. ) ;
#22659=CARTESIAN_POINT ( 'NONE',  ( -8.373664085718591110, 1414.913060387329779, 223.0268086914393848 ) ) ;
#22660=CARTESIAN_POINT ( 'NONE',  ( -5.392699262009999828, 1433.241572010809932, 154.6274253439979987 ) ) ;
#22669=VERTEX_POINT ( 'NONE', #104307 ) ;
#22673=CARTESIAN_POINT ( 'NONE',  ( 27.96976553579999702, 1509.201555290030001, 207.5796322327380210 ) ) ;
#22674=CONICAL_SURFACE ( 'NONE', #103099, 18.60900368820000850, 0.6981317007980000211 ) ;
#22675=CARTESIAN_POINT ( 'NONE',  ( 19.44122429240000116, 1456.941909337529978, 224.4539435408979955 ) ) ;
#22676=CARTESIAN_POINT ( 'NONE',  ( 7.872090775853918920, 1438.237761097329212, 153.7477460425555478 ) ) ;
#22678=ADVANCED_FACE ( 'NONE', ( #79127 ), #91257, .F. ) ;
#22680=FACE_OUTER_BOUND ( 'NONE', #97043, .T. ) ;
#22681=CARTESIAN_POINT ( 'NONE',  ( -3.684086113900000292, 1446.644897779309986, 159.4624714679980002 ) ) ;
#22682=CARTESIAN_POINT ( 'NONE',  ( -19.12894962059999671, 1426.100227420630063, 225.4496986463979908 ) ) ;
#22685=CARTESIAN_POINT ( 'NONE',  ( 18.82869366990000159, 1461.938562382830014, 190.8087292768979921 ) ) ;
#22688=CARTESIAN_POINT ( 'NONE',  ( -38.35150357969526169, 1453.387763860978112, 269.5822590821125573 ) ) ;
#22690=CARTESIAN_POINT ( 'NONE',  ( -10.81507089441019964, 1424.921187596680056, 144.1620444830689962 ) ) ;
#22694=CARTESIAN_POINT ( 'NONE',  ( -0.1431367926419999936, 1417.281368496930099, 234.8519457758980309 ) ) ;
#22696=CARTESIAN_POINT ( 'NONE',  ( -13.29029361451234159, 1444.600243103134289, 186.7172809443856920 ) ) ;
#22699=EDGE_CURVE ( 'NONE', #103179, #45409, #67902, .T. ) ;
#22702=CARTESIAN_POINT ( 'NONE',  ( 24.76239166610000098, 1435.860790453759819, 137.6237234474980085 ) ) ;
#22704=CARTESIAN_POINT ( 'NONE',  ( -13.39865269429999906, 1409.380951649529834, 225.6837777353979959 ) ) ;
#22709=ORIENTED_EDGE ( 'NONE', *, *, #61644, .F. ) ;
#22712=CARTESIAN_POINT ( 'NONE',  ( 41.25049345058425132, 1434.982249775052424, 269.6332951576844152 ) ) ;
#22713=CARTESIAN_POINT ( 'NONE',  ( -20.03573726089999596, 1460.150672173630028, 240.3194873113979781 ) ) ;
#22714=CARTESIAN_POINT ( 'NONE',  ( -19.69775028829999997, 1484.707692800029918, 190.1282803529979901 ) ) ;
#22715=CARTESIAN_POINT ( 'NONE',  ( -11.14272688560000013, 1433.633229230830011, 151.6530944731979957 ) ) ;
#22719=CARTESIAN_POINT ( 'NONE',  ( 2.500000000000000000, 1448.210448412289907, 170.6974824052979898 ) ) ;
#22722=CARTESIAN_POINT ( 'NONE',  ( -2.760778634279479782, 1409.009468901610035, 188.0459411385839985 ) ) ;
#22723=B_SPLINE_CURVE_WITH_KNOTS ( 'NONE', 3,
 ( #66506, #14944, #68159, #91670, #100610, #67046, #76521, #102266, #41274, #58635, #23894, #49690, #83819, #75447, #25546, #16044, #50245, #51317, #84374, #102803, #68698, #44037, #35070, #2609, #87704, #87134, #51889, #105045 ),
 .UNSPECIFIED., .F., .F.,
 ( 4, 3, 3, 3, 3, 3, 3, 3, 3, 4 ),
 ( 11.45157243117470003, 11.57484800204929876, 11.69873572308700105, 11.82299213567229934, 11.94767712729789899, 12.07285275658629864, 12.19896151394710060, 12.32556630458410041, 12.45304517163829949, 12.51194700650879987 ),
 .UNSPECIFIED. ) ;
#22725=CARTESIAN_POINT ( 'NONE',  ( -19.52630014007766945, 1509.713547991464338, 231.9178196453461283 ) ) ;
#22727=CARTESIAN_POINT ( 'NONE',  ( 1.447894037093860002E-08, 1408.513036702840054, 261.9187567895989446 ) ) ;
#22730=CARTESIAN_POINT ( 'NONE',  ( -11.86282332673470030, 1432.107038623590142, 149.9775339942419805 ) ) ;
#22733=CARTESIAN_POINT ( 'NONE',  ( -7.478702111819999665, 1472.804222987030016, 270.4228357808979695 ) ) ;
#22736=CARTESIAN_POINT ( 'NONE',  ( 35.10549739602630126, 1450.762126806190054, 136.1476404445799915 ) ) ;
#22737=CARTESIAN_POINT ( 'NONE',  ( 0.2070356852857530017, 1452.599831121419811, 183.2333262594050041 ) ) ;
#22742=CARTESIAN_POINT ( 'NONE',  ( -39.86365974965330139, 1422.738695774160078, 267.1848028950000185 ) ) ;
#22743=VERTEX_POINT ( 'NONE', #51564 ) ;
#22744=CARTESIAN_POINT ( 'NONE',  ( -3.541941751390889959, 1499.841325333280110, 181.2873610080370099 ) ) ;
#22746=AXIS2_PLACEMENT_3D ( 'NONE', #64737, #89899, #38933 ) ;
#22747=VERTEX_POINT ( 'NONE', #76759 ) ;
#22750=CARTESIAN_POINT ( 'NONE',  ( 37.73087422431532190, 1445.052233488290312, 136.8113442565054925 ) ) ;
#22751=DIRECTION ( 'NONE',  ( 0.000000000000000000, 1.000000000000000000, 0.000000000000000000 ) ) ;
#22753=CARTESIAN_POINT ( 'NONE',  ( -14.39948585115419988, 1509.538292535830124, 182.8035031149169924 ) ) ;
#22754=CARTESIAN_POINT ( 'NONE',  ( -16.26535344460000232, 1425.423310974930018, 190.7822913542979961 ) ) ;
#22755=DIRECTION ( 'NONE',  ( 0.000000000000000000, -1.000000000000000000, 0.000000000000000000 ) ) ;
#22756=VERTEX_POINT ( 'NONE', #59427 ) ;
#22757=CARTESIAN_POINT ( 'NONE',  ( -26.49906707450000098, 1436.567897694819976, 136.7771845898980132 ) ) ;
#22760=DIRECTION ( 'NONE',  ( -1.000000000000000000, 0.000000000000000000, 0.000000000000000000 ) ) ;
#22762=CARTESIAN_POINT ( 'NONE',  ( -40.78591513166909976, 1431.459864284900050, 269.6245610256719942 ) ) ;
#22764=CARTESIAN_POINT ( 'NONE',  ( -6.220302149359999255, 1397.477102017430070, 197.7753768589980155 ) ) ;
#22765=EDGE_CURVE ( 'NONE', #22209, #66863, #31772, .T. ) ;
#22768=VERTEX_POINT ( 'NONE', #87372 ) ;
#22769=CARTESIAN_POINT ( 'NONE',  ( 0.2381205061309999982, 1451.685209519130240, 183.0508848106979940 ) ) ;
#22777=CARTESIAN_POINT ( 'NONE',  ( 5.510117011110000185, 1440.199971711730086, 154.7606381671979818 ) ) ;
#22779=CARTESIAN_POINT ( 'NONE',  ( 18.80464302510000252, 1425.801049065629968, 225.6039134470979945 ) ) ;
#22784=CARTESIAN_POINT ( 'NONE',  ( -40.71747595839300260, 1448.637563203250011, 135.3761645363250068 ) ) ;
#22785=CARTESIAN_POINT ( 'NONE',  ( -11.16222505900650042, 1428.970455565040083, 101.8803122854220078 ) ) ;
#22786=CARTESIAN_POINT ( 'NONE',  ( -12.78776258889159934, 1416.851343895820037, 195.9645815067300134 ) ) ;
#22789=EDGE_CURVE ( 'NONE', #28487, #25667, #104163, .T. ) ;
#22790=CARTESIAN_POINT ( 'NONE',  ( 12.57551620087889788, 1435.697644940459895, 150.8998391666309828 ) ) ;
#22791=CARTESIAN_POINT ( 'NONE',  ( 14.04614445250000188, 1415.579607678529783, 197.0459619348980027 ) ) ;
#22793=CARTESIAN_POINT ( 'NONE',  ( -11.43993018048137245, 1425.780984131823061, 139.0081881035810341 ) ) ;
#22797=CARTESIAN_POINT ( 'NONE',  ( 23.15864443164504394, 1450.075779451102335, 217.7010643741785145 ) ) ;
#22798=ADVANCED_FACE ( 'NONE', ( #8994 ), #22307, .T. ) ;
#22800=CARTESIAN_POINT ( 'NONE',  ( 2.500000000000000000, 1439.588444383649858, 166.1975927366900123 ) ) ;
#22801=DIRECTION ( 'NONE',  ( -1.000000000000000000, 0.000000000000000000, 0.000000000000000000 ) ) ;
#22803=EDGE_LOOP ( 'NONE', ( #11524, #21066, #53449, #97053 ) ) ;
#22805=CARTESIAN_POINT ( 'NONE',  ( -20.94370973279999859, 1470.568016209030020, 270.0430967339979702 ) ) ;
#22806=CARTESIAN_POINT ( 'NONE',  ( -4.161387699379999638, 1448.641049173779948, 185.0955448841980342 ) ) ;
#22808=EDGE_CURVE ( 'NONE', #97581, #48553, #54420, .T. ) ;
#22809=CARTESIAN_POINT ( 'NONE',  ( 2.453594186590829734E-14, 1422.045703570280011, 122.9812613506829990 ) ) ;
#22811=CARTESIAN_POINT ( 'NONE',  ( 18.85256022773900142, 1509.571403847920010, 185.0368585482190156 ) ) ;
#22812=CARTESIAN_POINT ( 'NONE',  ( 11.60004869885216472, 1425.961673676839155, 138.7012799492945305 ) ) ;
#22813=CARTESIAN_POINT ( 'NONE',  ( 2.543548742221767966, 1417.726526468788506, 233.7963267752078877 ) ) ;
#22814=CARTESIAN_POINT ( 'NONE',  ( -2.640038298730670085, 1471.339824109930078, 183.8587828106460336 ) ) ;
#22816=CARTESIAN_POINT ( 'NONE',  ( 6.823004602010799484E-10, 1406.914363899970112, 222.1218459632040094 ) ) ;
#22817=CARTESIAN_POINT ( 'NONE',  ( 31.90208977857959738, 1440.913060383340053, 243.8577475931840013 ) ) ;
#22818=SPHERICAL_SURFACE ( 'NONE', #80520, 2.000000000000000000 ) ;
#22819=FACE_BOUND ( 'NONE', #25755, .T. ) ;
#22821=EDGE_LOOP ( 'NONE', ( #91526, #87664, #98159, #85220 ) ) ;
#22824=CARTESIAN_POINT ( 'NONE',  ( 13.51610093808349866, 1443.913060387330006, 206.7785865123599933 ) ) ;
#22826=CARTESIAN_POINT ( 'NONE',  ( 3.034663161748390348, 1440.440203176670138, 157.2490260270419924 ) ) ;
#22828=CARTESIAN_POINT ( 'NONE',  ( -1.546867746862319981, 1416.839692133689823, 228.0214409764060122 ) ) ;
#22837=CARTESIAN_POINT ( 'NONE',  ( -12.78776258900000151, 1416.851343898729965, 195.5391574245979882 ) ) ;
#22839=CARTESIAN_POINT ( 'NONE',  ( 2.745794554380000196, 1464.572481067230001, 236.3736730967980009 ) ) ;
#22845=CARTESIAN_POINT ( 'NONE',  ( -18.12896501130950000, 1435.130582088173014, 143.3945274439228683 ) ) ;
#22846=ORIENTED_EDGE ( 'NONE', *, *, #67347, .F. ) ;
#22848=CARTESIAN_POINT ( 'NONE',  ( 0.5624690339869999889, 1416.828040475229955, 190.4759594386979984 ) ) ;
#22849=CARTESIAN_POINT ( 'NONE',  ( 34.03221148485429381, 1437.015149023179902, 136.5575608309000017 ) ) ;
#22851=CARTESIAN_POINT ( 'NONE',  ( -11.60004869885204037, 1426.466820350880425, 135.9733956539067492 ) ) ;
#22852=B_SPLINE_CURVE_WITH_KNOTS ( 'NONE', 5,
 ( #17589, #61321, #9768, #9230, #78078, #76989 ),
 .UNSPECIFIED., .F., .F.,
 ( 6, 6 ),
 ( -2.000000000000000000, -3.790778899670499413E-06 ),
 .UNSPECIFIED. ) ;
#22854=CARTESIAN_POINT ( 'NONE',  ( -12.27608956948616026, 1509.341750881446160, 235.6884000609552174 ) ) ;
#22857=CARTESIAN_POINT ( 'NONE',  ( 5.533180669438849897, 1409.106283314009943, 195.2035214513250025 ) ) ;
#22858=CARTESIAN_POINT ( 'NONE',  ( 18.12085357038199973, 1425.008622401126104, 225.3887946363380195 ) ) ;
#22860=CARTESIAN_POINT ( 'NONE',  ( -18.77987601960000319, 1452.005536572529991, 191.4523375352979997 ) ) ;
#22861=CARTESIAN_POINT ( 'NONE',  ( -2.549034377637660054, 1448.919557215109990, 183.6707458025049959 ) ) ;
#22862=ORIENTED_EDGE ( 'NONE', *, *, #13885, .T. ) ;
#22865=CARTESIAN_POINT ( 'NONE',  ( 19.30835196975910151, 1456.473163433020090, 228.7023210262429984 ) ) ;
#22866=CARTESIAN_POINT ( 'NONE',  ( -12.03079994940000041, 1433.765461728309901, 150.2535422845980122 ) ) ;
#22867=CARTESIAN_POINT ( 'NONE',  ( 2.442485525661060236E-10, 1465.745499712829996, 240.5333668247809840 ) ) ;
#22873=CARTESIAN_POINT ( 'NONE',  ( -46.02294315243130285, 1440.251626319409979, 268.4962080042990351 ) ) ;
#22879=( LENGTH_UNIT ( ) NAMED_UNIT ( * ) SI_UNIT ( .MILLI., .METRE. ) );
#22883=CARTESIAN_POINT ( 'NONE',  ( 33.33289073430000116, 1436.626756256089948, 248.0947902361980084 ) ) ;
#22885=CARTESIAN_POINT ( 'NONE',  ( -0.5073518436949999710, 1478.157470870929956, 182.0636189244980017 ) ) ;
#22887=CARTESIAN_POINT ( 'NONE',  ( 1.585275487640332992, 1508.725511249230976, 180.2575163523052311 ) ) ;
#22888=CARTESIAN_POINT ( 'NONE',  ( -17.22939366680000361, 1424.306326232029960, 225.2395885692979789 ) ) ;
#22891=CARTESIAN_POINT ( 'NONE',  ( -18.52802004830289917, 1452.266047670050057, 144.8817897837620023 ) ) ;
#22892=CARTESIAN_POINT ( 'NONE',  ( 28.26594772519999665, 1451.926830112729931, 135.3157343196979809 ) ) ;
#22896=CARTESIAN_POINT ( 'NONE',  ( 16.72074854044890202, 1422.807583317619901, 227.2334935513920016 ) ) ;
#22897=CARTESIAN_POINT ( 'NONE',  ( -3.931500257436271184, 1448.981219870369159, 185.0407271323569489 ) ) ;
#22902=CARTESIAN_POINT ( 'NONE',  ( -24.08818477799610136, 1410.733297714309856, 209.1412261076660002 ) ) ;
#22903=ORIENTED_EDGE ( 'NONE', *, *, #505, .F. ) ;
#22907=AXIS2_PLACEMENT_3D ( 'NONE', #75629, #102448, #16767 ) ;
#22908=CARTESIAN_POINT ( 'NONE',  ( -0.6048355684939999977, 1507.643512198230155, 237.2981531702980078 ) ) ;
#22909=CARTESIAN_POINT ( 'NONE',  ( -17.38482318170000340, 1410.884444280730122, 225.7833539147979707 ) ) ;
#22910=AXIS2_PLACEMENT_3D ( 'NONE', #10705, #28040, #1209 ) ;
#22911=CARTESIAN_POINT ( 'NONE',  ( 45.23891030401149749, 1446.067212034520026, 266.2005835343620106 ) ) ;
#22913=CARTESIAN_POINT ( 'NONE',  ( -0.04185304873460000269, 1420.435852020029870, 183.3187823327980084 ) ) ;
#22917=CIRCLE ( 'NONE', #108794, 41.35631769782009570 ) ;
#22919=CARTESIAN_POINT ( 'NONE',  ( 12.86933871999277734, 1442.875697286375271, 186.9746649412792863 ) ) ;
#22920=VERTEX_POINT ( 'NONE', #94095 ) ;
#22925=CARTESIAN_POINT ( 'NONE',  ( -4.263034242833646736, 1424.151093693061966, 185.2294109041083345 ) ) ;
#22926=B_SPLINE_CURVE_WITH_KNOTS ( 'NONE', 3,
 ( #69802, #70358, #27765, #80384, #105030, #103920, #36721, #44581, #89327, #61956, #96071, #70914, #19905, #1475, #88235, #11526, #79840, #37280, #63073, #37828, #106132, #29405, #97725, #106671, #107782, #65794, #92081, #66361, #107228, #100480, #91536, #5880, #90972, #83134, #13693, #6430, #47878, #65247, #73650, #23762, #29960, #64153, #40575, #15356, #82589, #74745, #22633, #31067, #108334, #57949, #13143, #82016, #56282, #49001, #80931, #38362, #98825, #108884, #55756, #47327, #32177, #74203, #4229, #90413, #73088, #72540, #81457, #98272, #40024, #21544, #22086, #99916, #4762, #5321, #99359, #56839, #39480, #31617, #23211, #48451, #14261, #57411, #14814, #89874, #38906, #30518, #64708, #1954, #35524, #3064, #79757, #36092, #10890, #70832, #37192, #27136, #97099, #94883, #104942, #1382, #88154, #18160, #9769, #62989, #70278, #2512, #36636, #19251, #43935, #44494, #11442, #95985, #104387, #52357, #28232, #86474, #62420, #60759, #27684, #53457, #69717, #87601, #103836, #19819, #45617, #71386, #28791, #96545, #54026, #103255, #105499, #78638, #61322, #46169, #20364, #61868, #79206, #11985, #54571 ),
 .UNSPECIFIED., .F., .F.,
 ( 4, 3, 3, 3, 3, 3, 3, 3, 3, 3, 3, 3, 3, 3, 3, 3, 3, 3, 3, 3, 3, 3, 3, 3, 3, 3, 3, 3, 3, 3, 3, 3, 3, 3, 3, 3, 3, 3, 3, 3, 3, 3, 3, 3, 3, 3, 4 ),
 ( -29.89576149997330035, -27.93066200461270299, -25.77370346504809717, -23.34209498118620019, -21.15356506553399996, -19.17231324189400254, -17.32574871330879773, -15.57444149077680073, -13.93194560254629977, -12.30963008990289964, -10.75531893239759995, -9.233619782032960188, -7.754183433082701526, -6.990622735083189099, -5.857671294819962071, -4.582768379358419963, -3.327899758805628494, -2.055712155490059700, -0.7650328573970526236, 0.5655583436393420982, 1.790039819582720071, 3.161605655697446338, 4.341552028872310842, 5.758073910464208467, 7.176843838457021008, 8.662804671664009248, 10.14364948196800142, 11.62076542165629789, 13.16096764701680044, 14.68906546968660010, 15.67372708160739947, 16.66824346166319870, 17.65430721703309658, 18.64662466131919771, 19.64424912027570613, 20.64604275194010441, 21.65069957589760108, 22.65678741700699916, 23.66280606768819794, 24.66584900615290010, 25.66547144059130758, 26.66059974112859621, 27.65030847251239621, 28.63422864500930487, 29.60788831232530427, 30.59693873741260361, 31.58598916250000244 ),
 .UNSPECIFIED. ) ;
#22928=EDGE_CURVE ( 'NONE', #109266, #68079, #102557, .T. ) ;
#22933=CARTESIAN_POINT ( 'NONE',  ( 0.03684459895644798949, 1409.761386472454660, 233.0934521079545334 ) ) ;
#22934=CARTESIAN_POINT ( 'NONE',  ( -13.09172112396450061, 1434.821155476560079, 149.0943168348729841 ) ) ;
#22939=CARTESIAN_POINT ( 'NONE',  ( -24.77531906373999959, 1509.438340469299874, 222.6714807735559987 ) ) ;
#22941=ORIENTED_EDGE ( 'NONE', *, *, #58529, .T. ) ;
#22942=CARTESIAN_POINT ( 'NONE',  ( 19.00000000000000000, 1440.913060387330006, 209.1218459616979999 ) ) ;
#22943=DIRECTION ( 'NONE',  ( -1.000000000000000000, 0.000000000000000000, 0.000000000000000000 ) ) ;
#22949=ORIENTED_EDGE ( 'NONE', *, *, #91905, .T. ) ;
#22951=CARTESIAN_POINT ( 'NONE',  ( -5.551115123129999164E-15, 1443.913060387330006, 150.8032249175980155 ) ) ;
#22952=CARTESIAN_POINT ( 'NONE',  ( -14.20204673689999986, 1416.837080247930089, 221.7382503592980072 ) ) ;
#22953=CARTESIAN_POINT ( 'NONE',  ( 11.29458427579999835, 1433.957910099769833, 151.5308368996980164 ) ) ;
#22954=CARTESIAN_POINT ( 'NONE',  ( 42.15865170690000241, 1450.809155637750109, 271.1218459616979999 ) ) ;
#22955=CARTESIAN_POINT ( 'NONE',  ( 12.77961858748670032, 1414.913057834419988, 198.0260298875460023 ) ) ;
#22956=CARTESIAN_POINT ( 'NONE',  ( 0.003568499702431209702, 1467.142144108200000, 235.6416276161930057 ) ) ;
#22960=DIRECTION ( 'NONE',  ( 0.000000000000000000, 1.000000000000000000, 0.000000000000000000 ) ) ;
#22962=CARTESIAN_POINT ( 'NONE',  ( -17.67161397030000103, 1410.454767058429979, 225.2840158849979844 ) ) ;
#22963=EDGE_CURVE ( 'NONE', #8806, #71548, #72406, .T. ) ;
#22964=EDGE_CURVE ( 'NONE', #15749, #94550, #11638, .T. ) ;
#22967=CARTESIAN_POINT ( 'NONE',  ( -17.48733164209449953, 1410.446457955379856, 192.6364576323030064 ) ) ;
#22969=CARTESIAN_POINT ( 'NONE',  ( 11.14671379024469999, 1434.019377051509991, 151.6529839732360188 ) ) ;
#22971=EDGE_CURVE ( 'NONE', #50075, #76159, #10354, .T. ) ;
#22972=CARTESIAN_POINT ( 'NONE',  ( -8.506178470120000057, 1416.518532928330160, 225.1689260078979657 ) ) ;
#22973=CARTESIAN_POINT ( 'NONE',  ( 0.2127819998068850027, 1455.787616099680008, 183.1338090387140198 ) ) ;
#22975=CARTESIAN_POINT ( 'NONE',  ( -9.972378110560478959, 1407.313660260299912, 200.5612547303060182 ) ) ;
#22978=CARTESIAN_POINT ( 'NONE',  ( -29.17496190384160215, 1509.931872506899936, 211.7252048115940113 ) ) ;
#22979=CARTESIAN_POINT ( 'NONE',  ( 13.19869229439999891, 1434.900411147940304, 148.5018195976979882 ) ) ;
#22980=CARTESIAN_POINT ( 'NONE',  ( -36.70996913416379925, 1436.286710641700211, 134.0999999969339740 ) ) ;
#22984=CARTESIAN_POINT ( 'NONE',  ( -3.034143074970000242, 1440.440281792710039, 157.2495483846980164 ) ) ;
#22988=CARTESIAN_POINT ( 'NONE',  ( 16.41933790207369981, 1509.448631503890056, 232.9213397454749952 ) ) ;
#22989=CARTESIAN_POINT ( 'NONE',  ( 44.41513596800174923, 1432.959676725966801, 269.0091301501007592 ) ) ;
#22993=LINE ( 'NONE', #99149, #9680 ) ;
#22996=CARTESIAN_POINT ( 'NONE',  ( -24.61293950550089704, 1444.770188684140066, 210.8869336946189890 ) ) ;
#22998=AXIS2_PLACEMENT_3D ( 'NONE', #1181, #1736, #96326 ) ;
#23000=CARTESIAN_POINT ( 'NONE',  ( -15.83424720296929600, 1409.491973313159860, 225.5800623810480090 ) ) ;
#23001=CARTESIAN_POINT ( 'NONE',  ( 0.4872611956131389643, 1418.409299200879786, 184.7253510064639954 ) ) ;
#23003=CARTESIAN_POINT ( 'NONE',  ( -14.12786062849999880, 1509.345507838329922, 183.3895953394980154 ) ) ;
#23005=CARTESIAN_POINT ( 'NONE',  ( 40.26684313263383785, 1444.090643208445044, 137.1176951931856252 ) ) ;
#23006=CARTESIAN_POINT ( 'NONE',  ( 22.52609172630000245, 1509.699688844029879, 227.3081661019980118 ) ) ;
#23008=CARTESIAN_POINT ( 'NONE',  ( -0.07668964449979870368, 1420.270968488830249, 183.5370586615759976 ) ) ;
#23009=CARTESIAN_POINT ( 'NONE',  ( 1.300999044849999953, 1466.796436742230071, 235.1605608302979817 ) ) ;
#23010=CARTESIAN_POINT ( 'NONE',  ( 20.88842237349999920, 1409.642500170129779, 215.0570138386379710 ) ) ;
#23011=CARTESIAN_POINT ( 'NONE',  ( -0.03822279852769269737, 1452.916107821060223, 185.2425342979790059 ) ) ;
#23013=CARTESIAN_POINT ( 'NONE',  ( -16.85198166820000054, 1421.787005334130072, 226.9070353815980070 ) ) ;
#23015=CARTESIAN_POINT ( 'NONE',  ( 22.04844205597441231, 1506.512156832560095, 209.0500279883449934 ) ) ;
#23018=CARTESIAN_POINT ( 'NONE',  ( 21.39771952614790251, 1509.704955107219803, 188.4542851670070149 ) ) ;
#23019=CARTESIAN_POINT ( 'NONE',  ( -1.108882943119999798, 1417.340802340130040, 234.6777931048980008 ) ) ;
#23023=DIRECTION ( 'NONE',  ( -0.3741289577892935592, 0.04424996905086078791, 0.9263203890568829646 ) ) ;
#23026=CARTESIAN_POINT ( 'NONE',  ( -4.247058430120979722, 1441.377667071719998, 161.6040409347519926 ) ) ;
#23029=VERTEX_POINT ( 'NONE', #75943 ) ;
#23034=CARTESIAN_POINT ( 'NONE',  ( -11.44198449339859636, 1425.478516144404239, 144.4778108111833035 ) ) ;
#23035=CARTESIAN_POINT ( 'NONE',  ( 15.77937509389199988, 1409.566674589380000, 192.3662456604770341 ) ) ;
#23039=CARTESIAN_POINT ( 'NONE',  ( -0.4018488818434700072, 1508.986311531569754, 179.3607565668060033 ) ) ;
#23040=CARTESIAN_POINT ( 'NONE',  ( 17.03742609228944715, 1460.377087626990487, 228.7183869844807589 ) ) ;
#23043=CARTESIAN_POINT ( 'NONE',  ( -39.86280671402410292, 1441.327267167989930, 136.8612332179159807 ) ) ;
#23047=ORIENTED_EDGE ( 'NONE', *, *, #79743, .T. ) ;
#23048=CARTESIAN_POINT ( 'NONE',  ( 12.99443939928278979, 1410.739937348442027, 228.5427893857089998 ) ) ;
#23050=CARTESIAN_POINT ( 'NONE',  ( 0.1984587786619999850, 1451.686688576329971, 183.0460370019980019 ) ) ;
#23052=CARTESIAN_POINT ( 'NONE',  ( -2.500000000000000000, 1439.495310554470052, 163.5954663552189743 ) ) ;
#23054=CARTESIAN_POINT ( 'NONE',  ( 11.79480876540000089, 1441.728078750129953, 187.9005510439980071 ) ) ;
#23055=CARTESIAN_POINT ( 'NONE',  ( 36.37832870499009630, 1451.642701156129988, 135.0591089792199853 ) ) ;
#23057=CARTESIAN_POINT ( 'NONE',  ( 25.79236023700000047, 1440.625197361159962, 138.3752390835979895 ) ) ;
#23058=CARTESIAN_POINT ( 'NONE',  ( 0.9908529825249998702, 1414.913060387329779, 192.1420427703979783 ) ) ;
#23060=ORIENTED_EDGE ( 'NONE', *, *, #2427, .F. ) ;
#23064=CARTESIAN_POINT ( 'NONE',  ( 33.71823238038290071, 1440.913060387330006, 258.8638944021930115 ) ) ;
#23065=VECTOR ( 'NONE', #4705, 1000.000000000000227 ) ;
#23066=CARTESIAN_POINT ( 'NONE',  ( -0.002575616544385699036, 1451.742099234649004, 154.0620397922272105 ) ) ;
#23067=ORIENTED_EDGE ( 'NONE', *, *, #68464, .F. ) ;
#23071=CARTESIAN_POINT ( 'NONE',  ( -15.77403878809999860, 1409.463901959830082, 192.8704306968979836 ) ) ;
#23072=DIRECTION ( 'NONE',  ( 0.000000000000000000, -1.000000000000000000, 0.000000000000000000 ) ) ;
#23074=CARTESIAN_POINT ( 'NONE',  ( 21.30389884161289871, 1409.667087122100156, 206.3896467061680369 ) ) ;
#23076=CARTESIAN_POINT ( 'NONE',  ( -0.7414587291309999717, 1508.588857168030017, 180.2948226304979755 ) ) ;
#23079=CARTESIAN_POINT ( 'NONE',  ( 17.11189916109999842, 1459.589049907830031, 228.7027963470980012 ) ) ;
#23084=ORIENTED_EDGE ( 'NONE', *, *, #86219, .F. ) ;
#23085=AXIS2_PLACEMENT_3D ( 'NONE', #20184, #36441, #79029 ) ;
#23087=CARTESIAN_POINT ( 'NONE',  ( -0.07316533871274499834, 1508.573872468679838, 180.1735049589379969 ) ) ;
#23088=EDGE_CURVE ( 'NONE', #75280, #5728, #102239, .T. ) ;
#23090=CARTESIAN_POINT ( 'NONE',  ( 18.62528357307473925, 1445.660712737476615, 215.1045338314846731 ) ) ;
#23092=CARTESIAN_POINT ( 'NONE',  ( 18.51591337770000223, 1509.559650329829765, 187.1458710574979989 ) ) ;
#23095=ORIENTED_EDGE ( 'NONE', *, *, #91922, .F. ) ;
#23096=CARTESIAN_POINT ( 'NONE',  ( -19.08918019649999920, 1507.695924774130162, 229.6553491538980154 ) ) ;
#23097=CARTESIAN_POINT ( 'NONE',  ( 21.86388809379999998, 1452.023132390130058, 221.6453359476980154 ) ) ;
#23099=CARTESIAN_POINT ( 'NONE',  ( -11.84000682719999986, 1430.430028094429872, 150.0882633680979836 ) ) ;
#23102=CARTESIAN_POINT ( 'NONE',  ( -8.770759252174429504E-15, 1422.771840662260047, 151.0941882234770048 ) ) ;
#23105=CARTESIAN_POINT ( 'NONE',  ( -24.08096867289999565, 1444.797005272369915, 211.7711350123979912 ) ) ;
#23107=CARTESIAN_POINT ( 'NONE',  ( -2.248581038649999808, 1485.570063529730078, 182.6114682650980114 ) ) ;
#23108=AXIS2_PLACEMENT_3D ( 'NONE', #5458, #58631, #73787 ) ;
#23111=CARTESIAN_POINT ( 'NONE',  ( 12.73684339809999955, 1407.027259281629995, 267.7855128373979596 ) ) ;
#23112=CARTESIAN_POINT ( 'NONE',  ( 0.06622282237950000150, 1409.084365868529858, 185.5721059075980008 ) ) ;
#23114=CARTESIAN_POINT ( 'NONE',  ( 24.51223204819740786, 1438.674460532969078, 212.6365892752995421 ) ) ;
#23115=CARTESIAN_POINT ( 'NONE',  ( 12.54766037970713022, 1509.351234348180014, 182.3718845436952734 ) ) ;
#23116=CARTESIAN_POINT ( 'NONE',  ( 28.25086641300000068, 1508.135711190629991, 209.3856964555159834 ) ) ;
#23119=CARTESIAN_POINT ( 'NONE',  ( -1.976367997842130242, 1450.328871335550048, 155.3359410068990201 ) ) ;
#23120=CARTESIAN_POINT ( 'NONE',  ( -1.555918367431536442, 1451.038150671306767, 183.6095956534302900 ) ) ;
#23122=CARTESIAN_POINT ( 'NONE',  ( -14.13162141313859976, 1415.651572961190141, 221.0577713143219967 ) ) ;
#23124=CARTESIAN_POINT ( 'NONE',  ( -9.365681194936280818, 1409.240117181489950, 197.4562387521140181 ) ) ;
#23125=B_SPLINE_SURFACE_WITH_KNOTS ( 'NONE', 5, 5, ( 
 ( #11788, #64963, #81183, #4499, #45956, #63328, #5596, #22357, #99076 ),
 ( #98537, #80093, #3412, #106399, #46515, #73909, #56005, #21805, #38090 ),
 ( #105861, #48161, #82297, #89589, #88504, #99625, #80649, #39746, #29140 ),
 ( #54373, #71744, #38633, #3963, #97983, #97448, #29684, #5034, #73353 ),
 ( #13412, #39178, #108037, #37542, #20715, #90685, #90129, #54911, #31332 ),
 ( #13973, #64416, #12325, #65518, #89037, #107489, #72265, #72809, #106939 ) ),
 .UNSPECIFIED., .F., .F., .F.,
 ( 6, 6 ),
 ( 6, 3, 6 ),
 ( 0.4666582265190000189, 2.797885342507290041 ),
 ( -1.082961728884700041E-05, 1.000000000000000000, 2.000000000000000000 ),
 .UNSPECIFIED. ) ;
#23127=CARTESIAN_POINT ( 'NONE',  ( 3.115557368589999765, 1441.255753523060093, 168.7233852534980088 ) ) ;
#23128=CARTESIAN_POINT ( 'NONE',  ( -2.101430478369999744, 1475.725219423630051, 269.0439765300980639 ) ) ;
#23129=CARTESIAN_POINT ( 'NONE',  ( -4.221309154770310101, 1446.219907474799811, 169.0688074703510040 ) ) ;
#23140=CARTESIAN_POINT ( 'NONE',  ( -19.61370360329999940, 1409.597986017130097, 199.4731069177680070 ) ) ;
#23144=ORIENTED_EDGE ( 'NONE', *, *, #55611, .T. ) ;
#23145=B_SPLINE_SURFACE_WITH_KNOTS ( 'NONE', 5, 5, ( 
 ( #60840, #18234, #86555, #84350, #41253, #75426 ),
 ( #34502, #101681, #7640, #42348, #17107, #85435 ),
 ( #76503, #110652, #59718, #93837, #8733, #42916 ),
 ( #65100, #27758, #30372, #87112, #63474, #1465 ),
 ( #47738, #98680, #13007, #89733, #20864, #52980 ),
 ( #35600, #46661, #69793, #22491, #4100, #97592 ) ),
 .UNSPECIFIED., .F., .F., .F.,
 ( 6, 6 ),
 ( 6, 6 ),
 ( 23.15748662889999920, 93.48651207330000545 ),
 ( -1.387778780779999841E-17, 1.000000000000000000 ),
 .UNSPECIFIED. ) ;
#23149=CARTESIAN_POINT ( 'NONE',  ( 11.05149221029999929, 1425.226139737630092, 137.4273676322979725 ) ) ;
#23151=B_SPLINE_CURVE_WITH_KNOTS ( 'NONE', 5,
 ( #37701, #106019, #63490, #18122, #5758, #90288, #89203, #21959, #46678, #6295, #13022, #81335, #38241, #73523, #56152, #40442, #64580, #97610, #21416, #89750, #55627, #4116, #12496, #91411, #31486, #80810, #72423, #47209, #106554, #65118, #39899, #4649, #29842 ),
 .UNSPECIFIED., .F., .F.,
 ( 6, 3, 3, 3, 3, 3, 3, 3, 3, 3, 6 ),
 ( 0.000000000000000000, 0.007518056952438774941, 0.01525203516534743772, 0.03845860237258517250, 0.06166516957982287606, 0.1235369933248144647, 0.2623877845595162794, 0.4012385757933799035, 0.5405419652431506794, 0.8197911058882223490, 1.000000000000000000 ),
 .UNSPECIFIED. ) ;
#23158=CARTESIAN_POINT ( 'NONE',  ( -12.63312964746819667, 1398.287568163796323, 212.1890067615559019 ) ) ;
#23163=CARTESIAN_POINT ( 'NONE',  ( 20.20924716366269891, 1509.280845329529939, 229.6605187684139935 ) ) ;
#23168=CARTESIAN_POINT ( 'NONE',  ( -2.512417091500000144, 1396.184323656129891, 221.0598646773979965 ) ) ;
#23169=CARTESIAN_POINT ( 'NONE',  ( -22.32010538089999940, 1411.050761390129992, 213.5142330314379819 ) ) ;
#23171=CARTESIAN_POINT ( 'NONE',  ( -13.43774386648357400, 1444.332129055663245, 169.3644175787693200 ) ) ;
#23172=CARTESIAN_POINT ( 'NONE',  ( -0.2612772979118159755, 1416.851343897360039, 227.4677505453099968 ) ) ;
#23175=CARTESIAN_POINT ( 'NONE',  ( -13.82025443706379875, 1508.597244210279996, 183.9953287070100032 ) ) ;
#23176=CARTESIAN_POINT ( 'NONE',  ( 4.597825173950000455, 1468.702107850830089, 183.5732306118979977 ) ) ;
#23180=CARTESIAN_POINT ( 'NONE',  ( 11.01747428149709940, 1396.297799067110191, 208.0502089956040095 ) ) ;
#23181=CARTESIAN_POINT ( 'NONE',  ( 1.270728274670000157, 1414.996444518330009, 191.7853923519979844 ) ) ;
#23182=CARTESIAN_POINT ( 'NONE',  ( 11.48551835569999824, 1426.311945552029783, 147.9218383413980007 ) ) ;
#23183=CARTESIAN_POINT ( 'NONE',  ( 8.140171433879366703, 1509.197613402637671, 180.9403984144503852 ) ) ;
#23185=CARTESIAN_POINT ( 'NONE',  ( 12.92162038170519978, 1434.739176993439969, 149.3060585083890146 ) ) ;
#23189=CARTESIAN_POINT ( 'NONE',  ( -18.13595047818949979, 1468.171444148069895, 228.4032209057770046 ) ) ;
#23190=CARTESIAN_POINT ( 'NONE',  ( -12.70631653080000056, 1462.828418259130103, 230.7343418143979932 ) ) ;
#23197=CARTESIAN_POINT ( 'NONE',  ( 2.500000000000000000, 1448.208035806090038, 170.3313966091639884 ) ) ;
#23199=ORIENTED_EDGE ( 'NONE', *, *, #96638, .T. ) ;
#23202=EDGE_LOOP ( 'NONE', ( #61462, #109854, #77358, #36985 ) ) ;
#23206=CARTESIAN_POINT ( 'NONE',  ( -38.91479787275512336, 1429.388299853867238, 269.5915017202312924 ) ) ;
#23207=CARTESIAN_POINT ( 'NONE',  ( -1.616567575689999980, 1409.474956838429989, 232.6959444083979918 ) ) ;
#23208=CARTESIAN_POINT ( 'NONE',  ( -1.239262138312009931, 1414.972329067380088, 226.4897656787760241 ) ) ;
#23210=CARTESIAN_POINT ( 'NONE',  ( 2.500000000000000000, 1419.382893006970107, 144.1042006977590120 ) ) ;
#23211=CARTESIAN_POINT ( 'NONE',  ( -34.13585384247240029, 1440.913060389490056, 249.1457226945469756 ) ) ;
#23213=CARTESIAN_POINT ( 'NONE',  ( -0.3157405184142340060, 1466.373614858310248, 235.6705076282450193 ) ) ;
#23214=CARTESIAN_POINT ( 'NONE',  ( 5.035691840050000145, 1407.858053359329915, 270.1320510971980298 ) ) ;
#23216=CARTESIAN_POINT ( 'NONE',  ( 23.66166531129999839, 1410.128854677129993, 208.6849955005649804 ) ) ;
#23217=CARTESIAN_POINT ( 'NONE',  ( -20.15293516530000062, 1508.383239031330049, 189.0805060732980110 ) ) ;
#23222=CARTESIAN_POINT ( 'NONE',  ( 0.2576834098190000089, 1419.224531700530179, 184.6439150135979901 ) ) ;
#23224=CARTESIAN_POINT ( 'NONE',  ( 0.6369828065621148117, 1408.970539270458858, 231.8715245986919058 ) ) ;
#23229=CARTESIAN_POINT ( 'NONE',  ( 39.02588949829999621, 1459.481874369829939, 266.4772423242980040 ) ) ;
#23232=CARTESIAN_POINT ( 'NONE',  ( -8.768113839085080130, 1509.161991642730072, 236.4477861136639945 ) ) ;
#23236=CARTESIAN_POINT ( 'NONE',  ( 0.3740406207303079711, 1452.976564550639978, 183.2744760995269928 ) ) ;
#23241=ORIENTED_EDGE ( 'NONE', *, *, #2245, .T. ) ;
#23245=CARTESIAN_POINT ( 'NONE',  ( 0.3765640108789999885, 1477.420202996130001, 229.8311010043980218 ) ) ;
#23246=CARTESIAN_POINT ( 'NONE',  ( 20.06336068849999776, 1456.114497556030074, 223.5835209092980165 ) ) ;
#23250=CARTESIAN_POINT ( 'NONE',  ( 15.20036750253001756, 1420.718811329341179, 227.8626738659623356 ) ) ;
#23251=CARTESIAN_POINT ( 'NONE',  ( 38.78625493179519879, 1448.012161950920017, 136.4925098791590017 ) ) ;
#23252=CARTESIAN_POINT ( 'NONE',  ( -20.33636649369999816, 1427.581624735430069, 223.9337651306980206 ) ) ;
#23253=CARTESIAN_POINT ( 'NONE',  ( -13.58058603182956148, 1473.584022274761764, 269.5920743625052864 ) ) ;
#23257=CARTESIAN_POINT ( 'NONE',  ( -25.36238703422979412, 1465.239872904934600, 269.4273574237397497 ) ) ;
#23259=CARTESIAN_POINT ( 'NONE',  ( -24.61293950550089704, 1444.770188684140066, 210.8869336946189890 ) ) ;
#23263=CARTESIAN_POINT ( 'NONE',  ( -12.86224528119999988, 1519.913060387329779, 228.0025448475979886 ) ) ;
#23266=CARTESIAN_POINT ( 'NONE',  ( -12.53380580351000084, 1442.773887400870080, 185.9733686700720057 ) ) ;
#23267=B_SPLINE_SURFACE_WITH_KNOTS ( 'NONE', 5, 5, ( 
 ( #39047, #4909, #3846, #55339, #12767, #89471, #72155, #21687, #106273 ),
 ( #90012, #108477, #64851, #22784, #98961, #29559, #37973, #13289, #72687 ),
 ( #47481, #55894, #21132, #56432, #46945, #90563, #82724, #81604, #38508 ),
 ( #65396, #81064, #39624, #48027, #73792, #99501, #56989, #91120, #14396 ),
 ( #6014, #31760, #65946, #50773, #16578, #24447, #49139, #109583, #6569 ),
 ( #58088, #85453, #7661, #83272, #110126, #110671, #41818, #8751, #92768 ) ),
 .UNSPECIFIED., .F., .F., .F.,
 ( 6, 6 ),
 ( 6, 3, 6 ),
 ( 39.88384216566930007, 42.45432491120000407 ),
 ( 0.000000000000000000, 8.028376878260001348, 16.05675375649999737 ),
 .UNSPECIFIED. ) ;
#23270=CARTESIAN_POINT ( 'NONE',  ( -3.091188561554334413, 1415.773449501390360, 232.7382472471307153 ) ) ;
#23272=CARTESIAN_POINT ( 'NONE',  ( 25.03845205760000070, 1436.443508297579911, 137.7838405999980012 ) ) ;
#23274=CARTESIAN_POINT ( 'NONE',  ( -13.98887540559999998, 1409.902971829729950, 226.7724385780979901 ) ) ;
#23277=CARTESIAN_POINT ( 'NONE',  ( 1.190628175363690033, 1414.913057834419988, 192.2393642087460250 ) ) ;
#23284=CARTESIAN_POINT ( 'NONE',  ( 7.760422419640001065E-08, 1460.308496262029848, 216.2848421383880009 ) ) ;
#23286=CARTESIAN_POINT ( 'NONE',  ( -11.89091680820000008, 1433.344382350330079, 150.2411281519979980 ) ) ;
#23288=DIRECTION ( 'NONE',  ( 0.0002664982727862750633, -9.558500756205390916E-06, 0.9999999644436521340 ) ) ;
#23289=CARTESIAN_POINT ( 'NONE',  ( -27.07124288249999822, 1440.503322045070036, 137.2138250103980113 ) ) ;
#23290=CARTESIAN_POINT ( 'NONE',  ( -24.34163166689999969, 1440.051000972679958, 211.6712235465880099 ) ) ;
#23292=CARTESIAN_POINT ( 'NONE',  ( 1.603799458759999963, 1450.610278152239971, 181.7139904433980178 ) ) ;
#23294=CARTESIAN_POINT ( 'NONE',  ( -9.587247150298686904, 1509.374143047329653, 237.5563645247161162 ) ) ;
#23295=CARTESIAN_POINT ( 'NONE',  ( -2.670047520287639767E-10, 1412.356500757170124, 252.5818293650800115 ) ) ;
#23296=ORIENTED_EDGE ( 'NONE', *, *, #15225, .T. ) ;
#23297=ORIENTED_EDGE ( 'NONE', *, *, #69962, .T. ) ;
#23298=CARTESIAN_POINT ( 'NONE',  ( -11.85007381715819896, 1431.224519208780066, 149.8691846786930171 ) ) ;
#23302=CARTESIAN_POINT ( 'NONE',  ( -3.511242807609999961, 1473.164181487230053, 270.4277067457979911 ) ) ;
#23306=CARTESIAN_POINT ( 'NONE',  ( 37.14918443920200275, 1450.989562377319999, 134.7272541307739857 ) ) ;
#23314=CARTESIAN_POINT ( 'NONE',  ( -29.06316727068120187, 1413.561815854209954, 267.1797966645490305 ) ) ;
#23315=VECTOR ( 'NONE', #51822, 1000.000000000000000 ) ;
#23319=EDGE_LOOP ( 'NONE', ( #65509, #47990, #37406, #19827, #7307, #104488, #66747 ) ) ;
#23321=CARTESIAN_POINT ( 'NONE',  ( 16.90742456144258909, 1444.994950788469623, 162.4348202098878744 ) ) ;
#23322=CARTESIAN_POINT ( 'NONE',  ( 41.54209482800269626, 1444.082802428220020, 136.2297247852750104 ) ) ;
#23325=CARTESIAN_POINT ( 'NONE',  ( -18.01785038329999722, 1455.457996638230043, 190.4178173900980084 ) ) ;
#23327=CARTESIAN_POINT ( 'NONE',  ( -11.60004869885203682, 1428.983126981193436, 136.0999999980979851 ) ) ;
#23329=CARTESIAN_POINT ( 'NONE',  ( -26.53940720459999980, 1435.424242704579910, 135.2833523932980029 ) ) ;
#23332=CARTESIAN_POINT ( 'NONE',  ( 1.582067810090000045E-15, 1406.443991414029824, 137.0999999980979851 ) ) ;
#23333=ADVANCED_FACE ( 'NONE', ( #107209 ), #32277, .F. ) ;
#23335=CARTESIAN_POINT ( 'NONE',  ( -40.98920041333110476, 1431.365838692129955, 269.8604638295950053 ) ) ;
#23337=CARTESIAN_POINT ( 'NONE',  ( -2.562000323739999974, 1397.677063979329887, 196.2741722088979941 ) ) ;
#23339=EDGE_LOOP ( 'NONE', ( #23144, #109972, #18879, #103793, #46908 ) ) ;
#23340=EDGE_LOOP ( 'NONE', ( #105664, #72273, #87727, #5944 ) ) ;
#23341=CARTESIAN_POINT ( 'NONE',  ( -11.86703214218580094, 1432.405005609789896, 149.9822914483479792 ) ) ;
#23342=EDGE_CURVE ( 'NONE', #45774, #31602, #53394, .T. ) ;
#23343=CARTESIAN_POINT ( 'NONE',  ( 32.12914650970602537, 1465.185426907999272, 269.3130570102625825 ) ) ;
#23345=CARTESIAN_POINT ( 'NONE',  ( -12.93021894928120119, 1435.974380371249936, 150.7740590697349887 ) ) ;
#23346=AXIS2_PLACEMENT_3D ( 'NONE', #12510, #79731, #54547 ) ;
#23350=CARTESIAN_POINT ( 'NONE',  ( -0.2055871234762860489, 1452.986193708736664, 183.2455700960801437 ) ) ;
#23351=CARTESIAN_POINT ( 'NONE',  ( -14.10900654350000138, 1426.825383623629932, 222.2175365666979872 ) ) ;
#23352=CARTESIAN_POINT ( 'NONE',  ( -13.20846944190000016, 1414.988015876829877, 220.4537675707979929 ) ) ;
#23353=CARTESIAN_POINT ( 'NONE',  ( 11.74267910810000082, 1446.506701529569909, 187.7371912896979893 ) ) ;
#23355=ORIENTED_EDGE ( 'NONE', *, *, #3499, .T. ) ;
#23356=DIRECTION ( 'NONE',  ( -0.4794255385927466140, -4.329869795923643736E-12, -0.8775825618966315300 ) ) ;
#23357=CARTESIAN_POINT ( 'NONE',  ( -11.58689981238089928, 1425.690685868059973, 133.5556927527120195 ) ) ;
#23358=CARTESIAN_POINT ( 'NONE',  ( -20.92280442586893230, 1454.947889300366114, 223.3949133203993540 ) ) ;
#23362=CARTESIAN_POINT ( 'NONE',  ( -25.17103052259800933, 1509.792535868356936, 224.3142502091264134 ) ) ;
#23363=CARTESIAN_POINT ( 'NONE',  ( -4.155669664704369382, 1439.704322410719897, 185.4969487652249995 ) ) ;
#23366=CARTESIAN_POINT ( 'NONE',  ( 3.169329433935653029, 1451.405488132423443, 183.9445329269590559 ) ) ;
#23369=CARTESIAN_POINT ( 'NONE',  ( 4.261545393745459265, 1441.227666458910107, 159.2966476699340035 ) ) ;
#23370=CARTESIAN_POINT ( 'NONE',  ( -11.94046459599999999, 1438.194204504490017, 147.6340003373980210 ) ) ;
#23371=CARTESIAN_POINT ( 'NONE',  ( 35.28305654171062855, 1451.608437209524254, 134.6904889284648732 ) ) ;
#23375=CARTESIAN_POINT ( 'NONE',  ( -5.035691841070000230, 1473.968067415529958, 270.1320510969979978 ) ) ;
#23377=CARTESIAN_POINT ( 'NONE',  ( -9.061761650477359709, 1423.804865071479753, 133.5339198589369971 ) ) ;
#23380=DIRECTION ( 'NONE',  ( 0.000000000000000000, 1.000000000000000000, 0.000000000000000000 ) ) ;
#23386=CARTESIAN_POINT ( 'NONE',  ( 31.24132895666020104, 1440.913060383959873, 242.0645883728159902 ) ) ;
#23388=CARTESIAN_POINT ( 'NONE',  ( -14.71230246820326393, 1414.913060387329779, 216.6130014222923137 ) ) ;
#23390=ORIENTED_EDGE ( 'NONE', *, *, #34627, .F. ) ;
#23391=ORIENTED_EDGE ( 'NONE', *, *, #73439, .T. ) ;
#23394=CARTESIAN_POINT ( 'NONE',  ( -19.85899607061380223, 1484.600033915471386, 190.9336331781040883 ) ) ;
#23396=CARTESIAN_POINT ( 'NONE',  ( -27.68254006319999760, 1507.989615291430027, 210.5775529109679951 ) ) ;
#23398=ADVANCED_FACE ( 'NONE', ( #28727 ), #37125, .T. ) ;
#23399=CARTESIAN_POINT ( 'NONE',  ( 1.440662988484916918, 1507.675818290031202, 236.8848933736155118 ) ) ;
#23405=CARTESIAN_POINT ( 'NONE',  ( 4.500000000000000000, 1411.429641636930000, 137.0999999980979851 ) ) ;
#23406=CARTESIAN_POINT ( 'NONE',  ( -11.87973986237470037, 1433.324300388509982, 147.6568050210650256 ) ) ;
#23409=VERTEX_POINT ( 'NONE', #55602 ) ;
#23425=AXIS2_PLACEMENT_3D ( 'NONE', #35244, #41450, #43105 ) ;
#23427=CARTESIAN_POINT ( 'NONE',  ( 9.593214614660599437, 1409.248062823570081, 197.6440812670239779 ) ) ;
#23428=CARTESIAN_POINT ( 'NONE',  ( 18.02088773781200004, 1424.325293679698234, 225.2049038667060188 ) ) ;
#23431=CARTESIAN_POINT ( 'NONE',  ( -3.660095725623159879, 1441.479904334799812, 165.0935399751739965 ) ) ;
#23432=DIRECTION ( 'NONE',  ( 0.4868800090730913133, -0.8445173987901640755, 0.2230206714761694409 ) ) ;
#23435=CARTESIAN_POINT ( 'NONE',  ( 18.88936493758499680, 1456.871008693799922, 227.2529171743470044 ) ) ;
#23437=CARTESIAN_POINT ( 'NONE',  ( -12.22933646150000087, 1434.134881474460144, 150.1178554876979945 ) ) ;
#23438=CARTESIAN_POINT ( 'NONE',  ( 3.230487471805439744E-10, 1465.426655107609804, 239.3266822731660000 ) ) ;
#23439=CARTESIAN_POINT ( 'NONE',  ( -20.45978729620729908, 1503.323240196070174, 190.5211554919499974 ) ) ;
#23440=CARTESIAN_POINT ( 'NONE',  ( -24.00431565076883444, 1435.335602849082761, 137.4619998928296809 ) ) ;
#23444=CARTESIAN_POINT ( 'NONE',  ( 4.314829847434388022, 1413.913060387330006, 217.0200890187050504 ) ) ;
#23445=CARTESIAN_POINT ( 'NONE',  ( -2.500000000000000000, 1439.615672362009946, 183.5288080637979817 ) ) ;
#23446=CARTESIAN_POINT ( 'NONE',  ( -19.67294290438620052, 1440.103789594400041, 208.5487540470539898 ) ) ;
#23447=EDGE_CURVE ( 'NONE', #44473, #64662, #29012, .T. ) ;
#23449=CARTESIAN_POINT ( 'NONE',  ( 2.751944573164369690, 1408.825585930090028, 223.0235821367669757 ) ) ;
#23451=CARTESIAN_POINT ( 'NONE',  ( 11.29523459009999975, 1425.738185348830029, 112.3426556953979940 ) ) ;
#23456=CARTESIAN_POINT ( 'NONE',  ( 20.00477949819999779, 1428.885732890330019, 217.2611606326379956 ) ) ;
#23457=DIRECTION ( 'NONE',  ( 0.000000000000000000, 0.7071067811865475727, 0.7071067811865475727 ) ) ;
#23458=CARTESIAN_POINT ( 'NONE',  ( 1.456422591599999983, 1499.391639968829850, 181.4501326743979917 ) ) ;
#23459=CARTESIAN_POINT ( 'NONE',  ( 24.91017775802731649, 1509.782942962777497, 224.3120645653099245 ) ) ;
#23461=CARTESIAN_POINT ( 'NONE',  ( -21.71651236630000170, 1429.876880566229829, 220.8156635984979914 ) ) ;
#23462=CARTESIAN_POINT ( 'NONE',  ( -28.55509083404212944, 1509.910676538754842, 202.0965624507188636 ) ) ;
#23463=CARTESIAN_POINT ( 'NONE',  ( -12.56757494846049994, 1452.474190999480015, 149.3742479200809896 ) ) ;
#23464=FACE_OUTER_BOUND ( 'NONE', #106259, .T. ) ;
#23466=CARTESIAN_POINT ( 'NONE',  ( -2.500000000000000000, 1421.191390850129892, 151.1105839291980146 ) ) ;
#23468=CARTESIAN_POINT ( 'NONE',  ( 15.55407252301110077, 1422.604129201769865, 228.8743534404409843 ) ) ;
#23471=EDGE_LOOP ( 'NONE', ( #80999, #90798, #100052, #97238, #82873 ) ) ;
#23472=EDGE_CURVE ( 'NONE', #76166, #68839, #94418, .T. ) ;
#23474=CARTESIAN_POINT ( 'NONE',  ( -23.04342231024600096, 1409.747493226589995, 209.0991873506499985 ) ) ;
#23475=CARTESIAN_POINT ( 'NONE',  ( -4.146783142809999489, 1426.018316099529784, 186.1121553539979914 ) ) ;
#23476=CARTESIAN_POINT ( 'NONE',  ( 0.3628711435760000326, 1419.323187844430095, 227.2866819789979900 ) ) ;
#23478=ADVANCED_FACE ( 'NONE', ( #91921 ), #65643, .F. ) ;
#23479=CARTESIAN_POINT ( 'NONE',  ( -4.438764019890000689, 1507.637717467430093, 236.4803969381979982 ) ) ;
#23480=CARTESIAN_POINT ( 'NONE',  ( -19.40852230999999861, 1415.853157747729938, 222.6427874863980207 ) ) ;
#23482=CARTESIAN_POINT ( 'NONE',  ( 45.90364696054209759, 1443.726197624660017, 268.5001126654299810 ) ) ;
#23484=CARTESIAN_POINT ( 'NONE',  ( -0.005520699207629999571, 1419.740206832129843, 184.3860476924980105 ) ) ;
#23487=VERTEX_POINT ( 'NONE', #15195 ) ;
#23493=CARTESIAN_POINT ( 'NONE',  ( 26.58146304371889812, 1451.968400311360028, 135.1860841996399927 ) ) ;
#23495=CARTESIAN_POINT ( 'NONE',  ( 0.1216143914258819986, 1452.908813519200066, 152.5222040808779980 ) ) ;
#23497=CARTESIAN_POINT ( 'NONE',  ( -4.121959999953849874, 1425.947382011577702, 186.1095471754434243 ) ) ;
#23500=CARTESIAN_POINT ( 'NONE',  ( 2.112814772436390154, 1408.986841504970016, 186.9590526398459929 ) ) ;
#23501=CARTESIAN_POINT ( 'NONE',  ( -16.97624119622160066, 1420.556660208560061, 191.4662531876780065 ) ) ;
#23502=CARTESIAN_POINT ( 'NONE',  ( -18.36927172832351474, 1424.107301416295286, 225.2316973828278890 ) ) ;
#23503=CARTESIAN_POINT ( 'NONE',  ( 2.959300169439202044, 1440.912996883657570, 170.5323342380343092 ) ) ;
#23504=AXIS2_PLACEMENT_3D ( 'NONE', #20944, #81398, #28824 ) ;
#23506=CARTESIAN_POINT ( 'NONE',  ( 2.265645423020000049, 1414.246892558129957, 164.3383647881979925 ) ) ;
#23508=CARTESIAN_POINT ( 'NONE',  ( 21.37693748330000076, 1438.522492596059919, 224.8635561966979708 ) ) ;
#23514=CARTESIAN_POINT ( 'NONE',  ( 1.455000209906389896, 1507.073729425429974, 236.7651043255590082 ) ) ;
#23516=CARTESIAN_POINT ( 'NONE',  ( -43.50000000000000000, 1440.913060387330006, 271.1218459616979999 ) ) ;
#23519=CARTESIAN_POINT ( 'NONE',  ( 37.18025153319999276, 1449.733372704670273, 265.6112249940979950 ) ) ;
#23530=CARTESIAN_POINT ( 'NONE',  ( -25.42735443440000154, 1450.801672132440217, 137.2052187181979832 ) ) ;
#23531=CARTESIAN_POINT ( 'NONE',  ( -16.84515702779830093, 1409.666169224270106, 192.5998696085950144 ) ) ;
#23532=CARTESIAN_POINT ( 'NONE',  ( 12.78690732370000127, 1416.828044896230040, 222.7042044813979942 ) ) ;
#23534=( BOUNDED_CURVE ( )  B_SPLINE_CURVE ( 3, ( #99524, #13864, #73248, #4927 ),
 .UNSPECIFIED., .F., .F. ) 
 B_SPLINE_CURVE_WITH_KNOTS ( ( 4, 4 ),
 ( 4.745561737044720729, 4.756500625272940042 ),
 .UNSPECIFIED. ) 
 CURVE ( )  GEOMETRIC_REPRESENTATION_ITEM ( )  RATIONAL_B_SPLINE_CURVE ( ( 1.000000000000000000, 0.9999900284185523347, 0.9999900284185523347, 1.000000000000000000 ) ) 
 REPRESENTATION_ITEM ( '' )  );
#23536=CARTESIAN_POINT ( 'NONE',  ( 1.581901184577762853, 1426.946688134061105, 134.0999999980979851 ) ) ;
#23537=CARTESIAN_POINT ( 'NONE',  ( 0.2065023403792599910, 1459.318095313439926, 182.9823369938129929 ) ) ;
#23538=CARTESIAN_POINT ( 'NONE',  ( -6.157363072879999955, 1409.067554757129756, 222.6581951653980127 ) ) ;
#23540=CARTESIAN_POINT ( 'NONE',  ( -18.43688931543649190, 1444.994950788470533, 161.6100378850031234 ) ) ;
#23541=EDGE_CURVE ( 'NONE', #15766, #94444, #42484, .T. ) ;
#23542=CARTESIAN_POINT ( 'NONE',  ( -28.59140520858730028, 1509.720434423589950, 211.2156787647219858 ) ) ;
#23543=CARTESIAN_POINT ( 'NONE',  ( 12.40430713589999989, 1434.419976112569884, 147.9455075187979674 ) ) ;
#23544=CARTESIAN_POINT ( 'NONE',  ( -41.65974987178940125, 1443.430997014530021, 134.0999999981650035 ) ) ;
#23553=CARTESIAN_POINT ( 'NONE',  ( 35.58608576442487248, 1419.490279919586328, 269.2370718515488761 ) ) ;
#23560=ORIENTED_EDGE ( 'NONE', *, *, #103486, .T. ) ;
#23561=CARTESIAN_POINT ( 'NONE',  ( -28.40191814786259883, 1508.834101309289963, 208.8103828110809843 ) ) ;
#23562=CARTESIAN_POINT ( 'NONE',  ( -16.54489977905999964, 1410.128898629499872, 226.3156677813840076 ) ) ;
#23567=CARTESIAN_POINT ( 'NONE',  ( -20.89012358491003596, 1411.002044536383437, 218.6339710684976581 ) ) ;
#23569=CARTESIAN_POINT ( 'NONE',  ( -0.3711878547863939892, 1418.751852236400055, 184.7050034054750256 ) ) ;
#23570=ADVANCED_FACE ( 'NONE', ( #76232 ), #43072, .T. ) ;
#23571=CARTESIAN_POINT ( 'NONE',  ( 21.89160165000000191, 1409.841974678430006, 214.9120575694479669 ) ) ;
#23572=CARTESIAN_POINT ( 'NONE',  ( -2.920701990467229781, 1417.235411609819948, 186.3067063531650263 ) ) ;
#23573=CARTESIAN_POINT ( 'NONE',  ( -16.67802482740000158, 1423.369746731130135, 229.1820141820979870 ) ) ;
#23580=EDGE_CURVE ( 'NONE', #6969, #75505, #93854, .T. ) ;
#23581=AXIS2_PLACEMENT_3D ( 'NONE', #93654, #61228, #85830 ) ;
#23583=CARTESIAN_POINT ( 'NONE',  ( -12.71625625589999942, 1484.464918063330060, 185.9897890590980012 ) ) ;
#23586=DIRECTION ( 'NONE',  ( -0.6081597637245996779, 0.7938146520356244018, 0.000000000000000000 ) ) ;
#23594=CARTESIAN_POINT ( 'NONE',  ( -23.04597175440000001, 1410.910372373229848, 204.9159820316880030 ) ) ;
#23595=CARTESIAN_POINT ( 'NONE',  ( -11.15965917747685410, 1425.157781931322461, 144.4782180148434634 ) ) ;
#23596=CARTESIAN_POINT ( 'NONE',  ( 15.85178800091950002, 1409.849131890500075, 191.9518116726889900 ) ) ;
#23598=CARTESIAN_POINT ( 'NONE',  ( 41.51359561934580711, 1442.004548209790073, 135.9438258381890137 ) ) ;
#23601=CARTESIAN_POINT ( 'NONE',  ( -3.666694481987490040, 1509.114858341099989, 179.5219341129400163 ) ) ;
#23602=CARTESIAN_POINT ( 'NONE',  ( 9.783750736287140981, 1464.829832912111442, 232.4492286805421202 ) ) ;
#23614=CARTESIAN_POINT ( 'NONE',  ( -0.008321110301990000332, 1451.173510518130115, 182.5308026085980089 ) ) ;
#23616=CARTESIAN_POINT ( 'NONE',  ( -2.500000000000000000, 1439.611175468640113, 167.3041000418980104 ) ) ;
#23617=ADVANCED_FACE ( 'NONE', ( #28580 ), #42149, .T. ) ;
#23620=CARTESIAN_POINT ( 'NONE',  ( -28.07231162100000077, 1508.101920006030241, 207.7749232119980149 ) ) ;
#23621=CARTESIAN_POINT ( 'NONE',  ( 36.37832866288330536, 1451.642701157629745, 135.6938360142119961 ) ) ;
#23623=CARTESIAN_POINT ( 'NONE',  ( 27.50386082860000059, 1440.425502049640045, 137.1894327424980133 ) ) ;
#23632=CARTESIAN_POINT ( 'NONE',  ( 41.78528023106409961, 1440.913060387330006, 269.3547801055810282 ) ) ;
#23633=CARTESIAN_POINT ( 'NONE',  ( -0.0007848984903239803303, 1451.920411048226470, 154.0000879905409192 ) ) ;
#23635=CARTESIAN_POINT ( 'NONE',  ( -14.04614445250000188, 1415.579607678630055, 221.1977299884980255 ) ) ;
#23636=CARTESIAN_POINT ( 'NONE',  ( -11.65870824634879988, 1432.338283297729959, 150.9211958027459843 ) ) ;
#23639=CARTESIAN_POINT ( 'NONE',  ( -12.88992692469999923, 1429.132124773229862, 222.5285527285979867 ) ) ;
#23642=CARTESIAN_POINT ( 'NONE',  ( -11.94143867729999897, 1433.615104777220040, 147.8551380903979862 ) ) ;
#23643=CARTESIAN_POINT ( 'NONE',  ( 26.02020593944349969, 1489.081220952810099, 206.2263664854170031 ) ) ;
#23644=CARTESIAN_POINT ( 'NONE',  ( 17.51720238729999934, 1459.587282136729982, 228.3696857288979913 ) ) ;
#23645=DIRECTION ( 'NONE',  ( 0.000000000000000000, 1.000000000000000000, 0.000000000000000000 ) ) ;
#23649=CARTESIAN_POINT ( 'NONE',  ( -22.71351678742513158, 1409.706230938278395, 208.9920840151032735 ) ) ;
#23650=CARTESIAN_POINT ( 'NONE',  ( -0.03160925563740960703, 1508.847401064120049, 179.7329215851769959 ) ) ;
#23653=CARTESIAN_POINT ( 'NONE',  ( 18.46505082730000069, 1509.557874170530113, 187.1463136621979970 ) ) ;
#23654=CARTESIAN_POINT ( 'NONE',  ( -11.60004869885203505, 1425.163648245827062, 137.9639116245677997 ) ) ;
#23659=CARTESIAN_POINT ( 'NONE',  ( -11.85198087010000023, 1431.354781565790063, 149.8962517293980170 ) ) ;
#23662=CARTESIAN_POINT ( 'NONE',  ( 27.02941372530000308, 1451.801869924330049, 135.6489090826979975 ) ) ;
#23665=CARTESIAN_POINT ( 'NONE',  ( -25.76221643539999917, 1495.363080995530026, 215.5756636875879906 ) ) ;
#23666=CARTESIAN_POINT ( 'NONE',  ( -2.456317400796513173, 1421.792675212155928, 137.0999999980980704 ) ) ;
#23670=CARTESIAN_POINT ( 'NONE',  ( 6.176534431810000392, 1406.368378108629940, 269.0307194043979848 ) ) ;
#23671=CARTESIAN_POINT ( 'NONE',  ( -2.500000000000000000, 1439.114301494319989, 157.7261950941980331 ) ) ;
#23673=CARTESIAN_POINT ( 'NONE',  ( 24.16053673582425176, 1436.344787939296566, 213.4465298597629328 ) ) ;
#23676=DIRECTION ( 'NONE',  ( 0.000000000000000000, 0.000000000000000000, -1.000000000000000000 ) ) ;
#23678=CARTESIAN_POINT ( 'NONE',  ( -1.564574781134263626, 1451.289357135363161, 183.8180204487754565 ) ) ;
#23679=CARTESIAN_POINT ( 'NONE',  ( 1.466050869238679999, 1450.686205474260078, 155.3356453482439861 ) ) ;
#23682=CARTESIAN_POINT ( 'NONE',  ( -19.00000000000000000, 1438.871025162500018, 209.1218459616979999 ) ) ;
#23683=CARTESIAN_POINT ( 'NONE',  ( -11.60004869885203682, -0.000000000000000000, 135.5999999980979851 ) ) ;
#23684=CARTESIAN_POINT ( 'NONE',  ( 4.283856808220000367, 1440.956245581859775, 155.9230798038979913 ) ) ;
#23685=CARTESIAN_POINT ( 'NONE',  ( -7.055157488669999921, 1475.427864936029891, 266.9413125670979525 ) ) ;
#23686=CARTESIAN_POINT ( 'NONE',  ( -4.220676207128734703, 1446.230049502166139, 170.5366217123670083 ) ) ;
#23691=AXIS2_PLACEMENT_3D ( 'NONE', #105209, #28497, #29053 ) ;
#23692=CARTESIAN_POINT ( 'NONE',  ( 16.42420380379999756, 1507.212883763329955, 193.5443561786979956 ) ) ;
#23693=CARTESIAN_POINT ( 'NONE',  ( -24.61334319966909945, 1444.769530411740107, 210.8865013930089845 ) ) ;
#23696=CARTESIAN_POINT ( 'NONE',  ( -20.44853841340000145, 1410.549219022030002, 198.9863064543980329 ) ) ;
#23702=CARTESIAN_POINT ( 'NONE',  ( -6.934382790878020231, 1410.528793468874483, 231.1058639361037592 ) ) ;
#23703=CARTESIAN_POINT ( 'NONE',  ( 13.27254556628637872, 1414.941240495251577, 198.0499574059903694 ) ) ;
#23705=CARTESIAN_POINT ( 'NONE',  ( 11.13334565089999906, 1425.173446693529968, 142.7648904542980119 ) ) ;
#23712=CARTESIAN_POINT ( 'NONE',  ( -10.21388636078169299, 1398.215752035679088, 201.0479164178328801 ) ) ;
#23715=DIRECTION ( 'NONE',  ( -0.7071067811870476172, 0.000000000000000000, 0.7071067811860475283 ) ) ;
#23720=CARTESIAN_POINT ( 'NONE',  ( 11.29216247361090097, 1434.438968647419870, 151.5554298123269916 ) ) ;
#23722=CARTESIAN_POINT ( 'NONE',  ( -11.88194722309999918, 1396.505120844730072, 211.3071127478679898 ) ) ;
#23723=CARTESIAN_POINT ( 'NONE',  ( -20.06921834150000095, 1410.974364727830107, 220.7356942897980048 ) ) ;
#23724=VERTEX_POINT ( 'NONE', #69936 ) ;
#23725=CARTESIAN_POINT ( 'NONE',  ( -13.15334649152275404, 1444.754287284761403, 169.3979280245720247 ) ) ;
#23726=CARTESIAN_POINT ( 'NONE',  ( 22.03874496197475708, 1509.704128133699214, 228.9173456134791991 ) ) ;
#23729=CARTESIAN_POINT ( 'NONE',  ( -13.80442745998849929, 1508.531539859030090, 184.0281800264250194 ) ) ;
#23730=CARTESIAN_POINT ( 'NONE',  ( -0.02449593311879999860, 1468.711357958130066, 182.4995022349980047 ) ) ;
#23733=CARTESIAN_POINT ( 'NONE',  ( 9.951016712660660346, 1396.260557557309994, 204.2881766974590221 ) ) ;
#23734=CARTESIAN_POINT ( 'NONE',  ( 1.249587849179999877, 1415.128105756529976, 191.3153250033980157 ) ) ;
#23735=CARTESIAN_POINT ( 'NONE',  ( 10.96803698370000113, 1432.243966832229944, 151.7696189413979937 ) ) ;
#23736=CARTESIAN_POINT ( 'NONE',  ( 8.229600951721646851, 1509.200675254854787, 180.9700133782839941 ) ) ;
#23738=CARTESIAN_POINT ( 'NONE',  ( 13.27369308195070019, 1434.899823491839925, 149.1828079990220033 ) ) ;
#23739=VERTEX_POINT ( 'NONE', #61527 ) ;
#23741=CARTESIAN_POINT ( 'NONE',  ( 12.85075015980074298, 1444.958812780512289, 169.4430788496519824 ) ) ;
#23742=CARTESIAN_POINT ( 'NONE',  ( -7.139643389570000664, 1463.933016855429969, 236.1633026984980006 ) ) ;
#23751=EDGE_CURVE ( 'NONE', #59795, #18384, #18265, .T. ) ;
#23754=ORIENTED_EDGE ( 'NONE', *, *, #2233, .F. ) ;
#23756=CARTESIAN_POINT ( 'NONE',  ( -20.15452302159999931, 1507.845791376729949, 228.9024215066979764 ) ) ;
#23757=CARTESIAN_POINT ( 'NONE',  ( -35.91967445428193884, 1425.095412615255555, 269.5444895620009902 ) ) ;
#23759=CARTESIAN_POINT ( 'NONE',  ( -1.032249311085239984, 1415.090956648730071, 226.6967784922329940 ) ) ;
#23760=ORIENTED_EDGE ( 'NONE', *, *, #13807, .T. ) ;
#23761=CARTESIAN_POINT ( 'NONE',  ( 2.500000000000000000, 1432.302110539269961, 157.4936333739979943 ) ) ;
#23762=CARTESIAN_POINT ( 'NONE',  ( -28.69268220585919948, 1440.913060387330006, 233.8417140319710086 ) ) ;
#23764=CARTESIAN_POINT ( 'NONE',  ( -0.07116624666730259063, 1465.436517331040250, 236.3246395822949921 ) ) ;
#23765=CARTESIAN_POINT ( 'NONE',  ( 8.194407606919998699, 1409.116459709330002, 270.4215667397979814 ) ) ;
#23767=CARTESIAN_POINT ( 'NONE',  ( 23.95176194079999732, 1410.398731527629934, 209.1804549718790156 ) ) ;
#23768=DIRECTION ( 'NONE',  ( -1.989939052760000051E-13, -6.949020296389990473E-15, 1.000000000000000000 ) ) ;
#23772=CARTESIAN_POINT ( 'NONE',  ( -3.189772444258944351, 1447.442977096462073, 154.8380773011854501 ) ) ;
#23774=CARTESIAN_POINT ( 'NONE',  ( -6.420950019901092709, 1485.997607280482725, 182.7091661881264884 ) ) ;
#23778=CARTESIAN_POINT ( 'NONE',  ( 18.95862648649999826, 1416.832348283729971, 210.4638202831779950 ) ) ;
#23780=CARTESIAN_POINT ( 'NONE',  ( -11.22085813611739979, 1414.913060387329779, 220.6193216859199993 ) ) ;
#23783=CARTESIAN_POINT ( 'NONE',  ( -7.121584071090000023, 1409.161751583130126, 195.9581075130980139 ) ) ;
#23786=CARTESIAN_POINT ( 'NONE',  ( -25.93754856796245889, 1450.779557423562437, 136.7820379074420600 ) ) ;
#23792=CARTESIAN_POINT ( 'NONE',  ( 19.88559295760000012, 1455.744107332229987, 223.8027299929979961 ) ) ;
#23795=CARTESIAN_POINT ( 'NONE',  ( 26.61844847777970813, 1450.722186606933292, 136.4846925697592042 ) ) ;
#23796=CARTESIAN_POINT ( 'NONE',  ( 15.25750226104648810, 1420.759466697897551, 227.8319051552381609 ) ) ;
#23797=CARTESIAN_POINT ( 'NONE',  ( 29.70844085274949720, 1436.010927005220083, 136.4302040973799990 ) ) ;
#23798=CARTESIAN_POINT ( 'NONE',  ( 39.62454033826469413, 1446.691649570389927, 136.6910118460810111 ) ) ;
#23799=CARTESIAN_POINT ( 'NONE',  ( 20.25058512361396623, 1506.578946199967277, 217.9834787517386587 ) ) ;
#23800=CARTESIAN_POINT ( 'NONE',  ( -2.616722072391682197, 1475.048391684631042, 269.6500679664175095 ) ) ;
#23802=CARTESIAN_POINT ( 'NONE',  ( -17.52239435150000446, 1415.804866261129973, 225.9435871245979968 ) ) ;
#23804=CARTESIAN_POINT ( 'NONE',  ( -16.16453978850797313, 1469.071349536585103, 269.3697744449012816 ) ) ;
#23806=CARTESIAN_POINT ( 'NONE',  ( -4.074350933259999502E-15, 1428.579607037230062, 149.5143047311979672 ) ) ;
#23807=CARTESIAN_POINT ( 'NONE',  ( -27.36442814965441173, 1413.476243666040546, 269.4075121043655372 ) ) ;
#23810=B_SPLINE_CURVE_WITH_KNOTS ( 'NONE', 5,
 ( #23172, #92045, #108293, #33233, #7486, #82552 ),
 .UNSPECIFIED., .F., .F.,
 ( 6, 6 ),
 ( 0.000000000000000000, 1.000000000000000000 ),
 .UNSPECIFIED. ) ;
#23811=CARTESIAN_POINT ( 'NONE',  ( -14.69331829855070026, 1452.091493848030041, 222.9975758587799817 ) ) ;
#23812=CARTESIAN_POINT ( 'NONE',  ( -13.09515188823569076, 1443.020675217816461, 186.6586876594417106 ) ) ;
#23815=CARTESIAN_POINT ( 'NONE',  ( -4.958998528701818564, 1416.169772216195270, 232.1515073687287156 ) ) ;
#23816=CARTESIAN_POINT ( 'NONE',  ( -38.12974907660549917, 1444.894042496500106, 137.0546131931990033 ) ) ;
#23818=CARTESIAN_POINT ( 'NONE',  ( -13.20386921870955632, 1443.121265474914935, 169.3907368431102896 ) ) ;
#23819=CARTESIAN_POINT ( 'NONE',  ( -14.81131296149999876, 1410.375311526330051, 226.7082462524979860 ) ) ;
#23820=ORIENTED_EDGE ( 'NONE', *, *, #24815, .F. ) ;
#23822=CARTESIAN_POINT ( 'NONE',  ( 0.8265315298475599537, 1415.089948427370018, 191.7561489437229909 ) ) ;
#23823=CARTESIAN_POINT ( 'NONE',  ( -2.573074615509999941, 1409.002914132830028, 231.1540680731980046 ) ) ;
#23824=ORIENTED_EDGE ( 'NONE', *, *, #16557, .T. ) ;
#23825=EDGE_LOOP ( 'NONE', ( #14399, #88659, #79143, #52944, #68196, #33111 ) ) ;
#23826=CARTESIAN_POINT ( 'NONE',  ( 16.66147553287439820, 1414.913057846380070, 209.9988873639480005 ) ) ;
#23829=CARTESIAN_POINT ( 'NONE',  ( -8.166151876880000771, 1461.469839515129934, 225.2410124208979880 ) ) ;
#23831=CARTESIAN_POINT ( 'NONE',  ( -11.88593578010000051, 1433.200405512929819, 150.0669781585979763 ) ) ;
#23835=CARTESIAN_POINT ( 'NONE',  ( -24.35601318819999861, 1440.342902236149939, 211.6694219976479872 ) ) ;
#23837=CARTESIAN_POINT ( 'NONE',  ( 2.086716510760000087, 1452.155719858229986, 183.6328824817980205 ) ) ;
#23839=CARTESIAN_POINT ( 'NONE',  ( -27.55294438350654929, 1509.987280990239697, 197.2544469677627887 ) ) ;
#23840=CARTESIAN_POINT ( 'NONE',  ( -2.017359258820280141E-09, 1416.045455530739900, 240.6646644973519926 ) ) ;
#23841=ORIENTED_EDGE ( 'NONE', *, *, #13815, .F. ) ;
#23844=CARTESIAN_POINT ( 'NONE',  ( -11.79426874074069964, 1427.973425763779915, 147.8794941013190112 ) ) ;
#23846=CARTESIAN_POINT ( 'NONE',  ( -6.215218566849999959, 1471.256776971429872, 269.6190395958980162 ) ) ;
#23849=CARTESIAN_POINT ( 'NONE',  ( 40.76353202841180234, 1447.329558407210016, 136.0508387103639905 ) ) ;
#23850=CARTESIAN_POINT ( 'NONE',  ( 17.70665509759999878, 1431.113060387329824, 202.1814663873780091 ) ) ;
#23851=CARTESIAN_POINT ( 'NONE',  ( 19.76122774234984192, 1455.648809305226223, 227.1212724839211603 ) ) ;
#23856=CARTESIAN_POINT ( 'NONE',  ( -39.51454461767819737, 1423.024700941120045, 268.9460601137379854 ) ) ;
#23862=CARTESIAN_POINT ( 'NONE',  ( 4.844982144979842253, 1423.488028581556364, 184.1325588144100891 ) ) ;
#23865=CARTESIAN_POINT ( 'NONE',  ( -38.61927355701700293, 1444.188087899089851, 137.1592452686400065 ) ) ;
#23866=CARTESIAN_POINT ( 'NONE',  ( -17.85129570129999621, 1455.457398219630250, 190.3057806367980049 ) ) ;
#23867=CARTESIAN_POINT ( 'NONE',  ( -16.75617669327549919, 1479.756059428050094, 228.8978987931039910 ) ) ;
#23872=CARTESIAN_POINT ( 'NONE',  ( -33.91369114349999592, 1451.728768196330066, 134.7155300131979914 ) ) ;
#23876=CARTESIAN_POINT ( 'NONE',  ( -6.016808998109999251, 1396.654460029229995, 198.2004533603980008 ) ) ;
#23881=VECTOR ( 'NONE', #21492, 1000.000000000000114 ) ;
#23882=CARTESIAN_POINT ( 'NONE',  ( 3.749167825016557654, 1425.488083945166409, 185.1890168411832462 ) ) ;
#23884=CARTESIAN_POINT ( 'NONE',  ( -24.31979101810000188, 1435.530147504380011, 137.6066080458979854 ) ) ;
#23885=CARTESIAN_POINT ( 'NONE',  ( -24.67369719190000055, 1441.458996830729802, 210.7025079082280001 ) ) ;
#23889=CARTESIAN_POINT ( 'NONE',  ( -1.908211845303299903, 1484.244220179899912, 182.9087969337900006 ) ) ;
#23893=EDGE_LOOP ( 'NONE', ( #44659, #36589, #78964, #42056, #57531, #73336, #33131, #63520, #71829, #104338, #56314 ) ) ;
#23894=CARTESIAN_POINT ( 'NONE',  ( -2.386210315674730076, 1451.954674705370053, 184.6135196128299754 ) ) ;
#23896=CARTESIAN_POINT ( 'NONE',  ( -20.28084755118021576, 1456.032803552603809, 224.6711213126964708 ) ) ;
#23897=ORIENTED_EDGE ( 'NONE', *, *, #91306, .F. ) ;
#23899=CARTESIAN_POINT ( 'NONE',  ( -25.78156655170059608, 1509.813372604039841, 223.1298223243570078 ) ) ;
#23900=B_SPLINE_SURFACE_WITH_KNOTS ( 'NONE', 5, 1, ( 
 ( #93592, #77375 ),
 ( #67885, #8489 ),
 ( #86865, #10157 ),
 ( #68438, #101995 ),
 ( #43768, #7947 ),
 ( #76264, #52730 ),
 ( #51621, #110412 ),
 ( #25280, #35925 ),
 ( #59481, #60034 ),
 ( #9598, #16868 ),
 ( #84649, #95273 ),
 ( #33691, #26399 ),
 ( #1787, #44332 ),
 ( #42116, #43226 ),
 ( #17423, #76817 ) ),
 .UNSPECIFIED., .F., .F., .F.,
 ( 6, 3, 3, 3, 6 ),
 ( 2, 2 ),
 ( 91.71614156710000998, 91.73016858649999961, 144.2269611950000012, 165.2349012489999893, 166.7810826825559900 ),
 ( -7.070755615892880552E-05, 4.740550787240640496 ),
 .UNSPECIFIED. ) ;
#23901=CARTESIAN_POINT ( 'NONE',  ( -4.070270494153594321, 1440.756896449854594, 185.1152696589734319 ) ) ;
#23903=CARTESIAN_POINT ( 'NONE',  ( -11.39059366553855490, 1425.662989886324112, 138.8619651797782808 ) ) ;
#23906=CARTESIAN_POINT ( 'NONE',  ( 24.25228055134414262, 1445.991220302454849, 214.4993191193233883 ) ) ;
#23907=CARTESIAN_POINT ( 'NONE',  ( -11.96519809220000141, 1440.444625599219989, 147.6189886498980002 ) ) ;
#23908=CARTESIAN_POINT ( 'NONE',  ( 16.17523441753503022, 1409.477912220330381, 225.6432943692607296 ) ) ;
#23914=CARTESIAN_POINT ( 'NONE',  ( 0.5093327223650000457, 1419.917355073230055, 184.4471483751979974 ) ) ;
#23915=EDGE_CURVE ( 'NONE', #48999, #9907, #104917, .T. ) ;
#23921=CARTESIAN_POINT ( 'NONE',  ( 17.71719970781420628, 1423.378758011100444, 226.1827588889887863 ) ) ;
#23925=CARTESIAN_POINT ( 'NONE',  ( 42.45354694711880228, 1440.913060353240098, 262.5200983195459798 ) ) ;
#23927=DIRECTION ( 'NONE',  ( 0.000000000000000000, 1.000000000000000000, 0.000000000000000000 ) ) ;
#23930=ORIENTED_EDGE ( 'NONE', *, *, #56503, .F. ) ;
#23931=ORIENTED_EDGE ( 'NONE', *, *, #5811, .T. ) ;
#23934=CARTESIAN_POINT ( 'NONE',  ( -1.188177861046854300, 1416.835288266028101, 228.1251897816796941 ) ) ;
#23936=LINE ( 'NONE', #41864, #100242 ) ;
#23941=CARTESIAN_POINT ( 'NONE',  ( 2.499945006294769900, 1419.401634877229981, 143.2540554854240042 ) ) ;
#23942=CARTESIAN_POINT ( 'NONE',  ( -27.43651671978516404, 1509.328400563031892, 212.0833630515228378 ) ) ;
#23945=EDGE_LOOP ( 'NONE', ( #11816, #67177, #75040, #110809 ) ) ;
#23948=CARTESIAN_POINT ( 'NONE',  ( 19.82859500370260264, 1508.459386330439884, 229.4052108613220184 ) ) ;
#23950=ORIENTED_EDGE ( 'NONE', *, *, #71279, .T. ) ;
#23956=AXIS2_PLACEMENT_3D ( 'NONE', #47063, #29688, #48720 ) ;
#23959=CYLINDRICAL_SURFACE ( 'NONE', #19552, 2.000000000000001776 ) ;
#23963=CARTESIAN_POINT ( 'NONE',  ( 0.7287763451100000012, 1409.106502167329836, 185.6933822617980070 ) ) ;
#23966=CARTESIAN_POINT ( 'NONE',  ( 11.57646189039999918, 1432.336252720020184, 151.1966908187980039 ) ) ;
#23967=CIRCLE ( 'NONE', #86571, 1.999999999999961808 ) ;
#23968=CARTESIAN_POINT ( 'NONE',  ( -2.513809405447149814, 1451.504177376969892, 184.6655415589659981 ) ) ;
#23971=CARTESIAN_POINT ( 'NONE',  ( 18.71713341259120256, 1457.163765172349940, 229.5372674111999913 ) ) ;
#23972=CARTESIAN_POINT ( 'NONE',  ( -12.98106087750000093, 1435.572631767780194, 150.6458279223980128 ) ) ;
#23973=CARTESIAN_POINT ( 'NONE',  ( -1.150230247847569986E-08, 1474.257262691309961, 263.8864222916459994 ) ) ;
#23978=CARTESIAN_POINT ( 'NONE',  ( -0.1885928293499999908, 1482.195919647529990, 181.9611671400979844 ) ) ;
#23985=CARTESIAN_POINT ( 'NONE',  ( 1.478250974131940509, 1424.351089761499907, 227.4175086134767128 ) ) ;
#23987=ORIENTED_EDGE ( 'NONE', *, *, #12475, .F. ) ;
#23988=CARTESIAN_POINT ( 'NONE',  ( 24.93072418010000035, 1437.606125426900235, 217.2956629241979840 ) ) ;
#23989=CARTESIAN_POINT ( 'NONE',  ( 1.467228651769999948, 1489.039472797129974, 181.9015832661979744 ) ) ;
#23990=CARTESIAN_POINT ( 'NONE',  ( -16.19492410690000384, 1409.478599599030076, 194.0661808922979787 ) ) ;
#23992=SPHERICAL_SURFACE ( 'NONE', #8549, 2.000000000000000000 ) ;
#23993=CARTESIAN_POINT ( 'NONE',  ( -28.36433000254718806, 1509.903564542218646, 201.4659584704413930 ) ) ;
#23994=CARTESIAN_POINT ( 'NONE',  ( -9.826464246318440843, 1452.569912694470077, 150.6692168550179929 ) ) ;
#23996=EDGE_LOOP ( 'NONE', ( #64985, #64138, #5480, #7366 ) ) ;
#23998=CARTESIAN_POINT ( 'NONE',  ( -0.6192548831692870070, 1407.650904249920131, 270.1377146676910002 ) ) ;
#23999=CARTESIAN_POINT ( 'NONE',  ( 15.95518007350070100, 1422.893326400530214, 228.6357347565129885 ) ) ;
#24001=ORIENTED_EDGE ( 'NONE', *, *, #93987, .F. ) ;
#24002=ORIENTED_EDGE ( 'NONE', *, *, #77360, .T. ) ;
#24004=CARTESIAN_POINT ( 'NONE',  ( -23.74908638290310137, 1410.154450923110062, 208.9152455597699998 ) ) ;
#24006=CARTESIAN_POINT ( 'NONE',  ( -4.273589427560000154, 1425.970440093729849, 186.1370899423980063 ) ) ;
#24007=CARTESIAN_POINT ( 'NONE',  ( -12.49103604210455387, 1436.447564085543263, 151.1284240868977520 ) ) ;
#24008=CARTESIAN_POINT ( 'NONE',  ( -6.861707994109999653, 1428.078401598830169, 112.4493539157979995 ) ) ;
#24010=CARTESIAN_POINT ( 'NONE',  ( -2.474406870190000163, 1507.640282505830100, 236.9531809319980198 ) ) ;
#24011=CARTESIAN_POINT ( 'NONE',  ( -19.90339844620000065, 1415.851102572129776, 221.6293417451979906 ) ) ;
#24013=CARTESIAN_POINT ( 'NONE',  ( 44.63527855443649628, 1449.973421542959841, 268.2561587561260126 ) ) ;
#24015=CARTESIAN_POINT ( 'NONE',  ( -0.05142771962049999535, 1419.751625371630098, 184.3796591070980071 ) ) ;
#24018=CARTESIAN_POINT ( 'NONE',  ( 18.37125585514824166, 1459.035043778956151, 227.7538859344645061 ) ) ;
#24020=DIRECTION ( 'NONE',  ( -0.8023110876747339137, -0.5969061220947440294, 0.000000000000000000 ) ) ;
#24021=VERTEX_POINT ( 'NONE', #56704 ) ;
#24028=B_SPLINE_SURFACE_WITH_KNOTS ( 'NONE', 5, 5, ( 
 ( #25011, #85469, #8216, #95002, #50262, #110140, #51904, #44053, #33413 ),
 ( #51334, #67061, #68175, #59756, #33980, #17700, #24461, #84391, #59212 ),
 ( #7678, #41834, #75990, #86044, #93331, #18270, #16594, #93877, #110689 ),
 ( #50791, #84923, #43504, #25563, #42381, #8768, #77648, #42949, #77108 ),
 ( #416, #34534, #26677, #68716, #962, #69267, #26115, #103373, #60876 ),
 ( #95548, #78754, #37857, #45729, #35635, #106160, #19372, #72043, #11552 ),
 ( #29437, #63636, #20470, #69829, #96664, #62543, #18821, #36749, #97750 ),
 ( #12650, #19935, #105621, #45172, #46828, #44612, #2069, #2623, #79313 ),
 ( #1504, #79865, #55225, #103946, #10440, #54131, #21021, #89355, #11000 ) ),
 .UNSPECIFIED., .F., .F., .F.,
 ( 6, 3, 6 ),
 ( 6, 3, 6 ),
 ( 1.119759084200000032, 3.314659481400000107, 6.273351219260000278 ),
 ( 0.000000000000000000, 1.000000000000000000, 2.000000000000000000 ),
 .UNSPECIFIED. ) ;
#24031=CARTESIAN_POINT ( 'NONE',  ( 4.577122560907209703, 1409.072897029190017, 187.7508653761969981 ) ) ;
#24032=CARTESIAN_POINT ( 'NONE',  ( -13.78070311828070160, 1434.978583006209874, 148.5586138787649872 ) ) ;
#24033=FACE_OUTER_BOUND ( 'NONE', #83322, .T. ) ;
#24036=ADVANCED_FACE ( 'NONE', ( #81885 ), #24071, .T. ) ;
#24038=CARTESIAN_POINT ( 'NONE',  ( 11.59417695439999996, 1428.981093279630159, 133.6118001900980232 ) ) ;
#24040=CARTESIAN_POINT ( 'NONE',  ( 12.21873817507339943, 1415.431750870119913, 222.0592676625429931 ) ) ;
#24041=CIRCLE ( 'NONE', #102694, 2.000007000530037882 ) ;
#24045=EDGE_CURVE ( 'NONE', #68144, #26609, #95581, .T. ) ;
#24051=CARTESIAN_POINT ( 'NONE',  ( -34.97756117329999626, 1449.243413927999882, 262.6648722463980334 ) ) ;
#24052=CARTESIAN_POINT ( 'NONE',  ( -21.38849015939615583, 1509.000358152776244, 191.8600543660001279 ) ) ;
#24053=CARTESIAN_POINT ( 'NONE',  ( -12.78752272590105932, 1416.843574538714392, 195.5392800691490152 ) ) ;
#24054=CARTESIAN_POINT ( 'NONE',  ( 34.84383450159999285, 1453.969943368129861, 265.6112250856980381 ) ) ;
#24055=B_SPLINE_SURFACE_WITH_KNOTS ( 'NONE', 5, 5, ( 
 ( #65863, #17472, #14872, #49064, #49610, #6487 ),
 ( #7039, #41197, #51673, #725, #34855, #69044 ),
 ( #26447, #73719, #107842, #79644, #70164, #103718 ),
 ( #105943, #19135, #10774, #77965, #54453, #60641 ),
 ( #61209, #86916, #104276, #2401, #86363, #1273 ),
 ( #27563, #70712, #104826, #87487, #35412, #1839 ),
 ( #53339, #61747, #9644, #96430, #43819, #62303 ),
 ( #95869, #44946, #69600, #79093, #78528, #71823 ),
 ( #27020, #52780, #36519, #28112, #11872, #95323 ) ),
 .UNSPECIFIED., .F., .F., .F.,
 ( 6, 3, 6 ),
 ( 6, 6 ),
 ( 24.00348385615980007, 27.60499227840000103, 32.18191237814389893 ),
 ( -0.008403786540223459611, 2.000000000000000000 ),
 .UNSPECIFIED. ) ;
#24056=CARTESIAN_POINT ( 'NONE',  ( 12.82280136232900070, 1414.971993471380074, 197.7189074864900249 ) ) ;
#24057=ADVANCED_FACE ( 'NONE', ( #107096 ), #5753, .F. ) ;
#24058=CARTESIAN_POINT ( 'NONE',  ( 0.4435541702111918672, 1467.106087704137963, 235.5928625124542179 ) ) ;
#24059=CARTESIAN_POINT ( 'NONE',  ( 0.1144963318970000088, 1419.768049673130008, 184.3728032279979914 ) ) ;
#24062=CARTESIAN_POINT ( 'NONE',  ( -19.01829945129999899, 1486.473597083029972, 189.2492686670979936 ) ) ;
#24064=CARTESIAN_POINT ( 'NONE',  ( -17.68901833540000013, 1410.027722936829832, 224.9019810024979904 ) ) ;
#24065=CARTESIAN_POINT ( 'NONE',  ( 23.04597175290000166, 1410.910372357130200, 213.3277098939479686 ) ) ;
#24067=CARTESIAN_POINT ( 'NONE',  ( -26.69006509299999763, 1449.954382144920146, 136.5854975036980079 ) ) ;
#24071=CONICAL_SURFACE ( 'NONE', #11709, 26.99999999999998934, 0.2186689458740001812 ) ;
#24073=CARTESIAN_POINT ( 'NONE',  ( -12.37274144529999909, 1415.932840167130053, 221.9815654478979923 ) ) ;
#24074=EDGE_CURVE ( 'NONE', #51033, #76907, #56406, .T. ) ;
#24076=CARTESIAN_POINT ( 'NONE',  ( 0.1705841116430650006, 1479.986583045490079, 182.0949671867700204 ) ) ;
#24077=CARTESIAN_POINT ( 'NONE',  ( 0.01096404850135499973, 1407.225809182730018, 222.1218459625830235 ) ) ;
#24079=CARTESIAN_POINT ( 'NONE',  ( -20.75326766870000128, 1444.324653571829913, 176.0807405191980024 ) ) ;
#24080=CYLINDRICAL_SURFACE ( 'NONE', #53341, 1.500000000000001332 ) ;
#24081=CARTESIAN_POINT ( 'NONE',  ( 12.06088154280000069, 1433.903722001979986, 149.6992425274980008 ) ) ;
#24082=CARTESIAN_POINT ( 'NONE',  ( -41.37151551560999962, 1441.555306591699946, 134.0999999980749919 ) ) ;
#24084=ORIENTED_EDGE ( 'NONE', *, *, #53583, .F. ) ;
#24092=CARTESIAN_POINT ( 'NONE',  ( 22.16059216520000419, 1489.466620110430085, 210.4454289069080062 ) ) ;
#24093=LINE ( 'NONE', #66696, #18145 ) ;
#24098=CARTESIAN_POINT ( 'NONE',  ( 11.87502392341400004, 1433.007271648830056, 149.9804723818110119 ) ) ;
#24099=CARTESIAN_POINT ( 'NONE',  ( -16.61545066670979764, 1410.583136789100081, 226.4812420948509839 ) ) ;
#24100=CARTESIAN_POINT ( 'NONE',  ( 10.11781796957937551, 1428.435797280887527, 134.0999999980966777 ) ) ;
#24101=ORIENTED_EDGE ( 'NONE', *, *, #24941, .T. ) ;
#24106=DIRECTION ( 'NONE',  ( 0.000000000000000000, 0.000000000000000000, -1.000000000000000000 ) ) ;
#24107=CARTESIAN_POINT ( 'NONE',  ( -11.60004870196338445, 1428.704565730935656, 134.1356168154925967 ) ) ;
#24108=CARTESIAN_POINT ( 'NONE',  ( -17.20364854680000377, 1422.328583322830127, 226.7282386093980051 ) ) ;
#24112=CARTESIAN_POINT ( 'NONE',  ( 14.59882275810000074, 1475.513060387329915, 225.1032622602980098 ) ) ;
#24116=CARTESIAN_POINT ( 'NONE',  ( 2.707337067620000148, 1447.195466848630076, 162.7581449801980114 ) ) ;
#24117=ORIENTED_EDGE ( 'NONE', *, *, #95878, .F. ) ;
#24120=CARTESIAN_POINT ( 'NONE',  ( -0.1681676274470000065, 1420.473121337229941, 182.7663689088979879 ) ) ;
#24125=ORIENTED_EDGE ( 'NONE', *, *, #80371, .F. ) ;
#24128=CARTESIAN_POINT ( 'NONE',  ( -8.623178441291070584, 1441.178012937099993, 153.8582158015130119 ) ) ;
#24129=CARTESIAN_POINT ( 'NONE',  ( 15.79865788131630211, 1409.472960598209966, 192.7589945538530003 ) ) ;
#24132=CARTESIAN_POINT ( 'NONE',  ( 39.44884039036110579, 1439.526606209990177, 136.6633719441740027 ) ) ;
#24134=CARTESIAN_POINT ( 'NONE',  ( 33.91369110979999846, 1435.681798629080049, 135.0664268281979901 ) ) ;
#24136=CARTESIAN_POINT ( 'NONE',  ( 16.99003759221664467, 1460.417638315011573, 228.7506697972868039 ) ) ;
#24145=CARTESIAN_POINT ( 'NONE',  ( -29.49847430838659079, 1509.954514606188013, 211.0666888197964397 ) ) ;
#24146=CARTESIAN_POINT ( 'NONE',  ( 13.42479616400980014, 1453.338203267170002, 224.7140346886050111 ) ) ;
#24147=EDGE_CURVE ( 'NONE', #85990, #96481, #103721, .T. ) ;
#24151=CARTESIAN_POINT ( 'NONE',  ( -27.69670323179999727, 1508.056852025029912, 205.9292566894080210 ) ) ;
#24152=CARTESIAN_POINT ( 'NONE',  ( 42.60628464300240381, 1443.705283383309961, 135.3769922593340027 ) ) ;
#24153=CARTESIAN_POINT ( 'NONE',  ( 12.78776258895000062, 1416.851343899079893, 222.7045348340550106 ) ) ;
#24154=AXIS2_PLACEMENT_3D ( 'NONE', #86481, #9776, #43943 ) ;
#24155=CARTESIAN_POINT ( 'NONE',  ( 25.58202537360000051, 1438.616865385849906, 137.7521160916980136 ) ) ;
#24161=ORIENTED_EDGE ( 'NONE', *, *, #39751, .T. ) ;
#24162=CARTESIAN_POINT ( 'NONE',  ( 11.82387352787750068, 1429.526484542929893, 149.2201243832210196 ) ) ;
#24166=CARTESIAN_POINT ( 'NONE',  ( -13.20846943169999932, 1414.988017870030035, 220.4537675474979892 ) ) ;
#24167=CARTESIAN_POINT ( 'NONE',  ( -11.24996134802339931, 1432.343754011389819, 151.5214230697959863 ) ) ;
#24168=CARTESIAN_POINT ( 'NONE',  ( -2.382436964801009083, 1426.901689560119166, 137.0999999980979567 ) ) ;
#24171=CARTESIAN_POINT ( 'NONE',  ( -12.80774462770000000, 1422.978431755830115, 222.2455730111979904 ) ) ;
#24177=CARTESIAN_POINT ( 'NONE',  ( 24.64805363261919879, 1458.278292896679886, 206.2167562891609975 ) ) ;
#24178=CARTESIAN_POINT ( 'NONE',  ( 12.05130385160000017, 1461.808810158830056, 233.1312125915980005 ) ) ;
#24179=CARTESIAN_POINT ( 'NONE',  ( -13.72981806390609805, 1507.304744983219962, 190.9530748769740285 ) ) ;
#24184=CARTESIAN_POINT ( 'NONE',  ( -22.67879459162747224, 1409.704991073136853, 209.2849360770794362 ) ) ;
#24191=CARTESIAN_POINT ( 'NONE',  ( -11.19085206853407399, 1425.281374859042899, 138.5667630678716762 ) ) ;
#24195=CARTESIAN_POINT ( 'NONE',  ( -15.52481283598960005, 1507.483738429079949, 192.3367673041059902 ) ) ;
#24197=CARTESIAN_POINT ( 'NONE',  ( -11.72037271900000022, 1428.748239199529962, 149.7340254384980085 ) ) ;
#24204=CARTESIAN_POINT ( 'NONE',  ( -20.38765208069999701, 1482.730053243030170, 226.6937557411979753 ) ) ;
#24206=CARTESIAN_POINT ( 'NONE',  ( -1.725662463189999940, 1484.236887840130066, 182.7463278878979906 ) ) ;
#24207=EDGE_LOOP ( 'NONE', ( #1683, #59032, #94516, #12132 ) ) ;
#24209=CARTESIAN_POINT ( 'NONE',  ( 12.67286678700000024, 1407.348457837030082, 268.9829868799980090 ) ) ;
#24211=CARTESIAN_POINT ( 'NONE',  ( 22.58665416150000027, 1410.868456648429856, 206.5931427415680162 ) ) ;
#24213=CARTESIAN_POINT ( 'NONE',  ( 6.121052152493825282, 1506.452631422901959, 230.2562301517164656 ) ) ;
#24216=CARTESIAN_POINT ( 'NONE',  ( -1.835536234179999893, 1450.383119663930074, 182.7750508583980036 ) ) ;
#24217=CARTESIAN_POINT ( 'NONE',  ( -19.16951723229999871, 1456.627470220629903, 228.8719212425980061 ) ) ;
#24219=CARTESIAN_POINT ( 'NONE',  ( -13.59113641329999922, 1444.764193666879919, 188.0077009021979961 ) ) ;
#24220=CARTESIAN_POINT ( 'NONE',  ( -13.92102725570000032, 1408.913060387329779, 221.6645303301980050 ) ) ;
#24223=CARTESIAN_POINT ( 'NONE',  ( 1.459768879727899815, 1496.155829132160079, 181.5912509448299943 ) ) ;
#24226=CARTESIAN_POINT ( 'NONE',  ( 11.36285630521358136, 1425.645385257877024, 138.6334011581851087 ) ) ;
#24228=CARTESIAN_POINT ( 'NONE',  ( -3.767832703549999884, 1475.866516295129941, 267.2290101134979636 ) ) ;
#24229=B_SPLINE_CURVE_WITH_KNOTS ( 'NONE', 5,
 ( #40597, #84790, #16468, #49021, #74768, #93197 ),
 .UNSPECIFIED., .F., .F.,
 ( 6, 6 ),
 ( -84.90067530929999862, -19.14976305689999947 ),
 .UNSPECIFIED. ) ;
#24230=CARTESIAN_POINT ( 'NONE',  ( -4.240954185389510300, 1446.390260568540043, 162.6730374057570145 ) ) ;
#24236=CARTESIAN_POINT ( 'NONE',  ( 12.12507211432840037, 1416.051481377749951, 223.4385051997479934 ) ) ;
#24241=CARTESIAN_POINT ( 'NONE',  ( -16.87240674950000141, 1409.502257814230006, 196.1298176688979993 ) ) ;
#24242=B_SPLINE_CURVE_WITH_KNOTS ( 'NONE', 5,
 ( #38554, #80023, #3344, #12254, #47529, #81650 ),
 .UNSPECIFIED., .F., .F.,
 ( 6, 6 ),
 ( 0.000000000000000000, 1.000000000000000000 ),
 .UNSPECIFIED. ) ;
#24244=CARTESIAN_POINT ( 'NONE',  ( -15.08289094651999918, 1422.396364341253729, 228.4054957403699859 ) ) ;
#24245=CARTESIAN_POINT ( 'NONE',  ( -40.43468551219999796, 1425.927552745930143, 269.7751466411979777 ) ) ;
#24246=B_SPLINE_CURVE_WITH_KNOTS ( 'NONE', 3,
 ( #40178, #25977, #34404, #76969, #60176, #94293, #68577, #31770, #103237, #32336, #66516, #100082, #25423, #51771, #18684, #17571, #78060, #23366, #8633, #85907, #91679, #94864, #69133, #65957, #83281, #108487, #9212, #74902, #57556, #43372, #61303, #6579, #27118 ),
 .UNSPECIFIED., .F., .F.,
 ( 4, 2, 2, 2, 1, 1, 2, 2, 1, 2, 2, 2, 2, 2, 1, 1, 2, 2, 4 ),
 ( 0.000000000000000000, 0.1249999999959629515, 0.2499999999919259031, 0.3124999999898815939, 0.3203124999895942127, 0.3242187499894761404, 0.3261718749894179648, 0.3281249999893598446, 0.3437499999896028724, 0.3749999999900890391, 0.4999999999921616034, 0.5624999999931965533, 0.5703124999933014694, 0.5742187499933539829, 0.5781249999934063855, 0.5937499999936258765, 0.6249999999940646367, 0.7499999999959944263, 1.000000000000000000 ),
 .UNSPECIFIED. ) ;
#24248=CARTESIAN_POINT ( 'NONE',  ( -4.304798037349998904E-15, 1432.353341358199941, 150.3995506339979897 ) ) ;
#24250=CARTESIAN_POINT ( 'NONE',  ( 13.12775437374511078, 1414.913060581095351, 198.1894658563514895 ) ) ;
#24251=AXIS2_PLACEMENT_3D ( 'NONE', #39596, #73769, #31185 ) ;
#24253=CARTESIAN_POINT ( 'NONE',  ( 11.41672989679999972, 1425.493523444330094, 142.7646581281979934 ) ) ;
#24258=B_SPLINE_CURVE_WITH_KNOTS ( 'NONE', 3,
 ( #73695, #88270, #37870, #90457, #97761, #107266, #21033, #64751, #63110, #98862, #22126, #11563, #47919, #82054, #97209, #5360, #107821, #31109, #45739, #20482, #88818, #12104, #14299, #75343, #91576, #5920, #83717, #76422, #99955, #42272, #109484, #23796, #40066, #65838, #74245, #100518, #23250, #110576, #67497, #110026, #66944, #58537, #31657, #57448, #14849, #92662, #49040, #83176, #49586, #84267, #50673, #56879, #33302, #6466, #33861, #84806, #32761, #48488, #24885, #40615, #108375, #101601, #93215, #16484 ),
 .UNSPECIFIED., .F., .F.,
 ( 4, 2, 2, 1, 1, 1, 1, 1, 2, 2, 2, 2, 2, 1, 1, 1, 2, 2, 2, 2, 1, 1, 2, 2, 2, 2, 2, 2, 1, 1, 1, 2, 2, 2, 1, 1, 1, 2, 2, 4 ),
 ( 0.000000000000000000, 0.03124999999978876619, 0.04687499999969505643, 0.05468749999965903663, 0.05859374999963078839, 0.06054687499962693037, 0.06152343749961597386, 0.06201171874962137232, 0.06225585937461416280, 0.06249999999960695329, 0.09374999999852183519, 0.1093749999979896359, 0.1171874999977146059, 0.1210937499975777709, 0.1230468749975153486, 0.1240234374974771847, 0.1245117187474644865, 0.1249999999974517884, 0.1406249999974463760, 0.1484374999974328035, 0.1523437499974131804, 0.1542968749974160114, 0.1552734374974319986, 0.1562499999974480136, 0.1874999999975305587, 0.2187499999976131315, 0.2499999999976956766, 0.3749999999979625742, 0.4374999999980880294, 0.4687499999981594723, 0.4843749999981943888, 0.4921874999982117638, 0.4999999999982291943, 0.6249999999985961230, 0.6874999999987861932, 0.7187499999988812283, 0.7343749999989280797, 0.7421874999989571675, 0.7499999999989861443, 1.000000000000000000 ),
 .UNSPECIFIED. ) ;
#24262=CARTESIAN_POINT ( 'NONE',  ( -11.89217588495976230, 1398.265670798425390, 203.8704783742946063 ) ) ;
#24264=CARTESIAN_POINT ( 'NONE',  ( -22.52609270459879909, 1509.699688878229836, 190.3921826462719764 ) ) ;
#24266=CARTESIAN_POINT ( 'NONE',  ( 20.67662342439280110, 1509.571223683380140, 229.8561361637509890 ) ) ;
#24270=CARTESIAN_POINT ( 'NONE',  ( 11.44586080288440044, 1434.091157437989978, 151.3988925854559966 ) ) ;
#24271=CARTESIAN_POINT ( 'NONE',  ( -2.609101932360000209, 1396.541851151430137, 221.5905290407980033 ) ) ;
#24272=ORIENTED_EDGE ( 'NONE', *, *, #48064, .T. ) ;
#24274=CARTESIAN_POINT ( 'NONE',  ( -27.34571021120000012, 1509.867993630230103, 198.7006099054979700 ) ) ;
#24277=CARTESIAN_POINT ( 'NONE',  ( 17.01314077800000035, 1421.695136730729928, 226.8095292698980074 ) ) ;
#24278=CARTESIAN_POINT ( 'NONE',  ( 19.68479608726639896, 1507.817797212230062, 229.3453755810369898 ) ) ;
#24279=CARTESIAN_POINT ( 'NONE',  ( 13.95127933429999878, 1449.229478364299894, 189.0411395998980311 ) ) ;
#24280=CARTESIAN_POINT ( 'NONE',  ( -12.16691017849999845, 1415.934222461130048, 194.8513043958980120 ) ) ;
#24281=CARTESIAN_POINT ( 'NONE',  ( 42.28244370419900378, 1440.913053795810129, 269.8809842699980095 ) ) ;
#24283=B_SPLINE_CURVE_WITH_KNOTS ( 'NONE', 3,
 ( #51623, #86316, #61160, #109870, #76821, #34258, #101997, #26401, #93594, #9058, #16870, #9600, #43770, #60594, #85203, #679, #43229, #41569, #49968, #42664, #17425, #68440, #95277, #69551, #103672 ),
 .UNSPECIFIED., .F., .F.,
 ( 4, 3, 3, 3, 3, 3, 3, 3, 4 ),
 ( -1.000000000000000000, -0.7382082361762160039, -0.4751161948289650550, -0.2112166304481060131, 0.05257943943730047920, 0.3138547044834778532, 0.5710709172084329488, 0.8195866995882130634, 1.000000000000000000 ),
 .UNSPECIFIED. ) ;
#24284=CARTESIAN_POINT ( 'NONE',  ( 2.723978590149899848, 1396.008183815759821, 198.4466560475439962 ) ) ;
#24285=CARTESIAN_POINT ( 'NONE',  ( 1.433831019619999925, 1415.263254653229978, 191.0530033739979956 ) ) ;
#24286=CARTESIAN_POINT ( 'NONE',  ( 10.95713523929999944, 1431.451756866380038, 151.7157163214980073 ) ) ;
#24287=CARTESIAN_POINT ( 'NONE',  ( 8.429098512467547266, 1509.207532371149455, 181.0372478593424148 ) ) ;
#24289=CARTESIAN_POINT ( 'NONE',  ( 13.08462178706889922, 1434.901236159169912, 149.6929169018040113 ) ) ;
#24291=ORIENTED_EDGE ( 'NONE', *, *, #21895, .T. ) ;
#24292=CARTESIAN_POINT ( 'NONE',  ( 13.29125253233012849, 1444.599725294718382, 169.3795554700696755 ) ) ;
#24293=CARTESIAN_POINT ( 'NONE',  ( -12.54330649829999977, 1461.761650172629743, 231.4481574644979958 ) ) ;
#24298=VERTEX_POINT ( 'NONE', #44880 ) ;
#24300=CARTESIAN_POINT ( 'NONE',  ( 13.86092937120069912, 1410.765486813650114, 191.1266627561969926 ) ) ;
#24302=VECTOR ( 'NONE', #40705, 1000.000000000000000 ) ;
#24303=VECTOR ( 'NONE', #29921, 1000.000000000000000 ) ;
#24304=VERTEX_POINT ( 'NONE', #70094 ) ;
#24308=CARTESIAN_POINT ( 'NONE',  ( -20.07277539240000053, 1508.598349472430073, 229.2502111213980243 ) ) ;
#24309=CARTESIAN_POINT ( 'NONE',  ( -4.246424122129999645, 1409.061348784629899, 187.8200628337979765 ) ) ;
#24311=CARTESIAN_POINT ( 'NONE',  ( -0.8770414022454380287, 1414.913057846380070, 225.7833214945719931 ) ) ;
#24313=CARTESIAN_POINT ( 'NONE',  ( 24.26322120380000058, 1437.059134594650232, 214.0566016570280112 ) ) ;
#24317=CARTESIAN_POINT ( 'NONE',  ( 14.72001629658930000, 1412.288675752429981, 269.3627518331180113 ) ) ;
#24319=CARTESIAN_POINT ( 'NONE',  ( 24.11835951289999969, 1410.845629426529968, 209.1806383628220090 ) ) ;
#24323=DIRECTION ( 'NONE',  ( 0.000000000000000000, 0.000000000000000000, -1.000000000000000000 ) ) ;
#24329=ORIENTED_EDGE ( 'NONE', *, *, #49553, .F. ) ;
#24332=CARTESIAN_POINT ( 'NONE',  ( 36.81313714009999671, 1443.228346759079841, 254.5659540772979881 ) ) ;
#24338=CARTESIAN_POINT ( 'NONE',  ( -2.896892187767880156, 1484.263391075600111, 183.3160938869699805 ) ) ;
#24340=FACE_OUTER_BOUND ( 'NONE', #94915, .T. ) ;
#24347=EDGE_CURVE ( 'NONE', #98527, #64698, #42090, .T. ) ;
#24348=CARTESIAN_POINT ( 'NONE',  ( 23.15697666530000021, 1449.648812153099925, 217.7024929164979881 ) ) ;
#24351=CARTESIAN_POINT ( 'NONE',  ( 3.920879176457659820, 1439.701872010520219, 184.6839060028229937 ) ) ;
#24352=CARTESIAN_POINT ( 'NONE',  ( 29.18245906658470190, 1435.992869682629816, 136.4456868839280048 ) ) ;
#24353=CARTESIAN_POINT ( 'NONE',  ( 40.23461572603999059, 1444.564027027749944, 137.0370437261450149 ) ) ;
#24354=CARTESIAN_POINT ( 'NONE',  ( -23.26537802140000011, 1433.866345638330131, 213.9181200823180120 ) ) ;
#24355=CARTESIAN_POINT ( 'NONE',  ( -41.51616159369314829, 1455.119240858822195, 269.0887759631816607 ) ) ;
#24357=CARTESIAN_POINT ( 'NONE',  ( 10.82611846040000003, 1509.291116774529883, 182.2978684798979998 ) ) ;
#24359=CARTESIAN_POINT ( 'NONE',  ( -15.04391461419485054, 1469.400883903268323, 269.3648501238604922 ) ) ;
#24364=CARTESIAN_POINT ( 'NONE',  ( 15.89604526242030147, 1474.706294885379975, 189.1248889691710247 ) ) ;
#24365=CARTESIAN_POINT ( 'NONE',  ( -0.009098396902059999528, 1417.355061407530002, 235.2087950155979854 ) ) ;
#24366=CARTESIAN_POINT ( 'NONE',  ( -29.75012120250000081, 1509.993914124430148, 208.5595671623779879 ) ) ;
#24367=ADVANCED_FACE ( 'NONE', ( #44317 ), #52029, .F. ) ;
#24370=PRODUCT_DEFINITION_FORMATION_WITH_SPECIFIED_SOURCE ( 'ANY', '', #104493, .NOT_KNOWN. ) ;
#24371=CARTESIAN_POINT ( 'NONE',  ( 2.500000000000000000, 1432.302110539269961, 157.4936333739979943 ) ) ;
#24372=CARTESIAN_POINT ( 'NONE',  ( -5.943685272961615418, 1451.459285800949601, 153.4774835117595160 ) ) ;
#24373=CARTESIAN_POINT ( 'NONE',  ( 25.21503096769999885, 1435.882664665889934, 137.0280311863980103 ) ) ;
#24375=EDGE_CURVE ( 'NONE', #15354, #68835, #51563, .T. ) ;
#24376=CARTESIAN_POINT ( 'NONE',  ( -14.80327112760000041, 1409.939845700729848, 226.5217252883980166 ) ) ;
#24378=CARTESIAN_POINT ( 'NONE',  ( 1.674829163898249984, 1414.913060387399810, 192.1894932412249943 ) ) ;
#24381=ORIENTED_EDGE ( 'NONE', *, *, #103611, .F. ) ;
#24385=CARTESIAN_POINT ( 'NONE',  ( -21.72443950929999801, 1451.953218211529929, 220.8606415680980035 ) ) ;
#24388=CARTESIAN_POINT ( 'NONE',  ( -11.48286129179999904, 1433.329274650220214, 151.2855545196979961 ) ) ;
#24392=CARTESIAN_POINT ( 'NONE',  ( -24.28094609940000126, 1438.198944389940152, 211.0663462535580095 ) ) ;
#24394=CARTESIAN_POINT ( 'NONE',  ( -2.923521517025829741, 1410.394928878200062, 186.6127595807840009 ) ) ;
#24396=CARTESIAN_POINT ( 'NONE',  ( -29.52699855556750208, 1510.054681897895989, 203.5615033681672230 ) ) ;
#24398=CARTESIAN_POINT ( 'NONE',  ( -1.238275708498259911E-09, 1416.572336828779953, 238.6617246227660019 ) ) ;
#24399=VERTEX_POINT ( 'NONE', #39189 ) ;
#24400=ORIENTED_EDGE ( 'NONE', *, *, #62050, .F. ) ;
#24401=CARTESIAN_POINT ( 'NONE',  ( -11.74192897671919944, 1426.699235643070097, 144.5141135958380119 ) ) ;
#24403=CARTESIAN_POINT ( 'NONE',  ( -7.520399231549999008, 1473.125808901829942, 270.3839821968980459 ) ) ;
#24404=CARTESIAN_POINT ( 'NONE',  ( -1.556370157619999972, 1414.996444526030018, 226.5294865527980051 ) ) ;
#24408=DIRECTION ( 'NONE',  ( 0.2902388374169100338, -0.1068831630355692452, -0.9509665644566018816 ) ) ;
#24411=CARTESIAN_POINT ( 'NONE',  ( -10.65372266856249972, 1406.685601047840009, 268.4360227182569929 ) ) ;
#24413=CARTESIAN_POINT ( 'NONE',  ( -13.42238899811910002, 1434.957430979650098, 149.2077055965390002 ) ) ;
#24414=VERTEX_POINT ( 'NONE', #38643 ) ;
#24417=ORIENTED_EDGE ( 'NONE', *, *, #3542, .T. ) ;
#24418=CARTESIAN_POINT ( 'NONE',  ( 4.868531005982084103, 1422.373029460236467, 184.3158709850344508 ) ) ;
#24423=CARTESIAN_POINT ( 'NONE',  ( -16.85472157044729968, 1498.343964390320025, 229.6923633532749989 ) ) ;
#24427=CARTESIAN_POINT ( 'NONE',  ( -4.363122561674769528, 1421.971318449149976, 184.5104913919989826 ) ) ;
#24429=CARTESIAN_POINT ( 'NONE',  ( -1.430117442880000089, 1408.963001188930093, 194.1218459369979996 ) ) ;
#24430=FACE_OUTER_BOUND ( 'NONE', #85309, .T. ) ;
#24431=CARTESIAN_POINT ( 'NONE',  ( -37.88774006571790665, 1442.824633575369944, 137.1073183462600014 ) ) ;
#24433=CARTESIAN_POINT ( 'NONE',  ( -23.55026106900000116, 1411.110742672429751, 210.4800087176980128 ) ) ;
#24434=CARTESIAN_POINT ( 'NONE',  ( 28.18850436520000358, 1508.134789600230079, 209.7835208149050175 ) ) ;
#24437=CARTESIAN_POINT ( 'NONE',  ( -24.03198776159999994, 1435.355284493859926, 137.0425515896980073 ) ) ;
#24438=CARTESIAN_POINT ( 'NONE',  ( -24.34268549840000162, 1442.549315796029759, 212.2035716145279878 ) ) ;
#24441=CARTESIAN_POINT ( 'NONE',  ( -2.896892187767880156, 1484.263391075600111, 183.3160938869699805 ) ) ;
#24443=CARTESIAN_POINT ( 'NONE',  ( -14.00253459870000228, 1430.158944055929851, 222.3204534089979916 ) ) ;
#24447=CARTESIAN_POINT ( 'NONE',  ( -40.71747596959829707, 1438.773003713930166, 134.4203395907470053 ) ) ;
#24449=CARTESIAN_POINT ( 'NONE',  ( -19.54853263967898158, 1457.140775842711719, 225.9785477345730271 ) ) ;
#24450=ORIENTED_EDGE ( 'NONE', *, *, #62279, .T. ) ;
#24452=CARTESIAN_POINT ( 'NONE',  ( 12.72351525216199875, 1435.772547898509856, 150.8350212812320024 ) ) ;
#24453=CARTESIAN_POINT ( 'NONE',  ( -4.116135330806149462, 1441.427949229778278, 184.2827671596340906 ) ) ;
#24455=CARTESIAN_POINT ( 'NONE',  ( 2.471608048749999842, 1438.194204504490017, 150.4833623973980252 ) ) ;
#24460=CARTESIAN_POINT ( 'NONE',  ( -11.88140585900000090, 1433.447543843229823, 147.6490162021979984 ) ) ;
#24461=CARTESIAN_POINT ( 'NONE',  ( 20.11539126239999931, 1508.359231766530002, 189.1805378999980007 ) ) ;
#24465=FACE_OUTER_BOUND ( 'NONE', #9037, .T. ) ;
#24467=CARTESIAN_POINT ( 'NONE',  ( 2.412180996239999597, 1419.421713268930034, 185.1536642287979930 ) ) ;
#24476=CARTESIAN_POINT ( 'NONE',  ( 18.25964269232630599, 1425.332953396113226, 224.8491606838273356 ) ) ;
#24477=ADVANCED_FACE ( 'NONE', ( #30135 ), #20619, .T. ) ;
#24478=CARTESIAN_POINT ( 'NONE',  ( -8.335430188334420131E-07, 1408.657067462929945, 223.1089253223800313 ) ) ;
#24479=CARTESIAN_POINT ( 'NONE',  ( 27.50547257934209711, 1446.424453580260206, 137.1666655437190059 ) ) ;
#24480=B_SPLINE_CURVE_WITH_KNOTS ( 'NONE', 3,
 ( #61353, #41752, #94344, #68091, #69185, #42306, #103869, #67533, #102203, #93786, #59132, #75911, #334, #34460, #17062, #68637, #94921, #102737, #26598, #18194, #52391, #86514, #27169, #101633, #95473, #18740, #24922, #85392, #33895, #50709, #84840, #8140, #96018, #71967, #20397, #1990, #97128, #63558, #3647, #19290, #106078, #2546, #97673 ),
 .UNSPECIFIED., .F., .F.,
 ( 4, 3, 3, 3, 3, 3, 3, 3, 3, 3, 3, 3, 3, 3, 4 ),
 ( -2.000000000000000000, -1.920433884135369862, -1.776779042643749973, -1.631085684125360036, -1.484142407439499989, -1.335324404072970150, -1.185565806898190022, -1.035185577921500011, -0.8845459646997599901, -0.7342798813318649476, -0.5847724199270629697, -0.4363642902088080699, -0.2893200053190718712, -0.1438262832493450993, 0.000000000000000000 ),
 .UNSPECIFIED. ) ;
#24482=DIRECTION ( 'NONE',  ( -0.03489950421557262011, 0.9993908267567336301, 7.330759870573984416E-09 ) ) ;
#24483=CARTESIAN_POINT ( 'NONE',  ( 12.88130326439999784, 1419.881202692929946, 222.3734530188980045 ) ) ;
#24487=CARTESIAN_POINT ( 'NONE',  ( -19.66847414439826380, 1485.263780816827648, 190.3137200183769551 ) ) ;
#24489=CARTESIAN_POINT ( 'NONE',  ( -28.66995855460000087, 1509.914237400329966, 211.4901977112579914 ) ) ;
#24490=CARTESIAN_POINT ( 'NONE',  ( -12.87618670773889917, 1416.835419214280137, 221.9337012713420165 ) ) ;
#24491=LINE ( 'NONE', #93359, #102063 ) ;
#24495=CARTESIAN_POINT ( 'NONE',  ( 10.89003754610000030, 1451.711500069930025, 152.2142025596980091 ) ) ;
#24502=CARTESIAN_POINT ( 'NONE',  ( 19.78518508183620028, 1508.106391392640035, 229.3111777015780035 ) ) ;
#24504=VERTEX_POINT ( 'NONE', #88946 ) ;
#24506=CARTESIAN_POINT ( 'NONE',  ( 38.59693733168150231, 1439.219610169110183, 136.6571113115409730 ) ) ;
#24507=DIRECTION ( 'NONE',  ( 1.000000000000000000, 0.000000000000000000, 0.000000000000000000 ) ) ;
#24512=CARTESIAN_POINT ( 'NONE',  ( -12.02002121700249937, 1447.120365805550136, 187.5076542713389927 ) ) ;
#24513=CARTESIAN_POINT ( 'NONE',  ( -11.92890078398071552, 1435.343914765019463, 151.2188616800775094 ) ) ;
#24516=CARTESIAN_POINT ( 'NONE',  ( 1.031770593039999850, 1409.117028087930066, 185.7659931841980097 ) ) ;
#24517=CARTESIAN_POINT ( 'NONE',  ( 4.359264906129999950, 1423.889211762329978, 184.2836487311979852 ) ) ;
#24519=CARTESIAN_POINT ( 'NONE',  ( -2.499999999849909837, 1439.824763698960169, 159.3159658887090018 ) ) ;
#24521=CARTESIAN_POINT ( 'NONE',  ( 11.86590139589999815, 1432.348266868109931, 151.0567667964980103 ) ) ;
#24523=CARTESIAN_POINT ( 'NONE',  ( -0.8141018274779999730, 1430.453334911130241, 150.3332009510979788 ) ) ;
#24524=CARTESIAN_POINT ( 'NONE',  ( -3.949444845858078867, 1427.113443899376762, 134.0999999980980135 ) ) ;
#24525=( BOUNDED_CURVE ( )  B_SPLINE_CURVE ( 3, ( #98855, #46290, #47912, #82047 ),
 .UNSPECIFIED., .F., .F. ) 
 B_SPLINE_CURVE_WITH_KNOTS ( ( 4, 4 ),
 ( 1.036083073916405750, 2.105411660058823298 ),
 .UNSPECIFIED. ) 
 CURVE ( )  GEOMETRIC_REPRESENTATION_ITEM ( )  RATIONAL_B_SPLINE_CURVE ( ( 1.000000000000000000, 0.9069598253101942564, 0.9069598253101942564, 1.000000000000000000 ) ) 
 REPRESENTATION_ITEM ( '' )  );
#24526=CARTESIAN_POINT ( 'NONE',  ( 15.42454884180000008, 1430.140040983930021, 190.9214399110979912 ) ) ;
#24527=CARTESIAN_POINT ( 'NONE',  ( -8.328873504844570907E-09, 1475.098823578779957, 265.5557250396390145 ) ) ;
#24528=CARTESIAN_POINT ( 'NONE',  ( 20.48353907805949703, 1436.444560210333520, 144.9117583361570780 ) ) ;
#24529=FACE_OUTER_BOUND ( 'NONE', #55449, .T. ) ;
#24532=CARTESIAN_POINT ( 'NONE',  ( -0.06018024750005197820, 1486.202617829743531, 181.8162541669730103 ) ) ;
#24534=CARTESIAN_POINT ( 'NONE',  ( -46.01983168967480253, 1438.258892378159771, 268.2089072814339943 ) ) ;
#24535=CARTESIAN_POINT ( 'NONE',  ( -2.499999999859999988, 1439.640830480200293, 184.0873493999980042 ) ) ;
#24538=CARTESIAN_POINT ( 'NONE',  ( -5.386101783710000035, 1432.347042943159977, 154.6076477470979853 ) ) ;
#24541=CARTESIAN_POINT ( 'NONE',  ( -25.18522889079570248, 1452.033591493209769, 135.3780775317339931 ) ) ;
#24543=CARTESIAN_POINT ( 'NONE',  ( 7.587264836529999279, 1421.907226632029960, 217.1547583186280121 ) ) ;
#24547=CARTESIAN_POINT ( 'NONE',  ( -15.52964687406499955, 1451.324136384999974, 222.4830579234560162 ) ) ;
#24552=CARTESIAN_POINT ( 'NONE',  ( 1.600048698852036821, 1411.254281879943164, 135.5999999980979851 ) ) ;
#24553=CARTESIAN_POINT ( 'NONE',  ( 16.03409403789510179, 1422.997244933739921, 228.9049390009139984 ) ) ;
#24556=ORIENTED_EDGE ( 'NONE', *, *, #62414, .T. ) ;
#24557=CARTESIAN_POINT ( 'NONE',  ( -23.81602722030639896, 1410.419941936439955, 209.8068453827619919 ) ) ;
#24561=CARTESIAN_POINT ( 'NONE',  ( -8.968501251859999357, 1428.602659895330135, 101.8807690336980016 ) ) ;
#24562=CARTESIAN_POINT ( 'NONE',  ( -1.919144336779999849, 1507.641079666230098, 237.0664109672979976 ) ) ;
#24563=CARTESIAN_POINT ( 'NONE',  ( -18.99570766729999960, 1410.874976135429733, 222.9834657993979761 ) ) ;
#24564=CARTESIAN_POINT ( 'NONE',  ( 40.83400096486530373, 1456.643151761250010, 266.3273196274960242 ) ) ;
#24567=CARTESIAN_POINT ( 'NONE',  ( -17.12001958753553765, 1422.219426602513295, 226.7452668728065248 ) ) ;
#24570=CARTESIAN_POINT ( 'NONE',  ( 18.73173501632924953, 1458.223697907665837, 227.3016765217417401 ) ) ;
#24579=CARTESIAN_POINT ( 'NONE',  ( 22.27637251949999708, 1409.690968457230156, 211.0033668272880050 ) ) ;
#24581=CARTESIAN_POINT ( 'NONE',  ( 2.570960541213360262, 1409.002840307820179, 187.0877483113689834 ) ) ;
#24583=DIRECTION ( 'NONE',  ( 0.02978939777567089775, 0.9648997004021163670, 0.2609236668914279300 ) ) ;
#24585=CARTESIAN_POINT ( 'NONE',  ( 1.530059654846469996, 1452.704397329589938, 183.4894956925679992 ) ) ;
#24587=CARTESIAN_POINT ( 'NONE',  ( 16.19464330292652932, 1423.010950068178090, 229.4833128991568287 ) ) ;
#24591=CARTESIAN_POINT ( 'NONE',  ( 17.21411468017923596, 1414.941240534613826, 210.6779454605140813 ) ) ;
#24595=CARTESIAN_POINT ( 'NONE',  ( 13.15804437931859994, 1421.151500651059905, 221.7660300441250172 ) ) ;
#24596=CARTESIAN_POINT ( 'NONE',  ( -20.14739811709999984, 1469.497636830730016, 271.1218459616979999 ) ) ;
#24598=CARTESIAN_POINT ( 'NONE',  ( 11.84937012939999867, 1433.469328321039939, 150.5730835599980253 ) ) ;
#24599=CARTESIAN_POINT ( 'NONE',  ( 26.42894384599999924, 1460.505561531929970, 262.6648722511980054 ) ) ;
#24600=CARTESIAN_POINT ( 'NONE',  ( 12.13987205295800109, 1415.426207913209964, 196.5375152356580202 ) ) ;
#24601=CARTESIAN_POINT ( 'NONE',  ( 1.420259601960000229, 1466.712985171129958, 235.0376566307980113 ) ) ;
#24603=CARTESIAN_POINT ( 'NONE',  ( -15.06279480623459222, 1422.388301958798820, 229.4662111127462651 ) ) ;
#24604=CARTESIAN_POINT ( 'NONE',  ( -19.36475817619999873, 1485.943425245129902, 190.1135902501980013 ) ) ;
#24605=CARTESIAN_POINT ( 'NONE',  ( 12.84736500079448440, 1398.293695667951624, 211.5699839868841252 ) ) ;
#24606=CARTESIAN_POINT ( 'NONE',  ( 18.63578313170000200, 1416.568813547830132, 209.6898099495820134 ) ) ;
#24608=CARTESIAN_POINT ( 'NONE',  ( 22.14275666300000012, 1410.906117087829898, 215.7312451241079998 ) ) ;
#24609=DIRECTION ( 'NONE',  ( 0.000000000000000000, 0.000000000000000000, -1.000000000000000000 ) ) ;
#24614=CARTESIAN_POINT ( 'NONE',  ( 0.1692191542157840123, 1480.788586062970126, 182.0605159988109847 ) ) ;
#24615=CARTESIAN_POINT ( 'NONE',  ( 0.06764665397380001388, 1408.848989337130206, 223.4935224561980078 ) ) ;
#24616=ORIENTED_EDGE ( 'NONE', *, *, #69977, .T. ) ;
#24617=CARTESIAN_POINT ( 'NONE',  ( -18.64337105059427913, 1444.324653571828549, 162.1710875046049694 ) ) ;
#24618=FACE_OUTER_BOUND ( 'NONE', #4353, .T. ) ;
#24620=CARTESIAN_POINT ( 'NONE',  ( -41.61795676491179563, 1442.846609225109887, 134.0999999981039821 ) ) ;
#24626=CARTESIAN_POINT ( 'NONE',  ( -19.59053950279439960, 1486.265866315750145, 189.8955481462990065 ) ) ;
#24630=CARTESIAN_POINT ( 'NONE',  ( 0.4720966309508138892, 1418.692307282306956, 184.7100086785088138 ) ) ;
#24631=DIRECTION ( 'NONE',  ( -1.987380029059999976E-13, 6.832419524060000430E-15, 1.000000000000000000 ) ) ;
#24632=CARTESIAN_POINT ( 'NONE',  ( 7.121584085660000341, 1409.161751583630121, 222.2855843900980233 ) ) ;
#24633=CARTESIAN_POINT ( 'NONE',  ( 3.429372500519999978, 1436.958971107729894, 184.6577026058980096 ) ) ;
#24638=CARTESIAN_POINT ( 'NONE',  ( 11.89922653334599012, 1433.329005341657876, 149.9506340396733890 ) ) ;
#24639=CARTESIAN_POINT ( 'NONE',  ( 12.29654148988069373, 1442.773887286368335, 164.4841150006940325 ) ) ;
#24641=ORIENTED_EDGE ( 'NONE', *, *, #93320, .F. ) ;
#24646=CARTESIAN_POINT ( 'NONE',  ( 41.71654787359375405, 1444.824798330285603, 269.6421161746990265 ) ) ;
#24648=CARTESIAN_POINT ( 'NONE',  ( 15.51696353740144296, 1431.230679900481618, 219.3923223260254645 ) ) ;
#24653=CIRCLE ( 'NONE', #96235, 3.993878626057317582 ) ;
#24657=CARTESIAN_POINT ( 'NONE',  ( 3.116758655549999979, 1446.591766555970025, 170.5446539970980098 ) ) ;
#24660=CARTESIAN_POINT ( 'NONE',  ( 14.45771163620000088, 1416.835808384130132, 196.8517379759979917 ) ) ;
#24662=VERTEX_POINT ( 'NONE', #55921 ) ;
#24668=CARTESIAN_POINT ( 'NONE',  ( -23.30790377659999990, 1410.912174224829869, 205.7308725902679782 ) ) ;
#24669=CARTESIAN_POINT ( 'NONE',  ( -11.34647335060000017, 1426.876719822230143, 115.9728140669979979 ) ) ;
#24670=CARTESIAN_POINT ( 'NONE',  ( 15.78650398947750055, 1409.847271299810018, 191.9459370198140107 ) ) ;
#24673=CARTESIAN_POINT ( 'NONE',  ( 41.44218962868909983, 1442.560172593170137, 136.4421865476589915 ) ) ;
#24675=CARTESIAN_POINT ( 'NONE',  ( -33.67851661499999949, 1421.560016960630037, 261.9077615516980586 ) ) ;
#24676=CARTESIAN_POINT ( 'NONE',  ( -0.2678627835216980113, 1508.980470044890126, 179.3639230931030113 ) ) ;
#24677=ADVANCED_FACE ( 'NONE', ( #48059 ), #50201, .F. ) ;
#24678=CARTESIAN_POINT ( 'NONE',  ( 16.47155471125729420, 1460.849993040709023, 229.0965666438152937 ) ) ;
#24682=CARTESIAN_POINT ( 'NONE',  ( -36.78701199996249471, 1437.792136250990097, 136.5523556798590050 ) ) ;
#24683=ORIENTED_EDGE ( 'NONE', *, *, #27042, .F. ) ;
#24685=CARTESIAN_POINT ( 'NONE',  ( -18.62496937760000293, 1457.110903083630092, 228.9008583485980353 ) ) ;
#24686=EDGE_LOOP ( 'NONE', ( #84345, #12999, #35640 ) ) ;
#24687=ORIENTED_EDGE ( 'NONE', *, *, #107537, .F. ) ;
#24692=FACE_OUTER_BOUND ( 'NONE', #10970, .T. ) ;
#24695=CARTESIAN_POINT ( 'NONE',  ( 40.71747596959940552, 1438.773003713930166, 134.4205483767809994 ) ) ;
#24697=CARTESIAN_POINT ( 'NONE',  ( 25.47948162479999823, 1436.582469785759940, 137.1757940733980092 ) ) ;
#24705=CARTESIAN_POINT ( 'NONE',  ( 11.79866176452289928, 1428.170196302150089, 148.1141846266930031 ) ) ;
#24708=CARTESIAN_POINT ( 'NONE',  ( -14.35445997400000095, 1416.822690122629865, 221.5782749823979998 ) ) ;
#24709=CARTESIAN_POINT ( 'NONE',  ( -11.69294445086449841, 1432.337845643199898, 150.8474197947550124 ) ) ;
#24713=CARTESIAN_POINT ( 'NONE',  ( 21.84956437405869778, 1409.868736151659959, 206.3073818229169945 ) ) ;
#24717=CARTESIAN_POINT ( 'NONE',  ( -7.272433915116270242, 1410.543391134071953, 187.5337605366746629 ) ) ;
#24729=CARTESIAN_POINT ( 'NONE',  ( -2.945604300558919864, 1485.274571919582741, 182.9922692145212864 ) ) ;
#24730=CARTESIAN_POINT ( 'NONE',  ( -11.60004869885203505, 1426.083046513046838, 138.9256368688967314 ) ) ;
#24735=CARTESIAN_POINT ( 'NONE',  ( -11.54217015299999893, 1429.750359027530067, 150.6915807595979970 ) ) ;
#24736=CARTESIAN_POINT ( 'NONE',  ( 19.05886514166099843, 1456.926298666380035, 225.3128034416440073 ) ) ;
#24737=CARTESIAN_POINT ( 'NONE',  ( -5.930039503890000674, 1441.838256304279867, 183.8171696374980115 ) ) ;
#24738=CARTESIAN_POINT ( 'NONE',  ( 9.298374091227790572, 1424.634616539950230, 149.7551418246100070 ) ) ;
#24740=CARTESIAN_POINT ( 'NONE',  ( -2.488082932330000219, 1441.600846913620217, 150.5962877614979902 ) ) ;
#24741=CARTESIAN_POINT ( 'NONE',  ( -22.76497971890000116, 1482.723760643630158, 222.4289363302980007 ) ) ;
#24746=CARTESIAN_POINT ( 'NONE',  ( 23.72605694800000009, 1410.650267468229913, 267.6119861631980257 ) ) ;
#24749=CARTESIAN_POINT ( 'NONE',  ( 17.85928734389999661, 1430.310748820929803, 191.7175708229979705 ) ) ;
#24750=AXIS2_PLACEMENT_3D ( 'NONE', #104753, #44876, #96356 ) ;
#24751=CARTESIAN_POINT ( 'NONE',  ( -0.08548173663637460840, 1507.632698406310283, 237.3720899768290167 ) ) ;
#24753=CARTESIAN_POINT ( 'NONE',  ( -1.442473716300000097, 1451.217997451130032, 183.7279619786979765 ) ) ;
#24754=CARTESIAN_POINT ( 'NONE',  ( -9.822264486677861081E-06, 1450.913060148159957, 181.2410907034809782 ) ) ;
#24756=CARTESIAN_POINT ( 'NONE',  ( -14.34064213879999983, 1445.290870928000004, 188.7064315755980033 ) ) ;
#24757=CARTESIAN_POINT ( 'NONE',  ( -21.45452449210000267, 1497.713060387329961, 213.1853964382480058 ) ) ;
#24765=CARTESIAN_POINT ( 'NONE',  ( -7.031059539510000178, 1475.166475290029894, 269.2761626991979824 ) ) ;
#24772=CARTESIAN_POINT ( 'NONE',  ( 11.34486003903470142, 1415.059973078959956, 222.6680858266069833 ) ) ;
#24775=CYLINDRICAL_SURFACE ( 'NONE', #73318, 1.455175085940062507 ) ;
#24776=CARTESIAN_POINT ( 'NONE',  ( -17.99954287939999986, 1410.904693930530129, 195.2564708288979887 ) ) ;
#24786=CARTESIAN_POINT ( 'NONE',  ( -22.04779405809999915, 1409.847308038730034, 211.6317860905479904 ) ) ;
#24788=CARTESIAN_POINT ( 'NONE',  ( 11.73663431677760016, 1426.696239189569951, 144.1418624741639860 ) ) ;
#24790=DIRECTION ( 'NONE',  ( 2.343158368729999945E-19, 1.387778780780000088E-15, -1.000000000000000000 ) ) ;
#24792=CARTESIAN_POINT ( 'NONE',  ( -0.05087723766931040448, 1408.368774909099784, 222.6640242851099742 ) ) ;
#24795=CARTESIAN_POINT ( 'NONE',  ( -12.78681252341862340, 1398.292084349547167, 211.4732289992830374 ) ) ;
#24799=CARTESIAN_POINT ( 'NONE',  ( 20.30811166882689989, 1509.558778732829978, 230.1713494956079842 ) ) ;
#24803=ORIENTED_EDGE ( 'NONE', *, *, #36340, .T. ) ;
#24804=CARTESIAN_POINT ( 'NONE',  ( 12.00598652703259894, 1433.712414975789898, 150.0453429833439998 ) ) ;
#24805=CARTESIAN_POINT ( 'NONE',  ( -13.31360989399999895, 1398.307674596630022, 207.3550467807280029 ) ) ;
#24808=EDGE_CURVE ( 'NONE', #6602, #56560, #57027, .T. ) ;
#24810=DIRECTION ( 'NONE',  ( -1.000000000000000000, 0.000000000000000000, 0.000000000000000000 ) ) ;
#24812=CARTESIAN_POINT ( 'NONE',  ( -13.73987724751260053, 1508.184446304589983, 184.1670646690170088 ) ) ;
#24813=CARTESIAN_POINT ( 'NONE',  ( 18.89293537649999877, 1507.815827870629846, 229.9105837539979973 ) ) ;
#24814=CARTESIAN_POINT ( 'NONE',  ( 2.377993551410000350, 1468.705613521729902, 182.9807957255980000 ) ) ;
#24815=EDGE_CURVE ( 'NONE', #77110, #24021, #84409, .T. ) ;
#24816=CARTESIAN_POINT ( 'NONE',  ( -5.281923854050000422, 1415.931391677429929, 191.9559905162979874 ) ) ;
#24818=B_SPLINE_SURFACE_WITH_KNOTS ( 'NONE', 5, 5, ( 
 ( #75338, #110021, #99394, #22673, #61316, #42822 ),
 ( #17583, #69711, #52894, #18698, #93742, #26560 ),
 ( #85350, #43927, #78073, #1376, #10885, #10314 ),
 ( #34961, #1949, #25437, #53452, #69145, #103249 ),
 ( #8647, #76984, #68589, #59631, #17020, #9226 ),
 ( #291, #27678, #94305, #18153, #834, #51783 ) ),
 .UNSPECIFIED., .F., .F., .F.,
 ( 6, 6 ),
 ( 6, 6 ),
 ( 4.770714915030000114, 5.109858025250000324 ),
 ( 0.000000000000000000, 2.000000000000000000 ),
 .UNSPECIFIED. ) ;
#24820=CARTESIAN_POINT ( 'NONE',  ( 2.500020115319840031, 1419.382923540379807, 144.1035841389490031 ) ) ;
#24821=CARTESIAN_POINT ( 'NONE',  ( 11.75937283610000073, 1431.557362424269968, 150.7646243546980145 ) ) ;
#24823=ORIENTED_EDGE ( 'NONE', *, *, #104271, .F. ) ;
#24824=CARTESIAN_POINT ( 'NONE',  ( 13.04096353016549870, 1435.727353653040154, 150.6338561105279723 ) ) ;
#24825=ORIENTED_EDGE ( 'NONE', *, *, #75427, .T. ) ;
#24828=CARTESIAN_POINT ( 'NONE',  ( 13.36968693692587706, 1444.477217224934293, 169.3716362414181162 ) ) ;
#24829=CARTESIAN_POINT ( 'NONE',  ( -8.255467981419998935, 1463.782943827829968, 233.8280712257979985 ) ) ;
#24834=B_SPLINE_SURFACE_WITH_KNOTS ( 'NONE', 5, 5, ( 
 ( #94360, #104993, #69200, #61919, #87086, #54074 ),
 ( #10938, #43991, #103307, #1430, #2564, #10370 ),
 ( #27184, #18208, #88200, #52951, #86528, #78126 ),
 ( #60811, #17641, #52405, #45669, #70881, #28284 ),
 ( #96599, #19870, #11494, #44544, #102753, #61367 ),
 ( #51842, #9279, #95487, #43439, #78689, #77590 ) ),
 .UNSPECIFIED., .F., .F., .F.,
 ( 6, 6 ),
 ( 6, 6 ),
 ( 7.590234162189999800, 19.60754526079999849 ),
 ( 0.1222658846940000016, 0.5999999999999999778 ),
 .UNSPECIFIED. ) ;
#24836=EDGE_CURVE ( 'NONE', #56666, #98856, #62308, .T. ) ;
#24838=CARTESIAN_POINT ( 'NONE',  ( 2.500000000000000000, 1448.231796796869958, 166.4378714439059763 ) ) ;
#24840=( BOUNDED_CURVE ( )  B_SPLINE_CURVE ( 3, ( #85130, #36391, #86794, #77851 ),
 .UNSPECIFIED., .F., .F. ) 
 B_SPLINE_CURVE_WITH_KNOTS ( ( 4, 4 ),
 ( 1.953429545882020113, 2.601599304719214967 ),
 .UNSPECIFIED. ) 
 CURVE ( )  GEOMETRIC_REPRESENTATION_ITEM ( )  RATIONAL_B_SPLINE_CURVE ( ( 1.000000000000000000, 0.9652950237418777002, 0.9652950237418777002, 1.000000000000000000 ) ) 
 REPRESENTATION_ITEM ( '' )  );
#24843=ORIENTED_EDGE ( 'NONE', *, *, #43925, .F. ) ;
#24844=CARTESIAN_POINT ( 'NONE',  ( 20.57595172751539891, 1440.913060387330006, 219.9584118754960116 ) ) ;
#24845=CARTESIAN_POINT ( 'NONE',  ( -18.68654022859999841, 1509.565608751230002, 231.3997216384979936 ) ) ;
#24846=CARTESIAN_POINT ( 'NONE',  ( -12.92009008149999971, 1409.866466474230037, 189.8912044915980175 ) ) ;
#24848=CARTESIAN_POINT ( 'NONE',  ( 0.09392264341561619434, 1415.426561690370136, 226.6233626858019932 ) ) ;
#24849=ORIENTED_EDGE ( 'NONE', *, *, #46735, .T. ) ;
#24850=CARTESIAN_POINT ( 'NONE',  ( 21.66194437680000107, 1429.187467587929859, 218.7319503095280027 ) ) ;
#24854=CARTESIAN_POINT ( 'NONE',  ( 0.0007013484591967420129, 1465.026770150519951, 237.7732560087259799 ) ) ;
#24855=VECTOR ( 'NONE', #34631, 1000.000000000000114 ) ;
#24856=EDGE_CURVE ( 'NONE', #74077, #72398, #58695, .T. ) ;
#24863=CARTESIAN_POINT ( 'NONE',  ( 13.55937162340000057, 1409.552479690230030, 191.5919554294980003 ) ) ;
#24864=CARTESIAN_POINT ( 'NONE',  ( -9.140833745038642988, 1486.006228221076299, 183.5277714374079778 ) ) ;
#24866=ORIENTED_EDGE ( 'NONE', *, *, #65604, .T. ) ;
#24868=CARTESIAN_POINT ( 'NONE',  ( 33.66409353290000439, 1447.474031022650252, 250.0355534076980177 ) ) ;
#24873=CARTESIAN_POINT ( 'NONE',  ( -4.219439023932549659, 1446.230224804030058, 183.1418048969109975 ) ) ;
#24875=DIRECTION ( 'NONE',  ( 1.000000000000000000, 6.438966932878399974E-12, 0.000000000000000000 ) ) ;
#24877=VERTEX_POINT ( 'NONE', #70404 ) ;
#24879=CARTESIAN_POINT ( 'NONE',  ( 0.2302825872959999853, 1467.622811642030001, 229.4111514478979927 ) ) ;
#24881=CARTESIAN_POINT ( 'NONE',  ( -4.194822514691770311E-06, 1471.586156170330014, 269.6149383081970541 ) ) ;
#24885=CARTESIAN_POINT ( 'NONE',  ( 7.092997891250118592, 1416.799648712304588, 231.0433554185687512 ) ) ;
#24886=CARTESIAN_POINT ( 'NONE',  ( 32.03033759198009278, 1435.776089609319797, 136.0024512530590073 ) ) ;
#24888=CARTESIAN_POINT ( 'NONE',  ( 38.97393047930350463, 1447.767677101680192, 136.5281119700379975 ) ) ;
#24889=CARTESIAN_POINT ( 'NONE',  ( -4.038220123662581429, 1450.278798041637629, 185.0006713385352839 ) ) ;
#24891=CARTESIAN_POINT ( 'NONE',  ( 14.23428072729999982, 1509.239486858130022, 184.7798516627979666 ) ) ;
#24896=CARTESIAN_POINT ( 'NONE',  ( -2.802202849542238638, 1406.777768078013423, 269.6500898821890928 ) ) ;
#24900=CARTESIAN_POINT ( 'NONE',  ( 10.98324908544952727, 1424.969403672227372, 138.3333100251041401 ) ) ;
#24902=CARTESIAN_POINT ( 'NONE',  ( -12.89480376717877341, 1444.937738581603526, 186.1394114880380926 ) ) ;
#24907=CARTESIAN_POINT ( 'NONE',  ( -7.859519671404137320, 1451.394139414346682, 152.9865962971728663 ) ) ;
#24909=CARTESIAN_POINT ( 'NONE',  ( 24.88936805819999876, 1435.366663778739849, 135.7839653261980004 ) ) ;
#24910=CARTESIAN_POINT ( 'NONE',  ( -12.93237811294222439, 1442.909190189631317, 169.4316757962859299 ) ) ;
#24913=CARTESIAN_POINT ( 'NONE',  ( 0.5259141656908821183, 1414.913057855109855, 192.6235218337679953 ) ) ;
#24914=CARTESIAN_POINT ( 'NONE',  ( -2.820494496349999825, 1409.011554225530062, 231.0801550522980108 ) ) ;
#24915=ORIENTED_EDGE ( 'NONE', *, *, #65232, .F. ) ;
#24920=CARTESIAN_POINT ( 'NONE',  ( -10.70690149680000047, 1457.973036634730079, 211.8464313850780059 ) ) ;
#24922=CARTESIAN_POINT ( 'NONE',  ( 4.151090981929720591, 1424.289371950179884, 184.6289891318990044 ) ) ;
#24924=CONICAL_SURFACE ( 'NONE', #33828, 1.000000000000009104, 0.7853981633970000820 ) ;
#24925=CARTESIAN_POINT ( 'NONE',  ( -2.502901717667406434, 1421.086235556830388, 185.1090482811913489 ) ) ;
#24927=CARTESIAN_POINT ( 'NONE',  ( -24.82841969249999892, 1439.350353960880057, 210.4303024200779930 ) ) ;
#24931=CARTESIAN_POINT ( 'NONE',  ( -21.85598295049956619, 1509.793014696267164, 229.6769293903243749 ) ) ;
#24935=CARTESIAN_POINT ( 'NONE',  ( -11.80507841927059864, 1428.482117788079904, 148.4348042808990158 ) ) ;
#24936=DIRECTION ( 'NONE',  ( -3.828588921590000582E-16, 0.000000000000000000, 1.000000000000000000 ) ) ;
#24937=CARTESIAN_POINT ( 'NONE',  ( -7.932950196699999346, 1470.889844930330128, 269.3427102504979871 ) ) ;
#24940=CARTESIAN_POINT ( 'NONE',  ( 22.44565107540000071, 1519.913060387329779, 204.8661566055479852 ) ) ;
#24941=EDGE_CURVE ( 'NONE', #21200, #82793, #26148, .T. ) ;
#24944=CARTESIAN_POINT ( 'NONE',  ( -19.68294476550000027, 1431.113060387329824, 208.1462084707240194 ) ) ;
#24946=CARTESIAN_POINT ( 'NONE',  ( -15.36549428884569934, 1420.414141511310163, 227.0219848988409979 ) ) ;
#24947=CARTESIAN_POINT ( 'NONE',  ( -8.405094409318110138, 1406.273497697349967, 267.8245351791679809 ) ) ;
#24949=B_SPLINE_CURVE_WITH_KNOTS ( 'NONE', 3,
 ( #28710, #88081, #21917, #97566, #104863, #28151, #19746, #72383, #80767, #87523 ),
 .UNSPECIFIED., .F., .F.,
 ( 4, 2, 2, 2, 4 ),
 ( 0.000000000000000000, 0.2500000000000000000, 0.5000000000000000000, 0.7500000000000000000, 1.000000000000000000 ),
 .UNSPECIFIED. ) ;
#24950=CARTESIAN_POINT ( 'NONE',  ( -13.19292672295799917, 1435.822704715800000, 150.5785168366210200 ) ) ;
#24951=ORIENTED_EDGE ( 'NONE', *, *, #40680, .T. ) ;
#24953=CARTESIAN_POINT ( 'NONE',  ( 14.11724807090000056, 1444.027138891239929, 189.4625475421979957 ) ) ;
#24954=ORIENTED_EDGE ( 'NONE', *, *, #66624, .F. ) ;
#24955=ORIENTED_EDGE ( 'NONE', *, *, #86680, .T. ) ;
#24957=CARTESIAN_POINT ( 'NONE',  ( -22.01621720485236011, 1506.474306125368003, 209.2841005374792758 ) ) ;
#24961=EDGE_CURVE ( 'NONE', #51991, #48892, #20801, .T. ) ;
#24963=B_SPLINE_SURFACE_WITH_KNOTS ( 'NONE', 4, 5, ( 
 ( #72444, #98165, #56172, #71924, #64047, #21437 ),
 ( #62403, #106575, #2498, #96531, #80282, #106037 ),
 ( #19805, #62973, #45599, #54010, #97086, #29314 ),
 ( #88141, #90311, #11429, #20898, #89224, #79740 ),
 ( #70816, #81354, #98720, #13589, #55648, #3597 ) ),
 .UNSPECIFIED., .F., .F., .F.,
 ( 5, 5 ),
 ( 6, 6 ),
 ( 6.493025399899999606, 14.36013212639999992 ),
 ( -4.440892098500000003E-16, 2.000000000000000000 ),
 .UNSPECIFIED. ) ;
#24964=ORIENTED_EDGE ( 'NONE', *, *, #94018, .F. ) ;
#24967=CIRCLE ( 'NONE', #87602, 2.000212125018253406 ) ;
#24968=CARTESIAN_POINT ( 'NONE',  ( -28.40019560849999891, 1509.157491137930037, 208.4293195043489675 ) ) ;
#24969=B_SPLINE_SURFACE_WITH_KNOTS ( 'NONE', 5, 5, ( 
 ( #29456, #3197, #37324, #61444, #11570, #70961 ),
 ( #95568, #45747, #105076, #54148, #2088, #63652 ),
 ( #27818, #61998, #28365, #19955, #79884, #12110 ),
 ( #71520, #105640, #28925, #97216, #20488, #31115 ),
 ( #72585, #30567, #91016, #56332, #90464, #14305 ),
 ( #49046, #4805, #57455, #81503, #99964, #106713 ) ),
 .UNSPECIFIED., .F., .F., .F.,
 ( 6, 6 ),
 ( 6, 6 ),
 ( 6.267575576645930013, 7.848944788839999909 ),
 ( 0.000000000000000000, 1.444929468818969998 ),
 .UNSPECIFIED. ) ;
#24973=CARTESIAN_POINT ( 'NONE',  ( -2.605301666119999915, 1407.938395048229950, 196.0967308190980134 ) ) ;
#24976=CARTESIAN_POINT ( 'NONE',  ( 15.53981991842809585, 1506.512156833535528, 193.4804600942033801 ) ) ;
#24977=VERTEX_POINT ( 'NONE', #29458 ) ;
#24979=CARTESIAN_POINT ( 'NONE',  ( 27.25446695569999989, 1488.690170597129736, 210.3317447754679961 ) ) ;
#24983=B_SPLINE_CURVE_WITH_KNOTS ( 'NONE', 3,
 ( #106030, #46690, #29306, #29854, #12511, #90301 ),
 .UNSPECIFIED., .F., .F.,
 ( 4, 2, 4 ),
 ( 2.168404344971008868E-18, 0.003924659484584390456, 0.007849318969168777443 ),
 .UNSPECIFIED. ) ;
#24989=CARTESIAN_POINT ( 'NONE',  ( 18.80368967275888181, 1425.915424793447983, 225.1658295344082603 ) ) ;
#24992=ORIENTED_EDGE ( 'NONE', *, *, #10317, .F. ) ;
#24994=B_SPLINE_CURVE_WITH_KNOTS ( 'NONE', 5,
 ( #40086, #92144, #30020, #47400, #65860, #81522, #49061, #14870, #107840 ),
 .UNSPECIFIED., .F., .F.,
 ( 6, 3, 6 ),
 ( 0.000000000000000000, 0.4402423755028501695, 1.000000000000000000 ),
 .UNSPECIFIED. ) ;
#24996=CARTESIAN_POINT ( 'NONE',  ( -18.72407526530000155, 1458.246115540929850, 227.3156487912980026 ) ) ;
#24999=B_SPLINE_CURVE_WITH_KNOTS ( 'NONE', 3,
 ( #88792, #45155, #18802, #27227, #10981, #44590, #63082, #96645, #53554, #37839, #20455, #36183, #19354, #19914, #54664, #27775, #96079, #80395, #2606, #88243, #61407, #11536, #3159, #95530, #104482, #60857, #94982, #45711 ),
 .UNSPECIFIED., .F., .F.,
 ( 4, 2, 2, 1, 2, 2, 2, 1, 1, 1, 1, 1, 2, 2, 2, 2, 4 ),
 ( 0.000000000000000000, 0.2499999999999414912, 0.3749999999999151234, 0.4374999999999019118, 0.4687499999998977485, 0.4999999999998935296, 0.6249999999998722133, 0.6874999999998615552, 0.7187499999998566702, 0.7343749999998538946, 0.7421874999998498978, 0.7460937499998477884, 0.7480468749998462341, 0.7499999999998446798, 0.8749999999999199529, 0.9374999999999600320, 1.000000000000000000 ),
 .UNSPECIFIED. ) ;
#25000=CARTESIAN_POINT ( 'NONE',  ( 12.87808539635419969, 1435.336471212810011, 150.5288829532699992 ) ) ;
#25001=CARTESIAN_POINT ( 'NONE',  ( 12.94866893597960100, 1469.001480463319922, 231.3866629679569940 ) ) ;
#25003=CARTESIAN_POINT ( 'NONE',  ( 12.77587743780000018, 1416.568813547830132, 222.7009457741980327 ) ) ;
#25004=B_SPLINE_CURVE_WITH_KNOTS ( 'NONE', 3,
 ( #88757, #44549, #71446, #10376, #11500, #3672 ),
 .UNSPECIFIED., .F., .F.,
 ( 4, 2, 4 ),
 ( 0.000000000000000000, 0.5000000000000000000, 1.000000000000000000 ),
 .UNSPECIFIED. ) ;
#25007=CARTESIAN_POINT ( 'NONE',  ( 4.221851273025380102, 1441.601972411079942, 170.0739392326869961 ) ) ;
#25010=CARTESIAN_POINT ( 'NONE',  ( 41.66134420550000073, 1443.796851579070108, 135.6885409488979803 ) ) ;
#25011=CARTESIAN_POINT ( 'NONE',  ( 21.39772446809999806, 1509.704964749530063, 188.4542719777979869 ) ) ;
#25017=CARTESIAN_POINT ( 'NONE',  ( 0.6025240147529998813, 1420.628247535429864, 182.8370771391979872 ) ) ;
#25020=CARTESIAN_POINT ( 'NONE',  ( 9829.078716723830439, 2833.596074015639715, -1083.720023828199828 ) ) ;
#25024=CARTESIAN_POINT ( 'NONE',  ( 18.88752285780000051, 1416.568813549730066, 210.6689649478780098 ) ) ;
#25025=CARTESIAN_POINT ( 'NONE',  ( 18.03158832033268411, 1424.671894330125269, 224.6703068079623051 ) ) ;
#25026=DIRECTION ( 'NONE',  ( 3.828588921590000582E-16, 0.000000000000000000, 1.000000000000000000 ) ) ;
#25027=CARTESIAN_POINT ( 'NONE',  ( -4.989973902650000070, 1442.756953654919926, 150.3769280849980134 ) ) ;
#25028=CARTESIAN_POINT ( 'NONE',  ( 44.98655287106430478, 1440.913060372329937, 265.4537301890219965 ) ) ;
#25030=CARTESIAN_POINT ( 'NONE',  ( 11.41971426342585261, 1507.432269439749689, 184.3360310533326185 ) ) ;
#25034=CARTESIAN_POINT ( 'NONE',  ( 1.547519921729459957, 1416.512142023790148, 190.2622265145609788 ) ) ;
#25036=CARTESIAN_POINT ( 'NONE',  ( -27.72858371599999927, 1508.599279862329922, 210.5587065999479819 ) ) ;
#25038=CARTESIAN_POINT ( 'NONE',  ( 6.680091234600673111, 1440.117289966305634, 185.5007468843921004 ) ) ;
#25039=DIRECTION ( 'NONE',  ( -0.9958668876188416785, 0.000000000000000000, 0.09082478816029017354 ) ) ;
#25041=CARTESIAN_POINT ( 'NONE',  ( 12.98226561589999939, 1414.913060387329779, 198.3280246956980193 ) ) ;
#25043=CARTESIAN_POINT ( 'NONE',  ( -0.02753319299389999850, 1452.474300611429953, 153.7510437628980071 ) ) ;
#25047=EDGE_LOOP ( 'NONE', ( #24002, #24823, #102925 ) ) ;
#25048=CYLINDRICAL_SURFACE ( 'NONE', #77177, 1.999999999999912514 ) ;
#25054=CARTESIAN_POINT ( 'NONE',  ( 18.96841931012820126, 1508.814919057110046, 230.1294357287169987 ) ) ;
#25056=CARTESIAN_POINT ( 'NONE',  ( 40.27297052727078608, 1443.533075565821719, 137.1070167546214122 ) ) ;
#25057=CARTESIAN_POINT ( 'NONE',  ( -11.71103087170000023, 1438.058396846869982, 147.7520216503980066 ) ) ;
#25059=CIRCLE ( 'NONE', #69798, 2.000000000000001776 ) ;
#25065=CARTESIAN_POINT ( 'NONE',  ( 4.276093308640000146, 1410.438556067529817, 186.1213257426980192 ) ) ;
#25066=FACE_OUTER_BOUND ( 'NONE', #78960, .T. ) ;
#25068=CARTESIAN_POINT ( 'NONE',  ( 10.96966797059999799, 1432.360037085230033, 151.7701368415980028 ) ) ;
#25070=CARTESIAN_POINT ( 'NONE',  ( -23.39765034550000067, 1451.953609269630078, 140.1874901743979933 ) ) ;
#25071=CARTESIAN_POINT ( 'NONE',  ( 0.7760999072929999354, 1465.000431637629845, 237.6961790583980019 ) ) ;
#25074=CARTESIAN_POINT ( 'NONE',  ( 5.015673624609470416, 1509.218235651550003, 238.8061437059149910 ) ) ;
#25077=CARTESIAN_POINT ( 'NONE',  ( 14.48064082319999812, 1430.158253430729928, 190.5189584202980200 ) ) ;
#25078=CARTESIAN_POINT ( 'NONE',  ( -5.849681485717489748E-09, 1472.204232032089976, 259.4648360949830135 ) ) ;
#25081=CARTESIAN_POINT ( 'NONE',  ( -1.124394188919999982, 1416.535385209630022, 228.0704250668979682 ) ) ;
#25087=CARTESIAN_POINT ( 'NONE',  ( -45.77496015592539891, 1438.861072743580053, 268.7587536533030175 ) ) ;
#25088=CARTESIAN_POINT ( 'NONE',  ( 13.47402130151080080, 1508.487106454680088, 233.3457994875830082 ) ) ;
#25092=CARTESIAN_POINT ( 'NONE',  ( -5.451417714189999764, 1437.905383210109903, 154.7243314242980148 ) ) ;
#25093=B_SPLINE_SURFACE_WITH_KNOTS ( 'NONE', 5, 5, ( 
 ( #75316, #32738, #66918, #59064, #42249, #93187, #33836, #59608, #95275 ),
 ( #18537, #52732, #53291, #79588, #96375, #80119, #89067, #44334, #11817 ),
 ( #20202, #87429, #46542, #37569, #2893, #97473, #37011, #71204, #70110 ),
 ( #29709, #72292, #10159, #71770, #63894, #19654, #96934, #44897, #61697 ),
 ( #54400, #88533, #105886, #36460, #45987, #105325, #28618, #86867, #10725 ),
 ( #79046, #27510, #53858, #95819, #63356, #45446, #98009, #62821, #12352 ),
 ( #19087, #1789, #3438, #28060, #29167, #20743, #87995, #35927, #54938 ),
 ( #80677, #3989, #38114, #70659, #78476, #106425, #2348, #21280, #62250 ),
 ( #104775, #11282, #104223, #64445, #48741, #98562, #49286, #23508, #6158 ),
 ( #55488, #31912, #21830, #40313, #30808, #56029, #47626, #99102, #22380 ),
 ( #82866, #90154, #83415, #57700, #74496, #108624, #90713, #4525, #64986 ),
 ( #66101, #13436, #81208, #100228, #75041, #38659, #56580, #99651, #22942 ) ),
 .UNSPECIFIED., .F., .F., .F.,
 ( 6, 3, 3, 6 ),
 ( 6, 3, 6 ),
 ( 0.000000000000000000, 17.84603210599999912, 40.51038747020000130, 67.03953034199999195 ),
 ( 253.0908261149999987, 295.2726304679999885, 337.4544348200000172 ),
 .UNSPECIFIED. ) ;
#25096=CARTESIAN_POINT ( 'NONE',  ( -25.64740235160000026, 1451.776718248130010, 136.1276997542979927 ) ) ;
#25097=EDGE_LOOP ( 'NONE', ( #62548, #90127, #26359, #98115 ) ) ;
#25099=CARTESIAN_POINT ( 'NONE',  ( 16.11555329659999813, 1425.418868056930023, 217.2236249432280033 ) ) ;
#25102=CARTESIAN_POINT ( 'NONE',  ( -1.836122418284559910, 1419.498329967660084, 185.6833343230359787 ) ) ;
#25104=DIRECTION ( 'NONE',  ( 0.5450600352768949497, -0.8383970168982891602, 0.000000000000000000 ) ) ;
#25107=CARTESIAN_POINT ( 'NONE',  ( -17.74177080272650997, 1410.893628021574614, 194.9094938642074339 ) ) ;
#25110=CARTESIAN_POINT ( 'NONE',  ( -4.375893703611340335, 1407.803658742089965, 270.1335120727630397 ) ) ;
#25111=CARTESIAN_POINT ( 'NONE',  ( 8.985183074850001006, 1417.398376849329907, 230.5159961331980014 ) ) ;
#25112=CARTESIAN_POINT ( 'NONE',  ( -2.701663630316083697, 1448.935076026784827, 184.0154241898988232 ) ) ;
#25113=EDGE_LOOP ( 'NONE', ( #50777, #84559, #73723, #43139 ) ) ;
#25116=CARTESIAN_POINT ( 'NONE',  ( 0.01764073193947529941, 1409.855412122559983, 185.0387969038189908 ) ) ;
#25117=FACE_OUTER_BOUND ( 'NONE', #44094, .T. ) ;
#25119=CARTESIAN_POINT ( 'NONE',  ( -19.92563280199049913, 1472.425994622909911, 193.2981305741199947 ) ) ;
#25121=ORIENTED_EDGE ( 'NONE', *, *, #72708, .T. ) ;
#25122=CARTESIAN_POINT ( 'NONE',  ( 32.98914153328620102, 1465.411049489700190, 266.7912572958550186 ) ) ;
#25124=DIRECTION ( 'NONE',  ( -1.987898964669120000E-13, 0.000000000000000000, 1.000000000000000000 ) ) ;
#25126=EDGE_CURVE ( 'NONE', #32742, #77650, #14179, .T. ) ;
#25128=CARTESIAN_POINT ( 'NONE',  ( 18.46594417149771417, 1458.839898657651474, 227.6586181968465041 ) ) ;
#25130=VECTOR ( 'NONE', #71564, 1000.000000000000000 ) ;
#25131=CARTESIAN_POINT ( 'NONE',  ( -12.84239665067440050, 1435.935719077439899, 150.8114796122480072 ) ) ;
#25138=CARTESIAN_POINT ( 'NONE',  ( 22.70509004431190192, 1409.705939603270053, 209.2982552845940063 ) ) ;
#25140=CARTESIAN_POINT ( 'NONE',  ( 8.591778955288280173, 1409.213091919750013, 189.5189649568119989 ) ) ;
#25147=CARTESIAN_POINT ( 'NONE',  ( 12.33030208333319955, 1415.427621830080170, 221.6250288674360149 ) ) ;
#25155=CARTESIAN_POINT ( 'NONE',  ( 13.34862394727499968, 1427.267748017370195, 221.9543608694049794 ) ) ;
#25156=CARTESIAN_POINT ( 'NONE',  ( 1.176836406099999899E-14, 1468.063065667029832, 262.6648722463980334 ) ) ;
#25158=CARTESIAN_POINT ( 'NONE',  ( 11.15583049490000001, 1433.756731305959875, 151.6440224492980064 ) ) ;
#25159=CARTESIAN_POINT ( 'NONE',  ( 3.804422478559999821, 1458.952956299430070, 234.3916895697979612 ) ) ;
#25161=CIRCLE ( 'NONE', #41337, 12.50000000000001066 ) ;
#25164=CARTESIAN_POINT ( 'NONE',  ( 12.93261306534300026, 1416.826860677879949, 221.7400780573829877 ) ) ;
#25165=CIRCLE ( 'NONE', #23346, 29.84605316875909153 ) ;
#25166=CARTESIAN_POINT ( 'NONE',  ( -13.92276408390000064, 1412.700534325730132, 227.1776661936980020 ) ) ;
#25167=CARTESIAN_POINT ( 'NONE',  ( 0.05083158678110080014, 1508.992420415059996, 238.9842585609989953 ) ) ;
#25168=CARTESIAN_POINT ( 'NONE',  ( 23.61553526439999828, 1410.914738107329867, 211.4616251689280091 ) ) ;
#25170=CARTESIAN_POINT ( 'NONE',  ( 25.83285470672302253, 1436.659813480326420, 137.0377997444614380 ) ) ;
#25177=CARTESIAN_POINT ( 'NONE',  ( 0.1729020573706560038, 1478.627309218569962, 182.1533541099630042 ) ) ;
#25180=CARTESIAN_POINT ( 'NONE',  ( -17.11714625305222981, 1444.740067931810927, 162.7561045841209193 ) ) ;
#25183=CARTESIAN_POINT ( 'NONE',  ( 13.80510066409999936, 1434.979587830419860, 149.7893444102980141 ) ) ;
#25184=CARTESIAN_POINT ( 'NONE',  ( -40.27155789729510360, 1448.225093239489979, 134.0999999982899737 ) ) ;
#25186=EDGE_LOOP ( 'NONE', ( #53374, #107799, #104200, #31874 ) ) ;
#25189=CARTESIAN_POINT ( 'NONE',  ( -16.81460427359999699, 1415.425433635630043, 214.3135839119680099 ) ) ;
#25192=CARTESIAN_POINT ( 'NONE',  ( -0.8265242355799999885, 1408.941923249630008, 187.0792671738979891 ) ) ;
#25194=CARTESIAN_POINT ( 'NONE',  ( 8.196706623898419863, 1409.199295689860037, 221.6385046391639833 ) ) ;
#25200=CARTESIAN_POINT ( 'NONE',  ( -29.31937758650000347, 1451.433528204029926, 136.0808240385979957 ) ) ;
#25201=CARTESIAN_POINT ( 'NONE',  ( -15.80996491931430015, 1410.569114994490064, 226.6997803613269866 ) ) ;
#25203=EDGE_LOOP ( 'NONE', ( #4625, #14791, #59998, #52364, #22941 ) ) ;
#25210=CARTESIAN_POINT ( 'NONE',  ( 17.93831527589803443, 1434.889764120619475, 215.4602619631652942 ) ) ;
#25211=CARTESIAN_POINT ( 'NONE',  ( 1.362396098649999887, 1416.437840611730053, 232.9004600697980152 ) ) ;
#25214=CARTESIAN_POINT ( 'NONE',  ( 22.64728419264357129, 1509.725303465448860, 190.0246945496440105 ) ) ;
#25215=B_SPLINE_CURVE_WITH_KNOTS ( 'NONE', 5,
 ( #70509, #37428, #11135, #62103, #44181, #54253 ),
 .UNSPECIFIED., .F., .F.,
 ( 6, 6 ),
 ( 0.000000000000000000, 1.000000000000000000 ),
 .UNSPECIFIED. ) ;
#25218=CARTESIAN_POINT ( 'NONE',  ( 2.500000000000000000, 1448.555989962169861, 159.6014785455980132 ) ) ;
#25219=CARTESIAN_POINT ( 'NONE',  ( -2.500000000000000000, 1439.114301494319989, 157.7261950941980331 ) ) ;
#25222=ORIENTED_EDGE ( 'NONE', *, *, #89125, .F. ) ;
#25223=CARTESIAN_POINT ( 'NONE',  ( 40.76710640913900363, 1444.185691436559864, 136.9913394050109900 ) ) ;
#25227=CARTESIAN_POINT ( 'NONE',  ( -23.70212955649999742, 1410.915617643129963, 207.1033590604579899 ) ) ;
#25228=CARTESIAN_POINT ( 'NONE',  ( -10.52497800899770120, 1425.367411924009957, 103.8987780947440029 ) ) ;
#25229=CARTESIAN_POINT ( 'NONE',  ( 17.33016647839879809, 1410.462159060319891, 192.5037184876999845 ) ) ;
#25232=CARTESIAN_POINT ( 'NONE',  ( 18.39508751440705225, 1509.674679010870705, 185.4233143434903468 ) ) ;
#25233=CARTESIAN_POINT ( 'NONE',  ( -18.96350828799999988, 1416.837080254430020, 208.0006277515079773 ) ) ;
#25234=CARTESIAN_POINT ( 'NONE',  ( -44.59182306800000362, 1432.587450657589898, 266.2372469040980150 ) ) ;
#25237=EDGE_CURVE ( 'NONE', #7508, #10122, #87589, .T. ) ;
#25241=CARTESIAN_POINT ( 'NONE',  ( 9.933598901150000771, 1396.438403817630160, 201.0717090587579889 ) ) ;
#25245=VERTEX_POINT ( 'NONE', #9238 ) ;
#25246=CARTESIAN_POINT ( 'NONE',  ( -29.53763760329688637, 1509.959418432381881, 210.9330277046395565 ) ) ;
#25255=CARTESIAN_POINT ( 'NONE',  ( 25.18950438009999715, 1436.599308748099929, 137.5297815331979905 ) ) ;
#25258=EDGE_LOOP ( 'NONE', ( #85123, #108442, #40089, #9747 ) ) ;
#25261=ORIENTED_EDGE ( 'NONE', *, *, #62416, .T. ) ;
#25262=CARTESIAN_POINT ( 'NONE',  ( 11.78205866055090034, 1427.489864168300073, 147.1792652955979861 ) ) ;
#25265=ORIENTED_EDGE ( 'NONE', *, *, #18672, .T. ) ;
#25266=CARTESIAN_POINT ( 'NONE',  ( -13.31050682230000071, 1414.983773854429955, 220.3937082794980142 ) ) ;
#25267=CARTESIAN_POINT ( 'NONE',  ( -11.74913059853910013, 1432.337153556749854, 150.6947011568290122 ) ) ;
#25268=CARTESIAN_POINT ( 'NONE',  ( -1.590050350630178855, 1426.843352158476364, 137.0999999982234385 ) ) ;
#25269=CIRCLE ( 'NONE', #94995, 1.500000000000001332 ) ;
#25271=CARTESIAN_POINT ( 'NONE',  ( -4.519015011720000530, 1423.889711422029904, 184.9853378348980186 ) ) ;
#25274=CARTESIAN_POINT ( 'NONE',  ( -5.482624842517240360, 1410.482164323645065, 187.0654721365125397 ) ) ;
#25276=CARTESIAN_POINT ( 'NONE',  ( -16.48551040579999949, 1496.366555713729895, 224.3141742696979861 ) ) ;
#25277=CARTESIAN_POINT ( 'NONE',  ( 17.87794079920000101, 1458.605263598229840, 228.2755591389980054 ) ) ;
#25278=DIRECTION ( 'NONE',  ( 0.000000000000000000, 0.000000000000000000, 1.000000000000000000 ) ) ;
#25279=CARTESIAN_POINT ( 'NONE',  ( -4.904257884871542572, 1423.393875679067833, 184.6729318142273826 ) ) ;
#25280=CARTESIAN_POINT ( 'NONE',  ( -2.499954588792669963, 1419.918889429339970, 111.3715765239870024 ) ) ;
#25281=ORIENTED_EDGE ( 'NONE', *, *, #68688, .T. ) ;
#25282=VECTOR ( 'NONE', #90481, 1000.000000000000000 ) ;
#25285=CARTESIAN_POINT ( 'NONE',  ( -2.898871272187721004, 1484.376110530463620, 183.3081109901478669 ) ) ;
#25289=CARTESIAN_POINT ( 'NONE',  ( 1.525925909070000142, 1471.311257370530029, 187.8077771315979874 ) ) ;
#25290=CARTESIAN_POINT ( 'NONE',  ( -11.80475977109999874, 1428.187072569730162, 148.7521081752979910 ) ) ;
#25291=CARTESIAN_POINT ( 'NONE',  ( -10.94851406893937096, 1430.816032392971692, 151.6584449855879768 ) ) ;
#25293=CARTESIAN_POINT ( 'NONE',  ( -5.343479917770609156, 1396.099658817820000, 199.4684377796870081 ) ) ;
#25295=CARTESIAN_POINT ( 'NONE',  ( -2.451271202390000070, 1433.447543843880112, 150.3250444719979839 ) ) ;
#25296=CARTESIAN_POINT ( 'NONE',  ( -25.31266740589999742, 1495.362868818529932, 217.3509689723979932 ) ) ;
#25298=CARTESIAN_POINT ( 'NONE',  ( -16.13327988281299952, 1459.077551211970103, 230.3615990537609832 ) ) ;
#25299=VERTEX_POINT ( 'NONE', #93756 ) ;
#25301=CARTESIAN_POINT ( 'NONE',  ( 35.80076753759999519, 1418.783835402329942, 268.8110194917979925 ) ) ;
#25302=DIRECTION ( 'NONE',  ( 0.000000000000000000, 0.000000000000000000, -1.000000000000000000 ) ) ;
#25304=CARTESIAN_POINT ( 'NONE',  ( 20.53761168180000141, 1449.728047012690013, 194.5965259811979990 ) ) ;
#25306=CARTESIAN_POINT ( 'NONE',  ( 0.06657943191975031205, 1508.845581504609981, 238.3754151068810074 ) ) ;
#25310=PLANE ( 'NONE',  #60392 ) ;
#25312=CARTESIAN_POINT ( 'NONE',  ( -13.40404449519999908, 1444.440855884700113, 187.1602913364980054 ) ) ;
#25314=CARTESIAN_POINT ( 'NONE',  ( -19.60393592299999810, 1475.513060387329915, 216.8351853114679955 ) ) ;
#25318=VERTEX_POINT ( 'NONE', #1389 ) ;
#25320=CARTESIAN_POINT ( 'NONE',  ( -14.39277900435820001, 1409.415667305270063, 205.1427022228000112 ) ) ;
#25324=CARTESIAN_POINT ( 'NONE',  ( -14.40881992470000128, 1473.360613499030023, 269.5837026295979513 ) ) ;
#25327=CARTESIAN_POINT ( 'NONE',  ( -24.09045629887435069, 1444.422250552413971, 211.8863943959888161 ) ) ;
#25330=CARTESIAN_POINT ( 'NONE',  ( 12.20493293904160126, 1416.321686232750153, 223.5163099168240137 ) ) ;
#25334=CARTESIAN_POINT ( 'NONE',  ( -22.77843419010000048, 1410.203593476030164, 204.7359747443179856 ) ) ;
#25339=CARTESIAN_POINT ( 'NONE',  ( 16.66094735743510213, 1410.867388111209948, 226.5061907891179942 ) ) ;
#25344=DIRECTION ( 'NONE',  ( 0.01393861230742109505, 0.01013783823313249566, -0.9998514586291816775 ) ) ;
#25345=CARTESIAN_POINT ( 'NONE',  ( -22.51991132370000059, 1410.619212249830071, 212.0399852714280087 ) ) ;
#25347=CARTESIAN_POINT ( 'NONE',  ( 11.71642830186019957, 1426.709184726649937, 142.6946108399700108 ) ) ;
#25352=CARTESIAN_POINT ( 'NONE',  ( -10.98592888573429960, 1414.913372219064740, 196.0727560459370693 ) ) ;
#25354=CARTESIAN_POINT ( 'NONE',  ( -12.26707230937048365, 1398.276752517840350, 213.6251289080058484 ) ) ;
#25357=CARTESIAN_POINT ( 'NONE',  ( 1.401686974080000203, 1507.677644781729896, 236.8428152670980182 ) ) ;
#25358=CIRCLE ( 'NONE', #5736, 32.72294243206279418 ) ;
#25359=CARTESIAN_POINT ( 'NONE',  ( 20.59997055523719922, 1508.349664204210058, 227.9987446602079899 ) ) ;
#25363=CARTESIAN_POINT ( 'NONE',  ( 12.02659948205739937, 1433.794953934120031, 150.1257855643209780 ) ) ;
#25364=CARTESIAN_POINT ( 'NONE',  ( 0.04898382733899999536, 1396.985963199630305, 221.9366346537979950 ) ) ;
#25367=CARTESIAN_POINT ( 'NONE',  ( -22.59253512340000114, 1509.026248158530052, 193.6920252460979839 ) ) ;
#25370=CARTESIAN_POINT ( 'NONE',  ( -13.94340296021099945, 1508.954224554140183, 183.7492702217640215 ) ) ;
#25371=CARTESIAN_POINT ( 'NONE',  ( 19.14360834932719868, 1488.414938085379845, 228.7258892975569893 ) ) ;
#25373=CARTESIAN_POINT ( 'NONE',  ( 11.10982621349999988, 1449.228537578660053, 187.2287387423980078 ) ) ;
#25375=CARTESIAN_POINT ( 'NONE',  ( -24.19014952379989936, 1444.790439640009936, 211.5093900478289868 ) ) ;
#25378=CARTESIAN_POINT ( 'NONE',  ( 37.46849106787850303, 1436.652236075190103, 134.0999999968449856 ) ) ;
#25379=CARTESIAN_POINT ( 'NONE',  ( 11.85834799300000064, 1431.766924987119864, 150.3709389535979994 ) ) ;
#25382=CARTESIAN_POINT ( 'NONE',  ( 13.49389551315819880, 1436.020594185369873, 150.4744559408089799 ) ) ;
#25384=ORIENTED_EDGE ( 'NONE', *, *, #39751, .F. ) ;
#25386=CARTESIAN_POINT ( 'NONE',  ( -4.082666824149999485, 1466.262580571829858, 234.7294175710979971 ) ) ;
#25387=CARTESIAN_POINT ( 'NONE',  ( -12.34781077223220080, 1407.409374063429823, 203.9011771819639876 ) ) ;
#25391=CARTESIAN_POINT ( 'NONE',  ( -19.07790034667103285, 1442.172555339580185, 210.4727050325287223 ) ) ;
#25394=ORIENTED_EDGE ( 'NONE', *, *, #61267, .F. ) ;
#25397=CARTESIAN_POINT ( 'NONE',  ( 22.08278260508789970, 1440.913060387330006, 227.7515003150190012 ) ) ;
#25398=CARTESIAN_POINT ( 'NONE',  ( -19.28393528680000202, 1507.737928445829994, 229.5896611176980002 ) ) ;
#25399=CARTESIAN_POINT ( 'NONE',  ( -7.248290715579999599, 1409.670137264329924, 187.6984399624980142 ) ) ;
#25401=CARTESIAN_POINT ( 'NONE',  ( 0.3610913073109310312, 1416.520646088589956, 227.1639887257210262 ) ) ;
#25403=CARTESIAN_POINT ( 'NONE',  ( 24.43361483890000230, 1438.270030349950048, 213.2447553941780143 ) ) ;
#25405=DIRECTION ( 'NONE',  ( 0.5161917810414575758, -0.8564730265368828421, 0.000000000000000000 ) ) ;
#25406=ADVANCED_FACE ( 'NONE', ( #8113 ), #103261, .T. ) ;
#25411=CARTESIAN_POINT ( 'NONE',  ( 23.28443123535648240, 1409.830905082309982, 209.4348622450964115 ) ) ;
#25415=CARTESIAN_POINT ( 'NONE',  ( 13.82592919020000011, 1409.562390515329980, 191.7841888639979970 ) ) ;
#25422=CARTESIAN_POINT ( 'NONE',  ( 10.82132307070000010, 1467.865346125029873, 250.5360043798979746 ) ) ;
#25423=CARTESIAN_POINT ( 'NONE',  ( 2.838593810556235386, 1451.798153998362523, 183.8400884881581874 ) ) ;
#25424=CARTESIAN_POINT ( 'NONE',  ( -26.72684354202990065, 1509.846382329900280, 221.2472112117080201 ) ) ;
#25425=CARTESIAN_POINT ( 'NONE',  ( -5.276082853953459662, 1507.211509375310015, 236.2464089988909848 ) ) ;
#25426=CARTESIAN_POINT ( 'NONE',  ( -23.30326309200000168, 1448.852050024469918, 216.7100016161180065 ) ) ;
#25427=CARTESIAN_POINT ( 'NONE',  ( 2.798741256952680168, 1509.010794585639815, 238.1786444310339732 ) ) ;
#25428=CARTESIAN_POINT ( 'NONE',  ( 20.64978683589999875, 1464.413060387330006, 209.6104161236400216 ) ) ;
#25429=CARTESIAN_POINT ( 'NONE',  ( 17.67624996012689920, 1409.941488227490026, 222.7221753460849811 ) ) ;
#25432=ORIENTED_EDGE ( 'NONE', *, *, #8893, .F. ) ;
#25437=CARTESIAN_POINT ( 'NONE',  ( 28.23788172209999559, 1509.669894706129980, 207.1691932934379849 ) ) ;
#25439=CARTESIAN_POINT ( 'NONE',  ( 24.59648532329999782, 1442.354039869650023, 212.9848133149079956 ) ) ;
#25440=CARTESIAN_POINT ( 'NONE',  ( 38.12974907732069596, 1444.894042496080147, 137.0546131932600247 ) ) ;
#25445=CARTESIAN_POINT ( 'NONE',  ( 27.33350507148860231, 1435.453172591590146, 135.7066127169290155 ) ) ;
#25447=CARTESIAN_POINT ( 'NONE',  ( 3.644234494419170032E-15, 1459.964720571249927, 238.3189299478169971 ) ) ;
#25449=CARTESIAN_POINT ( 'NONE',  ( -16.63719475160000272, 1415.804827907129948, 226.7776979096980199 ) ) ;
#25453=ORIENTED_EDGE ( 'NONE', *, *, #86405, .T. ) ;
#25454=CARTESIAN_POINT ( 'NONE',  ( -25.18033061374759995, 1457.455288673970017, 210.8733860127310038 ) ) ;
#25458=CARTESIAN_POINT ( 'NONE',  ( 16.61028814131559983, 1497.249999798759973, 188.4200016273640017 ) ) ;
#25459=CARTESIAN_POINT ( 'NONE',  ( -0.4792323294310000259, 1416.456882655430036, 233.6761913835979954 ) ) ;
#25462=CARTESIAN_POINT ( 'NONE',  ( -28.27265633500000064, 1508.146186371529893, 208.9956447143910054 ) ) ;
#25466=DIRECTION ( 'NONE',  ( -0.006760929966149412801, 0.9987475664841024559, -0.04957406850437492268 ) ) ;
#25467=CARTESIAN_POINT ( 'NONE',  ( -12.39869315161027785, 1451.240234666110155, 151.2148383238678946 ) ) ;
#25468=CARTESIAN_POINT ( 'NONE',  ( -16.98743823132990016, 1415.088136167450102, 209.0991636084750098 ) ) ;
#25469=CARTESIAN_POINT ( 'NONE',  ( 25.73103649876719956, 1435.396100992830043, 135.5026723454229796 ) ) ;
#25470=LINE ( 'NONE', #78661, #45794 ) ;
#25471=EDGE_LOOP ( 'NONE', ( #31271, #54757, #21065, #59977 ) ) ;
#25472=B_SPLINE_CURVE_WITH_KNOTS ( 'NONE', 3,
 ( #98553, #89605, #11809, #71762, #54391, #107510, #98000, #21822, #105878, #80668, #30800, #80111, #3430, #56021, #90145, #5050, #4517 ),
 .UNSPECIFIED., .F., .F.,
 ( 4, 2, 2, 2, 2, 1, 2, 2, 4 ),
 ( 0.000000000000000000, 0.2499999999999752420, 0.3749999999999543698, 0.4999999999999334976, 0.6249999999999126254, 0.6874999999999087397, 0.7187499999999126254, 0.7499999999999165112, 1.000000000000000000 ),
 .UNSPECIFIED. ) ;
#25479=EDGE_CURVE ( 'NONE', #80100, #61056, #110378, .T. ) ;
#25480=CARTESIAN_POINT ( 'NONE',  ( 10.42064607629999884, 1425.390417346130107, 97.30158504869778824 ) ) ;
#25481=CARTESIAN_POINT ( 'NONE',  ( -24.41186846940000166, 1442.526119375989992, 212.0284777859579890 ) ) ;
#25484=CARTESIAN_POINT ( 'NONE',  ( -11.86957566529999930, 1433.007102185709755, 150.1775624469979675 ) ) ;
#25486=CARTESIAN_POINT ( 'NONE',  ( -2.561666046165639532, 1420.747219518938664, 185.5912888495579125 ) ) ;
#25488=CARTESIAN_POINT ( 'NONE',  ( -24.14541275720000257, 1438.310581897909969, 211.7943488613079808 ) ) ;
#25490=CARTESIAN_POINT ( 'NONE',  ( 2.612625988760000073, 1449.170853583729922, 183.0936082360980208 ) ) ;
#25493=CARTESIAN_POINT ( 'NONE',  ( -26.93976879576212013, 1509.966348417776089, 195.8375140788211866 ) ) ;
#25496=ORIENTED_EDGE ( 'NONE', *, *, #921, .T. ) ;
#25497=CARTESIAN_POINT ( 'NONE',  ( -11.74917500098110068, 1426.744637973110230, 145.0199627760420071 ) ) ;
#25499=CARTESIAN_POINT ( 'NONE',  ( -3.113156797959999889, 1472.539629439029795, 270.3710789736979905 ) ) ;
#25500=CARTESIAN_POINT ( 'NONE',  ( 12.67183603418154370, 1434.580315194757077, 147.1853303393423573 ) ) ;
#25501=( BOUNDED_CURVE ( )  B_SPLINE_CURVE ( 3, ( #110489, #61772, #43300, #102609 ),
 .UNSPECIFIED., .F., .F. ) 
 B_SPLINE_CURVE_WITH_KNOTS ( ( 4, 4 ),
 ( 1.268017778269938001, 1.928411133669210020 ),
 .UNSPECIFIED. ) 
 CURVE ( )  GEOMETRIC_REPRESENTATION_ITEM ( )  RATIONAL_B_SPLINE_CURVE ( ( 1.000000000000000000, 0.9639857287959530119, 0.9639857287959530119, 1.000000000000000000 ) ) 
 REPRESENTATION_ITEM ( '' )  );
#25503=CARTESIAN_POINT ( 'NONE',  ( 21.50121674829999918, 1519.913060387329779, 200.6355468375280111 ) ) ;
#25504=CARTESIAN_POINT ( 'NONE',  ( 14.55374896642978300, 1435.825240606026000, 149.7846887453127920 ) ) ;
#25505=CARTESIAN_POINT ( 'NONE',  ( -20.26030320659999617, 1497.713060387329961, 200.3164169727579917 ) ) ;
#25508=CARTESIAN_POINT ( 'NONE',  ( -15.35891919189770150, 1408.417119347609969, 269.4168528522860129 ) ) ;
#25509=CARTESIAN_POINT ( 'NONE',  ( -14.05872192255859865, 1435.084336612359948, 149.0797200086629744 ) ) ;
#25511=CARTESIAN_POINT ( 'NONE',  ( 13.98344342490000081, 1443.270835250810023, 189.4072587568979884 ) ) ;
#25514=CARTESIAN_POINT ( 'NONE',  ( -22.03054413770898279, 1506.491018781362527, 209.2384929680489449 ) ) ;
#25517=CARTESIAN_POINT ( 'NONE',  ( -10.31210393940000003, 1470.461415509729932, 185.6553077399979941 ) ) ;
#25519=B_SPLINE_CURVE_WITH_KNOTS ( 'NONE', 3,
 ( #69110, #7517, #61278, #110529, #9183, #85312, #68552, #102118, #67452, #101551, #24844, #33813, #9723, #18112, #103211, #26517, #252, #52308, #95394, #50091, #59046, #84764, #68007, #25397, #59589, #8607, #25952, #60147, #86432, #17544, #51746, #43888, #1340, #35479, #62945, #97056, #70783, #62371, #64019, #4106, #45016, #44450, #2469, #3017, #95943, #79162, #36586, #29285, #96497, #18658, #19776, #89192, #80800, #54526, #1910, #11937, #38230, #10844, #28185, #20320, #28740, #53978, #61820, #20870, #88111, #46667, #55065, #63481, #88660, #97599, #72414, #19203, #11400, #45569, #37689, #104896, #80248, #12485, #79710, #46117, #53405, #52856, #106544, #29833, #3566, #86984, #10273, #37140, #71893, #71337, #105451, #106009, #36048, #78594, #70235, #104341, #27634, #87556, #48866, #23064, #90835, #47745, #99775, #5747, #82450, #98131, #21949, #90278, #56142, #38778, #107647, #72954, #74609, #56699, #75162, #74057, #100343, #48309, #57814, #108744, #32035, #89740, #14118, #82992, #108186, #30379, #13559, #107091, #57274, #91938, #39890, #21406, #64569, #14679, #91401, #31477, #6284, #40432, #23632, #66224, #65658, #15212 ),
 .UNSPECIFIED., .F., .F.,
 ( 4, 3, 3, 3, 3, 3, 3, 3, 3, 3, 3, 3, 3, 3, 3, 3, 3, 3, 3, 3, 3, 3, 3, 3, 3, 3, 3, 3, 3, 3, 3, 3, 3, 3, 3, 3, 3, 3, 3, 3, 3, 3, 3, 3, 3, 3, 3, 4 ),
 ( -30.13994748849999894, -27.96748203595269899, -25.55492730130620060, -23.23438917604190124, -21.17793478234460025, -19.26470382119120117, -17.45260263486330032, -15.71699118168050013, -14.04216480072339834, -12.41738884950610000, -10.85332760853319911, -9.318777413941120358, -7.823271649228651370, -6.990622299191308286, -5.769753512368222204, -4.532961737479141107, -3.269848154182920297, -1.988543521522920798, -0.6878283704175984781, 0.6335739646309974660, 1.976953695996598981, 3.343532765747298185, 4.734321904188007579, 6.162678800765782228, 7.613445470389912373, 9.084622672767892482, 10.57254921413640147, 12.07472987505940409, 13.57779603196559748, 15.07203997055130174, 15.67373306504680386, 16.67002730872509630, 17.62945801330110385, 18.59514990580159832, 19.56632240333010486, 20.54202186413169784, 21.52113328980640006, 22.50240755822210303, 23.48450375772200260, 24.50074590849419565, 25.47886455692250252, 26.45346006570139963, 27.42358464403170615, 28.38842521988249956, 29.34425801996059846, 30.29438266051279527, 31.23569288928990062, 31.61444096390000880 ),
 .UNSPECIFIED. ) ;
#25520=B_SPLINE_CURVE_WITH_KNOTS ( 'NONE', 3,
 ( #109292, #84616, #100856, #32577, #75690, #66753, #7910, #42081, #76231, #67848, #84070, #102510, #25246, #24145, #58335, #59449, #92460, #68959, #9562, #61120, #87955, #9017, #61657, #43733, #78438, #104185, #77885, #643, #10123, #105287, #17948 ),
 .UNSPECIFIED., .F., .F.,
 ( 4, 2, 2, 2, 2, 2, 2, 2, 2, 2, 2, 2, 1, 2, 2, 4 ),
 ( 0.000000000000000000, 0.2499999999999730216, 0.3749999999999462652, 0.4999999999999195088, 0.6249999999998928635, 0.6874999999998921973, 0.7499999999998915312, 0.8124999999998908651, 0.8749999999998903100, 0.9374999999998896438, 0.9687499999998898659, 0.9843749999998919753, 0.9882812499999029665, 0.9902343749999205080, 0.9921874999999381606, 1.000000000000000000 ),
 .UNSPECIFIED. ) ;
#25521=CARTESIAN_POINT ( 'NONE',  ( -16.05668068212990107, 1479.766884033080032, 229.2771335141849818 ) ) ;
#25525=ADVANCED_FACE ( 'NONE', ( #106856 ), #26052, .F. ) ;
#25527=CARTESIAN_POINT ( 'NONE',  ( -28.65017519560000281, 1509.591492519529993, 207.6322003284180084 ) ) ;
#25530=CARTESIAN_POINT ( 'NONE',  ( -4.398770489489999491, 1409.066668837629777, 194.6843272123980171 ) ) ;
#25533=EDGE_LOOP ( 'NONE', ( #21164, #78724, #11922, #99357 ) ) ;
#25534=CARTESIAN_POINT ( 'NONE',  ( -25.68353141812590223, 1449.916372628639920, 209.9058930103780085 ) ) ;
#25535=CARTESIAN_POINT ( 'NONE',  ( 27.39000294680000280, 1488.691910935229998, 209.5725694969789856 ) ) ;
#25537=CARTESIAN_POINT ( 'NONE',  ( 19.44143630828250124, 1456.941519871360015, 224.4536055326989867 ) ) ;
#25538=EDGE_CURVE ( 'NONE', #88339, #32688, #29682, .T. ) ;
#25546=CARTESIAN_POINT ( 'NONE',  ( -2.199032837542779895, 1451.950542369889945, 184.5219133347679872 ) ) ;
#25547=CARTESIAN_POINT ( 'NONE',  ( -13.95687920409999982, 1412.831204937729808, 227.1595039112980317 ) ) ;
#25548=CARTESIAN_POINT ( 'NONE',  ( -20.03142830927689388, 1456.423548895029626, 225.1316417485375325 ) ) ;
#25549=VERTEX_POINT ( 'NONE', #41328 ) ;
#25553=CARTESIAN_POINT ( 'NONE',  ( 12.32474167489190009, 1434.386220826949966, 150.2103707558300130 ) ) ;
#25554=CARTESIAN_POINT ( 'NONE',  ( -4.085282425029218345, 1440.421590206651899, 185.3116467681438451 ) ) ;
#25559=FACE_OUTER_BOUND ( 'NONE', #73648, .T. ) ;
#25563=CARTESIAN_POINT ( 'NONE',  ( 20.35503613270000045, 1509.384884480429946, 188.3699781667980062 ) ) ;
#25566=CARTESIAN_POINT ( 'NONE',  ( -12.22219588455560135, 1415.434635989099888, 195.9645815201980099 ) ) ;
#25567=CARTESIAN_POINT ( 'NONE',  ( 15.78266869743918654, 1409.464195827833919, 192.9576493168518709 ) ) ;
#25573=CARTESIAN_POINT ( 'NONE',  ( 8576.261851438324811, 2833.596074015641989, -10892.29874055200526 ) ) ;
#25576=CARTESIAN_POINT ( 'NONE',  ( 17.74965683759114299, 1423.452220005456184, 226.1321863275825876 ) ) ;
#25577=CARTESIAN_POINT ( 'NONE',  ( 13.37406854550570046, 1507.496451373729997, 233.0472692220099873 ) ) ;
#25580=CARTESIAN_POINT ( 'NONE',  ( -7.346057189749999772, 1434.541746329560056, 149.5958201245979922 ) ) ;
#25581=CARTESIAN_POINT ( 'NONE',  ( 45.67177343720949523, 1440.913060382069943, 266.1885934449759930 ) ) ;
#25583=CARTESIAN_POINT ( 'NONE',  ( -18.89959486414000267, 1416.839692127460012, 207.5749783441650038 ) ) ;
#25585=ORIENTED_EDGE ( 'NONE', *, *, #17290, .T. ) ;
#25586=EDGE_CURVE ( 'NONE', #70446, #92411, #19536, .T. ) ;
#25587=ORIENTED_EDGE ( 'NONE', *, *, #22808, .T. ) ;
#25591=CARTESIAN_POINT ( 'NONE',  ( -24.41227777330000137, 1441.083062867809986, 212.0377087122379862 ) ) ;
#25592=CARTESIAN_POINT ( 'NONE',  ( 4.154679781990096465, 1410.434442818600701, 186.0820931863378860 ) ) ;
#25594=CARTESIAN_POINT ( 'NONE',  ( -7.789308819770000447, 1507.432058219530063, 181.7020214070979875 ) ) ;
#25595=EDGE_CURVE ( 'NONE', #36972, #88847, #26070, .T. ) ;
#25599=CARTESIAN_POINT ( 'NONE',  ( 3.639705460830000128, 1451.958765405729991, 154.0211597684979949 ) ) ;
#25603=VERTEX_POINT ( 'NONE', #104539 ) ;
#25606=CARTESIAN_POINT ( 'NONE',  ( 19.79774116257700101, 1508.248996258070065, 229.3423194934649700 ) ) ;
#25607=ORIENTED_EDGE ( 'NONE', *, *, #48788, .T. ) ;
#25611=CARTESIAN_POINT ( 'NONE',  ( 38.69602499724199873, 1439.330795836810012, 136.6667434724849954 ) ) ;
#25612=FACE_OUTER_BOUND ( 'NONE', #21431, .T. ) ;
#25613=FACE_OUTER_BOUND ( 'NONE', #53941, .T. ) ;
#25614=EDGE_CURVE ( 'NONE', #59443, #63161, #12892, .T. ) ;
#25618=CARTESIAN_POINT ( 'NONE',  ( -0.3166280365204529046, 1452.331784132522216, 183.2228567542290989 ) ) ;
#25619=CARTESIAN_POINT ( 'NONE',  ( -20.15452302159999931, 1507.845791376729949, 228.9024215066979764 ) ) ;
#25620=CARTESIAN_POINT ( 'NONE',  ( 1.834053397919999995, 1410.355893698830187, 185.3938420458979977 ) ) ;
#25625=CARTESIAN_POINT ( 'NONE',  ( -2.500000000000000000, 1439.072262259579929, 157.1874756602519767 ) ) ;
#25626=CARTESIAN_POINT ( 'NONE',  ( 11.79165749935659946, 1429.416858706420044, 146.4064136026630081 ) ) ;
#25627=CARTESIAN_POINT ( 'NONE',  ( 0.4604323351460000158, 1465.011193676930134, 237.3689745248979932 ) ) ;
#25630=CARTESIAN_POINT ( 'NONE',  ( -43.99260286630000394, 1444.142798274959887, 270.2177640581980427 ) ) ;
#25632=CARTESIAN_POINT ( 'NONE',  ( 22.19805589962659553, 1506.691119430664912, 209.3127852580865067 ) ) ;
#25633=CARTESIAN_POINT ( 'NONE',  ( 16.93884302589999891, 1507.634939823729837, 188.0954313829980151 ) ) ;
#25634=CARTESIAN_POINT ( 'NONE',  ( -1.081760175521900104E-08, 1473.331368512430117, 261.9578586066839421 ) ) ;
#25636=CARTESIAN_POINT ( 'NONE',  ( -1.433831019619999925, 1415.263254653229978, 227.1906885494979917 ) ) ;
#25637=CARTESIAN_POINT ( 'NONE',  ( -8.185464237450000624, 1418.160221195129907, 231.1370887997979935 ) ) ;
#25640=( BOUNDED_CURVE ( )  B_SPLINE_CURVE ( 3, ( #97690, #63039, #3666, #54619 ),
 .UNSPECIFIED., .F., .F. ) 
 B_SPLINE_CURVE_WITH_KNOTS ( ( 4, 4 ),
 ( 1.268017769446416088, 1.928411124454499914 ),
 .UNSPECIFIED. ) 
 CURVE ( )  GEOMETRIC_REPRESENTATION_ITEM ( )  RATIONAL_B_SPLINE_CURVE ( ( 1.000000000000000000, 0.9639857288382313039, 0.9639857288382313039, 1.000000000000000000 ) ) 
 REPRESENTATION_ITEM ( '' )  );
#25641=CARTESIAN_POINT ( 'NONE',  ( -0.6429601867158417638, 1485.414621978292644, 181.9392741304039305 ) ) ;
#25643=CARTESIAN_POINT ( 'NONE',  ( -46.03855999566639667, 1438.451647596259818, 268.2082775289269989 ) ) ;
#25649=CARTESIAN_POINT ( 'NONE',  ( -2.478941618209999920, 1432.378565395950091, 157.5169325447980100 ) ) ;
#25652=CARTESIAN_POINT ( 'NONE',  ( -26.68850062112660027, 1451.728563988709993, 135.8012203878940056 ) ) ;
#25653=ORIENTED_EDGE ( 'NONE', *, *, #30579, .T. ) ;
#25654=CARTESIAN_POINT ( 'NONE',  ( 23.18116579810000033, 1432.896189078000134, 217.2884692092180217 ) ) ;
#25657=CARTESIAN_POINT ( 'NONE',  ( 11.60004869885203682, 1425.894332500278097, 137.5113157688821275 ) ) ;
#25663=CARTESIAN_POINT ( 'NONE',  ( -4.950908079962929698, 1408.434846368340004, 270.3888801776009814 ) ) ;
#25664=CARTESIAN_POINT ( 'NONE',  ( 4.685675373058309390, 1417.752609642629977, 232.3318985854729988 ) ) ;
#25665=CARTESIAN_POINT ( 'NONE',  ( -0.4228489488307095034, 1508.822448670140602, 238.3614536558768577 ) ) ;
#25666=CARTESIAN_POINT ( 'NONE',  ( -2.500000000000000000, 1439.481493142219961, 163.2933147462130137 ) ) ;
#25667=VERTEX_POINT ( 'NONE', #21059 ) ;
#25669=CARTESIAN_POINT ( 'NONE',  ( -23.81374637684410089, 1410.984159143959914, 210.1595746859130145 ) ) ;
#25670=CARTESIAN_POINT ( 'NONE',  ( -0.0001149583598519999974, 1408.913064401730026, 186.4639625088979926 ) ) ;
#25672=CARTESIAN_POINT ( 'NONE',  ( -45.63203486222421645, 1439.443257688872563, 266.1896917324526726 ) ) ;
#25673=B_SPLINE_CURVE_WITH_KNOTS ( 'NONE', 3,
 ( #103454, #7210, #51416, #26760, #93954, #58720, #60949, #84463, #50869, #101232, #487, #24532, #9414, #34610, #42456, #101795, #50338, #68796, #102897, #59289, #102357, #7750, #86120, #76615, #76071, #84999, #110767, #34057, #25641, #17220, #95076, #85547, #26195, #43576, #60383, #41368, #3806, #1581, #35716, #96179, #104019, #97819, #21097, #71579, #44133, #106232, #69905, #19454, #20013, #28983, #18894, #79385, #29518, #72117, #2149, #63709 ),
 .UNSPECIFIED., .F., .F.,
 ( 4, 2, 1, 1, 1, 1, 2, 2, 2, 2, 1, 1, 1, 2, 2, 2, 2, 1, 2, 2, 2, 1, 1, 1, 2, 2, 2, 2, 1, 2, 2, 2, 2, 4 ),
 ( 0.000000000000000000, 0.06250000000058465732, 0.09375000000078338724, 0.1093750000008827661, 0.1171875000010262624, 0.1210937500010046269, 0.1230468750009933304, 0.1250000000009820478, 0.1875000000034836301, 0.2187500000048276938, 0.2343750000054989624, 0.2421875000058345828, 0.2460937500060023930, 0.2480468750060855210, 0.2500000000061686212, 0.3750000000050800475, 0.4375000000045334847, 0.4687500000042576498, 0.4843750000041224801, 0.5000000000039872550, 0.6250000000038240522, 0.6875000000037424508, 0.7187500000036169956, 0.7343750000035543790, 0.7421875000034289238, 0.7500000000033034686, 0.8125000000023775426, 0.8437500000019949598, 0.8593750000017285062, 0.8671875000015897283, 0.8750000000014510615, 0.9062500000010844659, 0.9375000000007178702, 1.000000000000000000 ),
 .UNSPECIFIED. ) ;
#25674=CARTESIAN_POINT ( 'NONE',  ( -20.90394540422069980, 1503.716088646810022, 192.3069530248390038 ) ) ;
#25675=CARTESIAN_POINT ( 'NONE',  ( -17.94945718479999996, 1425.820490840630100, 226.0414718358979940 ) ) ;
#25676=CARTESIAN_POINT ( 'NONE',  ( 30.14929311095689712, 1467.662589780429926, 268.0960305645629660 ) ) ;
#25678=CARTESIAN_POINT ( 'NONE',  ( -17.10883999351027995, 1422.201703527962763, 226.7517257450004990 ) ) ;
#25681=CARTESIAN_POINT ( 'NONE',  ( 18.29456550085305722, 1459.185740094880657, 227.8225150847868576 ) ) ;
#25685=CARTESIAN_POINT ( 'NONE',  ( 2.994691737410000165, 1448.276535293540064, 183.8510770426980230 ) ) ;
#25686=CARTESIAN_POINT ( 'NONE',  ( 26.90457551740000142, 1451.808372585929874, 135.6460129701980009 ) ) ;
#25688=CARTESIAN_POINT ( 'NONE',  ( -1.545842073307790221, 1419.284905465829979, 228.1300558533139906 ) ) ;
#25690=FACE_OUTER_BOUND ( 'NONE', #31721, .T. ) ;
#25691=CARTESIAN_POINT ( 'NONE',  ( 17.22592482065188335, 1444.324653571828321, 162.9227486220069352 ) ) ;
#25692=CARTESIAN_POINT ( 'NONE',  ( 0.8431686273640290885, 1408.942504484590017, 186.6283956538120208 ) ) ;
#25694=DIRECTION ( 'NONE',  ( 0.3282391760791590340, 0.000000000000000000, 0.9445946449598763284 ) ) ;
#25695=CARTESIAN_POINT ( 'NONE',  ( 5.558638042260000134, 1409.107172305129779, 229.7071683781979914 ) ) ;
#25697=CARTESIAN_POINT ( 'NONE',  ( 13.38476763809124392, 1421.175358059063910, 231.0590627358187987 ) ) ;
#25700=CARTESIAN_POINT ( 'NONE',  ( 11.69294537312310212, 1432.337845730949994, 150.8474185596319899 ) ) ;
#25701=CARTESIAN_POINT ( 'NONE',  ( 16.81223453394349932, 1414.913060391199906, 210.6693087035600058 ) ) ;
#25704=CARTESIAN_POINT ( 'NONE',  ( -35.36897276635060194, 1450.220808574710190, 136.2318720995220076 ) ) ;
#25707=CARTESIAN_POINT ( 'NONE',  ( -12.15345572500000060, 1468.554006641229989, 265.6112251771979800 ) ) ;
#25708=CARTESIAN_POINT ( 'NONE',  ( -21.30850104442570725, 1508.868632323871680, 191.9271483346492175 ) ) ;
#25709=CARTESIAN_POINT ( 'NONE',  ( 11.27545180150000093, 1433.597762786930161, 151.5307970856979978 ) ) ;
#25710=EDGE_CURVE ( 'NONE', #109266, #94676, #63135, .T. ) ;
#25711=CARTESIAN_POINT ( 'NONE',  ( 19.00000000000000000, 1440.913060387330006, 209.1218459616979999 ) ) ;
#25712=CARTESIAN_POINT ( 'NONE',  ( 12.61823209568870041, 1416.826860677879949, 196.1892328963569980 ) ) ;
#25717=CARTESIAN_POINT ( 'NONE',  ( 23.10442899973940101, 1411.095127650270115, 207.3185325528490068 ) ) ;
#25718=CARTESIAN_POINT ( 'NONE',  ( 12.26702939395647007, 1398.276750168901572, 204.6184358455272445 ) ) ;
#25719=CARTESIAN_POINT ( 'NONE',  ( -21.40702923872559893, 1509.660610321120203, 231.3015350172729825 ) ) ;
#25720=CARTESIAN_POINT ( 'NONE',  ( 23.18005801880000050, 1410.911243130629828, 212.9212581473880164 ) ) ;
#25723=CARTESIAN_POINT ( 'NONE',  ( 19.25375188179999952, 1464.258769156330118, 224.0689215379980226 ) ) ;
#25724=CARTESIAN_POINT ( 'NONE',  ( 25.44482548711661707, 1436.625151458925302, 137.3198232488083477 ) ) ;
#25726=CARTESIAN_POINT ( 'NONE',  ( 19.81155763900000011, 1453.313060387329870, 213.6835017937279986 ) ) ;
#25730=CARTESIAN_POINT ( 'NONE',  ( 0.2053818061695609765, 1459.950573050879939, 182.9551974283099867 ) ) ;
#25731=LINE ( 'NONE', #104668, #21106 ) ;
#25733=CARTESIAN_POINT ( 'NONE',  ( -24.17420166734180498, 1452.068876450862490, 137.1289955490235855 ) ) ;
#25734=CARTESIAN_POINT ( 'NONE',  ( -38.71377205869448801, 1443.913060387330233, 136.9322096537518973 ) ) ;
#25736=CARTESIAN_POINT ( 'NONE',  ( -39.63067020672009733, 1438.364472241019939, 134.0999999979140114 ) ) ;
#25739=B_SPLINE_SURFACE_WITH_KNOTS ( 'NONE', 5, 5, ( 
 ( #70520, #18955, #104635, #28486, #36877, #2757 ),
 ( #19516, #27932, #96240, #53721, #105195, #45856 ),
 ( #80251, #52860, #28743, #19206, #94840, #53408 ),
 ( #27638, #18661, #18116, #96500, #19780, #86987 ),
 ( #78035, #105454, #104899, #3021, #45019, #45572 ),
 ( #62948, #62374, #70787, #3569, #61823, #10276 ) ),
 .UNSPECIFIED., .F., .F., .F.,
 ( 6, 6 ),
 ( 6, 6 ),
 ( 6.877204621659999795, 14.95798807776640160 ),
 ( -0.002550205044612160153, 2.002549943480759875 ),
 .UNSPECIFIED. ) ;
#25742=CARTESIAN_POINT ( 'NONE',  ( -16.47341459099999739, 1414.971287085229960, 211.7498588889980056 ) ) ;
#25746=CARTESIAN_POINT ( 'NONE',  ( 22.64731540989999914, 1507.637957906029897, 209.7207049147999953 ) ) ;
#25747=CARTESIAN_POINT ( 'NONE',  ( -5.364455102291621813, 1422.311257715712372, 141.1472075467242462 ) ) ;
#25755=EDGE_LOOP ( 'NONE', ( #32228, #74018, #86672, #46996, #106199, #1699, #37512 ) ) ;
#25756=CARTESIAN_POINT ( 'NONE',  ( -29.31191257029999875, 1451.029043731829915, 136.3073297265979988 ) ) ;
#25757=CARTESIAN_POINT ( 'NONE',  ( 17.11714625305222981, 1443.086052842849995, 162.7561045841209193 ) ) ;
#25761=EDGE_CURVE ( 'NONE', #59101, #4103, #82199, .T. ) ;
#25765=CARTESIAN_POINT ( 'NONE',  ( 38.49563125392135277, 1453.175225740012138, 269.5844195324700650 ) ) ;
#25766=CARTESIAN_POINT ( 'NONE',  ( -22.52594230423108002, 1509.699683626128490, 190.3521439076764068 ) ) ;
#25767=CARTESIAN_POINT ( 'NONE',  ( 19.27691768841802045, 1439.085048996816795, 212.6567080453250753 ) ) ;
#25776=DIRECTION ( 'NONE',  ( 0.5412924984494058567, 0.1391731009594480151, 0.8292365640103740443 ) ) ;
#25777=CARTESIAN_POINT ( 'NONE',  ( 13.79577721849999961, 1416.837309283630020, 196.3345427477979968 ) ) ;
#25779=ORIENTED_EDGE ( 'NONE', *, *, #55141, .T. ) ;
#25783=CARTESIAN_POINT ( 'NONE',  ( -24.55148953109999965, 1430.358502428329984, 207.1124260302279652 ) ) ;
#25784=CARTESIAN_POINT ( 'NONE',  ( -11.40400955750629919, 1426.004897788209973, 127.8394256862669920 ) ) ;
#25785=CARTESIAN_POINT ( 'NONE',  ( 16.70811614616980023, 1409.743563081069851, 192.5257515985450141 ) ) ;
#25787=CARTESIAN_POINT ( 'NONE',  ( 17.77641320823512672, 1509.653574700879062, 184.9552422975178843 ) ) ;
#25789=CARTESIAN_POINT ( 'NONE',  ( -42.46016416089999979, 1427.243204226630041, 266.3334699379980179 ) ) ;
#25791=CARTESIAN_POINT ( 'NONE',  ( 44.93136772329302175, 1446.458183624383310, 269.6838061997164573 ) ) ;
#25793=CARTESIAN_POINT ( 'NONE',  ( -37.31136631233590606, 1438.104314947570174, 136.5707455465820033 ) ) ;
#25794=ORIENTED_EDGE ( 'NONE', *, *, #79495, .F. ) ;
#25795=CARTESIAN_POINT ( 'NONE',  ( 8.565474820639810360, 1396.738687322869964, 218.6445593244839927 ) ) ;
#25797=CARTESIAN_POINT ( 'NONE',  ( -17.96824696200000204, 1459.790589356729924, 228.0722388631980095 ) ) ;
#25802=CARTESIAN_POINT ( 'NONE',  ( -9.236167301360001858, 1423.625854809029988, 144.1549878472980026 ) ) ;
#25807=CARTESIAN_POINT ( 'NONE',  ( -2.896421349160000158, 1461.194462919229863, 234.8054986878979946 ) ) ;
#25810=CARTESIAN_POINT ( 'NONE',  ( 16.68463225827704122, 1442.773887286370382, 162.0935120918187806 ) ) ;
#25812=ORIENTED_EDGE ( 'NONE', *, *, #92471, .F. ) ;
#25815=VERTEX_POINT ( 'NONE', #34448 ) ;
#25816=CARTESIAN_POINT ( 'NONE',  ( 11.74539289358659921, 1426.717885751599852, 144.7561986137889960 ) ) ;
#25818=EDGE_LOOP ( 'NONE', ( #405, #69873, #82723, #49406 ) ) ;
#25819=CARTESIAN_POINT ( 'NONE',  ( 20.59269117493390056, 1507.766073655780019, 227.7908423917359926 ) ) ;
#25820=CARTESIAN_POINT ( 'NONE',  ( -11.86176259532119914, 1432.335962297939886, 150.1420601836709920 ) ) ;
#25821=CARTESIAN_POINT ( 'NONE',  ( 2.906876508539999904, 1508.504005161229998, 236.5181634588980160 ) ) ;
#25823=CARTESIAN_POINT ( 'NONE',  ( -4.983160662360000437, 1423.641753194130160, 185.4826375174980058 ) ) ;
#25824=CARTESIAN_POINT ( 'NONE',  ( -6.569253884907100272, 1446.774627395847801, 154.4165862851036195 ) ) ;
#25826=CARTESIAN_POINT ( 'NONE',  ( -9.603402670887449588, 1410.623332638303509, 188.2819919630825041 ) ) ;
#25828=CARTESIAN_POINT ( 'NONE',  ( -16.22876982940000090, 1473.844758900830129, 223.1935655822979925 ) ) ;
#25831=CARTESIAN_POINT ( 'NONE',  ( 15.21149316085690018, 1507.619498583100039, 226.3435933218330263 ) ) ;
#25834=CARTESIAN_POINT ( 'NONE',  ( -7.357910506076572155, 1506.503176757026722, 188.2719473218194821 ) ) ;
#25835=EDGE_LOOP ( 'NONE', ( #104986, #14217, #11666, #75259 ) ) ;
#25838=CARTESIAN_POINT ( 'NONE',  ( -2.921262571303605782, 1484.943831670156214, 183.1664153039595249 ) ) ;
#25841=ORIENTED_EDGE ( 'NONE', *, *, #79276, .F. ) ;
#25844=CARTESIAN_POINT ( 'NONE',  ( -11.77148215669999942, 1427.082524922729817, 146.5557703533980032 ) ) ;
#25845=CARTESIAN_POINT ( 'NONE',  ( -10.82298596616855590, 1424.914553627307214, 144.7927276520015880 ) ) ;
#25847=CARTESIAN_POINT ( 'NONE',  ( 14.17716488154820098, 1509.408135427139996, 234.9453616465329731 ) ) ;
#25850=CARTESIAN_POINT ( 'NONE',  ( -2.455820327400000114, 1434.541746329560056, 150.3615916412979914 ) ) ;
#25852=CARTESIAN_POINT ( 'NONE',  ( -19.22484529489999971, 1470.091603696130051, 227.4635202857980119 ) ) ;
#25855=VERTEX_POINT ( 'NONE', #103857 ) ;
#25857=CARTESIAN_POINT ( 'NONE',  ( 23.58347146439999875, 1410.948704344629959, 266.7402917337980170 ) ) ;
#25859=CARTESIAN_POINT ( 'NONE',  ( 21.76798767740000073, 1449.724426459390088, 197.1464471020979943 ) ) ;
#25860=EDGE_CURVE ( 'NONE', #93518, #62097, #25470, .T. ) ;
#25861=CARTESIAN_POINT ( 'NONE',  ( -0.2962894524850000488, 1508.149850360829987, 237.5387477236979805 ) ) ;
#25863=CARTESIAN_POINT ( 'NONE',  ( -40.23240883470000284, 1442.695644260940071, 137.0096571460979646 ) ) ;
#25864=FACE_OUTER_BOUND ( 'NONE', #33700, .T. ) ;
#25866=CARTESIAN_POINT ( 'NONE',  ( -12.91070994500000069, 1445.031679802599911, 186.8505891716980045 ) ) ;
#25867=EDGE_CURVE ( 'NONE', #58583, #106936, #92916, .T. ) ;
#25868=CARTESIAN_POINT ( 'NONE',  ( -19.67658020740000069, 1453.313060387329870, 209.1218459620799877 ) ) ;
#25871=ORIENTED_EDGE ( 'NONE', *, *, #91691, .F. ) ;
#25873=CARTESIAN_POINT ( 'NONE',  ( 1.467664789042199880, 1488.639595165949913, 181.9190109959569952 ) ) ;
#25874=CARTESIAN_POINT ( 'NONE',  ( -13.02339026569499936, 1409.367847196819866, 216.4483738165630200 ) ) ;
#25879=CARTESIAN_POINT ( 'NONE',  ( -21.85618413279999572, 1471.634021946630128, 266.7712522008980613 ) ) ;
#25882=CARTESIAN_POINT ( 'NONE',  ( 17.85701005936880037, 1417.692377606080072, 223.8866627408119712 ) ) ;
#25884=DIRECTION ( 'NONE',  ( -0.7074300732568278294, 0.02470400251969403355, -0.7063514732138287400 ) ) ;
#25886=CARTESIAN_POINT ( 'NONE',  ( -11.91388749740000108, 1435.945967586000052, 151.0354243678980026 ) ) ;
#25887=B_SPLINE_SURFACE_WITH_KNOTS ( 'NONE', 5, 1, ( 
 ( #98050, #72335 ),
 ( #106465, #62292 ),
 ( #90195, #80161 ),
 ( #105932, #107009 ),
 ( #71249, #29749 ),
 ( #21324, #105372 ),
 ( #12941, #29211 ),
 ( #20785, #47122 ),
 ( #99693, #14596 ) ),
 .UNSPECIFIED., .F., .F., .F.,
 ( 6, 3, 6 ),
 ( 2, 2 ),
 ( 2.977480884639999825, 6.317148707589999468, 12.84597182780000146 ),
 ( -13.57759716840000053, -1.277641461229999997 ),
 .UNSPECIFIED. ) ;
#25890=CARTESIAN_POINT ( 'NONE',  ( 38.60856580501570079, 1443.613625263020140, 137.1750438873210101 ) ) ;
#25891=CARTESIAN_POINT ( 'NONE',  ( -23.79341481419999837, 1411.104518318830060, 207.4167121037980053 ) ) ;
#25892=CARTESIAN_POINT ( 'NONE',  ( 14.27054156580000033, 1415.934222461130048, 196.9549357831980103 ) ) ;
#25894=CARTESIAN_POINT ( 'NONE',  ( -23.74108753817469974, 1436.296634041249945, 212.5883363871789982 ) ) ;
#25895=B_SPLINE_SURFACE_WITH_KNOTS ( 'NONE', 5, 1, ( 
 ( #71101, #98460 ),
 ( #2786, #36906 ),
 ( #11711, #30145 ),
 ( #3341, #89513 ),
 ( #87320, #10615 ),
 ( #36354, #37465 ),
 ( #21174, #104664 ),
 ( #105225, #28512 ),
 ( #71668, #63253 ),
 ( #88959, #12251 ),
 ( #46440, #38018 ),
 ( #72198, #29601 ),
 ( #65442, #66001 ),
 ( #23941, #90610 ),
 ( #56479, #74944 ) ),
 .UNSPECIFIED., .F., .F., .F.,
 ( 6, 3, 3, 3, 6 ),
 ( 2, 2 ),
 ( 62.08793508101459935, 77.35181134419998727, 110.5715862349999981, 131.5832540680000022, 137.5414126590000023 ),
 ( -8.966358544465320387E-05, 4.664442523398899532 ),
 .UNSPECIFIED. ) ;
#25900=CARTESIAN_POINT ( 'NONE',  ( -22.92334060740000368, 1411.083494322230081, 211.1057397514580032 ) ) ;
#25902=CARTESIAN_POINT ( 'NONE',  ( 11.72965050516489960, 1426.700625785630109, 143.6412421599850120 ) ) ;
#25906=DIRECTION ( 'NONE',  ( 0.000000000000000000, 0.000000000000000000, 1.000000000000000000 ) ) ;
#25908=CARTESIAN_POINT ( 'NONE',  ( -7.465699360109450566, 1398.134876652174398, 219.7837385695886212 ) ) ;
#25909=DIRECTION ( 'NONE',  ( 0.000000000000000000, 1.000000000000000000, 0.000000000000000000 ) ) ;
#25913=CARTESIAN_POINT ( 'NONE',  ( 40.70529000807259479, 1444.199214852859996, 137.0833980395239848 ) ) ;
#25917=CARTESIAN_POINT ( 'NONE',  ( 11.31987186643520005, 1434.499830821800060, 151.5385002157870247 ) ) ;
#25924=CARTESIAN_POINT ( 'NONE',  ( 16.07755494024289789, 1424.336998408409954, 191.1005968644109885 ) ) ;
#25925=CARTESIAN_POINT ( 'NONE',  ( 13.84277359751999903, 1452.957910650600070, 224.2058953944790005 ) ) ;
#25926=CARTESIAN_POINT ( 'NONE',  ( 15.93081432798890162, 1498.109692542990160, 231.2852987234049920 ) ) ;
#25927=CARTESIAN_POINT ( 'NONE',  ( 4.709678610000000099, 1507.637404285230105, 181.8385339875979980 ) ) ;
#25931=CARTESIAN_POINT ( 'NONE',  ( 3.512785867830420180E-12, 1395.913060387330006, 198.1220674046479928 ) ) ;
#25932=CARTESIAN_POINT ( 'NONE',  ( 14.14453214075280130, 1415.673583083940002, 197.1727595455269864 ) ) ;
#25934=CARTESIAN_POINT ( 'NONE',  ( 11.85636366039999956, 1431.657450769009984, 149.9409103546979907 ) ) ;
#25936=ORIENTED_EDGE ( 'NONE', *, *, #18144, .T. ) ;
#25937=CARTESIAN_POINT ( 'NONE',  ( 14.11983163027539945, 1435.196066153720039, 149.2983271376729988 ) ) ;
#25938=ORIENTED_EDGE ( 'NONE', *, *, #2794, .T. ) ;
#25940=CARTESIAN_POINT ( 'NONE',  ( -19.64047668580450079, 1507.861171522700261, 229.4570402217679828 ) ) ;
#25945=B_SPLINE_CURVE_WITH_KNOTS ( 'NONE', 3,
 ( #110175, #17736, #41327, #448, #67648, #60341, #34569, #42984, #76574, #8803, #100658, #23942, #66554, #34016, #58686, #77143, #59792, #101756, #68754 ),
 .UNSPECIFIED., .F., .F.,
 ( 4, 2, 2, 2, 1, 1, 1, 2, 2, 2, 4 ),
 ( 0.000000000000000000, 0.2499999999971138087, 0.3749999999957732699, 0.4374999999950133778, 0.4687499999947145057, 0.4843749999945661799, 0.4921874999944930718, 0.4960937499945325957, 0.4999999999945721196, 0.7499999999972859488, 1.000000000000000000 ),
 .UNSPECIFIED. ) ;
#25952=CARTESIAN_POINT ( 'NONE',  ( 22.43577763531170177, 1440.913060387330006, 229.3504540723680236 ) ) ;
#25953=CARTESIAN_POINT ( 'NONE',  ( -18.87155817529999879, 1509.015965077730016, 230.2334335948979742 ) ) ;
#25955=CARTESIAN_POINT ( 'NONE',  ( -11.36373753890000060, 1409.476796350030099, 189.5641612269979817 ) ) ;
#25957=CARTESIAN_POINT ( 'NONE',  ( -11.00355868719999997, 1414.913528139930122, 195.9181521845980001 ) ) ;
#25958=ORIENTED_EDGE ( 'NONE', *, *, #92623, .T. ) ;
#25959=CARTESIAN_POINT ( 'NONE',  ( 22.86920506520000274, 1432.244263168689940, 216.4472202372080005 ) ) ;
#25965=CARTESIAN_POINT ( 'NONE',  ( 24.07913224159999999, 1410.980207832730002, 209.6302583906470147 ) ) ;
#25966=CARTESIAN_POINT ( 'NONE',  ( -11.14671771210699980, 1434.019356486030119, 151.6529807626459956 ) ) ;
#25973=EDGE_LOOP ( 'NONE', ( #93036, #74971, #17969 ) ) ;
#25975=B_SPLINE_CURVE_WITH_KNOTS ( 'NONE', 5,
 ( #26906, #87367, #61628, #85693, #614, #44270 ),
 .UNSPECIFIED., .F., .F.,
 ( 6, 6 ),
 ( -22.60166147410000193, -9.285377787159999841 ),
 .UNSPECIFIED. ) ;
#25976=CARTESIAN_POINT ( 'NONE',  ( 35.51629366599999571, 1458.123799197230028, 261.8361074970979416 ) ) ;
#25977=CARTESIAN_POINT ( 'NONE',  ( 1.533207931480909281, 1452.703037475436531, 183.4902445653410155 ) ) ;
#25979=CARTESIAN_POINT ( 'NONE',  ( -6.854598081119999797, 1507.853711066930146, 235.7978674939980124 ) ) ;
#25982=CARTESIAN_POINT ( 'NONE',  ( 19.09048981950000012, 1456.312469618329942, 226.2254625276979709 ) ) ;
#25987=CARTESIAN_POINT ( 'NONE',  ( 0.3382504354559999760, 1405.989871386730101, 266.9611136494980315 ) ) ;
#25990=CARTESIAN_POINT ( 'NONE',  ( 12.89348889060000047, 1425.726071551529913, 223.5999069075979833 ) ) ;
#25991=CARTESIAN_POINT ( 'NONE',  ( -1.556370157619999972, 1414.996444526030018, 226.5294865527980051 ) ) ;
#25994=CARTESIAN_POINT ( 'NONE',  ( 28.38546418346980005, 1435.488905026550128, 135.6743912052290000 ) ) ;
#25995=CARTESIAN_POINT ( 'NONE',  ( -26.02650053749999870, 1446.299505181590121, 138.3420241739979986 ) ) ;
#25996=CARTESIAN_POINT ( 'NONE',  ( -45.63712966311000230, 1440.913059426480004, 268.9747523979869470 ) ) ;
#26003=ORIENTED_EDGE ( 'NONE', *, *, #5288, .F. ) ;
#26005=CARTESIAN_POINT ( 'NONE',  ( 2.500000001190000098, 1425.952486856224823, 183.8951078798580454 ) ) ;
#26007=CARTESIAN_POINT ( 'NONE',  ( 16.93884299705920071, 1507.634939766059915, 188.0954313100240256 ) ) ;
#26008=CARTESIAN_POINT ( 'NONE',  ( -0.5319847658459999629, 1417.295974482030033, 234.8116028735980194 ) ) ;
#26011=CARTESIAN_POINT ( 'NONE',  ( 19.36248556598933845, 1455.763297351556048, 225.9778007399211788 ) ) ;
#26012=B_SPLINE_SURFACE_WITH_KNOTS ( 'NONE', 5, 5, ( 
 ( #56625, #90760, #48231, #30301, #98055, #65584 ),
 ( #64493, #90198, #108108, #47672, #82372, #76039 ),
 ( #110184, #33455, #89113, #38701, #81800, #107565 ),
 ( #5671, #38158, #46587, #14600, #107013, #73978 ),
 ( #99696, #22988, #84435, #12402, #80722, #4030 ),
 ( #72339, #102323, #87197, #26164, #101765, #60350 ),
 ( #77693, #103989, #61468, #10489, #59801, #93921 ),
 ( #9930, #94473, #34579, #16641, #26730, #50837 ),
 ( #18863, #17746, #85516, #25054, #78238, #34026 ),
 ( #77153, #68218, #17188, #68763, #102867, #53060 ),
 ( #42995, #27286, #59257, #95047, #44660, #1005 ),
 ( #8262, #35683, #44100, #51384, #42426, #78801 ) ),
 .UNSPECIFIED., .F., .F., .F.,
 ( 6, 3, 3, 6 ),
 ( 6, 6 ),
 ( -3.831645261493030061E-05, 4.695069562340000502, 9.390139124690000116, 12.39571065745260015 ),
 ( 0.000000000000000000, 2.000038316452609877 ),
 .UNSPECIFIED. ) ;
#26015=CARTESIAN_POINT ( 'NONE',  ( 42.06228640162340326, 1440.913015538450054, 269.6487197970989769 ) ) ;
#26016=CARTESIAN_POINT ( 'NONE',  ( -12.97408886687033558, 1451.220703713921466, 150.9179168472272750 ) ) ;
#26018=CARTESIAN_POINT ( 'NONE',  ( 25.95593065371449981, 1435.599270252459974, 136.1659943809549986 ) ) ;
#26019=CARTESIAN_POINT ( 'NONE',  ( -8.759831409813630287, 1396.218960441809713, 202.3723544762349889 ) ) ;
#26023=CARTESIAN_POINT ( 'NONE',  ( 11.94046459599999999, 1438.194204504490017, 147.6340003373980210 ) ) ;
#26028=CARTESIAN_POINT ( 'NONE',  ( 11.08126927090000002, 1426.907418872530116, 96.53620495169779758 ) ) ;
#26030=CARTESIAN_POINT ( 'NONE',  ( 23.13309424899999911, 1409.720885835030003, 209.3985505581069901 ) ) ;
#26031=CARTESIAN_POINT ( 'NONE',  ( -11.85917953740000108, 1433.048083576320096, 150.2760150462979993 ) ) ;
#26032=ADVANCED_FACE ( 'NONE', ( #31549 ), #69030, .T. ) ;
#26033=CARTESIAN_POINT ( 'NONE',  ( -2.512979519748912871, 1421.005010328889739, 185.2548484884229367 ) ) ;
#26035=B_SPLINE_CURVE_WITH_KNOTS ( 'NONE', 3,
 ( #76261, #10155, #25831, #60032, #17421, #18533, #51619, #85755, #9051, #103667, #43224, #26965 ),
 .UNSPECIFIED., .F., .F.,
 ( 4, 2, 2, 2, 2, 4 ),
 ( -0.1123552072008140029, -0.09789080009285709705, -0.08345977780132710078, -0.05408602703201970119, -0.02844234071178690371, 0.000000000000000000 ),
 .UNSPECIFIED. ) ;
#26037=CARTESIAN_POINT ( 'NONE',  ( 8.247663932760000094, 1509.138309195029933, 181.6038655551980128 ) ) ;
#26038=CARTESIAN_POINT ( 'NONE',  ( 2.479936572040000176, 1449.203345246219897, 182.3137392801979786 ) ) ;
#26043=FACE_OUTER_BOUND ( 'NONE', #17617, .T. ) ;
#26044=AXIS2_PLACEMENT_3D ( 'NONE', #33838, #67471, #101576 ) ;
#26046=CARTESIAN_POINT ( 'NONE',  ( -1.476727087160000007, 1474.160226259529963, 270.1373298219979802 ) ) ;
#26052=B_SPLINE_SURFACE_WITH_KNOTS ( 'NONE', 5, 5, ( 
 ( #90053, #3889, #99002, #39097, #13892, #63255, #64895, #30148, #64339 ),
 ( #106321, #37467, #82211, #88962, #98462, #12806, #30709, #72731, #107413 ),
 ( #3343, #89515, #22279, #56481, #63789, #73839, #13336, #97363, #20635 ),
 ( #47528, #38020, #54838, #4427, #73275, #5516, #12253, #21731, #46986 ),
 ( #55934, #90612, #31263, #71670, #81110, #39671, #107966, #21175, #65445 ),
 ( #46442, #80574, #55383, #81649, #38553, #4954, #99555, #22839, #88423 ) ),
 .UNSPECIFIED., .F., .F., .F.,
 ( 6, 6 ),
 ( 6, 3, 6 ),
 ( 32.35314871179999585, 33.17903199610000087 ),
 ( 0.000000000000000000, 1.000000000000000000, 2.000000000000000000 ),
 .UNSPECIFIED. ) ;
#26053=CARTESIAN_POINT ( 'NONE',  ( -22.68012700156480221, 1507.275789587069767, 208.4743628061380036 ) ) ;
#26055=CARTESIAN_POINT ( 'NONE',  ( 3.320336327120199993, 1408.845769750169893, 195.0433881623220032 ) ) ;
#26056=CARTESIAN_POINT ( 'NONE',  ( -18.52619959329609856, 1409.651470360259964, 269.5393490716199949 ) ) ;
#26059=CARTESIAN_POINT ( 'NONE',  ( -11.86561511689999904, 1432.302094693870004, 149.9824189743979730 ) ) ;
#26060=CARTESIAN_POINT ( 'NONE',  ( 13.48763800459999906, 1443.604195705930124, 188.0280588922980201 ) ) ;
#26061=ORIENTED_EDGE ( 'NONE', *, *, #62287, .F. ) ;
#26063=CARTESIAN_POINT ( 'NONE',  ( -22.06852505282392229, 1506.535970898746427, 209.1479492043462187 ) ) ;
#26066=CARTESIAN_POINT ( 'NONE',  ( -2.901842622390000237, 1485.480021844630073, 183.2625817364980207 ) ) ;
#26070=CIRCLE ( 'NONE', #110102, 1.999999954393710588 ) ;
#26073=EDGE_CURVE ( 'NONE', #70574, #96461, #2123, .T. ) ;
#26076=CARTESIAN_POINT ( 'NONE',  ( -27.78811175689999757, 1509.876756555029942, 201.6112073881680260 ) ) ;
#26077=EDGE_CURVE ( 'NONE', #15423, #2577, #108344, .T. ) ;
#26078=CARTESIAN_POINT ( 'NONE',  ( 5.508554876272072853, 1427.333971811663332, 134.0999999980980135 ) ) ;
#26082=VECTOR ( 'NONE', #36455, 1000.000000000000114 ) ;
#26085=CARTESIAN_POINT ( 'NONE',  ( -7.386732042270000242, 1447.816120179589916, 185.7874553686979766 ) ) ;
#26086=ORIENTED_EDGE ( 'NONE', *, *, #31790, .F. ) ;
#26088=CARTESIAN_POINT ( 'NONE',  ( 27.49404549280000154, 1488.693617962429926, 208.9387129124660021 ) ) ;
#26089=EDGE_CURVE ( 'NONE', #24504, #18900, #94179, .T. ) ;
#26090=CARTESIAN_POINT ( 'NONE',  ( 19.69912643434309985, 1477.269676134359997, 225.7986965500050189 ) ) ;
#26091=CARTESIAN_POINT ( 'NONE',  ( -25.83444865290000081, 1435.692496567170110, 136.3622603797980162 ) ) ;
#26094=CARTESIAN_POINT ( 'NONE',  ( -15.12936268429999842, 1413.157696382230142, 226.7979570398979945 ) ) ;
#26099=CARTESIAN_POINT ( 'NONE',  ( -3.619881192149999816, 1412.838016826329977, 232.4469606129980264 ) ) ;
#26105=CARTESIAN_POINT ( 'NONE',  ( 12.52472169154620119, 1435.436724083190029, 150.8432062471219979 ) ) ;
#26106=CARTESIAN_POINT ( 'NONE',  ( -4.118451982573078318, 1441.437192870819899, 184.2612739964320099 ) ) ;
#26108=CARTESIAN_POINT ( 'NONE',  ( -23.32961689541300032, 1509.451491745719977, 225.2641564516229948 ) ) ;
#26110=EDGE_CURVE ( 'NONE', #36972, #12048, #61863, .T. ) ;
#26111=CARTESIAN_POINT ( 'NONE',  ( -20.01067139950000140, 1507.877425041529932, 188.9709217985979706 ) ) ;
#26115=CARTESIAN_POINT ( 'NONE',  ( 19.60066840860000070, 1508.321169339229982, 188.7280170016979923 ) ) ;
#26129=CARTESIAN_POINT ( 'NONE',  ( 17.80652095830000192, 1415.128105756529976, 210.3714338108779884 ) ) ;
#26131=FACE_OUTER_BOUND ( 'NONE', #66, .T. ) ;
#26133=CARTESIAN_POINT ( 'NONE',  ( 38.11840859848789620, 1440.913060382519916, 256.4711611452369766 ) ) ;
#26138=CARTESIAN_POINT ( 'NONE',  ( 1.552591573816870074, 1415.651572961190141, 190.6893068747150153 ) ) ;
#26140=CARTESIAN_POINT ( 'NONE',  ( -27.96976564920000285, 1509.201555287429983, 210.6640595776979978 ) ) ;
#26141=CARTESIAN_POINT ( 'NONE',  ( 2.449123001110840470, 1410.376692143526043, 185.5607414632172834 ) ) ;
#26143=FACE_OUTER_BOUND ( 'NONE', #92293, .T. ) ;
#26144=CARTESIAN_POINT ( 'NONE',  ( -14.44411435775000108, 1509.548839476979992, 182.8006741103589832 ) ) ;
#26145=EDGE_CURVE ( 'NONE', #93372, #109266, #88840, .T. ) ;
#26148=B_SPLINE_CURVE_WITH_KNOTS ( 'NONE', 5,
 ( #51924, #51356, #9362, #68738, #44075, #36219, #69848, #78213, #53036, #8789, #68195, #102842 ),
 .UNSPECIFIED., .F., .F.,
 ( 6, 3, 3, 6 ),
 ( 0.000000000000000000, 0.2753503963466049087, 0.7584501321178948041, 1.000000000000000000 ),
 .UNSPECIFIED. ) ;
#26152=CARTESIAN_POINT ( 'NONE',  ( 15.70760032500000136, 1452.364538897129933, 147.9013275455980079 ) ) ;
#26153=ADVANCED_FACE ( 'NONE', ( #27855 ), #43995, .F. ) ;
#26154=CARTESIAN_POINT ( 'NONE',  ( 0.000000000000000000, 1401.254281879943164, 137.0999999980979851 ) ) ;
#26157=CARTESIAN_POINT ( 'NONE',  ( 23.93532109230000060, 1509.062825906829858, 195.0658673578979858 ) ) ;
#26158=ORIENTED_EDGE ( 'NONE', *, *, #17536, .T. ) ;
#26159=CARTESIAN_POINT ( 'NONE',  ( -17.67443188212616434, 1460.218465826193324, 228.1753073352142849 ) ) ;
#26164=CARTESIAN_POINT ( 'NONE',  ( 16.93701544105510237, 1508.758026244639950, 231.4689131582919970 ) ) ;
#26166=CARTESIAN_POINT ( 'NONE',  ( 39.71405398454739100, 1440.955322443209980, 136.8225870968819891 ) ) ;
#26167=CARTESIAN_POINT ( 'NONE',  ( 5.451195050909999503E-14, 1410.389826760030019, 269.3346704430979912 ) ) ;
#26172=CARTESIAN_POINT ( 'NONE',  ( -12.84239665067440050, 1435.935719077439899, 150.8114796122480072 ) ) ;
#26173=CARTESIAN_POINT ( 'NONE',  ( -19.87824503550000088, 1484.486535651230042, 191.0390967410979783 ) ) ;
#26174=CARTESIAN_POINT ( 'NONE',  ( 1.337177534479999874, 1409.127636081429955, 185.8413015776979762 ) ) ;
#26176=CARTESIAN_POINT ( 'NONE',  ( -11.53918879130000086, 1434.258396904259826, 151.3471600665980077 ) ) ;
#26179=CARTESIAN_POINT ( 'NONE',  ( -2.080482507937010173, 1450.172760316540007, 183.1621233083120046 ) ) ;
#26180=CARTESIAN_POINT ( 'NONE',  ( 2.228957627849999845, 1464.745732024629888, 236.9236403881979811 ) ) ;
#26181=ORIENTED_EDGE ( 'NONE', *, *, #102233, .F. ) ;
#26183=CARTESIAN_POINT ( 'NONE',  ( -44.79032719779999638, 1444.249662561040168, 269.6864475883979821 ) ) ;
#26184=CARTESIAN_POINT ( 'NONE',  ( -23.72500815532294638, 1436.282246268031486, 212.5115884784333105 ) ) ;
#26188=ADVANCED_FACE ( 'NONE', ( #12149 ), #35025, .F. ) ;
#26189=CARTESIAN_POINT ( 'NONE',  ( -1.045136941292439999E-08, 1473.203432950090018, 261.6844113528200069 ) ) ;
#26190=CARTESIAN_POINT ( 'NONE',  ( 2.816490516637460306, 1409.065320745530244, 230.5891822038450130 ) ) ;
#26191=CARTESIAN_POINT ( 'NONE',  ( -1.184716195880000100, 1415.245980409529921, 227.1375410387979912 ) ) ;
#26192=CARTESIAN_POINT ( 'NONE',  ( -10.22449367669999987, 1419.740728945330147, 231.9262419709980065 ) ) ;
#26195=CARTESIAN_POINT ( 'NONE',  ( -0.8188256143092619288, 1485.179768421087147, 182.0112568513308133 ) ) ;
#26197=CARTESIAN_POINT ( 'NONE',  ( -45.81331811595649839, 1439.434550458239983, 268.7575993174490350 ) ) ;
#26198=CARTESIAN_POINT ( 'NONE',  ( -2.500000000000000000, 1431.404049859629822, 183.8987783686980038 ) ) ;
#26199=EDGE_CURVE ( 'NONE', #48650, #59045, #49188, .T. ) ;
#26200=CARTESIAN_POINT ( 'NONE',  ( 26.21857634852423047, 1435.413047617778602, 135.3174475323201591 ) ) ;
#26203=FACE_OUTER_BOUND ( 'NONE', #76452, .T. ) ;
#26206=CIRCLE ( 'NONE', #72753, 1.000002393159227010 ) ;
#26207=CARTESIAN_POINT ( 'NONE',  ( -26.86092681858010067, 1451.722180651600183, 135.7938040751629671 ) ) ;
#26208=EDGE_LOOP ( 'NONE', ( #24291, #37019, #61934, #8169, #98887 ) ) ;
#26211=CARTESIAN_POINT ( 'NONE',  ( 15.28316325029999945, 1506.811133727029983, 193.2980993196979966 ) ) ;
#26212=EDGE_CURVE ( 'NONE', #27637, #44414, #45237, .T. ) ;
#26214=CARTESIAN_POINT ( 'NONE',  ( -23.72150209009999955, 1436.115933882590070, 211.9493966405580068 ) ) ;
#26219=CARTESIAN_POINT ( 'NONE',  ( -4.199545054528389443, 1410.181605891940080, 269.8668074039729845 ) ) ;
#26221=CARTESIAN_POINT ( 'NONE',  ( 6.457394820134600089, 1416.588625856350063, 231.2278128514520006 ) ) ;
#26222=CARTESIAN_POINT ( 'NONE',  ( -0.2658540493943280514, 1507.120020986029886, 237.3289608297170048 ) ) ;
#26224=EDGE_LOOP ( 'NONE', ( #21085, #101645, #87232, #29166, #61387 ) ) ;
#26225=ORIENTED_EDGE ( 'NONE', *, *, #39138, .T. ) ;
#26226=CARTESIAN_POINT ( 'NONE',  ( -23.60449339185390016, 1410.417139340120002, 210.1580197820780143 ) ) ;
#26228=CARTESIAN_POINT ( 'NONE',  ( -4.159820404830000484, 1424.695346998130162, 185.9273424667980237 ) ) ;
#26230=CARTESIAN_POINT ( 'NONE',  ( -45.66959065914245031, 1440.472161357215555, 266.1886509646802779 ) ) ;
#26232=CARTESIAN_POINT ( 'NONE',  ( -18.87215647974419852, 1416.576002133260090, 207.5745059148389942 ) ) ;
#26233=ADVANCED_FACE ( 'NONE', ( #19857 ), #94941, .T. ) ;
#26234=CARTESIAN_POINT ( 'NONE',  ( -19.62275393000000179, 1430.792229069829773, 223.6261147419979807 ) ) ;
#26235=CARTESIAN_POINT ( 'NONE',  ( 35.73139755195909117, 1463.185613522950007, 267.0027651688810124 ) ) ;
#26236=CARTESIAN_POINT ( 'NONE',  ( -11.66472555445337633, 1463.778378584986285, 231.3814271317881150 ) ) ;
#26240=CARTESIAN_POINT ( 'NONE',  ( 18.75857324853270924, 1458.153377316558135, 227.2545901758803950 ) ) ;
#26241=CARTESIAN_POINT ( 'NONE',  ( 1.528009309627449852, 1453.500417136500118, 183.4545884030709999 ) ) ;
#26245=B_SPLINE_CURVE_WITH_KNOTS ( 'NONE', 3,
 ( #22179, #5406, #107862, #64798, #98907, #65340, #97805, #23294, #48532, #56376, #91615, #90506, #98361, #108420, #13784, #14342, #82671, #5962, #82108, #100006, #31151, #56927, #21083, #55287, #99448, #21634, #22725, #89961, #40107, #33347, #101643, #50189, #15987, #7062, #24931, #42314, #58031, #84315, #102213, #59142, #15439, #49631, #33904, #16527, #75389, #66444, #83767, #93264, #6507, #17070, #74834, #76469, #59683, #24396, #68099, #58581, #93796, #49083, #110622, #41217, #92168, #101097, #50718, #23839, #7606, #40662, #25493, #109526, #41760, #51267, #83218, #32802, #8148, #108977, #32264 ),
 .UNSPECIFIED., .F., .F.,
 ( 4, 2, 2, 2, 2, 2, 1, 2, 2, 1, 1, 1, 2, 2, 2, 2, 2, 2, 1, 1, 2, 2, 2, 2, 2, 1, 1, 1, 2, 2, 2, 2, 2, 2, 1, 1, 1, 1, 2, 2, 2, 2, 2, 4 ),
 ( 0.000000000000000000, 0.03124999999985165339, 0.06249999999970330677, 0.09374999999955496710, 0.1249999999994066135, 0.1406249999993321453, 0.1425781249993236521, 0.1428222656243233468, 0.1430664062493230415, 0.1435546874993231803, 0.1445312499993236244, 0.1484374999993233746, 0.1562499999993230138, 0.1874999999993217370, 0.2499999999993183786, 0.2812499999993166577, 0.2851562499993169353, 0.2871093749993167688, 0.2890624999993166022, 0.2968749999993162136, 0.3124999999993156030, 0.3749999999993113842, 0.4374999999993071653, 0.4687499999993049449, 0.4843749999993032795, 0.4921874999993019473, 0.4960937499993012811, 0.4980468749993015032, 0.4990234374993021693, 0.4999999999993027799, 0.6249999999993367528, 0.6874999999993542943, 0.7187499999993625099, 0.7343749999993666178, 0.7421874999993686162, 0.7460937499993696154, 0.7480468749993695043, 0.7490234374993699484, 0.7495117187493701705, 0.7499999999993703925, 0.8124999999995278221, 0.8749999999996852518, 0.9374999999998425704, 1.000000000000000000 ),
 .UNSPECIFIED. ) ;
#26246=CARTESIAN_POINT ( 'NONE',  ( 25.67981543420000179, 1451.858828621529938, 135.9465745059980009 ) ) ;
#26250=CARTESIAN_POINT ( 'NONE',  ( 17.44743351239999996, 1409.522338191229892, 195.3742125755979941 ) ) ;
#26251=CARTESIAN_POINT ( 'NONE',  ( 13.51610093809999924, 1444.324653571829913, 169.3501091259980171 ) ) ;
#26252=CARTESIAN_POINT ( 'NONE',  ( 3.363947596952667318, 1439.689793485319342, 184.4158855439752074 ) ) ;
#26253=CARTESIAN_POINT ( 'NONE',  ( 1.043151750310000070, 1416.586530163930092, 233.4334045153980242 ) ) ;
#26254=CARTESIAN_POINT ( 'NONE',  ( -21.57689972017744395, 1429.260891947445543, 219.1104016736593678 ) ) ;
#26257=CARTESIAN_POINT ( 'NONE',  ( 19.77969251879999746, 1507.818093401829856, 229.2755605921979907 ) ) ;
#26259=ADVANCED_FACE ( 'NONE', ( #67409 ), #57897, .T. ) ;
#26260=CARTESIAN_POINT ( 'NONE',  ( 14.36154233419531501, 1421.756987585290744, 230.5507565205384992 ) ) ;
#26261=ORIENTED_EDGE ( 'NONE', *, *, #109015, .T. ) ;
#26262=CARTESIAN_POINT ( 'NONE',  ( 12.80019129569889991, 1416.529254608160045, 221.9949054940630049 ) ) ;
#26264=CARTESIAN_POINT ( 'NONE',  ( -0.5150210539746830074, 1410.202340106000293, 233.1625166594439804 ) ) ;
#26268=CARTESIAN_POINT ( 'NONE',  ( -15.71554774059999815, 1452.384630541829893, 224.8635561783979711 ) ) ;
#26269=CARTESIAN_POINT ( 'NONE',  ( -21.77056747205107712, 1509.419234473328515, 191.5442852694430087 ) ) ;
#26270=CARTESIAN_POINT ( 'NONE',  ( 11.89682012279999945, 1433.280912625190012, 150.0673495551980068 ) ) ;
#26271=CARTESIAN_POINT ( 'NONE',  ( 15.71554773450000297, 1452.384630544830088, 224.8635562088979896 ) ) ;
#26273=CARTESIAN_POINT ( 'NONE',  ( 12.51099735422840098, 1416.825783990419950, 196.0986168021389915 ) ) ;
#26276=CARTESIAN_POINT ( 'NONE',  ( 14.89703407660000067, 1485.172368269729986, 224.4040237037980035 ) ) ;
#26277=CARTESIAN_POINT ( 'NONE',  ( -4.664011873159999766, 1486.047054426829845, 182.2406068358980065 ) ) ;
#26279=DIRECTION ( 'NONE',  ( 0.7074300732638268974, 0.02470400251906259420, -0.7063514732068408852 ) ) ;
#26280=CARTESIAN_POINT ( 'NONE',  ( -30.16083877470000019, 1510.094636368229885, 211.8907222485079842 ) ) ;
#26283=CARTESIAN_POINT ( 'NONE',  ( 2.964073292005991345, 1446.907476413705126, 170.5322007588701752 ) ) ;
#26284=CARTESIAN_POINT ( 'NONE',  ( 25.74953088568717163, 1436.651976592735537, 137.0890486594359459 ) ) ;
#26286=CARTESIAN_POINT ( 'NONE',  ( 22.78047381600000065, 1519.913060387329779, 214.2867222517980110 ) ) ;
#26290=CARTESIAN_POINT ( 'NONE',  ( 0.1636539809332889783, 1484.078125311330041, 181.9191924309680246 ) ) ;
#26298=ORIENTED_EDGE ( 'NONE', *, *, #45205, .T. ) ;
#26299=LINE ( 'NONE', #35265, #89610 ) ;
#26309=CARTESIAN_POINT ( 'NONE',  ( -17.32903452410000256, 1411.910626558729973, 192.2240021034980089 ) ) ;
#26311=ORIENTED_EDGE ( 'NONE', *, *, #60018, .T. ) ;
#26312=CARTESIAN_POINT ( 'NONE',  ( -15.80615402491370247, 1410.712807750240017, 226.7221385999669963 ) ) ;
#26313=CARTESIAN_POINT ( 'NONE',  ( 5.519891178750000016, 1440.499824924530003, 154.7645185998979969 ) ) ;
#26314=ORIENTED_EDGE ( 'NONE', *, *, #44853, .F. ) ;
#26317=CARTESIAN_POINT ( 'NONE',  ( 26.26214385720000166, 1509.606682185630007, 219.0507925541380132 ) ) ;
#26322=CARTESIAN_POINT ( 'NONE',  ( -11.60004869885203505, 1428.147403133767057, 134.2065354802118975 ) ) ;
#26323=CARTESIAN_POINT ( 'NONE',  ( 17.94073347927875872, 1434.894695372993056, 215.4556157790318309 ) ) ;
#26325=CARTESIAN_POINT ( 'NONE',  ( 1.600048698852036821, 1411.254281879943164, 137.0999999980979851 ) ) ;
#26330=AXIS2_PLACEMENT_3D ( 'NONE', #30241, #64976, #81197 ) ;
#26331=CARTESIAN_POINT ( 'NONE',  ( 3.701620314320000382, 1446.913866055039989, 156.0867562885979964 ) ) ;
#26332=CARTESIAN_POINT ( 'NONE',  ( -2.500000000000000000, 1433.175796427819932, 157.5194111165980075 ) ) ;
#26333=CARTESIAN_POINT ( 'NONE',  ( 44.92382427180000093, 1440.913060384100163, 269.6913831871979710 ) ) ;
#26337=ORIENTED_EDGE ( 'NONE', *, *, #103789, .T. ) ;
#26339=CARTESIAN_POINT ( 'NONE',  ( -24.41209542680000055, 1449.795792328920015, 203.6715618845580025 ) ) ;
#26341=CARTESIAN_POINT ( 'NONE',  ( -11.61237467649999999, 1426.780387251330012, 135.2650375955979882 ) ) ;
#26342=CARTESIAN_POINT ( 'NONE',  ( 16.75289443972269865, 1410.133484963379942, 192.0576568603480041 ) ) ;
#26344=CARTESIAN_POINT ( 'NONE',  ( 18.18605408113305799, 1509.667548394901132, 185.2623056092570266 ) ) ;
#26345=CARTESIAN_POINT ( 'NONE',  ( -22.91749086919999812, 1507.625766668030110, 207.6071136176580012 ) ) ;
#26346=CARTESIAN_POINT ( 'NONE',  ( -40.57810857620000178, 1433.211872144790050, 261.6156768307980087 ) ) ;
#26348=CARTESIAN_POINT ( 'NONE',  ( 29.34423976395289912, 1509.844966207019979, 209.6154881191580159 ) ) ;
#26352=CARTESIAN_POINT ( 'NONE',  ( -35.08468067933920054, 1437.159863514480094, 136.5376250597369960 ) ) ;
#26353=ORIENTED_EDGE ( 'NONE', *, *, #99676, .T. ) ;
#26354=CARTESIAN_POINT ( 'NONE',  ( 10.35663606681439930, 1396.797897193559947, 200.7170876621850084 ) ) ;
#26356=EDGE_CURVE ( 'NONE', #69273, #2114, #14444, .T. ) ;
#26357=CARTESIAN_POINT ( 'NONE',  ( 37.65047687761219919, 1442.773887286080026, 137.1096749932030150 ) ) ;
#26358=ORIENTED_EDGE ( 'NONE', *, *, #88850, .T. ) ;
#26359=ORIENTED_EDGE ( 'NONE', *, *, #40504, .T. ) ;
#26360=CIRCLE ( 'NONE', #35324, 2.000061678640922214 ) ;
#26362=CARTESIAN_POINT ( 'NONE',  ( -11.84030404028099781, 1430.236004227029980, 151.0624551439379957 ) ) ;
#26363=EDGE_CURVE ( 'NONE', #22756, #109851, #57119, .T. ) ;
#26367=CARTESIAN_POINT ( 'NONE',  ( -11.87502386937130083, 1433.007271227619867, 149.9804723889419904 ) ) ;
#26369=CARTESIAN_POINT ( 'NONE',  ( 28.17098211812724173, 1509.816545695249943, 206.0731778711173092 ) ) ;
#26372=DIRECTION ( 'NONE',  ( -0.3363363969979660806, -0.9417419115949053898, 0.000000000000000000 ) ) ;
#26378=CARTESIAN_POINT ( 'NONE',  ( 11.81236103907129831, 1428.866417594400218, 148.7658394821069692 ) ) ;
#26381=CARTESIAN_POINT ( 'NONE',  ( -1.465793917108519917, 1484.360957496709943, 182.4810413606819850 ) ) ;
#26385=CARTESIAN_POINT ( 'NONE',  ( -5.949769683449999569, 1423.165531658830105, 186.4741557280979976 ) ) ;
#26386=CARTESIAN_POINT ( 'NONE',  ( 10.86918694049999878, 1409.184211811729938, 270.3751304090980057 ) ) ;
#26391=CARTESIAN_POINT ( 'NONE',  ( -15.42411914529999883, 1451.321947525430005, 222.6614283628979933 ) ) ;
#26393=CARTESIAN_POINT ( 'NONE',  ( 15.70632159480000034, 1471.312091221729816, 194.7047488413979863 ) ) ;
#26394=CARTESIAN_POINT ( 'NONE',  ( -4.668567705819710589, 1423.680010517363371, 184.4694098598055803 ) ) ;
#26397=CARTESIAN_POINT ( 'NONE',  ( 17.97366410996650288, 1422.795681845899935, 225.1544947853240046 ) ) ;
#26399=CARTESIAN_POINT ( 'NONE',  ( -5.789249456297649310, 1423.399501566140088, 91.66914618043580276 ) ) ;
#26401=CARTESIAN_POINT ( 'NONE',  ( 18.22058378356810238, 1424.504050405589851, 223.7587054751699895 ) ) ;
#26403=CARTESIAN_POINT ( 'NONE',  ( -2.993081948865825570, 1485.686210600610138, 182.6348840854386140 ) ) ;
#26409=CARTESIAN_POINT ( 'NONE',  ( -15.31719378736699966, 1507.616838180409786, 191.9970397177449968 ) ) ;
#26410=CARTESIAN_POINT ( 'NONE',  ( -11.25570387199999978, 1428.983030176930015, 150.6823813367980165 ) ) ;
#26412=CARTESIAN_POINT ( 'NONE',  ( -5.698435440679999964, 1440.539195541149866, 185.7251249343980248 ) ) ;
#26416=CARTESIAN_POINT ( 'NONE',  ( 0.3641805750159999855, 1424.317995881729985, 227.5054904076980051 ) ) ;
#26419=CARTESIAN_POINT ( 'NONE',  ( -16.38967734719999925, 1460.095605315129887, 228.4964222805979830 ) ) ;
#26421=CARTESIAN_POINT ( 'NONE',  ( 21.88497915990000209, 1410.158872715429879, 268.8545754686979876 ) ) ;
#26422=CARTESIAN_POINT ( 'NONE',  ( 25.00977939330000055, 1436.598012869960030, 137.9330249918980087 ) ) ;
#26423=CARTESIAN_POINT ( 'NONE',  ( 23.35803260569999651, 1449.721564088129981, 201.4915734787180099 ) ) ;
#26424=CARTESIAN_POINT ( 'NONE',  ( 15.81201445386249915, 1506.433683730510211, 224.3933755863170063 ) ) ;
#26425=CARTESIAN_POINT ( 'NONE',  ( -0.4986853141550000035, 1508.982344982729956, 238.8510891614980096 ) ) ;
#26427=CARTESIAN_POINT ( 'NONE',  ( -41.61955346608320383, 1442.631757267950206, 136.0084039258269968 ) ) ;
#26428=CARTESIAN_POINT ( 'NONE',  ( -18.97170710130291127, 1506.426094405750746, 198.0110083291505703 ) ) ;
#26429=CARTESIAN_POINT ( 'NONE',  ( -18.81809407629999953, 1416.219761279530076, 207.5984327672580037 ) ) ;
#26430=CARTESIAN_POINT ( 'NONE',  ( -14.15644638650000076, 1445.184054452470036, 188.6148688927980004 ) ) ;
#26431=CARTESIAN_POINT ( 'NONE',  ( 18.89924248923649941, 1416.831923566683599, 210.6687426849658493 ) ) ;
#26436=CARTESIAN_POINT ( 'NONE',  ( -12.32543969330590095, 1409.343474225730006, 200.6744456079329950 ) ) ;
#26440=CARTESIAN_POINT ( 'NONE',  ( -18.39364418590000128, 1473.256894900929865, 268.3411905449979713 ) ) ;
#26441=CARTESIAN_POINT ( 'NONE',  ( -18.54648005354870222, 1507.559782640589901, 227.6869933707240250 ) ) ;
#26442=CARTESIAN_POINT ( 'NONE',  ( 0.3368680511838070268, 1419.194708778680024, 184.5876889618309917 ) ) ;
#26443=CARTESIAN_POINT ( 'NONE',  ( -24.04911540300000183, 1508.500175526130079, 222.3302192762980098 ) ) ;
#26447=CARTESIAN_POINT ( 'NONE',  ( 17.96271488095740310, 1423.981419269019852, 225.6927239374410306 ) ) ;
#26449=CARTESIAN_POINT ( 'NONE',  ( -9.663014860980000620, 1442.759804623820173, 153.0865865510980086 ) ) ;
#26450=CARTESIAN_POINT ( 'NONE',  ( -26.12012303998839968, 1482.704885440409953, 211.0358973181160138 ) ) ;
#26453=CARTESIAN_POINT ( 'NONE',  ( -22.52398816560000228, 1409.699615386230107, 206.4986819826179953 ) ) ;
#26454=CARTESIAN_POINT ( 'NONE',  ( 14.39499504100000138, 1414.971339025629959, 199.6144774512380025 ) ) ;
#26457=CARTESIAN_POINT ( 'NONE',  ( 0.8288084222790000899, 1440.444625599219989, 150.6821045058979962 ) ) ;
#26463=CARTESIAN_POINT ( 'NONE',  ( 11.70972657649789994, 1426.713614540399931, 142.2152413248659855 ) ) ;
#26467=CARTESIAN_POINT ( 'NONE',  ( -0.1681561557501680126, 1420.473116156940023, 182.7663335526739843 ) ) ;
#26469=VECTOR ( 'NONE', #88316, 999.9999999999998863 ) ;
#26473=CARTESIAN_POINT ( 'NONE',  ( -18.80245169759999868, 1449.640794194290038, 193.0678026872980126 ) ) ;
#26475=CARTESIAN_POINT ( 'NONE',  ( 37.73053733700000123, 1449.071358796530149, 136.3468597391979813 ) ) ;
#26479=CARTESIAN_POINT ( 'NONE',  ( 11.91460776122049836, 1433.652109726360095, 150.4736492753009998 ) ) ;
#26487=CARTESIAN_POINT ( 'NONE',  ( 13.88167667317130061, 1452.893272873260003, 224.0381707035730017 ) ) ;
#26488=CARTESIAN_POINT ( 'NONE',  ( 16.21991559299999963, 1507.811519393530261, 231.6071110291980233 ) ) ;
#26489=CARTESIAN_POINT ( 'NONE',  ( -0.1200844908460000082, 1507.645210318029967, 180.8332078508980203 ) ) ;
#26491=FACE_OUTER_BOUND ( 'NONE', #84960, .T. ) ;
#26495=CARTESIAN_POINT ( 'NONE',  ( 14.09832007171499946, 1415.595619977640126, 197.2198605877450177 ) ) ;
#26499=CARTESIAN_POINT ( 'NONE',  ( 13.77200850713100166, 1434.987125276089955, 148.8039589176320021 ) ) ;
#26501=ORIENTED_EDGE ( 'NONE', *, *, #33786, .F. ) ;
#26506=CARTESIAN_POINT ( 'NONE',  ( -5.629143959155359589, 1407.138657505239962, 221.3608015446720003 ) ) ;
#26513=CARTESIAN_POINT ( 'NONE',  ( -0.06540635796760001230, 1508.967893392429914, 238.8759467174980102 ) ) ;
#26517=CARTESIAN_POINT ( 'NONE',  ( 21.16084444640559781, 1440.913060387330006, 223.1877144379700155 ) ) ;
#26518=CARTESIAN_POINT ( 'NONE',  ( -19.56461557969999987, 1509.492094407029981, 230.7210067600980210 ) ) ;
#26521=EDGE_CURVE ( 'NONE', #660, #59669, #109276, .T. ) ;
#26522=CARTESIAN_POINT ( 'NONE',  ( -13.22111819830000101, 1410.747856120229926, 189.8101292799980229 ) ) ;
#26523=CARTESIAN_POINT ( 'NONE',  ( 0.1595995995380000143, 1486.508831850330125, 181.8147405652979671 ) ) ;
#26526=CARTESIAN_POINT ( 'NONE',  ( 20.44315793190000008, 1427.648655133030161, 220.7419575218979730 ) ) ;
#26530=CARTESIAN_POINT ( 'NONE',  ( 6.588066741534899684, 1432.346495030159986, 154.2384753665409960 ) ) ;
#26532=CARTESIAN_POINT ( 'NONE',  ( 5.405732451549999595, 1434.707887834109897, 154.6595955769979867 ) ) ;
#26542=EDGE_CURVE ( 'NONE', #101005, #24504, #101297, .T. ) ;
#26543=CARTESIAN_POINT ( 'NONE',  ( -16.95041357008780381, 1486.123329410929728, 187.6573714191846705 ) ) ;
#26547=CARTESIAN_POINT ( 'NONE',  ( 13.01667709480000035, 1472.524070381529782, 262.4459321295979635 ) ) ;
#26548=CARTESIAN_POINT ( 'NONE',  ( -33.91369265678890343, 1437.010538859309918, 136.5611844326260211 ) ) ;
#26550=CARTESIAN_POINT ( 'NONE',  ( -3.671418758874580135, 1507.725831406179850, 236.7601474078430215 ) ) ;
#26552=CARTESIAN_POINT ( 'NONE',  ( 11.87502394290000041, 1433.007271885549926, 149.9804723912980080 ) ) ;
#26553=CARTESIAN_POINT ( 'NONE',  ( 17.60715780957560028, 1409.859378988159960, 222.6687402345539795 ) ) ;
#26556=VECTOR ( 'NONE', #84744, 1000.000000000000000 ) ;
#26557=ORIENTED_EDGE ( 'NONE', *, *, #5896, .F. ) ;
#26559=CARTESIAN_POINT ( 'NONE',  ( 0.2161990375369999828, 1405.749718733130067, 267.5371521303979989 ) ) ;
#26560=CARTESIAN_POINT ( 'NONE',  ( 27.76495483950000320, 1507.998797214829892, 207.7528748142179609 ) ) ;
#26561=CARTESIAN_POINT ( 'NONE',  ( 24.67650857399999964, 1442.459111621740021, 212.6549697286179992 ) ) ;
#26564=CARTESIAN_POINT ( 'NONE',  ( 0.2178157486290130118, 1452.982786607829894, 183.2541296479709843 ) ) ;
#26565=CARTESIAN_POINT ( 'NONE',  ( -27.30961438860000001, 1446.324487285050054, 137.1908813208980291 ) ) ;
#26566=CARTESIAN_POINT ( 'NONE',  ( -12.59722456003193614, 1416.835288280216218, 194.8442844972019259 ) ) ;
#26570=CARTESIAN_POINT ( 'NONE',  ( -38.89645918617060971, 1452.470420418182130, 269.5913652274755918 ) ) ;
#26571=ORIENTED_EDGE ( 'NONE', *, *, #50187, .T. ) ;
#26572=CARTESIAN_POINT ( 'NONE',  ( 3.932775080253070321, 1448.980696629100066, 184.2693358254829832 ) ) ;
#26573=FACE_OUTER_BOUND ( 'NONE', #84729, .T. ) ;
#26576=CARTESIAN_POINT ( 'NONE',  ( -0.4034485627230000038, 1415.424111452130091, 233.4119044095980087 ) ) ;
#26579=CARTESIAN_POINT ( 'NONE',  ( 23.84533589473599946, 1452.080362908450070, 136.9869410992479857 ) ) ;
#26582=B_SPLINE_CURVE_WITH_KNOTS ( 'NONE', 3,
 ( #107123, #37722, #81912, #72985, #98167, #14157, #31510 ),
 .UNSPECIFIED., .F., .F.,
 ( 4, 3, 4 ),
 ( -157.7108139869999945, -101.4631973234740059, -30.86246212755040119 ),
 .UNSPECIFIED. ) ;
#26584=CARTESIAN_POINT ( 'NONE',  ( -18.64588652299999794, 1416.828040475229955, 208.5593769277110141 ) ) ;
#26585=CARTESIAN_POINT ( 'NONE',  ( -17.84204394271100114, 1415.932840154009909, 209.4661953843999811 ) ) ;
#26586=CARTESIAN_POINT ( 'NONE',  ( 24.94575029499999985, 1435.868986808510044, 137.3376222402980034 ) ) ;
#26587=CARTESIAN_POINT ( 'NONE',  ( -13.28785892136501090, 1443.221467901020333, 169.3801346219540847 ) ) ;
#26589=CARTESIAN_POINT ( 'NONE',  ( -16.34066499524799809, 1409.492051723080067, 225.1454641123489750 ) ) ;
#26590=CARTESIAN_POINT ( 'NONE',  ( 4.946284671489999951, 1438.194204504490017, 150.2421849576980151 ) ) ;
#26592=EDGE_LOOP ( 'NONE', ( #66242, #43434, #89191, #101674 ) ) ;
#26594=DIRECTION ( 'NONE',  ( 0.03489949670250328678, -0.9993908270190956511, 0.000000000000000000 ) ) ;
#26595=CARTESIAN_POINT ( 'NONE',  ( 10.67434751849999941, 1425.711863979930058, 92.68737539269790204 ) ) ;
#26598=CARTESIAN_POINT ( 'NONE',  ( 4.158758314750929941, 1424.719666987580013, 185.0501326411299772 ) ) ;
#26599=CARTESIAN_POINT ( 'NONE',  ( -2.805877869264751912, 1419.865265789671412, 186.1385795869015283 ) ) ;
#26605=CIRCLE ( 'NONE', #28379, 1.000000000000000000 ) ;
#26608=ORIENTED_EDGE ( 'NONE', *, *, #74694, .T. ) ;
#26609=VERTEX_POINT ( 'NONE', #34135 ) ;
#26613=CARTESIAN_POINT ( 'NONE',  ( -0.9478952718030000391, 1471.581311749730048, 269.6149987492980244 ) ) ;
#26615=CARTESIAN_POINT ( 'NONE',  ( -0.5359254698907657266, 1410.309918930317508, 185.0934049815310800 ) ) ;
#26617=B_SPLINE_CURVE_WITH_KNOTS ( 'NONE', 4,
 ( #104919, #69126, #95961, #27110, #10290 ),
 .UNSPECIFIED., .F., .F.,
 ( 5, 5 ),
 ( 1.967616199060000071, 3.613988937050000239 ),
 .UNSPECIFIED. ) ;
#26620=CARTESIAN_POINT ( 'NONE',  ( 22.57636543919999994, 1411.060965668830022, 206.4507511260079866 ) ) ;
#26622=CARTESIAN_POINT ( 'NONE',  ( -2.500000000000000000, 1448.204674875420096, 169.9458606413490145 ) ) ;
#26624=CARTESIAN_POINT ( 'NONE',  ( 13.39680589851269943, 1407.451641433219947, 204.6080239228549829 ) ) ;
#26625=CARTESIAN_POINT ( 'NONE',  ( -11.94938536144059960, 1407.933938028119883, 269.6043413872750421 ) ) ;
#26629=CARTESIAN_POINT ( 'NONE',  ( 13.39080007399999950, 1444.566365729019935, 188.1636725064979885 ) ) ;
#26630=ORIENTED_EDGE ( 'NONE', *, *, #81750, .F. ) ;
#26631=EDGE_LOOP ( 'NONE', ( #77997, #64018, #102082 ) ) ;
#26636=CARTESIAN_POINT ( 'NONE',  ( -18.73391074110000076, 1470.474872498130026, 190.1492551849979975 ) ) ;
#26641=CARTESIAN_POINT ( 'NONE',  ( -29.25495334789999902, 1509.872415968630094, 208.6412278715359889 ) ) ;
#26645=CARTESIAN_POINT ( 'NONE',  ( -3.897582650600000420, 1407.987767143230258, 196.4241821881980172 ) ) ;
#26646=CARTESIAN_POINT ( 'NONE',  ( -12.66827423740000036, 1410.284634327829963, 227.9748965595980223 ) ) ;
#26647=CARTESIAN_POINT ( 'NONE',  ( -12.29575548589999912, 1445.147284857479917, 186.2458214697980168 ) ) ;
#26650=CARTESIAN_POINT ( 'NONE',  ( 25.81147510750000151, 1488.682669033129741, 215.7372411931079910 ) ) ;
#26652=CARTESIAN_POINT ( 'NONE',  ( -24.82487920160000172, 1435.549279665109907, 136.8315248583980122 ) ) ;
#26654=CIRCLE ( 'NONE', #37389, 23.05825808840000946 ) ;
#26656=DIRECTION ( 'NONE',  ( 0.000000000000000000, 1.000000000000000000, 0.000000000000000000 ) ) ;
#26659=ORIENTED_EDGE ( 'NONE', *, *, #34974, .T. ) ;
#26660=DIRECTION ( 'NONE',  ( 0.7470743985697100298, 0.03252369126397396115, -0.6639443143127832236 ) ) ;
#26661=CARTESIAN_POINT ( 'NONE',  ( -1.927358540839999801, 1410.305851446330053, 232.8221572591980078 ) ) ;
#26667=CARTESIAN_POINT ( 'NONE',  ( 12.21725359463179927, 1434.113778757119917, 149.7882389495470079 ) ) ;
#26669=CARTESIAN_POINT ( 'NONE',  ( 14.40204153438889989, 1488.406232492609888, 231.6322952228059933 ) ) ;
#26670=CARTESIAN_POINT ( 'NONE',  ( -22.14848624618590023, 1507.850251992550056, 225.9298071555170111 ) ) ;
#26671=CARTESIAN_POINT ( 'NONE',  ( -1.682318697039999922, 1409.475163255830012, 186.2035163265980202 ) ) ;
#26674=EDGE_CURVE ( 'NONE', #94444, #15354, #6571, .T. ) ;
#26676=CARTESIAN_POINT ( 'NONE',  ( -4.649633098669999853, 1420.176632532630038, 186.4708447736979906 ) ) ;
#26677=CARTESIAN_POINT ( 'NONE',  ( 20.05348425099999687, 1509.507670995530134, 187.8272102738980038 ) ) ;
#26678=FACE_OUTER_BOUND ( 'NONE', #88514, .T. ) ;
#26679=ORIENTED_EDGE ( 'NONE', *, *, #26212, .T. ) ;
#26681=CARTESIAN_POINT ( 'NONE',  ( -6.240097849340000558, 1499.713794654230014, 181.2208793725980058 ) ) ;
#26683=AXIS2_PLACEMENT_3D ( 'NONE', #60576, #661, #78458 ) ;
#26684=CARTESIAN_POINT ( 'NONE',  ( 4.123035148590000531, 1421.670590998829766, 184.9173806918979892 ) ) ;
#26691=CARTESIAN_POINT ( 'NONE',  ( -16.66101146819999812, 1410.867390116229899, 191.7375337716979971 ) ) ;
#26692=CARTESIAN_POINT ( 'NONE',  ( 18.62061618460000290, 1416.021639796329964, 209.9108522146810003 ) ) ;
#26695=CARTESIAN_POINT ( 'NONE',  ( -7.467133905529999893, 1443.913060387330006, 149.7989312978980081 ) ) ;
#26696=CARTESIAN_POINT ( 'NONE',  ( -1.757532416683340148, 1451.933574871519795, 184.1885909450070073 ) ) ;
#26703=CARTESIAN_POINT ( 'NONE',  ( -11.87899307332345522, 1433.117273378820073, 149.9761472051002329 ) ) ;
#26704=CARTESIAN_POINT ( 'NONE',  ( 11.89856584206491874, 1410.698127348937987, 189.7512122486814974 ) ) ;
#26705=AXIS2_PLACEMENT_3D ( 'NONE', #36604, #1356, #35496 ) ;
#26707=B_SPLINE_SURFACE_WITH_KNOTS ( 'NONE', 5, 5, ( 
 ( #97269, #63167, #28979, #105131, #88878, #88329 ),
 ( #12163, #36820, #3801, #62620, #37931, #72113 ),
 ( #71010, #27309, #26753, #28422, #87222, #78830 ),
 ( #60941, #61490, #78262, #79932, #18337, #95619 ),
 ( #18886, #96738, #53084, #10512, #2141, #20008 ),
 ( #54203, #46900, #99458, #47978, #65898, #31712 ) ),
 .UNSPECIFIED., .F., .F., .F.,
 ( 6, 6 ),
 ( 6, 6 ),
 ( 19.64510849129999670, 96.65569525989999988 ),
 ( -2.775557561569999727E-17, 1.000000000000000000 ),
 .UNSPECIFIED. ) ;
#26714=EDGE_CURVE ( 'NONE', #103179, #59173, #6439, .T. ) ;
#26715=EDGE_CURVE ( 'NONE', #40553, #62944, #33023, .T. ) ;
#26716=CARTESIAN_POINT ( 'NONE',  ( 21.14467612950000230, 1450.943517307629918, 144.6008493241980091 ) ) ;
#26720=CARTESIAN_POINT ( 'NONE',  ( 23.36488590689999967, 1508.462599307330038, 194.4514040896980021 ) ) ;
#26722=CARTESIAN_POINT ( 'NONE',  ( -1.442946131772449903, 1414.913527292460003, 226.2142476967059963 ) ) ;
#26723=VECTOR ( 'NONE', #19019, 1000.000000000000000 ) ;
#26729=EDGE_CURVE ( 'NONE', #78872, #28184, #15367, .T. ) ;
#26730=CARTESIAN_POINT ( 'NONE',  ( 18.10666025242040078, 1508.254734886140113, 230.4759121335879968 ) ) ;
#26733=CARTESIAN_POINT ( 'NONE',  ( 22.18308977499999912, 1506.802866779730039, 209.2929401371579843 ) ) ;
#26737=CARTESIAN_POINT ( 'NONE',  ( -11.46423977836468744, 1434.765458290011566, 151.4552492457040387 ) ) ;
#26738=FACE_OUTER_BOUND ( 'NONE', #88812, .T. ) ;
#26739=CARTESIAN_POINT ( 'NONE',  ( 2.651685169959999921, 1409.005659273929950, 187.1129167388979795 ) ) ;
#26741=CARTESIAN_POINT ( 'NONE',  ( -10.15459880809999937, 1436.277525070270030, 152.4140741291979850 ) ) ;
#26742=CARTESIAN_POINT ( 'NONE',  ( 12.03552245250000041, 1436.199553546779953, 151.3007240698979956 ) ) ;
#26743=DIRECTION ( 'NONE',  ( 0.000000000000000000, 0.000000000000000000, -1.000000000000000000 ) ) ;
#26744=CARTESIAN_POINT ( 'NONE',  ( -14.75483871110000145, 1452.397810064229816, 149.0856641680979919 ) ) ;
#26749=CARTESIAN_POINT ( 'NONE',  ( -40.84706851859999688, 1449.487018346279910, 269.8579372096979796 ) ) ;
#26750=ADVANCED_FACE ( 'NONE', ( #103304 ), #81466, .T. ) ;
#26752=CARTESIAN_POINT ( 'NONE',  ( 17.72823807780000038, 1410.893857103729943, 223.4207927510979914 ) ) ;
#26753=CARTESIAN_POINT ( 'NONE',  ( -14.98670476610000080, 1485.045873338330011, 224.0415272780979876 ) ) ;
#26756=CARTESIAN_POINT ( 'NONE',  ( 2.926868927680989607, 1410.230421244640183, 231.6146595459809987 ) ) ;
#26758=CARTESIAN_POINT ( 'NONE',  ( -8.361365488320000594, 1417.261522080730174, 230.7875359346980133 ) ) ;
#26760=CARTESIAN_POINT ( 'NONE',  ( 0.03708545786814630707, 1486.336401889381705, 181.8124888147413003 ) ) ;
#26762=CARTESIAN_POINT ( 'NONE',  ( -45.97629855748849792, 1437.677199724009824, 266.9778860158930343 ) ) ;
#26767=EDGE_CURVE ( 'NONE', #77078, #46740, #103881, .T. ) ;
#26768=EDGE_LOOP ( 'NONE', ( #9273, #70770, #48939, #13320 ) ) ;
#26774=CARTESIAN_POINT ( 'NONE',  ( -27.03107691188749939, 1451.712358130050006, 135.7978697014619911 ) ) ;
#26776=CARTESIAN_POINT ( 'NONE',  ( -13.34233688319999978, 1434.814457747640063, 195.5472743009979979 ) ) ;
#26783=ORIENTED_EDGE ( 'NONE', *, *, #103754, .F. ) ;
#26784=CARTESIAN_POINT ( 'NONE',  ( -6.798292825562660013, 1408.601192976899711, 270.3857984775779641 ) ) ;
#26786=CARTESIAN_POINT ( 'NONE',  ( 12.35539357289999884, 1419.606906044829884, 229.3575800037980059 ) ) ;
#26790=ORIENTED_EDGE ( 'NONE', *, *, #49368, .F. ) ;
#26791=CARTESIAN_POINT ( 'NONE',  ( -22.70631399555909979, 1409.706076165010018, 209.4577935351849760 ) ) ;
#26793=CARTESIAN_POINT ( 'NONE',  ( 3.675435886750538117, 1425.136160367158254, 185.0298737722915519 ) ) ;
#26794=CIRCLE ( 'NONE', #100087, 1.999999999920172522 ) ;
#26796=CARTESIAN_POINT ( 'NONE',  ( -18.89905695062199698, 1416.828039266840278, 207.5749027128360069 ) ) ;
#26797=CARTESIAN_POINT ( 'NONE',  ( -20.02836947109999954, 1430.790674585230136, 222.8465340271980040 ) ) ;
#26799=CARTESIAN_POINT ( 'NONE',  ( 22.59632237563830159, 1471.921777372659790, 267.3281857808220252 ) ) ;
#26801=CARTESIAN_POINT ( 'NONE',  ( -16.26336930940977510, 1421.047042384238921, 227.0220306831831181 ) ) ;
#26804=CARTESIAN_POINT ( 'NONE',  ( 17.99954443082109989, 1410.904693892220166, 222.9872220945560173 ) ) ;
#26806=CARTESIAN_POINT ( 'NONE',  ( 22.73795006019999931, 1409.715685400830125, 208.6721383975130095 ) ) ;
#26810=CARTESIAN_POINT ( 'NONE',  ( 25.71786717807909994, 1451.999026050069915, 135.3980030440489770 ) ) ;
#26813=CARTESIAN_POINT ( 'NONE',  ( -18.64442766462446244, 1507.939506224431170, 229.7217055948968891 ) ) ;
#26814=CARTESIAN_POINT ( 'NONE',  ( 17.43919469369999931, 1409.522050485830050, 194.4592152026980045 ) ) ;
#26815=B_SPLINE_SURFACE_WITH_KNOTS ( 'NONE', 5, 5, ( 
 ( #70911, #69236, #87117, #19341, #103917, #17673, #11523, #19902, #60846 ),
 ( #27216, #69799, #44578, #18788, #96632, #96068, #94393, #52985, #86012 ),
 ( #54103, #94971, #2592, #44024, #10408, #53541, #88232, #102789, #26085 ),
 ( #60275, #9856, #78723, #51876, #105026, #931, #2038, #36171, #3144 ),
 ( #70355, #78160, #35055, #1472, #27763, #87688, #68682, #10969, #77619 ),
 ( #45142, #103345, #26647, #36718, #18239, #28319, #62510, #52434, #86560 ) ),
 .UNSPECIFIED., .F., .F., .F.,
 ( 6, 6 ),
 ( 6, 3, 6 ),
 ( 6.655359042069999731, 17.59398672700000077 ),
 ( 0.000000000000000000, 1.000000000000000000, 2.000000000000000000 ),
 .UNSPECIFIED. ) ;
#26816=CARTESIAN_POINT ( 'NONE',  ( 13.31869796660000027, 1444.740067931809790, 169.3753098992980028 ) ) ;
#26817=CARTESIAN_POINT ( 'NONE',  ( 2.654237714975077100, 1439.650388619271325, 183.5414635488324961 ) ) ;
#26819=CARTESIAN_POINT ( 'NONE',  ( -22.62148864339994958, 1431.812645719854345, 216.1894225434491830 ) ) ;
#26820=CARTESIAN_POINT ( 'NONE',  ( -15.36549427709999982, 1420.352425059129928, 229.0210324418980008 ) ) ;
#26822=DIRECTION ( 'NONE',  ( 0.01559025466217519272, 0.9998783227618376346, 0.0005325697541269488111 ) ) ;
#26824=EDGE_CURVE ( 'NONE', #49383, #93417, #30530, .T. ) ;
#26830=CARTESIAN_POINT ( 'NONE',  ( -0.5126689071185190905, 1409.979044830439989, 233.1189724269549970 ) ) ;
#26835=CARTESIAN_POINT ( 'NONE',  ( -23.42675388609999843, 1440.913060387330006, 234.3916895593979746 ) ) ;
#26836=VECTOR ( 'NONE', #5553, 1000.000000000000114 ) ;
#26837=EDGE_CURVE ( 'NONE', #11116, #18619, #22355, .T. ) ;
#26838=CARTESIAN_POINT ( 'NONE',  ( 22.48842373632798797, 1471.669969102955292, 266.7673555805813521 ) ) ;
#26839=CARTESIAN_POINT ( 'NONE',  ( 11.60789637760000126, 1433.302712684209837, 151.0870278953979948 ) ) ;
#26840=CARTESIAN_POINT ( 'NONE',  ( 19.62446893450000118, 1443.054186837139923, 214.3676144203579952 ) ) ;
#26842=CARTESIAN_POINT ( 'NONE',  ( 25.51103972045700274, 1440.913060399400138, 219.1553983413110132 ) ) ;
#26844=VECTOR ( 'NONE', #17552, 1000.000000000000114 ) ;
#26845=CARTESIAN_POINT ( 'NONE',  ( 22.94032544519500050, 1507.620489270479993, 210.4476540011760051 ) ) ;
#26847=CARTESIAN_POINT ( 'NONE',  ( 22.61598442209999860, 1409.702807929629898, 208.8472236539830078 ) ) ;
#26848=CARTESIAN_POINT ( 'NONE',  ( 6.232532001850000114, 1398.098440471829917, 220.5304192662980256 ) ) ;
#26849=CARTESIAN_POINT ( 'NONE',  ( -14.93146304581260075, 1509.434478566749931, 236.0736287727190188 ) ) ;
#26850=CARTESIAN_POINT ( 'NONE',  ( 23.81087019270000127, 1469.236087438830054, 218.4544119103479716 ) ) ;
#26851=CARTESIAN_POINT ( 'NONE',  ( 22.53878404599999641, 1411.058442739730026, 206.1986151668880041 ) ) ;
#26852=CARTESIAN_POINT ( 'NONE',  ( 26.14612021479581827, 1436.691281381861927, 136.8989692470566411 ) ) ;
#26854=ADVANCED_FACE ( 'NONE', ( #3109 ), #60998, .F. ) ;
#26858=CARTESIAN_POINT ( 'NONE',  ( 0.1607068516070830067, 1485.841473127519976, 181.8434205804739747 ) ) ;
#26862=DIRECTION ( 'NONE',  ( 0.000000000000000000, -1.000000000000000000, 0.000000000000000000 ) ) ;
#26865=CARTESIAN_POINT ( 'NONE',  ( -34.74890047483789601, 1451.658442319130017, 134.0999999982409747 ) ) ;
#26869=DIRECTION ( 'NONE',  ( 0.000000000000000000, -1.000000000000000000, -2.960594732333529473E-13 ) ) ;
#26872=DIRECTION ( 'NONE',  ( -1.000000000000000000, 0.000000000000000000, 0.000000000000000000 ) ) ;
#26876=VECTOR ( 'NONE', #66821, 1000.000000000000227 ) ;
#26878=DIRECTION ( 'NONE',  ( 0.0002664641286723620469, 9.557308255310623861E-06, -0.9999999644527624021 ) ) ;
#26881=CARTESIAN_POINT ( 'NONE',  ( -17.70260268349999677, 1414.015781091530016, 193.3445239933980133 ) ) ;
#26885=CARTESIAN_POINT ( 'NONE',  ( -15.68556824057530008, 1410.853906741479932, 226.7268389267310056 ) ) ;
#26886=CARTESIAN_POINT ( 'NONE',  ( -1.556370157619999972, 1414.996444526030018, 226.5294865527980051 ) ) ;
#26887=ORIENTED_EDGE ( 'NONE', *, *, #81571, .F. ) ;
#26889=ORIENTED_EDGE ( 'NONE', *, *, #78331, .T. ) ;
#26894=CARTESIAN_POINT ( 'NONE',  ( 8.410267065803780360E-17, 1471.436294031830130, 269.3346704751489824 ) ) ;
#26896=CARTESIAN_POINT ( 'NONE',  ( 18.15018407203804429, 1435.336561788914423, 215.0477887658213660 ) ) ;
#26897=CARTESIAN_POINT ( 'NONE',  ( 3.043251598679999947, 1417.779699930629931, 234.3208245700980115 ) ) ;
#26899=CARTESIAN_POINT ( 'NONE',  ( -19.87223104929999806, 1484.291808912129909, 191.2808552885979907 ) ) ;
#26901=EDGE_CURVE ( 'NONE', #4103, #93518, #89237, .T. ) ;
#26905=EDGE_CURVE ( 'NONE', #106936, #109851, #47790, .T. ) ;
#26906=CARTESIAN_POINT ( 'NONE',  ( -15.97230738210199696, 1420.722887419069821, 227.0315163971459924 ) ) ;
#26909=ORIENTED_EDGE ( 'NONE', *, *, #67976, .F. ) ;
#26910=CARTESIAN_POINT ( 'NONE',  ( -33.93529464457562028, 1436.159566638202477, 136.2997917599399500 ) ) ;
#26911=ORIENTED_EDGE ( 'NONE', *, *, #47038, .T. ) ;
#26913=CARTESIAN_POINT ( 'NONE',  ( -23.81975463399999882, 1410.917033286930064, 207.5563923665380059 ) ) ;
#26914=CARTESIAN_POINT ( 'NONE',  ( -11.23695071452640093, 1426.040567954700236, 115.9703727133710061 ) ) ;
#26915=CARTESIAN_POINT ( 'NONE',  ( 17.20744637360730067, 1410.879831455439898, 192.2037466765110025 ) ) ;
#26917=CARTESIAN_POINT ( 'NONE',  ( 30.16461248337728307, 1510.076493878218344, 208.1432171045278778 ) ) ;
#26919=CARTESIAN_POINT ( 'NONE',  ( -19.76254418480000297, 1434.994542537920097, 208.0022035227879940 ) ) ;
#26920=CARTESIAN_POINT ( 'NONE',  ( -30.28727319960000131, 1436.978278693949960, 240.1330978320980023 ) ) ;
#26922=CARTESIAN_POINT ( 'NONE',  ( 28.25996324251219960, 1508.267047287839887, 209.3916282000910201 ) ) ;
#26924=CARTESIAN_POINT ( 'NONE',  ( -37.89607820300650332, 1438.541137717810216, 136.6017170863420063 ) ) ;
#26926=CARTESIAN_POINT ( 'NONE',  ( 5.492325009455980123, 1396.104856602990139, 219.0480593849839863 ) ) ;
#26928=CARTESIAN_POINT ( 'NONE',  ( -18.27671705869999741, 1459.242480605829996, 227.8606357436979977 ) ) ;
#26934=CARTESIAN_POINT ( 'NONE',  ( -0.2617375006140000293, 1419.310405523930058, 227.5755756972980066 ) ) ;
#26938=B_SPLINE_CURVE_WITH_KNOTS ( 'NONE', 3,
 ( #32154, #51170, #59578, #93691, #16971, #110518, #33250, #58474, #93157, #109429, #84752, #8049, #100458, #67440, #59033, #32706, #68541, #8597, #239, #24828, #100996, #102640, #67994, #102106, #24292, #85298, #50619, #76368, #15875, #42769, #50077, #42217, #94255, #7503, #76930, #41665, #33800, #75822, #34367, #60136, #17529, #51732, #43334, #15334, #85867, #9169, #66342, #77482, #23741, #62359, #96483, #79146, #1896, #27081, #61807, #52294, #53393, #87542, #69097, #78580, #27621, #79697 ),
 .UNSPECIFIED., .F., .F.,
 ( 4, 2, 2, 2, 2, 2, 2, 2, 2, 2, 1, 2, 2, 2, 2, 1, 1, 1, 2, 2, 2, 2, 2, 1, 2, 2, 2, 1, 2, 2, 2, 2, 2, 4 ),
 ( 0.000000000000000000, 0.06249999999413463625, 0.09374999999120205152, 0.1093749999897352942, 0.1249999999882685370, 0.1874999999824022989, 0.2187499999793056094, 0.2343749999779313475, 0.2499999999765570302, 0.3124999999710579845, 0.3437499999684511809, 0.3593749999672830597, 0.3749999999661149386, 0.4374999999608228385, 0.4687499999580535537, 0.4843749999566689390, 0.4921874999560780783, 0.4960937499558828456, 0.4980468749556873354, 0.4999999999554918251, 0.5624999999632132042, 0.5937499999669603179, 0.6093749999689117569, 0.6171874999698874209, 0.6210937499703144127, 0.6249999999707414045, 0.6874999999758888425, 0.7187499999784625615, 0.7343749999797464234, 0.7499999999810301743, 0.8124999999857194233, 0.8437499999880609947, 0.8749999999904025660, 1.000000000000000000 ),
 .UNSPECIFIED. ) ;
#26947=EDGE_LOOP ( 'NONE', ( #107028, #15612, #97452, #63458 ) ) ;
#26948=CARTESIAN_POINT ( 'NONE',  ( 11.86566114180100051, 1432.305310558320116, 149.9823219675499786 ) ) ;
#26949=CARTESIAN_POINT ( 'NONE',  ( 12.59191600518032139, 1445.042944653935137, 186.1852526257982561 ) ) ;
#26952=CARTESIAN_POINT ( 'NONE',  ( -17.11714625305222981, 1443.086052842849995, 162.7561045841209193 ) ) ;
#26953=CARTESIAN_POINT ( 'NONE',  ( 2.953750800410000377, 1508.842156638330152, 237.0357385784979840 ) ) ;
#26956=CARTESIAN_POINT ( 'NONE',  ( -4.875918348960000870, 1422.177864437230028, 185.3310708335980053 ) ) ;
#26957=CARTESIAN_POINT ( 'NONE',  ( 2.230919469291039903, 1410.429474903630080, 269.3352092892910150 ) ) ;
#26965=CARTESIAN_POINT ( 'NONE',  ( 15.57748978360000081, 1507.212883781729943, 225.5460497861979832 ) ) ;
#26968=CARTESIAN_POINT ( 'NONE',  ( 17.63459991112690162, 1411.813115813379909, 224.8352634770240002 ) ) ;
#26969=CARTESIAN_POINT ( 'NONE',  ( -4.893927726379848409, 1506.405825327593448, 187.7130172094022100 ) ) ;
#26977=ORIENTED_EDGE ( 'NONE', *, *, #26145, .F. ) ;
#26983=CARTESIAN_POINT ( 'NONE',  ( -14.54063862746090052, 1419.501189642470081, 221.4764621185310034 ) ) ;
#26988=CARTESIAN_POINT ( 'NONE',  ( 14.42199049240000086, 1412.743552572030012, 227.9099018574979993 ) ) ;
#26990=CARTESIAN_POINT ( 'NONE',  ( -15.85075050099999849, 1459.333342989330049, 230.7228811812979927 ) ) ;
#26992=CARTESIAN_POINT ( 'NONE',  ( 35.85544596869999623, 1418.707560334130221, 266.7164716470979897 ) ) ;
#26993=CARTESIAN_POINT ( 'NONE',  ( 23.43375805480000196, 1435.459271872349973, 139.6354490908979926 ) ) ;
#26994=CARTESIAN_POINT ( 'NONE',  ( 21.00038310420000087, 1508.013874135629976, 190.5210545032980178 ) ) ;
#26995=CARTESIAN_POINT ( 'NONE',  ( -21.92914898369999932, 1430.600989885229865, 219.4305798082980061 ) ) ;
#26998=CARTESIAN_POINT ( 'NONE',  ( -1.438892233660000075, 1452.191231073930112, 183.8587012488980008 ) ) ;
#26999=DIRECTION ( 'NONE',  ( -2.745975287049403995E-15, -1.000000000000000000, 0.000000000000000000 ) ) ;
#27001=CARTESIAN_POINT ( 'NONE',  ( -12.94626818629999931, 1441.161188681390058, 188.2109162517980110 ) ) ;
#27003=CARTESIAN_POINT ( 'NONE',  ( -27.81074406628219720, 1508.344687507839808, 210.5011464727880082 ) ) ;
#27004=CARTESIAN_POINT ( 'NONE',  ( -29.16177349730000046, 1435.516078635969961, 135.2137962254980152 ) ) ;
#27009=CARTESIAN_POINT ( 'NONE',  ( -13.60185556200659995, 1409.388047650059889, 202.9415292635579817 ) ) ;
#27010=CARTESIAN_POINT ( 'NONE',  ( -2.478345701239999865, 1438.626251700270132, 157.7274745556979951 ) ) ;
#27012=CARTESIAN_POINT ( 'NONE',  ( -5.191234770863918158, 1422.191368612545830, 138.4296091694463655 ) ) ;
#27013=CARTESIAN_POINT ( 'NONE',  ( -23.45916826750000084, 1470.553228125530040, 269.3037833821979916 ) ) ;
#27016=CARTESIAN_POINT ( 'NONE',  ( 18.27178068149059698, 1424.508154551730058, 223.6268415059790016 ) ) ;
#27020=CARTESIAN_POINT ( 'NONE',  ( 17.03077326642920042, 1422.100639735759842, 226.8181581180180046 ) ) ;
#27021=CARTESIAN_POINT ( 'NONE',  ( 21.33101636929999856, 1509.431424277029919, 227.6967412429980300 ) ) ;
#27022=CARTESIAN_POINT ( 'NONE',  ( 15.22885431829999980, 1495.920296619829969, 224.7378832126979944 ) ) ;
#27024=CARTESIAN_POINT ( 'NONE',  ( -20.50000000000000000, 1443.913060387330006, 169.0968414572980123 ) ) ;
#27027=CARTESIAN_POINT ( 'NONE',  ( -22.84695657510000188, 1409.710893691230012, 207.6723829003780111 ) ) ;
#27029=CARTESIAN_POINT ( 'NONE',  ( 17.29183750270000175, 1416.216252248729916, 203.8075771790779811 ) ) ;
#27037=AXIS2_PLACEMENT_3D ( 'NONE', #49712, #16066, #75473 ) ;
#27042=EDGE_CURVE ( 'NONE', #48449, #106610, #102718, .T. ) ;
#27043=CARTESIAN_POINT ( 'NONE',  ( -23.32329893220000017, 1415.973289857730151, 210.9192745123079931 ) ) ;
#27047=CARTESIAN_POINT ( 'NONE',  ( -4.234262180109699791, 1398.039394699497734, 221.4129439625630482 ) ) ;
#27049=DIRECTION ( 'NONE',  ( 1.000000000000000000, 0.000000000000000000, 0.000000000000000000 ) ) ;
#27050=CARTESIAN_POINT ( 'NONE',  ( 1.893906785159999995, 1508.749492714529879, 237.3763040025980047 ) ) ;
#27053=CARTESIAN_POINT ( 'NONE',  ( 39.57440995424759933, 1448.587977546229922, 136.2060456146669765 ) ) ;
#27055=VERTEX_POINT ( 'NONE', #86951 ) ;
#27056=ORIENTED_EDGE ( 'NONE', *, *, #91961, .T. ) ;
#27057=CARTESIAN_POINT ( 'NONE',  ( 11.41050180535800074, 1433.984814470099991, 151.4218912366809775 ) ) ;
#27063=CARTESIAN_POINT ( 'NONE',  ( 16.04547803650780224, 1423.236165506360067, 191.1345828222399916 ) ) ;
#27064=CARTESIAN_POINT ( 'NONE',  ( 4.579624579470000789, 1427.832655172230034, 112.4493539157979995 ) ) ;
#27068=CARTESIAN_POINT ( 'NONE',  ( 2.284878824769999817, 1507.640563443429983, 181.2510407452979848 ) ) ;
#27069=CARTESIAN_POINT ( 'NONE',  ( -5.191737366139999921, 1415.425433635630043, 192.3072415768979795 ) ) ;
#27070=CARTESIAN_POINT ( 'NONE',  ( 15.96541745440000248, 1410.402655727529918, 226.9120801968979890 ) ) ;
#27072=DIRECTION ( 'NONE',  ( -1.000000000000000000, -5.823966869780190178E-19, 4.137698748469999823E-18 ) ) ;
#27076=EDGE_LOOP ( 'NONE', ( #96944, #89989, #79838, #84216 ) ) ;
#27077=CARTESIAN_POINT ( 'NONE',  ( 13.80090640870000129, 1435.296980361239775, 149.7022445371979984 ) ) ;
#27081=CARTESIAN_POINT ( 'NONE',  ( 12.76025368180385478, 1444.996096971014367, 169.4538372660288985 ) ) ;
#27082=CARTESIAN_POINT ( 'NONE',  ( -1.606022318079999955, 1464.996810821029840, 236.7393652189979889 ) ) ;
#27089=CARTESIAN_POINT ( 'NONE',  ( 4.240521952282210627, 1446.386233147809889, 162.7524229475580171 ) ) ;
#27090=CARTESIAN_POINT ( 'NONE',  ( 0.5968024102800000286, 1507.130435900830207, 237.3073193260979963 ) ) ;
#27091=VERTEX_POINT ( 'NONE', #21370 ) ;
#27093=EDGE_LOOP ( 'NONE', ( #90040, #38214, #5878, #3891 ) ) ;
#27095=CARTESIAN_POINT ( 'NONE',  ( -19.86721352349999847, 1507.838653463430092, 229.2281063170979678 ) ) ;
#27098=CARTESIAN_POINT ( 'NONE',  ( -14.54785189459999906, 1409.587746979729900, 191.1299195843979817 ) ) ;
#27099=CARTESIAN_POINT ( 'NONE',  ( -24.30324774889999873, 1442.429924160389874, 211.8155477906580018 ) ) ;
#27100=CARTESIAN_POINT ( 'NONE',  ( -10.79382126600000014, 1414.913060387329779, 196.1395803457980094 ) ) ;
#27108=CARTESIAN_POINT ( 'NONE',  ( 23.28443042909999861, 1409.830905058029884, 209.4348658987040039 ) ) ;
#27110=CARTESIAN_POINT ( 'NONE',  ( -17.22592475670000312, 1443.501467202829872, 162.9227486557980171 ) ) ;
#27112=CARTESIAN_POINT ( 'NONE',  ( 14.12346818419999828, 1409.573558249629968, 191.9327832110980125 ) ) ;
#27114=CARTESIAN_POINT ( 'NONE',  ( -15.46014185669380758, 1486.078827481694816, 186.6217453166497933 ) ) ;
#27117=CARTESIAN_POINT ( 'NONE',  ( 24.09667836379999883, 1455.346817057629778, 238.1639200605980022 ) ) ;
#27118=CARTESIAN_POINT ( 'NONE',  ( 3.932775080253070321, 1448.980696629100066, 184.2693358254829832 ) ) ;
#27119=CARTESIAN_POINT ( 'NONE',  ( -27.91227906400350278, 1509.887778650499968, 218.1998177527819962 ) ) ;
#27120=CARTESIAN_POINT ( 'NONE',  ( -1.586365103999400006, 1508.858152673860104, 238.2399376808540126 ) ) ;
#27121=CARTESIAN_POINT ( 'NONE',  ( -18.72407526530000155, 1458.246115540929850, 227.3156487912980026 ) ) ;
#27123=CARTESIAN_POINT ( 'NONE',  ( 10.98084429529999895, 1433.016923057050008, 151.7694244727979935 ) ) ;
#27129=CARTESIAN_POINT ( 'NONE',  ( 0.1062812984699999935, 1406.777728848529932, 269.6500679733979950 ) ) ;
#27131=CARTESIAN_POINT ( 'NONE',  ( 3.048828143997139861, 1509.019527812190063, 237.9289388395170306 ) ) ;
#27136=CARTESIAN_POINT ( 'NONE',  ( -37.32042369672969784, 1440.913060388040094, 255.1694497076479990 ) ) ;
#27137=CARTESIAN_POINT ( 'NONE',  ( 36.31051540993509974, 1449.892126659239921, 136.2553180242439907 ) ) ;
#27144=VERTEX_POINT ( 'NONE', #82953 ) ;
#27148=CARTESIAN_POINT ( 'NONE',  ( 11.16572705624736628, 1425.241472595376536, 138.5380445582760842 ) ) ;
#27150=CARTESIAN_POINT ( 'NONE',  ( -27.78452742370000195, 1508.000976255530077, 210.4681928078880162 ) ) ;
#27152=VECTOR ( 'NONE', #86327, 999.9999999999998863 ) ;
#27153=CARTESIAN_POINT ( 'NONE',  ( -17.56720881609999907, 1415.048591087029763, 207.8848073021879941 ) ) ;
#27155=CARTESIAN_POINT ( 'NONE',  ( 11.87064635662919976, 1432.676990320220057, 149.9815557213069894 ) ) ;
#27156=CARTESIAN_POINT ( 'NONE',  ( 26.21858036434699812, 1435.413047757679806, 135.3174467644430194 ) ) ;
#27158=CARTESIAN_POINT ( 'NONE',  ( -6.881200948753640745, 1396.153357219529880, 200.4803135408690196 ) ) ;
#27159=ORIENTED_EDGE ( 'NONE', *, *, #888, .F. ) ;
#27161=CARTESIAN_POINT ( 'NONE',  ( -17.31304841774549885, 1410.598387540080012, 225.8442784478359897 ) ) ;
#27162=CARTESIAN_POINT ( 'NONE',  ( 4.897375497219999652, 1432.353341358199941, 150.0655110971979980 ) ) ;
#27163=ORIENTED_EDGE ( 'NONE', *, *, #83005, .T. ) ;
#27166=CARTESIAN_POINT ( 'NONE',  ( 10.32455812189999911, 1425.433999229330084, 91.15122192769788967 ) ) ;
#27169=CARTESIAN_POINT ( 'NONE',  ( 4.144484579423279413, 1424.490014308070158, 184.8547326364549974 ) ) ;
#27170=CARTESIAN_POINT ( 'NONE',  ( 23.10442899973940101, 1411.095127650270115, 207.3185325528490068 ) ) ;
#27173=CARTESIAN_POINT ( 'NONE',  ( 7.629628877820000099, 1508.993558936030013, 181.6876041027980193 ) ) ;
#27174=CARTESIAN_POINT ( 'NONE',  ( 2.514853015309999940, 1449.255880420389985, 182.8296093962979967 ) ) ;
#27175=EDGE_CURVE ( 'NONE', #94600, #5500, #99927, .T. ) ;
#27178=ORIENTED_EDGE ( 'NONE', *, *, #34408, .F. ) ;
#27180=CARTESIAN_POINT ( 'NONE',  ( -41.49088794730000274, 1443.869659108800079, 136.5795274476980126 ) ) ;
#27182=CARTESIAN_POINT ( 'NONE',  ( -0.9815465312350000193, 1473.584474657329793, 270.3924816079979792 ) ) ;
#27184=CARTESIAN_POINT ( 'NONE',  ( -1.321799804340000106, 1485.974695964230023, 182.1001927673979992 ) ) ;
#27186=CARTESIAN_POINT ( 'NONE',  ( 22.22649075570000221, 1507.849990204029837, 192.4185849886980009 ) ) ;
#27188=CARTESIAN_POINT ( 'NONE',  ( -33.92643721410139790, 1451.728327248950109, 135.1498936377919904 ) ) ;
#27189=CARTESIAN_POINT ( 'NONE',  ( -2.500000000000000000, 1448.224516615570110, 166.8026561098010063 ) ) ;
#27191=CARTESIAN_POINT ( 'NONE',  ( 12.15499524530000031, 1407.709276878430046, 215.7704773373179989 ) ) ;
#27192=CARTESIAN_POINT ( 'NONE',  ( -1.525793978527139938, 1406.001425806299721, 266.9604480841060195 ) ) ;
#27193=CARTESIAN_POINT ( 'NONE',  ( -13.91014378093700010, 1434.990842025300026, 148.7054735720130054 ) ) ;
#27194=ORIENTED_EDGE ( 'NONE', *, *, #103727, .F. ) ;
#27195=PLANE ( 'NONE',  #66120 ) ;
#27196=CARTESIAN_POINT ( 'NONE',  ( 13.41353349150000085, 1442.422659372690077, 188.9779284783980131 ) ) ;
#27198=ORIENTED_EDGE ( 'NONE', *, *, #91975, .F. ) ;
#27210=CARTESIAN_POINT ( 'NONE',  ( -29.24389883310000116, 1509.942753386430013, 204.9097857627180019 ) ) ;
#27215=CARTESIAN_POINT ( 'NONE',  ( -27.41498742912919795, 1488.731319228159919, 208.8198958867089914 ) ) ;
#27216=CARTESIAN_POINT ( 'NONE',  ( -5.934959410920000344, 1445.987167410879920, 183.4479431745980094 ) ) ;
#27221=CARTESIAN_POINT ( 'NONE',  ( -24.68314314579999902, 1435.638739216969952, 137.2594662373980157 ) ) ;
#27226=FACE_OUTER_BOUND ( 'NONE', #104304, .T. ) ;
#27227=CARTESIAN_POINT ( 'NONE',  ( 21.64484447964171920, 1411.027633016495201, 201.9719268724466872 ) ) ;
#27230=DIRECTION ( 'NONE',  ( 0.000000000000000000, 1.000000000000000000, 0.000000000000000000 ) ) ;
#27231=CARTESIAN_POINT ( 'NONE',  ( -10.20816227200000093, 1412.829161712830000, 229.6472676344980073 ) ) ;
#27236=CARTESIAN_POINT ( 'NONE',  ( 11.98752746249999923, 1434.301235679619822, 150.7926998538980001 ) ) ;
#27237=CARTESIAN_POINT ( 'NONE',  ( 18.93888774064880209, 1478.713824472059969, 228.3712757747710214 ) ) ;
#27238=CARTESIAN_POINT ( 'NONE',  ( -21.35051360876400040, 1508.382796155649885, 227.2446047990909790 ) ) ;
#27239=CARTESIAN_POINT ( 'NONE',  ( -2.425152001779999900, 1410.373299902729968, 186.4984030417980136 ) ) ;
#27240=CARTESIAN_POINT ( 'NONE',  ( 0.3258471608539999509, 1410.291732689529908, 233.1866582016979805 ) ) ;
#27241=CARTESIAN_POINT ( 'NONE',  ( 0.1518848447092220055, 1420.467538266630072, 182.7318014650070097 ) ) ;
#27243=CARTESIAN_POINT ( 'NONE',  ( -3.423194496299999834, 1420.340339280129911, 186.2413968210979931 ) ) ;
#27249=ORIENTED_EDGE ( 'NONE', *, *, #61018, .F. ) ;
#27250=CARTESIAN_POINT ( 'NONE',  ( 0.9892016712189999339, 1417.304970919730067, 235.7878985900979956 ) ) ;
#27256=DIRECTION ( 'NONE',  ( -0.9993902469236103370, -0.03489947644258441228, 0.001077449766195770313 ) ) ;
#27257=CARTESIAN_POINT ( 'NONE',  ( -18.75767574410000194, 1425.635095768630208, 226.0811886220980114 ) ) ;
#27258=CARTESIAN_POINT ( 'NONE',  ( -17.30326228670000077, 1435.529124648550123, 147.5648915083980057 ) ) ;
#27259=CARTESIAN_POINT ( 'NONE',  ( -11.89544747750000120, 1434.541746328260160, 147.6465872843980094 ) ) ;
#27262=CARTESIAN_POINT ( 'NONE',  ( -19.05726004021619957, 1440.248441431409674, 209.7973887611863688 ) ) ;
#27265=CARTESIAN_POINT ( 'NONE',  ( 1.554710334620659884, 1415.393085341110009, 190.9507836336619846 ) ) ;
#27266=CARTESIAN_POINT ( 'NONE',  ( 22.77022259470000165, 1411.047177419029822, 206.9289107030080004 ) ) ;
#27267=CARTESIAN_POINT ( 'NONE',  ( -11.93818408299999945, 1433.480074519959999, 149.8972116839979947 ) ) ;
#27268=CARTESIAN_POINT ( 'NONE',  ( 3.015935646565480077, 1410.395869510137345, 185.7231583079203290 ) ) ;
#27269=CARTESIAN_POINT ( 'NONE',  ( -3.975393244031079742, 1426.016855281922062, 186.0738092297652884 ) ) ;
#27270=CARTESIAN_POINT ( 'NONE',  ( -14.17716072747469980, 1509.408135630319975, 183.2983236682360086 ) ) ;
#27277=CARTESIAN_POINT ( 'NONE',  ( -23.55007224577885339, 1410.927093357725198, 210.4721751823504690 ) ) ;
#27279=ORIENTED_EDGE ( 'NONE', *, *, #76917, .T. ) ;
#27280=CARTESIAN_POINT ( 'NONE',  ( -17.96439385675617828, 1459.774127481555070, 228.0505170696288246 ) ) ;
#27286=CARTESIAN_POINT ( 'NONE',  ( 20.01964129088910127, 1509.548583382980041, 230.4035799795959747 ) ) ;
#27291=CARTESIAN_POINT ( 'NONE',  ( -30.10637269909999958, 1468.180606183130067, 266.8104569320979635 ) ) ;
#27294=CARTESIAN_POINT ( 'NONE',  ( 28.51851353229999830, 1509.908948824629988, 203.7504615519080176 ) ) ;
#27295=CARTESIAN_POINT ( 'NONE',  ( -19.94044037020000104, 1485.838040724430130, 190.5384349266980166 ) ) ;
#27296=CARTESIAN_POINT ( 'NONE',  ( 2.896135874330000082, 1409.181763743129977, 186.2668185386979758 ) ) ;
#27297=CARTESIAN_POINT ( 'NONE',  ( 5.855088903640000453, 1423.239027948129888, 186.0981068077980183 ) ) ;
#27298=CARTESIAN_POINT ( 'NONE',  ( -5.630091727850000005, 1441.487383650409811, 154.7801822665980183 ) ) ;
#27299=CARTESIAN_POINT ( 'NONE',  ( 12.15187854179999860, 1435.108173852649770, 151.0159323405979990 ) ) ;
#27302=CARTESIAN_POINT ( 'NONE',  ( -15.94347048536829803, 1409.469818645040050, 192.9752432267480060 ) ) ;
#27306=CARTESIAN_POINT ( 'NONE',  ( -43.12011480509999473, 1450.389500078439823, 269.9366955693979548 ) ) ;
#27307=CARTESIAN_POINT ( 'NONE',  ( -27.27137786365319982, 1446.453610550540134, 137.2094999256019889 ) ) ;
#27308=CARTESIAN_POINT ( 'NONE',  ( 17.60618138139999900, 1410.892634160230045, 223.9222036297979912 ) ) ;
#27309=CARTESIAN_POINT ( 'NONE',  ( -15.13234893939999992, 1485.042171593129979, 224.0148604844980014 ) ) ;
#27310=CARTESIAN_POINT ( 'NONE',  ( 5.164876290100000489, 1519.913060387329779, 186.3413721456980170 ) ) ;
#27311=CARTESIAN_POINT ( 'NONE',  ( -13.58235846979999906, 1416.828040475229955, 221.9087530951979659 ) ) ;
#27313=CARTESIAN_POINT ( 'NONE',  ( -3.076054745830000048, 1415.755548294329856, 232.7548256247980021 ) ) ;
#27316=CARTESIAN_POINT ( 'NONE',  ( -45.75888640774939375, 1437.122255822999932, 268.5047239448639971 ) ) ;
#27317=DIRECTION ( 'NONE',  ( 1.000000000000000000, 0.000000000000000000, 0.000000000000000000 ) ) ;
#27322=CARTESIAN_POINT ( 'NONE',  ( 19.44117294853580091, 1456.941945407359981, 224.4539793896520052 ) ) ;
#27323=CARTESIAN_POINT ( 'NONE',  ( -11.00204100220000036, 1410.396409030930045, 188.8227745368980379 ) ) ;
#27326=CARTESIAN_POINT ( 'NONE',  ( -15.03597275369999942, 1488.809466528929988, 194.0187079571979893 ) ) ;
#27328=CARTESIAN_POINT ( 'NONE',  ( 14.40805950830000093, 1470.815019615529991, 194.5894316583980128 ) ) ;
#27334=CARTESIAN_POINT ( 'NONE',  ( -3.114907484115349678, 1408.000211163370068, 270.2910159990690317 ) ) ;
#27336=CARTESIAN_POINT ( 'NONE',  ( 4.187645461488620491, 1418.024921168729861, 233.4325071608510029 ) ) ;
#27337=CARTESIAN_POINT ( 'NONE',  ( -0.3886416839960190606, 1508.683136490621791, 238.1396719883204298 ) ) ;
#27340=ORIENTED_EDGE ( 'NONE', *, *, #5020, .T. ) ;
#27342=CARTESIAN_POINT ( 'NONE',  ( -3.956504371649999463, 1424.255369803030135, 185.4171806679979966 ) ) ;
#27343=CARTESIAN_POINT ( 'NONE',  ( 3.690176726703637389, 1424.194312783380838, 183.9655579347969478 ) ) ;
#27346=CARTESIAN_POINT ( 'NONE',  ( -17.99954540876850118, 1410.904693920620048, 195.2564682659330231 ) ) ;
#27347=CARTESIAN_POINT ( 'NONE',  ( -18.31548309940000152, 1420.838217743430050, 225.0570179786980134 ) ) ;
#27348=CARTESIAN_POINT ( 'NONE',  ( 32.87669591961419968, 1465.269253061860127, 266.5396782138440130 ) ) ;
#27350=CARTESIAN_POINT ( 'NONE',  ( -7.438002979262030578, 1465.685359695273746, 233.5328670419079344 ) ) ;
#27351=CARTESIAN_POINT ( 'NONE',  ( 7.201451958809999887, 1447.808573296560098, 185.4041577039979813 ) ) ;
#27354=CARTESIAN_POINT ( 'NONE',  ( 21.73282879226712083, 1411.032371074868252, 216.6638630078411438 ) ) ;
#27356=CARTESIAN_POINT ( 'NONE',  ( 23.65254864839999982, 1410.841227188329867, 207.9071628193579784 ) ) ;
#27357=ORIENTED_EDGE ( 'NONE', *, *, #79156, .T. ) ;
#27360=CARTESIAN_POINT ( 'NONE',  ( 24.93611935033429816, 1452.026605045649831, 135.8540817300889785 ) ) ;
#27362=CARTESIAN_POINT ( 'NONE',  ( 11.87563352516160009, 1433.006677200080048, 147.6591433499779953 ) ) ;
#27365=CARTESIAN_POINT ( 'NONE',  ( 17.38484768960000082, 1410.884447801129909, 192.4603983160980079 ) ) ;
#27367=CARTESIAN_POINT ( 'NONE',  ( 3.280909904081581008, 1439.687164527259256, 184.3576248092443848 ) ) ;
#27368=CARTESIAN_POINT ( 'NONE',  ( -0.01332681072910000056, 1417.281753988030005, 234.8503422950979882 ) ) ;
#27369=CARTESIAN_POINT ( 'NONE',  ( -19.08455381886165014, 1425.050945183270869, 224.0897855658817832 ) ) ;
#27370=CARTESIAN_POINT ( 'NONE',  ( 0.7437212546499240018, 1452.305686085940124, 183.2916024963490145 ) ) ;
#27375=VERTEX_POINT ( 'NONE', #76761 ) ;
#27377=B_SPLINE_SURFACE_WITH_KNOTS ( 'NONE', 5, 5, ( 
 ( #42394, #92799, #85482, #101736, #83300, #93891 ),
 ( #25024, #50805, #42963, #110704, #33996, #102293 ),
 ( #40744, #17157, #429, #34548, #74920, #32352 ),
 ( #49716, #66531, #100635, #95015, #26692, #54143 ),
 ( #94436, #61994, #96678, #77662, #104515, #19950 ),
 ( #36763, #103959, #11013, #78206, #87735, #28361 ),
 ( #53589, #60318, #69841, #26129, #35099, #96112 ),
 ( #87164, #44627, #45184, #18833, #1518, #17715 ),
 ( #62558, #95563, #35651, #44067, #36212, #88272 ) ),
 .UNSPECIFIED., .F., .F., .F.,
 ( 6, 3, 6 ),
 ( 6, 6 ),
 ( 0.7655572723410000169, 2.316155491860000026, 3.835724788519999873 ),
 ( 0.000000000000000000, 1.000000000000000000 ),
 .UNSPECIFIED. ) ;
#27379=CARTESIAN_POINT ( 'NONE',  ( -0.5153922977329320476, 1410.146051047059700, 233.1556763689120260 ) ) ;
#27381=CARTESIAN_POINT ( 'NONE',  ( -34.50882828746139808, 1450.391922407039829, 136.2327768001300115 ) ) ;
#27382=CARTESIAN_POINT ( 'NONE',  ( -0.1909393205278206718, 1506.691119452750399, 231.3199018796742337 ) ) ;
#27383=B_SPLINE_CURVE_WITH_KNOTS ( 'NONE', 3,
 ( #41714, #84263, #84803, #62273, #59633, #7560, #25440, #42269, #8102, #10182 ),
 .UNSPECIFIED., .F., .F.,
 ( 4, 2, 2, 2, 4 ),
 ( 0.000000000000000000, 0.02214642915447170152, 0.06470200879455109688, 0.1010821742375619947, 0.1380341206303599966 ),
 .UNSPECIFIED. ) ;
#27384=CARTESIAN_POINT ( 'NONE',  ( -6.215408291060000145, 1454.402584563930077, 214.3676144191779827 ) ) ;
#27385=CARTESIAN_POINT ( 'NONE',  ( 35.50739915879996289, 1462.949854392428279, 266.4727958076973664 ) ) ;
#27386=CARTESIAN_POINT ( 'NONE',  ( 11.87502391619999997, 1433.007272034859852, 149.9804603544980068 ) ) ;
#27387=CARTESIAN_POINT ( 'NONE',  ( 18.41412373400000035, 1444.997163189090088, 209.1218459616979999 ) ) ;
#27392=CARTESIAN_POINT ( 'NONE',  ( 22.71938917269999791, 1409.706427035829847, 209.1785880919549925 ) ) ;
#27393=CARTESIAN_POINT ( 'NONE',  ( -30.02739323485179668, 1510.039195650590045, 211.8782729601720121 ) ) ;
#27394=CARTESIAN_POINT ( 'NONE',  ( 25.48925201540000174, 1449.802587353020044, 210.7369667112079981 ) ) ;
#27396=CARTESIAN_POINT ( 'NONE',  ( -40.27308906366239682, 1443.612067134240078, 137.1163379626329970 ) ) ;
#27401=CARTESIAN_POINT ( 'NONE',  ( 0.1676281277942339998, 1481.725157098900127, 182.0202826403800032 ) ) ;
#27402=FACE_OUTER_BOUND ( 'NONE', #38074, .T. ) ;
#27408=CARTESIAN_POINT ( 'NONE',  ( -37.29624469558390132, 1450.849357696489960, 134.0999999986649698 ) ) ;
#27413=CARTESIAN_POINT ( 'NONE',  ( -16.63199885160000235, 1416.518938592030054, 216.8695166334780140 ) ) ;
#27418=CARTESIAN_POINT ( 'NONE',  ( 14.58630151190530100, 1409.422425260170030, 205.9107706399979918 ) ) ;
#27421=CARTESIAN_POINT ( 'NONE',  ( -17.00586071620000084, 1421.470251449630041, 191.4405153155979917 ) ) ;
#27423=ORIENTED_EDGE ( 'NONE', *, *, #82010, .F. ) ;
#27426=EDGE_LOOP ( 'NONE', ( #38880, #47588, #51708, #81729 ) ) ;
#27429=CARTESIAN_POINT ( 'NONE',  ( 22.39346815460000428, 1508.437849850330167, 224.3979271850979842 ) ) ;
#27433=CARTESIAN_POINT ( 'NONE',  ( 29.83189240543555698, 1462.372292350401267, 269.4690225947026647 ) ) ;
#27435=CARTESIAN_POINT ( 'NONE',  ( -0.001991323853590000036, 1395.912990848829850, 220.4358217571979992 ) ) ;
#27437=CARTESIAN_POINT ( 'NONE',  ( 22.28696231330000188, 1506.798305107829947, 209.3970118511340104 ) ) ;
#27438=CARTESIAN_POINT ( 'NONE',  ( -1.452061816759999902, 1467.474562141730075, 183.2045861867980250 ) ) ;
#27441=CARTESIAN_POINT ( 'NONE',  ( 10.81507089421240053, 1424.921187596799882, 144.1620444706739761 ) ) ;
#27445=FACE_OUTER_BOUND ( 'NONE', #23945, .T. ) ;
#27446=CARTESIAN_POINT ( 'NONE',  ( 6.721801505100000185, 1474.175172799430129, 270.1377427386980230 ) ) ;
#27448=ORIENTED_EDGE ( 'NONE', *, *, #67347, .T. ) ;
#27449=CARTESIAN_POINT ( 'NONE',  ( 40.49318544340329851, 1444.190211223800134, 137.0748560406749732 ) ) ;
#27451=CARTESIAN_POINT ( 'NONE',  ( 9.989727630039999957E-09, 1407.100401496229779, 264.8986986722979964 ) ) ;
#27452=CARTESIAN_POINT ( 'NONE',  ( -27.42581371189999828, 1488.692458008330050, 208.8841174044290199 ) ) ;
#27453=CARTESIAN_POINT ( 'NONE',  ( -1.545285848170000031, 1504.644139859730103, 180.9077348290979899 ) ) ;
#27454=CARTESIAN_POINT ( 'NONE',  ( 16.52699712982959923, 1409.590692121840220, 192.7142616149739922 ) ) ;
#27457=CARTESIAN_POINT ( 'NONE',  ( -29.66529950410000183, 1430.834809504130135, 244.2516413604979846 ) ) ;
#27459=CARTESIAN_POINT ( 'NONE',  ( 28.86205551402650116, 1509.507027960610003, 209.5284224540439766 ) ) ;
#27461=CARTESIAN_POINT ( 'NONE',  ( 30.82338973599999932, 1451.683219239730079, 135.6778805674979935 ) ) ;
#27463=CARTESIAN_POINT ( 'NONE',  ( 8.020322465218489683, 1396.252981828660040, 218.0167330499769776 ) ) ;
#27465=CARTESIAN_POINT ( 'NONE',  ( -17.14944014479999979, 1460.897692083130096, 228.2718297098980145 ) ) ;
#27467=ORIENTED_EDGE ( 'NONE', *, *, #50775, .F. ) ;
#27471=CARTESIAN_POINT ( 'NONE',  ( 0.09171298916310000049, 1419.319896810129876, 184.5979190233979921 ) ) ;
#27473=LINE ( 'NONE', #61663, #67255 ) ;
#27474=CARTESIAN_POINT ( 'NONE',  ( -1.739071167590000133, 1461.196621557430035, 235.0776999716979958 ) ) ;
#27480=CARTESIAN_POINT ( 'NONE',  ( 15.20160463690000086, 1496.666401959530049, 225.6166776728979642 ) ) ;
#27481=EDGE_LOOP ( 'NONE', ( #48088, #86146, #8448, #25432 ) ) ;
#27482=( BOUNDED_CURVE ( )  B_SPLINE_CURVE ( 3, ( #22848, #48653, #15001, #32383 ),
 .UNSPECIFIED., .F., .T. ) 
 B_SPLINE_CURVE_WITH_KNOTS ( ( 4, 4 ),
 ( 4.177898496904434822, 5.246901655145340015 ),
 .UNSPECIFIED. ) 
 CURVE ( )  GEOMETRIC_REPRESENTATION_ITEM ( )  RATIONAL_B_SPLINE_CURVE ( ( 1.000000000000000000, 0.9070150918854136268, 0.9070150918854136268, 1.000000000000000000 ) ) 
 REPRESENTATION_ITEM ( '' )  );
#27486=CARTESIAN_POINT ( 'NONE',  ( 11.86328075526730075, 1432.138978093059904, 149.9787975337250145 ) ) ;
#27488=CARTESIAN_POINT ( 'NONE',  ( 12.66538237952104673, 1445.025812281660365, 186.3114105575668304 ) ) ;
#27489=EDGE_LOOP ( 'NONE', ( #57202, #7238, #4622, #82710 ) ) ;
#27490=CARTESIAN_POINT ( 'NONE',  ( -15.81201443571409904, 1506.433683733589987, 193.8503163142329981 ) ) ;
#27491=ADVANCED_FACE ( 'NONE', ( #45390 ), #16179, .T. ) ;
#27492=CARTESIAN_POINT ( 'NONE',  ( -17.22623662315568893, 1443.913060387331598, 162.9225832754749490 ) ) ;
#27493=CARTESIAN_POINT ( 'NONE',  ( 6.918620528049999940, 1507.562034369630055, 235.3523762123979850 ) ) ;
#27496=CARTESIAN_POINT ( 'NONE',  ( -5.866240475749999739, 1421.246203026429839, 186.6777796954980033 ) ) ;
#27497=CARTESIAN_POINT ( 'NONE',  ( 2.303607911415140208, 1408.601389339190064, 270.4285322758109942 ) ) ;
#27498=CARTESIAN_POINT ( 'NONE',  ( -9.380124768717641004, 1428.163396101657781, 137.0999999980979851 ) ) ;
#27503=EDGE_CURVE ( 'NONE', #98841, #4207, #19599, .T. ) ;
#27505=CARTESIAN_POINT ( 'NONE',  ( 14.00912961620000097, 1416.839648768830102, 196.3913569366980028 ) ) ;
#27506=CARTESIAN_POINT ( 'NONE',  ( -4.833007409577117386, 1423.506200470894100, 184.6062591623307583 ) ) ;
#27507=CARTESIAN_POINT ( 'NONE',  ( 18.02093535799999913, 1424.326836137830014, 225.1991050518980160 ) ) ;
#27508=CARTESIAN_POINT ( 'NONE',  ( -1.268034562940015375, 1506.397833124954104, 187.1879512861502235 ) ) ;
#27510=CARTESIAN_POINT ( 'NONE',  ( 4.540901342749999792, 1419.211677879630088, 248.0989693021979861 ) ) ;
#27521=CARTESIAN_POINT ( 'NONE',  ( -15.57943187099139948, 1507.275789587220061, 192.6267346305599801 ) ) ;
#27522=CARTESIAN_POINT ( 'NONE',  ( -1.746205394668796762, 1450.465189299475924, 154.2919931100517772 ) ) ;
#27524=DIRECTION ( 'NONE',  ( 0.000000000000000000, 0.000000000000000000, -1.000000000000000000 ) ) ;
#27525=CARTESIAN_POINT ( 'NONE',  ( -8.970685674490001205, 1442.046922168800165, 185.8306878991980113 ) ) ;
#27526=ADVANCED_FACE ( 'NONE', ( #44705 ), #95089, .F. ) ;
#27530=CARTESIAN_POINT ( 'NONE',  ( -10.60236678890000128, 1431.113060387329824, 224.6557647168980338 ) ) ;
#27531=ADVANCED_FACE ( 'NONE', ( #72521 ), #77952, .F. ) ;
#27532=CARTESIAN_POINT ( 'NONE',  ( 15.72821513129999893, 1415.087486802329977, 227.2801319970979819 ) ) ;
#27534=CARTESIAN_POINT ( 'NONE',  ( -15.91456197569999986, 1459.203849340630086, 230.3656326198979798 ) ) ;
#27536=CARTESIAN_POINT ( 'NONE',  ( 46.02999043379999478, 1438.908956426789928, 268.4959127839979942 ) ) ;
#27540=CARTESIAN_POINT ( 'NONE',  ( 20.26569827480000185, 1469.158149366930047, 192.4428757755979973 ) ) ;
#27541=CARTESIAN_POINT ( 'NONE',  ( -22.09796275270000265, 1430.768449482030064, 219.6318221129980088 ) ) ;
#27544=CARTESIAN_POINT ( 'NONE',  ( -16.49693783299999694, 1410.833576558129835, 226.6232151731979911 ) ) ;
#27546=CARTESIAN_POINT ( 'NONE',  ( 20.61224126549999980, 1508.367040378830097, 227.7934948748979878 ) ) ;
#27547=CARTESIAN_POINT ( 'NONE',  ( -11.73709356400000026, 1426.695943141129874, 144.1748013759980154 ) ) ;
#27548=CARTESIAN_POINT ( 'NONE',  ( -17.27338612379999816, 1414.913060387329779, 208.0459408281480194 ) ) ;
#27549=CARTESIAN_POINT ( 'NONE',  ( -12.67591333549999888, 1442.786765023099861, 186.5187981297980002 ) ) ;
#27551=CARTESIAN_POINT ( 'NONE',  ( -29.16176511740000166, 1436.844852152720023, 136.7082758069980173 ) ) ;
#27553=DIRECTION ( 'NONE',  ( -0.3363363969979658030, -0.9417419115949056119, 0.000000000000000000 ) ) ;
#27554=CARTESIAN_POINT ( 'NONE',  ( -14.89215741792830094, 1409.433105983750011, 210.1887096901859877 ) ) ;
#27557=CARTESIAN_POINT ( 'NONE',  ( -46.15245045410000557, 1446.051659328119968, 268.2044218355979979 ) ) ;
#27559=CARTESIAN_POINT ( 'NONE',  ( 0.4382968505613619725, 1418.849865278630205, 184.6907702969609772 ) ) ;
#27560=CARTESIAN_POINT ( 'NONE',  ( -26.20833356250000179, 1507.984236983630126, 216.2555649815679999 ) ) ;
#27563=CARTESIAN_POINT ( 'NONE',  ( 17.47926118081009861, 1422.862077572759972, 226.4946375912610108 ) ) ;
#27564=CARTESIAN_POINT ( 'NONE',  ( 12.85971948620000127, 1415.932840167130053, 221.4945874069979936 ) ) ;
#27565=CARTESIAN_POINT ( 'NONE',  ( -6.464994551020000202, 1433.443311356699951, 154.6859263780980029 ) ) ;
#27568=CARTESIAN_POINT ( 'NONE',  ( 12.94448954231351223, 1512.413060387330006, 232.8165751327380519 ) ) ;
#27570=CARTESIAN_POINT ( 'NONE',  ( -22.64306613040000116, 1409.703773680230142, 208.6811978374589955 ) ) ;
#27571=EDGE_CURVE ( 'NONE', #88339, #92672, #70418, .T. ) ;
#27573=CARTESIAN_POINT ( 'NONE',  ( -12.60885230210000074, 1416.021639796329964, 195.3971703157980073 ) ) ;
#27577=CARTESIAN_POINT ( 'NONE',  ( -15.52168021169999967, 1422.715911009230012, 228.7996066201980057 ) ) ;
#27580=CARTESIAN_POINT ( 'NONE',  ( 1.361885589129999907, 1414.404335136930058, 232.8121858128980080 ) ) ;
#27583=CARTESIAN_POINT ( 'NONE',  ( -22.77022140789999938, 1411.047177455729752, 211.3147823620780059 ) ) ;
#27589=CARTESIAN_POINT ( 'NONE',  ( -18.38404635505749951, 1485.653075037670078, 189.0955620534189734 ) ) ;
#27590=CARTESIAN_POINT ( 'NONE',  ( 1.559371654100000004, 1508.275840731030030, 237.0359025730980136 ) ) ;
#27592=CARTESIAN_POINT ( 'NONE',  ( 40.93861322897850386, 1447.346027417549976, 135.6170675654770150 ) ) ;
#27597=CARTESIAN_POINT ( 'NONE',  ( 11.32737736758029889, 1433.997803480599941, 151.5041286862229981 ) ) ;
#27599=ORIENTED_EDGE ( 'NONE', *, *, #103398, .F. ) ;
#27602=LINE ( 'NONE', #52277, #51481 ) ;
#27603=CARTESIAN_POINT ( 'NONE',  ( -0.1593348516950000016, 1508.131906080129966, 180.6917150519979884 ) ) ;
#27604=CARTESIAN_POINT ( 'NONE',  ( -4.500000000000000000, 1425.929641636930000, 172.2701767054979882 ) ) ;
#27607=CARTESIAN_POINT ( 'NONE',  ( -23.99770110361529873, 1452.069770166940089, 137.0532919795800240 ) ) ;
#27609=CARTESIAN_POINT ( 'NONE',  ( -24.04659120089169733, 1444.796772349889807, 212.0316830080810178 ) ) ;
#27612=CARTESIAN_POINT ( 'NONE',  ( 14.25441464932749902, 1415.890045859410066, 197.0605362263979998 ) ) ;
#27616=CARTESIAN_POINT ( 'NONE',  ( 14.31101212421439861, 1435.533114237510063, 149.6577325083550249 ) ) ;
#27618=ORIENTED_EDGE ( 'NONE', *, *, #82371, .F. ) ;
#27619=ORIENTED_EDGE ( 'NONE', *, *, #35804, .F. ) ;
#27621=CARTESIAN_POINT ( 'NONE',  ( 12.54683115582590780, 1445.050387922648497, 169.4738476292419023 ) ) ;
#27622=CARTESIAN_POINT ( 'NONE',  ( -0.9888054234880000459, 1464.981437416829976, 237.6389206865979986 ) ) ;
#27623=CARTESIAN_POINT ( 'NONE',  ( 16.24128197971020526, 1451.109843354380473, 148.8744789175986512 ) ) ;
#27626=CARTESIAN_POINT ( 'NONE',  ( -18.98973562068158927, 1443.333582277293317, 211.5879291524545351 ) ) ;
#27629=EDGE_CURVE ( 'NONE', #62097, #86845, #86421, .T. ) ;
#27634=CARTESIAN_POINT ( 'NONE',  ( 33.19045541928569776, 1440.913060387330006, 258.0029463747879959 ) ) ;
#27637=VERTEX_POINT ( 'NONE', #85300 ) ;
#27638=CARTESIAN_POINT ( 'NONE',  ( 27.28304656200170086, 1449.116014730419920, 136.7093938965389839 ) ) ;
#27639=CARTESIAN_POINT ( 'NONE',  ( -14.04862573770000012, 1409.570344837929952, 190.8576452217980091 ) ) ;
#27641=CARTESIAN_POINT ( 'NONE',  ( -24.40934708730000224, 1441.356666723849912, 212.0571328731979861 ) ) ;
#27642=CARTESIAN_POINT ( 'NONE',  ( -11.30241272439999989, 1414.983771848829747, 195.8621715482979937 ) ) ;
#27644=CARTESIAN_POINT ( 'NONE',  ( -12.17346841087018561, 1434.039807595294860, 147.4869002435401342 ) ) ;
#27646=CARTESIAN_POINT ( 'NONE',  ( 22.15911651489999912, 1435.271885453649929, 140.1193622846980134 ) ) ;
#27647=EDGE_CURVE ( 'NONE', #83462, #27055, #29447, .T. ) ;
#27648=CARTESIAN_POINT ( 'NONE',  ( 7.934445985219999109, 1465.591001358030098, 233.1255853796979807 ) ) ;
#27650=B_SPLINE_SURFACE_WITH_KNOTS ( 'NONE', 4, 5, ( 
 ( #55142, #98207, #106068, #88725, #30454, #29348, #47266, #13081, #21476 ),
 ( #55687, #38298, #81389, #4702, #97663, #73023, #12557, #64638, #98758 ),
 ( #89261, #87624, #64086, #10912, #45087, #19843, #71957, #3638, #12008 ),
 ( #46737, #80869, #46188, #88174, #11466, #37213, #80319, #79227, #2536 ),
 ( #70854, #104964, #20936, #28254, #37766, #62446, #96570, #63548, #45641 ),
 ( #79781, #3086, #71409, #105525, #28814, #63012, #31001, #48380, #81950 ),
 ( #109385, #39410, #108816, #47815, #48937, #41056, #66298, #99293, #82523 ),
 ( #84157, #74684, #75235, #5820, #83603, #65181, #7458, #32111, #32662 ),
 ( #6901, #83067, #22567, #66839, #100949, #24244, #92553, #92017, #15287 ) ),
 .UNSPECIFIED., .F., .F., .F.,
 ( 5, 4, 5 ),
 ( 6, 3, 6 ),
 ( 52.85187863200000180, 54.35145002560000194, 54.36644573953599746 ),
 ( 0.000000000000000000, 1.000000000000000000, 2.000000000000000000 ),
 .UNSPECIFIED. ) ;
#27653=CARTESIAN_POINT ( 'NONE',  ( -14.43289921072090110, 1509.539432542180066, 182.8218189571549885 ) ) ;
#27662=CARTESIAN_POINT ( 'NONE',  ( 26.47164861350000109, 1444.397189212120111, 225.7812066110980140 ) ) ;
#27665=CARTESIAN_POINT ( 'NONE',  ( -6.986089899625779864, 1508.628476212760006, 236.2437696408319994 ) ) ;
#27667=CARTESIAN_POINT ( 'NONE',  ( -20.50175529719999901, 1455.144460757629986, 224.2427973570979702 ) ) ;
#27669=DIRECTION ( 'NONE',  ( 0.009162716345344929306, -0.1630249886365709999, -0.9865793925018000454 ) ) ;
#27670=CARTESIAN_POINT ( 'NONE',  ( 19.02805368359999960, 1456.948220378029873, 225.7924841714979891 ) ) ;
#27671=CARTESIAN_POINT ( 'NONE',  ( 0.04654594267750000042, 1452.815214894130122, 189.3840791623979953 ) ) ;
#27675=CARTESIAN_POINT ( 'NONE',  ( 5.565001792720000664E-10, 1406.264975254330011, 269.2947192204980524 ) ) ;
#27676=AXIS2_PLACEMENT_3D ( 'NONE', #11408, #36594, #37697 ) ;
#27678=CARTESIAN_POINT ( 'NONE',  ( 28.59841868990000080, 1509.911739173930073, 206.6816370787080075 ) ) ;
#27680=CARTESIAN_POINT ( 'NONE',  ( 19.45506404997480132, 1470.566269694860011, 270.3921699878309823 ) ) ;
#27681=CARTESIAN_POINT ( 'NONE',  ( 2.478483860230000335, 1437.758671269130218, 157.6934240700980183 ) ) ;
#27684=CARTESIAN_POINT ( 'NONE',  ( -41.50287196043939986, 1440.913060410020080, 261.3196605011079896 ) ) ;
#27685=CARTESIAN_POINT ( 'NONE',  ( 34.28525901495920181, 1450.415853699829995, 136.2365631467760068 ) ) ;
#27686=CARTESIAN_POINT ( 'NONE',  ( 2.235474299570370693, 1449.899086179656706, 154.3826606052703028 ) ) ;
#27688=CARTESIAN_POINT ( 'NONE',  ( 0.8724913224786620125, 1450.882592301979912, 154.2430449183819690 ) ) ;
#27691=ORIENTED_EDGE ( 'NONE', *, *, #100925, .T. ) ;
#27692=CARTESIAN_POINT ( 'NONE',  ( 2.500000726750000180, 1448.905931065010009, 182.6097889574979831 ) ) ;
#27695=CARTESIAN_POINT ( 'NONE',  ( -0.1080245130140000120, 1476.050155969029902, 268.4837719563980158 ) ) ;
#27702=CARTESIAN_POINT ( 'NONE',  ( 26.81196021308459621, 1435.986317847600048, 136.4844220934189991 ) ) ;
#27704=CARTESIAN_POINT ( 'NONE',  ( -13.51610093809999924, 1443.913060387330006, 169.3501091259980171 ) ) ;
#27705=CARTESIAN_POINT ( 'NONE',  ( -17.38130034684149905, 1410.742361519390215, 225.7780215077559944 ) ) ;
#27706=CARTESIAN_POINT ( 'NONE',  ( 11.91321771470000002, 1435.943783413959864, 147.6429393588979906 ) ) ;
#27708=CARTESIAN_POINT ( 'NONE',  ( 41.65675406397859604, 1443.992462633329978, 135.6790809494980010 ) ) ;
#27710=CIRCLE ( 'NONE', #42019, 0.5000000000000000000 ) ;
#27712=DIRECTION ( 'NONE',  ( 0.000000000000000000, -0.7071067811865475727, -0.7071067811865475727 ) ) ;
#27720=CARTESIAN_POINT ( 'NONE',  ( -11.87502393677010026, 1433.007271224430042, 149.9804568710339936 ) ) ;
#27725=ORIENTED_EDGE ( 'NONE', *, *, #15607, .T. ) ;
#27727=CARTESIAN_POINT ( 'NONE',  ( -41.66146602930000142, 1443.809371001679892, 136.1342613200980054 ) ) ;
#27728=CARTESIAN_POINT ( 'NONE',  ( 0.4231130519409999624, 1466.688341884629835, 235.6370719615979965 ) ) ;
#27729=CARTESIAN_POINT ( 'NONE',  ( -0.9761296588700000276, 1473.260042257729992, 270.4290152423980089 ) ) ;
#27733=CARTESIAN_POINT ( 'NONE',  ( -36.07230721274900276, 1450.585147499210052, 136.1439704596049864 ) ) ;
#27734=CARTESIAN_POINT ( 'NONE',  ( 33.92724067235770491, 1436.576420800989808, 136.5094946137080001 ) ) ;
#27735=CARTESIAN_POINT ( 'NONE',  ( 9.919156197434499944, 1396.259444956319840, 214.0198213256190058 ) ) ;
#27736=CARTESIAN_POINT ( 'NONE',  ( -0.02192818798958470067, 1407.539782041390026, 196.0601747775820058 ) ) ;
#27737=CARTESIAN_POINT ( 'NONE',  ( -14.26333330936780008, 1452.396687514240057, 223.0069981058830137 ) ) ;
#27738=CARTESIAN_POINT ( 'NONE',  ( -14.31417139289039930, 1435.588016961450194, 149.7074577630269800 ) ) ;
#27741=CARTESIAN_POINT ( 'NONE',  ( 12.88115801269999849, 1441.996360158710104, 188.6196260033980252 ) ) ;
#27743=ORIENTED_EDGE ( 'NONE', *, *, #83400, .F. ) ;
#27755=CARTESIAN_POINT ( 'NONE',  ( -26.42714720800000094, 1440.913060387330006, 243.9198229517980110 ) ) ;
#27757=B_SPLINE_SURFACE_WITH_KNOTS ( 'NONE', 5, 5, ( 
 ( #102326, #26733, #51951, #34582, #79360, #86638 ),
 ( #59804, #42998, #53063, #69877, #96148, #45222 ),
 ( #93924, #86093, #104551, #87200, #10492, #70433 ),
 ( #103992, #34030, #78241, #9387, #460, #87770 ),
 ( #35136, #69317, #62028, #102870, #85519, #44663 ),
 ( #77156, #68221, #11051, #17191, #43550, #1554 ) ),
 .UNSPECIFIED., .F., .F., .F.,
 ( 6, 6 ),
 ( 6, 6 ),
 ( 30.32814665560000122, 157.7108139880000124 ),
 ( -6.245004513519998715E-17, 1.000000000000000000 ),
 .UNSPECIFIED. ) ;
#27758=CARTESIAN_POINT ( 'NONE',  ( -1.324026618839999836, 1487.751343670030110, 231.2068259027980162 ) ) ;
#27759=CARTESIAN_POINT ( 'NONE',  ( -41.99751584039131558, 1438.963961567131264, 269.6474901557800763 ) ) ;
#27761=CARTESIAN_POINT ( 'NONE',  ( -4.481884685280000724, 1410.004874574130099, 232.0320561794979994 ) ) ;
#27762=B_SPLINE_CURVE_WITH_KNOTS ( 'NONE', 3,
 ( #11213, #104700, #2280, #103028, #27995, #1162, #27437 ),
 .UNSPECIFIED., .F., .F.,
 ( 4, 3, 4 ),
 ( -157.6565403119999758, -100.4036150152009981, -30.32814665559999412 ),
 .UNSPECIFIED. ) ;
#27763=CARTESIAN_POINT ( 'NONE',  ( -10.50159781620000210, 1445.883858324350058, 186.3320361473979858 ) ) ;
#27764=VERTEX_POINT ( 'NONE', #28174 ) ;
#27765=CARTESIAN_POINT ( 'NONE',  ( -24.58745215098610259, 1440.913060451950059, 213.2928209972399998 ) ) ;
#27766=CARTESIAN_POINT ( 'NONE',  ( 20.86442530855919841, 1507.787512642029924, 226.2753960300409801 ) ) ;
#27768=CARTESIAN_POINT ( 'NONE',  ( -24.55864424809999846, 1435.538845322140105, 137.1712378357980242 ) ) ;
#27771=EDGE_CURVE ( 'NONE', #104164, #5427, #32878, .T. ) ;
#27772=CARTESIAN_POINT ( 'NONE',  ( -7.911281457743720935, 1425.821179498857646, 225.8045002088393289 ) ) ;
#27775=CARTESIAN_POINT ( 'NONE',  ( 19.30007074693602576, 1410.948536389271567, 195.8605864048363117 ) ) ;
#27778=CARTESIAN_POINT ( 'NONE',  ( 2.500000000000000000, 1433.496992208500160, 157.5291644476980082 ) ) ;
#27781=VERTEX_POINT ( 'NONE', #10833 ) ;
#27784=CARTESIAN_POINT ( 'NONE',  ( 12.46581826982980168, 1434.413684206549988, 149.6162948891119981 ) ) ;
#27785=CARTESIAN_POINT ( 'NONE',  ( 13.86236365335560095, 1469.002559954369872, 230.9511697035910061 ) ) ;
#27786=CIRCLE ( 'NONE', #90353, 451.3444983786160947 ) ;
#27787=CARTESIAN_POINT ( 'NONE',  ( -25.78157324093470137, 1509.813372837629913, 223.1298088449100021 ) ) ;
#27788=CARTESIAN_POINT ( 'NONE',  ( -2.073863249510000006, 1408.985481286630147, 187.4413895757980129 ) ) ;
#27789=CARTESIAN_POINT ( 'NONE',  ( -0.1681250064260000066, 1408.918931400830161, 232.2238576234980201 ) ) ;
#27790=CARTESIAN_POINT ( 'NONE',  ( 0.09356662494084540260, 1420.452715721949971, 182.6929833556150129 ) ) ;
#27791=B_SPLINE_CURVE_WITH_KNOTS ( 'NONE', 5,
 ( #84784, #74221, #110552, #108350, #75319, #101029, #65811, #15373, #14273 ),
 .UNSPECIFIED., .F., .F.,
 ( 6, 3, 6 ),
 ( 2.234462700939999991, 2.575722133019999749, 3.155688525630194974 ),
 .UNSPECIFIED. ) ;
#27793=CARTESIAN_POINT ( 'NONE',  ( -2.727274045799999769, 1420.080670998130017, 186.1515345996979818 ) ) ;
#27800=CARTESIAN_POINT ( 'NONE',  ( -6.150877690909999806, 1490.513422154930140, 181.6085158044980119 ) ) ;
#27804=CARTESIAN_POINT ( 'NONE',  ( 9.609510489164891922, 1436.202073637698732, 152.7520764886153870 ) ) ;
#27805=EDGE_CURVE ( 'NONE', #96903, #109412, #40249, .T. ) ;
#27807=B_SPLINE_CURVE_WITH_KNOTS ( 'NONE', 5,
 ( #58504, #15907, #94854, #76393, #59061, #68023, #93184, #25411, #51197, #86450, #85327, #8623 ),
 .UNSPECIFIED., .F., .F.,
 ( 6, 3, 3, 6 ),
 ( 0.000000000000000000, 0.3076635699321720319, 0.7692211899778510498, 1.000000000000000000 ),
 .UNSPECIFIED. ) ;
#27811=SPHERICAL_SURFACE ( 'NONE', #81776, 2.000000000550000046 ) ;
#27812=B_SPLINE_CURVE_WITH_KNOTS ( 'NONE', 3,
 ( #13455, #72313, #39793, #73952, #22398, #71790 ),
 .UNSPECIFIED., .F., .F.,
 ( 4, 2, 4 ),
 ( 0.000000000000000000, 0.5000000000000000000, 1.000000000000000000 ),
 .UNSPECIFIED. ) ;
#27813=CARTESIAN_POINT ( 'NONE',  ( -4.271711423730000234, 1446.704873953880224, 157.7711695664980027 ) ) ;
#27814=CARTESIAN_POINT ( 'NONE',  ( -18.35972178970000357, 1424.606442804230028, 225.2895523400979982 ) ) ;
#27815=CARTESIAN_POINT ( 'NONE',  ( -17.08284985680000290, 1435.239220910890026, 147.2844623966980180 ) ) ;
#27816=CARTESIAN_POINT ( 'NONE',  ( -4.897375497219999652, 1432.353341358199941, 150.0655110971979980 ) ) ;
#27817=CARTESIAN_POINT ( 'NONE',  ( 17.24394154959999881, 1413.517467163129822, 192.0312209363980003 ) ) ;
#27818=CARTESIAN_POINT ( 'NONE',  ( 0.2483634325632210205, 1408.921733429509914, 231.7190040910680011 ) ) ;
#27820=CARTESIAN_POINT ( 'NONE',  ( 10.87371602109691970, 1426.219295122016547, 148.5295350641272591 ) ) ;
#27822=CARTESIAN_POINT ( 'NONE',  ( 12.51099983133400073, 1416.825784014559986, 196.0986189223339977 ) ) ;
#27823=CARTESIAN_POINT ( 'NONE',  ( 9856.831406526702267, 2833.746317950241519, 1378.242120268380177 ) ) ;
#27824=CARTESIAN_POINT ( 'NONE',  ( -24.07870975389999657, 1437.132368761460157, 211.2127430859480057 ) ) ;
#27827=CARTESIAN_POINT ( 'NONE',  ( -3.872181927699717363, 1426.015247764028345, 186.0427167524304082 ) ) ;
#27829=CARTESIAN_POINT ( 'NONE',  ( -18.85772126319670150, 1509.650461852630087, 185.3681582559849801 ) ) ;
#27835=CARTESIAN_POINT ( 'NONE',  ( -16.93884325354670040, 1507.634939694479954, 230.1482608329069990 ) ) ;
#27837=CARTESIAN_POINT ( 'NONE',  ( 24.48015091930000153, 1509.748507779630017, 193.8668277333979972 ) ) ;
#27839=CARTESIAN_POINT ( 'NONE',  ( -17.62175316511144985, 1460.293634674704435, 228.1921996207679797 ) ) ;
#27844=CARTESIAN_POINT ( 'NONE',  ( 18.18162401578809906, 1416.230844595159851, 209.3331246004520096 ) ) ;
#27845=CARTESIAN_POINT ( 'NONE',  ( 18.12088407619999941, 1425.009777113730024, 225.3844322571980001 ) ) ;
#27848=CARTESIAN_POINT ( 'NONE',  ( -33.93598460830000363, 1457.486625415129993, 259.3467912259980039 ) ) ;
#27850=CARTESIAN_POINT ( 'NONE',  ( -11.92957103340000202, 1433.515502532339951, 150.1951483352979722 ) ) ;
#27851=CARTESIAN_POINT ( 'NONE',  ( 24.27333642870000219, 1509.087578010229890, 195.8034309281979972 ) ) ;
#27852=CARTESIAN_POINT ( 'NONE',  ( -19.45985541978930300, 1483.862530646330015, 228.1370256266669969 ) ) ;
#27853=CARTESIAN_POINT ( 'NONE',  ( 5.230272464420000489, 1409.599014443830129, 186.6733164947980015 ) ) ;
#27854=CARTESIAN_POINT ( 'NONE',  ( 5.004094174289999586, 1423.187700235230068, 184.8599579744980019 ) ) ;
#27855=FACE_OUTER_BOUND ( 'NONE', #109768, .T. ) ;
#27856=CARTESIAN_POINT ( 'NONE',  ( 11.36665852199999982, 1437.938651650400061, 152.0461524011979861 ) ) ;
#27858=CARTESIAN_POINT ( 'NONE',  ( -14.98881544730000037, 1452.245887789929839, 149.4533671292980159 ) ) ;
#27864=CARTESIAN_POINT ( 'NONE',  ( -42.16354462729999852, 1445.439307631620068, 270.0644491700979870 ) ) ;
#27866=CARTESIAN_POINT ( 'NONE',  ( 6.655787406570000009, 1441.606255579999925, 154.8401361813980088 ) ) ;
#27867=DIRECTION ( 'NONE',  ( 0.000000000000000000, -1.000000000000000000, 0.000000000000000000 ) ) ;
#27868=CARTESIAN_POINT ( 'NONE',  ( 8.805428988939999257, 1497.713060387329961, 188.8615427550980144 ) ) ;
#27870=CARTESIAN_POINT ( 'NONE',  ( -1.352297191969999979, 1415.128105759529944, 226.9541798989980066 ) ) ;
#27871=CARTESIAN_POINT ( 'NONE',  ( -7.807415031859999743, 1418.825582515029964, 232.7594164784979966 ) ) ;
#27875=CARTESIAN_POINT ( 'NONE',  ( -45.39090023088340331, 1434.413450932079968, 266.9978870292519559 ) ) ;
#27876=CARTESIAN_POINT ( 'NONE',  ( -2.500000000000000000, 1431.429175495760319, 184.4562418606980145 ) ) ;
#27883=CARTESIAN_POINT ( 'NONE',  ( -16.49339310219999888, 1410.410615637530100, 191.6555828938980142 ) ) ;
#27885=ORIENTED_EDGE ( 'NONE', *, *, #91628, .T. ) ;
#27886=CARTESIAN_POINT ( 'NONE',  ( -15.56483135600000089, 1506.802866779329861, 193.3150509027980206 ) ) ;
#27887=CARTESIAN_POINT ( 'NONE',  ( 0.3740406207303079711, 1452.976564550639978, 183.2744760995269928 ) ) ;
#27894=CARTESIAN_POINT ( 'NONE',  ( -23.03491636582509727, 1413.194898312140140, 270.3705240770690352 ) ) ;
#27899=VERTEX_POINT ( 'NONE', #66209 ) ;
#27901=CARTESIAN_POINT ( 'NONE',  ( 44.79110309957884084, 1447.468097970602912, 268.9984334317801995 ) ) ;
#27903=CARTESIAN_POINT ( 'NONE',  ( 3.648172162208111580, 1424.944969327661283, 184.9068109353121940 ) ) ;
#27904=CARTESIAN_POINT ( 'NONE',  ( -0.01186867620443360014, 1408.939236553560022, 186.1929645843580090 ) ) ;
#27906=CARTESIAN_POINT ( 'NONE',  ( -18.44487993178400131, 1415.666200586320201, 207.5693722478499978 ) ) ;
#27907=CARTESIAN_POINT ( 'NONE',  ( -20.60769613969999980, 1425.808610859230157, 221.1268796063979778 ) ) ;
#27909=ADVANCED_FACE ( 'NONE', ( #83514 ), #110084, .T. ) ;
#27910=CARTESIAN_POINT ( 'NONE',  ( 15.61100558644629999, 1473.362487039310054, 269.5822769614250092 ) ) ;
#27911=CARTESIAN_POINT ( 'NONE',  ( -5.330260781521928060, 1466.317908316536659, 234.3275359498189800 ) ) ;
#27912=CARTESIAN_POINT ( 'NONE',  ( 10.27848897229999992, 1446.428916322279974, 186.7328515026979971 ) ) ;
#27914=EDGE_LOOP ( 'NONE', ( #79007, #39510, #83442, #38739, #93961 ) ) ;
#27916=CARTESIAN_POINT ( 'NONE',  ( 1.482817440028709965, 1476.038795360169843, 182.4686008787339802 ) ) ;
#27919=CARTESIAN_POINT ( 'NONE',  ( 25.43929575127770093, 1451.150448064199963, 137.0720221098989953 ) ) ;
#27921=CARTESIAN_POINT ( 'NONE',  ( -13.43605234887320243, 1430.070734077150064, 196.2030595958090089 ) ) ;
#27924=CARTESIAN_POINT ( 'NONE',  ( 17.39803002860000092, 1409.685664280330002, 193.5282844070979991 ) ) ;
#27925=CARTESIAN_POINT ( 'NONE',  ( 18.64337105059429689, 1443.913060387331825, 162.1710875046050830 ) ) ;
#27926=CARTESIAN_POINT ( 'NONE',  ( 3.625788738682097279, 1439.697084659004531, 184.5692930381153758 ) ) ;
#27928=CARTESIAN_POINT ( 'NONE',  ( -19.88588797745208581, 1426.224259812586979, 222.6860395134592920 ) ) ;
#27929=CARTESIAN_POINT ( 'NONE',  ( 0.6545676963618470845, 1450.893079684980194, 181.6462381494110048 ) ) ;
#27932=CARTESIAN_POINT ( 'NONE',  ( 27.15680186111980277, 1447.232003934320119, 137.0388483343459995 ) ) ;
#27933=ORIENTED_EDGE ( 'NONE', *, *, #25860, .F. ) ;
#27936=CARTESIAN_POINT ( 'NONE',  ( -0.4098070700370579633, 1409.180871098390071, 232.5580995887669928 ) ) ;
#27937=CIRCLE ( 'NONE', #22542, 95.87933833688167340 ) ;
#27938=CARTESIAN_POINT ( 'NONE',  ( 9788.078716724870901, 2833.596074015789782, 1421.913706743000148 ) ) ;
#27942=CARTESIAN_POINT ( 'NONE',  ( -9.019386502799999761, 1461.887471368730075, 248.0989693022980020 ) ) ;
#27943=CARTESIAN_POINT ( 'NONE',  ( 45.55047695329995605, 1443.690990841655321, 266.1919662023980777 ) ) ;
#27944=CARTESIAN_POINT ( 'NONE',  ( 11.06650222010000029, 1433.167564766650003, 151.7066924991980272 ) ) ;
#27945=CARTESIAN_POINT ( 'NONE',  ( -2.383927472408579717, 1474.129566312720044, 270.1365026341109683 ) ) ;
#27946=CARTESIAN_POINT ( 'NONE',  ( 26.90416343740999849, 1440.913060391219915, 226.3888494030570087 ) ) ;
#27947=CARTESIAN_POINT ( 'NONE',  ( -21.43945572710000036, 1508.012730663529737, 227.0658374796979899 ) ) ;
#27951=CARTESIAN_POINT ( 'NONE',  ( 23.61230825720000226, 1435.322028862560046, 137.2857987807979896 ) ) ;
#27952=CARTESIAN_POINT ( 'NONE',  ( -7.033373300310000964, 1486.517874593030001, 182.5016472222980042 ) ) ;
#27954=CARTESIAN_POINT ( 'NONE',  ( 2.890489019979999963, 1507.108937782129942, 235.9439513777979869 ) ) ;
#27955=CARTESIAN_POINT ( 'NONE',  ( 24.81840806639999997, 1430.361839715729730, 209.9936183716149856 ) ) ;
#27957=CARTESIAN_POINT ( 'NONE',  ( -11.97142003969999990, 1507.754042655929879, 233.5465281419980101 ) ) ;
#27960=CARTESIAN_POINT ( 'NONE',  ( 18.64646848244989741, 1416.843574548044216, 209.6840263755165381 ) ) ;
#27962=CARTESIAN_POINT ( 'NONE',  ( 0.1682346187407569860, 1481.367886108869925, 182.0356305680300011 ) ) ;
#27964=ORIENTED_EDGE ( 'NONE', *, *, #110442, .F. ) ;
#27967=CARTESIAN_POINT ( 'NONE',  ( -37.10988369677580323, 1450.944967383530184, 134.0999999986949831 ) ) ;
#27973=CARTESIAN_POINT ( 'NONE',  ( -2.818453812998270802, 1509.034654136871495, 238.5774661494029090 ) ) ;
#27974=CARTESIAN_POINT ( 'NONE',  ( 4.291176059336820003, 1446.971469614359876, 154.7965853925720126 ) ) ;
#27977=CARTESIAN_POINT ( 'NONE',  ( 11.61231359760869886, 1409.318571304570014, 218.5364820568740072 ) ) ;
#27980=FACE_OUTER_BOUND ( 'NONE', #18453, .T. ) ;
#27983=CARTESIAN_POINT ( 'NONE',  ( 11.12217965309999812, 1433.940707244100167, 151.6712567464980168 ) ) ;
#27984=DIRECTION ( 'NONE',  ( 0.01793599824082334204, -0.9688514294439565244, 0.2469923230213998122 ) ) ;
#27985=CARTESIAN_POINT ( 'NONE',  ( -1.581901184577762409, 1426.946688134061105, 137.0999999980979567 ) ) ;
#27988=CARTESIAN_POINT ( 'NONE',  ( -11.90198537395339962, 1415.595619977640126, 195.0235258899830058 ) ) ;
#27991=CARTESIAN_POINT ( 'NONE',  ( 29.83201784440627335, 1462.372200568356220, 269.4690239067755329 ) ) ;
#27993=CARTESIAN_POINT ( 'NONE',  ( 5.033382749860000338, 1397.146220404329824, 220.9814784287979990 ) ) ;
#27995=CARTESIAN_POINT ( 'NONE',  ( 20.84167173783890092, 1473.796610273650003, 209.3926063897190204 ) ) ;
#27996=CARTESIAN_POINT ( 'NONE',  ( -1.206033063790000082, 1476.687496009330061, 182.5563120943979811 ) ) ;
#27998=CARTESIAN_POINT ( 'NONE',  ( -26.16739620090311291, 1436.693404600586746, 136.8894152260586452 ) ) ;
#28003=CARTESIAN_POINT ( 'NONE',  ( 41.20764152666490077, 1444.152539026100158, 136.7061128974409883 ) ) ;
#28005=CARTESIAN_POINT ( 'NONE',  ( 37.00345306050000005, 1420.039538152829891, 266.5575588314979996 ) ) ;
#28006=CARTESIAN_POINT ( 'NONE',  ( -27.14725374240000022, 1488.689090778130094, 207.3572097627179858 ) ) ;
#28007=CARTESIAN_POINT ( 'NONE',  ( 1.451130014660000134, 1504.651021693529856, 181.2207292498980280 ) ) ;
#28008=CARTESIAN_POINT ( 'NONE',  ( 13.57909981250000087, 1416.568813547830132, 196.3459685238979944 ) ) ;
#28011=B_SPLINE_CURVE_WITH_KNOTS ( 'NONE', 3,
 ( #46687, #80818, #29851, #107111, #20888, #74081, #4124, #38249, #64037, #98154, #29303, #81344, #89759, #82470, #81898, #90297, #5205, #23090, #107667, #21427, #37710, #31498, #63500, #12508, #5768, #13578, #80272, #39911, #55637, #65678, #56161, #72433, #99796, #91423, #65128, #71911, #30399, #64590, #97619 ),
 .UNSPECIFIED., .F., .F.,
 ( 4, 2, 2, 2, 1, 1, 1, 2, 2, 2, 2, 1, 1, 1, 2, 2, 2, 2, 1, 1, 1, 2, 2, 4 ),
 ( 0.000000000000000000, 0.1249999999999992506, 0.1874999999999988343, 0.2187500000000000278, 0.2343749999999804323, 0.2421874999999872324, 0.2460937499999715228, 0.2480468749999621692, 0.2499999999999528433, 0.3749999999997775668, 0.4374999999996881939, 0.4687499999996582734, 0.4843749999996572742, 0.4921874999996567746, 0.4960937499996547762, 0.4999999999996528333, 0.6249999999998488986, 0.6874999999999484857, 0.7187499999999996669, 0.7343750000000252021, 0.7421875000000365263, 0.7460937500000437428, 0.7500000000000508482, 1.000000000000000000 ),
 .UNSPECIFIED. ) ;
#28012=CARTESIAN_POINT ( 'NONE',  ( -22.71362857409999947, 1419.354696850730079, 250.3594883093980172 ) ) ;
#28014=CARTESIAN_POINT ( 'NONE',  ( 28.61821586768189718, 1509.224669306330043, 209.4805676029000097 ) ) ;
#28016=CARTESIAN_POINT ( 'NONE',  ( 33.91369255499999724, 1451.728777076330061, 134.7155730073980067 ) ) ;
#28020=CARTESIAN_POINT ( 'NONE',  ( -18.63536074199999959, 1457.257477148429871, 229.6471845788980204 ) ) ;
#28026=VERTEX_POINT ( 'NONE', #646 ) ;
#28030=CARTESIAN_POINT ( 'NONE',  ( -2.866976920500000414, 1479.772520933030137, 235.6353344876980032 ) ) ;
#28032=CARTESIAN_POINT ( 'NONE',  ( 45.88361912325480318, 1441.846453202439989, 266.4122209686929637 ) ) ;
#28034=CARTESIAN_POINT ( 'NONE',  ( 13.93012033159999952, 1463.781730353329976, 224.9320934324980215 ) ) ;
#28035=EDGE_LOOP ( 'NONE', ( #10423, #48980, #96384, #78236 ) ) ;
#28039=CARTESIAN_POINT ( 'NONE',  ( 11.85752262936500045, 1431.737903649139980, 149.9496635218089864 ) ) ;
#28040=DIRECTION ( 'NONE',  ( -0.000000000000000000, -0.000000000000000000, -1.000000000000000000 ) ) ;
#28044=CARTESIAN_POINT ( 'NONE',  ( -0.1681681984989999989, 1418.913060387330006, 172.2701767054979882 ) ) ;
#28046=CARTESIAN_POINT ( 'NONE',  ( -4.275814211600000192, 1424.445698836229894, 185.6670158391980010 ) ) ;
#28047=CARTESIAN_POINT ( 'NONE',  ( 3.196891693280000002, 1407.733286134229957, 270.1354749225980072 ) ) ;
#28060=CARTESIAN_POINT ( 'NONE',  ( 12.48077398309999886, 1422.454772915230024, 243.9198229250980035 ) ) ;
#28062=AXIS2_PLACEMENT_3D ( 'NONE', #37062, #103142, #60637 ) ;
#28068=ORIENTED_EDGE ( 'NONE', *, *, #25614, .T. ) ;
#28070=CARTESIAN_POINT ( 'NONE',  ( -24.04512698680000327, 1444.427565174400115, 211.8281269584280153 ) ) ;
#28071=B_SPLINE_CURVE_WITH_KNOTS ( 'NONE', 3,
 ( #46953, #37432, #81073, #71630, #54794, #97326, #72695, #21696, #105750, #4389 ),
 .UNSPECIFIED., .F., .F.,
 ( 4, 2, 2, 2, 4 ),
 ( 0.000000000000000000, 0.2500000000000000000, 0.5000000000000000000, 0.7500000000000000000, 1.000000000000000000 ),
 .UNSPECIFIED. ) ;
#28072=CARTESIAN_POINT ( 'NONE',  ( -2.494317414332789529, 1449.209847618189542, 154.5141281627416561 ) ) ;
#28075=CARTESIAN_POINT ( 'NONE',  ( -10.55869165969999912, 1442.273726812979930, 186.3969298045979883 ) ) ;
#28076=CARTESIAN_POINT ( 'NONE',  ( 27.60850322493959652, 1509.877168147730117, 194.6763840514340131 ) ) ;
#28079=CARTESIAN_POINT ( 'NONE',  ( 15.56606087930000015, 1415.086919075230071, 227.3762381457980268 ) ) ;
#28080=ADVANCED_FACE ( 'NONE', ( #34777 ), #84072, .T. ) ;
#28082=CARTESIAN_POINT ( 'NONE',  ( -16.06782005780000233, 1459.209651374430223, 230.7189234877979800 ) ) ;
#28084=CARTESIAN_POINT ( 'NONE',  ( 43.90552978530000416, 1429.946926731829990, 266.4740132303979863 ) ) ;
#28085=CIRCLE ( 'NONE', #51336, 29.82803840400378803 ) ;
#28087=CARTESIAN_POINT ( 'NONE',  ( 21.03533413319999923, 1435.660194803150034, 143.7853187944979823 ) ) ;
#28088=CARTESIAN_POINT ( 'NONE',  ( 19.43264287389999723, 1488.590530053829980, 189.7255375135980273 ) ) ;
#28089=CARTESIAN_POINT ( 'NONE',  ( 5.366477781255650115, 1426.058802480919894, 152.4456445666100137 ) ) ;
#28091=CARTESIAN_POINT ( 'NONE',  ( 12.61640438649999929, 1416.837080248530128, 223.3238927091979917 ) ) ;
#28094=CARTESIAN_POINT ( 'NONE',  ( -21.41666160454324697, 1506.776553291482287, 202.5225393536939009 ) ) ;
#28096=CARTESIAN_POINT ( 'NONE',  ( -12.59298689929999959, 1442.703280217149995, 186.7739262576980082 ) ) ;
#28098=FACE_OUTER_BOUND ( 'NONE', #86697, .T. ) ;
#28102=CARTESIAN_POINT ( 'NONE',  ( -2.881436550369800287, 1409.013682368930176, 223.8287015832810027 ) ) ;
#28103=DIRECTION ( 'NONE',  ( -1.000000000000000000, 0.000000000000000000, -1.989556701369999986E-13 ) ) ;
#28105=VECTOR ( 'NONE', #48336, 1000.000000000000000 ) ;
#28106=CARTESIAN_POINT ( 'NONE',  ( -45.02947505619999902, 1451.249933470530095, 267.6322170074980136 ) ) ;
#28109=CARTESIAN_POINT ( 'NONE',  ( -27.93022619350000113, 1509.888405378130074, 214.3883701560380075 ) ) ;
#28112=CARTESIAN_POINT ( 'NONE',  ( 16.61248850094990104, 1423.423305472560060, 227.8798840990210124 ) ) ;
#28113=CARTESIAN_POINT ( 'NONE',  ( 20.61224126859999828, 1508.367040381230026, 227.7934947756980080 ) ) ;
#28114=CARTESIAN_POINT ( 'NONE',  ( -11.88064286090000010, 1433.444786854229960, 151.0525681022980109 ) ) ;
#28119=CARTESIAN_POINT ( 'NONE',  ( -24.08425369710000297, 1411.115211429229930, 208.6111293678600020 ) ) ;
#28121=CARTESIAN_POINT ( 'NONE',  ( 15.13954211869999966, 1415.426091369230107, 199.2823809441580067 ) ) ;
#28122=CARTESIAN_POINT ( 'NONE',  ( -11.95871496589999872, 1415.628674276829770, 194.9673395089980090 ) ) ;
#28123=CARTESIAN_POINT ( 'NONE',  ( -0.0001732888907949209931, 1456.398128790439841, 144.1938086916980239 ) ) ;
#28125=CARTESIAN_POINT ( 'NONE',  ( 22.92656559199999933, 1409.713673699430046, 210.2581852642179854 ) ) ;
#28130=DIRECTION ( 'NONE',  ( 0.000000000000000000, 0.000000000000000000, -1.000000000000000000 ) ) ;
#28135=FACE_OUTER_BOUND ( 'NONE', #85429, .T. ) ;
#28137=CARTESIAN_POINT ( 'NONE',  ( -1.410150725348159995, 1420.916685646099950, 183.2158715699029869 ) ) ;
#28139=CARTESIAN_POINT ( 'NONE',  ( -22.09796275270000265, 1430.768449482030064, 219.6318221129980088 ) ) ;
#28140=CARTESIAN_POINT ( 'NONE',  ( -18.69874064677919634, 1486.217926523959932, 189.0579342009679920 ) ) ;
#28142=CARTESIAN_POINT ( 'NONE',  ( -4.253357141732059254, 1441.312379553120081, 160.5446465494569850 ) ) ;
#28143=AXIS2_PLACEMENT_3D ( 'NONE', #42429, #24507, #48655 ) ;
#28145=ORIENTED_EDGE ( 'NONE', *, *, #59133, .F. ) ;
#28151=CARTESIAN_POINT ( 'NONE',  ( -15.72514096998889066, 1409.739244463557043, 226.1586303163210800 ) ) ;
#28152=CARTESIAN_POINT ( 'NONE',  ( 0.1625281483599999854, 1507.112338238429857, 180.9288958984979843 ) ) ;
#28156=CARTESIAN_POINT ( 'NONE',  ( 15.44339577220000059, 1507.633509799529975, 186.9079894093979988 ) ) ;
#28158=CARTESIAN_POINT ( 'NONE',  ( 7.168422058350000015, 1409.330743147429985, 230.2017730211979938 ) ) ;
#28159=FILL_AREA_STYLE ('',( #87530 ) ) ;
#28162=CARTESIAN_POINT ( 'NONE',  ( 41.06928241250569300, 1446.732447649089863, 134.0999999985529882 ) ) ;
#28164=CARTESIAN_POINT ( 'NONE',  ( -5399.972634328954882, 2837.742859910729294, -8135.989823645887554 ) ) ;
#28169=ORIENTED_EDGE ( 'NONE', *, *, #44711, .F. ) ;
#28170=ADVANCED_FACE ( 'NONE', ( #71736 ), #86902, .F. ) ;
#28174=CARTESIAN_POINT ( 'NONE',  ( 13.15671565689999944, 1428.802034784529951, 222.6511392629980151 ) ) ;
#28176=CARTESIAN_POINT ( 'NONE',  ( -1.530900592538410043, 1457.980095062469900, 229.8454460011110143 ) ) ;
#28178=EDGE_CURVE ( 'NONE', #22756, #58583, #90284, .T. ) ;
#28179=CARTESIAN_POINT ( 'NONE',  ( -17.94888193757963890, 1447.286725237485371, 216.7531926085807470 ) ) ;
#28182=VERTEX_POINT ( 'NONE', #87396 ) ;
#28184=VERTEX_POINT ( 'NONE', #36426 ) ;
#28185=CARTESIAN_POINT ( 'NONE',  ( 26.22923941070369835, 1440.913060387330006, 242.8863953517110019 ) ) ;
#28186=CARTESIAN_POINT ( 'NONE',  ( -0.0001467037859797497713, 1452.764096049401132, 153.2008905006179020 ) ) ;
#28189=CARTESIAN_POINT ( 'NONE',  ( -14.43454037350000085, 1409.919030993929937, 190.6684835116980139 ) ) ;
#28191=CARTESIAN_POINT ( 'NONE',  ( -24.39234957080000044, 1440.942612022289950, 211.3352087105480166 ) ) ;
#28193=CARTESIAN_POINT ( 'NONE',  ( -4.738498500012391368, 1427.169020172040746, 137.0999999980979851 ) ) ;
#28194=CARTESIAN_POINT ( 'NONE',  ( 0.0002693575158267318766, 1396.632379581024907, 196.5747687561042767 ) ) ;
#28195=CARTESIAN_POINT ( 'NONE',  ( -13.09824453989481974, 1434.823787125280205, 146.9138453073250616 ) ) ;
#28196=CARTESIAN_POINT ( 'NONE',  ( -11.87921130439999828, 1433.311613823580274, 149.2720837588979919 ) ) ;
#28198=CARTESIAN_POINT ( 'NONE',  ( 10.04917727119999959, 1464.412817549529791, 232.3873387124980070 ) ) ;
#28204=CARTESIAN_POINT ( 'NONE',  ( 27.78452743450000284, 1508.000976256729928, 207.7754991279980175 ) ) ;
#28206=CARTESIAN_POINT ( 'NONE',  ( -18.06710007320000244, 1416.825245919329973, 209.3442279612220034 ) ) ;
#28209=EDGE_LOOP ( 'NONE', ( #65889, #28971, #75484, #82688 ) ) ;
#28211=CARTESIAN_POINT ( 'NONE',  ( 29.63060655169999791, 1444.770721089869994, 238.0637411752979915 ) ) ;
#28214=CARTESIAN_POINT ( 'NONE',  ( -1.437936433978639794, 1507.910105588649913, 237.3166670950480182 ) ) ;
#28215=CARTESIAN_POINT ( 'NONE',  ( -19.36515920259999746, 1456.378690096930086, 228.5344338431980304 ) ) ;
#28217=ADVANCED_FACE ( 'NONE', ( #104738 ), #2732, .F. ) ;
#28218=CARTESIAN_POINT ( 'NONE',  ( -22.75994491043178058, 1411.068131679461885, 204.0207675248701094 ) ) ;
#28219=CARTESIAN_POINT ( 'NONE',  ( 2.500000000000000000, 1420.168334228329968, 149.0935893383980044 ) ) ;
#28220=CARTESIAN_POINT ( 'NONE',  ( -0.3670406238980000180, 1434.822844257019824, 190.2779712162979990 ) ) ;
#28224=CARTESIAN_POINT ( 'NONE',  ( 2.776335336629999873, 1405.836660839130218, 268.4805445416980092 ) ) ;
#28225=EDGE_CURVE ( 'NONE', #78889, #60804, #81331, .T. ) ;
#28227=AXIS2_PLACEMENT_3D ( 'NONE', #96015, #103288, #42303 ) ;
#28229=CARTESIAN_POINT ( 'NONE',  ( 19.03738911459980088, 1469.388104986470125, 270.0854773280680092 ) ) ;
#28230=CARTESIAN_POINT ( 'NONE',  ( 2.478279119729999813, 1438.995264557609971, 157.7427228779980055 ) ) ;
#28232=CARTESIAN_POINT ( 'NONE',  ( -40.72444163363370251, 1440.913060406799787, 260.2869945447760074 ) ) ;
#28234=CARTESIAN_POINT ( 'NONE',  ( -26.34572671679999800, 1447.163110651519901, 137.4477041290980139 ) ) ;
#28235=CARTESIAN_POINT ( 'NONE',  ( 2.382666182145900091, 1449.574453021285308, 154.4426451947454382 ) ) ;
#28237=CARTESIAN_POINT ( 'NONE',  ( 1.172951571615530098, 1450.815013399510008, 154.5169618134089831 ) ) ;
#28239=CARTESIAN_POINT ( 'NONE',  ( 12.26979804483799974, 1416.828039243390094, 223.5793509210460002 ) ) ;
#28241=CARTESIAN_POINT ( 'NONE',  ( -42.15865170690000241, 1431.016965136909903, 271.1218459616979999 ) ) ;
#28242=CARTESIAN_POINT ( 'NONE',  ( -1.266763281143285402, 1450.741562714445536, 181.7950901315468570 ) ) ;
#28244=CARTESIAN_POINT ( 'NONE',  ( -0.8878292600469999130, 1475.977008401730018, 267.2346354036980074 ) ) ;
#28245=AXIS2_PLACEMENT_3D ( 'NONE', #4447, #45905, #46463 ) ;
#28246=CARTESIAN_POINT ( 'NONE',  ( -28.24318413590000176, 1508.132100804830088, 209.6063173613950141 ) ) ;
#28247=CARTESIAN_POINT ( 'NONE',  ( -3.513170386600249273, 1448.288673971990193, 184.8796385662358546 ) ) ;
#28249=CARTESIAN_POINT ( 'NONE',  ( -17.33645360970000127, 1414.996444518330009, 207.8511176870179895 ) ) ;
#28250=CARTESIAN_POINT ( 'NONE',  ( -6.232532106187401055, 1407.162969929529936, 197.7132727037109987 ) ) ;
#28251=CARTESIAN_POINT ( 'NONE',  ( 26.43520611626190231, 1435.427582101930057, 135.4748900071289768 ) ) ;
#28253=CARTESIAN_POINT ( 'NONE',  ( -11.03746375029680138, 1396.298497114720021, 210.0060340494559910 ) ) ;
#28254=CARTESIAN_POINT ( 'NONE',  ( -15.49281168989999813, 1421.632443114230000, 227.2929369300979943 ) ) ;
#28255=CARTESIAN_POINT ( 'NONE',  ( -17.21806449221460156, 1410.146609974180137, 225.6635716917170100 ) ) ;
#28259=CARTESIAN_POINT ( 'NONE',  ( 1.724138604399999997, 1408.973268634130136, 230.9767750068980092 ) ) ;
#28260=CARTESIAN_POINT ( 'NONE',  ( -15.45533207179999913, 1484.705735421829786, 187.3543539206980029 ) ) ;
#28261=CARTESIAN_POINT ( 'NONE',  ( 11.30045313650000161, 1426.459762359429988, 112.6498394735979929 ) ) ;
#28264=CARTESIAN_POINT ( 'NONE',  ( -12.53380498098199602, 1442.773887284840612, 151.6125157144320212 ) ) ;
#28271=CARTESIAN_POINT ( 'NONE',  ( 1.447786046720000108, 1507.396806431330106, 181.1008358460979935 ) ) ;
#28275=ADVANCED_FACE ( 'NONE', ( #25117 ), #101823, .T. ) ;
#28276=CARTESIAN_POINT ( 'NONE',  ( -14.05757238939644260, 1460.648840875784572, 232.1449228860425080 ) ) ;
#28278=EDGE_LOOP ( 'NONE', ( #106200, #40823, #32717, #24992 ) ) ;
#28279=CARTESIAN_POINT ( 'NONE',  ( -41.66021910349999757, 1443.875694946319754, 135.6929188412979954 ) ) ;
#28280=CARTESIAN_POINT ( 'NONE',  ( 0.4380014478882280349, 1474.776185545679937, 235.9802319278450113 ) ) ;
#28281=CARTESIAN_POINT ( 'NONE',  ( 9.668109322589998555, 1408.913060387329779, 224.6723891271980165 ) ) ;
#28284=CARTESIAN_POINT ( 'NONE',  ( -2.056387895720000358, 1486.516979218729830, 181.7077744939979880 ) ) ;
#28287=CARTESIAN_POINT ( 'NONE',  ( 12.55840807187700037, 1425.933963207659872, 223.8625469537460049 ) ) ;
#28289=CARTESIAN_POINT ( 'NONE',  ( 6.235478689385840489, 1396.130808101319872, 218.2352667451380057 ) ) ;
#28290=CARTESIAN_POINT ( 'NONE',  ( -0.06979926259237639874, 1408.910622943330054, 194.1218459608980140 ) ) ;
#28291=CARTESIAN_POINT ( 'NONE',  ( 5.574750653145040338E-05, 1406.066344387250183, 269.0457483805509469 ) ) ;
#28292=CARTESIAN_POINT ( 'NONE',  ( 41.66146276220000289, 1443.809306595659791, 136.1342541931979895 ) ) ;
#28293=ORIENTED_EDGE ( 'NONE', *, *, #47350, .F. ) ;
#28294=CARTESIAN_POINT ( 'NONE',  ( -11.86593337649999924, 1432.333319972560048, 150.3971781300980126 ) ) ;
#28295=CARTESIAN_POINT ( 'NONE',  ( 12.67807438250000018, 1442.703181404250017, 187.4495022272980123 ) ) ;
#28299=EDGE_LOOP ( 'NONE', ( #87133, #23820, #42296, #25585 ) ) ;
#28306=B_SPLINE_SURFACE_WITH_KNOTS ( 'NONE', 5, 5, ( 
 ( #51083, #8499, #42125, #142, #15774, #76273 ),
 ( #34816, #59490, #109339, #9065, #49976, #92507 ),
 ( #51629, #50534, #84658, #33701, #102549, #102003 ),
 ( #25289, #69003, #93600, #16878, #103107, #42671 ),
 ( #76828, #34264, #68446, #83556, #60043, #94721 ),
 ( #94162, #6849, #84112, #43235, #77383, #41577 ) ),
 .UNSPECIFIED., .F., .F., .F.,
 ( 6, 6 ),
 ( 6, 6 ),
 ( 29.50720980459999865, 158.0245753780000086 ),
 ( -5.551115123129999410E-17, 1.000000000000000000 ),
 .UNSPECIFIED. ) ;
#28308=ORIENTED_EDGE ( 'NONE', *, *, #54960, .F. ) ;
#28311=AXIS2_PLACEMENT_3D ( 'NONE', #89211, #13028, #61839 ) ;
#28312=VECTOR ( 'NONE', #104159, 1000.000000000000000 ) ;
#28318=CARTESIAN_POINT ( 'NONE',  ( -8.286009866380000588, 1409.704129222430083, 230.3000291798979902 ) ) ;
#28319=CARTESIAN_POINT ( 'NONE',  ( -11.96787629350000159, 1446.201514831819850, 187.3303138752980033 ) ) ;
#28321=CARTESIAN_POINT ( 'NONE',  ( 8.907440304832482170, 1432.353341358199941, 149.1004941873906660 ) ) ;
#28322=CARTESIAN_POINT ( 'NONE',  ( 11.44665326297827335, 1425.798162341591706, 139.1345266541928538 ) ) ;
#28324=CARTESIAN_POINT ( 'NONE',  ( -25.72910798539999888, 1436.492646657430214, 137.0497317554980157 ) ) ;
#28326=CARTESIAN_POINT ( 'NONE',  ( 42.44869904479999434, 1432.149879290850095, 270.3370793111479884 ) ) ;
#28329=CARTESIAN_POINT ( 'NONE',  ( 5.511665417999469900E-05, 1508.970066526555001, 238.8757070596369942 ) ) ;
#28335=CARTESIAN_POINT ( 'NONE',  ( -11.66816036250000010, 1420.438647421430005, 229.1834824673979938 ) ) ;
#28337=ORIENTED_EDGE ( 'NONE', *, *, #99058, .F. ) ;
#28340=CARTESIAN_POINT ( 'NONE',  ( 16.08217969103819911, 1469.006061218260129, 229.7393514651440114 ) ) ;
#28343=CARTESIAN_POINT ( 'NONE',  ( -0.02529539845109999782, 1409.857530525830043, 233.2156916876980119 ) ) ;
#28345=EDGE_CURVE ( 'NONE', #67449, #87841, #27710, .T. ) ;
#28350=ORIENTED_EDGE ( 'NONE', *, *, #7058, .F. ) ;
#28351=CARTESIAN_POINT ( 'NONE',  ( -12.58433072603950009, 1415.426207913209964, 196.9819739087400023 ) ) ;
#28352=CARTESIAN_POINT ( 'NONE',  ( -16.67342217799999915, 1504.313428625830056, 185.6524960304979857 ) ) ;
#28353=ORIENTED_EDGE ( 'NONE', *, *, #95927, .F. ) ;
#28354=CARTESIAN_POINT ( 'NONE',  ( 4.234467186019998941, 1420.712403710529998, 185.6414431274980075 ) ) ;
#28355=PLANE ( 'NONE',  #72626 ) ;
#28361=CARTESIAN_POINT ( 'NONE',  ( 17.92792478850000037, 1415.296882282229944, 210.0737307021219920 ) ) ;
#28362=CARTESIAN_POINT ( 'NONE',  ( -17.49524353049999803, 1436.343070723249866, 147.8329090225980167 ) ) ;
#28363=CARTESIAN_POINT ( 'NONE',  ( 33.91369968912619726, 1451.728767897860052, 134.7155302171979940 ) ) ;
#28365=CARTESIAN_POINT ( 'NONE',  ( 0.6531460927897710933, 1409.103080214060128, 232.5176971054530100 ) ) ;
#28368=ORIENTED_EDGE ( 'NONE', *, *, #84370, .F. ) ;
#28370=CARTESIAN_POINT ( 'NONE',  ( 25.51721860929999863, 1469.158424523229769, 207.1962240684080143 ) ) ;
#28371=CARTESIAN_POINT ( 'NONE',  ( -23.86337105550000004, 1436.937184565879988, 212.0334657536579925 ) ) ;
#28372=LINE ( 'NONE', #28934, #50937 ) ;
#28373=COLOUR_RGB ( '', 0.08235294, 0.09019608, 0.10196078) ;
#28374=CARTESIAN_POINT ( 'NONE',  ( -18.55970593940000057, 1508.848287783829846, 229.9905654330979985 ) ) ;
#28375=CARTESIAN_POINT ( 'NONE',  ( -2.880413542612040079, 1425.982839100257934, 185.3253768740765963 ) ) ;
#28376=CARTESIAN_POINT ( 'NONE',  ( 11.86890500783672842, 1435.287397482030201, 151.2475232226828439 ) ) ;
#28378=CARTESIAN_POINT ( 'NONE',  ( -14.31460220670079941, 1509.452787612570091, 183.0438844114540018 ) ) ;
#28379=AXIS2_PLACEMENT_3D ( 'NONE', #36959, #103620, #70602 ) ;
#28388=ORIENTED_EDGE ( 'NONE', *, *, #64583, .T. ) ;
#28389=CARTESIAN_POINT ( 'NONE',  ( 17.12480624395889706, 1507.616838180409786, 193.8046521743370079 ) ) ;
#28392=CARTESIAN_POINT ( 'NONE',  ( -11.74015320060000001, 1428.979986575930070, 144.1938086916980239 ) ) ;
#28394=VERTEX_POINT ( 'NONE', #8874 ) ;
#28395=CARTESIAN_POINT ( 'NONE',  ( 13.74650104269999851, 1441.983649238280123, 189.3366583681979876 ) ) ;
#28397=CARTESIAN_POINT ( 'NONE',  ( 12.83564499065948716, 1442.860052983879996, 169.4451046929141853 ) ) ;
#28398=CARTESIAN_POINT ( 'NONE',  ( 27.06247215711447396, 1417.591791844086856, 269.4421024428557985 ) ) ;
#28399=CARTESIAN_POINT ( 'NONE',  ( -5.805165725770000229, 1470.400760091029952, 255.2684105097979739 ) ) ;
#28400=EDGE_CURVE ( 'NONE', #85568, #8717, #66565, .T. ) ;
#28402=CARTESIAN_POINT ( 'NONE',  ( -11.88717770409999908, 1433.553338367350079, 150.4897835633980208 ) ) ;
#28403=EDGE_CURVE ( 'NONE', #104141, #28836, #8042, .T. ) ;
#28405=CARTESIAN_POINT ( 'NONE',  ( -19.14160362779999858, 1485.709425685830183, 189.6559982148980055 ) ) ;
#28407=CARTESIAN_POINT ( 'NONE',  ( 11.34224779750000067, 1409.809526181430101, 189.6148948717980147 ) ) ;
#28410=CARTESIAN_POINT ( 'NONE',  ( 11.83477883539999986, 1434.684743758880131, 151.1661215832980076 ) ) ;
#28413=CARTESIAN_POINT ( 'NONE',  ( -20.19751881499999868, 1450.975641626430161, 145.7773103342979937 ) ) ;
#28419=CARTESIAN_POINT ( 'NONE',  ( -13.03174027510000066, 1470.346600428830243, 269.8790079804980451 ) ) ;
#28421=CARTESIAN_POINT ( 'NONE',  ( 16.87240840930000019, 1409.502257872129803, 222.1138758984979802 ) ) ;
#28422=CARTESIAN_POINT ( 'NONE',  ( -14.84750872589999915, 1485.048555357530176, 224.0947347056979879 ) ) ;
#28423=CARTESIAN_POINT ( 'NONE',  ( 15.28420222199999934, 1497.713060387329961, 193.8376437393980325 ) ) ;
#28424=CARTESIAN_POINT ( 'NONE',  ( -4.363122647530000009, 1421.075575420230052, 170.1076616725979989 ) ) ;
#28427=CARTESIAN_POINT ( 'NONE',  ( -45.35503536899049948, 1436.791125258660031, 266.1974304159290341 ) ) ;
#28428=ORIENTED_EDGE ( 'NONE', *, *, #61063, .F. ) ;
#28433=EDGE_CURVE ( 'NONE', #47384, #104047, #35673, .T. ) ;
#28437=CARTESIAN_POINT ( 'NONE',  ( -27.03140942220920095, 1451.490713798300249, 136.0731937540990089 ) ) ;
#28448=CARTESIAN_POINT ( 'NONE',  ( -9.682670043730421838, 1409.984507541440053, 270.3686428832239699 ) ) ;
#28450=CARTESIAN_POINT ( 'NONE',  ( -0.7484295816749999553, 1428.043997280830126, 101.8807690336980016 ) ) ;
#28453=ORIENTED_EDGE ( 'NONE', *, *, #18575, .F. ) ;
#28455=CARTESIAN_POINT ( 'NONE',  ( 45.63029764463163929, 1441.507770731200935, 268.9749386593517784 ) ) ;
#28457=CARTESIAN_POINT ( 'NONE',  ( -10.74904557270209082, 1438.632470347905837, 152.4698233941169008 ) ) ;
#28460=CARTESIAN_POINT ( 'NONE',  ( -18.28144489529720218, 1415.492117401540099, 207.5679474733179859 ) ) ;
#28463=CARTESIAN_POINT ( 'NONE',  ( 10.61930341568279879, 1475.185691052500033, 269.0172316872100282 ) ) ;
#28464=CARTESIAN_POINT ( 'NONE',  ( -1.565064790564475894, 1467.010193131020060, 235.3666753383823504 ) ) ;
#28465=CARTESIAN_POINT ( 'NONE',  ( -17.64968521348830421, 1423.160730800522060, 226.3068084200317287 ) ) ;
#28466=( BOUNDED_CURVE ( )  B_SPLINE_CURVE ( 3, ( #109563, #59177, #69229, #16023 ),
 .UNSPECIFIED., .F., .F. ) 
 B_SPLINE_CURVE_WITH_KNOTS ( ( 4, 4 ),
 ( 0.05347086468394689901, 0.09168413669265079724 ),
 .UNSPECIFIED. ) 
 CURVE ( )  GEOMETRIC_REPRESENTATION_ITEM ( )  RATIONAL_B_SPLINE_CURVE ( ( 1.000000000000000000, 0.9998783158554702677, 0.9998783158554702677, 1.000000000000000000 ) ) 
 REPRESENTATION_ITEM ( '' )  );
#28469=CARTESIAN_POINT ( 'NONE',  ( 23.24354977585844040, 1411.085069985731025, 212.7460856263411415 ) ) ;
#28470=CARTESIAN_POINT ( 'NONE',  ( 1.498256283064010042, 1466.857882684819970, 182.8697145444330090 ) ) ;
#28471=ORIENTED_EDGE ( 'NONE', *, *, #82371, .T. ) ;
#28472=CARTESIAN_POINT ( 'NONE',  ( 7.303366077162626091, 1456.574606934232634, 227.6099195461272870 ) ) ;
#28473=CARTESIAN_POINT ( 'NONE',  ( 24.70673247591740207, 1451.987717812959772, 136.4510166997479814 ) ) ;
#28475=CARTESIAN_POINT ( 'NONE',  ( -10.70847609427080016, 1506.854789404229905, 189.5201119528840081 ) ) ;
#28477=CARTESIAN_POINT ( 'NONE',  ( -18.63535451612431970, 1508.532394786728901, 229.9190513451956690 ) ) ;
#28478=CARTESIAN_POINT ( 'NONE',  ( 18.33529589289999961, 1410.049765793829692, 194.4554404145980016 ) ) ;
#28479=CARTESIAN_POINT ( 'NONE',  ( 18.29245442332558014, 1445.052233488288721, 161.2175811807109937 ) ) ;
#28482=CARTESIAN_POINT ( 'NONE',  ( 19.87695271833857902, 1456.362367750117528, 223.8442701291641015 ) ) ;
#28483=AXIS2_PLACEMENT_3D ( 'NONE', #40215, #57595, #14991 ) ;
#28486=CARTESIAN_POINT ( 'NONE',  ( 26.50104796915090333, 1446.255561005059917, 137.5974644915019951 ) ) ;
#28487=VERTEX_POINT ( 'NONE', #1067 ) ;
#28489=DIRECTION ( 'NONE',  ( -0.7257730359255160080, 1.512900915589710975E-09, 0.6879342267422517976 ) ) ;
#28490=DIRECTION ( 'NONE',  ( 1.000000000000000000, 0.000000000000000000, 0.000000000000000000 ) ) ;
#28491=CARTESIAN_POINT ( 'NONE',  ( -11081.89558201059481, 2833.596074015790236, 8724.858692896474167 ) ) ;
#28492=CARTESIAN_POINT ( 'NONE',  ( -39.50712975707070029, 1446.923889365939885, 136.6550386957819967 ) ) ;
#28494=CARTESIAN_POINT ( 'NONE',  ( -27.19819525190000320, 1447.435760031770087, 248.0989693021979861 ) ) ;
#28495=CARTESIAN_POINT ( 'NONE',  ( 45.23908986689997391, 1446.067266319080318, 266.2007832802979124 ) ) ;
#28497=DIRECTION ( 'NONE',  ( 4.255490039221486549E-06, 0.03086473865808741363, -0.9995235704521724385 ) ) ;
#28499=CARTESIAN_POINT ( 'NONE',  ( -23.19979839009999978, 1508.008613658229933, 224.0655036725979983 ) ) ;
#28502=CARTESIAN_POINT ( 'NONE',  ( -27.04494122719999893, 1509.634156654429944, 201.2636815846580021 ) ) ;
#28503=CARTESIAN_POINT ( 'NONE',  ( 20.51044083260000050, 1453.146242307730063, 210.6541360869379957 ) ) ;
#28504=CARTESIAN_POINT ( 'NONE',  ( -3.526881412259999848, 1486.384130060029975, 181.8597813580979903 ) ) ;
#28507=AXIS2_PLACEMENT_3D ( 'NONE', #55481, #64438, #4518 ) ;
#28508=CARTESIAN_POINT ( 'NONE',  ( 23.86310425499999965, 1449.793994881729986, 216.0471939728780058 ) ) ;
#28511=CARTESIAN_POINT ( 'NONE',  ( -15.68560764121220252, 1410.853875961199947, 226.7268370761429992 ) ) ;
#28512=CARTESIAN_POINT ( 'NONE',  ( 5.456938789187089967, 1422.711578738400021, 123.3297044728370082 ) ) ;
#28514=CARTESIAN_POINT ( 'NONE',  ( 0.1627114960534379873, 1484.640266453030108, 181.8950381876209690 ) ) ;
#28515=CARTESIAN_POINT ( 'NONE',  ( 12.53380499169999851, 1445.052233488290085, 181.5854552579979782 ) ) ;
#28517=CARTESIAN_POINT ( 'NONE',  ( -0.5620977655390000383, 1416.851343894929869, 227.7685710125980165 ) ) ;
#28523=ORIENTED_EDGE ( 'NONE', *, *, #96527, .T. ) ;
#28528=CARTESIAN_POINT ( 'NONE',  ( -2.674529714745956355, 1509.030966574465992, 238.5990776960643132 ) ) ;
#28530=CARTESIAN_POINT ( 'NONE',  ( -11.60004869885203860, 1426.765778568870473, 134.3812644074278069 ) ) ;
#28532=DIRECTION ( 'NONE',  ( 0.6840490078599928969, -0.2249866269914024275, -0.6938717262727969182 ) ) ;
#28533=CARTESIAN_POINT ( 'NONE',  ( 11.17685589271990132, 1409.303364787639794, 219.0471118356899751 ) ) ;
#28536=CARTESIAN_POINT ( 'NONE',  ( -17.93301568280000069, 1421.479046128729806, 192.7257549160979977 ) ) ;
#28539=B_SPLINE_CURVE_WITH_KNOTS ( 'NONE', 3,
 ( #11193, #28530, #90625, #89530, #47543, #38033, #65460, #64908, #73852, #4968, #5531, #39684, #22851, #22294, #56496, #21189 ),
 .UNSPECIFIED., .F., .F.,
 ( 4, 2, 2, 2, 2, 2, 2, 4 ),
 ( 0.000000000000000000, 6.242631834405030047E-05, 0.0001248526366881006009, 0.0002497052733760278379, 0.0004994105467520596874, 0.0009988210935039975105, 0.001997642187007867085, 0.003995284374015670853 ),
 .UNSPECIFIED. ) ;
#28541=EDGE_CURVE ( 'NONE', #9907, #19921, #90400, .T. ) ;
#28544=CARTESIAN_POINT ( 'NONE',  ( -12.17244369484309985, 1416.196255300809980, 194.7590107260170100 ) ) ;
#28545=CARTESIAN_POINT ( 'NONE',  ( -11.95703516740000083, 1433.553083509069893, 150.3051793736979960 ) ) ;
#28547=CARTESIAN_POINT ( 'NONE',  ( 27.65869848730375580, 1463.963929344026837, 269.4462227895727437 ) ) ;
#28549=CARTESIAN_POINT ( 'NONE',  ( -0.04898381728909999983, 1396.985963199730122, 221.9366346587979706 ) ) ;
#28553=CARTESIAN_POINT ( 'NONE',  ( 6.280317093924558058, 1507.235120824685737, 235.5599512983970669 ) ) ;
#28557=B_SPLINE_SURFACE_WITH_KNOTS ( 'NONE', 5, 5, ( 
 ( #108546, #75521, #93936, #92841, #8275, #31837 ),
 ( #58161, #17202, #92291, #59271, #109655, #49762 ),
 ( #41896, #66022, #7735, #101777, #15014, #15561 ),
 ( #100145, #23431, #91740, #32931, #6636, #32397 ),
 ( #7197, #68232, #49212, #41354, #42440, #74968 ),
 ( #59816, #100683, #67120, #101221, #24519, #50852 ),
 ( #58709, #16117, #76053, #110196, #16655, #33470 ),
 ( #93389, #76599, #110750, #34041, #102338, #25625 ),
 ( #51398, #19998, #70443, #36255, #60931, #77168 ) ),
 .UNSPECIFIED., .F., .F., .F.,
 ( 6, 3, 6 ),
 ( 6, 6 ),
 ( 51.68681987850000326, 64.13305301190000307, 71.37864106410030729 ),
 ( -0.0007601185783282820218, 2.000000000000000000 ),
 .UNSPECIFIED. ) ;
#28558=CARTESIAN_POINT ( 'NONE',  ( 0.5620975286139998639, 1416.851343894929869, 190.4751211476980188 ) ) ;
#28559=CARTESIAN_POINT ( 'NONE',  ( -0.3719917208641120299, 1456.560529944520113, 189.3260140039109842 ) ) ;
#28561=CARTESIAN_POINT ( 'NONE',  ( 41.28926753630349822, 1444.140857746640222, 136.6209720351870089 ) ) ;
#28563=CARTESIAN_POINT ( 'NONE',  ( 19.16279675359999857, 1411.291488917830065, 262.3396920791980165 ) ) ;
#28564=CARTESIAN_POINT ( 'NONE',  ( -25.67898337120000107, 1449.805023464449960, 208.3992226959499874 ) ) ;
#28565=CARTESIAN_POINT ( 'NONE',  ( -9.946004468827549516, 1425.248700426040159, 91.15452372544520188 ) ) ;
#28568=B_SPLINE_CURVE_WITH_KNOTS ( 'NONE', 1,
 ( #74862, #109006 ),
 .UNSPECIFIED., .F., .F.,
 ( 2, 2 ),
 ( 0.000000000000000000, 1.000000000000000000 ),
 .UNSPECIFIED. ) ;
#28570=CARTESIAN_POINT ( 'NONE',  ( -5.442004254910000505, 1413.088571900130091, 250.5651368536980215 ) ) ;
#28571=CARTESIAN_POINT ( 'NONE',  ( 20.38555278956989980, 1509.665894582069996, 230.7615064735390149 ) ) ;
#28573=CARTESIAN_POINT ( 'NONE',  ( 31.77002005290000142, 1451.803664145230186, 134.7784598387979997 ) ) ;
#28576=CARTESIAN_POINT ( 'NONE',  ( 11.63092933939999973, 1509.332558450729948, 236.5028663931980191 ) ) ;
#28580=FACE_OUTER_BOUND ( 'NONE', #83744, .T. ) ;
#28582=DIRECTION ( 'NONE',  ( -0.4794256325653583617, -1.076139176629626574E-09, -0.8775825105591531505 ) ) ;
#28584=CARTESIAN_POINT ( 'NONE',  ( 0.4834647446390000214, 1450.896177426419854, 181.9315483554979949 ) ) ;
#28585=CARTESIAN_POINT ( 'NONE',  ( -6.683495332149999690, 1479.767561397530017, 234.4915808808979989 ) ) ;
#28587=VERTEX_POINT ( 'NONE', #56978 ) ;
#28588=CARTESIAN_POINT ( 'NONE',  ( 11.73707087880000088, 1426.695959143629807, 144.1731741463979972 ) ) ;
#28590=FACE_OUTER_BOUND ( 'NONE', #51249, .T. ) ;
#28591=VERTEX_POINT ( 'NONE', #99490 ) ;
#28593=ORIENTED_EDGE ( 'NONE', *, *, #2873, .F. ) ;
#28594=CARTESIAN_POINT ( 'NONE',  ( 11.83743466531329958, 1430.378478851539967, 149.6260558822839926 ) ) ;
#28600=CARTESIAN_POINT ( 'NONE',  ( -1.465793917108519917, 1484.360957496709943, 182.4810413606819850 ) ) ;
#28602=( BOUNDED_SURFACE ( )  B_SPLINE_SURFACE ( 3, 2, ( 
 ( #74645, #83031, #75198 ),
 ( #39375, #5787, #101453 ),
 ( #32073, #33166, #84122 ),
 ( #74097, #109349, #73550 ),
 ( #49443, #81916, #66264 ),
 ( #6322, #109886, #108781 ),
 ( #32630, #107684, #67356 ),
 ( #13593, #23666, #31513 ) ),
 .UNSPECIFIED., .F., .F., .F. ) 
 B_SPLINE_SURFACE_WITH_KNOTS ( ( 4, 2, 2, 4 ),
 ( 3, 3 ),
 ( -1.766815860282378026E-15, 0.004949486174159700019, 0.007424229261240433871, 0.009898972348321167722 ),
 ( 0.000000000000000000, 1.000000000000000000 ),
 .UNSPECIFIED. ) 
 GEOMETRIC_REPRESENTATION_ITEM ( )  RATIONAL_B_SPLINE_SURFACE ( (
 ( 1.000000000000000000, 0.7008167338404790447, 1.000000000000000000),
 ( 1.000000000000000000, 0.6998717715541517004, 1.000000000000000000),
 ( 1.000000000000000000, 0.6996362482572846542, 1.000000000000000000),
 ( 1.000000000000000000, 0.6996543733527801345, 1.000000000000000000),
 ( 1.000000000000000000, 0.6997206268242501803, 1.000000000000000000),
 ( 1.000000000000000000, 0.6997875685291419234, 1.000000000000000000),
 ( 1.000000000000000000, 0.6997874718065202337, 1.000000000000000000),
 ( 1.000000000000000000, 0.6996393088224879264, 1.000000000000000000) ) ) 
 REPRESENTATION_ITEM ( '' )  SURFACE ( )  );
#28604=CARTESIAN_POINT ( 'NONE',  ( -4.255765417200000122, 1424.084099830230116, 185.1505376682980000 ) ) ;
#28606=CARTESIAN_POINT ( 'NONE',  ( 3.511242806360000301, 1408.661939287229870, 270.4277067456980035 ) ) ;
#28618=CARTESIAN_POINT ( 'NONE',  ( 30.40113727430000168, 1433.623945461559742, 255.3819207742980097 ) ) ;
#28620=CARTESIAN_POINT ( 'NONE',  ( 13.06732508390000014, 1434.812095170660086, 149.1115247062979847 ) ) ;
#28628=CARTESIAN_POINT ( 'NONE',  ( -24.86063957340000030, 1443.226756493010043, 210.5718459218879843 ) ) ;
#28629=CARTESIAN_POINT ( 'NONE',  ( -2.200595920237713443, 1449.951443106519264, 154.3737305154650414 ) ) ;
#28632=LINE ( 'NONE', #70674, #4419 ) ;
#28633=CARTESIAN_POINT ( 'NONE',  ( 19.56575328779210210, 1509.675102991920312, 232.0410837715500065 ) ) ;
#28634=DIRECTION ( 'NONE',  ( 0.000000000000000000, 0.000000000000000000, 1.000000000000000000 ) ) ;
#28635=CARTESIAN_POINT ( 'NONE',  ( 12.03371223569974546, 1433.763409174216577, 149.8203876007945041 ) ) ;
#28636=CARTESIAN_POINT ( 'NONE',  ( 7.307429526299999978, 1412.733471104129876, 230.8457520919979800 ) ) ;
#28638=CARTESIAN_POINT ( 'NONE',  ( -16.16439218409000134, 1459.158912558008069, 229.6201563168629889 ) ) ;
#28641=CARTESIAN_POINT ( 'NONE',  ( 45.45312728100000044, 1434.909613172649870, 268.5145791497980099 ) ) ;
#28642=CARTESIAN_POINT ( 'NONE',  ( -17.06951414919999621, 1409.509140956229885, 223.5446133271979932 ) ) ;
#28643=B_SPLINE_CURVE_WITH_KNOTS ( 'NONE', 5,
 ( #97747, #44609, #103943, #70939, #71498, #54678 ),
 .UNSPECIFIED., .F., .F.,
 ( 6, 6 ),
 ( 0.000000000000000000, 1.000000000000000000 ),
 .UNSPECIFIED. ) ;
#28644=CARTESIAN_POINT ( 'NONE',  ( 17.84168301100000065, 1435.550183323570081, 147.0878683823979998 ) ) ;
#28646=CARTESIAN_POINT ( 'NONE',  ( 20.59881216440000173, 1488.586115637029934, 191.4156880852980009 ) ) ;
#28647=CARTESIAN_POINT ( 'NONE',  ( 29.58091120952471087, 1509.965401515384656, 207.4724573392817035 ) ) ;
#28649=CARTESIAN_POINT ( 'NONE',  ( -17.14836123659999600, 1420.862901227730163, 226.7325726209979848 ) ) ;
#28650=DIRECTION ( 'NONE',  ( -0.4990868181313579677, -0.2476038100682859955, 0.8304244102910179892 ) ) ;
#28651=CARTESIAN_POINT ( 'NONE',  ( -40.15194941080000035, 1442.235659217200009, 136.9582246599980238 ) ) ;
#28652=CARTESIAN_POINT ( 'NONE',  ( 27.43355929049999986, 1507.980920699130138, 207.4175378521480013 ) ) ;
#28653=CARTESIAN_POINT ( 'NONE',  ( -18.12194535329999923, 1416.217772597929979, 205.1982926197480026 ) ) ;
#28655=CARTESIAN_POINT ( 'NONE',  ( -12.37413385660000031, 1442.559515703879924, 186.8960802690980074 ) ) ;
#28657=CARTESIAN_POINT ( 'NONE',  ( 13.50155420149999941, 1434.968988600800230, 146.4346117040979891 ) ) ;
#28658=CARTESIAN_POINT ( 'NONE',  ( -33.53719532080000221, 1435.668427015990119, 135.5141658639980164 ) ) ;
#28659=FACE_OUTER_BOUND ( 'NONE', #25818, .T. ) ;
#28662=CARTESIAN_POINT ( 'NONE',  ( -10.10721564661269944, 1409.266012135149822, 220.1412772847010046 ) ) ;
#28664=CARTESIAN_POINT ( 'NONE',  ( 7.000000000000000000, 1432.413060387330006, 146.1721969590979882 ) ) ;
#28665=CARTESIAN_POINT ( 'NONE',  ( -4.554264956864240155, 1421.567767465303632, 137.7199131393125526 ) ) ;
#28666=CARTESIAN_POINT ( 'NONE',  ( -37.64035307139999986, 1461.657675810230103, 268.7654384304980226 ) ) ;
#28667=CARTESIAN_POINT ( 'NONE',  ( -17.20774676790000157, 1505.417530106830100, 224.1865155378980035 ) ) ;
#28668=CARTESIAN_POINT ( 'NONE',  ( 0.2427754188691099713, 1419.580316797580053, 184.3807419939530234 ) ) ;
#28673=CARTESIAN_POINT ( 'NONE',  ( 14.33002530890000159, 1414.913060387329779, 216.6125821906579745 ) ) ;
#28674=CARTESIAN_POINT ( 'NONE',  ( 13.91144599429999928, 1452.416393839029979, 223.0990526455979932 ) ) ;
#28680=CARTESIAN_POINT ( 'NONE',  ( 3.014988837336279204, 1420.039847312813663, 137.0999999980979851 ) ) ;
#28682=CARTESIAN_POINT ( 'NONE',  ( -11.68483146220000002, 1415.296882296330068, 195.2371074489979890 ) ) ;
#28683=AXIS2_PLACEMENT_3D ( 'NONE', #83382, #66071, #99072 ) ;
#28686=CARTESIAN_POINT ( 'NONE',  ( 22.00569631529999981, 1409.681516235830031, 211.9427731882580304 ) ) ;
#28687=B_SPLINE_SURFACE_WITH_KNOTS ( 'NONE', 5, 5, ( 
 ( #78632, #833, #19241, #53451, #103829, #110569, #27675, #93741, #69144 ),
 ( #61315, #8646, #103248, #95980, #8098, #34415, #42266, #18696, #27129 ),
 ( #52893, #42821, #26559, #76981, #1947, #68588, #102692, #60752, #69710 ),
 ( #25987, #9761, #60187, #94875, #94304, #86468, #18152, #52347, #43926 ),
 ( #78072, #87022, #1375, #35518, #47237, #62412, #3057, #10884, #79200 ),
 ( #62983, #97094, #45056, #96539, #105491, #20907, #88149, #81364, #12528 ),
 ( #46706, #38817, #98728, #98176, #2506, #28782, #4678, #19813, #37183 ),
 ( #36627, #107131, #20359, #54564, #70825, #54019, #88698, #55109, #11437 ),
 ( #80836, #72994, #11979, #46160, #71933, #97638, #87596, #80291, #71380 ),
 ( #37729, #64057, #3606, #89233, #106045, #29322, #21989, #63522, #4144 ),
 ( #45608, #104937, #38268, #72453, #28224, #106583, #29870, #21446, #55656 ),
 ( #79750, #89779, #30422, #13048, #64609, #49990, #22539, #99817, #13597 ),
 ( #39379, #58395, #15256, #56741, #100911, #67360, #40475, #49447, #48350 ),
 ( #107688, #5226, #41591, #90877, #33170, #75202, #109353, #92521, #91981 ),
 ( #56181, #100385, #108230, #14165, #109890, #23670, #57315, #32078, #75746 ),
 ( #91442, #101457, #90319, #41024, #47786, #81921, #73554, #65699, #57853 ),
 ( #99261, #48908, #30972, #65148, #82489, #5791, #66810, #32634, #39932 ),
 ( #83571, #74101, #31517, #23111, #6864, #24209, #14718, #83035, #15789 ),
 ( #84126, #7425, #108786, #6326, #74650, #66268, #95298, #102564, #103120 ),
 ( #17447, #1812, #94736, #59502, #70134, #85222, #699, #69015, #103692 ),
 ( #34279, #16892, #35948, #102018, #93075, #26421, #78498, #16349, #7971 ),
 ( #25857, #9081, #34828, #24746, #68460, #51097, #93613, #85782, #1246 ),
 ( #60614, #157, #60058, #58945, #51645, #94176, #18559, #67910, #50547 ),
 ( #43248, #84672, #18014, #42688, #9620, #52207, #52753, #43789, #110438 ),
 ( #42138, #86886, #77397, #10180, #76845, #86334, #77939, #35384, #8514 ),
 ( #69573, #26992, #61181, #44355, #76288, #33717, #25301, #20224, #2372 ),
 ( #105351, #70684, #36487, #104797, #96401, #37034, #71229, #55508, #53312 ),
 ( #106447, #44920, #89636, #21303, #19108, #87454, #2917, #10748, #38134 ),
 ( #88019, #28084, #79067, #3462, #4009, #46012, #12923, #89091, #29730 ),
 ( #47103, #88558, #81229, #62272, #11303, #37590, #28641, #62845, #71792 ),
 ( #19677, #4544, #54964, #105911, #53882, #96958, #63916, #38678, #29190 ),
 ( #45471, #63381, #97497, #98031, #54425, #104246, #27536, #79613, #61719 ),
 ( #12378, #95841, #46565, #11841, #80143, #20765, #80699, #72315, #100772 ) ),
 .UNSPECIFIED., .F., .F., .F.,
 ( 6, 3, 3, 3, 3, 3, 3, 3, 3, 3, 6 ),
 ( 6, 3, 6 ),
 ( 24.21111657910000048, 25.10793423650000022, 26.03050881489999924, 28.79878516220000151, 31.56706150950000023, 38.94765790310000142, 55.51095904740000009, 72.07426019160000408, 88.69155109330000641, 122.0027592590000012, 143.4996508910000159 ),
 ( 0.000000000000000000, 1.000000000000000000, 2.000000000000000000 ),
 .UNSPECIFIED. ) ;
#28690=CARTESIAN_POINT ( 'NONE',  ( -5.385042926340570801, 1432.007300083129849, 154.5986668458859867 ) ) ;
#28693=CARTESIAN_POINT ( 'NONE',  ( 0.7201256557630000277, 1415.745261378530131, 233.3682385266980077 ) ) ;
#28698=CARTESIAN_POINT ( 'NONE',  ( -20.33636649369999816, 1427.581624735430069, 223.9337651306980206 ) ) ;
#28699=CARTESIAN_POINT ( 'NONE',  ( -18.41867143110519933, 1486.196793196990029, 188.8168638707130071 ) ) ;
#28706=CARTESIAN_POINT ( 'NONE',  ( 27.78683896639999773, 1509.618348729030004, 214.6924127718480122 ) ) ;
#28707=ORIENTED_EDGE ( 'NONE', *, *, #15751, .F. ) ;
#28710=CARTESIAN_POINT ( 'NONE',  ( -15.68560764121220252, 1410.853875961199947, 226.7268370761429992 ) ) ;
#28711=CARTESIAN_POINT ( 'NONE',  ( 1.539395910930000166, 1508.628951913829951, 180.5172630586980063 ) ) ;
#28713=CARTESIAN_POINT ( 'NONE',  ( -25.20238731644419872, 1451.152274905429977, 137.4649534155230128 ) ) ;
#28714=CARTESIAN_POINT ( 'NONE',  ( 9.055564386196214954, 1440.382423718937844, 153.5303063279175433 ) ) ;
#28715=CARTESIAN_POINT ( 'NONE',  ( 13.40311307709999866, 1409.883220066930107, 228.1200985806979702 ) ) ;
#28717=CARTESIAN_POINT ( 'NONE',  ( 41.53765979141579834, 1445.128430570580122, 134.0999999984609872 ) ) ;
#28719=CARTESIAN_POINT ( 'NONE',  ( -11.36018337610000195, 1414.996442546130083, 195.9645814914979951 ) ) ;
#28727=FACE_OUTER_BOUND ( 'NONE', #685, .T. ) ;
#28729=CARTESIAN_POINT ( 'NONE',  ( 15.10981120460822957, 1451.148210361404836, 149.6511074968155981 ) ) ;
#28730=CARTESIAN_POINT ( 'NONE',  ( -3.008276117979999942, 1485.138067935930167, 183.1683143970979870 ) ) ;
#28734=CARTESIAN_POINT ( 'NONE',  ( 4.251649916467110657, 1446.494082692860047, 160.8451567543189924 ) ) ;
#28737=VERTEX_POINT ( 'NONE', #72145 ) ;
#28740=CARTESIAN_POINT ( 'NONE',  ( 26.52681755028470079, 1440.913060387330006, 243.7300046518169836 ) ) ;
#28741=CARTESIAN_POINT ( 'NONE',  ( -16.93968655440000148, 1509.443694557030085, 185.0606162848980034 ) ) ;
#28743=CARTESIAN_POINT ( 'NONE',  ( 26.57123036162979801, 1448.090663227739924, 137.0341373801179827 ) ) ;
#28744=CARTESIAN_POINT ( 'NONE',  ( -13.57503295039999891, 1410.760072987729927, 189.9862946811979896 ) ) ;
#28746=CARTESIAN_POINT ( 'NONE',  ( -24.39265439800000124, 1441.035345296090100, 211.3385326736879790 ) ) ;
#28752=CARTESIAN_POINT ( 'NONE',  ( -11.94130205119999921, 1433.615242452219945, 148.5637080951979669 ) ) ;
#28753=CARTESIAN_POINT ( 'NONE',  ( 23.61230825720000226, 1435.322028862560046, 137.2857987807979896 ) ) ;
#28754=CARTESIAN_POINT ( 'NONE',  ( 12.23138524880000055, 1463.686947130230010, 231.4510838504980086 ) ) ;
#28759=CARTESIAN_POINT ( 'NONE',  ( 29.12559690860000217, 1509.873774306529867, 207.7706034996080007 ) ) ;
#28761=EDGE_CURVE ( 'NONE', #69813, #7138, #105093, .T. ) ;
#28762=CARTESIAN_POINT ( 'NONE',  ( -18.34422345790000008, 1416.813004075630033, 208.8605758367380076 ) ) ;
#28768=CARTESIAN_POINT ( 'NONE',  ( -1.133866162019999861E-09, 1468.084175535529994, 248.5896189568980219 ) ) ;
#28770=CARTESIAN_POINT ( 'NONE',  ( -11.57713237839999998, 1432.387637135029991, 151.1965105832979930 ) ) ;
#28772=EDGE_CURVE ( 'NONE', #23409, #47384, #63667, .T. ) ;
#28773=CARTESIAN_POINT ( 'NONE',  ( -0.2885899904230180280, 1507.883288131039990, 237.4859410355080058 ) ) ;
#28774=CARTESIAN_POINT ( 'NONE',  ( -19.13404846440000284, 1457.718989482430061, 226.6686308623980040 ) ) ;
#28775=B_SPLINE_CURVE_WITH_KNOTS ( 'NONE', 5,
 ( #26572, #61877, #44502, #95448, #87041, #18168, #86483, #27692, #9779 ),
 .UNSPECIFIED., .F., .F.,
 ( 6, 3, 6 ),
 ( 0.000000000000000000, 0.5000000000000000000, 1.000000000000000000 ),
 .UNSPECIFIED. ) ;
#28776=CARTESIAN_POINT ( 'NONE',  ( -21.30784275718657028, 1411.017705672756620, 200.6768285256719082 ) ) ;
#28777=CARTESIAN_POINT ( 'NONE',  ( 2.500000000000000000, 1432.353950668519929, 157.4944280282979889 ) ) ;
#28780=ORIENTED_EDGE ( 'NONE', *, *, #46294, .T. ) ;
#28782=CARTESIAN_POINT ( 'NONE',  ( 0.8851054190410000411, 1406.072537395830068, 269.0453913371979979 ) ) ;
#28785=CARTESIAN_POINT ( 'NONE',  ( 6.516345065877910514, 1472.619501843580110, 270.3713698276869195 ) ) ;
#28786=CARTESIAN_POINT ( 'NONE',  ( 2.478932746460000391, 1432.564745886140145, 157.5224116325979935 ) ) ;
#28788=CARTESIAN_POINT ( 'NONE',  ( 11.60004869885203682, 1422.222932908421853, 135.5999999980979567 ) ) ;
#28791=CARTESIAN_POINT ( 'NONE',  ( -43.11122459500789716, 1440.913060409440050, 263.3173459173530091 ) ) ;
#28795=CARTESIAN_POINT ( 'NONE',  ( 14.41619641355878478, 1509.538862670986418, 235.4310391072028494 ) ) ;
#28801=CARTESIAN_POINT ( 'NONE',  ( -11.06589456070000033, 1424.668795903030286, 234.3916895697979612 ) ) ;
#28804=CARTESIAN_POINT ( 'NONE',  ( -0.7749238296759999312, 1475.832189872029858, 266.9609160975979876 ) ) ;
#28805=CARTESIAN_POINT ( 'NONE',  ( -4.288435981061489599, 1446.932127814390014, 155.2226307056990038 ) ) ;
#28808=CARTESIAN_POINT ( 'NONE',  ( -18.58720762869999987, 1416.311719779230089, 208.5274638254259969 ) ) ;
#28810=CARTESIAN_POINT ( 'NONE',  ( 26.68805691732229946, 1436.277521234780124, 136.6581429669300007 ) ) ;
#28811=CARTESIAN_POINT ( 'NONE',  ( -7.475863647388560018, 1396.174123299650091, 217.2595793039530179 ) ) ;
#28814=CARTESIAN_POINT ( 'NONE',  ( -15.23090723337400121, 1422.122923179038025, 227.7537106409200192 ) ) ;
#28815=CARTESIAN_POINT ( 'NONE',  ( -16.08386308296240230, 1409.482933452620046, 225.3901198913439998 ) ) ;
#28816=CARTESIAN_POINT ( 'NONE',  ( -44.91834551880000248, 1440.343506779659947, 269.6914828722979678 ) ) ;
#28821=CARTESIAN_POINT ( 'NONE',  ( -19.06723915664710134, 1485.490521620860136, 189.6150037022410118 ) ) ;
#28822=CARTESIAN_POINT ( 'NONE',  ( 11.51812271839999902, 1426.832871545830130, 128.4954513222980097 ) ) ;
#28824=DIRECTION ( 'NONE',  ( 0.000000000000000000, 0.000000000000000000, -1.000000000000000000 ) ) ;
#28825=CARTESIAN_POINT ( 'NONE',  ( -12.53380498098199602, 1442.773887284840612, 205.2015002797237173 ) ) ;
#28828=CARTESIAN_POINT ( 'NONE',  ( -2.424063131930000115, 1427.257651041929876, 147.9020499575979954 ) ) ;
#28829=CARTESIAN_POINT ( 'NONE',  ( 3.573194667510000144, 1509.053513020129913, 179.7696517855980005 ) ) ;
#28830=CARTESIAN_POINT ( 'NONE',  ( 0.04548916784448110012, 1416.835419214280137, 190.9576572557899965 ) ) ;
#28832=VECTOR ( 'NONE', #96549, 1000.000000000000000 ) ;
#28835=CARTESIAN_POINT ( 'NONE',  ( -1.835915877731372658, 1464.997577545588001, 237.8268834563425287 ) ) ;
#28836=VERTEX_POINT ( 'NONE', #41808 ) ;
#28838=CARTESIAN_POINT ( 'NONE',  ( -8.582734512730000986, 1398.167885046430001, 198.9971942070980049 ) ) ;
#28839=CARTESIAN_POINT ( 'NONE',  ( -15.43255204080000098, 1409.451976979829851, 192.6616394286979812 ) ) ;
#28840=CARTESIAN_POINT ( 'NONE',  ( 11.34090880850000005, 1475.513060387329915, 227.1982711657979905 ) ) ;
#28843=CARTESIAN_POINT ( 'NONE',  ( -1.363077736744499946, 1415.332184859939844, 185.3921874643629906 ) ) ;
#28844=B_SPLINE_CURVE_WITH_KNOTS ( 'NONE', 3,
 ( #93547, #76767, #76218, #42067, #51574, #74178, #99334, #94104, #38882, #5859, #51021, #108308, #102499, #22608, #101945, #47854, #93003, #64682, #65770 ),
 .UNSPECIFIED., .F., .F.,
 ( 4, 2, 1, 2, 2, 2, 2, 2, 2, 4 ),
 ( 0.000000000000000000, 0.1250000000001602329, 0.1875000000002953748, 0.2187500000003569645, 0.2500000000004185541, 0.3750000000005341283, 0.4375000000005920264, 0.5000000000006499246, 0.7500000000003249623, 1.000000000000000000 ),
 .UNSPECIFIED. ) ;
#28845=CARTESIAN_POINT ( 'NONE',  ( 10.74246380849999838, 1429.760558640729869, 188.0236792812979729 ) ) ;
#28847=CARTESIAN_POINT ( 'NONE',  ( -38.72664573631579543, 1449.455593765829917, 136.0882868071720395 ) ) ;
#28848=CARTESIAN_POINT ( 'NONE',  ( -2.500000000000000000, 1448.201359996650126, 168.5754994529100088 ) ) ;
#28850=DIRECTION ( 'NONE',  ( 0.000000000000000000, 6.429979419034159461E-12, -1.000000000000000000 ) ) ;
#28851=CARTESIAN_POINT ( 'NONE',  ( -5.353064078697809869, 1406.074448326960010, 267.2230922050150070 ) ) ;
#28852=DIRECTION ( 'NONE',  ( 0.000000000000000000, 0.000000000000000000, -1.000000000000000000 ) ) ;
#28853=VERTEX_POINT ( 'NONE', #68149 ) ;
#28854=DIRECTION ( 'NONE',  ( -0.9822959463204248287, 0.1391731009605849945, -0.1254014426211909616 ) ) ;
#28855=CARTESIAN_POINT ( 'NONE',  ( 12.81356597149999921, 1442.366100173290079, 188.3022465221979758 ) ) ;
#28856=ORIENTED_EDGE ( 'NONE', *, *, #45319, .T. ) ;
#28857=ORIENTED_EDGE ( 'NONE', *, *, #75568, .T. ) ;
#28858=ADVANCED_FACE ( 'NONE', ( #109573 ), #109892, .F. ) ;
#28859=CARTESIAN_POINT ( 'NONE',  ( 0.03326177659115069768, 1408.911898860609881, 187.0499707311110171 ) ) ;
#28865=ORIENTED_EDGE ( 'NONE', *, *, #44711, .T. ) ;
#28866=CARTESIAN_POINT ( 'NONE',  ( 2.500000000000039968, 1448.773875821790170, 156.9803059956940103 ) ) ;
#28868=AXIS2_PLACEMENT_3D ( 'NONE', #60285, #61406, #94404 ) ;
#28872=CARTESIAN_POINT ( 'NONE',  ( -41.71656132900650960, 1437.001393571195194, 269.6421165700213578 ) ) ;
#28873=CARTESIAN_POINT ( 'NONE',  ( -10.71339925790000080, 1409.287180533330002, 227.5724378756979718 ) ) ;
#28880=EDGE_CURVE ( 'NONE', #30887, #25245, #58251, .T. ) ;
#28881=CARTESIAN_POINT ( 'NONE',  ( 41.20035157204440424, 1427.456943461399987, 270.1350674680870156 ) ) ;
#28884=CARTESIAN_POINT ( 'NONE',  ( 0.02009666217332761046, 1507.207408199481961, 237.3586634061521750 ) ) ;
#28887=EDGE_CURVE ( 'NONE', #68290, #105027, #89990, .T. ) ;
#28891=CARTESIAN_POINT ( 'NONE',  ( -12.94419629340000100, 1420.439331177430176, 228.3355065355980003 ) ) ;
#28893=EDGE_CURVE ( 'NONE', #101455, #28836, #67427, .T. ) ;
#28898=CARTESIAN_POINT ( 'NONE',  ( 18.65451742820949832, 1507.632629731499947, 188.5326158842280222 ) ) ;
#28900=CARTESIAN_POINT ( 'NONE',  ( -0.1880784674069999884, 1408.919628232130208, 231.7730996565980206 ) ) ;
#28901=CARTESIAN_POINT ( 'NONE',  ( -0.1168129828940950021, 1420.457736004669869, 182.7197010214190129 ) ) ;
#28908=CARTESIAN_POINT ( 'NONE',  ( -12.95840410776020057, 1416.218047878440075, 196.6656636057070102 ) ) ;
#28914=DIRECTION ( 'NONE',  ( -1.000000000000000000, 0.000000000000000000, -1.989567262110869994E-13 ) ) ;
#28919=CARTESIAN_POINT ( 'NONE',  ( -27.81797958387629777, 1509.852926761900108, 200.9687172335360117 ) ) ;
#28920=CARTESIAN_POINT ( 'NONE',  ( -2.500000000000000000, 1448.197706736029886, 167.4845663601980164 ) ) ;
#28921=CARTESIAN_POINT ( 'NONE',  ( -18.07950054330000000, 1423.749692319529913, 225.6737955892980096 ) ) ;
#28922=CARTESIAN_POINT ( 'NONE',  ( -18.37019422750000075, 1435.283622672170168, 146.1498534422979958 ) ) ;
#28924=CARTESIAN_POINT ( 'NONE',  ( -2.500000000000000000, 1439.615672362369878, 170.5246407198980023 ) ) ;
#28925=CARTESIAN_POINT ( 'NONE',  ( 0.4455705167121439825, 1409.096190068570195, 232.6073811540130123 ) ) ;
#28926=CARTESIAN_POINT ( 'NONE',  ( -18.59402987153349684, 1437.048336213511902, 212.3086441927383134 ) ) ;
#28928=CARTESIAN_POINT ( 'NONE',  ( -0.04830720914946320249, 1457.855805554629796, 229.0971631259880041 ) ) ;
#28929=VERTEX_POINT ( 'NONE', #75951 ) ;
#28932=EDGE_CURVE ( 'NONE', #43923, #64525, #41791, .T. ) ;
#28933=CARTESIAN_POINT ( 'NONE',  ( -23.78094776239999675, 1436.491024829749904, 211.7413630244279830 ) ) ;
#28934=CARTESIAN_POINT ( 'NONE',  ( -20.83094015030000179, 1452.185627928030044, 134.0999999980979851 ) ) ;
#28935=CARTESIAN_POINT ( 'NONE',  ( -18.62446834819999708, 1507.629699710430032, 229.7127857518979965 ) ) ;
#28937=CARTESIAN_POINT ( 'NONE',  ( 12.84239221398829933, 1435.935692713660046, 150.8114773724069835 ) ) ;
#28939=CARTESIAN_POINT ( 'NONE',  ( -16.81223226430000039, 1414.913060387329779, 207.5743821216680089 ) ) ;
#28947=CARTESIAN_POINT ( 'NONE',  ( 21.87325955929999921, 1509.710279403030199, 189.0200286462979875 ) ) ;
#28951=ORIENTED_EDGE ( 'NONE', *, *, #17206, .T. ) ;
#28956=CARTESIAN_POINT ( 'NONE',  ( 35.03185245808725767, 1424.085991366112466, 269.5319528758505498 ) ) ;
#28957=CARTESIAN_POINT ( 'NONE',  ( -34.48978217770000043, 1443.099005945160116, 250.0021841883980471 ) ) ;
#28959=CARTESIAN_POINT ( 'NONE',  ( -11.93337251310000013, 1433.461400490700044, 149.9038012133979976 ) ) ;
#28960=VECTOR ( 'NONE', #46905, 1000.000000000000114 ) ;
#28961=CARTESIAN_POINT ( 'NONE',  ( 27.50468030500000083, 1509.873544990630080, 201.6580215447480100 ) ) ;
#28962=CARTESIAN_POINT ( 'NONE',  ( -19.04715201249999978, 1486.119048487729970, 189.4490706170979877 ) ) ;
#28963=CARTESIAN_POINT ( 'NONE',  ( 11.42779433089999941, 1410.681993053729911, 189.4262149395979975 ) ) ;
#28964=CARTESIAN_POINT ( 'NONE',  ( 4.776594320200000077, 1423.601635148929972, 184.0375701292979898 ) ) ;
#28966=CARTESIAN_POINT ( 'NONE',  ( 6.686616336669999328, 1441.247407971460007, 154.4574208692980051 ) ) ;
#28967=CARTESIAN_POINT ( 'NONE',  ( 13.15339637540530049, 1428.694520551590131, 223.1160257848979995 ) ) ;
#28968=CARTESIAN_POINT ( 'NONE',  ( 0.01367056495459999937, 1452.767332469230041, 153.3854680590980024 ) ) ;
#28971=ORIENTED_EDGE ( 'NONE', *, *, #56827, .T. ) ;
#28976=CARTESIAN_POINT ( 'NONE',  ( -27.88458103209999805, 1464.440568686830147, 269.9356493381980044 ) ) ;
#28978=CARTESIAN_POINT ( 'NONE',  ( 16.26032963000000109, 1409.480883610230194, 223.2931273867980053 ) ) ;
#28979=CARTESIAN_POINT ( 'NONE',  ( -15.65975627419999938, 1506.806593729730139, 224.7138568134979835 ) ) ;
#28982=DIRECTION ( 'NONE',  ( 0.000000000000000000, 1.000000000000000000, 0.000000000000000000 ) ) ;
#28983=CARTESIAN_POINT ( 'NONE',  ( -1.295008548611806143, 1484.564168690730639, 182.3200671755110420 ) ) ;
#28985=CARTESIAN_POINT ( 'NONE',  ( -43.92682917671319842, 1430.745472343149913, 266.4731560355739930 ) ) ;
#28987=CARTESIAN_POINT ( 'NONE',  ( -3.537187223599389529, 1495.340936109010045, 181.4789602020310042 ) ) ;
#28992=CARTESIAN_POINT ( 'NONE',  ( -21.33073281779999775, 1509.431426448229786, 190.3502236015980031 ) ) ;
#28993=CARTESIAN_POINT ( 'NONE',  ( -13.52632867340000189, 1425.416544542129941, 189.2536498548980148 ) ) ;
#29000=B_SPLINE_CURVE_WITH_KNOTS ( 'NONE', 5,
 ( #55122, #62428, #45069, #46174, #51359, #89245, #80303, #4154, #45624, #61874, #11448, #71942 ),
 .UNSPECIFIED., .F., .F.,
 ( 6, 3, 3, 6 ),
 ( 0.000000000000000000, 0.5001987333065609498, 0.8483151769418431076, 1.000000000000000000 ),
 .UNSPECIFIED. ) ;
#29004=VERTEX_POINT ( 'NONE', #8604 ) ;
#29005=CARTESIAN_POINT ( 'NONE',  ( -23.29476211502619876, 1412.627406204969930, 270.1903322620909762 ) ) ;
#29006=CARTESIAN_POINT ( 'NONE',  ( 3.684551893115589394, 1417.858094126330116, 234.2256683103420016 ) ) ;
#29012=B_SPLINE_CURVE_WITH_KNOTS ( 'NONE', 3,
 ( #98673, #88648, #56128, #90263, #101395, #84617 ),
 .UNSPECIFIED., .F., .F.,
 ( 4, 2, 4 ),
 ( 9.242101507433989461E-07, 0.4978491653051179688, 0.9954968279883259497 ),
 .UNSPECIFIED. ) ;
#29013=CARTESIAN_POINT ( 'NONE',  ( 44.75793395845553846, 1447.593610556694557, 268.9993686022775137 ) ) ;
#29015=CARTESIAN_POINT ( 'NONE',  ( 3.649417161288583511, 1424.955166412201606, 184.9140735895639978 ) ) ;
#29016=CARTESIAN_POINT ( 'NONE',  ( -1.525828703510382134, 1406.001374342115014, 266.9605462712685835 ) ) ;
#29017=CARTESIAN_POINT ( 'NONE',  ( -17.60066553444309889, 1415.059973079419933, 207.5652353588600079 ) ) ;
#29018=CARTESIAN_POINT ( 'NONE',  ( -18.51553952359999755, 1435.777052104869881, 225.9247619741979918 ) ) ;
#29019=CARTESIAN_POINT ( 'NONE',  ( -14.66481730340000134, 1423.493437503330142, 221.6029759380979840 ) ) ;
#29020=CARTESIAN_POINT ( 'NONE',  ( 12.33246611440000073, 1415.579607672129896, 222.7360816577980245 ) ) ;
#29021=CARTESIAN_POINT ( 'NONE',  ( 3.853748796670000143, 1447.370069209109943, 184.1245004005980093 ) ) ;
#29025=CARTESIAN_POINT ( 'NONE',  ( -13.02322703936409987, 1416.825784014559986, 196.6108461303639672 ) ) ;
#29027=CARTESIAN_POINT ( 'NONE',  ( 10.36609672684421390, 1455.263332276473875, 226.3870373070946300 ) ) ;
#29028=EDGE_CURVE ( 'NONE', #106196, #36359, #98334, .T. ) ;
#29029=CARTESIAN_POINT ( 'NONE',  ( 24.72916343099570113, 1451.812305069729973, 137.1077481279560004 ) ) ;
#29032=CARTESIAN_POINT ( 'NONE',  ( 2.416798835000000256, 1426.601114010129777, 146.0361887655980127 ) ) ;
#29033=CARTESIAN_POINT ( 'NONE',  ( 19.23829242040000054, 1410.080596241930152, 196.1913699390979957 ) ) ;
#29034=CARTESIAN_POINT ( 'NONE',  ( 23.10251669230000360, 1410.654477903330189, 207.3358591529579940 ) ) ;
#29035=CARTESIAN_POINT ( 'NONE',  ( -24.89775095376042202, 1442.835547651392517, 210.5176539946395451 ) ) ;
#29036=CARTESIAN_POINT ( 'NONE',  ( -24.22803231680000025, 1427.085958910729914, 210.4997307367480062 ) ) ;
#29039=CARTESIAN_POINT ( 'NONE',  ( 2.500000000000000000, 1439.534675992210168, 164.5282227258210241 ) ) ;
#29048=CARTESIAN_POINT ( 'NONE',  ( -38.76639204100970204, 1448.036160168320066, 136.4890662579730076 ) ) ;
#29049=CARTESIAN_POINT ( 'NONE',  ( 11.60004869885002776, 1425.287569105003968, 138.0581718968657583 ) ) ;
#29051=CARTESIAN_POINT ( 'NONE',  ( -1.756474080180989938, 1451.931903963289869, 184.1876047667690273 ) ) ;
#29052=CARTESIAN_POINT ( 'NONE',  ( 11.22179870490000120, 1433.227936539949951, 151.5695467236979823 ) ) ;
#29053=DIRECTION ( 'NONE',  ( -0.5518846470010263516, -0.8335230848462815700, -0.02574108453214526276 ) ) ;
#29054=CARTESIAN_POINT ( 'NONE',  ( -17.22540062639860281, 1409.514585605769980, 195.8673745312759991 ) ) ;
#29059=CARTESIAN_POINT ( 'NONE',  ( -1.600048698852036821, 1411.254281879943164, 134.0999999980979851 ) ) ;
#29060=CARTESIAN_POINT ( 'NONE',  ( 12.53380498098208840, 1442.773887284840384, 206.9039879563480326 ) ) ;
#29065=CIRCLE ( 'NONE', #23691, 20.82269076393892249 ) ;
#29067=CARTESIAN_POINT ( 'NONE',  ( -10.23452338969999964, 1508.269285187629748, 234.6133565388980173 ) ) ;
#29070=CARTESIAN_POINT ( 'NONE',  ( 6.448255093290000239, 1408.606950372430219, 221.0175999117980155 ) ) ;
#29071=CARTESIAN_POINT ( 'NONE',  ( -7.191383064323740193, 1407.162969927880113, 195.9581075134270236 ) ) ;
#29074=CARTESIAN_POINT ( 'NONE',  ( -1.197747051619999947, 1451.638021728929971, 183.5066748651979935 ) ) ;
#29076=CARTESIAN_POINT ( 'NONE',  ( 2.500000000000000000, 1432.302110539269961, 157.4936333739979943 ) ) ;
#29077=CARTESIAN_POINT ( 'NONE',  ( -17.94598849933589690, 1415.434635989099888, 208.4606526442179870 ) ) ;
#29078=ORIENTED_EDGE ( 'NONE', *, *, #109189, .T. ) ;
#29080=ORIENTED_EDGE ( 'NONE', *, *, #101450, .F. ) ;
#29082=CARTESIAN_POINT ( 'NONE',  ( -18.05542495199999919, 1416.825784011830137, 209.4840452931180153 ) ) ;
#29083=CARTESIAN_POINT ( 'NONE',  ( 11.47918630980880472, 1425.866204196556282, 139.0913388880763364 ) ) ;
#29087=CARTESIAN_POINT ( 'NONE',  ( 13.33898638527650071, 1409.378868052919870, 215.8521671009030172 ) ) ;
#29090=CARTESIAN_POINT ( 'NONE',  ( -19.40739355430000046, 1478.163464013930025, 190.3421420625980147 ) ) ;
#29096=CARTESIAN_POINT ( 'NONE',  ( -2.663421700517105251, 1419.688210328091600, 137.0999999980980135 ) ) ;
#29098=CARTESIAN_POINT ( 'NONE',  ( 35.04542388930794772, 1457.725280349715376, 269.5321273768489618 ) ) ;
#29099=CARTESIAN_POINT ( 'NONE',  ( -22.70509189929999749, 1409.705932116229860, 208.9454376012710100 ) ) ;
#29100=CARTESIAN_POINT ( 'NONE',  ( -0.06016800169540000021, 1397.283812744130046, 222.0600360894979701 ) ) ;
#29102=CARTESIAN_POINT ( 'NONE',  ( -0.1656437318690000271, 1467.449396149929953, 182.5917868815979830 ) ) ;
#29104=CARTESIAN_POINT ( 'NONE',  ( -25.76949925306854894, 1436.653851094284846, 137.0767669179255677 ) ) ;
#29106=CARTESIAN_POINT ( 'NONE',  ( -13.09695741303050021, 1435.388910325369807, 150.3946318658950361 ) ) ;
#29108=CARTESIAN_POINT ( 'NONE',  ( 0.5623041189709999665, 1416.835809767730098, 190.4756568789979951 ) ) ;
#29109=CYLINDRICAL_SURFACE ( 'NONE', #75141, 23.99999999999999289 ) ;
#29111=CARTESIAN_POINT ( 'NONE',  ( 41.24981031477440041, 1444.146950527760055, 136.6647296086840129 ) ) ;
#29112=EDGE_LOOP ( 'NONE', ( #86214, #74223, #52965, #77838 ) ) ;
#29113=CARTESIAN_POINT ( 'NONE',  ( 21.01922275720000144, 1409.015071317029879, 267.0603661001979958 ) ) ;
#29114=CARTESIAN_POINT ( 'NONE',  ( -26.64485081080000128, 1469.250187273330084, 209.1448408980039915 ) ) ;
#29115=CARTESIAN_POINT ( 'NONE',  ( -10.32454341532539921, 1425.433986580120063, 91.15122188942740422 ) ) ;
#29116=CARTESIAN_POINT ( 'NONE',  ( -16.87240953879999950, 1409.502257911630068, 196.1298159851979790 ) ) ;
#29118=CARTESIAN_POINT ( 'NONE',  ( -35.38895424947720159, 1419.603261908680224, 269.8627654472495578 ) ) ;
#29119=CARTESIAN_POINT ( 'NONE',  ( -36.81312562770000341, 1440.913060390769942, 254.5659314719980273 ) ) ;
#29122=CARTESIAN_POINT ( 'NONE',  ( 33.54167281650000376, 1451.588757459429871, 135.5984676536979805 ) ) ;
#29123=ORIENTED_EDGE ( 'NONE', *, *, #15837, .T. ) ;
#29126=CARTESIAN_POINT ( 'NONE',  ( 14.17717777510000055, 1509.408138344429972, 234.9453854129980073 ) ) ;
#29128=ORIENTED_EDGE ( 'NONE', *, *, #29742, .F. ) ;
#29131=ORIENTED_EDGE ( 'NONE', *, *, #51936, .T. ) ;
#29132=CARTESIAN_POINT ( 'NONE',  ( 0.09694917001379999011, 1417.474897329329906, 184.6760764755979949 ) ) ;
#29134=CARTESIAN_POINT ( 'NONE',  ( 0.3980295580039999725, 1450.899160888880260, 181.9202001828980144 ) ) ;
#29135=CARTESIAN_POINT ( 'NONE',  ( -9.606425101199999261, 1479.765168659229857, 233.3218314666980291 ) ) ;
#29138=CARTESIAN_POINT ( 'NONE',  ( 45.67158527630730447, 1440.912968828189832, 266.1883948345449653 ) ) ;
#29140=CARTESIAN_POINT ( 'NONE',  ( -12.87618670773889917, 1416.835419214280137, 221.9337012713420165 ) ) ;
#29141=CARTESIAN_POINT ( 'NONE',  ( 15.30113400989999839, 1507.624001478829996, 226.2897674745979941 ) ) ;
#29142=ORIENTED_EDGE ( 'NONE', *, *, #31676, .T. ) ;
#29145=CARTESIAN_POINT ( 'NONE',  ( 11.86473597889290055, 1432.240644767480035, 149.9815416248509905 ) ) ;
#29146=ADVANCED_FACE ( 'NONE', ( #89184 ), #77981, .F. ) ;
#29147=CARTESIAN_POINT ( 'NONE',  ( 12.85619364388517738, 1444.956372886574400, 186.6503089507870357 ) ) ;
#29155=CARTESIAN_POINT ( 'NONE',  ( 23.20970012627410028, 1452.102559799250002, 138.3498196778160150 ) ) ;
#29156=CARTESIAN_POINT ( 'NONE',  ( 0.4790140997571979975, 1409.206633244769819, 270.3713656712309898 ) ) ;
#29158=CARTESIAN_POINT ( 'NONE',  ( 11.05525581825247450, 1433.694738207780119, 151.7203265431317618 ) ) ;
#29159=CARTESIAN_POINT ( 'NONE',  ( -10.97749909317680128, 1432.820767003169749, 151.7697165876629981 ) ) ;
#29160=CARTESIAN_POINT ( 'NONE',  ( 0.03267392400940041103, 1410.103089868323195, 233.2006946390937969 ) ) ;
#29164=CARTESIAN_POINT ( 'NONE',  ( -25.32400484384510264, 1509.734017743870027, 222.9228364901310044 ) ) ;
#29166=ORIENTED_EDGE ( 'NONE', *, *, #25595, .T. ) ;
#29167=CARTESIAN_POINT ( 'NONE',  ( 19.47651264659999626, 1426.266543404630283, 243.9198229294980251 ) ) ;
#29168=CARTESIAN_POINT ( 'NONE',  ( 18.70459388984919968, 1509.566239199539950, 186.5372755781170042 ) ) ;
#29177=CARTESIAN_POINT ( 'NONE',  ( 17.40764061960000220, 1414.996442553730049, 210.6782162702180017 ) ) ;
#29178=CARTESIAN_POINT ( 'NONE',  ( -24.61293842550000122, 1444.770194088929884, 210.8869350105979947 ) ) ;
#29179=CARTESIAN_POINT ( 'NONE',  ( -1.194091358764769906, 1450.771796404168981, 154.2531665394261609 ) ) ;
#29182=CARTESIAN_POINT ( 'NONE',  ( 5.363491954609552970, 1422.300497992083137, 141.6191263096993396 ) ) ;
#29183=CARTESIAN_POINT ( 'NONE',  ( 19.65254182433579899, 1509.729709204669916, 232.1452871772020217 ) ) ;
#29184=CARTESIAN_POINT ( 'NONE',  ( -41.49257164404139786, 1443.691024955536477, 136.5669757872581442 ) ) ;
#29185=CARTESIAN_POINT ( 'NONE',  ( -2.500000000000000000, 1432.302173844710069, 157.4936352153980010 ) ) ;
#29186=CARTESIAN_POINT ( 'NONE',  ( 15.55932329569999872, 1410.406700292830010, 227.1523413082980198 ) ) ;
#29188=CARTESIAN_POINT ( 'NONE',  ( 41.66134420550000073, 1443.796851579070108, 135.6885409488979803 ) ) ;
#29190=CARTESIAN_POINT ( 'NONE',  ( 45.44661339499999997, 1436.958365765089866, 268.9799159559980239 ) ) ;
#29191=CARTESIAN_POINT ( 'NONE',  ( -18.09603717179999904, 1409.709851216229936, 223.5038430802979974 ) ) ;
#29192=EDGE_CURVE ( 'NONE', #52345, #36240, #108926, .T. ) ;
#29193=CARTESIAN_POINT ( 'NONE',  ( 16.63847852929999860, 1435.207672684450017, 147.6320463620980092 ) ) ;
#29194=CARTESIAN_POINT ( 'NONE',  ( 20.03220479750000038, 1469.158896213129992, 192.0694551358980107 ) ) ;
#29195=FACE_OUTER_BOUND ( 'NONE', #58689, .T. ) ;
#29197=CARTESIAN_POINT ( 'NONE',  ( -16.78053953839999934, 1420.867358303729816, 226.9349730632980311 ) ) ;
#29199=CARTESIAN_POINT ( 'NONE',  ( -35.96042261120520322, 1435.915483823489922, 135.4632522523019986 ) ) ;
#29202=CARTESIAN_POINT ( 'NONE',  ( -13.31488284758549945, 1407.448340439549838, 207.9555150571470108 ) ) ;
#29203=CARTESIAN_POINT ( 'NONE',  ( 2.918143513847768445E-16, 1426.814114634534008, 137.0999999980979851 ) ) ;
#29206=CARTESIAN_POINT ( 'NONE',  ( 11.94165044080000015, 1433.614891514819874, 146.7587909720979837 ) ) ;
#29207=CARTESIAN_POINT ( 'NONE',  ( -34.31734398647500228, 1435.703512753839959, 134.0999999980490145 ) ) ;
#29208=CARTESIAN_POINT ( 'NONE',  ( -0.6104134479315243000, 1418.823153084925707, 184.7568843877850782 ) ) ;
#29211=CARTESIAN_POINT ( 'NONE',  ( 27.13956170239999821, 1438.563708552820117, 136.9826111156980062 ) ) ;
#29215=CARTESIAN_POINT ( 'NONE',  ( -31.50880186010000017, 1466.258756145929965, 266.5723332967979786 ) ) ;
#29217=CARTESIAN_POINT ( 'NONE',  ( -19.79380256296796858, 1500.877691764588917, 189.1734504439409363 ) ) ;
#29218=CARTESIAN_POINT ( 'NONE',  ( -26.86204968970000095, 1508.007394745729925, 212.0120970167880046 ) ) ;
#29220=B_SPLINE_SURFACE_WITH_KNOTS ( 'NONE', 4, 5, ( 
 ( #75433, #28584, #65932, #62785, #105856, #100054 ),
 ( #97443, #96900, #54367, #74876, #54907, #39609 ),
 ( #11782, #29134, #57533, #90549, #91105, #48576 ),
 ( #5449, #91657, #14931, #22769, #48012, #14383 ),
 ( #82150, #107903, #109027, #100599, #45949, #32309 ) ),
 .UNSPECIFIED., .F., .F., .F.,
 ( 5, 5 ),
 ( 6, 6 ),
 ( 7.045302831979999958, 7.554698048799999732 ),
 ( 0.000000000000000000, 2.000000000000000000 ),
 .UNSPECIFIED. ) ;
#29223=CARTESIAN_POINT ( 'NONE',  ( 14.64149002350000117, 1416.824060884929850, 219.7189340838980058 ) ) ;
#29224=CARTESIAN_POINT ( 'NONE',  ( 14.89301817989999854, 1485.042290100730042, 224.3999831303979988 ) ) ;
#29225=CARTESIAN_POINT ( 'NONE',  ( 18.02574679518840028, 1424.482682570480165, 224.6196048480980210 ) ) ;
#29227=VERTEX_POINT ( 'NONE', #16297 ) ;
#29229=CARTESIAN_POINT ( 'NONE',  ( 5.370527602886283169, 1422.356908813907012, 139.1416118586824666 ) ) ;
#29231=CARTESIAN_POINT ( 'NONE',  ( -12.44325168979999852, 1415.996778985530000, 195.0334447333979995 ) ) ;
#29233=CARTESIAN_POINT ( 'NONE',  ( 23.11858565820000067, 1409.884865691529967, 211.2355702977880014 ) ) ;
#29239=CARTESIAN_POINT ( 'NONE',  ( 1.077911720219999925, 1415.753832296730025, 233.1550800001979837 ) ) ;
#29242=CARTESIAN_POINT ( 'NONE',  ( -22.57618069069999933, 1411.056460445829998, 211.7928261235179832 ) ) ;
#29243=CARTESIAN_POINT ( 'NONE',  ( -0.6544075182467720131, 1420.442518575000122, 184.0330262823659950 ) ) ;
#29246=CARTESIAN_POINT ( 'NONE',  ( -14.82166838865560088, 1486.064940468489795, 186.2093746475509874 ) ) ;
#29250=ORIENTED_EDGE ( 'NONE', *, *, #27647, .T. ) ;
#29251=VERTEX_POINT ( 'NONE', #110385 ) ;
#29252=CARTESIAN_POINT ( 'NONE',  ( 28.53450901119999727, 1509.594688344129963, 211.3361516935080147 ) ) ;
#29255=CARTESIAN_POINT ( 'NONE',  ( 1.547463840030000037, 1414.913060387329779, 192.3096136973980208 ) ) ;
#29256=CARTESIAN_POINT ( 'NONE',  ( 15.99649503710709730, 1421.554318619909964, 191.1865063950630201 ) ) ;
#29257=CARTESIAN_POINT ( 'NONE',  ( 0.8719743115910000286, 1508.600324595230177, 180.4235865536979873 ) ) ;
#29258=CARTESIAN_POINT ( 'NONE',  ( 11.96661585360000046, 1440.449248668989867, 150.8629738177980073 ) ) ;
#29259=CARTESIAN_POINT ( 'NONE',  ( -25.57905335200330299, 1450.800917333740017, 137.0692583773119964 ) ) ;
#29260=CARTESIAN_POINT ( 'NONE',  ( 4.399927595769999478, 1410.004273022730104, 231.3928942499979939 ) ) ;
#29263=CARTESIAN_POINT ( 'NONE',  ( 40.90250537874639747, 1447.119793117639801, 134.0999999985199906 ) ) ;
#29264=( BOUNDED_CURVE ( )  B_SPLINE_CURVE ( 3, ( #62542, #45728, #4786, #82042 ),
 .UNSPECIFIED., .F., .T. ) 
 B_SPLINE_CURVE_WITH_KNOTS ( ( 4, 4 ),
 ( 5.921924288096549915, 6.231904421257119964 ),
 .UNSPECIFIED. ) 
 CURVE ( )  GEOMETRIC_REPRESENTATION_ITEM ( )  RATIONAL_B_SPLINE_CURVE ( ( 1.000000000000000000, 0.9920087094985445830, 0.9920087094985445830, 1.000000000000000000 ) ) 
 REPRESENTATION_ITEM ( '' )  );
#29270=ORIENTED_EDGE ( 'NONE', *, *, #7669, .T. ) ;
#29274=CARTESIAN_POINT ( 'NONE',  ( 7.904476258595151350, 1451.392616462666638, 152.9734174004545366 ) ) ;
#29277=CARTESIAN_POINT ( 'NONE',  ( -17.00854892524643347, 1449.165472411616520, 219.4054542577865163 ) ) ;
#29280=CARTESIAN_POINT ( 'NONE',  ( 1.160958422820000058, 1414.971439108430104, 191.5548729526980196 ) ) ;
#29282=ORIENTED_EDGE ( 'NONE', *, *, #87921, .F. ) ;
#29285=CARTESIAN_POINT ( 'NONE',  ( 24.76605716182779915, 1440.913060387330006, 238.3302827077500012 ) ) ;
#29286=CARTESIAN_POINT ( 'NONE',  ( -13.77714796350000093, 1508.637939676529868, 184.0711857673979921 ) ) ;
#29288=FACE_OUTER_BOUND ( 'NONE', #61606, .T. ) ;
#29289=CARTESIAN_POINT ( 'NONE',  ( -13.97293528600000023, 1409.401006039529875, 191.8161164125979781 ) ) ;
#29291=CARTESIAN_POINT ( 'NONE',  ( -24.41216396249999931, 1440.964695643669984, 212.0310679874179982 ) ) ;
#29294=CARTESIAN_POINT ( 'NONE',  ( 0.0002087548573902462442, 1397.282671569474587, 196.2061409705553103 ) ) ;
#29295=CARTESIAN_POINT ( 'NONE',  ( -12.28708495595255279, 1434.198421465742285, 147.4194680967047475 ) ) ;
#29297=CARTESIAN_POINT ( 'NONE',  ( 2.848137854069999975, 1464.611669510630009, 235.5053002295980207 ) ) ;
#29300=CARTESIAN_POINT ( 'NONE',  ( 10.81518794224679958, 1424.921099295370141, 144.1705737284439977 ) ) ;
#29303=CARTESIAN_POINT ( 'NONE',  ( 19.13409869423357534, 1443.853562509159246, 213.6555041989591643 ) ) ;
#29306=CARTESIAN_POINT ( 'NONE',  ( -5.315917822019888384, 1420.217656571705220, 137.0999999980980135 ) ) ;
#29310=CARTESIAN_POINT ( 'NONE',  ( 29.87497052580000201, 1442.835664583690004, 238.0574391274980144 ) ) ;
#29314=CARTESIAN_POINT ( 'NONE',  ( 1.800869729310000000, 1413.124895085329854, 232.3173401135979930 ) ) ;
#29316=CARTESIAN_POINT ( 'NONE',  ( -19.11605526869999849, 1444.805919307749946, 225.6841260797980055 ) ) ;
#29320=ORIENTED_EDGE ( 'NONE', *, *, #110275, .T. ) ;
#29322=CARTESIAN_POINT ( 'NONE',  ( 2.101138442839999954, 1406.100891733030039, 269.0439770072979968 ) ) ;
#29324=CARTESIAN_POINT ( 'NONE',  ( 44.43457533159219963, 1446.348491390079971, 270.0922382052800117 ) ) ;
#29328=CARTESIAN_POINT ( 'NONE',  ( 2.531940903048510086E-08, 1457.850589566970029, 229.0733431205499926 ) ) ;
#29330=CARTESIAN_POINT ( 'NONE',  ( 0.5709835175930680906, 1450.893121203520195, 154.5155266294819967 ) ) ;
#29332=CARTESIAN_POINT ( 'NONE',  ( -1.546867746862319981, 1416.839692133689823, 228.0214409764060122 ) ) ;
#29333=ORIENTED_EDGE ( 'NONE', *, *, #100041, .F. ) ;
#29334=CARTESIAN_POINT ( 'NONE',  ( -21.34957048430000270, 1432.854863364579842, 234.3916895436979928 ) ) ;
#29337=CARTESIAN_POINT ( 'NONE',  ( -0.7746087140290000006, 1475.755075091830122, 269.0454657403980150 ) ) ;
#29338=CARTESIAN_POINT ( 'NONE',  ( 10.77451535478706290, 1424.915582317967164, 138.4825886073255958 ) ) ;
#29343=B_SPLINE_SURFACE_WITH_KNOTS ( 'NONE', 5, 5, ( 
 ( #19216, #79724, #87569, #47212, #97613, #29297, #46681, #89753, #4652 ),
 ( #38790, #70798, #63493, #62958, #54539, #64031, #4119, #79176, #97069 ),
 ( #2483, #38244, #55631, #36599, #72966, #88673, #3031, #71350, #20335 ),
 ( #27648, #45582, #37705, #71906, #104910, #72426, #20883, #55080, #106558 ),
 ( #21419, #28198, #19790, #53991, #29845, #88125, #98145, #11414, #105465 ),
 ( #28754, #90291, #57286, #13572, #99233, #83006, #24178, #66784, #108201 ),
 ( #100883, #39903, #32048, #82463, #32607, #40995, #74622, #6836, #90847 ),
 ( #41564, #48322, #56712, #83542, #57826, #65670, #58367, #74072, #84098 ),
 ( #15226, #108756, #5761, #91952, #91414, #47757, #14691, #49962, #92492 ),
 ( #49418, #7399, #5195, #81892, #98703, #48880, #75174, #14132, #65121 ),
 ( #39350, #6298, #40445, #15761, #21962, #31490, #73526, #107104, #109324 ),
 ( #66237, #99788, #23079, #30393, #64584, #56156, #107660, #30946, #100356 ),
 ( #22510, #23644, #109865, #17419, #110408, #59478, #34803, #51617, #9594 ),
 ( #67331, #9049, #68991, #67882, #61153, #101991, #60030, #129, #93589 ),
 ( #68435, #84646, #85752, #25277, #103092, #43222, #35357, #85198, #16865 ) ),
 .UNSPECIFIED., .F., .F., .F.,
 ( 6, 3, 3, 3, 6 ),
 ( 6, 3, 6 ),
 ( 24.26857305089999883, 41.67781792160000265, 49.51652399259999981, 57.35523006350000230, 61.88671852840000298 ),
 ( 0.000000000000000000, 1.000000000000000000, 2.000000000000000000 ),
 .UNSPECIFIED. ) ;
#29346=CARTESIAN_POINT ( 'NONE',  ( 26.80344781114780162, 1436.440813660759886, 136.7218762079120040 ) ) ;
#29347=CARTESIAN_POINT ( 'NONE',  ( -10.00562653641270039, 1396.262464565250184, 213.8494479798769703 ) ) ;
#29348=CARTESIAN_POINT ( 'NONE',  ( -14.50783621480000107, 1422.103482364530009, 228.3959130620980034 ) ) ;
#29349=CARTESIAN_POINT ( 'NONE',  ( 19.26683521067225868, 1456.110280151028292, 225.0772932314519892 ) ) ;
#29351=CARTESIAN_POINT ( 'NONE',  ( -15.70021566718022399, 1414.913060387329779, 204.0157239446980668 ) ) ;
#29352=CARTESIAN_POINT ( 'NONE',  ( 2.680552910549999890, 1409.943153456129949, 231.6453896010980031 ) ) ;
#29354=CARTESIAN_POINT ( 'NONE',  ( 11.15531093709999944, 1426.887873589030050, 101.9087401586980093 ) ) ;
#29356=CARTESIAN_POINT ( 'NONE',  ( -16.19086242769280304, 1409.478452467050147, 225.0103265570539861 ) ) ;
#29357=CARTESIAN_POINT ( 'NONE',  ( -13.51610093808349333, 1442.913060377700731, 205.0760988357353654 ) ) ;
#29361=CARTESIAN_POINT ( 'NONE',  ( 1.469929971880000075, 1507.915326702530137, 180.9459708343979969 ) ) ;
#29365=CARTESIAN_POINT ( 'NONE',  ( 16.41723189518601700, 1410.863437090559046, 191.6246442130024263 ) ) ;
#29366=ORIENTED_EDGE ( 'NONE', *, *, #33719, .F. ) ;
#29368=ORIENTED_EDGE ( 'NONE', *, *, #109927, .T. ) ;
#29369=CARTESIAN_POINT ( 'NONE',  ( -13.73335268700000000, 1441.669543367469942, 188.5645195036979942 ) ) ;
#29370=CARTESIAN_POINT ( 'NONE',  ( 1.455060923660010053, 1507.152178126010085, 236.7684687559849976 ) ) ;
#29375=CARTESIAN_POINT ( 'NONE',  ( 6.757182283909999754, 1429.763710591829977, 186.1422234325980014 ) ) ;
#29377=CARTESIAN_POINT ( 'NONE',  ( -40.70526567241159910, 1444.199263182009872, 137.0833905334800136 ) ) ;
#29378=CARTESIAN_POINT ( 'NONE',  ( 40.24340914364780275, 1439.067764445909916, 135.6665089828919974 ) ) ;
#29379=CARTESIAN_POINT ( 'NONE',  ( 30.84775898762307023, 1435.574754682624643, 135.1614303800634502 ) ) ;
#29380=CARTESIAN_POINT ( 'NONE',  ( 0.7133824534919999127, 1416.822690122329959, 190.3253679635979836 ) ) ;
#29381=CARTESIAN_POINT ( 'NONE',  ( -1.529674265799359834, 1405.855034992639958, 267.2342419976400265 ) ) ;
#29383=ORIENTED_EDGE ( 'NONE', *, *, #70015, .F. ) ;
#29386=ORIENTED_EDGE ( 'NONE', *, *, #30579, .F. ) ;
#29388=CARTESIAN_POINT ( 'NONE',  ( -22.19805590008481389, 1506.691119431217430, 208.9309066648677913 ) ) ;
#29393=CARTESIAN_POINT ( 'NONE',  ( -11.69665699774160039, 1509.376109397690016, 181.5816757439210107 ) ) ;
#29395=B_SPLINE_CURVE_WITH_KNOTS ( 'NONE', 3,
 ( #15867, #50070, #59025, #56806, #84199, #8041, #110510, #67986, #5854, #22603, #39995, #9161, #10252, #68534, #43325, #93684, #17522, #27612, #78572, #103770, #69649, #25932, #44428, #94814, #16963, #26495, #51163, #2447, #18090, #77473, #95919, #34358, #36563, #60691, #52285, #8590, #19180, #102097, #231, #102632, #51725, #43867, #85291 ),
 .UNSPECIFIED., .F., .F.,
 ( 4, 3, 3, 3, 3, 3, 3, 3, 3, 3, 3, 3, 3, 3, 4 ),
 ( 0.7655572723400000390, 0.9910019213991279052, 1.224379696602929890, 1.462078613820340101, 1.704827352800629914, 1.793853281190000093, 2.038466587763309690, 2.281256468240929980, 2.316155491850000026, 2.583989317130000352, 2.855920919032060024, 3.139267318808710350, 3.387490792969999998, 3.680707184002069976, 3.835724788489999426 ),
 .UNSPECIFIED. ) ;
#29396=CARTESIAN_POINT ( 'NONE',  ( 0.3621993314770000083, 1416.825784011830137, 227.1772709136979813 ) ) ;
#29398=B_SPLINE_CURVE_WITH_KNOTS ( 'NONE', 3,
 ( #69287, #11019, #61445, #45190, #36770, #103392, #36218, #95020, #18290, #79331 ),
 .UNSPECIFIED., .F., .F.,
 ( 4, 3, 3, 4 ),
 ( -157.4228452129300138, -134.4932552904479905, -78.88175342727269879, -29.50720979924130916 ),
 .UNSPECIFIED. ) ;
#29400=CARTESIAN_POINT ( 'NONE',  ( 10.98083629090000102, 1433.016921068679949, 151.7694307944979926 ) ) ;
#29401=CARTESIAN_POINT ( 'NONE',  ( -7.956249640850000304, 1409.190898750130145, 229.5825722790980024 ) ) ;
#29402=CARTESIAN_POINT ( 'NONE',  ( -13.91344329460000040, 1453.313060387329870, 193.8272260107980003 ) ) ;
#29403=VERTEX_POINT ( 'NONE', #59457 ) ;
#29404=CARTESIAN_POINT ( 'NONE',  ( -13.91014548664164430, 1434.990849513932744, 148.7055284007215334 ) ) ;
#29405=CARTESIAN_POINT ( 'NONE',  ( -26.77477579971149879, 1440.913060431829763, 225.7736581942319845 ) ) ;
#29408=B_SPLINE_CURVE_WITH_KNOTS ( 'NONE', 5,
 ( #307, #17599, #85938, #93759, #26005, #9781 ),
 .UNSPECIFIED., .F., .F.,
 ( 6, 6 ),
 ( 0.000000000000000000, 1.000000000000000000 ),
 .UNSPECIFIED. ) ;
#29409=CARTESIAN_POINT ( 'NONE',  ( -1.590905566307312169, 1484.788648649911920, 182.5874796340517605 ) ) ;
#29411=CARTESIAN_POINT ( 'NONE',  ( 36.30653363867440220, 1420.740886386239936, 270.0454586556700178 ) ) ;
#29415=VECTOR ( 'NONE', #16390, 1000.000000000000000 ) ;
#29416=CARTESIAN_POINT ( 'NONE',  ( 23.28494588540000265, 1410.121302984230169, 208.0652278728080091 ) ) ;
#29417=CARTESIAN_POINT ( 'NONE',  ( -9.968725191709733480, 1426.791337612255802, 224.6101419120311959 ) ) ;
#29423=CARTESIAN_POINT ( 'NONE',  ( 4.367919453601240676, 1420.283793878259985, 185.7030090601730024 ) ) ;
#29424=CARTESIAN_POINT ( 'NONE',  ( -4.423956996199999381, 1420.445634857929917, 232.5284400546979953 ) ) ;
#29429=ADVANCED_FACE ( 'NONE', ( #7376 ), #93567, .F. ) ;
#29431=CARTESIAN_POINT ( 'NONE',  ( -20.54724545888079845, 1508.877283812049882, 228.7275089972629871 ) ) ;
#29434=CARTESIAN_POINT ( 'NONE',  ( 0.08318261387021998188, 1420.450964567450228, 182.6885337629809953 ) ) ;
#29437=CARTESIAN_POINT ( 'NONE',  ( 19.41936330180000070, 1509.602163029830081, 186.8298580870979890 ) ) ;
#29442=ORIENTED_EDGE ( 'NONE', *, *, #78287, .F. ) ;
#29443=CARTESIAN_POINT ( 'NONE',  ( -0.04767993734059999822, 1497.009589119729981, 230.7918941427979860 ) ) ;
#29444=CARTESIAN_POINT ( 'NONE',  ( 10.07052880280942908, 1435.587077992309560, 152.4438796952450446 ) ) ;
#29447=( BOUNDED_CURVE ( )  B_SPLINE_CURVE ( 3, ( #61268, #95383, #42219, #76933 ),
 .UNSPECIFIED., .F., .F. ) 
 B_SPLINE_CURVE_WITH_KNOTS ( ( 4, 4 ),
 ( 6.111083944147519986, 6.515951168162740004 ),
 .UNSPECIFIED. ) 
 CURVE ( )  GEOMETRIC_REPRESENTATION_ITEM ( )  RATIONAL_B_SPLINE_CURVE ( ( 1.000000000000000000, 0.9863867946965088063, 0.9863867946965088063, 1.000000000000000000 ) ) 
 REPRESENTATION_ITEM ( '' )  );
#29449=CARTESIAN_POINT ( 'NONE',  ( -26.37463876368559923, 1508.216329634349904, 201.5356496705930169 ) ) ;
#29450=B_SPLINE_CURVE_WITH_KNOTS ( 'NONE', 5,
 ( #73372, #54929, #47075, #72825, #46534, #106958 ),
 .UNSPECIFIED., .F., .F.,
 ( 6, 6 ),
 ( 0.000000000000000000, 1.000000000000000000 ),
 .UNSPECIFIED. ) ;
#29451=CARTESIAN_POINT ( 'NONE',  ( 4.853127557110000545, 1425.657129708029970, 185.6214293445979990 ) ) ;
#29452=CARTESIAN_POINT ( 'NONE',  ( -18.55525628600000232, 1424.342884875230084, 224.9435532434980018 ) ) ;
#29453=CARTESIAN_POINT ( 'NONE',  ( -18.76321975249999952, 1435.968681994980216, 146.5949445436979772 ) ) ;
#29455=CARTESIAN_POINT ( 'NONE',  ( 17.56617749740000178, 1509.356465172729941, 187.2275717433980162 ) ) ;
#29456=CARTESIAN_POINT ( 'NONE',  ( 0.3788395847950430384, 1408.926289757150016, 231.6114269033369908 ) ) ;
#29457=FACE_OUTER_BOUND ( 'NONE', #44251, .T. ) ;
#29458=CARTESIAN_POINT ( 'NONE',  ( 20.59987592950000135, 1509.677367935830262, 230.5839143914980127 ) ) ;
#29462=CARTESIAN_POINT ( 'NONE',  ( 11.63679813930000151, 1439.363771630820111, 147.7934734181980048 ) ) ;
#29463=ORIENTED_EDGE ( 'NONE', *, *, #87176, .T. ) ;
#29464=EDGE_CURVE ( 'NONE', #88507, #38170, #42227, .T. ) ;
#29469=CARTESIAN_POINT ( 'NONE',  ( 21.62349440730000083, 1475.513060387329915, 210.0994872298300038 ) ) ;
#29471=CARTESIAN_POINT ( 'NONE',  ( -17.38235994490000280, 1414.983771850430003, 207.6803065375279971 ) ) ;
#29483=CARTESIAN_POINT ( 'NONE',  ( 27.43028940841649899, 1502.108409533960184, 207.6706673447280025 ) ) ;
#29486=CARTESIAN_POINT ( 'NONE',  ( 38.87758531470136347, 1429.322872991726626, 269.5908715927216690 ) ) ;
#29487=CARTESIAN_POINT ( 'NONE',  ( -14.01630619240000009, 1463.409576320030055, 240.3753821224980243 ) ) ;
#29490=CARTESIAN_POINT ( 'NONE',  ( -11.90119129059999992, 1433.600010809670039, 150.4754670856979999 ) ) ;
#29491=CARTESIAN_POINT ( 'NONE',  ( 25.63705379909999849, 1507.963168667929949, 199.9117834894379939 ) ) ;
#29492=CARTESIAN_POINT ( 'NONE',  ( -19.75357342619999912, 1485.455168234730081, 190.4162906186979853 ) ) ;
#29493=DIRECTION ( 'NONE',  ( 0.000000000000000000, 0.000000000000000000, 1.000000000000000000 ) ) ;
#29495=CARTESIAN_POINT ( 'NONE',  ( 4.749626518910000428, 1420.878300781530015, 185.8027267283979995 ) ) ;
#29498=CARTESIAN_POINT ( 'NONE',  ( 6.472929441039998899, 1440.851741079749900, 154.4738948603979907 ) ) ;
#29501=CARTESIAN_POINT ( 'NONE',  ( 1.393491831154829911E-08, 1407.187418594129895, 264.6521298086510114 ) ) ;
#29502=EDGE_LOOP ( 'NONE', ( #10915, #61409, #16846, #46704, #4891 ) ) ;
#29505=EDGE_CURVE ( 'NONE', #104636, #86228, #34975, .T. ) ;
#29508=CARTESIAN_POINT ( 'NONE',  ( -10.80862676880000173, 1472.323376642129915, 270.4164080859980004 ) ) ;
#29509=CARTESIAN_POINT ( 'NONE',  ( -23.81682389853370196, 1436.006617566450132, 211.5115497514818514 ) ) ;
#29512=CARTESIAN_POINT ( 'NONE',  ( 38.19124013942580831, 1450.350426091419877, 134.7937114414860105 ) ) ;
#29513=CARTESIAN_POINT ( 'NONE',  ( 0.3008760843888489966, 1451.060995806890105, 182.0476195407850071 ) ) ;
#29515=CARTESIAN_POINT ( 'NONE',  ( -11.39124975620000058, 1419.317003928930035, 229.3344809721980084 ) ) ;
#29516=EDGE_CURVE ( 'NONE', #65987, #36273, #43742, .T. ) ;
#29518=CARTESIAN_POINT ( 'NONE',  ( -1.357091273329259939, 1484.488606510706177, 182.3747662795626923 ) ) ;
#29520=CARTESIAN_POINT ( 'NONE',  ( -45.78687059534480142, 1437.115450045800117, 266.6856014455760260 ) ) ;
#29522=CARTESIAN_POINT ( 'NONE',  ( -3.535553491242379831, 1493.818507742730162, 181.5437437456840257 ) ) ;
#29528=CARTESIAN_POINT ( 'NONE',  ( 16.56042414419820119, 1409.526307809821674, 224.8086540885646798 ) ) ;
#29529=CARTESIAN_POINT ( 'NONE',  ( -7.074511979060000399, 1410.392875876630114, 187.4399194922980030 ) ) ;
#29530=FACE_OUTER_BOUND ( 'NONE', #93411, .T. ) ;
#29534=B_SPLINE_CURVE_WITH_KNOTS ( 'NONE', 5,
 ( #96881, #20150, #12856, #38068, #81162, #21226, #53803, #105274, #19601, #46493, #62764, #87940 ),
 .UNSPECIFIED., .F., .F.,
 ( 6, 3, 3, 6 ),
 ( -14.75003859432340114, -6.990622299139999996, 15.67373306499999863, 31.20981119710000229 ),
 .UNSPECIFIED. ) ;
#29537=EDGE_CURVE ( 'NONE', #11318, #74815, #84825, .T. ) ;
#29539=VERTEX_POINT ( 'NONE', #80646 ) ;
#29540=CARTESIAN_POINT ( 'NONE',  ( -9.945122577541358311, 1408.453178102650099, 270.1158524044950013 ) ) ;
#29541=CARTESIAN_POINT ( 'NONE',  ( 2.986439680811220132, 1417.855500646999872, 233.9854127040079845 ) ) ;
#29547=CARTESIAN_POINT ( 'NONE',  ( 44.51678373992154292, 1448.484642947900738, 269.0061672408559161 ) ) ;
#29549=CARTESIAN_POINT ( 'NONE',  ( -14.09009566611259956, 1436.250362699700190, 150.1829504920789873 ) ) ;
#29550=CARTESIAN_POINT ( 'NONE',  ( -0.03615109642835009907, 1409.488087751360126, 185.3130394953689688 ) ) ;
#29552=CARTESIAN_POINT ( 'NONE',  ( -17.86421487526029850, 1415.184612913570163, 207.5656586035410101 ) ) ;
#29553=CARTESIAN_POINT ( 'NONE',  ( -19.08968851999999927, 1435.774291999059869, 224.9956671329980225 ) ) ;
#29554=CARTESIAN_POINT ( 'NONE',  ( -14.00467695169999871, 1423.498461949430293, 222.1148246841979983 ) ) ;
#29555=CARTESIAN_POINT ( 'NONE',  ( 11.83559671189999918, 1415.245980412430072, 222.8086952457979919 ) ) ;
#29556=CARTESIAN_POINT ( 'NONE',  ( 7.560826431379999768, 1445.756812236420046, 183.8406469472979836 ) ) ;
#29559=CARTESIAN_POINT ( 'NONE',  ( -40.71747595839320155, 1438.773003563489965, 135.3761635789150262 ) ) ;
#29562=LINE ( 'NONE', #62664, #105354 ) ;
#29563=CARTESIAN_POINT ( 'NONE',  ( 24.53925018798819835, 1451.993264915540067, 136.6785377935909764 ) ) ;
#29566=CARTESIAN_POINT ( 'NONE',  ( 18.97990684999999900, 1409.575853339430068, 198.5868976705980060 ) ) ;
#29567=CARTESIAN_POINT ( 'NONE',  ( 22.30625523140000155, 1409.857389917029877, 207.2280132821280176 ) ) ;
#29568=CARTESIAN_POINT ( 'NONE',  ( -24.94579848589999926, 1435.368615134259926, 135.7553688025980136 ) ) ;
#29570=CARTESIAN_POINT ( 'NONE',  ( 0.9686598153761089014, 1450.845731688880051, 181.4217000318980126 ) ) ;
#29571=CARTESIAN_POINT ( 'NONE',  ( 2.500000000000000000, 1439.624608404519904, 169.5728743624090100 ) ) ;
#29575=CARTESIAN_POINT ( 'NONE',  ( -0.9912863951520000105, 1474.170141985030114, 270.1376065698979687 ) ) ;
#29576=CARTESIAN_POINT ( 'NONE',  ( -18.34590456075780196, 1416.851343895820037, 208.8605686865189739 ) ) ;
#29577=CARTESIAN_POINT ( 'NONE',  ( -8.690384483830820628, 1424.104242022259996, 112.3001764364740183 ) ) ;
#29579=EDGE_CURVE ( 'NONE', #75280, #25855, #7512, .T. ) ;
#29580=CARTESIAN_POINT ( 'NONE',  ( -39.63715609436299303, 1446.664237654140152, 136.6953018245600049 ) ) ;
#29581=CARTESIAN_POINT ( 'NONE',  ( 11.60004869884913070, 1425.167079614044951, 137.9682444091046420 ) ) ;
#29582=CARTESIAN_POINT ( 'NONE',  ( 2.068048313059574372, 1417.341179972549753, 233.1878878483405231 ) ) ;
#29583=CARTESIAN_POINT ( 'NONE',  ( 17.82742679679007480, 1423.642332963798935, 225.9916762313126242 ) ) ;
#29584=CARTESIAN_POINT ( 'NONE',  ( 11.58989588439999885, 1433.067267885580122, 151.1017417262979734 ) ) ;
#29585=CARTESIAN_POINT ( 'NONE',  ( -0.6052730379878279443, 1475.056357020409905, 269.6445050902949561 ) ) ;
#29587=CARTESIAN_POINT ( 'NONE',  ( 27.81399413693910105, 1440.913060387569885, 230.3950460944500094 ) ) ;
#29591=CARTESIAN_POINT ( 'NONE',  ( 13.51610093808350577, 1445.063428794548372, 150.6358704321319806 ) ) ;
#29593=CARTESIAN_POINT ( 'NONE',  ( -19.28960628685421952, 1485.613772762859981, 189.7904103076950264 ) ) ;
#29595=CARTESIAN_POINT ( 'NONE',  ( 2.633995852980000052, 1482.821221012130081, 234.8958063198980142 ) ) ;
#29597=CARTESIAN_POINT ( 'NONE',  ( -16.94063806799999838, 1507.935533831129987, 230.1637782476980192 ) ) ;
#29601=CARTESIAN_POINT ( 'NONE',  ( 5.363529431139269832, 1422.300429797930065, 141.6243240101889853 ) ) ;
#29604=CARTESIAN_POINT ( 'NONE',  ( -7.625096704207815712, 1438.527495425920733, 153.8927455731590328 ) ) ;
#29607=CARTESIAN_POINT ( 'NONE',  ( -0.6632445612200000840, 1450.894163472750051, 181.6521849990980115 ) ) ;
#29611=CARTESIAN_POINT ( 'NONE',  ( 1.552364032401126082, 1414.913060581098307, 192.1087617152385008 ) ) ;
#29612=ORIENTED_EDGE ( 'NONE', *, *, #16679, .T. ) ;
#29617=DIRECTION ( 'NONE',  ( -0.5121697454732879740, 0.04449972806152376059, 0.8577306838537828160 ) ) ;
#29621=B_SPLINE_CURVE_WITH_KNOTS ( 'NONE', 5,
 ( #24351, #74786, #91009, #7011, #101053, #57986 ),
 .UNSPECIFIED., .F., .F.,
 ( 6, 6 ),
 ( 0.000000000000000000, 1.000000000000000000 ),
 .UNSPECIFIED. ) ;
#29624=CARTESIAN_POINT ( 'NONE',  ( 14.84736599141850100, 1409.431541832679841, 207.5470409763789803 ) ) ;
#29627=CARTESIAN_POINT ( 'NONE',  ( -19.45266374790000086, 1470.701691425329955, 191.2979019387979918 ) ) ;
#29628=CARTESIAN_POINT ( 'NONE',  ( 5.273680924645899992, 1398.098440471860158, 218.7752541425170136 ) ) ;
#29630=ORIENTED_EDGE ( 'NONE', *, *, #104187, .T. ) ;
#29632=ADVANCED_FACE ( 'NONE', ( #67167 ), #69758, .F. ) ;
#29634=FACE_OUTER_BOUND ( 'NONE', #83257, .T. ) ;
#29638=CARTESIAN_POINT ( 'NONE',  ( -20.09679227796999967, 1491.565535399339979, 190.8618222658760146 ) ) ;
#29639=CARTESIAN_POINT ( 'NONE',  ( 1.143705719820000022, 1395.952999471229759, 220.4423849542980065 ) ) ;
#29640=CARTESIAN_POINT ( 'NONE',  ( 19.67294328819050264, 1440.103798296560171, 209.6949378802180206 ) ) ;
#29641=CARTESIAN_POINT ( 'NONE',  ( -19.38775984613145908, 1486.273308771174698, 189.6873704809262051 ) ) ;
#29643=CARTESIAN_POINT ( 'NONE',  ( -25.95396204517641081, 1436.671747891054565, 136.9772620809131354 ) ) ;
#29644=CARTESIAN_POINT ( 'NONE',  ( 13.89512612635319933, 1452.719752330199981, 223.3357008107990112 ) ) ;
#29645=EDGE_CURVE ( 'NONE', #36118, #34381, #27786, .T. ) ;
#29647=CARTESIAN_POINT ( 'NONE',  ( 11.32042664782710162, 1433.973776647149862, 151.5090680528710152 ) ) ;
#29648=CARTESIAN_POINT ( 'NONE',  ( -13.12645755140609971, 1434.861060459049895, 149.4023126016570018 ) ) ;
#29650=CARTESIAN_POINT ( 'NONE',  ( 20.28125873362029807, 1409.621297548600069, 202.2274700573379960 ) ) ;
#29654=CIRCLE ( 'NONE', #76184, 1.000002392508526627 ) ;
#29656=CARTESIAN_POINT ( 'NONE',  ( 32.18001715519999806, 1422.275298650230070, 259.4130760070980273 ) ) ;
#29657=CARTESIAN_POINT ( 'NONE',  ( -27.09023322290000380, 1488.688618555330095, 207.0766447722079988 ) ) ;
#29658=CARTESIAN_POINT ( 'NONE',  ( 0.4664314455240000101, 1502.016106112629814, 181.1536437472979912 ) ) ;
#29660=CARTESIAN_POINT ( 'NONE',  ( -0.8261674427231310291, 1507.439223847129824, 231.9334160780449849 ) ) ;
#29662=CARTESIAN_POINT ( 'NONE',  ( -25.73196790559999769, 1440.913060585610083, 220.8240077246979922 ) ) ;
#29665=CARTESIAN_POINT ( 'NONE',  ( 33.53414597829999622, 1450.881089635289982, 136.1829610295979762 ) ) ;
#29666=EDGE_LOOP ( 'NONE', ( #38560, #73361, #26261, #44812 ) ) ;
#29667=CARTESIAN_POINT ( 'NONE',  ( -0.08249068136597970113, 1397.911857760039993, 196.1221076742430114 ) ) ;
#29669=CARTESIAN_POINT ( 'NONE',  ( 8.792433923980000898, 1509.220098945629843, 237.4619125690979899 ) ) ;
#29672=CARTESIAN_POINT ( 'NONE',  ( 2.894070330896479692, 1493.616686583509818, 235.3440883567899959 ) ) ;
#29673=CARTESIAN_POINT ( 'NONE',  ( -23.32798702916920064, 1409.842805623620052, 208.9046620917229689 ) ) ;
#29677=EDGE_CURVE ( 'NONE', #5728, #104546, #104891, .T. ) ;
#29678=CARTESIAN_POINT ( 'NONE',  ( -11.97220943660000003, 1489.053879525330103, 232.5750221901979842 ) ) ;
#29681=ORIENTED_EDGE ( 'NONE', *, *, #88460, .F. ) ;
#29682=CIRCLE ( 'NONE', #42166, 2.000000001200720856 ) ;
#29683=CARTESIAN_POINT ( 'NONE',  ( 11.73648056819999930, 1426.280364960429779, 144.1673147891980022 ) ) ;
#29684=CARTESIAN_POINT ( 'NONE',  ( -12.70648376454910000, 1416.221314539489867, 221.9053760979749654 ) ) ;
#29685=CARTESIAN_POINT ( 'NONE',  ( 15.10082833669999935, 1496.663755438529961, 225.8002586636980027 ) ) ;
#29688=DIRECTION ( 'NONE',  ( 0.000000000000000000, 0.7071067811865475727, 0.7071067811865475727 ) ) ;
#29689=DIRECTION ( 'NONE',  ( -0.9831857282343242632, -0.1185196346870388412, 0.1389205527990460265 ) ) ;
#29697=CARTESIAN_POINT ( 'NONE',  ( 8.410267065803780360E-17, 1471.436294031830130, 269.3346704751489824 ) ) ;
#29698=CARTESIAN_POINT ( 'NONE',  ( 0.4703715106335689677, 1410.239988018240183, 269.6149086376819923 ) ) ;
#29702=CARTESIAN_POINT ( 'NONE',  ( 0.03395513245188531287, 1410.034063517130335, 233.1861139216583467 ) ) ;
#29706=CARTESIAN_POINT ( 'NONE',  ( -24.27081182540139892, 1508.823454366900023, 222.4349774664410120 ) ) ;
#29709=CARTESIAN_POINT ( 'NONE',  ( 1.021405182659999929E-14, 1413.763055110029882, 262.6648722463980334 ) ) ;
#29710=B_SPLINE_CURVE_WITH_KNOTS ( 'NONE', 5,
 ( #83927, #8864, #8316, #86139, #92319, #84483 ),
 .UNSPECIFIED., .F., .F.,
 ( 6, 6 ),
 ( 5.175829887319999933, 13.45293097300000085 ),
 .UNSPECIFIED. ) ;
#29711=CARTESIAN_POINT ( 'NONE',  ( 19.74393297465665142, 1455.407987973826721, 226.2017192373469072 ) ) ;
#29715=CARTESIAN_POINT ( 'NONE',  ( 44.92382594201649937, 1434.805869292970101, 269.6913831597940430 ) ) ;
#29723=CARTESIAN_POINT ( 'NONE',  ( -11.98374141780000102, 1442.037920581979961, 187.4992083556979878 ) ) ;
#29725=CARTESIAN_POINT ( 'NONE',  ( 12.44506479032133228, 1434.392593279323364, 149.5199551435223100 ) ) ;
#29726=CARTESIAN_POINT ( 'NONE',  ( 14.15980981120000060, 1419.763654237730179, 228.3914994946979959 ) ) ;
#29727=EDGE_CURVE ( 'NONE', #64548, #75280, #72974, .T. ) ;
#29730=CARTESIAN_POINT ( 'NONE',  ( 43.61890073000000001, 1430.078080930229817, 269.0317426087980266 ) ) ;
#29731=CARTESIAN_POINT ( 'NONE',  ( -18.48711282149999846, 1410.482182154930115, 223.8902303684980097 ) ) ;
#29732=CARTESIAN_POINT ( 'NONE',  ( 19.79232125780000118, 1435.617562599800067, 145.2032765877980012 ) ) ;
#29734=CARTESIAN_POINT ( 'NONE',  ( 5.383048381580209707, 1431.499937560449780, 154.5621489401540032 ) ) ;
#29735=CARTESIAN_POINT ( 'NONE',  ( -45.67177895054734194, 1445.962983056130724, 266.1885922345551876 ) ) ;
#29737=CARTESIAN_POINT ( 'NONE',  ( -39.29199511529999711, 1440.043273471179873, 136.7298370636979712 ) ) ;
#29738=CARTESIAN_POINT ( 'NONE',  ( 0.2080955792599850085, 1458.419842128130085, 183.0208787316280166 ) ) ;
#29739=CARTESIAN_POINT ( 'NONE',  ( -14.34547416000000020, 1409.237120669629803, 210.6641495597280027 ) ) ;
#29740=CARTESIAN_POINT ( 'NONE',  ( -11.96393163419999972, 1414.971352895729979, 197.5065629898979864 ) ) ;
#29742=EDGE_CURVE ( 'NONE', #73277, #68085, #72560, .T. ) ;
#29744=CARTESIAN_POINT ( 'NONE',  ( 12.06092026859999855, 1433.903687484779994, 149.4776502453979958 ) ) ;
#29745=CARTESIAN_POINT ( 'NONE',  ( -38.19279632269630298, 1437.094169276000002, 134.0999999969999692 ) ) ;
#29746=CARTESIAN_POINT ( 'NONE',  ( 7.671879397589999705, 1442.085042682959966, 183.9124572552979657 ) ) ;
#29749=CARTESIAN_POINT ( 'NONE',  ( 27.58075381470000309, 1440.826362455070011, 137.2340171046979833 ) ) ;
#29751=EDGE_LOOP ( 'NONE', ( #95571, #27249, #96031, #41086 ) ) ;
#29754=CARTESIAN_POINT ( 'NONE',  ( -30.23606167549999668, 1467.592994008429969, 267.4627077489980138 ) ) ;
#29757=CARTESIAN_POINT ( 'NONE',  ( -26.34628868930000323, 1509.610132138230028, 218.5686156305380052 ) ) ;
#29765=CARTESIAN_POINT ( 'NONE',  ( 11.49747572422220188, 1414.913060387329779, 220.3427040978150160 ) ) ;
#29767=CARTESIAN_POINT ( 'NONE',  ( 3.192504087185560113, 1426.553239361320038, 224.5880228764589788 ) ) ;
#29768=CARTESIAN_POINT ( 'NONE',  ( 4.554137863063505876, 1421.567652250969786, 137.7197909783843670 ) ) ;
#29771=CARTESIAN_POINT ( 'NONE',  ( -12.30733358380000020, 1416.021639799829927, 194.8879084977980085 ) ) ;
#29773=EDGE_CURVE ( 'NONE', #27781, #44537, #2188, .T. ) ;
#29774=CARTESIAN_POINT ( 'NONE',  ( 23.43703390090000127, 1411.091823681130109, 212.1167532368579884 ) ) ;
#29777=CARTESIAN_POINT ( 'NONE',  ( -5.379917643342909450, 1430.657135788060032, 154.4490610592320081 ) ) ;
#29778=CARTESIAN_POINT ( 'NONE',  ( -11.58636794539999926, 1433.009610086610110, 151.1946776885979773 ) ) ;
#29780=CARTESIAN_POINT ( 'NONE',  ( 24.16765931996930306, 1411.086006809529863, 208.8198375941539950 ) ) ;
#29783=EDGE_CURVE ( 'NONE', #86466, #50703, #46210, .T. ) ;
#29785=CARTESIAN_POINT ( 'NONE',  ( -1.714310246450000186, 1417.458497559930038, 235.2631534898980021 ) ) ;
#29789=CARTESIAN_POINT ( 'NONE',  ( -12.88114576569580016, 1485.825225328749866, 185.4416202657009762 ) ) ;
#29794=EDGE_LOOP ( 'NONE', ( #83200, #12437, #80397, #77565 ) ) ;
#29797=CARTESIAN_POINT ( 'NONE',  ( 28.19408364699999936, 1508.123162656630029, 209.7484684564449822 ) ) ;
#29801=CARTESIAN_POINT ( 'NONE',  ( 1.554562095370000119, 1427.328278510630071, 123.0297916884979941 ) ) ;
#29802=DIRECTION ( 'NONE',  ( 0.9993902469235412811, -0.03489947644508400310, -0.001077449749359506159 ) ) ;
#29804=CARTESIAN_POINT ( 'NONE',  ( -25.39633370633140075, 1450.805127515380036, 137.3302824775919930 ) ) ;
#29806=CARTESIAN_POINT ( 'NONE',  ( 14.78510249340000016, 1410.361618668330038, 227.6029314014980116 ) ) ;
#29809=CARTESIAN_POINT ( 'NONE',  ( 40.02226351607779975, 1448.570981149600129, 134.0999999981999906 ) ) ;
#29811=ORIENTED_EDGE ( 'NONE', *, *, #51557, .F. ) ;
#29812=CARTESIAN_POINT ( 'NONE',  ( 14.09229571774920053, 1435.068515943999955, 149.0020687653649816 ) ) ;
#29814=VERTEX_POINT ( 'NONE', #65939 ) ;
#29823=CARTESIAN_POINT ( 'NONE',  ( -18.29888576657991806, 1446.389289291960040, 215.5040569812714182 ) ) ;
#29826=CARTESIAN_POINT ( 'NONE',  ( 5399.972634567438945, 2837.742859962510465, -8135.989823930170132 ) ) ;
#29828=CARTESIAN_POINT ( 'NONE',  ( 3.346431401090000257, 1414.913060387329779, 192.5065129705980098 ) ) ;
#29830=EDGE_LOOP ( 'NONE', ( #35882, #52273, #71112, #58527 ) ) ;
#29832=ORIENTED_EDGE ( 'NONE', *, *, #59162, .F. ) ;
#29833=CARTESIAN_POINT ( 'NONE',  ( 30.90535300673260011, 1440.913060387330006, 253.9123373970340083 ) ) ;
#29834=CARTESIAN_POINT ( 'NONE',  ( 19.03075101710000183, 1457.035589272129982, 226.5471405812980095 ) ) ;
#29835=ORIENTED_EDGE ( 'NONE', *, *, #92867, .T. ) ;
#29836=CARTESIAN_POINT ( 'NONE',  ( -0.3797365229449999879, 1451.158458254029938, 182.5593410785980097 ) ) ;
#29837=CARTESIAN_POINT ( 'NONE',  ( -16.13865951880000082, 1410.848995608429959, 191.4167396153979723 ) ) ;
#29839=CARTESIAN_POINT ( 'NONE',  ( -24.41186848160000267, 1440.913060429599909, 212.0284777738579862 ) ) ;
#29840=CARTESIAN_POINT ( 'NONE',  ( 22.48215601709099687, 1410.706993422959840, 206.2088699951190165 ) ) ;
#29842=CARTESIAN_POINT ( 'NONE',  ( 45.67177343720949523, 1440.913060382069943, 266.1885934449759930 ) ) ;
#29843=CARTESIAN_POINT ( 'NONE',  ( -12.06120403350000103, 1433.903434619470090, 147.8551727352979981 ) ) ;
#29844=CARTESIAN_POINT ( 'NONE',  ( 25.61452959376079974, 1479.968245174939966, 206.2236738490990149 ) ) ;
#29845=CARTESIAN_POINT ( 'NONE',  ( 9.838112090859999270, 1463.224994908330018, 233.1087581964980018 ) ) ;
#29846=CARTESIAN_POINT ( 'NONE',  ( -10.37023892357026611, 1423.186503347903454, 137.2231747537963429 ) ) ;
#29851=CARTESIAN_POINT ( 'NONE',  ( 19.41153299114838759, 1441.868806216761413, 212.6349187631244035 ) ) ;
#29853=CARTESIAN_POINT ( 'NONE',  ( -19.63212482909999679, 1452.819910077329951, 209.4932260605140186 ) ) ;
#29854=CARTESIAN_POINT ( 'NONE',  ( -7.790452417740089786, 1421.055847862326800, 137.0999999980979567 ) ) ;
#29856=ORIENTED_EDGE ( 'NONE', *, *, #40817, .T. ) ;
#29858=CARTESIAN_POINT ( 'NONE',  ( 24.51530987499999981, 1445.843072706799830, 217.4968709922580103 ) ) ;
#29861=CARTESIAN_POINT ( 'NONE',  ( -1.417593344014799861, 1507.391024683259729, 237.1614008355199701 ) ) ;
#29864=CARTESIAN_POINT ( 'NONE',  ( -20.17861002410000282, 1444.801920322949854, 223.8644076282979825 ) ) ;
#29865=CARTESIAN_POINT ( 'NONE',  ( 19.02704169760000141, 1456.915441327430017, 225.6706379882980116 ) ) ;
#29867=CARTESIAN_POINT ( 'NONE',  ( -2.201054711479999870, 1485.573836360929818, 182.5778603406980096 ) ) ;
#29870=CARTESIAN_POINT ( 'NONE',  ( 2.754936409899999994, 1406.324493345930023, 269.2919060128980391 ) ) ;
#29872=CARTESIAN_POINT ( 'NONE',  ( 23.75101318751531210, 1434.596239882524515, 214.4266028146048768 ) ) ;
#29874=CARTESIAN_POINT ( 'NONE',  ( 11.60004869885203860, 1422.462448494397904, 137.0350196580168642 ) ) ;
#29876=CARTESIAN_POINT ( 'NONE',  ( -1.172951605644029893, 1450.815013396339964, 154.5169658199289984 ) ) ;
#29877=CARTESIAN_POINT ( 'NONE',  ( -11.96786612770000069, 1446.201513125040037, 187.3303122566979937 ) ) ;
#29878=CARTESIAN_POINT ( 'NONE',  ( 11.60004869885203682, 1428.983126981193436, 134.0999999980966777 ) ) ;
#29879=CARTESIAN_POINT ( 'NONE',  ( -14.32414760834769929, 1416.073666499319870, 221.2545971180610138 ) ) ;
#29881=CARTESIAN_POINT ( 'NONE',  ( -4.290289619920000241, 1420.418457352130190, 243.9198229428980085 ) ) ;
#29882=CARTESIAN_POINT ( 'NONE',  ( 3.125595126769999954, 1441.073642980700015, 162.1945237037980121 ) ) ;
#29883=CARTESIAN_POINT ( 'NONE',  ( -0.7656945474359999615, 1475.043758653330087, 269.6498827581980322 ) ) ;
#29884=CARTESIAN_POINT ( 'NONE',  ( -33.29550038720000060, 1451.750386302530160, 134.7337860542980081 ) ) ;
#29886=CARTESIAN_POINT ( 'NONE',  ( -3.958930064598830789, 1448.297290140811356, 185.0655646505161087 ) ) ;
#29891=CARTESIAN_POINT ( 'NONE',  ( -8.743415935682730122, 1396.218387199900008, 215.8871218720089757 ) ) ;
#29893=CARTESIAN_POINT ( 'NONE',  ( -45.55153353979999764, 1438.765428390510124, 268.9770687238979576 ) ) ;
#29897=CARTESIAN_POINT ( 'NONE',  ( 2.559318562519999674, 1409.169965889630021, 231.1158913475979944 ) ) ;
#29900=CARTESIAN_POINT ( 'NONE',  ( 11.46601636529999979, 1425.973735423729750, 132.2042239505979921 ) ) ;
#29902=CARTESIAN_POINT ( 'NONE',  ( 9230.682934795011533, 2837.541834147232294, -5630.801423131496449 ) ) ;
#29907=CARTESIAN_POINT ( 'NONE',  ( -4.866999017969999564, 1428.784516533529995, 149.2390836726979728 ) ) ;
#29912=B_SPLINE_CURVE_WITH_KNOTS ( 'NONE', 3,
 ( #43557, #101775, #75519, #77707 ),
 .UNSPECIFIED., .F., .F.,
 ( 4, 4 ),
 ( -157.6565403015839877, -140.7391984879999995 ),
 .UNSPECIFIED. ) ;
#29917=CARTESIAN_POINT ( 'NONE',  ( -9.777403739020000373, 1396.433055053929820, 201.5769308046579908 ) ) ;
#29918=CARTESIAN_POINT ( 'NONE',  ( 2.922846155700570048, 1409.846762780129893, 231.4964038402399922 ) ) ;
#29920=CARTESIAN_POINT ( 'NONE',  ( 0.4901645137037970446, 1507.127656893030007, 237.3576198934299839 ) ) ;
#29921=DIRECTION ( 'NONE',  ( 0.000000000000000000, 0.000000000000000000, -1.000000000000000000 ) ) ;
#29922=CARTESIAN_POINT ( 'NONE',  ( 18.11157372306810132, 1509.545530478630099, 186.5307137986639816 ) ) ;
#29924=CARTESIAN_POINT ( 'NONE',  ( -1.361571319557159931, 1414.169512293919979, 185.4414444276949894 ) ) ;
#29925=CARTESIAN_POINT ( 'NONE',  ( 4.507398563669999803, 1429.767108183030132, 185.3173098813979891 ) ) ;
#29927=CARTESIAN_POINT ( 'NONE',  ( -41.47274599670710415, 1445.558650626129975, 135.4388875029059989 ) ) ;
#29929=CARTESIAN_POINT ( 'NONE',  ( 41.49257586737849834, 1443.690994743030160, 136.5669662302249776 ) ) ;
#29930=CARTESIAN_POINT ( 'NONE',  ( 7.279683625616689469, 1396.167272541620150, 217.4296586424180191 ) ) ;
#29931=CARTESIAN_POINT ( 'NONE',  ( -39.43944535410179952, 1438.613980986869819, 136.5560418723989926 ) ) ;
#29932=CARTESIAN_POINT ( 'NONE',  ( 11.76685707319999885, 1426.512066191629856, 146.4443102791980209 ) ) ;
#29936=CARTESIAN_POINT ( 'NONE',  ( 12.20994210559999971, 1442.197620241679942, 187.8251864636980031 ) ) ;
#29938=ORIENTED_EDGE ( 'NONE', *, *, #57916, .T. ) ;
#29941=CARTESIAN_POINT ( 'NONE',  ( -13.89796033290000032, 1452.811554596829865, 194.9888671150980031 ) ) ;
#29947=CARTESIAN_POINT ( 'NONE',  ( 2.500000000000000000, 1448.758219215480040, 157.1656513900349807 ) ) ;
#29950=CARTESIAN_POINT ( 'NONE',  ( 18.18905553120000107, 1416.520322350429979, 213.0710787703080200 ) ) ;
#29952=B_SPLINE_CURVE_WITH_KNOTS ( 'NONE', 3,
 ( #41924, #35727, #44142, #85009, #43585, #85556, #93965, #68804, #8852, #78278 ),
 .UNSPECIFIED., .F., .F.,
 ( 4, 2, 2, 2, 4 ),
 ( -0.2248365648612329903, -0.1535262906595619981, -0.1118204630139870148, -0.05103592384959870776, -1.415349781819230657E-10 ),
 .UNSPECIFIED. ) ;
#29955=CARTESIAN_POINT ( 'NONE',  ( -31.14511482488981287, 1420.453826065711155, 269.4834250285384201 ) ) ;
#29956=CARTESIAN_POINT ( 'NONE',  ( -3.805207261640000116, 1409.045941153030071, 230.7650822874980179 ) ) ;
#29957=CARTESIAN_POINT ( 'NONE',  ( -14.59882275810000074, 1475.513060387329915, 193.1404296630979900 ) ) ;
#29959=CARTESIAN_POINT ( 'NONE',  ( 2.500000000000000000, 1421.075716575930073, 150.9130928818979953 ) ) ;
#29960=CARTESIAN_POINT ( 'NONE',  ( -28.78732923508430019, 1440.913060387340010, 234.1936472594090048 ) ) ;
#29961=AXIS2_PLACEMENT_3D ( 'NONE', #828, #84796, #24875 ) ;
#29964=CARTESIAN_POINT ( 'NONE',  ( 42.85026807650999814, 1436.651183019170048, 270.2009488495780261 ) ) ;
#29968=CARTESIAN_POINT ( 'NONE',  ( 23.85008871109999973, 1410.843070914130294, 208.1757528339269925 ) ) ;
#29973=CARTESIAN_POINT ( 'NONE',  ( 4.228665902068920346, 1420.870217351630117, 185.4828094967849950 ) ) ;
#29974=CARTESIAN_POINT ( 'NONE',  ( -0.9921696537889999057, 1415.381620563129900, 233.2736997477979912 ) ) ;
#29976=ORIENTED_EDGE ( 'NONE', *, *, #70508, .T. ) ;
#29979=CARTESIAN_POINT ( 'NONE',  ( 0.4681594785439999740, 1415.795094203329882, 233.3996825305979996 ) ) ;
#29983=CARTESIAN_POINT ( 'NONE',  ( -11.86716023049999968, 1432.353341358199941, 147.6509521729980179 ) ) ;
#29986=CARTESIAN_POINT ( 'NONE',  ( -0.08276393048689759113, 1408.915950567679829, 231.1937673021830051 ) ) ;
#29989=EDGE_LOOP ( 'NONE', ( #76265, #60369, #9857, #83132, #79284 ) ) ;
#29991=CARTESIAN_POINT ( 'NONE',  ( -3.827327205999999649, 1419.393213449430050, 165.4910337701979870 ) ) ;
#29997=CARTESIAN_POINT ( 'NONE',  ( -27.06354385267519902, 1509.473110589510043, 201.2587778061670178 ) ) ;
#29998=CARTESIAN_POINT ( 'NONE',  ( -4.222550915200000254, 1446.229941110429991, 170.5491765577980061 ) ) ;
#29999=CARTESIAN_POINT ( 'NONE',  ( -20.17846522170000156, 1427.578677867830038, 222.8742699695980320 ) ) ;
#30002=CARTESIAN_POINT ( 'NONE',  ( 15.66025028199999980, 1508.960093224430011, 186.3692160812979921 ) ) ;
#30004=CARTESIAN_POINT ( 'NONE',  ( 29.27919548120000215, 1509.872435206929822, 209.3677808018739768 ) ) ;
#30011=CARTESIAN_POINT ( 'NONE',  ( -16.19493240869999795, 1409.478599888930148, 193.4350318414979881 ) ) ;
#30013=CARTESIAN_POINT ( 'NONE',  ( -18.70459388229999931, 1509.566239198729818, 231.7064163648979900 ) ) ;
#30015=CARTESIAN_POINT ( 'NONE',  ( -13.51471643657749233, 1443.999204071515123, 187.1185524397720314 ) ) ;
#30016=CARTESIAN_POINT ( 'NONE',  ( -17.35267692490000258, 1414.988015876730060, 207.7949262638379935 ) ) ;
#30020=CARTESIAN_POINT ( 'NONE',  ( 18.71421116979999866, 1425.460417338532807, 226.6184583000981547 ) ) ;
#30022=CARTESIAN_POINT ( 'NONE',  ( 21.92317828190000029, 1509.363426959629805, 190.7737838525980294 ) ) ;
#30029=CARTESIAN_POINT ( 'NONE',  ( 13.20876367099999982, 1507.490208233330122, 233.1223600710980008 ) ) ;
#30031=CARTESIAN_POINT ( 'NONE',  ( 29.82222091440462819, 1419.446744514379134, 269.4689231808105205 ) ) ;
#30032=CARTESIAN_POINT ( 'NONE',  ( -29.43658766909999969, 1455.581846392329908, 250.1802633725980343 ) ) ;
#30034=AXIS2_PLACEMENT_3D ( 'NONE', #98601, #100266, #98047 ) ;
#30035=CARTESIAN_POINT ( 'NONE',  ( -11.53856147429999979, 1433.624126597800114, 151.2408432088979851 ) ) ;
#30036=B_SPLINE_CURVE_WITH_KNOTS ( 'NONE', 5,
 ( #98442, #5490, #39649, #31239, #73253, #13868, #74376, #46423, #72712, #91147, #21712, #99529, #57021, #81630, #106835, #39076, #55916, #30128, #90035, #14422, #48618 ),
 .UNSPECIFIED., .F., .F.,
 ( 6, 3, 3, 3, 3, 3, 6 ),
 ( 21.28770806440000030, 21.63383848259999809, 29.22288786549999884, 33.07574020050000030, 38.86051041610000567, 44.90455290039999880, 44.92446774270000276 ),
 .UNSPECIFIED. ) ;
#30038=CARTESIAN_POINT ( 'NONE',  ( -19.11638574819999903, 1485.531016413629914, 189.6477890060980087 ) ) ;
#30043=CARTESIAN_POINT ( 'NONE',  ( 6.823170627169999669, 1439.352237894180007, 154.2706161131980025 ) ) ;
#30048=CARTESIAN_POINT ( 'NONE',  ( 6.691069722549889836E-09, 1409.748499752379985, 259.1747490247929591 ) ) ;
#30050=ORIENTED_EDGE ( 'NONE', *, *, #22111, .T. ) ;
#30051=CARTESIAN_POINT ( 'NONE',  ( -11.86440526039950072, 1432.217533829589911, 149.9810751051169859 ) ) ;
#30052=VECTOR ( 'NONE', #33118, 1000.000000000000114 ) ;
#30054=CARTESIAN_POINT ( 'NONE',  ( -27.75954458800000069, 1464.244195522129985, 269.7078801315980172 ) ) ;
#30057=CARTESIAN_POINT ( 'NONE',  ( 33.93383221862509913, 1451.576073990769828, 135.5842236506620111 ) ) ;
#30059=CARTESIAN_POINT ( 'NONE',  ( -11.56485986500000074, 1418.759067621630265, 229.1292871074979871 ) ) ;
#30060=CARTESIAN_POINT ( 'NONE',  ( -15.95951032299999817, 1459.271785846329976, 230.7209114582980192 ) ) ;
#30063=CARTESIAN_POINT ( 'NONE',  ( -27.20455118562970043, 1413.128951532790097, 269.2362726868500431 ) ) ;
#30065=CARTESIAN_POINT ( 'NONE',  ( -3.531105454731040094, 1489.723025786869812, 181.7179317627199850 ) ) ;
#30066=ORIENTED_EDGE ( 'NONE', *, *, #106664, .T. ) ;
#30067=EDGE_LOOP ( 'NONE', ( #71041, #66138, #42369, #29131 ) ) ;
#30069=CARTESIAN_POINT ( 'NONE',  ( 4.726680758722174858, 1423.629136535139196, 183.9804056333954065 ) ) ;
#30070=VECTOR ( 'NONE', #11331, 1000.000000000000000 ) ;
#30073=CARTESIAN_POINT ( 'NONE',  ( -13.98188209669999971, 1440.433068879009852, 188.7552081789980036 ) ) ;
#30074=CARTESIAN_POINT ( 'NONE',  ( -8.324962519149999840E-16, 1519.913060387329779, 209.1218459616979999 ) ) ;
#30079=DIRECTION ( 'NONE',  ( -0.000000000000000000, -0.000000000000000000, 1.000000000000000000 ) ) ;
#30081=CARTESIAN_POINT ( 'NONE',  ( -18.71766394247640264, 1412.839174955069893, 270.0884054360959681 ) ) ;
#30082=CARTESIAN_POINT ( 'NONE',  ( -29.16177349730000046, 1435.516078635969961, 135.2137962254980152 ) ) ;
#30085=ORIENTED_EDGE ( 'NONE', *, *, #59616, .T. ) ;
#30087=CARTESIAN_POINT ( 'NONE',  ( 35.99660812079667949, 1461.957472332656607, 269.2276724049037284 ) ) ;
#30093=CARTESIAN_POINT ( 'NONE',  ( -18.33450183844069770, 1415.542389211280124, 207.5683613237780207 ) ) ;
#30095=CARTESIAN_POINT ( 'NONE',  ( -14.66444439270000011, 1426.817899515830049, 221.8925448643979905 ) ) ;
#30096=CARTESIAN_POINT ( 'NONE',  ( 12.00387303569999986, 1415.296882282229944, 222.4718873070980294 ) ) ;
#30102=CARTESIAN_POINT ( 'NONE',  ( -23.55479550185249948, 1448.068792179548609, 215.4543074554471787 ) ) ;
#30104=CARTESIAN_POINT ( 'NONE',  ( 17.95976239039625355, 1458.835784221633276, 228.1005955697006300 ) ) ;
#30106=CARTESIAN_POINT ( 'NONE',  ( -4.116702583572917185, 1440.040413356634190, 185.4452710716742558 ) ) ;
#30107=CARTESIAN_POINT ( 'NONE',  ( 2.409586283469999923, 1426.663880916129983, 144.1938086916980239 ) ) ;
#30108=CARTESIAN_POINT ( 'NONE',  ( 21.63007974809999823, 1410.588455781430184, 201.8364362340880120 ) ) ;
#30110=CARTESIAN_POINT ( 'NONE',  ( -27.12363451785340018, 1494.958770392079941, 210.5675194828440056 ) ) ;
#30113=CARTESIAN_POINT ( 'NONE',  ( 24.34316872452072644, 1445.447417981560648, 214.1587588598165723 ) ) ;
#30114=CARTESIAN_POINT ( 'NONE',  ( 2.500000000000000000, 1439.595905107460112, 166.5328618461109897 ) ) ;
#30119=B_SPLINE_SURFACE_WITH_KNOTS ( 'NONE', 5, 5, ( 
 ( #74588, #74036, #57253, #33110, #101390, #6263, #110371, #101957, #91379 ),
 ( #48846, #108724, #15191, #5727, #59446, #33651, #24685, #58881, #93014 ),
 ( #93557, #16286, #32014, #48288, #82431, #76776, #68403, #10120, #28020 ),
 ( #26928, #17945, #62208, #44291, #61117, #70069, #18496, #60553, #78435 ),
 ( #25797, #94115, #34769, #93, #68956, #95232, #16829, #69509, #61653 ),
 ( #8451, #9013, #102507, #103059, #59996, #103631, #17386, #104181, #52692 ),
 ( #19047, #51584, #35321, #1748, #52141, #34217, #70611, #79006, #43186 ),
 ( #86273, #94674, #86828, #9559, #44854, #35886, #42624, #43729, #85716 ),
 ( #27465, #95780, #77882, #104731, #1190, #53249, #2308, #51031, #77338 ) ),
 .UNSPECIFIED., .F., .F., .F.,
 ( 6, 3, 6 ),
 ( 6, 3, 6 ),
 ( 1.672764195910000140, 7.352908628769999844, 11.41845199609999995 ),
 ( 0.000000000000000000, 1.000000000000000000, 2.000000000000000000 ),
 .UNSPECIFIED. ) ;
#30124=CARTESIAN_POINT ( 'NONE',  ( -2.977093675850119858, 1421.750415281239839, 122.8791396966890090 ) ) ;
#30125=EDGE_CURVE ( 'NONE', #22625, #51991, #44813, .T. ) ;
#30126=CARTESIAN_POINT ( 'NONE',  ( -36.56841705501010154, 1449.771330042539830, 136.2670577573030073 ) ) ;
#30127=CARTESIAN_POINT ( 'NONE',  ( 2.050360166999971590, 1417.315232216300956, 233.1613795969499847 ) ) ;
#30128=CARTESIAN_POINT ( 'NONE',  ( -2.500000000000000000, 1419.382781980330037, 144.1108508878979819 ) ) ;
#30129=ADVANCED_FACE ( 'NONE', ( #14133 ), #108757, .T. ) ;
#30131=CARTESIAN_POINT ( 'NONE',  ( -44.84558622350979817, 1443.398794768399966, 269.6928110531539460 ) ) ;
#30132=CARTESIAN_POINT ( 'NONE',  ( 36.30692425169570470, 1440.913060387340010, 253.4096818480309707 ) ) ;
#30133=EDGE_CURVE ( 'NONE', #7608, #28737, #78099, .T. ) ;
#30135=FACE_OUTER_BOUND ( 'NONE', #90874, .T. ) ;
#30138=CARTESIAN_POINT ( 'NONE',  ( -1.831351320822103057, 1484.703635175746513, 182.8316381206172139 ) ) ;
#30141=SPHERICAL_SURFACE ( 'NONE', #55694, 2.000000000000000000 ) ;
#30142=CARTESIAN_POINT ( 'NONE',  ( -11.97313827979999878, 1507.452590393829951, 233.5302037296980018 ) ) ;
#30145=CARTESIAN_POINT ( 'NONE',  ( 5.731992211021079697, 1423.315380817839923, 95.16526208845120038 ) ) ;
#30147=DIRECTION ( 'NONE',  ( -0.03489949670250495212, 0.9993908270190956511, 0.000000000000000000 ) ) ;
#30148=CARTESIAN_POINT ( 'NONE',  ( 2.439426257200000059, 1464.676489092029897, 236.7027241286980086 ) ) ;
#30151=CARTESIAN_POINT ( 'NONE',  ( -0.7117640835210000683, 1450.958351866529938, 182.0239507108979922 ) ) ;
#30152=B_SPLINE_CURVE_WITH_KNOTS ( 'NONE', 3,
 ( #83256, #41800, #385, #101685, #49672, #24976, #59182, #93301, #84893, #42920, #100051 ),
 .UNSPECIFIED., .F., .F.,
 ( 4, 2, 1, 2, 2, 4 ),
 ( 0.000000000000000000, 0.2500000000008079648, 0.3750000000012119195, 0.4375000000012428947, 0.5000000000012738699, 1.000000000000000000 ),
 .UNSPECIFIED. ) ;
#30159=EDGE_CURVE ( 'NONE', #85608, #85844, #8183, .T. ) ;
#30164=ADVANCED_FACE ( 'NONE', ( #57287 ), #1469, .T. ) ;
#30167=DIRECTION ( 'NONE',  ( 0.000000000000000000, 0.000000000000000000, -1.000000000000000000 ) ) ;
#30168=CARTESIAN_POINT ( 'NONE',  ( 0.3281382665975389745, 1408.924519228060035, 194.1235352895430140 ) ) ;
#30169=CARTESIAN_POINT ( 'NONE',  ( 18.03509922239999952, 1424.785625889029916, 224.8563120260980099 ) ) ;
#30171=CARTESIAN_POINT ( 'NONE',  ( -18.91006071820000045, 1470.687815694929895, 190.2614882949980029 ) ) ;
#30172=CARTESIAN_POINT ( 'NONE',  ( -3.920301378251832780, 1425.361100976067974, 186.0700639595226278 ) ) ;
#30173=ORIENTED_EDGE ( 'NONE', *, *, #14490, .F. ) ;
#30174=ORIENTED_EDGE ( 'NONE', *, *, #43168, .F. ) ;
#30176=CARTESIAN_POINT ( 'NONE',  ( 2.500000000000000000, 1423.874532569730036, 167.3087045231979744 ) ) ;
#30177=CARTESIAN_POINT ( 'NONE',  ( -12.07610166159999920, 1433.870589910030048, 149.7869025145980117 ) ) ;
#30179=CARTESIAN_POINT ( 'NONE',  ( -20.43090246067709970, 1502.387636806920000, 190.5483151450440005 ) ) ;
#30182=CARTESIAN_POINT ( 'NONE',  ( 0.1668199292400000255, 1482.197866754329880, 181.9999787962979951 ) ) ;
#30185=CARTESIAN_POINT ( 'NONE',  ( -13.15726454016349933, 1414.996443537369942, 220.4820293315119955 ) ) ;
#30188=CARTESIAN_POINT ( 'NONE',  ( 6.688848995729999913, 1408.965348139829985, 221.4809136123979840 ) ) ;
#30190=CARTESIAN_POINT ( 'NONE',  ( -13.69143447902490074, 1435.956672119230007, 150.3296684258739901 ) ) ;
#30198=CARTESIAN_POINT ( 'NONE',  ( -5.356004379399999768E-09, 1414.987262868229891, 244.5742075744979900 ) ) ;
#30200=CARTESIAN_POINT ( 'NONE',  ( -1.539676316830000058, 1499.384663382030112, 181.1309619126980124 ) ) ;
#30201=CARTESIAN_POINT ( 'NONE',  ( -17.84751309889999860, 1410.898165759730091, 195.0518225682980074 ) ) ;
#30202=CARTESIAN_POINT ( 'NONE',  ( -9.945114259093980280, 1408.453226861988469, 270.1158808274767011 ) ) ;
#30204=CARTESIAN_POINT ( 'NONE',  ( -21.02448267839999829, 1430.224264779530131, 216.3628553705179911 ) ) ;
#30207=CARTESIAN_POINT ( 'NONE',  ( 27.03405864349999987, 1451.816809924330073, 135.7882993078979723 ) ) ;
#30211=CARTESIAN_POINT ( 'NONE',  ( 2.933320418000000096, 1509.029007662530148, 238.7073699979980006 ) ) ;
#30215=CARTESIAN_POINT ( 'NONE',  ( -23.59088797105159685, 1410.013994075070059, 208.8666440682279983 ) ) ;
#30216=EDGE_CURVE ( 'NONE', #19615, #6924, #6189, .T. ) ;
#30222=CARTESIAN_POINT ( 'NONE',  ( -5.750276878030000205, 1489.057775212530032, 235.2475806271980048 ) ) ;
#30225=CARTESIAN_POINT ( 'NONE',  ( 45.88361587542109987, 1440.912968092909750, 266.4122210649330214 ) ) ;
#30229=ORIENTED_EDGE ( 'NONE', *, *, #38446, .T. ) ;
#30232=CARTESIAN_POINT ( 'NONE',  ( 12.91578402941177117, 1442.900078521421165, 187.0543600294182625 ) ) ;
#30233=VERTEX_POINT ( 'NONE', #34253 ) ;
#30234=ORIENTED_EDGE ( 'NONE', *, *, #50251, .F. ) ;
#30237=CARTESIAN_POINT ( 'NONE',  ( 10.83158213179999940, 1507.705498442529915, 234.1612671678980178 ) ) ;
#30239=CARTESIAN_POINT ( 'NONE',  ( 18.87058201889760412, 1452.254085142500116, 144.5211760892889856 ) ) ;
#30241=CARTESIAN_POINT ( 'NONE',  ( -1.737082865695850131, 1434.406546800360047, 227.4539720509420135 ) ) ;
#30244=CARTESIAN_POINT ( 'NONE',  ( 0.03557119914497085950, 1409.441096220073405, 232.8945654604514175 ) ) ;
#30245=CARTESIAN_POINT ( 'NONE',  ( -13.78893342798370014, 1434.978972382549955, 148.5514418732119850 ) ) ;
#30246=CARTESIAN_POINT ( 'NONE',  ( -3.526376118873112198, 1486.285438481868141, 181.8638835509612761 ) ) ;
#30249=EDGE_CURVE ( 'NONE', #64180, #52333, #56818, .T. ) ;
#30254=CARTESIAN_POINT ( 'NONE',  ( -17.33645362950000290, 1414.996442546130083, 207.8511177337479978 ) ) ;
#30256=B_SPLINE_SURFACE_WITH_KNOTS ( 'NONE', 5, 5, ( 
 ( #60769, #104950, #28241, #51798, #61330, #10329, #62430, #9240, #94893 ),
 ( #19828, #85366, #78649, #43397, #42839, #76999, #1964, #77547, #36101 ),
 ( #95994, #70287, #89247, #106057, #97106, #20922, #12543, #90332, #99277 ),
 ( #81935, #88163, #80305, #22003, #54034, #65161, #37749, #62999, #106596 ),
 ( #11993, #37200, #38283, #38829, #56198, #47250, #97651, #13612, #47799 ),
 ( #20372, #30436, #81375, #89793, #64622, #46176, #71395, #55125, #105510 ),
 ( #98189, #46722, #5238, #80855, #11450, #30986, #45626, #29881, #71945 ),
 ( #3622, #39394, #3073, #29334, #63536, #28801, #79766, #54578, #4157 ),
 ( #64071, #55671, #4690, #21461, #107702, #13065, #88713, #73569, #98742 ),
 ( #72466, #73008, #107144, #67376, #57867, #7986, #41039, #14733, #6884 ),
 ( #76304, #48364, #58959, #91455, #74667, #41605, #15803, #75218, #100927 ),
 ( #66282, #23682, #75759, #100398, #84688, #33186, #90892, #92535, #14177 ) ),
 .UNSPECIFIED., .F., .F., .F.,
 ( 6, 3, 3, 6 ),
 ( 6, 3, 6 ),
 ( 0.000000000000000000, 17.84603210599999912, 40.51038747020000130, 67.03953034199999195 ),
 ( 168.7272174100000086, 210.9090217629999984, 253.0908261149999987 ),
 .UNSPECIFIED. ) ;
#30262=EDGE_CURVE ( 'NONE', #60533, #106936, #92493, .T. ) ;
#30264=CARTESIAN_POINT ( 'NONE',  ( -2.471608048749999842, 1438.194204504490017, 150.4833623973980252 ) ) ;
#30265=AXIS2_PLACEMENT_3D ( 'NONE', #10788, #18596, #79657 ) ;
#30272=CARTESIAN_POINT ( 'NONE',  ( 14.65669493600000095, 1419.764842872129975, 228.1228079084980038 ) ) ;
#30273=EDGE_CURVE ( 'NONE', #80494, #85181, #65456, .T. ) ;
#30277=CARTESIAN_POINT ( 'NONE',  ( -18.39234877020000170, 1409.555335359829996, 222.0045018765979705 ) ) ;
#30278=CARTESIAN_POINT ( 'NONE',  ( 15.08830123919999977, 1435.136539919019924, 148.7677820923979937 ) ) ;
#30280=CARTESIAN_POINT ( 'NONE',  ( -1.120746172849999889, 1422.344552812930033, 228.3276896694979996 ) ) ;
#30281=EDGE_CURVE ( 'NONE', #23487, #8175, #76846, .T. ) ;
#30282=CARTESIAN_POINT ( 'NONE',  ( -10.32735784461773498, 1511.163060387329779, 184.1749888460368538 ) ) ;
#30285=CARTESIAN_POINT ( 'NONE',  ( -36.36970013105189992, 1437.503838517560098, 136.5330191489490232 ) ) ;
#30286=CARTESIAN_POINT ( 'NONE',  ( 0.2133752674872349819, 1455.455537353240061, 183.1480552562999833 ) ) ;
#30287=CARTESIAN_POINT ( 'NONE',  ( -8.866214871307620982, 1407.269089423789865, 199.4203128504979929 ) ) ;
#30288=CARTESIAN_POINT ( 'NONE',  ( -13.01304944610000192, 1416.520646107730045, 196.6194520801979877 ) ) ;
#30291=CARTESIAN_POINT ( 'NONE',  ( 13.19881100609999969, 1434.900409811350073, 147.9457237049980165 ) ) ;
#30292=CARTESIAN_POINT ( 'NONE',  ( -39.48425676843219634, 1438.208629469910193, 134.0999999978120059 ) ) ;
#30293=CARTESIAN_POINT ( 'NONE',  ( 3.918670472299999208, 1441.329835342249908, 183.9132893515979958 ) ) ;
#30297=CARTESIAN_POINT ( 'NONE',  ( -8.169456507803459999, 1409.198344094930007, 221.6608919718729851 ) ) ;
#30299=ADVANCED_FACE ( 'NONE', ( #674 ), #100884, .F. ) ;
#30301=CARTESIAN_POINT ( 'NONE',  ( 13.45330080894279945, 1508.683615153560140, 233.3158278350460080 ) ) ;
#30302=CARTESIAN_POINT ( 'NONE',  ( 31.99856245131003263, 1416.544800951289290, 269.3157470449859829 ) ) ;
#30304=CARTESIAN_POINT ( 'NONE',  ( 19.44845634410000201, 1435.008643399599805, 209.6929102032310084 ) ) ;
#30310=CARTESIAN_POINT ( 'NONE',  ( 21.92444878910000483, 1509.678679009930192, 227.6602567687980070 ) ) ;
#30312=CARTESIAN_POINT ( 'NONE',  ( -28.43277596700509946, 1508.901247236620065, 208.8032485517010173 ) ) ;
#30319=CARTESIAN_POINT ( 'NONE',  ( -0.07918980841199839416, 1420.035738981420081, 183.9208618171100227 ) ) ;
#30322=CARTESIAN_POINT ( 'NONE',  ( 21.35611516500000207, 1409.658832362230214, 213.8729625945780128 ) ) ;
#30323=DIRECTION ( 'NONE',  ( 1.000000000000000000, 6.438963419392920087E-12, 0.000000000000000000 ) ) ;
#30325=CARTESIAN_POINT ( 'NONE',  ( -17.55365457510000127, 1423.589371376930103, 226.5287493268980086 ) ) ;
#30327=CARTESIAN_POINT ( 'NONE',  ( -11.65394379379999990, 1426.751588810729800, 138.2311371409980154 ) ) ;
#30328=CARTESIAN_POINT ( 'NONE',  ( 28.27965853590280076, 1508.150912785780065, 208.6308833624889587 ) ) ;
#30331=CARTESIAN_POINT ( 'NONE',  ( -2.077940277580000217, 1417.511812052730193, 234.8008807337979817 ) ) ;
#30334=CARTESIAN_POINT ( 'NONE',  ( 9.061547143302210117, 1507.228277554160059, 181.2342642626959730 ) ) ;
#30336=DIRECTION ( 'NONE',  ( -0.9417419115949053898, -0.3363363969979660806, 5.735553207809421716E-15 ) ) ;
#30337=CARTESIAN_POINT ( 'NONE',  ( -4.269964158086879458, 1441.123616076540202, 157.9266249594060127 ) ) ;
#30340=ORIENTED_EDGE ( 'NONE', *, *, #23580, .T. ) ;
#30341=CARTESIAN_POINT ( 'NONE',  ( 27.12601720510000192, 1508.017486052629920, 214.4687222129780082 ) ) ;
#30345=CARTESIAN_POINT ( 'NONE',  ( 15.71445409271430016, 1411.849835564349860, 191.4861124036179945 ) ) ;
#30346=CARTESIAN_POINT ( 'NONE',  ( 0.8080234665550000139, 1507.121502733429907, 181.0049083015979932 ) ) ;
#30349=CARTESIAN_POINT ( 'NONE',  ( -24.14851371715629824, 1452.064661293180052, 136.7193580640750099 ) ) ;
#30351=CARTESIAN_POINT ( 'NONE',  ( 10.89346138620000026, 1409.460417998529920, 228.8764123045980057 ) ) ;
#30354=CARTESIAN_POINT ( 'NONE',  ( 40.33550002370660081, 1439.280879844779975, 134.0999999981289932 ) ) ;
#30355=CARTESIAN_POINT ( 'NONE',  ( 11.99512495389999955, 1410.769353063830067, 192.9566925809980091 ) ) ;
#30356=EDGE_LOOP ( 'NONE', ( #14514, #89580, #102078, #67315 ) ) ;
#30357=CARTESIAN_POINT ( 'NONE',  ( 14.50701484619730053, 1436.101394055689980, 149.8878390185780063 ) ) ;
#30359=CARTESIAN_POINT ( 'NONE',  ( -17.38483621660000011, 1410.884422118429939, 225.7833436061980024 ) ) ;
#30362=CARTESIAN_POINT ( 'NONE',  ( 7.276816673734427532, 1410.543541011706338, 230.7087126424827659 ) ) ;
#30365=B_SPLINE_CURVE_WITH_KNOTS ( 'NONE', 3,
 ( #110419, #17994, #102000, #51626, #94718, #683 ),
 .UNSPECIFIED., .F., .F.,
 ( 4, 2, 4 ),
 ( 0.000000000000000000, 0.5000000000000000000, 1.000000000000000000 ),
 .UNSPECIFIED. ) ;
#30367=CARTESIAN_POINT ( 'NONE',  ( -3.482404635510000013, 1485.996524294529991, 182.2044824803980134 ) ) ;
#30369=CARTESIAN_POINT ( 'NONE',  ( 12.38749917709999870, 1442.753158610539913, 186.6620494205980094 ) ) ;
#30372=CARTESIAN_POINT ( 'NONE',  ( -1.116031910300000041, 1487.751631717630062, 231.2019806963980102 ) ) ;
#30373=CARTESIAN_POINT ( 'NONE',  ( 10.54743240270000015, 1416.216739748630062, 194.5501240980979958 ) ) ;
#30376=DIRECTION ( 'NONE',  ( 0.000000000000000000, 0.000000000000000000, 1.000000000000000000 ) ) ;
#30378=EDGE_LOOP ( 'NONE', ( #84007, #17525, #40344, #98944 ) ) ;
#30379=CARTESIAN_POINT ( 'NONE',  ( 38.91212894784649734, 1440.913060387330006, 266.0890524397909758 ) ) ;
#30380=EDGE_CURVE ( 'NONE', #50836, #94989, #53852, .T. ) ;
#30381=CARTESIAN_POINT ( 'NONE',  ( 18.80757778630000132, 1477.359834168530142, 228.3934860436980046 ) ) ;
#30382=EDGE_LOOP ( 'NONE', ( #52564, #35322, #30174, #32873 ) ) ;
#30383=CARTESIAN_POINT ( 'NONE',  ( -0.1414919779163680280, 1452.990816719059922, 183.2406312828490229 ) ) ;
#30384=CARTESIAN_POINT ( 'NONE',  ( -11.73709356416840066, 1426.695943276110029, 144.1748013770919954 ) ) ;
#30385=CARTESIAN_POINT ( 'NONE',  ( -7.105427357599999217E-15, 1410.913060387329779, 146.1721969590979882 ) ) ;
#30387=CARTESIAN_POINT ( 'NONE',  ( 22.34437782794419647, 1410.382989033719923, 206.2310609402520072 ) ) ;
#30390=CARTESIAN_POINT ( 'NONE',  ( -2.924372520659999530, 1509.089207866029938, 179.4306743669980051 ) ) ;
#30391=CARTESIAN_POINT ( 'NONE',  ( -13.80561504080000113, 1434.979606281209954, 147.8556475097979899 ) ) ;
#30393=CARTESIAN_POINT ( 'NONE',  ( 17.03246454329999793, 1459.348684287830110, 228.8776382905979858 ) ) ;
#30398=CARTESIAN_POINT ( 'NONE',  ( -0.1613635714646410035, 1507.107001889669846, 180.9028745560509890 ) ) ;
#30399=CARTESIAN_POINT ( 'NONE',  ( 15.95332790094227171, 1450.491793965960142, 220.3255767516768344 ) ) ;
#30408=ADVANCED_FACE ( 'NONE', ( #70104 ), #85784, .T. ) ;
#30409=CARTESIAN_POINT ( 'NONE',  ( -11.86115818179999870, 1431.976378517910007, 150.3873481853979968 ) ) ;
#30412=CARTESIAN_POINT ( 'NONE',  ( -0.2669431423167949458, 1507.379250670300053, 237.3398778801180242 ) ) ;
#30415=CARTESIAN_POINT ( 'NONE',  ( 11.76669623969999989, 1446.210547857770052, 187.6280433733980146 ) ) ;
#30417=CARTESIAN_POINT ( 'NONE',  ( -22.10800917430000112, 1457.439287980229892, 221.1683851152979798 ) ) ;
#30418=CARTESIAN_POINT ( 'NONE',  ( 2.500000000000000000, 1422.854123512330034, 153.3880924786980131 ) ) ;
#30419=CARTESIAN_POINT ( 'NONE',  ( -1.995213577869999755, 1485.172489985530092, 182.7707872721979925 ) ) ;
#30422=CARTESIAN_POINT ( 'NONE',  ( 3.441335375089999982, 1405.846167703030005, 267.5320912995980507 ) ) ;
#30424=CARTESIAN_POINT ( 'NONE',  ( 20.32935570889999966, 1410.869484758429962, 198.1387192155980017 ) ) ;
#30425=EDGE_CURVE ( 'NONE', #80080, #56812, #61875, .T. ) ;
#30426=CARTESIAN_POINT ( 'NONE',  ( 22.04553792400322365, 1430.060189992810137, 217.9753957608339192 ) ) ;
#30428=CARTESIAN_POINT ( 'NONE',  ( 10.47358766403681329, 1423.539380447800568, 137.3342994606528009 ) ) ;
#30431=CARTESIAN_POINT ( 'NONE',  ( -1.456572815626359985, 1450.690862357650076, 154.5176491767769846 ) ) ;
#30432=CARTESIAN_POINT ( 'NONE',  ( -1.631223015250512276, 1450.677821982117393, 183.2260624137571199 ) ) ;
#30433=CARTESIAN_POINT ( 'NONE',  ( -19.77942753878213722, 1485.921887965895849, 190.2803841538269012 ) ) ;
#30436=CARTESIAN_POINT ( 'NONE',  ( -28.02005515429999960, 1437.694013771309983, 248.0989693021979861 ) ) ;
#30439=CARTESIAN_POINT ( 'NONE',  ( 2.500000000000000000, 1439.638128487469885, 168.7284197398979870 ) ) ;
#30440=CARTESIAN_POINT ( 'NONE',  ( -1.749553261970000051, 1475.024750578529847, 269.6491148499980568 ) ) ;
#30441=CARTESIAN_POINT ( 'NONE',  ( -4.240547926179750071, 1446.386475563049999, 162.7475928564280139 ) ) ;
#30443=EDGE_CURVE ( 'NONE', #39980, #55879, #55960, .T. ) ;
#30444=CARTESIAN_POINT ( 'NONE',  ( -4.161170142461470434, 1448.299083512420111, 185.1109003841999936 ) ) ;
#30446=DIRECTION ( 'NONE',  ( 1.000000000000000000, 0.000000000000000000, 0.000000000000000000 ) ) ;
#30452=CARTESIAN_POINT ( 'NONE',  ( -6.426487077828900496, 1396.137478263319963, 218.0991803394280169 ) ) ;
#30453=EDGE_CURVE ( 'NONE', #29814, #68290, #104759, .T. ) ;
#30454=CARTESIAN_POINT ( 'NONE',  ( -14.65376645209999928, 1421.828940461630054, 227.7443339645980132 ) ) ;
#30455=CARTESIAN_POINT ( 'NONE',  ( -44.87824051230000322, 1439.395394557790041, 269.6922195959979831 ) ) ;
#30460=CARTESIAN_POINT ( 'NONE',  ( 10.90287724760000110, 1425.661448047130079, 108.0463068396980049 ) ) ;
#30462=PLANE ( 'NONE',  #96897 ) ;
#30468=CARTESIAN_POINT ( 'NONE',  ( 1.514918641279999978, 1508.378724870829956, 180.6682338044980156 ) ) ;
#30474=ORIENTED_EDGE ( 'NONE', *, *, #18488, .T. ) ;
#30475=CARTESIAN_POINT ( 'NONE',  ( -9.542476768429999368, 1396.305783361229942, 201.7625145225379981 ) ) ;
#30476=CARTESIAN_POINT ( 'NONE',  ( -21.56891384639999742, 1409.666263457130071, 211.8934866540579947 ) ) ;
#30478=CARTESIAN_POINT ( 'NONE',  ( -0.0002361465808533021280, 1396.089833730190094, 220.9538863869404395 ) ) ;
#30479=CARTESIAN_POINT ( 'NONE',  ( 3.820241900599999510E-10, 1475.513060387329915, 229.7676991014980104 ) ) ;
#30482=CARTESIAN_POINT ( 'NONE',  ( -1.366886485456169975, 1418.311017005800068, 185.2659375928420218 ) ) ;
#30483=CARTESIAN_POINT ( 'NONE',  ( 3.255198176620000439, 1410.302478098729807, 185.7993969742980198 ) ) ;
#30484=CARTESIAN_POINT ( 'NONE',  ( -11.99296593569999914, 1415.426952350729835, 195.1671397404979871 ) ) ;
#30485=CARTESIAN_POINT ( 'NONE',  ( -39.80824191364419562, 1446.385170600749916, 136.7374670100940079 ) ) ;
#30487=CARTESIAN_POINT ( 'NONE',  ( 11.05917849935010011, 1396.299255410490105, 208.6381233312569918 ) ) ;
#30488=CARTESIAN_POINT ( 'NONE',  ( -40.14607055839999816, 1442.238457364259830, 136.9587614600980032 ) ) ;
#30489=CARTESIAN_POINT ( 'NONE',  ( 11.78195448370000165, 1427.013926546230095, 147.4989304475980134 ) ) ;
#30490=CARTESIAN_POINT ( 'NONE',  ( 40.71170371759999540, 1443.968700575979938, 137.1160033506980085 ) ) ;
#30491=ORIENTED_EDGE ( 'NONE', *, *, #12475, .T. ) ;
#30495=ORIENTED_EDGE ( 'NONE', *, *, #33197, .T. ) ;
#30497=CARTESIAN_POINT ( 'NONE',  ( -15.24459383950000024, 1460.671739161529786, 228.9091320249980015 ) ) ;
#30499=CARTESIAN_POINT ( 'NONE',  ( 4.026786250540000722, 1418.913060387330006, 172.2701767054979882 ) ) ;
#30504=CARTESIAN_POINT ( 'NONE',  ( -8.899613412776929522, 1509.290876792079871, 180.4257793158479899 ) ) ;
#30506=CARTESIAN_POINT ( 'NONE',  ( 0.2465318334700000169, 1414.971352895729979, 225.7948685045980142 ) ) ;
#30508=ORIENTED_EDGE ( 'NONE', *, *, #79491, .F. ) ;
#30512=B_SPLINE_SURFACE_WITH_KNOTS ( 'NONE', 5, 5, ( 
 ( #61763, #37636, #89140, #29778, #12426, #98081 ),
 ( #80194, #63966, #3512, #44961, #97005, #20268 ),
 ( #4055, #54469, #95889, #88607, #70730, #71841 ),
 ( #53356, #105959, #20815, #96446, #38181, #79109 ),
 ( #89684, #19725, #12966, #106493, #81274, #2416 ),
 ( #88061, #11346, #45518, #79660, #56096, #66716 ) ),
 .UNSPECIFIED., .F., .F., .F.,
 ( 6, 6 ),
 ( 6, 6 ),
 ( 12.29943241800000031, 13.29386860920000046 ),
 ( 0.000000000000000000, 2.241783168430000028 ),
 .UNSPECIFIED. ) ;
#30513=CARTESIAN_POINT ( 'NONE',  ( -39.91344421577615265, 1431.322027499858677, 269.6087553545235096 ) ) ;
#30514=CARTESIAN_POINT ( 'NONE',  ( -0.4960463521180000224, 1409.436440922629799, 232.9663683892980259 ) ) ;
#30515=CARTESIAN_POINT ( 'NONE',  ( -11.86629849059999842, 1432.349867583040123, 149.9824147457980246 ) ) ;
#30518=CARTESIAN_POINT ( 'NONE',  ( -35.60841938633720360, 1440.913060387850010, 252.1178284797530011 ) ) ;
#30521=CARTESIAN_POINT ( 'NONE',  ( 34.59210919570099918, 1422.480570821680203, 269.7685429993599655 ) ) ;
#30525=CARTESIAN_POINT ( 'NONE',  ( 22.74061145230000136, 1409.707167064430223, 208.8534835263149887 ) ) ;
#30527=CARTESIAN_POINT ( 'NONE',  ( -0.1955981723043500320, 1414.913060387329779, 193.0575580317509718 ) ) ;
#30530=B_SPLINE_CURVE_WITH_KNOTS ( 'NONE', 3,
 ( #93269, #50723, #84854, #8154 ),
 .UNSPECIFIED., .F., .F.,
 ( 4, 4 ),
 ( 0.000000000000000000, 1.000000000000000000 ),
 .UNSPECIFIED. ) ;
#30531=CARTESIAN_POINT ( 'NONE',  ( 4.174991371165319265, 1421.544129702939927, 184.8960725920030086 ) ) ;
#30532=CARTESIAN_POINT ( 'NONE',  ( -1.350311178199999906, 1415.380319686529901, 233.1877845536980089 ) ) ;
#30533=CARTESIAN_POINT ( 'NONE',  ( 10.73499317030565869, 1424.972940667893681, 139.1354242632224611 ) ) ;
#30537=CARTESIAN_POINT ( 'NONE',  ( 18.90690578109999720, 1416.819760216030090, 210.0263053688559864 ) ) ;
#30538=EDGE_CURVE ( 'NONE', #58564, #93915, #20480, .T. ) ;
#30539=CARTESIAN_POINT ( 'NONE',  ( -0.02606214974820000169, 1415.758200430030001, 233.4550495725979999 ) ) ;
#30540=AXIS2_PLACEMENT_3D ( 'NONE', #86666, #87227, #62624 ) ;
#30547=FACE_OUTER_BOUND ( 'NONE', #41674, .T. ) ;
#30548=CARTESIAN_POINT ( 'NONE',  ( -33.91369269983620427, 1450.440666099120108, 136.2454419983430114 ) ) ;
#30549=CARTESIAN_POINT ( 'NONE',  ( 10.81000252826892094, 1424.640867483547481, 137.9989916216163692 ) ) ;
#30550=ORIENTED_EDGE ( 'NONE', *, *, #98649, .T. ) ;
#30555=B_SPLINE_CURVE_WITH_KNOTS ( 'NONE', 3,
 ( #24098, #92412, #24638, #58836 ),
 .UNSPECIFIED., .F., .F.,
 ( 4, 4 ),
 ( 0.000000000000000000, 1.000000000000000000 ),
 .UNSPECIFIED. ) ;
#30556=AXIS2_PLACEMENT_3D ( 'NONE', #92831, #101212, #7724 ) ;
#30557=CARTESIAN_POINT ( 'NONE',  ( 19.25328782020000062, 1456.551502757129811, 224.6704391798980112 ) ) ;
#30558=CARTESIAN_POINT ( 'NONE',  ( 7.338487941162202155, 1438.798250299839538, 154.0100661331221090 ) ) ;
#30562=CARTESIAN_POINT ( 'NONE',  ( -2.500000000000000000, 1448.346004333310020, 162.8188153768979873 ) ) ;
#30563=CARTESIAN_POINT ( 'NONE',  ( -19.25079509060000049, 1425.764729490530044, 223.8566527953979914 ) ) ;
#30566=CARTESIAN_POINT ( 'NONE',  ( 19.00619812820000121, 1498.085718000629868, 188.9130380066980024 ) ) ;
#30567=CARTESIAN_POINT ( 'NONE',  ( 0.1586669955048189973, 1408.918601621900279, 232.2155333696709931 ) ) ;
#30568=CARTESIAN_POINT ( 'NONE',  ( -14.87168881317970026, 1430.147188212150240, 221.8136313441650032 ) ) ;
#30573=CARTESIAN_POINT ( 'NONE',  ( 11.84289190199999986, 1435.906080920110071, 147.6777950973980182 ) ) ;
#30576=CARTESIAN_POINT ( 'NONE',  ( 1.458547904730420175, 1497.341003214500006, 181.5395634206250008 ) ) ;
#30578=CARTESIAN_POINT ( 'NONE',  ( -13.19308827171470888, 1443.110898837626110, 186.7803926656672218 ) ) ;
#30579=EDGE_CURVE ( 'NONE', #42283, #94490, #85057, .T. ) ;
#30580=CARTESIAN_POINT ( 'NONE',  ( 3.125347622798469782, 1407.037771531689941, 196.1218459610850005 ) ) ;
#30587=FACE_OUTER_BOUND ( 'NONE', #29794, .T. ) ;
#30589=B_SPLINE_CURVE_WITH_KNOTS ( 'NONE', 5,
 ( #87999, #95821, #103673, #53293, #87433, #52187, #10729, #83286, #89070, #23371, #49154, #92235 ),
 .UNSPECIFIED., .F., .F.,
 ( 6, 3, 3, 6 ),
 ( 0.000000000000000000, 0.5352712372119943218, 0.7510396948904395353, 1.000000000000000000 ),
 .UNSPECIFIED. ) ;
#30592=ORIENTED_EDGE ( 'NONE', *, *, #40504, .F. ) ;
#30593=ORIENTED_EDGE ( 'NONE', *, *, #105901, .T. ) ;
#30595=CARTESIAN_POINT ( 'NONE',  ( 13.60476386450000064, 1509.388149220730156, 235.0937967613979822 ) ) ;
#30597=CARTESIAN_POINT ( 'NONE',  ( 38.85519404911526209, 1429.283679779192880, 269.5904935888122509 ) ) ;
#30598=CARTESIAN_POINT ( 'NONE',  ( -15.89627787809999937, 1466.157227580030167, 250.4785789529980207 ) ) ;
#30599=CARTESIAN_POINT ( 'NONE',  ( -19.98678683960000058, 1488.002369500329905, 190.9648164086979705 ) ) ;
#30601=CARTESIAN_POINT ( 'NONE',  ( -11.08593463959999958, 1433.241398677389952, 151.6928038766980080 ) ) ;
#30603=CARTESIAN_POINT ( 'NONE',  ( 11.69113150085549968, 1426.726128796750118, 140.8862638668499869 ) ) ;
#30604=CARTESIAN_POINT ( 'NONE',  ( 17.06941271609999689, 1409.674943327129995, 224.1775087769979962 ) ) ;
#30606=CARTESIAN_POINT ( 'NONE',  ( -24.89939555210000321, 1440.978114073919869, 210.4300215348880272 ) ) ;
#30612=CARTESIAN_POINT ( 'NONE',  ( -6.421987433647831033E-11, 1412.000809220129895, 253.5556736965889968 ) ) ;
#30617=CARTESIAN_POINT ( 'NONE',  ( -14.82025763449999900, 1469.894974939130179, 269.8832922682979643 ) ) ;
#30618=CARTESIAN_POINT ( 'NONE',  ( -0.01304300961527469875, 1452.999749643619907, 183.2385070609109903 ) ) ;
#30619=DIRECTION ( 'NONE',  ( 0.000000000000000000, 1.000000000000000000, 0.000000000000000000 ) ) ;
#30628=CARTESIAN_POINT ( 'NONE',  ( -24.11323544790549889, 1410.974473862270088, 266.9955217767330282 ) ) ;
#30630=CARTESIAN_POINT ( 'NONE',  ( -3.545807321122369959, 1503.565769337949860, 181.1286887016880200 ) ) ;
#30631=VERTEX_POINT ( 'NONE', #75592 ) ;
#30635=CARTESIAN_POINT ( 'NONE',  ( 4.838327971944561767, 1423.497383055442015, 184.1236938972197663 ) ) ;
#30638=CARTESIAN_POINT ( 'NONE',  ( -4.463743402560000462, 1455.444639251629951, 184.7997051687979706 ) ) ;
#30639=CARTESIAN_POINT ( 'NONE',  ( -2.138103891696413239, 1450.041837599050496, 182.8913454565717984 ) ) ;
#30640=ORIENTED_EDGE ( 'NONE', *, *, #90530, .T. ) ;
#30641=CARTESIAN_POINT ( 'NONE',  ( -26.55738301740000296, 1435.430825181030059, 135.4649699188979923 ) ) ;
#30644=B_SPLINE_CURVE_WITH_KNOTS ( 'NONE', 3,
 ( #31965, #6211, #47133, #40362, #31409, #56632, #30859, #65591, #55542, #73985 ),
 .UNSPECIFIED., .F., .F.,
 ( 4, 2, 2, 2, 4 ),
 ( 0.000000000000000000, 0.2500000000000000000, 0.5000000000000000000, 0.7500000000000000000, 1.000000000000000000 ),
 .UNSPECIFIED. ) ;
#30647=CARTESIAN_POINT ( 'NONE',  ( -34.35685943343030146, 1420.725836707379813, 270.3439669880020233 ) ) ;
#30649=CARTESIAN_POINT ( 'NONE',  ( -3.844029647620000212, 1397.403954980429944, 196.6621108047980044 ) ) ;
#30652=EDGE_LOOP ( 'NONE', ( #108707, #37101, #15711, #76539, #46519, #31097, #21741 ) ) ;
#30653=CARTESIAN_POINT ( 'NONE',  ( 3.848752177033039068, 1425.850564267019990, 185.2803273145039213 ) ) ;
#30655=CARTESIAN_POINT ( 'NONE',  ( -14.50871316107370035, 1436.250700070630046, 149.9254544324789720 ) ) ;
#30660=CARTESIAN_POINT ( 'NONE',  ( -22.03783030909999852, 1435.764492934740019, 218.8250799062580256 ) ) ;
#30662=CARTESIAN_POINT ( 'NONE',  ( 12.37159932449999822, 1415.628674266529742, 222.5813136582980007 ) ) ;
#30667=CARTESIAN_POINT ( 'NONE',  ( -23.49345842294626863, 1448.339281494577790, 215.7559275228670117 ) ) ;
#30669=CARTESIAN_POINT ( 'NONE',  ( 3.464549481511450590, 1457.536217099257783, 228.5903248826067795 ) ) ;
#30670=CARTESIAN_POINT ( 'NONE',  ( 24.29597249405740200, 1452.001349292369923, 137.1828877068549843 ) ) ;
#30671=CARTESIAN_POINT ( 'NONE',  ( -4.088909611310605818, 1440.365459761272177, 185.3369552776610192 ) ) ;
#30673=CARTESIAN_POINT ( 'NONE',  ( 21.13430999730000082, 1409.651086755129882, 206.4149715960279821 ) ) ;
#30674=CARTESIAN_POINT ( 'NONE',  ( 16.87998458460000251, 1410.001061276529981, 226.1250098154980037 ) ) ;
#30677=CARTESIAN_POINT ( 'NONE',  ( 24.65284846709989708, 1440.998862877870124, 212.5088464049670165 ) ) ;
#30682=CARTESIAN_POINT ( 'NONE',  ( -4.301461581549999913, 1474.025770959829970, 270.1336327149980434 ) ) ;
#30687=CARTESIAN_POINT ( 'NONE',  ( 11.60004869885203682, 1426.384977201060110, 138.5819896183834601 ) ) ;
#30688=CARTESIAN_POINT ( 'NONE',  ( 2.736421577379605896, 1417.780736651565576, 234.0078274331876571 ) ) ;
#30689=CARTESIAN_POINT ( 'NONE',  ( -2.131931780892150297, 1484.252787751960113, 183.0899073119249749 ) ) ;
#30693=CARTESIAN_POINT ( 'NONE',  ( 32.50007417919399444, 1440.913060383219772, 245.3806142123629854 ) ) ;
#30697=ORIENTED_EDGE ( 'NONE', *, *, #54613, .F. ) ;
#30699=CARTESIAN_POINT ( 'NONE',  ( -19.08897089080889131, 1485.508016899335416, 189.6297277018092871 ) ) ;
#30707=CARTESIAN_POINT ( 'NONE',  ( -13.99233004660000113, 1471.311257370429985, 192.9715307993979820 ) ) ;
#30709=CARTESIAN_POINT ( 'NONE',  ( 2.256582165209999769, 1464.688065807730254, 236.3855123389979838 ) ) ;
#30711=ORIENTED_EDGE ( 'NONE', *, *, #17257, .F. ) ;
#30712=CARTESIAN_POINT ( 'NONE',  ( -0.5038386193489999831, 1452.963758663529916, 183.2902632327979973 ) ) ;
#30717=ORIENTED_EDGE ( 'NONE', *, *, #105777, .T. ) ;
#30726=CARTESIAN_POINT ( 'NONE',  ( 1.969460191385499659, 1408.981835452669884, 194.2610538800710174 ) ) ;
#30727=CARTESIAN_POINT ( 'NONE',  ( 0.8170660012889999768, 1410.321412113530187, 185.1427924109980268 ) ) ;
#30728=CARTESIAN_POINT ( 'NONE',  ( 2.967683387859999744, 1419.631902151829991, 185.2975656967979887 ) ) ;
#30730=CARTESIAN_POINT ( 'NONE',  ( 11.86572145839999948, 1432.317385115999969, 150.3971827882980108 ) ) ;
#30731=VECTOR ( 'NONE', #100390, 1000.000000000000000 ) ;
#30734=ORIENTED_EDGE ( 'NONE', *, *, #88087, .F. ) ;
#30735=( BOUNDED_CURVE ( )  B_SPLINE_CURVE ( 3, ( #3887, #27960, #19546, #70546 ),
 .UNSPECIFIED., .F., .F. ) 
 B_SPLINE_CURVE_WITH_KNOTS ( ( 4, 4 ),
 ( 6.205854994376239553, 6.217764911156499430 ),
 .UNSPECIFIED. ) 
 CURVE ( )  GEOMETRIC_REPRESENTATION_ITEM ( )  RATIONAL_B_SPLINE_CURVE ( ( 1.000000000000000000, 0.9999881795251216454, 0.9999881795251216454, 1.000000000000000000 ) ) 
 REPRESENTATION_ITEM ( '' )  );
#30737=CARTESIAN_POINT ( 'NONE',  ( 19.46683531208329754, 1455.865237448739890, 226.9917334617080087 ) ) ;
#30739=CARTESIAN_POINT ( 'NONE',  ( -12.77411984480000129, 1435.106351996289959, 150.5216832075980165 ) ) ;
#30741=CARTESIAN_POINT ( 'NONE',  ( -20.59467299441400101, 1507.692298009320211, 190.3942269768830045 ) ) ;
#30742=DIRECTION ( 'NONE',  ( -0.9993908270190948739, 0.03489949670252338876, 0.000000000000000000 ) ) ;
#30744=CARTESIAN_POINT ( 'NONE',  ( 0.3821805048270000005, 1506.433683729329914, 231.1012307613979999 ) ) ;
#30746=CARTESIAN_POINT ( 'NONE',  ( -46.05034235197370407, 1440.465840779690097, 266.6770621315579888 ) ) ;
#30750=CARTESIAN_POINT ( 'NONE',  ( 2.599891563601349986, 1407.016599241430185, 221.9593604902549941 ) ) ;
#30751=CARTESIAN_POINT ( 'NONE',  ( -13.09971517241789840, 1434.834136867550114, 149.3121823613580261 ) ) ;
#30753=CARTESIAN_POINT ( 'NONE',  ( 6.037826478620000437, 1422.573110035629952, 122.8776253759980079 ) ) ;
#30756=CARTESIAN_POINT ( 'NONE',  ( 31.95512683339999427, 1438.870446869690113, 244.1805851180980085 ) ) ;
#30757=CARTESIAN_POINT ( 'NONE',  ( -27.89257148229999927, 1508.131979113730040, 206.8378734316980285 ) ) ;
#30761=CARTESIAN_POINT ( 'NONE',  ( -3.129456141073420294, 1407.723287498587752, 270.1357490256495453 ) ) ;
#30762=CARTESIAN_POINT ( 'NONE',  ( -28.01490336700000228, 1439.098491831259935, 231.6874816054980215 ) ) ;
#30763=CARTESIAN_POINT ( 'NONE',  ( -29.34276002924985605, 1509.949525637511897, 205.4620678841161237 ) ) ;
#30764=ADVANCED_FACE ( 'NONE', ( #24033 ), #67187, .T. ) ;
#30766=CARTESIAN_POINT ( 'NONE',  ( -16.28005140691599806, 1452.344548464809804, 146.9042424669629838 ) ) ;
#30767=CARTESIAN_POINT ( 'NONE',  ( 27.86006176749999952, 1451.482664390230184, 136.1185673336979676 ) ) ;
#30770=CARTESIAN_POINT ( 'NONE',  ( 14.45750538832999865, 1416.828039266780024, 196.8520486936070029 ) ) ;
#30771=CARTESIAN_POINT ( 'NONE',  ( 14.44412043019999992, 1509.548839716430166, 235.4430145842979982 ) ) ;
#30773=VERTEX_POINT ( 'NONE', #66646 ) ;
#30774=CARTESIAN_POINT ( 'NONE',  ( -10.81004456478011022, 1424.641001814318315, 137.9990871386040965 ) ) ;
#30775=CARTESIAN_POINT ( 'NONE',  ( -24.12012278076839777, 1411.115370491980002, 208.7864916066450007 ) ) ;
#30779=CARTESIAN_POINT ( 'NONE',  ( -1.355861272130000073, 1507.642012711630059, 237.1707191107980179 ) ) ;
#30782=CARTESIAN_POINT ( 'NONE',  ( 44.67025355869130010, 1449.989991176380045, 267.0226189060550155 ) ) ;
#30788=AXIS2_PLACEMENT_3D ( 'NONE', #72730, #55382, #74397 ) ;
#30791=ORIENTED_EDGE ( 'NONE', *, *, #105016, .T. ) ;
#30794=CARTESIAN_POINT ( 'NONE',  ( -22.32273759649999789, 1409.692587561330129, 207.4115339668879869 ) ) ;
#30799=CARTESIAN_POINT ( 'NONE',  ( 19.12386044593656464, 1456.237284512719043, 225.8522710147555870 ) ) ;
#30800=CARTESIAN_POINT ( 'NONE',  ( -19.68012578990143879, 1509.621020740076119, 231.2488516338165994 ) ) ;
#30801=CARTESIAN_POINT ( 'NONE',  ( 0.03683343699197529769, 1409.591418101985710, 233.0054887270072470 ) ) ;
#30802=CARTESIAN_POINT ( 'NONE',  ( -17.12205713392949846, 1425.049461331939938, 191.3399107580359839 ) ) ;
#30806=CARTESIAN_POINT ( 'NONE',  ( 11.73563908010000034, 1425.610159190430068, 144.1657657165980027 ) ) ;
#30808=CARTESIAN_POINT ( 'NONE',  ( 14.97660093000000003, 1430.165149126429924, 219.6133832206979832 ) ) ;
#30809=VECTOR ( 'NONE', #13166, 999.9999999999998863 ) ;
#30810=CARTESIAN_POINT ( 'NONE',  ( -12.78690713350000152, 1416.828040475229955, 195.5394874918979724 ) ) ;
#30817=CARTESIAN_POINT ( 'NONE',  ( -1.643576684049999903, 1435.943783413959864, 150.4860296878979682 ) ) ;
#30819=CARTESIAN_POINT ( 'NONE',  ( 11.93316829419999969, 1433.461071242199978, 150.0216595702979703 ) ) ;
#30821=CARTESIAN_POINT ( 'NONE',  ( 23.03655028440000052, 1458.194572356429944, 255.3819207682979595 ) ) ;
#30826=CARTESIAN_POINT ( 'NONE',  ( 16.30658698069999701, 1422.109838810029942, 227.2734734342979834 ) ) ;
#30828=LINE ( 'NONE', #75063, #50235 ) ;
#30829=CARTESIAN_POINT ( 'NONE',  ( -18.03119042859999865, 1409.707603974429958, 223.6208843684979968 ) ) ;
#30830=CARTESIAN_POINT ( 'NONE',  ( 1.548533272784429871, 1416.259629939349907, 190.3356629014230066 ) ) ;
#30834=CARTESIAN_POINT ( 'NONE',  ( 2.869862706494750323E-07, 1407.180374304939960, 196.1048350723650060 ) ) ;
#30837=CARTESIAN_POINT ( 'NONE',  ( -10.59708786280000048, 1416.824060884729988, 223.7633362045980050 ) ) ;
#30838=CARTESIAN_POINT ( 'NONE',  ( 0.2151085986704019959, 1454.487371074299745, 183.1895884522399740 ) ) ;
#30839=CARTESIAN_POINT ( 'NONE',  ( -12.34660213732820111, 1407.716881338870053, 203.8968045877159909 ) ) ;
#30840=CARTESIAN_POINT ( 'NONE',  ( -16.05891525839999900, 1416.823418193329871, 200.6086608930380066 ) ) ;
#30841=CARTESIAN_POINT ( 'NONE',  ( -27.98425287095180281, 1508.960817695580090, 210.6693023723670137 ) ) ;
#30842=CARTESIAN_POINT ( 'NONE',  ( 13.19854548049999998, 1434.900412801370067, 149.1898584671980075 ) ) ;
#30843=CARTESIAN_POINT ( 'NONE',  ( -27.68326325459999993, 1436.793383437599914, 136.7538416525980267 ) ) ;
#30847=CARTESIAN_POINT ( 'NONE',  ( -2.382436964801009083, 1426.901689560119166, 137.0999999980979567 ) ) ;
#30853=CARTESIAN_POINT ( 'NONE',  ( 14.25697645713727368, 1408.402952620560427, 269.5859324265298369 ) ) ;
#30856=CARTESIAN_POINT ( 'NONE',  ( 3.431952426600000106, 1439.695211740410059, 184.5361447059979980 ) ) ;
#30859=CARTESIAN_POINT ( 'NONE',  ( -26.81029417419344085, 1435.596821286595059, 135.9924056800833227 ) ) ;
#30860=CARTESIAN_POINT ( 'NONE',  ( -29.75012120250000081, 1509.993914124430148, 208.5595671623779879 ) ) ;
#30861=DIRECTION ( 'NONE',  ( 0.9445946449598763284, 0.000000000000000000, -0.3282391760791590340 ) ) ;
#30862=CARTESIAN_POINT ( 'NONE',  ( -16.22808440654519657, 1409.858776212460043, 226.2137158441180134 ) ) ;
#30864=ORIENTED_EDGE ( 'NONE', *, *, #9971, .T. ) ;
#30867=CARTESIAN_POINT ( 'NONE',  ( -22.53878221424140094, 1411.058442688259902, 212.0450776560099939 ) ) ;
#30869=CARTESIAN_POINT ( 'NONE',  ( -0.08494223902299619100, 1420.329338498939933, 183.4000416936310103 ) ) ;
#30870=CARTESIAN_POINT ( 'NONE',  ( 0.1397974034109999986, 1466.394005007729902, 235.6966919797980040 ) ) ;
#30871=CARTESIAN_POINT ( 'NONE',  ( 17.72062905389999798, 1409.531878389729854, 220.9701597516980200 ) ) ;
#30872=CARTESIAN_POINT ( 'NONE',  ( -1.793243496752610078, 1419.496505211239764, 185.6405350652080131 ) ) ;
#30879=CARTESIAN_POINT ( 'NONE',  ( -23.64337474990000132, 1435.765697120489904, 212.0350067752380028 ) ) ;
#30882=CARTESIAN_POINT ( 'NONE',  ( -4.362798112068619005, 1485.138149384289818, 183.3481005963789983 ) ) ;
#30885=CARTESIAN_POINT ( 'NONE',  ( -4.235431282328379510, 1441.481098832679891, 163.6249080756429919 ) ) ;
#30887=VERTEX_POINT ( 'NONE', #110821 ) ;
#30888=ORIENTED_EDGE ( 'NONE', *, *, #17808, .T. ) ;
#30889=CARTESIAN_POINT ( 'NONE',  ( 28.89895421770000183, 1509.870172254329873, 212.1721160078579942 ) ) ;
#30892=EDGE_CURVE ( 'NONE', #77352, #68144, #38045, .T. ) ;
#30894=CARTESIAN_POINT ( 'NONE',  ( -11.10916966042679910, 1425.188513315250020, 141.1903306950420074 ) ) ;
#30895=CARTESIAN_POINT ( 'NONE',  ( 15.73565734446670206, 1409.462549778659877, 192.9527420705210261 ) ) ;
#30898=CARTESIAN_POINT ( 'NONE',  ( -25.08087365037879835, 1451.311483103210094, 137.5322042608940194 ) ) ;
#30900=CARTESIAN_POINT ( 'NONE',  ( -3.139202535909999980, 1484.175171382029930, 181.3327878135980313 ) ) ;
#30904=EDGE_CURVE ( 'NONE', #20305, #70446, #72757, .T. ) ;
#30905=CARTESIAN_POINT ( 'NONE',  ( 33.91369120165509798, 1451.728768194249824, 134.0999999980979851 ) ) ;
#30906=CARTESIAN_POINT ( 'NONE',  ( -39.76726435491990230, 1441.080129826450047, 136.8354390711329813 ) ) ;
#30913=CARTESIAN_POINT ( 'NONE',  ( 2.923521462801879967, 1410.394928839790055, 231.6309329194170061 ) ) ;
#30915=CARTESIAN_POINT ( 'NONE',  ( 0.1153852296620000162, 1450.909031046320024, 181.2445446237979922 ) ) ;
#30917=DIRECTION ( 'NONE',  ( 0.000000000000000000, 0.000000000000000000, 1.000000000000000000 ) ) ;
#30923=CARTESIAN_POINT ( 'NONE',  ( 12.45618503180000047, 1416.218047894730262, 196.1634441665979978 ) ) ;
#30926=ORIENTED_EDGE ( 'NONE', *, *, #8986, .T. ) ;
#30930=ORIENTED_EDGE ( 'NONE', *, *, #104902, .T. ) ;
#30931=CARTESIAN_POINT ( 'NONE',  ( 11.20854072760000086, 1414.996442553830093, 222.5314266876980014 ) ) ;
#30932=CARTESIAN_POINT ( 'NONE',  ( 19.38230263350000016, 1477.357356100929792, 227.8777628270980244 ) ) ;
#30938=CARTESIAN_POINT ( 'NONE',  ( 23.79000940093961347, 1411.113050310996186, 208.0033309891347812 ) ) ;
#30940=B_SPLINE_CURVE_WITH_KNOTS ( 'NONE', 5,
 ( #85306, #33256, #41672, #31604, #75290, #109436 ),
 .UNSPECIFIED., .F., .F.,
 ( 6, 6 ),
 ( -36.72426843339999891, -23.77825875729999794 ),
 .UNSPECIFIED. ) ;
#30942=CARTESIAN_POINT ( 'NONE',  ( -2.176538401690000235, 1507.722933799829889, 180.8157319044980227 ) ) ;
#30946=CARTESIAN_POINT ( 'NONE',  ( 17.25891509299999882, 1458.394333519329848, 230.3479255126979979 ) ) ;
#30947=CARTESIAN_POINT ( 'NONE',  ( -10.81441200649847190, 1424.654785931436436, 138.0165107421119046 ) ) ;
#30948=CARTESIAN_POINT ( 'NONE',  ( 19.76074652845624158, 1471.421996062696735, 270.0618306119852718 ) ) ;
#30952=CARTESIAN_POINT ( 'NONE',  ( -0.1193023033433100039, 1508.062965917820065, 180.6164617310760150 ) ) ;
#30956=CARTESIAN_POINT ( 'NONE',  ( -11.60004869885203682, 1426.461377484368768, 139.0976633225263015 ) ) ;
#30958=EDGE_LOOP ( 'NONE', ( #9344, #48826, #68030, #91635 ) ) ;
#30960=CARTESIAN_POINT ( 'NONE',  ( 20.61309283089999767, 1451.396441790530162, 213.2979450416279974 ) ) ;
#30961=CARTESIAN_POINT ( 'NONE',  ( -11.75672898480000050, 1431.354866972360014, 150.7379580337980087 ) ) ;
#30967=CARTESIAN_POINT ( 'NONE',  ( -18.47369489899999806, 1444.809210807949967, 226.6829861377979967 ) ) ;
#30969=CARTESIAN_POINT ( 'NONE',  ( -1.902213919270000053, 1485.189568804029932, 182.6864153717980059 ) ) ;
#30972=CARTESIAN_POINT ( 'NONE',  ( 9.927171082400001012, 1406.526425255430013, 267.4967810687980432 ) ) ;
#30973=CARTESIAN_POINT ( 'NONE',  ( 0.5133736986269999969, 1410.311097483629965, 185.0719951505979850 ) ) ;
#30974=CARTESIAN_POINT ( 'NONE',  ( 18.35208442190000255, 1410.878106859430090, 194.0788163582980133 ) ) ;
#30976=CARTESIAN_POINT ( 'NONE',  ( 24.54210601322609975, 1438.972376264970535, 212.5794209063584219 ) ) ;
#30978=DIRECTION ( 'NONE',  ( 0.09060005235378243427, 0.000000000000000000, 0.9958873583460591261 ) ) ;
#30979=CARTESIAN_POINT ( 'NONE',  ( 11.60004869885203682, 1425.463724408334429, 136.9266941120787919 ) ) ;
#30981=CARTESIAN_POINT ( 'NONE',  ( -2.425481787957049828, 1449.557072802999983, 154.2478782243809974 ) ) ;
#30982=CARTESIAN_POINT ( 'NONE',  ( -12.60275825409999939, 1445.063511714940205, 186.1741640718979909 ) ) ;
#30983=CARTESIAN_POINT ( 'NONE',  ( 0.8755637861606549999, 1450.882485026169888, 155.3353120183400051 ) ) ;
#30986=CARTESIAN_POINT ( 'NONE',  ( -12.48077398309999886, 1422.454772915230024, 243.9198229428980085 ) ) ;
#30987=ADVANCED_FACE ( 'NONE', ( #44048 ), #67912, .F. ) ;
#30988=CARTESIAN_POINT ( 'NONE',  ( -27.43355922089999765, 1507.980920696029898, 210.8261541407979962 ) ) ;
#30989=CARTESIAN_POINT ( 'NONE',  ( 4.261975124720000174, 1441.226018928259919, 159.2131618765980079 ) ) ;
#30990=CARTESIAN_POINT ( 'NONE',  ( -3.713685391600000330, 1474.937103713529950, 269.6455928562979807 ) ) ;
#30991=CARTESIAN_POINT ( 'NONE',  ( -11.04285492396053314, 1425.185071086764538, 139.1363384239375023 ) ) ;
#30993=CARTESIAN_POINT ( 'NONE',  ( -11.81076840317520649, 1486.509818544849622, 184.2931069832207243 ) ) ;
#30996=CARTESIAN_POINT ( 'NONE',  ( 11.60004869885206880, 1428.983126981192754, 137.0999999980979851 ) ) ;
#31000=CARTESIAN_POINT ( 'NONE',  ( -21.08955099079999940, 1409.649523736130050, 203.6792363195980045 ) ) ;
#31001=CARTESIAN_POINT ( 'NONE',  ( -15.03709947301200067, 1422.462674465683904, 228.7610913021540000 ) ) ;
#31002=ADVANCED_FACE ( 'NONE', ( #61420 ), #18264, .F. ) ;
#31003=CARTESIAN_POINT ( 'NONE',  ( 19.27715895977949145, 1456.031238095710933, 225.1558865330630397 ) ) ;
#31004=VERTEX_POINT ( 'NONE', #59750 ) ;
#31005=CARTESIAN_POINT ( 'NONE',  ( -3.749717822977947979, 1410.420720693452722, 232.2953181525738842 ) ) ;
#31010=CARTESIAN_POINT ( 'NONE',  ( -15.91560388664723824, 1409.468828761781651, 225.2517153350140688 ) ) ;
#31011=EDGE_CURVE ( 'NONE', #59795, #5604, #70576, .T. ) ;
#31012=CARTESIAN_POINT ( 'NONE',  ( 39.35235217899570159, 1449.784370637009943, 136.1661491917279818 ) ) ;
#31022=ORIENTED_EDGE ( 'NONE', *, *, #28403, .T. ) ;
#31023=CARTESIAN_POINT ( 'NONE',  ( -7.332112344980000529, 1396.169103392430088, 200.5548326435979902 ) ) ;
#31024=CARTESIAN_POINT ( 'NONE',  ( -22.12171058789999734, 1410.179612746230077, 213.4701572216380043 ) ) ;
#31025=CARTESIAN_POINT ( 'NONE',  ( -13.14575342714752360, 1444.761353586959785, 169.3990435656776015 ) ) ;
#31026=EDGE_CURVE ( 'NONE', #107294, #27091, #16573, .T. ) ;
#31027=CARTESIAN_POINT ( 'NONE',  ( 21.38883640680690945, 1509.706499414715836, 229.8114585089465152 ) ) ;
#31031=EDGE_CURVE ( 'NONE', #106344, #80080, #47353, .T. ) ;
#31032=CARTESIAN_POINT ( 'NONE',  ( -10.03977927579999907, 1416.217772597929979, 193.5333243407980035 ) ) ;
#31033=CARTESIAN_POINT ( 'NONE',  ( -40.51897750172089729, 1445.566678767979965, 136.8537167310219900 ) ) ;
#31034=CARTESIAN_POINT ( 'NONE',  ( 10.46340173671210039, 1396.278450429100076, 205.5098926540979960 ) ) ;
#31035=CARTESIAN_POINT ( 'NONE',  ( 1.121465867070000177, 1416.819756528530206, 190.1591350936980120 ) ) ;
#31036=CARTESIAN_POINT ( 'NONE',  ( 11.17161729519999902, 1425.146288952430041, 145.5104394328979822 ) ) ;
#31037=CARTESIAN_POINT ( 'NONE',  ( 2.911036452777519212, 1509.035170506769646, 179.6587957555915125 ) ) ;
#31041=VERTEX_POINT ( 'NONE', #45723 ) ;
#31046=CARTESIAN_POINT ( 'NONE',  ( -13.41813859969999889, 1434.820761659759910, 195.8250830286980033 ) ) ;
#31054=CARTESIAN_POINT ( 'NONE',  ( -8.884906359809958687, 1509.278151300639820, 180.4749538926859884 ) ) ;
#31056=CARTESIAN_POINT ( 'NONE',  ( 5.191738023060000096, 1415.425433635630043, 225.9364502213980188 ) ) ;
#31058=ORIENTED_EDGE ( 'NONE', *, *, #108252, .T. ) ;
#31060=CARTESIAN_POINT ( 'NONE',  ( -21.19481754039999899, 1509.644157119530064, 229.6418610316979994 ) ) ;
#31061=CARTESIAN_POINT ( 'NONE',  ( -16.18783066347087285, 1412.761876852201794, 269.3698687316306177 ) ) ;
#31066=CARTESIAN_POINT ( 'NONE',  ( -0.01304429014381880067, 1452.995120068570031, 183.2387050828319843 ) ) ;
#31067=CARTESIAN_POINT ( 'NONE',  ( -29.54320591851210409, 1440.913060386779989, 236.8530523014009930 ) ) ;
#31069=CARTESIAN_POINT ( 'NONE',  ( -0.4854401037883160352, 1465.014776865540171, 237.7376948412489810 ) ) ;
#31070=CARTESIAN_POINT ( 'NONE',  ( 7.395434848029290187, 1409.662563599529904, 270.3697498994749822 ) ) ;
#31074=CARTESIAN_POINT ( 'NONE',  ( 24.04079115580000092, 1410.979580360030013, 208.5492527449709996 ) ) ;
#31076=CARTESIAN_POINT ( 'NONE',  ( -9.911041288964989704, 1424.405074346095262, 139.1388764670732598 ) ) ;
#31088=DIRECTION ( 'NONE',  ( -0.002120872317203444275, 0.9999913661844078705, 0.003573437736364524098 ) ) ;
#31089=CARTESIAN_POINT ( 'NONE',  ( 9.726491193908251375E-12, 1408.913060387299993, 194.1220083575990145 ) ) ;
#31097=ORIENTED_EDGE ( 'NONE', *, *, #65232, .T. ) ;
#31100=ORIENTED_EDGE ( 'NONE', *, *, #101405, .T. ) ;
#31101=CARTESIAN_POINT ( 'NONE',  ( 1.472772998086409935, 1415.954755710899917, 191.9874378180679741 ) ) ;
#31102=B_SPLINE_CURVE_WITH_KNOTS ( 'NONE', 3,
 ( #58329, #108166, #39316, #90256, #14096, #92454, #81305, #4621, #38756, #22477, #31456, #107623, #72931, #13540, #47724, #23043, #5158, #30906, #65084, #99199, #82429, #76224, #636, #60548, #67841, #94110, #50487, #9555, #68952, #17381, #59442, #34765, #34213, #33106, #68399, #103626, #35317, #84063, #103054, #26924, #7361, #110368, #43725, #93553, #51580, #102503, #25793, #43182, #61113, #69504, #95228, #24682, #16825, #51026, #85712, #75684, #59992, #93010, #109825, #94670, #67295, #9008, #52137, #17941, #33647, #26352, #86269, #85161, #77878, #101952, #1186, #101387, #77334, #8447, #49926, #41526 ),
 .UNSPECIFIED., .F., .F.,
 ( 4, 3, 3, 3, 3, 3, 3, 3, 3, 3, 3, 3, 3, 3, 3, 3, 3, 3, 3, 3, 3, 3, 3, 3, 3, 4 ),
 ( 14.42287683710000046, 15.38027101718479983, 16.28803242362360137, 17.17436300713509922, 18.03299319179360083, 18.25245355743909670, 18.88350267378229930, 19.53205862555210004, 20.18761089655719942, 20.84551208257209964, 21.50053011586949836, 22.14300480878290145, 22.77552979124989818, 23.39142327888709971, 23.76042384637030125, 24.22815370064810025, 24.70787457184220060, 25.19935369834729855, 25.70478207845420116, 26.21374533000209794, 26.72094108690890124, 27.22151789532390254, 27.70638377802430341, 28.18141454126959999, 28.64088071977139904, 29.04792982929999923 ),
 .UNSPECIFIED. ) ;
#31104=B_SPLINE_CURVE_WITH_KNOTS ( 'NONE', 5,
 ( #32096, #107145, #65163, #66283, #31537, #40491, #82506, #83051, #6344 ),
 .UNSPECIFIED., .F., .F.,
 ( 6, 3, 6 ),
 ( 0.000000000000000000, 0.4236215395309710918, 1.000000000000000000 ),
 .UNSPECIFIED. ) ;
#31105=CARTESIAN_POINT ( 'NONE',  ( 22.87505597199999841, 1449.859370063780034, 219.3153813166979944 ) ) ;
#31106=CARTESIAN_POINT ( 'NONE',  ( 7.981679316644171074, 1438.119269022099388, 153.6915228190263178 ) ) ;
#31109=CARTESIAN_POINT ( 'NONE',  ( 15.95000232293457643, 1421.267744195325577, 227.4487368220951282 ) ) ;
#31110=CARTESIAN_POINT ( 'NONE',  ( -3.655438681029999692, 1446.309375400119961, 170.5481836841979941 ) ) ;
#31111=CARTESIAN_POINT ( 'NONE',  ( -18.76864046240000050, 1424.623155651629986, 224.6048661548979908 ) ) ;
#31114=CARTESIAN_POINT ( 'NONE',  ( 19.07205183430000162, 1488.300534546829795, 189.3974363681980151 ) ) ;
#31115=CARTESIAN_POINT ( 'NONE',  ( 0.5840752967518939576, 1410.310972847609946, 233.1572170071730170 ) ) ;
#31116=CARTESIAN_POINT ( 'NONE',  ( -34.65398121300953704, 1458.146139331663790, 269.5268082531298433 ) ) ;
#31117=ORIENTED_EDGE ( 'NONE', *, *, #52290, .T. ) ;
#31121=CARTESIAN_POINT ( 'NONE',  ( -4.159508860199999880, 1408.913060387329779, 226.9541261483979895 ) ) ;
#31122=CARTESIAN_POINT ( 'NONE',  ( -1.443308773824269364, 1409.130619237754445, 186.4549414979184689 ) ) ;
#31123=CARTESIAN_POINT ( 'NONE',  ( -12.69557643223229881, 1442.808827016684518, 186.1671471355434448 ) ) ;
#31127=CARTESIAN_POINT ( 'NONE',  ( -14.62022782577733082, 1410.806204324935607, 226.7253561846267758 ) ) ;
#31129=CARTESIAN_POINT ( 'NONE',  ( 23.79680546489999671, 1435.328500499490019, 137.0919807913980151 ) ) ;
#31130=CARTESIAN_POINT ( 'NONE',  ( -13.13810362587316050, 1443.057752665512453, 169.4001936047692425 ) ) ;
#31131=CARTESIAN_POINT ( 'NONE',  ( -13.85929582179999997, 1410.325638522630015, 227.0940391209979907 ) ) ;
#31137=CARTESIAN_POINT ( 'NONE',  ( 16.40028066370599902, 1414.913057860449953, 209.2777006334819987 ) ) ;
#31138=CARTESIAN_POINT ( 'NONE',  ( 12.96261739959999915, 1509.136740573229872, 234.0631307178979910 ) ) ;
#31140=CARTESIAN_POINT ( 'NONE',  ( -31.20802388950000150, 1451.456139917630026, 248.1710554650979930 ) ) ;
#31141=CARTESIAN_POINT ( 'NONE',  ( -19.90008872329999789, 1491.252934255230002, 189.9399603158979914 ) ) ;
#31142=CARTESIAN_POINT ( 'NONE',  ( -11.33778558790000091, 1433.696525961220004, 151.4746538488979866 ) ) ;
#31144=CARTESIAN_POINT ( 'NONE',  ( 11.69617228600709957, 1426.722709022770005, 141.2463821871190248 ) ) ;
#31145=CARTESIAN_POINT ( 'NONE',  ( 26.78593482470590104, 1474.097921906449983, 209.4579982356089829 ) ) ;
#31146=CARTESIAN_POINT ( 'NONE',  ( -26.26372997560000044, 1440.614374483860047, 137.6218707767980334 ) ) ;
#31151=CARTESIAN_POINT ( 'NONE',  ( -11.71000892829403206, 1509.446600626986992, 236.7426052959320089 ) ) ;
#31152=CARTESIAN_POINT ( 'NONE',  ( 1.255340816988079985E-08, 1408.894734928509934, 261.0927290538760417 ) ) ;
#31157=CARTESIAN_POINT ( 'NONE',  ( -5.207740107420000264, 1471.814797097629935, 270.0726242057979789 ) ) ;
#31158=DIRECTION ( 'NONE',  ( 0.000000000000000000, 1.000000000000000000, 0.000000000000000000 ) ) ;
#31160=CARTESIAN_POINT ( 'NONE',  ( 0.2051679708434860083, 1452.385543061679982, 183.1882097260399860 ) ) ;
#31166=CARTESIAN_POINT ( 'NONE',  ( -33.71036013506279971, 1416.517407414779882, 268.0042259019550102 ) ) ;
#31169=CARTESIAN_POINT ( 'NONE',  ( -3.548560001899690342, 1506.246208310000156, 181.0144377455499978 ) ) ;
#31170=AXIS2_PLACEMENT_3D ( 'NONE', #79281, #95516, #107087 ) ;
#31171=VERTEX_POINT ( 'NONE', #63631 ) ;
#31172=EDGE_LOOP ( 'NONE', ( #5844, #69635, #10686, #52855 ) ) ;
#31175=DIRECTION ( 'NONE',  ( 0.000000000000000000, 0.000000000000000000, -1.000000000000000000 ) ) ;
#31176=DIRECTION ( 'NONE',  ( -1.000000000000000000, 0.000000000000000000, 0.000000000000000000 ) ) ;
#31179=CARTESIAN_POINT ( 'NONE',  ( -15.95246779919999902, 1455.452439780930035, 189.1034377625979914 ) ) ;
#31182=CARTESIAN_POINT ( 'NONE',  ( -2.211711111070695068, 1449.929476652820540, 182.9238327313504442 ) ) ;
#31183=B_SPLINE_SURFACE_WITH_KNOTS ( 'NONE', 5, 5, ( 
 ( #93753, #14855, #85361, #27544, #300, #104253 ),
 ( #41176, #49045, #32224, #66404, #75350, #100523 ),
 ( #23802, #83724, #57994, #25449, #92127, #109490 ),
 ( #101060, #92669, #50147, #84274, #87464, #46021 ),
 ( #10755, #61726, #28649, #29197, #96965, #2925 ),
 ( #12928, #72321, #20230, #88564, #105358, #11848 ) ),
 .UNSPECIFIED., .F., .F., .F.,
 ( 6, 6 ),
 ( 6, 6 ),
 ( 9.285377752849999666, 26.18270615990000039 ),
 ( 0.000000000000000000, 2.000000000000000000 ),
 .UNSPECIFIED. ) ;
#31185=DIRECTION ( 'NONE',  ( 0.000000000000000000, 0.000000000000000000, -1.000000000000000000 ) ) ;
#31187=B_SPLINE_SURFACE_WITH_KNOTS ( 'NONE', 5, 5, ( 
 ( #98142, #32045, #20880, #72963, #107101, #48319 ),
 ( #30390, #98699, #74068, #13569, #47754, #81889 ),
 ( #55077, #5192, #39347, #107656, #30942, #99229 ),
 ( #22507, #56709, #90844, #14129, #82460, #108198 ),
 ( #14688, #65667, #23076, #57283, #48877, #83002 ),
 ( #8481, #49414, #7939, #57823, #58913, #51064 ) ),
 .UNSPECIFIED., .F., .F., .F.,
 ( 6, 6 ),
 ( 6, 6 ),
 ( 3.432284486139999924, 15.04427212800000113 ),
 ( 0.000000000000000000, 2.000000000000000000 ),
 .UNSPECIFIED. ) ;
#31188=CARTESIAN_POINT ( 'NONE',  ( -41.47274544121170692, 1445.558652941947912, 135.4389022873576778 ) ) ;
#31189=CARTESIAN_POINT ( 'NONE',  ( 1.343905436027461819, 1508.993419142904713, 238.7384818784190941 ) ) ;
#31190=CARTESIAN_POINT ( 'NONE',  ( -42.54898663771669476, 1436.084673314200018, 270.0692056436710118 ) ) ;
#31192=CARTESIAN_POINT ( 'NONE',  ( -5.776215019550000385, 1396.296062261430052, 198.6637670179979693 ) ) ;
#31197=CARTESIAN_POINT ( 'NONE',  ( 3.874528905232604625, 1425.932572816098173, 185.2903555449227326 ) ) ;
#31200=CARTESIAN_POINT ( 'NONE',  ( -2.062285449869999621, 1486.118212117930170, 181.8549132572979943 ) ) ;
#31201=B_SPLINE_CURVE_WITH_KNOTS ( 'NONE', 3,
 ( #79602, #2906, #37025, #54954 ),
 .UNSPECIFIED., .F., .F.,
 ( 4, 4 ),
 ( -49.62857964555200141, -30.36953107781529937 ),
 .UNSPECIFIED. ) ;
#31206=CARTESIAN_POINT ( 'NONE',  ( -2.177011892179100183, 1484.252254114900097, 183.0856693271300060 ) ) ;
#31207=CARTESIAN_POINT ( 'NONE',  ( -14.21330248699999999, 1430.152305291330094, 222.3202484490980169 ) ) ;
#31208=CARTESIAN_POINT ( 'NONE',  ( 0.000000000000000000, 1445.052233488290085, 126.8032249175980155 ) ) ;
#31209=CARTESIAN_POINT ( 'NONE',  ( 11.76669761379999990, 1446.210547856740050, 187.6280415629979927 ) ) ;
#31211=EDGE_CURVE ( 'NONE', #107129, #54363, #5914, .T. ) ;
#31214=CARTESIAN_POINT ( 'NONE',  ( -11.30499956576250042, 1428.976642403380083, 112.4490109703959888 ) ) ;
#31215=AXIS2_PLACEMENT_3D ( 'NONE', #38245, #64032, #98146 ) ;
#31216=CARTESIAN_POINT ( 'NONE',  ( -23.83335724643239573, 1446.583467845320911, 213.8372151209257481 ) ) ;
#31219=CARTESIAN_POINT ( 'NONE',  ( 25.23107375087169757, 1451.155107251089930, 137.3931022878719830 ) ) ;
#31220=CARTESIAN_POINT ( 'NONE',  ( 13.28956057169999916, 1415.163755984130148, 197.3206489009980089 ) ) ;
#31222=CARTESIAN_POINT ( 'NONE',  ( 19.78689921630000015, 1409.768476627529935, 198.2512349542980132 ) ) ;
#31225=CARTESIAN_POINT ( 'NONE',  ( -0.1622545728502209350, 1506.474306126712690, 187.1056287556957045 ) ) ;
#31226=CARTESIAN_POINT ( 'NONE',  ( 4.245220697766579399, 1441.395571263719830, 161.9150406115920191 ) ) ;
#31233=CARTESIAN_POINT ( 'NONE',  ( -0.2459700386814729911, 1408.921650059179910, 231.8163769252240058 ) ) ;
#31234=CARTESIAN_POINT ( 'NONE',  ( -2.755131347899999916, 1422.216165794629887, 90.98709265669789659 ) ) ;
#31236=CARTESIAN_POINT ( 'NONE',  ( 30.24726669678259938, 1509.969318215629983, 207.3401543782560168 ) ) ;
#31237=CARTESIAN_POINT ( 'NONE',  ( 11.60004869885391443, 1426.112340653894762, 139.0390921710123564 ) ) ;
#31239=CARTESIAN_POINT ( 'NONE',  ( -2.500000000000000000, 1432.110435327849927, 157.4891270399980101 ) ) ;
#31242=CARTESIAN_POINT ( 'NONE',  ( 28.69268220582149809, 1440.913060387340010, 233.8417140319789951 ) ) ;
#31245=CARTESIAN_POINT ( 'NONE',  ( 10.81518794224679958, 1424.921099295370141, 144.1705737284439977 ) ) ;
#31248=AXIS2_PLACEMENT_3D ( 'NONE', #42934, #15492, #77092 ) ;
#31249=CARTESIAN_POINT ( 'NONE',  ( 12.53380498098208840, 1442.773887284840384, 206.9039879563480326 ) ) ;
#31254=AXIS2_PLACEMENT_3D ( 'NONE', #20748, #12359, #98566 ) ;
#31255=CARTESIAN_POINT ( 'NONE',  ( 23.68614698517409067, 1509.855248197463879, 227.6068541032486223 ) ) ;
#31256=CIRCLE ( 'NONE', #22272, 4.014133627551895067 ) ;
#31257=CARTESIAN_POINT ( 'NONE',  ( -17.38483621660000011, 1410.884422118429939, 225.7833436061980024 ) ) ;
#31261=CARTESIAN_POINT ( 'NONE',  ( -13.02791578709999953, 1434.994518313060098, 194.2036555078979632 ) ) ;
#31263=CARTESIAN_POINT ( 'NONE',  ( 1.604557024660000053, 1465.957280275429866, 234.9244852315979699 ) ) ;
#31265=ORIENTED_EDGE ( 'NONE', *, *, #26905, .T. ) ;
#31266=CARTESIAN_POINT ( 'NONE',  ( -0.8347645832880000727, 1451.405209460129981, 182.9461533385980090 ) ) ;
#31270=EDGE_LOOP ( 'NONE', ( #71727, #80658, #10135, #8865, #92187, #45344 ) ) ;
#31271=ORIENTED_EDGE ( 'NONE', *, *, #77821, .T. ) ;
#31274=CARTESIAN_POINT ( 'NONE',  ( 34.88060122484030501, 1437.118155287319951, 136.5398807287430145 ) ) ;
#31275=CARTESIAN_POINT ( 'NONE',  ( 11.90000415720300175, 1434.913060496859998, 147.6452464505769910 ) ) ;
#31279=CARTESIAN_POINT ( 'NONE',  ( -3.321447364419999548, 1484.261043626330093, 183.3707343507980170 ) ) ;
#31280=CARTESIAN_POINT ( 'NONE',  ( 13.45932853639649984, 1409.383070496670143, 202.6355491842259937 ) ) ;
#31281=CARTESIAN_POINT ( 'NONE',  ( 18.80464664967999866, 1425.799544216437880, 225.6097399491019928 ) ) ;
#31283=CARTESIAN_POINT ( 'NONE',  ( -18.59366407810000155, 1470.691086342629887, 190.0416152128979945 ) ) ;
#31284=CARTESIAN_POINT ( 'NONE',  ( 10.96867220289999878, 1432.296152391259739, 151.7700998162980000 ) ) ;
#31285=CARTESIAN_POINT ( 'NONE',  ( -2.402297588538860218, 1450.020914723239912, 183.8092250355219903 ) ) ;
#31290=CARTESIAN_POINT ( 'NONE',  ( -12.30110944409999973, 1435.657202184449943, 151.0470392402980053 ) ) ;
#31291=CARTESIAN_POINT ( 'NONE',  ( 3.347731885920769895E-10, 1465.323236593859974, 238.9305512232619719 ) ) ;
#31292=CARTESIAN_POINT ( 'NONE',  ( -20.35676096567760140, 1499.986133293800094, 190.6179917588589774 ) ) ;
#31297=CARTESIAN_POINT ( 'NONE',  ( -46.27186622794469884, 1440.245173416720036, 267.5896806125069816 ) ) ;
#31301=CARTESIAN_POINT ( 'NONE',  ( -26.35475552313950232, 1507.985742420310089, 201.5462045797129917 ) ) ;
#31302=B_SPLINE_SURFACE_WITH_KNOTS ( 'NONE', 5, 5, ( 
 ( #91868, #90765, #49332, #84568, #30856, #108112 ),
 ( #7317, #22427, #66697, #108672, #24633, #58829 ),
 ( #6753, #92407, #57198, #41481, #83458, #75642 ),
 ( #31406, #14604, #65588, #48794, #92967, #31962 ),
 ( #66155, #7858, #107569, #56629, #14045, #6208 ),
 ( #39821, #74540, #48235, #57748, #82376, #101903 ) ),
 .UNSPECIFIED., .F., .F., .F.,
 ( 6, 6 ),
 ( 6, 6 ),
 ( 123.8981301339999987, 143.2822930469999960 ),
 ( 0.000000000000000000, 2.000000000000000000 ),
 .UNSPECIFIED. ) ;
#31306=EDGE_CURVE ( 'NONE', #100091, #32688, #35799, .T. ) ;
#31307=CARTESIAN_POINT ( 'NONE',  ( 39.71667995010000141, 1438.440173428300113, 259.0958843804980347 ) ) ;
#31308=DIRECTION ( 'NONE',  ( -1.000000000000000000, 0.000000000000000000, 0.000000000000000000 ) ) ;
#31309=CARTESIAN_POINT ( 'NONE',  ( -1.490778394210000135, 1464.110353063229923, 182.6238274118979916 ) ) ;
#31310=CARTESIAN_POINT ( 'NONE',  ( -17.60627563539999940, 1410.895669414830081, 194.0661810347980065 ) ) ;
#31311=CARTESIAN_POINT ( 'NONE',  ( -1.255439442925828430, 1407.658910741955879, 270.1375224078223596 ) ) ;
#31312=CARTESIAN_POINT ( 'NONE',  ( -25.89722382409999923, 1435.736014097309862, 225.2448095317979835 ) ) ;
#31313=CARTESIAN_POINT ( 'NONE',  ( -28.93366682225746089, 1509.926821294354568, 203.5275689439237965 ) ) ;
#31315=CARTESIAN_POINT ( 'NONE',  ( -10.29290297689570011, 1452.553624295069994, 150.4708687035819992 ) ) ;
#31316=CARTESIAN_POINT ( 'NONE',  ( 18.12896501882653411, 1435.130582088436313, 143.3945274339172329 ) ) ;
#31317=ORIENTED_EDGE ( 'NONE', *, *, #104403, .T. ) ;
#31319=CARTESIAN_POINT ( 'NONE',  ( 3.718673206215620104E-05, 1408.561116146350059, 270.4290838584209951 ) ) ;
#31325=CARTESIAN_POINT ( 'NONE',  ( -24.13064078950060320, 1411.115359567930000, 208.8754834058540268 ) ) ;
#31328=CARTESIAN_POINT ( 'NONE',  ( -13.93783161230000012, 1507.632723584029918, 232.3716436017979845 ) ) ;
#31330=CARTESIAN_POINT ( 'NONE',  ( 45.57954469825010335, 1446.130764200959902, 268.5106337247650004 ) ) ;
#31332=CARTESIAN_POINT ( 'NONE',  ( -12.61823209568500026, 1416.826860677879949, 222.0544590270410197 ) ) ;
#31333=CARTESIAN_POINT ( 'NONE',  ( 0.2417153426969999852, 1418.558758520830224, 184.6769579382979884 ) ) ;
#31338=CARTESIAN_POINT ( 'NONE',  ( 22.12673968580000050, 1409.685743163530105, 208.3470067452770138 ) ) ;
#31339=B_SPLINE_CURVE_WITH_KNOTS ( 'NONE', 5,
 ( #25219, #68934, #1168, #95211, #9538, #86804, #103607, #59423, #42599, #101932, #17921, #34195, #93535, #26332, #19024, #76755, #95759, #86247 ),
 .UNSPECIFIED., .F., .F.,
 ( 6, 3, 3, 3, 3, 6 ),
 ( 15.88432520349999955, 16.90079360149999843, 18.14364336469999728, 21.12354018079999918, 24.53920724549999832, 25.22570695429999788 ),
 .UNSPECIFIED. ) ;
#31340=CARTESIAN_POINT ( 'NONE',  ( 12.98890325061326756, 1442.943211643413406, 187.1799295177850695 ) ) ;
#31341=EDGE_LOOP ( 'NONE', ( #14382, #54359, #52125, #108902, #62336 ) ) ;
#31348=CARTESIAN_POINT ( 'NONE',  ( -4.140517654259704194, 1426.000593950702523, 186.1118291128992155 ) ) ;
#31350=B_SPLINE_CURVE_WITH_KNOTS ( 'NONE', 3,
 ( #36265, #1578, #38321, #87224, #26756, #17771, #62051, #4723, #104575, #18890, #10514, #29918, #60378, #47288, #18339, #96176, #19451, #53650, #35712, #69341, #72500, #106629, #52530, #86116, #38867, #86663, #87794, #2144, #9957, #11078, #70454, #45245, #26190, #60944, #44129, #95073, #78264, #13105, #61492, #51974 ),
 .UNSPECIFIED., .F., .F.,
 ( 4, 3, 3, 3, 3, 3, 3, 3, 3, 3, 3, 3, 3, 4 ),
 ( -1.449276807229999964, -1.377900617911430148, -1.266157031164990121, -1.152673605843979932, -1.038158481000059918, -0.9221425583362260481, -0.8054446481160930649, -0.6883773969095410283, -0.5712841841444460389, -0.4548595335433320841, -0.3393020229786609665, -0.2248662951613220606, -0.1117297126499861015, 0.000000000000000000 ),
 .UNSPECIFIED. ) ;
#31352=CARTESIAN_POINT ( 'NONE',  ( 33.91369120209999721, 1435.681798817170147, 134.0999999980979851 ) ) ;
#31356=CARTESIAN_POINT ( 'NONE',  ( -24.20611828920600317, 1508.692521244279988, 222.4038325357350061 ) ) ;
#31359=CARTESIAN_POINT ( 'NONE',  ( 12.58190538649999901, 1415.948532225030021, 222.2791103911980031 ) ) ;
#31367=CARTESIAN_POINT ( 'NONE',  ( 11.60004869885206880, 1428.983126981192754, 137.0999999980979851 ) ) ;
#31370=CARTESIAN_POINT ( 'NONE',  ( 11.21036242749999978, 1433.950538822089811, 151.6031954420979844 ) ) ;
#31371=CARTESIAN_POINT ( 'NONE',  ( 1.776356839399999804E-15, 1469.463552837929910, 265.6112251771979800 ) ) ;
#31374=CARTESIAN_POINT ( 'NONE',  ( 2.921131820879320440, 1415.930151663460038, 231.8786077272699799 ) ) ;
#31379=CARTESIAN_POINT ( 'NONE',  ( -17.19048262749999978, 1409.513365268830057, 224.2117643060980186 ) ) ;
#31381=CARTESIAN_POINT ( 'NONE',  ( -1.339831530989999964, 1424.180425965929999, 228.4049732387980214 ) ) ;
#31383=CARTESIAN_POINT ( 'NONE',  ( 5.451195050909999503E-14, 1410.389826760030019, 269.3346704430979912 ) ) ;
#31384=CARTESIAN_POINT ( 'NONE',  ( 3.810920848475609887E-07, 1407.244912221920004, 196.0950346751619691 ) ) ;
#31386=( BOUNDED_CURVE ( )  B_SPLINE_CURVE ( 3, ( #31279, #57062, #16651, #50317 ),
 .UNSPECIFIED., .F., .F. ) 
 B_SPLINE_CURVE_WITH_KNOTS ( ( 4, 4 ),
 ( 4.159034560815309867, 5.265743431342809977 ),
 .UNSPECIFIED. ) 
 CURVE ( )  GEOMETRIC_REPRESENTATION_ITEM ( )  RATIONAL_B_SPLINE_CURVE ( ( 1.000000000000000000, 0.9005109389839739409, 0.9005109389839739409, 1.000000000000000000 ) ) 
 REPRESENTATION_ITEM ( '' )  );
#31388=CARTESIAN_POINT ( 'NONE',  ( -8.218607532720000108, 1415.425433635630043, 224.6826798189979968 ) ) ;
#31390=CARTESIAN_POINT ( 'NONE',  ( -13.40477891429999957, 1409.381165581829919, 216.6964573264080229 ) ) ;
#31392=CARTESIAN_POINT ( 'NONE',  ( -14.64149002350000117, 1416.824060884929850, 198.5247578393980064 ) ) ;
#31395=CARTESIAN_POINT ( 'NONE',  ( 12.91318184880000075, 1434.774345493619876, 147.9456464303979715 ) ) ;
#31396=CARTESIAN_POINT ( 'NONE',  ( -26.79413161609999960, 1436.761919078669962, 136.7821860783980128 ) ) ;
#31397=CARTESIAN_POINT ( 'NONE',  ( 5.767944999630000069, 1441.815290517450194, 183.8476023479979915 ) ) ;
#31398=ORIENTED_EDGE ( 'NONE', *, *, #4863, .F. ) ;
#31404=CARTESIAN_POINT ( 'NONE',  ( 33.97073229624528778, 1418.068708379463715, 269.2736084937218379 ) ) ;
#31406=CARTESIAN_POINT ( 'NONE',  ( 2.500000000000000000, 1431.405490208399897, 183.1416673773980222 ) ) ;
#31409=CARTESIAN_POINT ( 'NONE',  ( -26.81185740190621303, 1435.935043934885243, 136.4231258368600663 ) ) ;
#31411=CARTESIAN_POINT ( 'NONE',  ( -27.78835038220000087, 1451.943064120830059, 135.3296735906980075 ) ) ;
#31412=CARTESIAN_POINT ( 'NONE',  ( -16.33802103553490070, 1410.720457927129928, 226.6282205582409972 ) ) ;
#31413=CARTESIAN_POINT ( 'NONE',  ( 0.4918970380822089705, 1416.941427595080086, 184.7882001716829734 ) ) ;
#31414=ORIENTED_EDGE ( 'NONE', *, *, #85617, .T. ) ;
#31420=CARTESIAN_POINT ( 'NONE',  ( -0.1687673399551990194, 1419.486623560560020, 184.4224968243179887 ) ) ;
#31421=CARTESIAN_POINT ( 'NONE',  ( 1.172684541229999988, 1466.870711192130102, 235.2669543350980064 ) ) ;
#31422=CARTESIAN_POINT ( 'NONE',  ( 19.25129681859999664, 1409.750010412430129, 220.2447021582979971 ) ) ;
#31423=B_SPLINE_SURFACE_WITH_KNOTS ( 'NONE', 5, 5, ( 
 ( #88573, #77953, #19694, #53897, #37049, #36503 ),
 ( #61193, #28658, #70147, #62288, #43803, #52220 ),
 ( #88032, #104810, #19124, #96416, #53324, #1825 ),
 ( #86347, #11316, #45486, #11856, #70699, #35398 ),
 ( #18570, #87472, #2386, #79628, #34840, #78514 ),
 ( #46029, #1259, #69031, #2932, #54440, #103132 ),
 ( #71245, #9631, #105368, #62863, #69586, #103704 ),
 ( #27004, #35960, #52765, #86904, #104260, #27551 ),
 ( #61733, #99137, #89651, #12394, #90752, #56617 ),
 ( #98600, #64485, #37606, #81791, #22414, #30843 ),
 ( #107004, #21864, #13474, #73969, #56063, #20781 ),
 ( #80157, #65576, #91309, #14031, #38151, #31396 ) ),
 .UNSPECIFIED., .F., .F., .F.,
 ( 6, 3, 3, 6 ),
 ( 6, 6 ),
 ( 13.64477700820000017, 16.39774826220000037, 20.55756172009999716, 23.69575850009999840 ),
 ( 0.000000000000000000, 1.506046440610000037 ),
 .UNSPECIFIED. ) ;
#31424=CARTESIAN_POINT ( 'NONE',  ( -1.981971470188760298, 1412.641733730590204, 186.1285722913719951 ) ) ;
#31426=CARTESIAN_POINT ( 'NONE',  ( -17.42096267240000174, 1423.098173955330140, 226.5666896228979965 ) ) ;
#31436=CARTESIAN_POINT ( 'NONE',  ( -3.481831347839449808, 1485.997118152289886, 182.2030801867670107 ) ) ;
#31437=CARTESIAN_POINT ( 'NONE',  ( -4.221414803702270291, 1441.605272108680083, 169.3185911052280233 ) ) ;
#31446=CARTESIAN_POINT ( 'NONE',  ( -11.74292464122704160, 1426.692342792548061, 144.5930205200747025 ) ) ;
#31447=CARTESIAN_POINT ( 'NONE',  ( 16.15586037378450257, 1410.120038459840089, 191.7753741660440028 ) ) ;
#31449=CARTESIAN_POINT ( 'NONE',  ( -11.43737779389999965, 1425.481201409729920, 144.1652972830979991 ) ) ;
#31455=B_SPLINE_CURVE_WITH_KNOTS ( 'NONE', 5,
 ( #83775, #73746, #107870, #13791, #99456, #39002, #73179, #107323, #47975 ),
 .UNSPECIFIED., .F., .F.,
 ( 6, 3, 6 ),
 ( 0.000000000000000000, 0.5000000000000000000, 1.000000000000000000 ),
 .UNSPECIFIED. ) ;
#31456=CARTESIAN_POINT ( 'NONE',  ( -40.01879385046350279, 1441.795747474259997, 136.9110126192350094 ) ) ;
#31461=VERTEX_POINT ( 'NONE', #5720 ) ;
#31462=CARTESIAN_POINT ( 'NONE',  ( 9.609922565670512284, 1410.623556455364223, 229.9593671579381464 ) ) ;
#31464=CARTESIAN_POINT ( 'NONE',  ( 0.1257759720830000094, 1452.989722137430135, 183.2438651275979851 ) ) ;
#31467=CARTESIAN_POINT ( 'NONE',  ( -28.25086642335310216, 1508.135711581739997, 208.8579954535609886 ) ) ;
#31468=CARTESIAN_POINT ( 'NONE',  ( 38.81202642569470385, 1436.797832264049930, 135.0591075470150031 ) ) ;
#31473=EDGE_LOOP ( 'NONE', ( #28780, #91404, #94951, #24964 ) ) ;
#31477=CARTESIAN_POINT ( 'NONE',  ( 41.10790882195649942, 1440.913060387330006, 268.6213595677239709 ) ) ;
#31478=CARTESIAN_POINT ( 'NONE',  ( -0.002351591770409689267, 1451.792435456469320, 154.0463020581492515 ) ) ;
#31479=ORIENTED_EDGE ( 'NONE', *, *, #36006, .T. ) ;
#31481=CARTESIAN_POINT ( 'NONE',  ( -16.40416249119999748, 1409.987717225529877, 191.8167551617980280 ) ) ;
#31483=CARTESIAN_POINT ( 'NONE',  ( 23.55087631299999984, 1411.110694763729953, 207.7642880164279973 ) ) ;
#31484=CARTESIAN_POINT ( 'NONE',  ( -4.363122395629999595, 1421.971318393930005, 184.5104903241980026 ) ) ;
#31486=CARTESIAN_POINT ( 'NONE',  ( 31.50789225850000008, 1415.566663160229837, 266.5723572024979831 ) ) ;
#31487=CARTESIAN_POINT ( 'NONE',  ( -12.40455451760000116, 1434.419853495040115, 146.4343135272980021 ) ) ;
#31490=CARTESIAN_POINT ( 'NONE',  ( 16.26126431490000002, 1459.229823316930151, 230.3673621847979973 ) ) ;
#31491=CARTESIAN_POINT ( 'NONE',  ( -11.60004869886986789, 1424.304888195492822, 137.2804668087435118 ) ) ;
#31492=CARTESIAN_POINT ( 'NONE',  ( -4.363122561674769528, 1421.971318449149976, 184.5104913919989826 ) ) ;
#31494=ORIENTED_EDGE ( 'NONE', *, *, #87635, .F. ) ;
#31498=CARTESIAN_POINT ( 'NONE',  ( 18.29465319566073234, 1446.505244253307637, 215.9117699586604999 ) ) ;
#31500=CARTESIAN_POINT ( 'NONE',  ( 18.59438456350000024, 1507.626747898329995, 188.5297968183980117 ) ) ;
#31501=CARTESIAN_POINT ( 'NONE',  ( -11.44980511867515993, 1425.806253551034388, 139.0985862314396684 ) ) ;
#31504=CARTESIAN_POINT ( 'NONE',  ( -19.59880086690000311, 1507.802454088529885, 229.4381582326980151 ) ) ;
#31506=CARTESIAN_POINT ( 'NONE',  ( -10.95785036490000053, 1431.503689836019930, 151.7245498010980214 ) ) ;
#31507=CARTESIAN_POINT ( 'NONE',  ( 19.02764298761669792, 1456.917174445179853, 225.6166628802600087 ) ) ;
#31509=CARTESIAN_POINT ( 'NONE',  ( 11.78818150890059968, 1426.417842412089840, 148.5075604377779825 ) ) ;
#31510=CARTESIAN_POINT ( 'NONE',  ( -21.97938480444670262, 1506.433683733529961, 209.5040264213440082 ) ) ;
#31512=CARTESIAN_POINT ( 'NONE',  ( -23.96120601207324796, 1411.110625406946610, 208.0854022759841655 ) ) ;
#31513=CARTESIAN_POINT ( 'NONE',  ( -2.685939447044066952, 1419.763153556473526, 137.0999999980978430 ) ) ;
#31514=CARTESIAN_POINT ( 'NONE',  ( -3.002432322850000279, 1486.001776092530008, 182.1376723879980091 ) ) ;
#31515=ORIENTED_EDGE ( 'NONE', *, *, #100121, .T. ) ;
#31517=CARTESIAN_POINT ( 'NONE',  ( 12.72718513819999941, 1407.064594780429843, 267.4694263162979837 ) ) ;
#31518=FACE_OUTER_BOUND ( 'NONE', #60292, .T. ) ;
#31519=CARTESIAN_POINT ( 'NONE',  ( 17.57165883560000097, 1410.882996087329957, 192.7623837702980154 ) ) ;
#31523=CARTESIAN_POINT ( 'NONE',  ( 23.14416256224673063, 1432.663507748254688, 215.7929284277614954 ) ) ;
#31524=EDGE_CURVE ( 'NONE', #14678, #105869, #35385, .T. ) ;
#31525=CARTESIAN_POINT ( 'NONE',  ( -24.86308739729999928, 1452.044818012130236, 135.5986755553979890 ) ) ;
#31526=CARTESIAN_POINT ( 'NONE',  ( 27.93978865640000109, 1508.083000434530049, 211.1815961025180286 ) ) ;
#31530=CARTESIAN_POINT ( 'NONE',  ( -12.19576017219999997, 1445.284187945309895, 186.5171125204979887 ) ) ;
#31532=CARTESIAN_POINT ( 'NONE',  ( -19.74181951150670500, 1486.027887478371213, 190.1836019666429820 ) ) ;
#31533=EDGE_CURVE ( 'NONE', #37815, #54528, #99416, .T. ) ;
#31536=CARTESIAN_POINT ( 'NONE',  ( -7.121584071090000023, 1409.161751583130126, 195.9581075130980139 ) ) ;
#31537=CARTESIAN_POINT ( 'NONE',  ( 20.31245888920532394, 1507.850143714011892, 228.7302838063898207 ) ) ;
#31538=CARTESIAN_POINT ( 'NONE',  ( 4.219804471239999799, 1441.618635230429845, 168.7222761371980084 ) ) ;
#31539=CARTESIAN_POINT ( 'NONE',  ( -3.776688141959999800, 1475.993142067930194, 267.8478539070980560 ) ) ;
#31540=FACE_OUTER_BOUND ( 'NONE', #101953, .T. ) ;
#31542=CARTESIAN_POINT ( 'NONE',  ( -9.324653930165572646, 1486.515044582724386, 183.2464455839941593 ) ) ;
#31544=CARTESIAN_POINT ( 'NONE',  ( 1.457628745286551286, 1507.679360684215908, 236.7889182220722546 ) ) ;
#31546=CARTESIAN_POINT ( 'NONE',  ( -45.67177343128329881, 1440.913044206929953, 266.1885934837860077 ) ) ;
#31549=FACE_OUTER_BOUND ( 'NONE', #9325, .T. ) ;
#31550=EDGE_CURVE ( 'NONE', #59085, #98070, #46136, .T. ) ;
#31552=CARTESIAN_POINT ( 'NONE',  ( -25.70445440479999988, 1412.495827564830051, 269.4333631909979658 ) ) ;
#31554=CARTESIAN_POINT ( 'NONE',  ( -7.554020802055777750, 1410.549877764319717, 230.8257970151002780 ) ) ;
#31561=CARTESIAN_POINT ( 'NONE',  ( 1.204096590079999967E-15, 1406.443991414029824, 146.1721969590979882 ) ) ;
#31563=EDGE_CURVE ( 'NONE', #52385, #94751, #17894, .T. ) ;
#31567=CARTESIAN_POINT ( 'NONE',  ( -2.416798835000000256, 1426.601114010129777, 146.0361887655980127 ) ) ;
#31571=CARTESIAN_POINT ( 'NONE',  ( 22.22116651786569719, 1509.699978059410114, 228.6323576840410112 ) ) ;
#31575=CARTESIAN_POINT ( 'NONE',  ( -10.84028228440000063, 1397.329407496930116, 216.7606694918979713 ) ) ;
#31576=CARTESIAN_POINT ( 'NONE',  ( -21.06868771289999742, 1409.648795181130026, 214.7337414265580264 ) ) ;
#31578=CARTESIAN_POINT ( 'NONE',  ( -7.075873090581220301E-12, 1395.913060387330006, 220.1216245177919859 ) ) ;
#31581=CARTESIAN_POINT ( 'NONE',  ( 0.7910245917146940808, 1426.918876941764893, 137.0999999980980135 ) ) ;
#31582=CARTESIAN_POINT ( 'NONE',  ( -13.77385084366710011, 1508.394378971780043, 184.0922798201980299 ) ) ;
#31583=CARTESIAN_POINT ( 'NONE',  ( 3.798153425019999752, 1449.235780910159974, 184.2153987367980221 ) ) ;
#31587=CARTESIAN_POINT ( 'NONE',  ( 8.082860218267720498, 1396.195320171349977, 201.5809466256010012 ) ) ;
#31588=CARTESIAN_POINT ( 'NONE',  ( 1.309033247469999717, 1415.245980412430072, 191.0747513254979992 ) ) ;
#31589=CARTESIAN_POINT ( 'NONE',  ( 11.66762902670000024, 1426.112960980830167, 146.5933604607980101 ) ) ;
#31590=CARTESIAN_POINT ( 'NONE',  ( 8.111736945090072481, 1509.196641154956069, 180.9310382456955608 ) ) ;
#31592=CARTESIAN_POINT ( 'NONE',  ( 12.84231544366310018, 1435.935755016759913, 150.8115345589289973 ) ) ;
#31593=CARTESIAN_POINT ( 'NONE',  ( 1.525930004160000131, 1471.299568758030091, 187.8082942405980020 ) ) ;
#31595=EDGE_LOOP ( 'NONE', ( #12315, #102117, #56238, #26889, #101646, #72515, #58033 ) ) ;
#31596=CARTESIAN_POINT ( 'NONE',  ( -18.72409591074379875, 1458.246134293049863, 227.3156199550079748 ) ) ;
#31602=VERTEX_POINT ( 'NONE', #91954 ) ;
#31604=CARTESIAN_POINT ( 'NONE',  ( -1.799807112810000165, 1414.009329215630032, 185.8866739651980140 ) ) ;
#31606=ORIENTED_EDGE ( 'NONE', *, *, #110417, .T. ) ;
#31610=B_SPLINE_CURVE_WITH_KNOTS ( 'NONE', 5,
 ( #21783, #22335, #13946, #65495, #99604, #22887, #45933, #71722, #105839 ),
 .UNSPECIFIED., .F., .F.,
 ( 6, 3, 6 ),
 ( 0.000000000000000000, 0.5000000000000000000, 1.000000000000000000 ),
 .UNSPECIFIED. ) ;
#31612=CARTESIAN_POINT ( 'NONE',  ( -33.74130636077602929, 1422.741317463423002, 269.5146518279480006 ) ) ;
#31614=CARTESIAN_POINT ( 'NONE',  ( -0.2612772523530000335, 1416.851343897030119, 227.4677504995979973 ) ) ;
#31616=CARTESIAN_POINT ( 'NONE',  ( -0.01306239367006429945, 1452.951700076570205, 183.2402720810920016 ) ) ;
#31617=CARTESIAN_POINT ( 'NONE',  ( -33.94015795350929920, 1440.913060389670136, 248.7268766980600105 ) ) ;
#31619=CARTESIAN_POINT ( 'NONE',  ( -0.2432179624465790058, 1465.024700022039951, 237.7670363050069682 ) ) ;
#31622=CARTESIAN_POINT ( 'NONE',  ( 4.986174232479999802, 1408.440924972429912, 270.3887730021980360 ) ) ;
#31624=CARTESIAN_POINT ( 'NONE',  ( 23.98088334710000069, 1410.978996304829934, 208.3903162892720218 ) ) ;
#31630=CARTESIAN_POINT ( 'NONE',  ( 0.09078858057499999967, 1420.445484879229980, 183.3263106172979917 ) ) ;
#31633=ORIENTED_EDGE ( 'NONE', *, *, #34980, .T. ) ;
#31635=ADVANCED_FACE ( 'NONE', ( #93050 ), #15763, .F. ) ;
#31639=CARTESIAN_POINT ( 'NONE',  ( -8.991795041622840046, 1509.227063482730046, 237.0095535837990326 ) ) ;
#31644=DIRECTION ( 'NONE',  ( -0.9993779842017727066, -0.0009463033499147846571, -0.03525264816679202218 ) ) ;
#31649=CARTESIAN_POINT ( 'NONE',  ( 28.32265147467229838, 1509.673549449270013, 207.2611521541350044 ) ) ;
#31650=CARTESIAN_POINT ( 'NONE',  ( 0.3785491535969999766, 1487.217178801030059, 230.2600272812980222 ) ) ;
#31657=CARTESIAN_POINT ( 'NONE',  ( 14.16828006819016395, 1420.021719220239902, 228.3966679742590031 ) ) ;
#31659=CARTESIAN_POINT ( 'NONE',  ( 38.88267750156879998, 1447.890902847689858, 136.5100495134630023 ) ) ;
#31660=CARTESIAN_POINT ( 'NONE',  ( -18.93172946400000356, 1424.841178919430149, 224.3420561942980100 ) ) ;
#31665=CARTESIAN_POINT ( 'NONE',  ( -15.60993031491385707, 1469.237360295198414, 269.3672923534541042 ) ) ;
#31668=CARTESIAN_POINT ( 'NONE',  ( 11.11083760155161748, 1506.426094404281002, 190.1501388411886637 ) ) ;
#31669=EDGE_CURVE ( 'NONE', #17250, #43307, #103375, .T. ) ;
#31671=CARTESIAN_POINT ( 'NONE',  ( -9.202936508599998788, 1519.913060387329779, 230.3262217860979888 ) ) ;
#31673=CARTESIAN_POINT ( 'NONE',  ( -12.99496264364580256, 1442.946651945849453, 186.5341436481298274 ) ) ;
#31676=EDGE_CURVE ( 'NONE', #76166, #86228, #26035, .T. ) ;
#31677=DIRECTION ( 'NONE',  ( 0.000000000000000000, 0.000000000000000000, -1.000000000000000000 ) ) ;
#31679=CARTESIAN_POINT ( 'NONE',  ( -7.105427357599999217E-15, 1405.913060387330006, 137.0999999980979851 ) ) ;
#31680=CARTESIAN_POINT ( 'NONE',  ( -13.06317481566171068, 1442.994605609547762, 169.4117022543989890 ) ) ;
#31683=CARTESIAN_POINT ( 'NONE',  ( 0.2112786387551819911, 1416.230844595159851, 190.9402219459099967 ) ) ;
#31684=CARTESIAN_POINT ( 'NONE',  ( 21.83810631170608474, 1509.467311289125064, 226.7543823560263547 ) ) ;
#31687=CARTESIAN_POINT ( 'NONE',  ( 18.02416168173120070, 1416.221314539589912, 209.0673659498179973 ) ) ;
#31690=CARTESIAN_POINT ( 'NONE',  ( -25.95416491200000308, 1449.827894582669842, 231.7292227871980117 ) ) ;
#31693=CARTESIAN_POINT ( 'NONE',  ( -11.29872328070000087, 1433.512132546310113, 151.5043843572979938 ) ) ;
#31696=CARTESIAN_POINT ( 'NONE',  ( 16.63506016420000222, 1409.493969489730034, 224.1775087685979884 ) ) ;
#31697=CARTESIAN_POINT ( 'NONE',  ( -26.28587293000000003, 1436.455679608809987, 136.7639433163979845 ) ) ;
#31698=CARTESIAN_POINT ( 'NONE',  ( -12.00387303569999986, 1415.296882282229944, 195.7718046162979704 ) ) ;
#31701=CARTESIAN_POINT ( 'NONE',  ( 2.389941574139999858, 1450.533795919260001, 183.3353223396979956 ) ) ;
#31703=CARTESIAN_POINT ( 'NONE',  ( -29.02628104977890189, 1509.926680457060002, 211.9910930732060024 ) ) ;
#31704=CARTESIAN_POINT ( 'NONE',  ( -4.244249385787189894E-10, 1412.540523501239932, 252.0669699321499877 ) ) ;
#31707=CARTESIAN_POINT ( 'NONE',  ( -11.78952479729490044, 1427.771338190059851, 147.6174756818780054 ) ) ;
#31709=CARTESIAN_POINT ( 'NONE',  ( -3.549205704360000269, 1473.795584311630137, 270.2903253923980174 ) ) ;
#31710=CYLINDRICAL_SURFACE ( 'NONE', #10467, 29.99999999999999645 ) ;
#31712=CARTESIAN_POINT ( 'NONE',  ( -13.60685608969999905, 1452.409494112630000, 223.2534408495980074 ) ) ;
#31713=CARTESIAN_POINT ( 'NONE',  ( -7.075873090581220301E-12, 1395.913060387330006, 220.1216245177919859 ) ) ;
#31714=CARTESIAN_POINT ( 'NONE',  ( 18.72022026493218405, 1457.160368941672687, 229.5334714930285713 ) ) ;
#31715=DIRECTION ( 'NONE',  ( -0.04471266514373050532, 0.9989992949979481507, -0.001089114019438660068 ) ) ;
#31718=CARTESIAN_POINT ( 'NONE',  ( -37.07982229246980665, 1420.640666704749947, 269.2047045636169855 ) ) ;
#31719=ORIENTED_EDGE ( 'NONE', *, *, #36631, .F. ) ;
#31721=EDGE_LOOP ( 'NONE', ( #96687, #56856, #40829, #5448 ) ) ;
#31726=CARTESIAN_POINT ( 'NONE',  ( 41.16307904399219808, 1444.157581002339839, 136.7448092931550150 ) ) ;
#31729=CARTESIAN_POINT ( 'NONE',  ( -15.85109824379999921, 1440.436905774210118, 189.7893843040980073 ) ) ;
#31730=CIRCLE ( 'NONE', #53172, 8.500000000000000000 ) ;
#31734=CARTESIAN_POINT ( 'NONE',  ( -26.47025460449999912, 1435.961592063199760, 136.4857856691980089 ) ) ;
#31735=( BOUNDED_CURVE ( )  B_SPLINE_CURVE ( 3, ( #74446, #81699, #98511, #99052 ),
 .UNSPECIFIED., .F., .T. ) 
 B_SPLINE_CURVE_WITH_KNOTS ( ( 4, 4 ),
 ( 1.036306151091926031, 2.105316129261890268 ),
 .UNSPECIFIED. ) 
 CURVE ( )  GEOMETRIC_REPRESENTATION_ITEM ( )  RATIONAL_B_SPLINE_CURVE ( ( 1.000000000000000000, 0.9070139338303890852, 0.9070139338303890852, 1.000000000000000000 ) ) 
 REPRESENTATION_ITEM ( '' )  );
#31737=CARTESIAN_POINT ( 'NONE',  ( -41.65674268029999894, 1443.992461967939789, 135.6790812281979868 ) ) ;
#31739=CARTESIAN_POINT ( 'NONE',  ( -40.40952010682039486, 1425.380211256870098, 269.9834891395850036 ) ) ;
#31741=CARTESIAN_POINT ( 'NONE',  ( -3.851962676559999910, 1397.715880058830180, 196.6003271923979980 ) ) ;
#31744=ORIENTED_EDGE ( 'NONE', *, *, #74348, .F. ) ;
#31745=CARTESIAN_POINT ( 'NONE',  ( -11.86930535227000050, 1432.575968667860025, 149.9818528069360184 ) ) ;
#31749=CARTESIAN_POINT ( 'NONE',  ( -14.53429262354389984, 1436.249209451070101, 149.9090136612170170 ) ) ;
#31750=CARTESIAN_POINT ( 'NONE',  ( -1.202963480870000046, 1486.064486177629988, 181.8233092472979990 ) ) ;
#31751=AXIS2_PLACEMENT_3D ( 'NONE', #10411, #2595, #45702 ) ;
#31756=CARTESIAN_POINT ( 'NONE',  ( -13.36059443979999983, 1414.988015881329829, 220.3623400978979987 ) ) ;
#31759=EDGE_LOOP ( 'NONE', ( #38394, #64573, #89517, #14361, #17251 ) ) ;
#31760=CARTESIAN_POINT ( 'NONE',  ( -36.37832874669039995, 1451.642701154630004, 134.4203408178500183 ) ) ;
#31762=CARTESIAN_POINT ( 'NONE',  ( -20.19776133349999014, 1456.164861684272637, 224.8266744640568504 ) ) ;
#31766=CARTESIAN_POINT ( 'NONE',  ( 12.79711581523170061, 1435.583474523099994, 150.7184249802959926 ) ) ;
#31767=CARTESIAN_POINT ( 'NONE',  ( 13.73564804769999981, 1415.163755998629995, 197.5875405738979964 ) ) ;
#31769=CARTESIAN_POINT ( 'NONE',  ( 11.36018337630000019, 1414.996442546230128, 222.2791104318980047 ) ) ;
#31770=CARTESIAN_POINT ( 'NONE',  ( 2.762616382466477560, 1451.876908917511173, 183.8170818175215970 ) ) ;
#31772=B_SPLINE_CURVE_WITH_KNOTS ( 'NONE', 5,
 ( #52673, #17926, #26910, #34199, #44274, #86251 ),
 .UNSPECIFIED., .F., .F.,
 ( 6, 6 ),
 ( 0.000000000000000000, 1.000000000000000000 ),
 .UNSPECIFIED. ) ;
#31773=CARTESIAN_POINT ( 'NONE',  ( -0.2545641238315171084, 1506.446781340913049, 187.1295352870444901 ) ) ;
#31774=CARTESIAN_POINT ( 'NONE',  ( 24.34257435393226032, 1445.451185733568082, 214.1610445365998032 ) ) ;
#31776=CARTESIAN_POINT ( 'NONE',  ( -11.97724519069999971, 1441.600846913620217, 147.6096801420980000 ) ) ;
#31781=CARTESIAN_POINT ( 'NONE',  ( -15.45910334130000052, 1472.202164814229945, 270.0849031532980007 ) ) ;
#31785=CARTESIAN_POINT ( 'NONE',  ( 30.25602947823919919, 1509.982583641990004, 213.6645168607980168 ) ) ;
#31788=CARTESIAN_POINT ( 'NONE',  ( 17.97140328465984638, 1424.060494694068439, 225.5988178466726595 ) ) ;
#31790=EDGE_CURVE ( 'NONE', #62931, #83528, #66153, .T. ) ;
#31792=CARTESIAN_POINT ( 'NONE',  ( 29.45229671441789776, 1440.913060386809775, 236.5454254465630015 ) ) ;
#31794=CARTESIAN_POINT ( 'NONE',  ( -22.11554775090000291, 1489.452917662329810, 207.6017475386279898 ) ) ;
#31795=CARTESIAN_POINT ( 'NONE',  ( 13.19072720129999965, 1429.093818030529974, 222.3773134601979962 ) ) ;
#31796=ORIENTED_EDGE ( 'NONE', *, *, #80295, .F. ) ;
#31797=ADVANCED_FACE ( 'NONE', ( #16726 ), #95159, .T. ) ;
#31802=CARTESIAN_POINT ( 'NONE',  ( 17.34616664546187081, 1410.519557093256935, 192.4923973019862729 ) ) ;
#31803=CARTESIAN_POINT ( 'NONE',  ( 14.71230246817723142, 1414.913060387329779, 201.6306905010262369 ) ) ;
#31811=AXIS2_PLACEMENT_3D ( 'NONE', #88066, #2422, #95894 ) ;
#31813=CARTESIAN_POINT ( 'NONE',  ( -14.16616822539999987, 1471.309244717429920, 193.0783035305979922 ) ) ;
#31814=CARTESIAN_POINT ( 'NONE',  ( -11.87563350447849864, 1433.006677213540115, 147.6591432354780125 ) ) ;
#31822=EDGE_LOOP ( 'NONE', ( #32576, #62828, #58494, #110730, #76949, #99731, #92612, #21813 ) ) ;
#31832=CARTESIAN_POINT ( 'NONE',  ( 11.91057031607170025, 1409.328986667859908, 200.0892353780850215 ) ) ;
#31833=CARTESIAN_POINT ( 'NONE',  ( -3.899071993169999590E-16, 1420.943991414029824, 172.2701767054979882 ) ) ;
#31837=CARTESIAN_POINT ( 'NONE',  ( -2.500000000000000000, 1439.615672362369878, 170.5246407198980023 ) ) ;
#31838=CARTESIAN_POINT ( 'NONE',  ( -3.724487131215511670, 1424.082886414761788, 184.7380720752485956 ) ) ;
#31840=EDGE_CURVE ( 'NONE', #49915, #25603, #83357, .T. ) ;
#31841=CARTESIAN_POINT ( 'NONE',  ( -2.431412526649999961, 1428.647745098929818, 149.4227846719979880 ) ) ;
#31842=CARTESIAN_POINT ( 'NONE',  ( 18.31156613494090024, 1457.716607816860005, 228.0465888042749896 ) ) ;
#31843=CARTESIAN_POINT ( 'NONE',  ( -12.64307430949999933, 1435.023293913380030, 150.5876313343979973 ) ) ;
#31846=CARTESIAN_POINT ( 'NONE',  ( -25.00976051679999657, 1436.598010167069788, 137.9330532114979917 ) ) ;
#31850=CARTESIAN_POINT ( 'NONE',  ( -45.67170290102849606, 1440.913066807300083, 266.1885079402800329 ) ) ;
#31851=CARTESIAN_POINT ( 'NONE',  ( -23.20318578650891794, 1433.765053652970209, 215.6666533212324168 ) ) ;
#31852=CARTESIAN_POINT ( 'NONE',  ( 13.89991610216109841, 1452.702855433150035, 223.2766279111739891 ) ) ;
#31856=FILL_AREA_STYLE_COLOUR ( '', #28373 ) ;
#31857=CARTESIAN_POINT ( 'NONE',  ( 2.809892388859999812, 1422.122748426330190, 101.6305461396979979 ) ) ;
#31860=CARTESIAN_POINT ( 'NONE',  ( 26.00754374119999923, 1427.792721087130076, 240.2274372948979817 ) ) ;
#31862=CARTESIAN_POINT ( 'NONE',  ( -0.4526181979879999595, 1452.693343343929882, 183.1469136533980020 ) ) ;
#31865=CARTESIAN_POINT ( 'NONE',  ( -23.79286722360000184, 1428.843115172530133, 231.7321643605979773 ) ) ;
#31866=CARTESIAN_POINT ( 'NONE',  ( -29.04414693871334308, 1509.932335316460922, 204.0080394800089039 ) ) ;
#31867=CARTESIAN_POINT ( 'NONE',  ( -8.876970405461879210, 1452.603069750020040, 151.0241627572419816 ) ) ;
#31868=CARTESIAN_POINT ( 'NONE',  ( 27.02655593769999953, 1451.108952154630060, 136.3738421987980018 ) ) ;
#31870=CARTESIAN_POINT ( 'NONE',  ( -2.500000000000000000, 1424.046630307830128, 154.4234530583979961 ) ) ;
#31871=CARTESIAN_POINT ( 'NONE',  ( 6.691728662302649767E-05, 1410.389828169050134, 269.3346513474109543 ) ) ;
#31872=CARTESIAN_POINT ( 'NONE',  ( 15.59164432048419968, 1421.661620995860176, 227.7520908980149841 ) ) ;
#31874=ORIENTED_EDGE ( 'NONE', *, *, #66459, .F. ) ;
#31878=CARTESIAN_POINT ( 'NONE',  ( -23.73958735709999956, 1410.154131308830074, 209.3402010283099912 ) ) ;
#31884=CARTESIAN_POINT ( 'NONE',  ( -2.900078654861840022, 1473.495617646690107, 183.7954459137889955 ) ) ;
#31885=CARTESIAN_POINT ( 'NONE',  ( -21.24403838879999995, 1415.846602379829847, 218.4048111434979944 ) ) ;
#31887=CARTESIAN_POINT ( 'NONE',  ( 45.98765409508450830, 1442.794819212339917, 268.4974154456440374 ) ) ;
#31891=ORIENTED_EDGE ( 'NONE', *, *, #105901, .F. ) ;
#31898=CARTESIAN_POINT ( 'NONE',  ( 26.56840054362369585, 1451.979948467160057, 135.1038962431699986 ) ) ;
#31902=CARTESIAN_POINT ( 'NONE',  ( 21.63150929049999860, 1409.668449337029870, 213.1599398232280009 ) ) ;
#31905=DIRECTION ( 'NONE',  ( 1.000000000000000000, 0.000000000000000000, 0.000000000000000000 ) ) ;
#31906=CARTESIAN_POINT ( 'NONE',  ( -13.80541478530910027, 1434.979604282769969, 148.5370187744020143 ) ) ;
#31907=CARTESIAN_POINT ( 'NONE',  ( -18.22449011683852760, 1423.927591919610677, 225.4533452331210412 ) ) ;
#31912=CARTESIAN_POINT ( 'NONE',  ( 3.268607741949999923, 1425.981674191930097, 219.6133831120980062 ) ) ;
#31914=DIRECTION ( 'NONE',  ( 1.000000000000000000, 5.309750374689999822E-19, 2.343158368729999945E-19 ) ) ;
#31919=CARTESIAN_POINT ( 'NONE',  ( 16.81223226430000039, 1414.913060387329779, 210.6693098017280192 ) ) ;
#31922=CARTESIAN_POINT ( 'NONE',  ( -12.63252536770000134, 1420.772946692730102, 222.2681001552979865 ) ) ;
#31923=EDGE_CURVE ( 'NONE', #67251, #16145, #3990, .T. ) ;
#31924=CARTESIAN_POINT ( 'NONE',  ( 39.47393889809999479, 1455.502555575530096, 271.1218459616979999 ) ) ;
#31925=CARTESIAN_POINT ( 'NONE',  ( 0.9233357834264179775, 1450.850097690670054, 181.4078119359379855 ) ) ;
#31927=CARTESIAN_POINT ( 'NONE',  ( 0.4435022289555869968, 1418.672171135500093, 184.7048927309859891 ) ) ;
#31928=CARTESIAN_POINT ( 'NONE',  ( 11.35225316950000085, 1419.758531043530184, 229.7208292713979745 ) ) ;
#31931=CARTESIAN_POINT ( 'NONE',  ( -18.01164195190000328, 1410.466195698429829, 224.7175291131979975 ) ) ;
#31932=FACE_OUTER_BOUND ( 'NONE', #6071, .T. ) ;
#31933=B_SPLINE_CURVE_WITH_KNOTS ( 'NONE', 5,
 ( #88551, #106983, #81224, #29184, #106442, #48201 ),
 .UNSPECIFIED., .F., .F.,
 ( 6, 6 ),
 ( 0.000000000000000000, 1.000000000000000000 ),
 .UNSPECIFIED. ) ;
#31934=CARTESIAN_POINT ( 'NONE',  ( -25.55912388069999963, 1449.022877353309923, 137.9013602817979915 ) ) ;
#31935=CARTESIAN_POINT ( 'NONE',  ( -17.58999536348959936, 1410.451648346190041, 193.0352298804580187 ) ) ;
#31937=CARTESIAN_POINT ( 'NONE',  ( 1.346199663083729914E-06, 1408.510422093800116, 195.3530119415600268 ) ) ;
#31938=DIRECTION ( 'NONE',  ( -1.000000000000000000, 0.000000000000000000, 0.000000000000000000 ) ) ;
#31940=CARTESIAN_POINT ( 'NONE',  ( -3.560380890149999811, 1415.087974640030097, 226.2956427098980043 ) ) ;
#31941=CARTESIAN_POINT ( 'NONE',  ( 0.1872740515456740029, 1470.279753032280041, 182.5118344780429709 ) ) ;
#31943=ORIENTED_EDGE ( 'NONE', *, *, #19428, .T. ) ;
#31944=CARTESIAN_POINT ( 'NONE',  ( -20.17294526779999941, 1444.994950788469851, 161.5349527656980229 ) ) ;
#31945=ADVANCED_FACE ( 'NONE', ( #76124 ), #71612, .T. ) ;
#31947=CARTESIAN_POINT ( 'NONE',  ( 11.94112614929999872, 1433.615419815239875, 149.4776156485979755 ) ) ;
#31948=CARTESIAN_POINT ( 'NONE',  ( -40.33550002387350020, 1439.280879845010077, 134.0999999981289932 ) ) ;
#31950=ORIENTED_EDGE ( 'NONE', *, *, #99420, .T. ) ;
#31951=B_SPLINE_SURFACE_WITH_KNOTS ( 'NONE', 5, 5, ( 
 ( #109063, #67066, #65970, #93884, #50799, #49159 ),
 ( #25017, #6035, #50267, #23914, #48610, #7141 ),
 ( #16064, #84396, #110145, #109604, #32877, #32347 ),
 ( #76543, #7684, #59218, #33419, #57567, #41296 ),
 ( #40739, #58656, #92791, #93337, #59763, #110695 ),
 ( #49710, #33988, #74369, #82743, #101172, #24467 ),
 ( #74914, #66526, #58109, #92240, #15512, #103380 ),
 ( #102827, #11007, #77655, #1512, #95009, #968 ),
 ( #422, #62550, #96104, #60311, #18276, #104507 ),
 ( #18827, #69275, #17150, #86599, #94430, #95555 ),
 ( #10446, #78199, #44059, #35092, #87157, #19378 ),
 ( #44619, #68724, #26684, #17708, #28354, #35642 ) ),
 .UNSPECIFIED., .F., .F., .F.,
 ( 6, 3, 3, 6 ),
 ( 6, 6 ),
 ( 4.119532581660000581, 6.664003371819999799, 7.493366175190000256, 9.981901822019999315 ),
 ( 0.000000000000000000, 2.000000000000000000 ),
 .UNSPECIFIED. ) ;
#31957=CARTESIAN_POINT ( 'NONE',  ( -46.02997362520000735, 1440.913038198389813, 268.4959101188979957 ) ) ;
#31960=DIRECTION ( 'NONE',  ( 0.000000000000000000, 0.000000000000000000, 1.000000000000000000 ) ) ;
#31962=CARTESIAN_POINT ( 'NONE',  ( 3.910028042040000429, 1431.491579035269979, 185.0507363215979808 ) ) ;
#31965=CARTESIAN_POINT ( 'NONE',  ( -26.79413167943010166, 1436.761919080860025, 136.7821860765010058 ) ) ;
#31966=EDGE_LOOP ( 'NONE', ( #28865, #6070, #84763, #8606 ) ) ;
#31968=CARTESIAN_POINT ( 'NONE',  ( -27.26775404520000023, 1451.960960096730105, 134.9110166487979825 ) ) ;
#31969=CARTESIAN_POINT ( 'NONE',  ( -17.00746236582520154, 1410.591278265990013, 226.2082703236820009 ) ) ;
#31973=AXIS2_PLACEMENT_3D ( 'NONE', #49287, #15095, #74497 ) ;
#31975=EDGE_CURVE ( 'NONE', #75650, #108306, #34416, .T. ) ;
#31976=CARTESIAN_POINT ( 'NONE',  ( 22.97508917209999879, 1509.490924000130008, 224.8302120705980087 ) ) ;
#31978=CARTESIAN_POINT ( 'NONE',  ( -0.1548877673338640015, 1419.548927902510059, 184.3830762897939906 ) ) ;
#31979=CARTESIAN_POINT ( 'NONE',  ( 0.9551731419629999609, 1466.226277197029958, 235.4680291051979850 ) ) ;
#31980=CARTESIAN_POINT ( 'NONE',  ( 17.22539861130000105, 1409.514584562929940, 222.3763154799979986 ) ) ;
#31981=CARTESIAN_POINT ( 'NONE',  ( -2.666035071639449860, 1419.521156420629950, 186.1676433668029915 ) ) ;
#31982=CARTESIAN_POINT ( 'NONE',  ( -17.71700096680000058, 1424.354672622029966, 228.0407626086980031 ) ) ;
#31987=B_SPLINE_CURVE_WITH_KNOTS ( 'NONE', 5,
 ( #11719, #36914, #36362, #53185, #61589, #53760, #97370, #87327, #95174 ),
 .UNSPECIFIED., .F., .F.,
 ( 6, 3, 6 ),
 ( 0.000000000000000000, 0.6021179571096993977, 1.000000000000000000 ),
 .UNSPECIFIED. ) ;
#31991=CARTESIAN_POINT ( 'NONE',  ( -10.49533061896650032, 1485.816092626590034, 184.3926849958960190 ) ) ;
#31992=VERTEX_POINT ( 'NONE', #10579 ) ;
#31993=CARTESIAN_POINT ( 'NONE',  ( 2.890489020090289962, 1507.108937781499890, 235.9439513786750240 ) ) ;
#31994=CARTESIAN_POINT ( 'NONE',  ( -0.9080294960061148224, 1420.737356635930155, 182.9235011294603055 ) ) ;
#32001=CARTESIAN_POINT ( 'NONE',  ( -22.35979953749999893, 1410.906900737730211, 203.0403674361979824 ) ) ;
#32002=CARTESIAN_POINT ( 'NONE',  ( -9.939393947103138061, 1441.236512651819794, 153.4167241843420300 ) ) ;
#32003=CARTESIAN_POINT ( 'NONE',  ( 15.93913202865929968, 1410.714489637869974, 191.5350724760020285 ) ) ;
#32005=CARTESIAN_POINT ( 'NONE',  ( 41.61584690620330207, 1442.586878941469877, 136.0036615449459987 ) ) ;
#32006=CARTESIAN_POINT ( 'NONE',  ( -10.81515773970000005, 1424.921120067930133, 144.1684135307980057 ) ) ;
#32011=CARTESIAN_POINT ( 'NONE',  ( -14.88313348660000024, 1507.431571772529878, 231.7094224802980023 ) ) ;
#32012=ORIENTED_EDGE ( 'NONE', *, *, #68131, .F. ) ;
#32014=CARTESIAN_POINT ( 'NONE',  ( -18.21986176780000122, 1458.468391452929836, 227.9546142145979957 ) ) ;
#32015=ORIENTED_EDGE ( 'NONE', *, *, #40642, .T. ) ;
#32016=ORIENTED_EDGE ( 'NONE', *, *, #69304, .F. ) ;
#32017=CARTESIAN_POINT ( 'NONE',  ( 15.83309290234510414, 1410.837657475366996, 227.0154553047771913 ) ) ;
#32020=CARTESIAN_POINT ( 'NONE',  ( 0.000000000000000000, 1518.913060387330006, 209.1218459616979999 ) ) ;
#32024=VECTOR ( 'NONE', #92314, 1000.000000000000114 ) ;
#32026=CARTESIAN_POINT ( 'NONE',  ( 33.91369120209999721, 1451.728768194229815, 134.0999999980979851 ) ) ;
#32027=CARTESIAN_POINT ( 'NONE',  ( 2.606069733071630257, 1421.343799577720119, 183.3146730432610241 ) ) ;
#32028=FACE_OUTER_BOUND ( 'NONE', #36980, .T. ) ;
#32035=CARTESIAN_POINT ( 'NONE',  ( 37.85189106831440142, 1440.913060387330006, 264.7684821643020427 ) ) ;
#32036=CARTESIAN_POINT ( 'NONE',  ( 18.48154349909999539, 1467.192605361630058, 228.1015105461979999 ) ) ;
#32043=FACE_OUTER_BOUND ( 'NONE', #68972, .T. ) ;
#32045=CARTESIAN_POINT ( 'NONE',  ( -3.611923964340000293, 1508.978187008830218, 180.0004836359980231 ) ) ;
#32046=CARTESIAN_POINT ( 'NONE',  ( -12.06145328200000044, 1433.903212736319801, 146.4342169817980164 ) ) ;
#32047=CARTESIAN_POINT ( 'NONE',  ( 26.49460307026359729, 1499.744025783769985, 206.2293708431749906 ) ) ;
#32048=CARTESIAN_POINT ( 'NONE',  ( 12.60568905610000101, 1462.740100782129957, 231.3171901606980043 ) ) ;
#32049=CARTESIAN_POINT ( 'NONE',  ( -10.57448040964888492, 1423.877913334070627, 137.4727699158958956 ) ) ;
#32050=CARTESIAN_POINT ( 'NONE',  ( -4.603585632142040751, 1422.096080299584173, 184.6430019781807346 ) ) ;
#32052=ORIENTED_EDGE ( 'NONE', *, *, #80306, .T. ) ;
#32053=VECTOR ( 'NONE', #40864, 1000.000000000000227 ) ;
#32054=CARTESIAN_POINT ( 'NONE',  ( -1.098784916811339940, 1486.285180436948394, 181.7858322622153935 ) ) ;
#32055=CARTESIAN_POINT ( 'NONE',  ( -0.03770439129968750080, 1508.815788562569878, 179.7994759633430135 ) ) ;
#32059=CARTESIAN_POINT ( 'NONE',  ( 18.56428471230000099, 1507.623776012629833, 188.5292884487979848 ) ) ;
#32066=CARTESIAN_POINT ( 'NONE',  ( -11.86301030670000145, 1432.114658971819836, 150.3940075513980048 ) ) ;
#32067=CARTESIAN_POINT ( 'NONE',  ( 19.02704169900689735, 1456.915441405320053, 225.6706379604710264 ) ) ;
#32069=CARTESIAN_POINT ( 'NONE',  ( 3.149355032655189568, 1421.363409079380062, 147.6430073452349916 ) ) ;
#32071=CARTESIAN_POINT ( 'NONE',  ( 11.74267738989999899, 1446.506701540040012, 187.7371936343980110 ) ) ;
#32072=CARTESIAN_POINT ( 'NONE',  ( -20.43674167330000202, 1495.372756435230258, 227.5904186109980003 ) ) ;
#32073=CARTESIAN_POINT ( 'NONE',  ( -8.160972540127728436, 1423.396019259317200, 139.1420364792214457 ) ) ;
#32075=CIRCLE ( 'NONE', #94647, 24.94174191160003318 ) ;
#32078=CARTESIAN_POINT ( 'NONE',  ( 6.132762384200000305, 1406.804540994629861, 269.4856206602979682 ) ) ;
#32079=CARTESIAN_POINT ( 'NONE',  ( 0.2331116816730000041, 1408.921200826630184, 186.4825379344979694 ) ) ;
#32080=B_SPLINE_CURVE_WITH_KNOTS ( 'NONE', 3,
 ( #37842, #82600, #108897, #92092, #99928, #23772, #14824, #58508, #108347, #109459, #101574, #15911, #49011, #32188 ),
 .UNSPECIFIED., .F., .F.,
 ( 4, 2, 2, 2, 2, 2, 4 ),
 ( 0.000000000000000000, 0.2500000000000011657, 0.3750000000000017764, 0.5000000000000023315, 0.6250000000000028866, 0.7500000000000035527, 1.000000000000000000 ),
 .UNSPECIFIED. ) ;
#32081=CARTESIAN_POINT ( 'NONE',  ( 22.08950919660000167, 1410.866032929729954, 203.5800407805880070 ) ) ;
#32083=CARTESIAN_POINT ( 'NONE',  ( 23.87292829602066391, 1435.060528072440775, 214.1385913967735917 ) ) ;
#32085=DIRECTION ( 'NONE',  ( -1.000000000000000000, 1.110223024625156540E-13, 0.000000000000000000 ) ) ;
#32086=CARTESIAN_POINT ( 'NONE',  ( 15.80576098240000071, 1459.642315333929901, 231.7528682457979983 ) ) ;
#32089=CARTESIAN_POINT ( 'NONE',  ( -1.835536242490369840, 1450.383119622699951, 182.7750508701979868 ) ) ;
#32091=CARTESIAN_POINT ( 'NONE',  ( 1.976367954473379873, 1450.328871374169921, 155.3359367358600309 ) ) ;
#32094=CARTESIAN_POINT ( 'NONE',  ( -10.37541004874250028, 1409.275377690029927, 198.3562446834129958 ) ) ;
#32095=B_SPLINE_SURFACE_WITH_KNOTS ( 'NONE', 5, 5, ( 
 ( #23058, #82443, #29280, #48303, #81874, #81320, #82986, #80795, #38225 ),
 ( #4634, #29828, #37684, #106539, #4101, #91395, #72408, #56136, #57268 ),
 ( #47194, #48860, #14672, #71889, #89187, #55610, #106004, #98681, #63475 ),
 ( #99768, #72948, #13008, #97594, #38772, #64563, #55060, #12479, #13553 ),
 ( #107084, #89734, #46662, #5741, #64014, #98125, #30373, #21943, #90271 ),
 ( #47739, #73505, #5176, #39332, #39884, #107640, #30923, #65102, #99214 ) ),
 .UNSPECIFIED., .F., .F., .F.,
 ( 6, 6 ),
 ( 6, 3, 6 ),
 ( 39.30566959800000149, 56.26181209559999985 ),
 ( 0.000000000000000000, 1.000000000000000000, 2.000000000000000000 ),
 .UNSPECIFIED. ) ;
#32096=CARTESIAN_POINT ( 'NONE',  ( 19.77969251879999746, 1507.818093401829856, 229.2755605921979907 ) ) ;
#32097=CARTESIAN_POINT ( 'NONE',  ( 2.499999995770000094, 1440.150490393029941, 165.1395456438979750 ) ) ;
#32098=CARTESIAN_POINT ( 'NONE',  ( -6.179141267909999513, 1475.525926640629905, 266.9460417852980072 ) ) ;
#32099=CARTESIAN_POINT ( 'NONE',  ( -4.234073038696310576, 1446.327642199189995, 164.0207583150770176 ) ) ;
#32100=CARTESIAN_POINT ( 'NONE',  ( -20.99468044909999875, 1509.712668440929974, 187.9191382749980050 ) ) ;
#32105=CARTESIAN_POINT ( 'NONE',  ( 12.21876415499199986, 1416.384967872819971, 223.5297635905479865 ) ) ;
#32107=CARTESIAN_POINT ( 'NONE',  ( -24.04648193933079980, 1444.796109374620073, 212.0322675289330050 ) ) ;
#32111=CARTESIAN_POINT ( 'NONE',  ( -15.03580570476699840, 1422.460868293147996, 229.1221787420450084 ) ) ;
#32119=CARTESIAN_POINT ( 'NONE',  ( 11.33800672749999983, 1425.544273751829905, 137.4271120788979772 ) ) ;
#32126=CARTESIAN_POINT ( 'NONE',  ( 10.96966286673369950, 1432.359740019160199, 151.7701370213850112 ) ) ;
#32127=CARTESIAN_POINT ( 'NONE',  ( -11.86359345204703786, 1398.264825172677774, 203.8060210069523350 ) ) ;
#32130=FACE_OUTER_BOUND ( 'NONE', #98541, .T. ) ;
#32131=CARTESIAN_POINT ( 'NONE',  ( 20.57820410168999814, 1507.771244142579917, 228.0150965724730270 ) ) ;
#32135=CARTESIAN_POINT ( 'NONE',  ( 12.00222499182989999, 1433.736528012170083, 150.1432766994780081 ) ) ;
#32136=CARTESIAN_POINT ( 'NONE',  ( -13.13104840879999990, 1397.401700877830081, 207.3834689486880052 ) ) ;
#32137=CARTESIAN_POINT ( 'NONE',  ( -20.09807828239999949, 1410.109999577329745, 220.1458087410979942 ) ) ;
#32139=CARTESIAN_POINT ( 'NONE',  ( -13.45615543559949145, 1444.281848265668714, 169.3621925482611346 ) ) ;
#32142=CARTESIAN_POINT ( 'NONE',  ( -13.70995644358860055, 1507.826637856930120, 184.2436392040419832 ) ) ;
#32143=CARTESIAN_POINT ( 'NONE',  ( 3.809409616780000007, 1468.703253529829908, 183.3440034161980066 ) ) ;
#32146=CARTESIAN_POINT ( 'NONE',  ( 8.906967729100440323, 1396.224098604110168, 202.5685376797749768 ) ) ;
#32147=CARTESIAN_POINT ( 'NONE',  ( 1.549353400650000046, 1416.067629296030191, 190.3885695989980036 ) ) ;
#32148=CARTESIAN_POINT ( 'NONE',  ( 11.18838110630000138, 1425.436776285730048, 146.8505530396979850 ) ) ;
#32149=CARTESIAN_POINT ( 'NONE',  ( 16.68463225901000158, 1442.773887286389936, 162.0935120915889911 ) ) ;
#32151=CARTESIAN_POINT ( 'NONE',  ( 13.27152677196249897, 1435.087436992850144, 149.8492268114800368 ) ) ;
#32153=EDGE_LOOP ( 'NONE', ( #83326, #88193, #10059, #105435, #48482 ) ) ;
#32154=CARTESIAN_POINT ( 'NONE',  ( 13.51610093809999924, 1443.913060387330006, 169.3501091259980171 ) ) ;
#32155=CARTESIAN_POINT ( 'NONE',  ( -6.996308864409999551, 1463.880774057229928, 235.8431045883980062 ) ) ;
#32156=CIRCLE ( 'NONE', #94734, 477.3522486052488034 ) ;
#32160=ORIENTED_EDGE ( 'NONE', *, *, #58849, .T. ) ;
#32162=CARTESIAN_POINT ( 'NONE',  ( 2.500000000000000000, 1448.206572385129903, 168.0224266773309978 ) ) ;
#32165=VERTEX_POINT ( 'NONE', #105191 ) ;
#32167=ORIENTED_EDGE ( 'NONE', *, *, #107501, .F. ) ;
#32170=EDGE_CURVE ( 'NONE', #38319, #69349, #64768, .T. ) ;
#32171=CARTESIAN_POINT ( 'NONE',  ( -35.06679765450265052, 1424.124224229928814, 269.5324321545449493 ) ) ;
#32172=EDGE_CURVE ( 'NONE', #4923, #45986, #71952, .T. ) ;
#32174=CARTESIAN_POINT ( 'NONE',  ( -1.674829163958580169, 1414.913060387399810, 226.0541986821700107 ) ) ;
#32176=CARTESIAN_POINT ( 'NONE',  ( -9.822264486677861081E-06, 1450.913060148159957, 181.2410907034809782 ) ) ;
#32177=CARTESIAN_POINT ( 'NONE',  ( -31.17697957079580107, 1440.913060388259964, 241.8836480397630169 ) ) ;
#32181=CARTESIAN_POINT ( 'NONE',  ( 6.501109236959999649, 1407.992916451829842, 270.1283629016979830 ) ) ;
#32183=CARTESIAN_POINT ( 'NONE',  ( 23.57777505329999812, 1409.993680146930046, 209.2866710572280056 ) ) ;
#32184=CARTESIAN_POINT ( 'NONE',  ( -20.87372870449999951, 1509.581281395429869, 188.4712523506979949 ) ) ;
#32188=CARTESIAN_POINT ( 'NONE',  ( -2.500574544111449971, 1448.942056179399970, 154.5733147259969940 ) ) ;
#32189=CARTESIAN_POINT ( 'NONE',  ( 0.4756500442839999843, 1418.694808079630093, 184.7107058538980198 ) ) ;
#32190=CARTESIAN_POINT ( 'NONE',  ( 3.515215440921866552, 1419.856978125559863, 137.0999999980978430 ) ) ;
#32192=ORIENTED_EDGE ( 'NONE', *, *, #96276, .T. ) ;
#32195=B_SPLINE_SURFACE_WITH_KNOTS ( 'NONE', 5, 5, ( 
 ( #38447, #31697, #40102, #5401, #81010, #98356 ),
 ( #82103, #21628, #14887, #57485, #98902, #6502 ),
 ( #74284, #108414, #40656, #74828, #4843, #65880 ),
 ( #14337, #73734, #107857, #55834, #81542, #56921 ),
 ( #100001, #23289, #89413, #31146, #91051, #89955 ),
 ( #48526, #107311, #91610, #49078, #55283, #13229 ) ),
 .UNSPECIFIED., .F., .F., .F.,
 ( 6, 6 ),
 ( 6, 6 ),
 ( 5.133465978379999406, 14.11476443669999981 ),
 ( 0.000000000000000000, 2.000000000000000000 ),
 .UNSPECIFIED. ) ;
#32196=CARTESIAN_POINT ( 'NONE',  ( 17.60616633871843106, 1410.892144412839798, 225.1414472891892729 ) ) ;
#32198=EDGE_CURVE ( 'NONE', #39621, #83528, #33982, .T. ) ;
#32200=CARTESIAN_POINT ( 'NONE',  ( -6.733539913119999554, 1418.366792801529982, 233.9669031324980040 ) ) ;
#32202=CARTESIAN_POINT ( 'NONE',  ( -24.03284404440000088, 1444.467324254849927, 212.3598065616679946 ) ) ;
#32204=B_SPLINE_CURVE_WITH_KNOTS ( 'NONE', 5,
 ( #95967, #54551, #62399, #97081, #63508, #68169 ),
 .UNSPECIFIED., .F., .F.,
 ( 6, 6 ),
 ( 0.000000000000000000, 1.000000000000000000 ),
 .UNSPECIFIED. ) ;
#32207=PLANE ( 'NONE',  #22746 ) ;
#32209=ORIENTED_EDGE ( 'NONE', *, *, #99232, .T. ) ;
#32212=CIRCLE ( 'NONE', #7198, 28.99999999999999645 ) ;
#32213=CARTESIAN_POINT ( 'NONE',  ( 14.46822985410000051, 1463.223607397130081, 223.0618228778980097 ) ) ;
#32214=CARTESIAN_POINT ( 'NONE',  ( 19.24972504899999848, 1455.799292141330170, 225.3448411794979904 ) ) ;
#32218=DIRECTION ( 'NONE',  ( 0.03489949670250328678, -0.9993908270190956511, 0.000000000000000000 ) ) ;
#32219=CARTESIAN_POINT ( 'NONE',  ( 40.25496866969060505, 1444.330520920399977, 137.0766690124500258 ) ) ;
#32220=CARTESIAN_POINT ( 'NONE',  ( -20.26396079519999915, 1427.262199077629930, 222.0222826655979702 ) ) ;
#32224=CARTESIAN_POINT ( 'NONE',  ( -16.93636994520000272, 1413.292055451130182, 226.4943808309979829 ) ) ;
#32225=B_SPLINE_CURVE_WITH_KNOTS ( 'NONE', 5,
 ( #97474, #105327, #62822, #20203, #54402, #88534, #105889, #3439, #29168 ),
 .UNSPECIFIED., .F., .F.,
 ( 6, 3, 6 ),
 ( 0.000000000000000000, 0.5000000000000000000, 1.000000000000000000 ),
 .UNSPECIFIED. ) ;
#32227=CARTESIAN_POINT ( 'NONE',  ( -24.21249802766532255, 1465.849153120822621, 269.4183097923577179 ) ) ;
#32228=ORIENTED_EDGE ( 'NONE', *, *, #43333, .F. ) ;
#32229=CARTESIAN_POINT ( 'NONE',  ( 1.628202555219999903, 1430.465083930730088, 150.2970716576980124 ) ) ;
#32230=CARTESIAN_POINT ( 'NONE',  ( -42.57897977376345011, 1428.602532329936821, 269.0600478115077294 ) ) ;
#32231=CARTESIAN_POINT ( 'NONE',  ( 3.439855069772169809E-11, 1452.913060387330006, 150.8032249182200246 ) ) ;
#32233=CIRCLE ( 'NONE', #64467, 29.84605316859531143 ) ;
#32234=CARTESIAN_POINT ( 'NONE',  ( -0.1142305270560000086, 1416.107866688329977, 233.5491553016980220 ) ) ;
#32235=CARTESIAN_POINT ( 'NONE',  ( -13.33531041039106668, 1443.287836672654976, 186.9550018447848743 ) ) ;
#32236=B_SPLINE_SURFACE_WITH_KNOTS ( 'NONE', 5, 5, ( 
 ( #4736, #97153, #12043, #38334, #96608, #79263 ),
 ( #70889, #72514, #88760, #107202, #106105, #13118 ),
 ( #37251, #47301, #38879, #63047, #30490, #46226 ),
 ( #96045, #87660, #19316, #2573, #36695, #37803 ),
 ( #105004, #28292, #54084, #55175, #88209, #11503 ),
 ( #63583, #89301, #73624, #57924, #107754, #58468 ) ),
 .UNSPECIFIED., .F., .F., .F.,
 ( 6, 6 ),
 ( 6, 6 ),
 ( 6.379889989409999629, 6.971779114740000338 ),
 ( 0.000000000000000000, 1.455840041380000116 ),
 .UNSPECIFIED. ) ;
#32240=CARTESIAN_POINT ( 'NONE',  ( -37.79051013476979648, 1445.035584066110005, 137.0421779799580122 ) ) ;
#32241=CARTESIAN_POINT ( 'NONE',  ( 23.61230407060000047, 1435.322065071379939, 137.2857908826979951 ) ) ;
#32242=CARTESIAN_POINT ( 'NONE',  ( -13.14246787946174422, 1443.061742832075879, 169.3995334515947491 ) ) ;
#32243=CARTESIAN_POINT ( 'NONE',  ( -14.66467552210000136, 1409.425162140929842, 225.2836404500980052 ) ) ;
#32246=CARTESIAN_POINT ( 'NONE',  ( 0.6362176846909819439, 1414.913060387399810, 192.9136500303789887 ) ) ;
#32247=CARTESIAN_POINT ( 'NONE',  ( 21.95659374958953691, 1509.539900942172380, 226.8505570154440534 ) ) ;
#32249=EDGE_LOOP ( 'NONE', ( #37422, #25394, #23950, #39271, #88684, #7719, #54305, #16826, #64403 ) ) ;
#32250=CARTESIAN_POINT ( 'NONE',  ( 16.70118312301820040, 1414.971390223319986, 209.2094541707220117 ) ) ;
#32252=CARTESIAN_POINT ( 'NONE',  ( -11.68426330212614417, 1428.980873612041023, 140.1562216286908154 ) ) ;
#32253=CARTESIAN_POINT ( 'NONE',  ( -19.28618930569999890, 1452.501336721830057, 211.9649570637480167 ) ) ;
#32255=CARTESIAN_POINT ( 'NONE',  ( -11.03393269049999859, 1433.573953115969971, 151.7352805125980240 ) ) ;
#32258=EDGE_CURVE ( 'NONE', #67278, #43673, #78022, .T. ) ;
#32259=CARTESIAN_POINT ( 'NONE',  ( 13.58235846979999906, 1416.828040475229955, 196.3349388281980055 ) ) ;
#32260=CARTESIAN_POINT ( 'NONE',  ( -11.80119706069999985, 1415.163755984130148, 195.8322853899979918 ) ) ;
#32264=CARTESIAN_POINT ( 'NONE',  ( -14.43289921072090110, 1509.539432542180066, 182.8218189571549885 ) ) ;
#32265=CARTESIAN_POINT ( 'NONE',  ( -1.875238357586299756E-09, 1416.153069931509890, 240.2634071211490152 ) ) ;
#32268=CARTESIAN_POINT ( 'NONE',  ( -11.81434188762340121, 1428.975514852789956, 148.8502864864200035 ) ) ;
#32270=CARTESIAN_POINT ( 'NONE',  ( -4.801572058700000589, 1471.236463740830231, 269.3376025177980182 ) ) ;
#32275=CARTESIAN_POINT ( 'NONE',  ( -13.97867491850210087, 1429.402194067919709, 222.2970902837259928 ) ) ;
#32277=B_SPLINE_SURFACE_WITH_KNOTS ( 'NONE', 5, 5, ( 
 ( #37810, #73631, #30497, #13669, #64686, #90391, #40004, #13125, #108313 ),
 ( #106112, #82571, #56815, #47309, #80914, #98804, #47858, #72520, #90953 ),
 ( #14239, #63590, #48429, #65775, #20429, #88767, #20979, #55183, #4210 ),
 ( #12605, #23190, #84208, #15876, #24293, #33801, #51171, #6409, #109430 ),
 ( #15335, #92062, #83115, #6949, #33251, #240, #41666, #75284, #16972 ),
 ( #101540, #92602, #110519, #74728, #66343, #108862, #76369, #75823, #7504 ),
 ( #100997, #57390, #48982, #57930, #24829, #100459, #50078, #109974, #8050 ),
 ( #14796, #58475, #67995, #102107, #32707, #85299, #59034, #32155, #23742 ),
 ( #93158, #49530, #83655, #67441, #50620, #8598, #91516, #16428, #41106 ),
 ( #40555, #25386, #42770, #66888, #84753, #42218, #59579, #93692, #76931 ),
 ( #34368, #99892, #10261, #43877, #96484, #44438, #70224, #61266, #79147 ),
 ( #17530, #34913, #60137, #78581, #3004, #27082, #1897, #18100, #11386 ),
 ( #95382, #78020, #51733, #783, #85868, #35468, #69098, #45558, #2458 ),
 ( #36034, #103199, #104328, #19764, #94256, #18646, #53966, #27622, #61808 ),
 ( #88099, #102641, #95930, #77483, #79698, #9170, #19190, #43335, #70772 ) ),
 .UNSPECIFIED., .F., .F., .F.,
 ( 6, 3, 3, 3, 6 ),
 ( 6, 3, 6 ),
 ( 76.61796729980000009, 89.38050170190000188, 98.82656461499999523, 108.2726275280000010, 112.1339374929999906 ),
 ( 0.000000000000000000, 1.000000000000000000, 2.000000000000000000 ),
 .UNSPECIFIED. ) ;
#32278=CARTESIAN_POINT ( 'NONE',  ( -24.08426305480000451, 1411.115211393229856, 208.6111285346999864 ) ) ;
#32279=LINE ( 'NONE', #12724, #28960 ) ;
#32281=CARTESIAN_POINT ( 'NONE',  ( -37.60268983529039843, 1420.124584829160085, 267.2573160899880236 ) ) ;
#32287=CARTESIAN_POINT ( 'NONE',  ( 38.71370889343818078, 1444.324653571829003, 136.9324510732293732 ) ) ;
#32292=CARTESIAN_POINT ( 'NONE',  ( -14.71271264950000024, 1455.450119958330106, 188.4035724979979989 ) ) ;
#32295=CARTESIAN_POINT ( 'NONE',  ( -26.56630858009999940, 1435.444835103639889, 135.5553490494979769 ) ) ;
#32304=CARTESIAN_POINT ( 'NONE',  ( 45.97228714287020068, 1578.884309444509881, 188.3086953514500124 ) ) ;
#32305=CARTESIAN_POINT ( 'NONE',  ( 0.04898334450229999831, 1396.985963204730069, 196.3070572679980046 ) ) ;
#32306=CARTESIAN_POINT ( 'NONE',  ( 0.000000000000000000, 1502.413060387330006, 209.1218459616979999 ) ) ;
#32307=EDGE_LOOP ( 'NONE', ( #16789, #9686, #24084, #84049 ) ) ;
#32308=ORIENTED_EDGE ( 'NONE', *, *, #94079, .F. ) ;
#32309=CARTESIAN_POINT ( 'NONE',  ( 0.2178156354970000319, 1452.982786352329867, 183.2541304307979999 ) ) ;
#32311=EDGE_CURVE ( 'NONE', #25245, #14800, #94420, .T. ) ;
#32313=CARTESIAN_POINT ( 'NONE',  ( -23.85691843449999894, 1435.349182908609919, 137.3960071424980072 ) ) ;
#32314=CARTESIAN_POINT ( 'NONE',  ( -24.67190123920000033, 1441.699982178919981, 210.7126285418079874 ) ) ;
#32317=CARTESIAN_POINT ( 'NONE',  ( -0.1681681984989999989, 1416.866694505930127, 168.0175527136979667 ) ) ;
#32320=CARTESIAN_POINT ( 'NONE',  ( -13.17906415938499975, 1414.913527275050001, 220.1406906569499995 ) ) ;
#32321=B_SPLINE_CURVE_WITH_KNOTS ( 'NONE', 3,
 ( #30444, #12000, #97657, #37758, #29886, #54040, #96000, #71950, #19270, #53473, #87617, #10905, #45078, #46182, #80311, #104957, #72471, #3627, #62437, #28247, #96563, #21469, #12549, #46728, #2528, #63541, #106062, #19835, #70848, #80861, #4162, #38289, #88169, #55679, #64078, #11457, #45633, #79773, #22010 ),
 .UNSPECIFIED., .F., .F.,
 ( 4, 2, 2, 1, 1, 2, 2, 2, 2, 1, 1, 2, 2, 2, 2, 2, 1, 1, 1, 2, 2, 2, 4 ),
 ( 0.000000000000000000, 0.06250000000013596069, 0.09375000000020394797, 0.1093750000002379347, 0.1171875000002547407, 0.1210937500002617073, 0.1250000000002686462, 0.1875000000003115841, 0.2187500000003269607, 0.2343750000003285150, 0.2421875000003315404, 0.2460937500003291256, 0.2500000000003266831, 0.3750000000005528356, 0.4375000000006535328, 0.4687500000006948331, 0.4843750000007214784, 0.4921875000007256973, 0.4960937500007246426, 0.4980468750007239764, 0.5000000000007233103, 0.7500000000003617107, 1.000000000000000000 ),
 .UNSPECIFIED. ) ;
#32329=CARTESIAN_POINT ( 'NONE',  ( -8.178500771994089646, 1441.152429774469965, 153.9860759686779943 ) ) ;
#32331=CARTESIAN_POINT ( 'NONE',  ( 13.04561791671889992, 1435.047968860360015, 150.0615661932069997 ) ) ;
#32332=CARTESIAN_POINT ( 'NONE',  ( 14.00211218169999938, 1416.535385209229844, 196.4050012923980262 ) ) ;
#32335=CARTESIAN_POINT ( 'NONE',  ( -11.32634609552117411, 1425.525426998061675, 138.7434885827603637 ) ) ;
#32336=CARTESIAN_POINT ( 'NONE',  ( 2.817354810100396456, 1451.820641374121124, 183.8336154107607854 ) ) ;
#32338=EDGE_CURVE ( 'NONE', #64407, #71213, #90274, .T. ) ;
#32339=CARTESIAN_POINT ( 'NONE',  ( 2.393268998928310687, 1426.806556743500096, 139.9374969045731518 ) ) ;
#32340=CARTESIAN_POINT ( 'NONE',  ( 24.66473933617894687, 1441.732816492871962, 212.5822908973776180 ) ) ;
#32344=CARTESIAN_POINT ( 'NONE',  ( -12.70951029399999932, 1416.237488680629895, 195.9645815363980148 ) ) ;
#32346=EDGE_CURVE ( 'NONE', #90692, #94444, #96660, .T. ) ;
#32347=CARTESIAN_POINT ( 'NONE',  ( 1.166167165090000069, 1418.953384179930026, 184.8577940441979877 ) ) ;
#32352=CARTESIAN_POINT ( 'NONE',  ( 18.58720762869999987, 1416.311719779230089, 209.7162280979700029 ) ) ;
#32354=CARTESIAN_POINT ( 'NONE',  ( -6.278986562220500571E-07, 1407.561930675709846, 222.2258005058740196 ) ) ;
#32357=CARTESIAN_POINT ( 'NONE',  ( 26.35471571933159751, 1507.985750330240080, 216.6976075425179999 ) ) ;
#32362=CARTESIAN_POINT ( 'NONE',  ( -8.861637179848576906, 1506.578945819425144, 229.3724288155509043 ) ) ;
#32366=AXIS2_PLACEMENT_3D ( 'NONE', #6019, #109047, #15497 ) ;
#32367=EDGE_CURVE ( 'NONE', #27144, #38088, #28643, .T. ) ;
#32372=CARTESIAN_POINT ( 'NONE',  ( -14.31281836590000012, 1471.309462467430194, 193.2293590363979945 ) ) ;
#32381=ORIENTED_EDGE ( 'NONE', *, *, #46825, .T. ) ;
#32383=CARTESIAN_POINT ( 'NONE',  ( 1.546943247107299912, 1416.828039266790029, 190.2227890105679933 ) ) ;
#32384=CARTESIAN_POINT ( 'NONE',  ( 35.37723571902410669, 1437.232678306320167, 136.5359279969920010 ) ) ;
#32386=DIRECTION ( 'NONE',  ( -0.8383970168982891602, -0.5450600352768949497, 0.000000000000000000 ) ) ;
#32393=CARTESIAN_POINT ( 'NONE',  ( 7.656439366225840537, 1409.180429141550121, 196.2649065922109912 ) ) ;
#32394=CARTESIAN_POINT ( 'NONE',  ( 18.12088407619999941, 1425.009777113730024, 225.3844322571980001 ) ) ;
#32397=CARTESIAN_POINT ( 'NONE',  ( -2.500000000000000000, 1439.577074560980009, 165.1593652794979903 ) ) ;
#32398=CARTESIAN_POINT ( 'NONE',  ( -21.05488988819999818, 1452.177807430829944, 142.3440031108980008 ) ) ;
#32399=EDGE_LOOP ( 'NONE', ( #102778, #48958, #83221, #23841 ) ) ;
#32403=CARTESIAN_POINT ( 'NONE',  ( -12.89608628189999884, 1434.724840674140069, 149.2206162816979997 ) ) ;
#32405=EDGE_CURVE ( 'NONE', #56464, #65089, #60798, .T. ) ;
#32406=CARTESIAN_POINT ( 'NONE',  ( -4.921730754668429691E-10, 1470.815717837130023, 256.1342986906989836 ) ) ;
#32414=CARTESIAN_POINT ( 'NONE',  ( 13.54178722023820036, 1508.727572038920016, 233.5140146356369826 ) ) ;
#32419=CARTESIAN_POINT ( 'NONE',  ( 3.862639946661079904, 1407.379789369289938, 221.6375632500230211 ) ) ;
#32423=ORIENTED_EDGE ( 'NONE', *, *, #9653, .F. ) ;
#32424=CARTESIAN_POINT ( 'NONE',  ( 26.44959072580000026, 1437.431546973660033, 225.6828644691980230 ) ) ;
#32425=CARTESIAN_POINT ( 'NONE',  ( -3.530374461310000100, 1489.044399826630070, 181.7468199677979896 ) ) ;
#32427=ADVANCED_FACE ( 'NONE', ( #38930 ), #56309, .T. ) ;
#32428=CARTESIAN_POINT ( 'NONE',  ( -2.781364391544570047, 1419.521710623789886, 186.1806238305539978 ) ) ;
#32429=CARTESIAN_POINT ( 'NONE',  ( -10.70017680549999994, 1423.864995475129945, 211.7704828164379762 ) ) ;
#32432=CARTESIAN_POINT ( 'NONE',  ( -3.469412232211699809, 1452.791905842489996, 152.3220070113180213 ) ) ;
#32433=B_SPLINE_CURVE_WITH_KNOTS ( 'NONE', 5,
 ( #7374, #41538, #75152, #23054, #91928, #57804, #90266, #30369, #14668 ),
 .UNSPECIFIED., .F., .F.,
 ( 6, 3, 6 ),
 ( 0.000000000000000000, 0.5000000000000000000, 1.000000000000000000 ),
 .UNSPECIFIED. ) ;
#32434=CARTESIAN_POINT ( 'NONE',  ( -18.79707643829999952, 1416.837309283529976, 208.4087471548650115 ) ) ;
#32435=EDGE_LOOP ( 'NONE', ( #107917, #106221, #91154, #44519 ) ) ;
#32436=CARTESIAN_POINT ( 'NONE',  ( -5.360342550372870107, 1422.242822755830048, 144.1527768786770025 ) ) ;
#32437=CARTESIAN_POINT ( 'NONE',  ( 5.764621990845120029E-05, 1409.781064299669879, 270.0713832058750086 ) ) ;
#32438=CARTESIAN_POINT ( 'NONE',  ( 16.28387335898309729, 1423.071578876830017, 229.4312782304039899 ) ) ;
#32443=CARTESIAN_POINT ( 'NONE',  ( -22.71969927661109878, 1409.706431297170184, 209.0865112504420154 ) ) ;
#32446=CARTESIAN_POINT ( 'NONE',  ( -11.60015079993175036, 1437.619279042158723, 151.8496192710196340 ) ) ;
#32447=CARTESIAN_POINT ( 'NONE',  ( 0.000000000000000000, 1508.913060387330006, 209.1218459616979999 ) ) ;
#32449=CARTESIAN_POINT ( 'NONE',  ( -3.191653983950000217, 1507.639293120730144, 236.7936837086979835 ) ) ;
#32450=CARTESIAN_POINT ( 'NONE',  ( -22.33198887150000189, 1410.866712961029862, 213.4112846406879953 ) ) ;
#32451=ORIENTED_EDGE ( 'NONE', *, *, #105777, .F. ) ;
#32452=CARTESIAN_POINT ( 'NONE',  ( 41.83092555681560043, 1455.428899374940102, 266.5381060907129722 ) ) ;
#32453=CARTESIAN_POINT ( 'NONE',  ( -0.6346444654042239231, 1424.181128449899916, 228.1611430178420221 ) ) ;
#32454=CARTESIAN_POINT ( 'NONE',  ( -0.3212355716730000421, 1418.619114157530021, 184.6997714626980098 ) ) ;
#32457=ORIENTED_EDGE ( 'NONE', *, *, #44853, .T. ) ;
#32458=CARTESIAN_POINT ( 'NONE',  ( 18.96133265953471181, 1457.509259180501431, 226.7471396993940687 ) ) ;
#32462=CARTESIAN_POINT ( 'NONE',  ( 2.500000000000000000, 1448.552414630679777, 182.3688072228979991 ) ) ;
#32463=CARTESIAN_POINT ( 'NONE',  ( 26.91229608229999926, 1451.721307008429903, 135.7917609875980247 ) ) ;
#32465=CARTESIAN_POINT ( 'NONE',  ( 9.120907800999310311, 1452.594551268460009, 150.9409900070750155 ) ) ;
#32470=CARTESIAN_POINT ( 'NONE',  ( 1.806552148200949892, 1408.976146578469979, 186.8750707912049904 ) ) ;
#32471=CARTESIAN_POINT ( 'NONE',  ( -13.39822223261879941, 1434.924425846410031, 148.8729776175770212 ) ) ;
#32476=EDGE_CURVE ( 'NONE', #69390, #64966, #40600, .T. ) ;
#32481=CARTESIAN_POINT ( 'NONE',  ( -0.1681681984989999989, 1432.413060387330006, 146.1721969590979882 ) ) ;
#32487=FACE_OUTER_BOUND ( 'NONE', #23893, .T. ) ;
#32491=CARTESIAN_POINT ( 'NONE',  ( 13.15726442299999910, 1416.543503932829935, 196.3435872999980063 ) ) ;
#32492=CARTESIAN_POINT ( 'NONE',  ( 0.6916575409457245138, 1467.050682359807524, 235.5170429814173474 ) ) ;
#32497=CARTESIAN_POINT ( 'NONE',  ( 18.50064172359999759, 1416.067629290630066, 209.7633006632509876 ) ) ;
#32498=CIRCLE ( 'NONE', #50416, 2.000000000000000000 ) ;
#32503=CARTESIAN_POINT ( 'NONE',  ( -17.59271046137119754, 1410.455526649410103, 193.4350316739960078 ) ) ;
#32507=CARTESIAN_POINT ( 'NONE',  ( -7.646910556199999931, 1414.913060387329779, 223.7159594430980007 ) ) ;
#32508=CARTESIAN_POINT ( 'NONE',  ( 0.2051560345590330015, 1460.078046002440033, 182.9497274072810171 ) ) ;
#32509=CARTESIAN_POINT ( 'NONE',  ( -5.636364295891119980, 1407.760601417009866, 221.4271416552059861 ) ) ;
#32510=EDGE_LOOP ( 'NONE', ( #67730, #90368, #96241, #99430 ) ) ;
#32511=CARTESIAN_POINT ( 'NONE',  ( -17.22592482065197927, 1443.913060387330233, 162.9227486220069920 ) ) ;
#32514=CARTESIAN_POINT ( 'NONE',  ( -41.14836836638649942, 1446.538313981779993, 134.0999999985649822 ) ) ;
#32518=CARTESIAN_POINT ( 'NONE',  ( -11.99447448239999936, 1410.787978745530154, 198.2808973881980137 ) ) ;
#32522=CARTESIAN_POINT ( 'NONE',  ( 40.82574024660451784, 1425.625456410858988, 269.1071013978336168 ) ) ;
#32530=CARTESIAN_POINT ( 'NONE',  ( -29.29916080650000154, 1450.601733552070073, 136.3811420100980172 ) ) ;
#32531=CARTESIAN_POINT ( 'NONE',  ( -15.92198785269019901, 1410.714326797879949, 226.7129421669140186 ) ) ;
#32532=CARTESIAN_POINT ( 'NONE',  ( 3.947090874974254149, 1427.113278099589934, 134.0999999980980704 ) ) ;
#32536=CARTESIAN_POINT ( 'NONE',  ( -18.24877744519994138, 1410.913188608474002, 224.3502044276641527 ) ) ;
#32540=CARTESIAN_POINT ( 'NONE',  ( 20.29357770150000206, 1410.117248657430082, 219.1572836432980012 ) ) ;
#32541=CARTESIAN_POINT ( 'NONE',  ( -22.52609270576707701, 1509.699688878261213, 190.3721629464874638 ) ) ;
#32542=CARTESIAN_POINT ( 'NONE',  ( -17.44047523940000133, 1423.641482825129970, 226.7779220472980057 ) ) ;
#32550=CARTESIAN_POINT ( 'NONE',  ( 2.499999987259999834, 1447.625363422479950, 167.4763715502979835 ) ) ;
#32553=CARTESIAN_POINT ( 'NONE',  ( -4.224734712525329172, 1441.578183378099993, 166.5712083107650017 ) ) ;
#32560=CARTESIAN_POINT ( 'NONE',  ( -20.59678673803600546, 1507.763197061015035, 190.3721465278125606 ) ) ;
#32561=CARTESIAN_POINT ( 'NONE',  ( 15.97496008288169733, 1409.470830777089986, 192.9108099150550117 ) ) ;
#32563=CARTESIAN_POINT ( 'NONE',  ( 40.57510725528580053, 1442.092273678310221, 136.9264308840439810 ) ) ;
#32566=CARTESIAN_POINT ( 'NONE',  ( -11.63661014589999887, 1425.864895317229866, 144.1626081073980004 ) ) ;
#32568=CARTESIAN_POINT ( 'NONE',  ( 15.40019697367809570, 1461.678762082152616, 229.7684540114784966 ) ) ;
#32569=EDGE_CURVE ( 'NONE', #66425, #94251, #19083, .T. ) ;
#32570=CARTESIAN_POINT ( 'NONE',  ( 14.45783227242900004, 1416.839692127189892, 196.8516148535319985 ) ) ;
#32571=CARTESIAN_POINT ( 'NONE',  ( -7.075873090581220301E-12, 1395.913060387330006, 220.1216245177919859 ) ) ;
#32576=ORIENTED_EDGE ( 'NONE', *, *, #82224, .T. ) ;
#32577=CARTESIAN_POINT ( 'NONE',  ( -29.76861393075075668, 1509.997849702723215, 209.5183840890453837 ) ) ;
#32579=CARTESIAN_POINT ( 'NONE',  ( 0.1923572142570000032, 1452.340214348429754, 183.2784190975980039 ) ) ;
#32581=CARTESIAN_POINT ( 'NONE',  ( -19.06723915664710134, 1485.490521620860136, 189.6150037022410118 ) ) ;
#32585=EDGE_CURVE ( 'NONE', #57683, #52165, #33766, .T. ) ;
#32586=CARTESIAN_POINT ( 'NONE',  ( 42.60628464680300453, 1443.705283352369861, 135.6938352391079832 ) ) ;
#32587=CARTESIAN_POINT ( 'NONE',  ( 2.598899143124699940, 1421.341238652740003, 183.3127735487479981 ) ) ;
#32595=CARTESIAN_POINT ( 'NONE',  ( 11.27186228809999946, 1414.983771850430003, 222.4323528540979851 ) ) ;
#32598=CARTESIAN_POINT ( 'NONE',  ( -13.40958059889999987, 1414.996444526030018, 220.3303867755979866 ) ) ;
#32602=CARTESIAN_POINT ( 'NONE',  ( -13.44341642900000089, 1426.042751063429932, 222.1933743934980043 ) ) ;
#32606=CARTESIAN_POINT ( 'NONE',  ( -15.52964665090000018, 1451.324133669029834, 222.4830580725980269 ) ) ;
#32607=CARTESIAN_POINT ( 'NONE',  ( 12.47197601159999891, 1461.938359065629811, 231.9335636622980132 ) ) ;
#32608=CARTESIAN_POINT ( 'NONE',  ( -1.729960644012338955, 1451.871857846600051, 184.1618444272322108 ) ) ;
#32609=CARTESIAN_POINT ( 'NONE',  ( -4.550835815579397092, 1422.060929357180612, 184.6135640397586712 ) ) ;
#32619=CARTESIAN_POINT ( 'NONE',  ( -11.60004869885203682, 1426.175846117266929, 138.0317712997469073 ) ) ;
#32623=CARTESIAN_POINT ( 'NONE',  ( -15.41004399704489991, 1507.593738162499903, 192.1064836414840045 ) ) ;
#32624=CARTESIAN_POINT ( 'NONE',  ( -11.75996506569999944, 1431.602545802069926, 150.7723106216979829 ) ) ;
#32626=CARTESIAN_POINT ( 'NONE',  ( 27.01381218759999925, 1450.681579806120226, 136.4483250053980044 ) ) ;
#32629=CARTESIAN_POINT ( 'NONE',  ( -21.13276769859999860, 1482.727891398330030, 225.4958365253980048 ) ) ;
#32630=CARTESIAN_POINT ( 'NONE',  ( -3.194520716545333094, 1421.833028466792484, 139.1411856592992820 ) ) ;
#32632=ORIENTED_EDGE ( 'NONE', *, *, #13224, .F. ) ;
#32634=CARTESIAN_POINT ( 'NONE',  ( 9.813457517070000691, 1407.253461234630095, 269.4661102456980188 ) ) ;
#32636=CARTESIAN_POINT ( 'NONE',  ( 18.81101837559999979, 1410.875859629429897, 194.9135330840980203 ) ) ;
#32637=CARTESIAN_POINT ( 'NONE',  ( -0.3240745752627050003, 1508.859753704990226, 238.3613378923800212 ) ) ;
#32639=CARTESIAN_POINT ( 'NONE',  ( 2.500000000000000000, 1448.894380902750072, 155.6080914261119972 ) ) ;
#32640=CARTESIAN_POINT ( 'NONE',  ( 10.27415084429999936, 1462.789161984029761, 234.7156815036980220 ) ) ;
#32642=CARTESIAN_POINT ( 'NONE',  ( -13.94141741770000031, 1444.723632129780071, 188.4161808736979822 ) ) ;
#32643=CARTESIAN_POINT ( 'NONE',  ( -15.55054316549999882, 1408.913060387329779, 218.7899552842880269 ) ) ;
#32645=CARTESIAN_POINT ( 'NONE',  ( 5.402393448019999767, 1407.889686284330082, 270.1311850753980366 ) ) ;
#32646=CARTESIAN_POINT ( 'NONE',  ( 1.449741897432649917, 1506.060387600080048, 181.1592481886430051 ) ) ;
#32650=CARTESIAN_POINT ( 'NONE',  ( -3.441813313009999487, 1475.979926173929925, 267.5320898906979892 ) ) ;
#32651=CARTESIAN_POINT ( 'NONE',  ( -4.221566735949540572, 1446.221982441119962, 169.5773968837689836 ) ) ;
#32653=CARTESIAN_POINT ( 'NONE',  ( -10.65998469088088285, 1486.512546998173775, 183.7751546670934886 ) ) ;
#32656=CARTESIAN_POINT ( 'NONE',  ( -4.884981308350000102E-15, 1441.600846913620217, 155.7224805731980268 ) ) ;
#32657=CARTESIAN_POINT ( 'NONE',  ( -24.99371936868969968, 1457.420242470830090, 211.0583525782739969 ) ) ;
#32659=CARTESIAN_POINT ( 'NONE',  ( 11.99447453070000158, 1410.787978747230227, 198.2808974363979928 ) ) ;
#32660=CARTESIAN_POINT ( 'NONE',  ( -1.270643054695779872, 1395.957432220560122, 220.0592832377249977 ) ) ;
#32662=CARTESIAN_POINT ( 'NONE',  ( -15.06702969580600104, 1422.390513282080065, 229.4662855426749672 ) ) ;
#32665=CARTESIAN_POINT ( 'NONE',  ( -4.069377925904865023, 1410.431552160933734, 232.1899145600301324 ) ) ;
#32673=CARTESIAN_POINT ( 'NONE',  ( 27.87287880629999748, 1445.634712509609926, 137.2901166997980056 ) ) ;
#32676=CARTESIAN_POINT ( 'NONE',  ( 20.83094015040000002, 1452.185627928030044, 134.0999999980979851 ) ) ;
#32677=CARTESIAN_POINT ( 'NONE',  ( -11.91237982683207441, 1398.266268150713813, 203.9165306044730244 ) ) ;
#32679=CARTESIAN_POINT ( 'NONE',  ( -21.92444879442203742, 1509.678679009930875, 190.3921826424486312 ) ) ;
#32681=CARTESIAN_POINT ( 'NONE',  ( 20.59987047751410216, 1509.677367640170132, 230.5839189361119850 ) ) ;
#32685=CARTESIAN_POINT ( 'NONE',  ( 11.30148062330549941, 1434.205170771390158, 151.5393079379209951 ) ) ;
#32686=CARTESIAN_POINT ( 'NONE',  ( -10.99057042539999962, 1396.296859563830139, 212.4415749538880220 ) ) ;
#32687=CARTESIAN_POINT ( 'NONE',  ( -20.10955669739999863, 1409.615301589730052, 218.0117348428780133 ) ) ;
#32688=VERTEX_POINT ( 'NONE', #23783 ) ;
#32690=CARTESIAN_POINT ( 'NONE',  ( -27.59578993569999739, 1509.876726607029923, 201.0523566146180201 ) ) ;
#32692=DIRECTION ( 'NONE',  ( -0.9993779840209170429, 0.0009463042317009280006, 0.03525265327019704714 ) ) ;
#32693=CARTESIAN_POINT ( 'NONE',  ( -14.07629452796359892, 1509.199332581739782, 183.4924235105400214 ) ) ;
#32694=CARTESIAN_POINT ( 'NONE',  ( 5.445834981259999985, 1449.233209377699950, 184.7342386783979862 ) ) ;
#32698=CARTESIAN_POINT ( 'NONE',  ( 7.500488151212729271, 1396.174983287849955, 201.0066138490270191 ) ) ;
#32699=CARTESIAN_POINT ( 'NONE',  ( 0.5943821362729999613, 1416.311719779230089, 190.5346383329979858 ) ) ;
#32700=CARTESIAN_POINT ( 'NONE',  ( 11.76831692830000087, 1432.246165101169936, 150.8114755703979881 ) ) ;
#32701=CARTESIAN_POINT ( 'NONE',  ( 5.561506164031474242, 1509.113139076760490, 180.2055687771843679 ) ) ;
#32703=CARTESIAN_POINT ( 'NONE',  ( 13.15418294748539907, 1434.930549361600015, 149.6534202118089922 ) ) ;
#32705=ORIENTED_EDGE ( 'NONE', *, *, #55628, .T. ) ;
#32706=CARTESIAN_POINT ( 'NONE',  ( 13.44021863898581159, 1444.325653863644675, 169.3641315964260343 ) ) ;
#32707=CARTESIAN_POINT ( 'NONE',  ( -6.622597241890000319, 1464.346823720030216, 234.5437523557980057 ) ) ;
#32708=CARTESIAN_POINT ( 'NONE',  ( -12.81144342830000049, 1416.820969729830040, 196.2462494151980081 ) ) ;
#32715=EDGE_CURVE ( 'NONE', #59085, #59795, #50125, .T. ) ;
#32717=ORIENTED_EDGE ( 'NONE', *, *, #76082, .F. ) ;
#32721=CARTESIAN_POINT ( 'NONE',  ( -20.06869840700000296, 1507.849569109330105, 229.0200580499979992 ) ) ;
#32722=EDGE_CURVE ( 'NONE', #90510, #84504, #59622, .T. ) ;
#32723=CARTESIAN_POINT ( 'NONE',  ( -11.06559390560000011, 1410.233130097329877, 188.8575565919979908 ) ) ;
#32724=CARTESIAN_POINT ( 'NONE',  ( -1.261572150459999930, 1410.336495002929951, 232.9947536822979828 ) ) ;
#32725=CARTESIAN_POINT ( 'NONE',  ( 0.05448001190707260633, 1416.221314539489867, 227.1460076434290158 ) ) ;
#32727=CARTESIAN_POINT ( 'NONE',  ( 18.24053064509999800, 1425.259887461229937, 223.9475156350980285 ) ) ;
#32730=CARTESIAN_POINT ( 'NONE',  ( -0.2608622107377010502, 1466.756006659810055, 235.6083744819270009 ) ) ;
#32731=CARTESIAN_POINT ( 'NONE',  ( 10.68754207573829973, 1410.138259118899896, 270.3681159542280170 ) ) ;
#32733=CARTESIAN_POINT ( 'NONE',  ( 24.06407462299999978, 1410.713862210129946, 208.8709579670279766 ) ) ;
#32738=CARTESIAN_POINT ( 'NONE',  ( 6.832964021560000489, 1409.413060387330006, 271.1218459616979999 ) ) ;
#32740=CARTESIAN_POINT ( 'NONE',  ( 3.194497190068566361, 1421.833025343917370, 139.1411856790333843 ) ) ;
#32742=VERTEX_POINT ( 'NONE', #102146 ) ;
#32744=CARTESIAN_POINT ( 'NONE',  ( -2.831258933819999884E-09, 1475.995240999430052, 267.2559760609979662 ) ) ;
#32753=DIRECTION ( 'NONE',  ( 0.4763271851929161138, 0.000000000000000000, 0.8792681119238848764 ) ) ;
#32756=CARTESIAN_POINT ( 'NONE',  ( -0.2697921844439999939, 1467.610413176630118, 229.6924542576979889 ) ) ;
#32757=CARTESIAN_POINT ( 'NONE',  ( 19.88034263189999962, 1455.027112605630009, 224.4525163018979868 ) ) ;
#32758=CARTESIAN_POINT ( 'NONE',  ( 8.660742842291162091, 1437.358295876703323, 153.3239294377561635 ) ) ;
#32761=CARTESIAN_POINT ( 'NONE',  ( 7.489142240313679366, 1416.917596226978048, 230.9382929016721562 ) ) ;
#32762=CARTESIAN_POINT ( 'NONE',  ( 30.86131930287799818, 1436.470231434929929, 136.6051523533310217 ) ) ;
#32763=CARTESIAN_POINT ( 'NONE',  ( 40.09012144279480339, 1445.376175965129960, 136.9018312957269927 ) ) ;
#32764=CARTESIAN_POINT ( 'NONE',  ( -23.28544946739999943, 1434.322615792679926, 214.3287644136879919 ) ) ;
#32767=CARTESIAN_POINT ( 'NONE',  ( 12.05022103600000172, 1508.335016562029978, 184.5151076142980173 ) ) ;
#32769=CARTESIAN_POINT ( 'NONE',  ( -34.27281677136750915, 1458.542448025342537, 269.5216919828922073 ) ) ;
#32770=ORIENTED_EDGE ( 'NONE', *, *, #33158, .F. ) ;
#32772=CARTESIAN_POINT ( 'NONE',  ( 15.27152964737910068, 1506.433683733550197, 193.3098315259690025 ) ) ;
#32774=CARTESIAN_POINT ( 'NONE',  ( -8.805428988939999257, 1497.713060387329961, 229.3821491682979854 ) ) ;
#32775=CARTESIAN_POINT ( 'NONE',  ( -0.02518341440730000394, 1415.404722957129934, 233.4400562564979964 ) ) ;
#32776=CARTESIAN_POINT ( 'NONE',  ( -12.76951649852674286, 1444.992622299949517, 185.9723966557366737 ) ) ;
#32779=CARTESIAN_POINT ( 'NONE',  ( -6.910691058390185937, 1416.743833086882205, 231.4108548000287726 ) ) ;
#32780=CARTESIAN_POINT ( 'NONE',  ( -18.84855559419433391, 1451.021439095374490, 146.7293775064046599 ) ) ;
#32781=CARTESIAN_POINT ( 'NONE',  ( 25.74428607489999976, 1435.913748434279796, 136.6865143993979927 ) ) ;
#32783=CARTESIAN_POINT ( 'NONE',  ( -14.55268370649999987, 1410.361136006629977, 226.7453334963979898 ) ) ;
#32785=CARTESIAN_POINT ( 'NONE',  ( 0.3106767230383539746, 1415.088506334920112, 192.0574112331409822 ) ) ;
#32788=VERTEX_POINT ( 'NONE', #25427 ) ;
#32792=CARTESIAN_POINT ( 'NONE',  ( -16.58880512860000067, 1456.884093369330003, 220.8293426371980104 ) ) ;
#32793=CARTESIAN_POINT ( 'NONE',  ( -20.53924275249999809, 1507.908979316930072, 189.7573387548980008 ) ) ;
#32794=CARTESIAN_POINT ( 'NONE',  ( -11.71913435010000093, 1433.163605237980164, 150.8449725526980103 ) ) ;
#32798=CARTESIAN_POINT ( 'NONE',  ( -24.34803299149999845, 1439.482366230929983, 212.0309832708680062 ) ) ;
#32800=CARTESIAN_POINT ( 'NONE',  ( -0.1155235852791031970, 1467.141897078556440, 235.6414018107566335 ) ) ;
#32802=CARTESIAN_POINT ( 'NONE',  ( -20.18749645201030063, 1509.735829383545934, 186.8627948558383878 ) ) ;
#32806=CARTESIAN_POINT ( 'NONE',  ( -11.77540867291269855, 1427.269330905989818, 146.7706912077400148 ) ) ;
#32808=CARTESIAN_POINT ( 'NONE',  ( -5.260636025280000183, 1472.387947547730164, 270.3705385644980197 ) ) ;
#32812=CARTESIAN_POINT ( 'NONE',  ( 21.45452449210000267, 1497.713060387329961, 205.0582954851479940 ) ) ;
#32815=CARTESIAN_POINT ( 'NONE',  ( -6.833118095721640195, 1429.964654908410012, 222.3013511789650067 ) ) ;
#32818=CARTESIAN_POINT ( 'NONE',  ( -15.41942199670529945, 1408.188993866129977, 269.2062666358880278 ) ) ;
#32819=CARTESIAN_POINT ( 'NONE',  ( -13.21521023968930031, 1435.711572018790093, 150.5102260760120032 ) ) ;
#32822=VERTEX_POINT ( 'NONE', #110561 ) ;
#32824=CARTESIAN_POINT ( 'NONE',  ( 4.882230504881198030, 1422.395003669154676, 184.3285600118643117 ) ) ;
#32827=CARTESIAN_POINT ( 'NONE',  ( -16.72315470559999895, 1470.469491759329912, 188.8178631691980058 ) ) ;
#32828=CARTESIAN_POINT ( 'NONE',  ( -16.93883337398300171, 1507.634953145470035, 230.1482688801679899 ) ) ;
#32829=ORIENTED_EDGE ( 'NONE', *, *, #26542, .F. ) ;
#32834=FACE_OUTER_BOUND ( 'NONE', #88302, .T. ) ;
#32837=CARTESIAN_POINT ( 'NONE',  ( -38.59236949370799863, 1443.548215515760148, 137.1678974980329997 ) ) ;
#32840=CARTESIAN_POINT ( 'NONE',  ( 26.14369035709999878, 1488.683671327730053, 214.7624555471579981 ) ) ;
#32841=AXIS2_PLACEMENT_3D ( 'NONE', #46499, #96331, #88483 ) ;
#32842=CARTESIAN_POINT ( 'NONE',  ( 5.808733308747313195, 1474.842457401947740, 269.6417025878172353 ) ) ;
#32845=CARTESIAN_POINT ( 'NONE',  ( -24.46154330250000086, 1442.364448987709920, 211.0683006204080243 ) ) ;
#32848=CIRCLE ( 'NONE', #755, 1.500000000000001332 ) ;
#32849=CARTESIAN_POINT ( 'NONE',  ( -0.3328314641405109575, 1452.976685807730291, 183.2631399573310205 ) ) ;
#32851=CARTESIAN_POINT ( 'NONE',  ( -13.08238251380000072, 1414.913528139129994, 220.2039091924980028 ) ) ;
#32854=FACE_OUTER_BOUND ( 'NONE', #107207, .T. ) ;
#32856=CARTESIAN_POINT ( 'NONE',  ( -19.59641516460481725, 1457.071779919169330, 225.8968562730828467 ) ) ;
#32859=CARTESIAN_POINT ( 'NONE',  ( 12.85396610232849923, 1434.713524430809912, 149.4748486273309993 ) ) ;
#32860=B_SPLINE_SURFACE_WITH_KNOTS ( 'NONE', 5, 5, ( 
 ( #39514, #3184, #73688, #19942, #88265, #63106 ),
 ( #20477, #72049, #29443, #63642, #67490, #101595 ),
 ( #50668, #91569, #58530, #5912, #40609, #31650 ),
 ( #83711, #56874, #109479, #14844, #15391, #23245 ),
 ( #32756, #110570, #42267, #65832, #24879, #84800 ),
 ( #101046, #83169, #41164, #91003, #40059, #108920 ) ),
 .UNSPECIFIED., .F., .F., .F.,
 ( 6, 6 ),
 ( 6, 6 ),
 ( 19.55448171529999968, 88.89713672540000289 ),
 ( -2.775557561569999727E-17, 1.000000000000000000 ),
 .UNSPECIFIED. ) ;
#32861=CARTESIAN_POINT ( 'NONE',  ( -4.074500880610250064, 1440.601538448055862, 185.2207594585182164 ) ) ;
#32864=CARTESIAN_POINT ( 'NONE',  ( -11.44902708475428987, 1425.804265263478555, 139.1023607573540630 ) ) ;
#32866=LINE ( 'NONE', #92779, #50169 ) ;
#32867=CARTESIAN_POINT ( 'NONE',  ( -15.06903107870000191, 1410.389868148830146, 226.7125060204980116 ) ) ;
#32873=ORIENTED_EDGE ( 'NONE', *, *, #110454, .F. ) ;
#32875=B_SPLINE_SURFACE_WITH_KNOTS ( 'NONE', 5, 3, ( 
 ( #45823, #45273, #88901, #79411 ),
 ( #54769, #71037, #96205, #97299 ),
 ( #2723, #21669, #3829, #37403 ),
 ( #38489, #36845, #62079, #37957 ),
 ( #63728, #28450, #62644, #72666 ),
 ( #72137, #97838, #106792, #79956 ) ),
 .UNSPECIFIED., .F., .F., .F.,
 ( 6, 6 ),
 ( 4, 4 ),
 ( 0.000000000000000000, 52.98902693510000006 ),
 ( 37.69911184309999896, 40.20365518519999881 ),
 .UNSPECIFIED. ) ;
#32877=CARTESIAN_POINT ( 'NONE',  ( 0.9849188036980001115, 1419.502007416729839, 184.7914211646979936 ) ) ;
#32878=B_SPLINE_CURVE_WITH_KNOTS ( 'NONE', 3,
 ( #1899, #104884, #45559, #62361, #52846, #36035, #96485, #79700, #19766, #53967, #97585, #3005, #104330, #11387, #71326, #61809, #70225, #106532, #27623, #105440, #46105, #80235, #2459, #4094, #55053, #28729, #88649, #62934, #37678, #20857, #3555, #86972, #97046, #71882, #20309, #89180, #54512, #95931, #29274, #19191, #63466, #12472, #64007, #53395, #46656, #38219, #98119, #72401 ),
 .UNSPECIFIED., .F., .F.,
 ( 4, 2, 2, 1, 1, 1, 1, 2, 2, 2, 2, 2, 1, 1, 1, 1, 2, 2, 2, 2, 2, 1, 1, 1, 1, 1, 1, 2, 2, 2, 4 ),
 ( 0.000000000000000000, 0.1249999999999676648, 0.1874999999999503175, 0.2187499999999427680, 0.2343749999999387990, 0.2421874999999371336, 0.2460937499999352185, 0.2480468749999343858, 0.2499999999999335532, 0.3749999999998849809, 0.4374999999998616662, 0.4687499999998501754, 0.4843749999998440137, 0.4921874999998419598, 0.4960937499998416267, 0.4980468749998407385, 0.4990234374998410161, 0.4999999999998412381, 0.6249999999996845856, 0.6874999999996069810, 0.7187499999995685673, 0.7343749999995491384, 0.7421874999995393685, 0.7460937499995340394, 0.7480468749995313749, 0.7490234374995307087, 0.7495117187495299316, 0.7497558593745294875, 0.7499999999995291544, 0.8749999999997645217, 1.000000000000000000 ),
 .UNSPECIFIED. ) ;
#32884=CARTESIAN_POINT ( 'NONE',  ( 17.25473568693964665, 1422.487072245637364, 226.6732862807842821 ) ) ;
#32886=CARTESIAN_POINT ( 'NONE',  ( 39.91818200059610433, 1440.913060366189939, 259.1711454722760095 ) ) ;
#32891=EDGE_LOOP ( 'NONE', ( #31100, #76346, #2455, #81173 ) ) ;
#32892=DIRECTION ( 'NONE',  ( 2.148885482424154438E-07, 0.03085800255252074339, 0.9995237784457268182 ) ) ;
#32896=DIRECTION ( 'NONE',  ( -0.7835778918569903384, -0.02736314294039966441, -0.6206907005919922726 ) ) ;
#32901=EDGE_CURVE ( 'NONE', #39470, #80762, #31201, .T. ) ;
#32902=EDGE_CURVE ( 'NONE', #48553, #88847, #94520, .T. ) ;
#32903=CARTESIAN_POINT ( 'NONE',  ( -12.27023095390000051, 1416.839692139930094, 194.6640140145979956 ) ) ;
#32904=LINE ( 'NONE', #8251, #42886 ) ;
#32914=VERTEX_POINT ( 'NONE', #99115 ) ;
#32915=ADVANCED_FACE ( 'NONE', ( #75609 ), #104289, .F. ) ;
#32928=CARTESIAN_POINT ( 'NONE',  ( 18.03146720619200138, 1424.667981931974055, 225.2975763146619954 ) ) ;
#32929=CARTESIAN_POINT ( 'NONE',  ( 4.408868868459999923, 1425.824683875729988, 185.4670087524980033 ) ) ;
#32930=CARTESIAN_POINT ( 'NONE',  ( -10.96966273854589957, 1432.359729197300112, 151.7701366752919796 ) ) ;
#32931=CARTESIAN_POINT ( 'NONE',  ( -2.705839759132969924, 1440.724342078179916, 165.1197109057160048 ) ) ;
#32934=CARTESIAN_POINT ( 'NONE',  ( 4.196074440480000121E-15, 1430.453334911130241, 150.3332009510979788 ) ) ;
#32935=EDGE_CURVE ( 'NONE', #18384, #35589, #14743, .T. ) ;
#32936=CARTESIAN_POINT ( 'NONE',  ( 18.74257907359240249, 1456.927692655689953, 228.0561368610119928 ) ) ;
#32939=CARTESIAN_POINT ( 'NONE',  ( 20.19452632973207784, 1436.434739331579522, 145.2312131346681667 ) ) ;
#32940=CARTESIAN_POINT ( 'NONE',  ( -1.342110557989999897, 1416.822690122629865, 228.0800073794979994 ) ) ;
#32943=ADVANCED_FACE ( 'NONE', ( #20615 ), #36341, .F. ) ;
#32946=CARTESIAN_POINT ( 'NONE',  ( -45.63704539349389933, 1440.913071918759897, 268.9748468665420091 ) ) ;
#32951=CARTESIAN_POINT ( 'NONE',  ( -2.478936252380000038, 1432.480737126569920, 157.5199335589979910 ) ) ;
#32955=CARTESIAN_POINT ( 'NONE',  ( -26.51713393923600037, 1451.737905241030148, 135.8255081778609963 ) ) ;
#32957=CARTESIAN_POINT ( 'NONE',  ( 4.123065267750000373, 1419.629243940029937, 225.6556823394980142 ) ) ;
#32961=CARTESIAN_POINT ( 'NONE',  ( -21.38445639499393636, 1453.349625645140804, 224.4824140893579170 ) ) ;
#32964=CARTESIAN_POINT ( 'NONE',  ( -5399.190776299624304, 2837.541834147241843, -8134.792049093260175 ) ) ;
#32966=FACE_OUTER_BOUND ( 'NONE', #32307, .T. ) ;
#32967=CARTESIAN_POINT ( 'NONE',  ( 13.16549422024820082, 1421.079389199930120, 230.1572586433449885 ) ) ;
#32972=CARTESIAN_POINT ( 'NONE',  ( -24.07249582042329905, 1410.733237779120145, 208.8823328027320088 ) ) ;
#32973=ORIENTED_EDGE ( 'NONE', *, *, #49528, .T. ) ;
#32975=CARTESIAN_POINT ( 'NONE',  ( -9.534219445089998857, 1428.030197386430018, 144.1938086916980239 ) ) ;
#32976=CARTESIAN_POINT ( 'NONE',  ( -5.800026419229999064, 1498.346957321030231, 235.6600973397979999 ) ) ;
#32979=CARTESIAN_POINT ( 'NONE',  ( 45.40562959789710362, 1446.095626619519862, 268.7700954888649676 ) ) ;
#32985=CARTESIAN_POINT ( 'NONE',  ( 19.00284581381210103, 1457.321592500673205, 226.5478147772149953 ) ) ;
#32990=CARTESIAN_POINT ( 'NONE',  ( 26.67349319650000083, 1451.732280616630078, 135.8047305359980044 ) ) ;
#32992=CARTESIAN_POINT ( 'NONE',  ( 3.484502295585529819, 1452.791378885890026, 152.3153881425679970 ) ) ;
#32995=B_SPLINE_SURFACE_WITH_KNOTS ( 'NONE', 4, 5, ( 
 ( #7968, #100908, #59499, #49986, #34276, #7422, #42135, #76841, #33167 ),
 ( #93072, #76285, #110435, #16889, #67906, #60055, #66265, #25298, #17444 ),
 ( #51641, #85779, #77395, #697, #37032, #70682, #71227, #96399, #18012 ),
 ( #62843, #70132, #69013, #80141, #61179, #28638, #86332, #46010, #34826 ),
 ( #11301, #88556, #88017, #69570, #52751, #61717, #9618, #96956, #35382 ),
 ( #18557, #86884, #52205, #104244, #78495, #105349, #104795, #79065, #28082 ),
 ( #19674, #10178, #103118, #26419, #53880, #36485, #43787, #27534, #45469 ),
 ( #1244, #53310, #20222, #62270, #103689, #77937, #79611, #94733, #26990 ),
 ( #44353, #54423, #95296, #1809, #2915, #11839, #35946, #60611, #87451 ) ),
 .UNSPECIFIED., .F., .F., .F.,
 ( 5, 4, 5 ),
 ( 6, 3, 6 ),
 ( 74.12006598165800142, 74.13176850000000684, 75.30202033419999452 ),
 ( 0.000000000000000000, 1.000000000000000000, 2.000000000000000000 ),
 .UNSPECIFIED. ) ;
#32998=CARTESIAN_POINT ( 'NONE',  ( 2.139403947300960063, 1408.987770019419941, 186.9664919645120165 ) ) ;
#33002=EDGE_CURVE ( 'NONE', #99650, #27637, #29065, .T. ) ;
#33004=AXIS2_PLACEMENT_3D ( 'NONE', #36469, #62255, #71775 ) ;
#33007=CARTESIAN_POINT ( 'NONE',  ( 12.95840410776399843, 1416.218047878440075, 221.5780283176839873 ) ) ;
#33010=B_SPLINE_SURFACE_WITH_KNOTS ( 'NONE', 5, 5, ( 
 ( #64460, #98576, #90727, #64998, #81768, #40878, #109206, #32491, #66663 ),
 ( #100766, #22955, #24056, #89628, #12916, #90168, #47096, #13450, #39220 ),
 ( #73396, #107532, #99116, #110286, #94580, #9483, #68873, #16743, #85075 ),
 ( #8367, #34683, #42535, #34133, #59913, #35238, #84534, #86191, #68321 ),
 ( #33022, #67208, #59364, #33562, #50409, #94033, #43647, #8924, #25712 ),
 ( #17857, #58794, #52056, #102974, #24600, #15644, #67756, #7822, #26273 ) ),
 .UNSPECIFIED., .F., .F., .F.,
 ( 6, 6 ),
 ( 6, 3, 6 ),
 ( 0.4666582265010000286, 2.797885342409359932 ),
 ( -1.082959936422979947E-05, 1.000000000000000000, 2.000000000000000000 ),
 .UNSPECIFIED. ) ;
#33012=( BOUNDED_SURFACE ( )  B_SPLINE_SURFACE ( 4, 2, ( 
 ( #109003, #65911, #100029 ),
 ( #47447, #107884, #32287 ),
 ( #39016, #90531, #6534 ),
 ( #23321, #98930, #55863 ),
 ( #14914, #46914, #22750 ) ),
 .UNSPECIFIED., .F., .F., .F. ) 
 B_SPLINE_SURFACE_WITH_KNOTS ( ( 5, 5 ),
 ( 3, 3 ),
 ( 3.613988937040000238, 5.260361675040000407 ),
 ( 5.300753508049940166, 6.150216337544540224 ),
 .UNSPECIFIED. ) 
 GEOMETRIC_REPRESENTATION_ITEM ( )  RATIONAL_B_SPLINE_SURFACE ( (
 ( 0.8627701935039370218, 0.8230341786337309617, 0.9546103739810829492),
 ( 0.8627701935039370218, 0.8230341786337309617, 0.9546103739810829492),
 ( 0.8627701935039370218, 0.8230341786337309617, 0.9546103739810829492),
 ( 0.8627701935039370218, 0.8230341786337309617, 0.9546103739810829492),
 ( 0.8627701935039370218, 0.8230341786337309617, 0.9546103739810829492) ) ) 
 REPRESENTATION_ITEM ( '' )  SURFACE ( )  );
#33016=CARTESIAN_POINT ( 'NONE',  ( -26.86204968941349946, 1508.007394745769943, 212.0120970035400205 ) ) ;
#33018=CARTESIAN_POINT ( 'NONE',  ( -21.18003089992732768, 1508.593876776232719, 192.0369185836293013 ) ) ;
#33019=CARTESIAN_POINT ( 'NONE',  ( 11.44209389759999951, 1433.338294488139809, 151.3396440961979863 ) ) ;
#33020=CARTESIAN_POINT ( 'NONE',  ( 36.99165393049999295, 1454.692295987030093, 268.3665355201979992 ) ) ;
#33022=CARTESIAN_POINT ( 'NONE',  ( 11.54244540325870005, 1414.913060387399810, 197.8963259754790158 ) ) ;
#33023=LINE ( 'NONE', #67212, #20713 ) ;
#33027=CARTESIAN_POINT ( 'NONE',  ( 12.49661969954494900, 1398.283518850857035, 212.9844610132695664 ) ) ;
#33029=CARTESIAN_POINT ( 'NONE',  ( 23.99427320690000087, 1410.919622257430092, 209.9798509652409848 ) ) ;
#33037=CARTESIAN_POINT ( 'NONE',  ( -3.456072659400000191, 1414.971339025629959, 226.0233698056979961 ) ) ;
#33040=CARTESIAN_POINT ( 'NONE',  ( 0.1734663674328389971, 1478.296956495260247, 182.1675436825559871 ) ) ;
#33042=CARTESIAN_POINT ( 'NONE',  ( -20.24673233129999872, 1443.913060387330006, 162.1129423953979938 ) ) ;
#33043=EDGE_CURVE ( 'NONE', #28487, #92672, #41923, .T. ) ;
#33046=CARTESIAN_POINT ( 'NONE',  ( -40.90250537898710093, 1447.119793117110021, 134.0999999985199906 ) ) ;
#33048=ORIENTED_EDGE ( 'NONE', *, *, #11395, .F. ) ;
#33059=CARTESIAN_POINT ( 'NONE',  ( 18.05542497264820057, 1416.825784014559986, 208.7596466293869923 ) ) ;
#33063=ORIENTED_EDGE ( 'NONE', *, *, #82941, .T. ) ;
#33064=CARTESIAN_POINT ( 'NONE',  ( -33.29550093079999584, 1450.462297931059993, 136.2636478384980023 ) ) ;
#33066=CARTESIAN_POINT ( 'NONE',  ( 3.827327205999999649, 1418.913060387330006, 172.2701767054979882 ) ) ;
#33068=ORIENTED_EDGE ( 'NONE', *, *, #66255, .F. ) ;
#33070=CARTESIAN_POINT ( 'NONE',  ( -15.10371725490000117, 1409.440493816029857, 225.2902966875980155 ) ) ;
#33073=CARTESIAN_POINT ( 'NONE',  ( 41.32342021774600482, 1446.574054804671050, 269.6346703930319677 ) ) ;
#33074=CARTESIAN_POINT ( 'NONE',  ( -11.60004869885203505, 1427.693913909466573, 134.2641720911346681 ) ) ;
#33075=CARTESIAN_POINT ( 'NONE',  ( 16.17016470285728857, 1432.043082342410344, 218.4496149275423988 ) ) ;
#33076=CARTESIAN_POINT ( 'NONE',  ( 2.407361919430000441, 1417.795499740929927, 234.0370795184979897 ) ) ;
#33077=CARTESIAN_POINT ( 'NONE',  ( 2.500000000000000000, 1434.142768437249970, 183.0182394769479970 ) ) ;
#33079=FACE_OUTER_BOUND ( 'NONE', #36751, .T. ) ;
#33084=CARTESIAN_POINT ( 'NONE',  ( 2.715357296970000167, 1447.820972075539885, 154.4673902800980159 ) ) ;
#33088=CARTESIAN_POINT ( 'NONE',  ( 13.89869200000000049, 1452.835253893030085, 223.8385666725980059 ) ) ;
#33089=CARTESIAN_POINT ( 'NONE',  ( -2.109056957580000002, 1421.166295015029846, 183.8085771866980167 ) ) ;
#33095=CARTESIAN_POINT ( 'NONE',  ( -23.75028666920000120, 1410.916158857830169, 207.2858998927080165 ) ) ;
#33096=CARTESIAN_POINT ( 'NONE',  ( -11.73996803256352095, 1426.694174138938934, 144.3809647795363560 ) ) ;
#33097=CARTESIAN_POINT ( 'NONE',  ( 15.78476754123740022, 1409.716999194859909, 192.1026167944760061 ) ) ;
#33099=CARTESIAN_POINT ( 'NONE',  ( 38.76435533041719594, 1438.005125630080101, 136.3470787082570155 ) ) ;
#33100=B_SPLINE_SURFACE_WITH_KNOTS ( 'NONE', 5, 5, ( 
 ( #9772, #78081, #1384, #35526, #61324, #95442, #30981, #65706, #81370 ),
 ( #74110, #107697, #29876, #30431, #108240, #39940, #90887, #21455, #55665 ),
 ( #81930, #66277, #40485, #91450, #48357, #56750, #14726, #107138, #47244 ),
 ( #89788, #13058, #99827, #5233, #20914, #74660, #48916, #82497, #14172 ),
 ( #64617, #4685, #38824, #73003, #23119, #55118, #5799, #98737, #13606 ),
 ( #21998, #56191, #90327, #65156, #99270, #47794, #39387, #73564, #22548 ) ),
 .UNSPECIFIED., .F., .F., .F.,
 ( 6, 6 ),
 ( 6, 3, 6 ),
 ( 10.26165209716149995, 12.52004467320000103 ),
 ( 0.000000000000000000, 1.000000000000000000, 2.000000000000000000 ),
 .UNSPECIFIED. ) ;
#33101=CARTESIAN_POINT ( 'NONE',  ( -11.63658410760000095, 1425.864915301529891, 144.1607460166979990 ) ) ;
#33103=CARTESIAN_POINT ( 'NONE',  ( 16.79818491188742513, 1460.579683146600928, 228.8802028025106665 ) ) ;
#33105=CARTESIAN_POINT ( 'NONE',  ( 37.84675541841409796, 1450.538956397299899, 134.0999999985309898 ) ) ;
#33106=CARTESIAN_POINT ( 'NONE',  ( -38.53567264009640070, 1439.151675925619884, 136.6512514728599967 ) ) ;
#33109=B_SPLINE_CURVE_WITH_KNOTS ( 'NONE', 5,
 ( #101211, #50840, #89660, #76042, #12946, #83330, #25057, #40227, #49202, #82781, #74410, #84971 ),
 .UNSPECIFIED., .F., .F.,
 ( 6, 3, 3, 6 ),
 ( 0.000000000000000000, 3.329846645400000416, 4.930332151970000076, 12.58720418400000085 ),
 .UNSPECIFIED. ) ;
#33110=CARTESIAN_POINT ( 'NONE',  ( -18.57062135440000006, 1457.638594930429917, 227.6943395327979829 ) ) ;
#33111=ORIENTED_EDGE ( 'NONE', *, *, #97559, .T. ) ;
#33118=DIRECTION ( 'NONE',  ( 0.3390050494208853293, -0.7071067811868682051, 0.6205445805634673961 ) ) ;
#33119=CARTESIAN_POINT ( 'NONE',  ( 40.71747596219820053, 1438.773003613790024, 135.0591077376159888 ) ) ;
#33122=CARTESIAN_POINT ( 'NONE',  ( 26.28888947440000123, 1436.471222792599974, 136.7656709048980019 ) ) ;
#33123=CARTESIAN_POINT ( 'NONE',  ( 38.12323339995595006, 1442.831169986191526, 136.9072173714204723 ) ) ;
#33131=ORIENTED_EDGE ( 'NONE', *, *, #6246, .F. ) ;
#33132=CARTESIAN_POINT ( 'NONE',  ( -13.91384509699999938, 1415.996778984329922, 221.6684481777979840 ) ) ;
#33136=CARTESIAN_POINT ( 'NONE',  ( -13.06606033770000153, 1422.974160590630163, 222.1234525822980004 ) ) ;
#33139=CARTESIAN_POINT ( 'NONE',  ( 8.178501070643639181, 1441.152429762079919, 153.9860758848200248 ) ) ;
#33141=CARTESIAN_POINT ( 'NONE',  ( -15.08386190559999918, 1451.324666099630122, 222.9201800246979985 ) ) ;
#33148=ORIENTED_EDGE ( 'NONE', *, *, #26077, .F. ) ;
#33149=LINE ( 'NONE', #58923, #53346 ) ;
#33152=CARTESIAN_POINT ( 'NONE',  ( -2.908982738435793802, 1484.703267874767107, 183.2481867733562240 ) ) ;
#33155=EDGE_LOOP ( 'NONE', ( #13918, #22949, #8973, #74930 ) ) ;
#33158=EDGE_CURVE ( 'NONE', #102491, #67527, #64878, .T. ) ;
#33159=CARTESIAN_POINT ( 'NONE',  ( -11.52457544480000173, 1428.535701648929944, 150.0557210695980075 ) ) ;
#33160=CARTESIAN_POINT ( 'NONE',  ( 19.04937065429340137, 1456.924701486199865, 225.3692720049160130 ) ) ;
#33161=CARTESIAN_POINT ( 'NONE',  ( -4.078211669849999943, 1440.299026235899873, 185.4566092242980062 ) ) ;
#33164=CARTESIAN_POINT ( 'NONE',  ( 0.2637998666456179975, 1430.332984592310140, 190.1847976646700147 ) ) ;
#33165=CARTESIAN_POINT ( 'NONE',  ( -22.75471552770000017, 1495.366693290230160, 223.7173521039980244 ) ) ;
#33166=CARTESIAN_POINT ( 'NONE',  ( -8.141993531839686327, 1423.434677666080006, 137.0999999981440851 ) ) ;
#33167=CARTESIAN_POINT ( 'NONE',  ( -16.17998770715999868, 1459.144433622870110, 230.7168371058380103 ) ) ;
#33170=CARTESIAN_POINT ( 'NONE',  ( 4.991008440799999946, 1405.971275674329945, 268.4734096741979670 ) ) ;
#33171=CARTESIAN_POINT ( 'NONE',  ( -0.1426365273169999948, 1409.853703886329868, 185.0414845334979930 ) ) ;
#33172=CARTESIAN_POINT ( 'NONE',  ( 18.52231723690000464, 1430.306689337430043, 192.7617654628980119 ) ) ;
#33173=FACE_OUTER_BOUND ( 'NONE', #79392, .T. ) ;
#33176=CARTESIAN_POINT ( 'NONE',  ( 11.90000415720300175, 1434.913060496859998, 147.6452464505769910 ) ) ;
#33179=CARTESIAN_POINT ( 'NONE',  ( -12.88374579789999963, 1445.168051104930100, 187.0888182765980048 ) ) ;
#33183=CARTESIAN_POINT ( 'NONE',  ( 13.58968549309999929, 1409.153350369530017, 270.0972160545979932 ) ) ;
#33185=CARTESIAN_POINT ( 'NONE',  ( 1.461819939759239961, 1494.181313383729730, 181.6773600568459983 ) ) ;
#33186=CARTESIAN_POINT ( 'NONE',  ( -8.800012970690000103, 1429.116251061429921, 209.1218459616979999 ) ) ;
#33188=EDGE_CURVE ( 'NONE', #6013, #79565, #64556, .T. ) ;
#33190=CARTESIAN_POINT ( 'NONE',  ( -6.972260506549999626, 1474.659203917630066, 269.6344785065979863 ) ) ;
#33195=CARTESIAN_POINT ( 'NONE',  ( 1.951029616821370327, 1508.751449870507940, 237.3205679132474870 ) ) ;
#33196=CARTESIAN_POINT ( 'NONE',  ( 11.57234447799390153, 1415.219159638040082, 222.8946685903029845 ) ) ;
#33197=EDGE_CURVE ( 'NONE', #86349, #98568, #60321, .T. ) ;
#33202=CARTESIAN_POINT ( 'NONE',  ( -21.49788281959999736, 1409.663783000529975, 203.5162482710680081 ) ) ;
#33213=CARTESIAN_POINT ( 'NONE',  ( 11.72262950227709943, 1426.705135300079974, 143.1384147304339933 ) ) ;
#33217=CARTESIAN_POINT ( 'NONE',  ( 11.60004869885204748, 1428.977684734793684, 135.1000015630646089 ) ) ;
#33225=CARTESIAN_POINT ( 'NONE',  ( 20.33996727594809784, 1508.367434211329964, 228.7312766114060310 ) ) ;
#33227=VERTEX_POINT ( 'NONE', #34551 ) ;
#33229=CARTESIAN_POINT ( 'NONE',  ( 11.68034705308759946, 1434.603008417340106, 151.2598176529760394 ) ) ;
#33230=CARTESIAN_POINT ( 'NONE',  ( -13.25226091950000118, 1397.693633465330095, 207.3660310399680213 ) ) ;
#33231=ORIENTED_EDGE ( 'NONE', *, *, #13224, .T. ) ;
#33233=CARTESIAN_POINT ( 'NONE',  ( 0.08492873675443529669, 1416.830086716310007, 227.2254341622459890 ) ) ;
#33237=EDGE_CURVE ( 'NONE', #27375, #102562, #60892, .T. ) ;
#33239=CARTESIAN_POINT ( 'NONE',  ( 0.1442700600540000044, 1449.244366658050012, 183.3525652805980144 ) ) ;
#33243=CARTESIAN_POINT ( 'NONE',  ( 0.9063479630919999419, 1415.579607672129896, 190.7747571620979841 ) ) ;
#33244=CARTESIAN_POINT ( 'NONE',  ( 10.95578206839999957, 1431.353415687319966, 151.7028741494979727 ) ) ;
#33246=ORIENTED_EDGE ( 'NONE', *, *, #62192, .F. ) ;
#33247=CARTESIAN_POINT ( 'NONE',  ( 13.04378404802559999, 1435.095357528140084, 150.1247056565019875 ) ) ;
#33250=CARTESIAN_POINT ( 'NONE',  ( 13.50674943976829923, 1444.060515704980617, 169.3531493163527841 ) ) ;
#33251=CARTESIAN_POINT ( 'NONE',  ( -10.86270151549999952, 1462.682638981130140, 232.4998425783980167 ) ) ;
#33256=CARTESIAN_POINT ( 'NONE',  ( -1.795474957570000196, 1417.667352959230129, 185.7226290440979994 ) ) ;
#33258=VECTOR ( 'NONE', #20994, 1000.000000000000000 ) ;
#33259=CIRCLE ( 'NONE', #51101, 95.87902101811344835 ) ;
#33264=CARTESIAN_POINT ( 'NONE',  ( -19.41936053389999728, 1509.602162800930046, 231.4138353120980014 ) ) ;
#33265=CARTESIAN_POINT ( 'NONE',  ( -2.825023580110000321, 1409.011712384230123, 187.6092932735979844 ) ) ;
#33267=CARTESIAN_POINT ( 'NONE',  ( -0.04548916784355099691, 1416.835419214280137, 227.2860346676060033 ) ) ;
#33268=ORIENTED_EDGE ( 'NONE', *, *, #23541, .T. ) ;
#33269=CARTESIAN_POINT ( 'NONE',  ( 20.47396129670000064, 1428.228733271429974, 221.3183212327980129 ) ) ;
#33271=DIRECTION ( 'NONE',  ( -0.7122454525621805255, 0.000000000000000000, -0.7019304917899598095 ) ) ;
#33272=CARTESIAN_POINT ( 'NONE',  ( 0.003131168146805529684, 1465.436577107210042, 236.3247334268170050 ) ) ;
#33275=VECTOR ( 'NONE', #24323, 1000.000000000000000 ) ;
#33276=CARTESIAN_POINT ( 'NONE',  ( -21.29838079570000176, 1509.400478363229922, 190.2048059474979880 ) ) ;
#33277=CARTESIAN_POINT ( 'NONE',  ( -11.60004869885203682, 1422.222932908413441, 135.5999999980979851 ) ) ;
#33280=CARTESIAN_POINT ( 'NONE',  ( 0.3035063570619999651, 1419.252315944230077, 184.6483515716980151 ) ) ;
#33281=CARTESIAN_POINT ( 'NONE',  ( 0.3788332004054269508, 1408.926289534200123, 231.6114332047860103 ) ) ;
#33285=CARTESIAN_POINT ( 'NONE',  ( 5.805167347800000321, 1470.400767513130177, 255.2684315055980164 ) ) ;
#33286=CARTESIAN_POINT ( 'NONE',  ( -16.99532478110185352, 1414.913372219064513, 207.6629708034409987 ) ) ;
#33287=CARTESIAN_POINT ( 'NONE',  ( -5.106121334268481249, 1414.913060387329779, 224.8220620046302258 ) ) ;
#33289=CARTESIAN_POINT ( 'NONE',  ( -23.97381281639999884, 1445.664824722570074, 212.8527451534280033 ) ) ;
#33295=ORIENTED_EDGE ( 'NONE', *, *, #93946, .F. ) ;
#33298=CARTESIAN_POINT ( 'NONE',  ( -4.348753001182549001E-06, 1471.791680084430027, 269.8654495627969823 ) ) ;
#33302=CARTESIAN_POINT ( 'NONE',  ( 10.05619454328154028, 1417.844773168630354, 230.1417765312870358 ) ) ;
#33303=CARTESIAN_POINT ( 'NONE',  ( 27.07894067153570106, 1435.916767153840055, 136.5177824053259883 ) ) ;
#33304=CARTESIAN_POINT ( 'NONE',  ( 39.32311757029869170, 1447.249813977000031, 136.6052348694120155 ) ) ;
#33305=CARTESIAN_POINT ( 'NONE',  ( -41.78301679711650962, 1454.669324826605816, 269.0815855111645760 ) ) ;
#33308=CARTESIAN_POINT ( 'NONE',  ( 10.37139043059999999, 1508.772077727729993, 183.3025791525980139 ) ) ;
#33310=CARTESIAN_POINT ( 'NONE',  ( -18.42949978517250642, 1468.381198263613442, 269.3800990424684869 ) ) ;
#33313=CARTESIAN_POINT ( 'NONE',  ( -32.03120862260659152, 1416.568755244754811, 269.3150988356668449 ) ) ;
#33315=CARTESIAN_POINT ( 'NONE',  ( 10.87197521136500633, 1424.812830435537762, 138.2079135145058046 ) ) ;
#33317=CARTESIAN_POINT ( 'NONE',  ( -28.26971844339999862, 1508.651302072330054, 208.8373477021380324 ) ) ;
#33322=CARTESIAN_POINT ( 'NONE',  ( -14.45746094946127869, 1451.170343819680056, 150.0640874590992269 ) ) ;
#33323=ADVANCED_FACE ( 'NONE', ( #18287 ), #917, .T. ) ;
#33324=CARTESIAN_POINT ( 'NONE',  ( -11.60004869885203682, 1411.254281879943164, 134.0999999980979851 ) ) ;
#33325=CARTESIAN_POINT ( 'NONE',  ( 24.13987143119999956, 1435.346625637479974, 136.7217067365980085 ) ) ;
#33328=CARTESIAN_POINT ( 'NONE',  ( -0.3622025830936350110, 1416.825783990419950, 191.0664212414500014 ) ) ;
#33329=CARTESIAN_POINT ( 'NONE',  ( -13.04207679966010147, 1409.368499744919745, 225.9431846064669855 ) ) ;
#33336=CARTESIAN_POINT ( 'NONE',  ( -28.01911545699999806, 1442.727873585590032, 231.7019063253979994 ) ) ;
#33338=CARTESIAN_POINT ( 'NONE',  ( -11.07594373419999911, 1433.015750972510205, 151.6980226098980040 ) ) ;
#33340=B_SPLINE_CURVE_WITH_KNOTS ( 'NONE', 4,
 ( #30847, #90756, #89109, #72873, #73973 ),
 .UNSPECIFIED., .F., .F.,
 ( 5, 5 ),
 ( 9.931291899967220616E-17, 0.009483690916888028524 ),
 .UNSPECIFIED. ) ;
#33341=CARTESIAN_POINT ( 'NONE',  ( -2.740720916264808515, 1420.074197278511519, 186.0641697093491302 ) ) ;
#33343=CARTESIAN_POINT ( 'NONE',  ( -24.63975812940000054, 1440.017819941759853, 210.6779373860979945 ) ) ;
#33345=CARTESIAN_POINT ( 'NONE',  ( -2.825023819243769996, 1409.011713080599975, 187.6092914852009983 ) ) ;
#33347=CARTESIAN_POINT ( 'NONE',  ( -20.55130959458017870, 1509.748513648901735, 230.9769706060577903 ) ) ;
#33348=CARTESIAN_POINT ( 'NONE',  ( -2.407902493171400187E-09, 1415.709304463629906, 241.9018706941139669 ) ) ;
#33349=VERTEX_POINT ( 'NONE', #11568 ) ;
#33351=CARTESIAN_POINT ( 'NONE',  ( -11.80969502400810001, 1428.721338179349914, 148.6497889493599871 ) ) ;
#33353=CARTESIAN_POINT ( 'NONE',  ( -4.832500121020000705, 1471.592195475830067, 269.8673040278980011 ) ) ;
#33354=CARTESIAN_POINT ( 'NONE',  ( 11.89349302229567407, 1433.282476700868756, 147.6489928588556779 ) ) ;
#33355=( BOUNDED_CURVE ( )  B_SPLINE_CURVE ( 3, ( #66613, #66060, #67155, #30770 ),
 .UNSPECIFIED., .F., .F. ) 
 B_SPLINE_CURVE_WITH_KNOTS ( ( 4, 4 ),
 ( 4.177898400101880405, 5.246901559513639235 ),
 .UNSPECIFIED. ) 
 CURVE ( )  GEOMETRIC_REPRESENTATION_ITEM ( )  RATIONAL_B_SPLINE_CURVE ( ( 1.000000000000000000, 0.9070150916865978852, 0.9070150916865978852, 1.000000000000000000 ) ) 
 REPRESENTATION_ITEM ( '' )  );
#33358=CARTESIAN_POINT ( 'NONE',  ( 20.55257633559999775, 1497.713060387329961, 201.0220267247279935 ) ) ;
#33361=CARTESIAN_POINT ( 'NONE',  ( -14.59882275880000080, 1475.513060387329915, 194.5230232033979973 ) ) ;
#33364=CARTESIAN_POINT ( 'NONE',  ( -18.68320425524010275, 1409.179517572200211, 269.1629733292540436 ) ) ;
#33365=CARTESIAN_POINT ( 'NONE',  ( -13.25378446100000041, 1435.222382017790096, 150.0797423395979990 ) ) ;
#33370=CARTESIAN_POINT ( 'NONE',  ( -21.98270307515648270, 1506.436298853318931, 209.4394080128124074 ) ) ;
#33373=CARTESIAN_POINT ( 'NONE',  ( -17.93127365029999964, 1485.487435208230181, 188.8314909439980056 ) ) ;
#33378=CARTESIAN_POINT ( 'NONE',  ( -29.21606572689999837, 1509.871156552030016, 208.2743117722099839 ) ) ;
#33379=CARTESIAN_POINT ( 'NONE',  ( 8.598096571001718758, 1427.995879741943554, 134.0999999980979567 ) ) ;
#33381=CARTESIAN_POINT ( 'NONE',  ( -5.257351103029999528, 1408.563318624929934, 196.5782129565980085 ) ) ;
#33383=CARTESIAN_POINT ( 'NONE',  ( -38.48250450509210197, 1443.291876352919871, 137.1415221903179997 ) ) ;
#33385=CARTESIAN_POINT ( 'NONE',  ( -27.45150841124540264, 1488.737809751009991, 209.5843002502519994 ) ) ;
#33386=CARTESIAN_POINT ( 'NONE',  ( 26.53391208749999919, 1488.685287627230082, 213.4463815460780154 ) ) ;
#33390=CARTESIAN_POINT ( 'NONE',  ( 0.1595995995380000143, 1486.508831850330125, 181.8147405652979671 ) ) ;
#33393=CARTESIAN_POINT ( 'NONE',  ( -2.418881086572150174, 1484.257535334039858, 183.1979755142290003 ) ) ;
#33396=CARTESIAN_POINT ( 'NONE',  ( 11.33192158579999820, 1414.988017870030035, 222.3303153933979956 ) ) ;
#33404=CARTESIAN_POINT ( 'NONE',  ( 12.97215231279360026, 1434.791734578659998, 149.5093031009719766 ) ) ;
#33405=CARTESIAN_POINT ( 'NONE',  ( 17.80303567514379992, 1459.309267358430134, 228.1638295836210375 ) ) ;
#33407=CARTESIAN_POINT ( 'NONE',  ( 2.446787376320000096, 1432.353341358199941, 150.2884730787980061 ) ) ;
#33410=CARTESIAN_POINT ( 'NONE',  ( -15.10371725490000117, 1409.440493816029857, 225.2902966875980155 ) ) ;
#33413=CARTESIAN_POINT ( 'NONE',  ( 20.15452299509999889, 1507.845791384329914, 189.3412703934979788 ) ) ;
#33415=ORIENTED_EDGE ( 'NONE', *, *, #76082, .T. ) ;
#33419=CARTESIAN_POINT ( 'NONE',  ( 1.196415586119999874, 1420.167066172730074, 184.5944197207980153 ) ) ;
#33422=CARTESIAN_POINT ( 'NONE',  ( 1273.316865285499944, 2833.596074015639715, 9977.675558181130327 ) ) ;
#33426=CARTESIAN_POINT ( 'NONE',  ( 18.06510344782403621, 1424.836155016811063, 224.7141253419370344 ) ) ;
#33427=CARTESIAN_POINT ( 'NONE',  ( 11.84242369139999873, 1431.324257919750153, 147.6543138610979895 ) ) ;
#33428=CARTESIAN_POINT ( 'NONE',  ( -7.419509149259999603, 1440.444625599219989, 149.7273825585979807 ) ) ;
#33429=CARTESIAN_POINT ( 'NONE',  ( 45.65827091464620224, 1440.913060379439912, 266.1743358949399862 ) ) ;
#33431=CARTESIAN_POINT ( 'NONE',  ( -20.51044083270000229, 1453.146242308330102, 207.5895558364179863 ) ) ;
#33432=CARTESIAN_POINT ( 'NONE',  ( 12.78657892559999887, 1416.813004075630033, 222.2779166417979866 ) ) ;
#33433=ORIENTED_EDGE ( 'NONE', *, *, #41792, .T. ) ;
#33435=CARTESIAN_POINT ( 'NONE',  ( 14.59276606620000116, 1436.244837803880046, 149.8707691859979718 ) ) ;
#33436=CARTESIAN_POINT ( 'NONE',  ( -19.67818152874250259, 1485.241807130695179, 190.3342238627110419 ) ) ;
#33437=AXIS2_PLACEMENT_3D ( 'NONE', #105478, #61848, #19801 ) ;
#33440=CARTESIAN_POINT ( 'NONE',  ( -13.15726448721240160, 1416.851343896870048, 221.9096085506390068 ) ) ;
#33455=CARTESIAN_POINT ( 'NONE',  ( 14.90569475453980175, 1509.413384249990031, 233.7754132121639827 ) ) ;
#33457=CARTESIAN_POINT ( 'NONE',  ( 36.93857276712569870, 1437.876021133649829, 136.5569222567030181 ) ) ;
#33463=CARTESIAN_POINT ( 'NONE',  ( -6.867847813526624101, 1447.894038402013166, 185.5948811633518574 ) ) ;
#33464=CARTESIAN_POINT ( 'NONE',  ( -11.42381040596369246, 1434.696338602614333, 151.4779332080243250 ) ) ;
#33467=CARTESIAN_POINT ( 'NONE',  ( 1.910568182230000023, 1408.979778898429913, 186.9030642623980043 ) ) ;
#33470=CARTESIAN_POINT ( 'NONE',  ( -2.500000000000000000, 1439.162586052440020, 158.2749544336289773 ) ) ;
#33472=CARTESIAN_POINT ( 'NONE',  ( -1.806676058779320027, 1450.408993861640056, 183.0756166235049989 ) ) ;
#33475=CARTESIAN_POINT ( 'NONE',  ( -0.8066080222970000158, 1426.500992774829911, 146.0666368882980066 ) ) ;
#33476=CARTESIAN_POINT ( 'NONE',  ( -2.189515144162804905, 1407.000063894707182, 196.1218408969885161 ) ) ;
#33478=CARTESIAN_POINT ( 'NONE',  ( 16.04953034249999888, 1449.500693692240020, 190.3237195885979816 ) ) ;
#33479=CARTESIAN_POINT ( 'NONE',  ( -4.654638212716369785E-09, 1475.687699392280138, 266.6817061415500234 ) ) ;
#33487=CARTESIAN_POINT ( 'NONE',  ( -46.09936160196500055, 1439.223420885880159, 268.2062399438970033 ) ) ;
#33492=CIRCLE ( 'NONE', #55054, 1.999999999862774658 ) ;
#33493=CARTESIAN_POINT ( 'NONE',  ( 19.29679066396858289, 1456.533063871148443, 224.7183538900586655 ) ) ;
#33495=CARTESIAN_POINT ( 'NONE',  ( -25.98931941724259786, 1450.776361986090023, 136.7278132101320125 ) ) ;
#33497=CARTESIAN_POINT ( 'NONE',  ( 25.86260026499999753, 1439.222596320959838, 221.4996202120980229 ) ) ;
#33504=CARTESIAN_POINT ( 'NONE',  ( -9230.682934426007705, 2837.541834147241843, -5630.801423372711724 ) ) ;
#33506=CARTESIAN_POINT ( 'NONE',  ( -1.847327201898169902, 1408.584742853789976, 270.4287613073750549 ) ) ;
#33507=CARTESIAN_POINT ( 'NONE',  ( 6.270129375719379894, 1418.078661284499958, 232.0014322324400098 ) ) ;
#33511=CARTESIAN_POINT ( 'NONE',  ( -22.82353090123229933, 1409.710023875719799, 209.0053221533019894 ) ) ;
#33512=CARTESIAN_POINT ( 'NONE',  ( -3.696362419970000257, 1424.349081209429869, 185.3675292160980064 ) ) ;
#33515=CARTESIAN_POINT ( 'NONE',  ( -7.214502255410000231, 1427.316505021429975, 144.1938086916980239 ) ) ;
#33516=CARTESIAN_POINT ( 'NONE',  ( -18.89036777432109915, 1416.702560751849887, 207.5747689616710261 ) ) ;
#33517=CARTESIAN_POINT ( 'NONE',  ( -22.55028051829999924, 1415.846227990229863, 213.4522806374379797 ) ) ;
#33519=CARTESIAN_POINT ( 'NONE',  ( 28.57628399200979885, 1468.636142906849955, 267.5038535851290362 ) ) ;
#33520=EDGE_CURVE ( 'NONE', #102192, #42879, #67334, .T. ) ;
#33522=CARTESIAN_POINT ( 'NONE',  ( -16.78273306371495721, 1421.715029943856734, 226.9035938626332438 ) ) ;
#33527=CARTESIAN_POINT ( 'NONE',  ( 22.99329315949999852, 1409.822368751529893, 208.3677801514749888 ) ) ;
#33531=CARTESIAN_POINT ( 'NONE',  ( 26.86339342382879991, 1451.975050932460135, 134.9994894959820044 ) ) ;
#33538=CARTESIAN_POINT ( 'NONE',  ( 1.358157591254900209, 1408.960488295489995, 186.7573064037119934 ) ) ;
#33542=CARTESIAN_POINT ( 'NONE',  ( 1.099392875928770108, 1450.807449935850173, 181.4766395928249949 ) ) ;
#33543=B_SPLINE_CURVE_WITH_KNOTS ( 'NONE', 5,
 ( #94742, #27546, #2380, #51651, #162, #102569 ),
 .UNSPECIFIED., .F., .F.,
 ( 6, 6 ),
 ( -2.000000000000000000, 0.000000000000000000 ),
 .UNSPECIFIED. ) ;
#33546=ORIENTED_EDGE ( 'NONE', *, *, #106146, .F. ) ;
#33547=CARTESIAN_POINT ( 'NONE',  ( 11.48654377539569893, 1414.913057860449953, 220.8288015276069984 ) ) ;
#33548=CARTESIAN_POINT ( 'NONE',  ( 11.72314628525600000, 1432.337468529400212, 150.7717701949150069 ) ) ;
#33549=VECTOR ( 'NONE', #14066, 1000.000000000000114 ) ;
#33551=TOROIDAL_SURFACE ( 'NONE', #74756, 7.016581249619999738, 2.000000000000000000 ) ;
#33553=EDGE_CURVE ( 'NONE', #94371, #18109, #71327, .T. ) ;
#33557=CARTESIAN_POINT ( 'NONE',  ( -1.636503137890000126, 1433.447543843880112, 150.4001344053979778 ) ) ;
#33558=B_SPLINE_CURVE_WITH_KNOTS ( 'NONE', 5,
 ( #45029, #80812, #35489, #37156, #103805, #10283, #71349, #10857, #44460, #79175, #36598, #27646, #61833, #2482, #28753 ),
 .UNSPECIFIED., .F., .F.,
 ( 6, 3, 3, 3, 6 ),
 ( 0.000000000000000000, 0.3169994908698778313, 0.4228046033745412324, 0.6719997599498082064, 1.000000000000000000 ),
 .UNSPECIFIED. ) ;
#33559=CARTESIAN_POINT ( 'NONE',  ( -21.33887670626219801, 1508.922069394937125, 191.9015789802110703 ) ) ;
#33560=CARTESIAN_POINT ( 'NONE',  ( 11.87929288849999843, 1433.122288330840092, 150.0887009630980060 ) ) ;
#33561=CARTESIAN_POINT ( 'NONE',  ( 6.215408291410000174, 1454.402584563930077, 214.3676144197379756 ) ) ;
#33562=CARTESIAN_POINT ( 'NONE',  ( 12.02797161417169924, 1415.088136167450102, 197.1259520390879914 ) ) ;
#33568=FACE_OUTER_BOUND ( 'NONE', #52891, .T. ) ;
#33570=CARTESIAN_POINT ( 'NONE',  ( 0.04886115394894129799, 1508.952074335740008, 238.8419220553400351 ) ) ;
#33572=CARTESIAN_POINT ( 'NONE',  ( 23.67770893690000023, 1410.915352766729939, 211.2317889356880016 ) ) ;
#33574=CARTESIAN_POINT ( 'NONE',  ( -34.93121270820218172, 1435.717331548646598, 135.0378024103818575 ) ) ;
#33580=CARTESIAN_POINT ( 'NONE',  ( 0.1926304896301150038, 1467.201837219709887, 182.6439754155339870 ) ) ;
#33583=CARTESIAN_POINT ( 'NONE',  ( -25.00312495901935250, 1451.477102942365264, 137.4959198732346408 ) ) ;
#33584=CARTESIAN_POINT ( 'NONE',  ( -34.00767267269074523, 1443.913060387329324, 154.9192896682974663 ) ) ;
#33585=CARTESIAN_POINT ( 'NONE',  ( 11.87507418750000099, 1433.007222232190088, 149.7888126920979914 ) ) ;
#33586=CARTESIAN_POINT ( 'NONE',  ( -41.65030538158350026, 1443.228731900419916, 134.0999999981379744 ) ) ;
#33587=CARTESIAN_POINT ( 'NONE',  ( -34.35673827249829770, 1445.503283575680143, 137.0830489703820092 ) ) ;
#33588=ORIENTED_EDGE ( 'NONE', *, *, #29773, .T. ) ;
#33591=CARTESIAN_POINT ( 'NONE',  ( -17.36177561119999879, 1416.518532928330160, 214.4540685280980199 ) ) ;
#33597=CARTESIAN_POINT ( 'NONE',  ( 7.926558117193340358, 1409.189861896230013, 221.8168932242559777 ) ) ;
#33603=CARTESIAN_POINT ( 'NONE',  ( -33.91369268630000278, 1451.728774195029928, 134.7155787906980038 ) ) ;
#33604=CARTESIAN_POINT ( 'NONE',  ( 12.73318793669440829, 1442.831169986190389, 164.6858276811441328 ) ) ;
#33605=CARTESIAN_POINT ( 'NONE',  ( 2.370970874524633398, 1427.002265528473799, 134.0999999980980135 ) ) ;
#33608=CARTESIAN_POINT ( 'NONE',  ( -17.38483621660000011, 1410.884422118429939, 225.7833436061980024 ) ) ;
#33611=CARTESIAN_POINT ( 'NONE',  ( 37.99560157342931177, 1453.980171722192608, 269.5760773822823921 ) ) ;
#33613=CARTESIAN_POINT ( 'NONE',  ( 17.49699257007802089, 1434.033957849185526, 216.2913140874469775 ) ) ;
#33615=CARTESIAN_POINT ( 'NONE',  ( 2.500000000000039968, 1439.615672328189930, 182.7715275322960053 ) ) ;
#33617=CARTESIAN_POINT ( 'NONE',  ( 11.89850863680000082, 1497.713060387329961, 228.0402318450979919 ) ) ;
#33618=AXIS2_PLACEMENT_3D ( 'NONE', #7552, #31644, #107807 ) ;
#33623=CARTESIAN_POINT ( 'NONE',  ( 2.500000000000000000, 1448.831169023560051, 156.2564136193980175 ) ) ;
#33625=CARTESIAN_POINT ( 'NONE',  ( 1.121218327409999826, 1416.837080243330092, 190.1583373011980029 ) ) ;
#33626=CARTESIAN_POINT ( 'NONE',  ( 14.00886214219999992, 1416.826388498530150, 196.3918802162980057 ) ) ;
#33630=CARTESIAN_POINT ( 'NONE',  ( 40.60394929974220446, 1444.189591584570053, 137.0481280076579935 ) ) ;
#33631=VERTEX_POINT ( 'NONE', #88157 ) ;
#33634=CARTESIAN_POINT ( 'NONE',  ( -25.48925201569999999, 1449.802587361850101, 207.5067252115079839 ) ) ;
#33635=CARTESIAN_POINT ( 'NONE',  ( -10.23174647188330155, 1425.154542701060109, 108.4581586724669933 ) ) ;
#33636=CARTESIAN_POINT ( 'NONE',  ( 16.41296274929999655, 1409.863099034130073, 192.1158788459979974 ) ) ;
#33639=EDGE_CURVE ( 'NONE', #46740, #88970, #79209, .T. ) ;
#33640=CARTESIAN_POINT ( 'NONE',  ( -18.95884613770000016, 1416.837177098929942, 207.7798960437979758 ) ) ;
#33641=CARTESIAN_POINT ( 'NONE',  ( -10.81506866279999990, 1424.921186100929845, 144.1620444789979842 ) ) ;
#33642=CARTESIAN_POINT ( 'NONE',  ( 19.12646062745870168, 1509.604355955109895, 231.7508453187430177 ) ) ;
#33643=CARTESIAN_POINT ( 'NONE',  ( 10.30873441802069657, 1464.609330832652631, 232.2540526936852814 ) ) ;
#33647=CARTESIAN_POINT ( 'NONE',  ( -35.20867138851480149, 1437.188504188790148, 136.5366439520919926 ) ) ;
#33648=ORIENTED_EDGE ( 'NONE', *, *, #90466, .T. ) ;
#33649=CARTESIAN_POINT ( 'NONE',  ( 9.759055691533209398, 1396.253854122790017, 215.8358679858959874 ) ) ;
#33651=CARTESIAN_POINT ( 'NONE',  ( -18.51931868289999983, 1457.242090721130126, 228.6951897570979781 ) ) ;
#33652=ORIENTED_EDGE ( 'NONE', *, *, #2147, .T. ) ;
#33653=ORIENTED_EDGE ( 'NONE', *, *, #98518, .F. ) ;
#33655=CARTESIAN_POINT ( 'NONE',  ( -9.400735546954820165, 1432.346475316169972, 153.1462981359680100 ) ) ;
#33658=DIRECTION ( 'NONE',  ( -0.3363363969979655810, -0.9417419115949056119, 0.000000000000000000 ) ) ;
#33662=CARTESIAN_POINT ( 'NONE',  ( -13.64528653743296793, 1409.389564293140211, 225.5043415784803926 ) ) ;
#33667=CARTESIAN_POINT ( 'NONE',  ( 37.71876581398180406, 1442.773887286369245, 136.8568823567051709 ) ) ;
#33672=ORIENTED_EDGE ( 'NONE', *, *, #94644, .T. ) ;
#33673=CARTESIAN_POINT ( 'NONE',  ( 11.75441003104140059, 1426.806845251099958, 145.3811685653730024 ) ) ;
#33674=EDGE_CURVE ( 'NONE', #73741, #55526, #7404, .T. ) ;
#33677=CARTESIAN_POINT ( 'NONE',  ( -13.53550618839999942, 1416.067629290630066, 221.7501982114980308 ) ) ;
#33678=CARTESIAN_POINT ( 'NONE',  ( -12.73318793669440829, 1442.831169986190389, 164.6858276811441328 ) ) ;
#33681=CARTESIAN_POINT ( 'NONE',  ( -13.53916864039999979, 1429.119334014829747, 222.2883575813980030 ) ) ;
#33682=CARTESIAN_POINT ( 'NONE',  ( 14.44257447436980080, 1436.255103877649844, 149.9682557532709950 ) ) ;
#33684=CARTESIAN_POINT ( 'NONE',  ( 5.389719913101400195, 1440.971386073809981, 154.8246291173960003 ) ) ;
#33686=CARTESIAN_POINT ( 'NONE',  ( -15.37779627350000133, 1473.856793900130015, 223.6695348900979923 ) ) ;
#33691=CARTESIAN_POINT ( 'NONE',  ( -2.499950939289320218, 1420.110720408840052, 91.61080890135978905 ) ) ;
#33694=CARTESIAN_POINT ( 'NONE',  ( -1.266603054566116215, 1486.256723992427851, 181.7971939238652226 ) ) ;
#33697=CARTESIAN_POINT ( 'NONE',  ( -2.995264515017130424, 1485.700673117452425, 182.6181475772214924 ) ) ;
#33700=EDGE_LOOP ( 'NONE', ( #58897, #69510, #28145, #34633, #23095, #105008 ) ) ;
#33701=CARTESIAN_POINT ( 'NONE',  ( 0.9093771269469999030, 1453.154616238429981, 188.6184110473980127 ) ) ;
#33703=CARTESIAN_POINT ( 'NONE',  ( -11.74266240329999889, 1430.299105537730156, 150.4823647192980047 ) ) ;
#33705=FACE_OUTER_BOUND ( 'NONE', #364, .T. ) ;
#33706=EDGE_CURVE ( 'NONE', #61502, #10270, #4613, .T. ) ;
#33711=CARTESIAN_POINT ( 'NONE',  ( -26.30611563449999935, 1495.365312711930073, 211.9622044710779960 ) ) ;
#33717=CARTESIAN_POINT ( 'NONE',  ( 35.90626991010000069, 1418.667692805230217, 268.5344559059980156 ) ) ;
#33719=EDGE_CURVE ( 'NONE', #8175, #94093, #60590, .T. ) ;
#33720=CARTESIAN_POINT ( 'NONE',  ( 24.93912320480000133, 1469.150327946329753, 204.6358346344680115 ) ) ;
#33722=CARTESIAN_POINT ( 'NONE',  ( -0.02424329741014210129, 1507.629757353219702, 237.3744802823229918 ) ) ;
#33725=CARTESIAN_POINT ( 'NONE',  ( -18.61729373446216584, 1457.059787195335730, 228.1786572006384972 ) ) ;
#33727=CARTESIAN_POINT ( 'NONE',  ( -12.65996588039999970, 1445.259821888419992, 186.8996239715980039 ) ) ;
#33730=CARTESIAN_POINT ( 'NONE',  ( 8.322172261349999545, 1408.217606231929949, 270.1222559176979416 ) ) ;
#33731=CARTESIAN_POINT ( 'NONE',  ( 1.462200250809050139, 1493.817013747780038, 181.6932468947250072 ) ) ;
#33735=CARTESIAN_POINT ( 'NONE',  ( -18.31336108710000232, 1473.001052085330002, 268.9136774873980471 ) ) ;
#33738=CARTESIAN_POINT ( 'NONE',  ( -20.99625264690000392, 1509.712722401030078, 187.9206951049980034 ) ) ;
#33739=CARTESIAN_POINT ( 'NONE',  ( -24.36918344492354649, 1444.649591787489271, 211.1821244689920434 ) ) ;
#33742=CARTESIAN_POINT ( 'NONE',  ( -9.587366264599999965, 1440.450814879359996, 153.1449006345979740 ) ) ;
#33744=CARTESIAN_POINT ( 'NONE',  ( -25.17882212385940122, 1457.411782445480185, 210.8729951149459794 ) ) ;
#33747=CARTESIAN_POINT ( 'NONE',  ( -23.65074497499999850, 1410.660584268429830, 206.9527459116580133 ) ) ;
#33749=B_SPLINE_CURVE_WITH_KNOTS ( 'NONE', 3,
 ( #27822, #69850, #53038, #53599, #17724, #105080, #96121 ),
 .UNSPECIFIED., .F., .F.,
 ( 4, 3, 4 ),
 ( -157.7844419379999863, -101.5362237811699941, -30.93609007946849943 ),
 .UNSPECIFIED. ) ;
#33751=CARTESIAN_POINT ( 'NONE',  ( -31.11217220549999851, 1415.581976973229757, 269.3348318802979975 ) ) ;
#33752=PLANE ( 'NONE',  #37396 ) ;
#33755=LINE ( 'NONE', #102061, #105421 ) ;
#33756=CARTESIAN_POINT ( 'NONE',  ( -22.15124423910000218, 1409.851346931930038, 211.3136525823379941 ) ) ;
#33757=CARTESIAN_POINT ( 'NONE',  ( 13.89764133033322580, 1452.801221801048314, 223.6909718731195085 ) ) ;
#33758=CARTESIAN_POINT ( 'NONE',  ( 11.72168562826050042, 1426.705748779369969, 143.0708505248780114 ) ) ;
#33762=CARTESIAN_POINT ( 'NONE',  ( -11.36018337610000195, 1414.996442546130083, 195.9645814914979951 ) ) ;
#33763=ADVANCED_FACE ( 'NONE', ( #48358 ), #100037, .T. ) ;
#33766=B_SPLINE_CURVE_WITH_KNOTS ( 'NONE', 3,
 ( #23236, #57434, #91560, #89352, #46824, #50661, #68038, #6996, #41154, #59079, #75863, #51211, #84253, #93199, #75329, #66929 ),
 .UNSPECIFIED., .F., .F.,
 ( 4, 3, 3, 3, 3, 4 ),
 ( -6.921060107978769693, -6.805780737513280165, -5.885806138044639368, -4.993439783500069673, -4.118990261660390395, -3.271583732334530037 ),
 .UNSPECIFIED. ) ;
#33770=CARTESIAN_POINT ( 'NONE',  ( 2.716629276539999971, 1509.007927172130167, 238.2585658352980147 ) ) ;
#33771=CARTESIAN_POINT ( 'NONE',  ( 20.00300088520139852, 1507.847439178179911, 229.0979933904550023 ) ) ;
#33774=VERTEX_POINT ( 'NONE', #71242 ) ;
#33776=CARTESIAN_POINT ( 'NONE',  ( 12.02944668659279870, 1433.769975373530087, 150.0279833908939793 ) ) ;
#33777=CARTESIAN_POINT ( 'NONE',  ( -7.331557526720001050, 1396.349310000530068, 219.0774438792280137 ) ) ;
#33783=CARTESIAN_POINT ( 'NONE',  ( -14.28944875984979923, 1509.439638412510021, 183.0899159983670188 ) ) ;
#33784=CARTESIAN_POINT ( 'NONE',  ( 15.61733546277139872, 1498.109274936660086, 231.4603964206870330 ) ) ;
#33786=EDGE_CURVE ( 'NONE', #52697, #90692, #56399, .T. ) ;
#33787=CARTESIAN_POINT ( 'NONE',  ( 2.585682588340000088, 1449.237988204799876, 183.8872507908980083 ) ) ;
#33790=B_SPLINE_SURFACE_WITH_KNOTS ( 'NONE', 5, 5, ( 
 ( #106548, #4643, #29836, #40435, #47748, #89196 ),
 ( #89743, #56145, #64022, #22501, #107650, #106012 ),
 ( #98135, #65661, #14682, #14123, #65111, #13016 ),
 ( #12488, #47202, #38781, #107094, #56702, #30383 ),
 ( #64574, #108190, #21952, #90281, #48870, #82996 ),
 ( #81883, #5186, #90838, #48312, #82454, #39893 ) ),
 .UNSPECIFIED., .F., .F., .F.,
 ( 6, 6 ),
 ( 6, 6 ),
 ( 3.723869972580000187, 4.458425423349980043 ),
 ( 0.000000000000000000, 2.000000000000000000 ),
 .UNSPECIFIED. ) ;
#33791=CARTESIAN_POINT ( 'NONE',  ( 4.073985546776730082, 1396.055327098900079, 198.8729011744260049 ) ) ;
#33792=CARTESIAN_POINT ( 'NONE',  ( 1.362314668290000030, 1416.021639799829927, 190.3543332225980009 ) ) ;
#33793=CARTESIAN_POINT ( 'NONE',  ( 10.96595508919999951, 1432.092997362309916, 151.7666336219979826 ) ) ;
#33795=VERTEX_POINT ( 'NONE', #3475 ) ;
#33796=CARTESIAN_POINT ( 'NONE',  ( 13.45603295267449973, 1435.141892408729973, 149.7441957230019796 ) ) ;
#33800=CARTESIAN_POINT ( 'NONE',  ( 13.11924748619371783, 1444.785942371835063, 169.4030629633686829 ) ) ;
#33801=CARTESIAN_POINT ( 'NONE',  ( -12.69622108839999974, 1461.420101681630058, 231.9855631372980156 ) ) ;
#33802=CARTESIAN_POINT ( 'NONE',  ( -13.31488284758549945, 1407.448340439549838, 207.9555150571470108 ) ) ;
#33805=B_SPLINE_SURFACE_WITH_KNOTS ( 'NONE', 5, 5, ( 
 ( #478, #34602, #60373, #94496, #17767, #51971 ),
 ( #5128, #39284, #73459, #69338, #1031, #27308 ),
 ( #28978, #88328, #44683, #61489, #104012, #96173 ),
 ( #95618, #103446, #78828, #2140, #35154, #26752 ),
 ( #97267, #60940, #19448, #87221, #20543, #79379 ),
 ( #28421, #87790, #18885, #2695, #18336, #86112 ) ),
 .UNSPECIFIED., .F., .F., .F.,
 ( 6, 6 ),
 ( 6, 6 ),
 ( 8.897216823040000833, 11.87860904800000128 ),
 ( 0.000000000000000000, 1.460858415939999988 ),
 .UNSPECIFIED. ) ;
#33808=DIRECTION ( 'NONE',  ( 0.9417419115949662300, -0.2378257470769920556, 0.2378257470769920556 ) ) ;
#33813=CARTESIAN_POINT ( 'NONE',  ( 20.69345393905350150, 1440.913060387330006, 220.6334537215260241 ) ) ;
#33814=CARTESIAN_POINT ( 'NONE',  ( -19.28053373810000082, 1508.539880042930236, 229.7797826120979892 ) ) ;
#33816=CARTESIAN_POINT ( 'NONE',  ( -7.164186635890001043, 1409.330595797830028, 188.0408233170979884 ) ) ;
#33819=ADVANCED_FACE ( 'NONE', ( #94455 ), #58063, .F. ) ;
#33820=CARTESIAN_POINT ( 'NONE',  ( -0.3106767230313050021, 1415.088506334920112, 226.1862806902549892 ) ) ;
#33822=CARTESIAN_POINT ( 'NONE',  ( 24.54570628209999938, 1439.590004835240052, 212.8530392935280133 ) ) ;
#33828=AXIS2_PLACEMENT_3D ( 'NONE', #20339, #53425, #78048 ) ;
#33829=B_SPLINE_SURFACE_WITH_KNOTS ( 'NONE', 5, 5, ( 
 ( #60245, #27188, #35577, #69770, #95490, #94363 ),
 ( #19872, #51846, #103888, #18758, #78694, #36145 ),
 ( #35024, #69203, #103312, #70329, #27733, #61923 ),
 ( #21511, #107197, #37246, #106637, #45673, #46770 ),
 ( #64119, #97148, #46219, #28847, #81980, #72508 ),
 ( #80353, #55170, #5289, #54622, #20416, #73056 ),
 ( #90379, #89841, #13114, #54077, #98240, #106099 ),
 ( #22053, #37797, #107749, #55723, #98792, #30485 ),
 ( #29927, #99327, #47297, #47847, #31033, #64674 ),
 ( #79811, #39446, #88754, #11498, #81421, #65215 ),
 ( #73620, #56250, #12037, #38329, #80900, #20966 ),
 ( #88203, #3670, #71986, #13657, #29377, #3117 ) ),
 .UNSPECIFIED., .F., .F., .F.,
 ( 6, 3, 3, 6 ),
 ( 6, 6 ),
 ( -1.028409222517709891E-05, 6.405353355340000832, 10.57568960840000116, 14.18574420394130087 ),
 ( -1.028409222599429936E-05, 1.510873114410000051 ),
 .UNSPECIFIED. ) ;
#33833=CARTESIAN_POINT ( 'NONE',  ( -21.33073281829999956, 1509.431426448229786, 190.3502236029979997 ) ) ;
#33834=LINE ( 'NONE', #15368, #33275 ) ;
#33836=CARTESIAN_POINT ( 'NONE',  ( 42.15865170690000241, 1431.016965136909903, 271.1218459616979999 ) ) ;
#33838=CARTESIAN_POINT ( 'NONE',  ( 20.81306254364009689, 1578.884139734249857, 255.0940092270310231 ) ) ;
#33842=CARTESIAN_POINT ( 'NONE',  ( 19.16281588599999708, 1470.534656580030060, 262.3397497982979871 ) ) ;
#33843=CARTESIAN_POINT ( 'NONE',  ( -28.63327877612760020, 1509.912956515240012, 215.5831518558169932 ) ) ;
#33844=CARTESIAN_POINT ( 'NONE',  ( -4.045189757455589508, 1509.066000099900066, 238.3989657214699776 ) ) ;
#33849=CARTESIAN_POINT ( 'NONE',  ( 17.98629411888249763, 1410.716562210689972, 222.9725041732099839 ) ) ;
#33855=EDGE_CURVE ( 'NONE', #67278, #102730, #61866, .T. ) ;
#33857=CARTESIAN_POINT ( 'NONE',  ( 12.27023112350000211, 1416.839692139429872, 223.5796784320980066 ) ) ;
#33861=CARTESIAN_POINT ( 'NONE',  ( 8.510016363196779565, 1417.253316583138258, 230.6448116059823121 ) ) ;
#33862=CARTESIAN_POINT ( 'NONE',  ( 32.66530384042000179, 1436.114947058330017, 136.3376366257210179 ) ) ;
#33864=CARTESIAN_POINT ( 'NONE',  ( -42.02418941567508881, 1454.249290662224666, 269.0750561195100090 ) ) ;
#33866=FACE_OUTER_BOUND ( 'NONE', #79953, .T. ) ;
#33869=B_SPLINE_CURVE_WITH_KNOTS ( 'NONE', 5,
 ( #26222, #52561, #7774, #9437, #102383, #27337, #25665, #69373, #43052 ),
 .UNSPECIFIED., .F., .F.,
 ( 6, 3, 6 ),
 ( 0.000000000000000000, 0.4999964781214675247, 1.000000000000000000 ),
 .UNSPECIFIED. ) ;
#33870=ORIENTED_EDGE ( 'NONE', *, *, #71271, .T. ) ;
#33874=CARTESIAN_POINT ( 'NONE',  ( 14.30089278887709980, 1424.546528003230151, 190.6949013431569995 ) ) ;
#33875=CARTESIAN_POINT ( 'NONE',  ( 10.86613173150421296, 1424.804654287561107, 138.2012213579507147 ) ) ;
#33878=CARTESIAN_POINT ( 'NONE',  ( -29.78452513100000232, 1510.001069743030257, 209.1046444409799960 ) ) ;
#33881=CARTESIAN_POINT ( 'NONE',  ( 44.43455570398290178, 1440.913041958179974, 270.0922447040700263 ) ) ;
#33882=CARTESIAN_POINT ( 'NONE',  ( -16.06427069504690053, 1414.913060387399810, 209.3174525065670082 ) ) ;
#33883=CARTESIAN_POINT ( 'NONE',  ( 25.88156921539999900, 1436.664060738580019, 136.9978706268979920 ) ) ;
#33884=CARTESIAN_POINT ( 'NONE',  ( -7.489155007101369499, 1396.174587443169912, 200.9962419971890313 ) ) ;
#33885=VERTEX_POINT ( 'NONE', #24371 ) ;
#33887=CARTESIAN_POINT ( 'NONE',  ( 21.53951928259277082, 1509.203566000515593, 226.5093279692427188 ) ) ;
#33888=ORIENTED_EDGE ( 'NONE', *, *, #102706, .T. ) ;
#33892=CARTESIAN_POINT ( 'NONE',  ( 11.03772332119999966, 1426.504772946829917, 93.46069203369791012 ) ) ;
#33893=CARTESIAN_POINT ( 'NONE',  ( -27.31923407390000236, 1446.350545702490081, 231.7128707201979978 ) ) ;
#33895=CARTESIAN_POINT ( 'NONE',  ( 4.161911742251380275, 1424.201536654089978, 184.5072953679090233 ) ) ;
#33897=VECTOR ( 'NONE', #65311, 1000.000000000000114 ) ;
#33898=CARTESIAN_POINT ( 'NONE',  ( -2.807571324851497963, 1419.859960676956007, 186.1401237969660656 ) ) ;
#33900=CARTESIAN_POINT ( 'NONE',  ( -24.28401183249999917, 1438.913208742730149, 212.0820208524479824 ) ) ;
#33904=CARTESIAN_POINT ( 'NONE',  ( -28.64971979848531802, 1510.024744496989797, 218.0290981197058215 ) ) ;
#33908=CARTESIAN_POINT ( 'NONE',  ( -11.82581238847500060, 1429.643984554019880, 149.2867293954069794 ) ) ;
#33910=CARTESIAN_POINT ( 'NONE',  ( 8.881784196999999612E-15, 1434.913060387330006, 126.8032249175980155 ) ) ;
#33911=CARTESIAN_POINT ( 'NONE',  ( -0.4742355963789999795, 1472.045055685530087, 270.0713874948980333 ) ) ;
#33914=AXIS2_PLACEMENT_3D ( 'NONE', #73016, #30446, #79347 ) ;
#33915=FACE_OUTER_BOUND ( 'NONE', #40458, .T. ) ;
#33918=CARTESIAN_POINT ( 'NONE',  ( -23.56404405089999798, 1519.913060387329779, 208.1422009162390054 ) ) ;
#33921=CARTESIAN_POINT ( 'NONE',  ( -23.91557117702000212, 1411.440207489660224, 269.2971849165700178 ) ) ;
#33922=CARTESIAN_POINT ( 'NONE',  ( -13.66262475276990074, 1434.970346796020067, 148.6600349200319897 ) ) ;
#33925=CARTESIAN_POINT ( 'NONE',  ( 13.50156143719999946, 1443.545633684710083, 188.4056194818979861 ) ) ;
#33926=B_SPLINE_SURFACE_WITH_KNOTS ( 'NONE', 5, 1, ( 
 ( #11974, #45051 ),
 ( #45603, #46155 ),
 ( #37178, #2501 ),
 ( #98724, #36622 ),
 ( #63517, #64605 ),
 ( #54559, #105486 ),
 ( #104932, #96534 ),
 ( #28219, #97633 ),
 ( #80285, #107126 ),
 ( #20354, #64052 ),
 ( #30418, #98171 ),
 ( #62406, #21985 ),
 ( #106579, #47233 ),
 ( #19808, #54014 ),
 ( #21442, #81360 ),
 ( #80831, #88144 ),
 ( #55652, #71928 ),
 ( #79745, #3052 ),
 ( #4674, #89775 ),
 ( #20901, #71374 ),
 ( #28777, #38812 ) ),
 .UNSPECIFIED., .F., .F., .F.,
 ( 6, 3, 3, 3, 3, 3, 6 ),
 ( 2, 2 ),
 ( 122.5058924469999937, 122.5666549750000058, 128.3589772969999956, 134.1528038509999874, 139.9378092970000012, 146.0761118390000206, 146.2671766279999872 ),
 ( 0.000000000000000000, 4.092150885356249823 ),
 .UNSPECIFIED. ) ;
#33927=VERTEX_POINT ( 'NONE', #91030 ) ;
#33932=CARTESIAN_POINT ( 'NONE',  ( -4.702036906180000031, 1485.478603201629994, 183.4821513001980122 ) ) ;
#33934=B_SPLINE_SURFACE_WITH_KNOTS ( 'NONE', 5, 5, ( 
 ( #18551, #25847, #104238, #61712, #7963, #93605 ),
 ( #42130, #60049, #43240, #20757, #88549, #46556 ),
 ( #71785, #87445, #105904, #79060, #28633, #29183 ),
 ( #104790, #2364, #65419, #71220, #79605, #105344 ),
 ( #11295, #62838, #63374, #97490, #89083, #4002 ),
 ( #54956, #62264, #31785, #2909, #65976, #96951 ),
 ( #31236, #48615, #53304, #45463, #99526, #19101 ),
 ( #37027, #28076, #12370, #10740, #88012, #36478 ),
 ( #38128, #22811, #80692, #20217, #54416, #11833 ),
 ( #57018, #46004, #70676, #80135, #72309, #96393 ),
 ( #19669, #106441, #91143, #3454, #37582, #44913 ),
 ( #14420, #82747, #6039, #40191, #53874, #74373 ) ),
 .UNSPECIFIED., .F., .F., .F.,
 ( 6, 3, 3, 6 ),
 ( 6, 6 ),
 ( -1.511236047250149958E-08, 21.98079552259999758, 65.92107459599999686, 113.3791245040000035 ),
 ( -2.177276631571330257E-05, 0.4689188558010000119 ),
 .UNSPECIFIED. ) ;
#33938=EDGE_CURVE ( 'NONE', #68673, #106239, #41378, .T. ) ;
#33940=B_SPLINE_CURVE_WITH_KNOTS ( 'NONE', 3,
 ( #79987, #106825, #72700, #105754, #81078, #65409, #90577, #37437, #22247, #55906, #89485, #57005, #54799, #12217, #12780, #4395, #3859, #11677, #21701, #99515, #45854, #29039, #97330, #13857, #63224, #73806, #22800, #30114, #38522, #80544, #20600, #106286, #98429, #46412, #29571, #90024, #39062 ),
 .UNSPECIFIED., .F., .F.,
 ( 4, 3, 3, 3, 3, 3, 3, 3, 3, 3, 3, 3, 4 ),
 ( -67.60074812010000755, -65.74721505525899090, -64.06766111199499392, -62.52389936639999490, -62.11498414264809753, -60.91890502392639917, -59.67710013614709652, -58.39611896704169425, -57.02019216725560113, -55.62461436954049532, -54.01815956887700310, -52.05859542260679973, -50.07766623440000586 ),
 .UNSPECIFIED. ) ;
#33941=CARTESIAN_POINT ( 'NONE',  ( -28.99152844629999848, 1509.869562750330033, 206.5812832654980014 ) ) ;
#33944=DIRECTION ( 'NONE',  ( -1.000000000000000000, 0.000000000000000000, 0.000000000000000000 ) ) ;
#33946=CARTESIAN_POINT ( 'NONE',  ( -3.872760563090000385, 1407.067887183629864, 196.6093298303979964 ) ) ;
#33951=CARTESIAN_POINT ( 'NONE',  ( -27.12610615285149862, 1488.751143559889897, 210.2942340960309764 ) ) ;
#33952=CARTESIAN_POINT ( 'NONE',  ( 26.79586899809999778, 1488.686659793930176, 212.4508664459980025 ) ) ;
#33955=CARTESIAN_POINT ( 'NONE',  ( -25.05784678700000256, 1436.599307041280099, 137.8256365093980094 ) ) ;
#33959=EDGE_CURVE ( 'NONE', #12156, #102960, #91419, .T. ) ;
#33961=CARTESIAN_POINT ( 'NONE',  ( -12.98226561589999939, 1414.913060387329779, 219.9156672276980089 ) ) ;
#33964=CARTESIAN_POINT ( 'NONE',  ( 7.191383079060839734, 1407.162969929539940, 222.2855843901380126 ) ) ;
#33966=CARTESIAN_POINT ( 'NONE',  ( -19.60082009959915439, 1457.065427842446070, 225.8893376101511592 ) ) ;
#33967=VERTEX_POINT ( 'NONE', #65309 ) ;
#33970=CARTESIAN_POINT ( 'NONE',  ( 12.61799612763599931, 1435.605627051659894, 150.8454502525350165 ) ) ;
#33971=CARTESIAN_POINT ( 'NONE',  ( -4.069861486464248834, 1440.920437169861543, 184.9827668850385294 ) ) ;
#33980=CARTESIAN_POINT ( 'NONE',  ( 20.38220676649999774, 1509.051558510829864, 188.9487562874980142 ) ) ;
#33982=B_SPLINE_CURVE_WITH_KNOTS ( 'NONE', 3,
 ( #83831, #100086, #82736, #66519, #57004, #58101, #56444, #23369, #49701, #64864, #38521, #72699, #82176, #107381, #5476, #39636, #31226, #14409, #106822, #35082, #68713, #17696, #102817, #43501, #7675, #77645, #51900, #84387, #94999, #101715, #67058, #959, #41831, #59752, #16055, #76533, #75462, #86041, #25007, #109596 ),
 .UNSPECIFIED., .F., .F.,
 ( 4, 3, 3, 3, 3, 3, 3, 3, 3, 3, 3, 3, 3, 4 ),
 ( -69.76875995564780908, -68.67202237711899215, -65.92006359279810113, -64.08310293337700614, -62.52400609995530090, -62.22018943289130277, -61.00809290194970202, -59.74958159879579966, -58.45048782992339653, -57.09264840657949946, -55.60843193452539879, -53.96858821142179607, -51.98595283854560023, -50.09514683520000489 ),
 .UNSPECIFIED. ) ;
#33984=FACE_OUTER_BOUND ( 'NONE', #74016, .T. ) ;
#33986=CARTESIAN_POINT ( 'NONE',  ( 15.93867488059997761, 1409.469629780827972, 193.0035952271976782 ) ) ;
#33988=CARTESIAN_POINT ( 'NONE',  ( 2.134333270180000408, 1421.175322270330071, 183.7859593446980000 ) ) ;
#33990=EDGE_CURVE ( 'NONE', #110334, #102960, #83195, .T. ) ;
#33994=CARTESIAN_POINT ( 'NONE',  ( 1.758995549052309482, 1416.415802373853694, 232.5708266743504566 ) ) ;
#33996=CARTESIAN_POINT ( 'NONE',  ( 18.78419925920000111, 1416.547221146729953, 209.8405087369400235 ) ) ;
#33998=CARTESIAN_POINT ( 'NONE',  ( -4.946284671489999951, 1438.194204504490017, 150.2421849576980151 ) ) ;
#33999=CARTESIAN_POINT ( 'NONE',  ( 44.31826854632529944, 1440.913060365109914, 264.7143195917649905 ) ) ;
#34002=CARTESIAN_POINT ( 'NONE',  ( 10.83054619811773023, 1424.983886448836756, 145.3935680669089834 ) ) ;
#34004=ORIENTED_EDGE ( 'NONE', *, *, #79417, .T. ) ;
#34005=CARTESIAN_POINT ( 'NONE',  ( 1.549183660830179887, 1416.134159091179981, 190.3847494287900020 ) ) ;
#34006=CARTESIAN_POINT ( 'NONE',  ( 17.38027391549962530, 1410.701563970856796, 192.4672136578822688 ) ) ;
#34007=CARTESIAN_POINT ( 'NONE',  ( -24.37050405849999990, 1442.224873102559968, 212.1537385852479929 ) ) ;
#34008=CARTESIAN_POINT ( 'NONE',  ( 7.603309374910287133, 1410.551554993347054, 187.4403096356234926 ) ) ;
#34009=CARTESIAN_POINT ( 'NONE',  ( -3.336075057610619066, 1426.003189273603766, 185.7745020016922695 ) ) ;
#34010=DIRECTION ( 'NONE',  ( -0.1402804634180439824, -0.9901118076173108795, 0.000000000000000000 ) ) ;
#34011=CARTESIAN_POINT ( 'NONE',  ( -1.523962952789999825, 1477.830549788930057, 230.7236636456979966 ) ) ;
#34012=CARTESIAN_POINT ( 'NONE',  ( 13.20369377709999981, 1414.913528139930122, 198.1182872744979875 ) ) ;
#34014=CARTESIAN_POINT ( 'NONE',  ( 7.089350657599999828, 1452.665494806429933, 152.4157077411979913 ) ) ;
#34016=CARTESIAN_POINT ( 'NONE',  ( -27.44625323641425751, 1509.338203236318805, 212.0845200277061906 ) ) ;
#34018=CARTESIAN_POINT ( 'NONE',  ( 23.69809918860000053, 1507.890500233530020, 195.1972782134980093 ) ) ;
#34023=CARTESIAN_POINT ( 'NONE',  ( -16.28817577849460108, 1409.481856019149973, 224.8534995302130142 ) ) ;
#34026=CARTESIAN_POINT ( 'NONE',  ( 18.88376639685650105, 1507.757527395500119, 229.9162007811029866 ) ) ;
#34027=B_SPLINE_CURVE_WITH_KNOTS ( 'NONE', 3,
 ( #30867, #65044, #99159, #42037, #101353, #49344, #6764, #23567, #40926, #67261, #75105, #66708, #92417, #109791, #84028, #15153, #100816, #48245, #58843, #7329, #41492, #66166, #7870, #32536, #15690, #75652, #58295, #33608 ),
 .UNSPECIFIED., .F., .F.,
 ( 4, 2, 2, 1, 2, 2, 2, 1, 1, 1, 1, 1, 2, 2, 2, 2, 4 ),
 ( 0.000000000000000000, 0.2499999999999318878, 0.3749999999998951394, 0.4374999999998763767, 0.4687499999998644973, 0.4999999999998526734, 0.6249999999998108180, 0.6874999999997875033, 0.7187499999997730704, 0.7343749999997656319, 0.7421874999997594147, 0.7460937499997561950, 0.7480468749997573052, 0.7499999999997585265, 0.8749999999998818723, 0.9374999999999408251, 1.000000000000000000 ),
 .UNSPECIFIED. ) ;
#34029=CARTESIAN_POINT ( 'NONE',  ( 39.95031265526250763, 1441.572021889720190, 136.8870288321719784 ) ) ;
#34030=CARTESIAN_POINT ( 'NONE',  ( 19.82086717690000199, 1452.811554597230042, 209.2880291464769869 ) ) ;
#34036=CARTESIAN_POINT ( 'NONE',  ( 41.65927937599999353, 1443.915252855300196, 135.6909788338979865 ) ) ;
#34038=CARTESIAN_POINT ( 'NONE',  ( 1.411045156649999965, 1409.467890906029879, 185.4969889618979835 ) ) ;
#34039=CARTESIAN_POINT ( 'NONE',  ( 4.520455601509999255, 1424.084465838330061, 184.9550280210980020 ) ) ;
#34041=CARTESIAN_POINT ( 'NONE',  ( -2.712996093226240024, 1440.235714014299901, 157.0895377761229952 ) ) ;
#34042=AXIS2_PLACEMENT_3D ( 'NONE', #62632, #88341, #63717 ) ;
#34043=CARTESIAN_POINT ( 'NONE',  ( 11.84242365151049903, 1431.324256260269976, 147.6543138665190043 ) ) ;
#34044=CARTESIAN_POINT ( 'NONE',  ( 0.1422329807200000129, 1466.041212668930029, 235.8555543989980094 ) ) ;
#34048=CARTESIAN_POINT ( 'NONE',  ( -25.98102620619109970, 1446.564900598659960, 138.2990622187889755 ) ) ;
#34051=CARTESIAN_POINT ( 'NONE',  ( -9.599706269345578398E-10, 1471.041207172160057, 256.6978854479500001 ) ) ;
#34053=CARTESIAN_POINT ( 'NONE',  ( -0.9063479630909999640, 1415.579607672129896, 227.4689347612980157 ) ) ;
#34054=CARTESIAN_POINT ( 'NONE',  ( -6.479667820239999543, 1418.395698601130107, 233.3433503499980191 ) ) ;
#34057=CARTESIAN_POINT ( 'NONE',  ( -0.6140284191404157266, 1485.453369257635131, 181.9287747154768908 ) ) ;
#34059=CARTESIAN_POINT ( 'NONE',  ( -45.74118403190329474, 1438.479771586579773, 268.7597751522629324 ) ) ;
#34065=CARTESIAN_POINT ( 'NONE',  ( -5.402319840979999732, 1434.355786217680134, 154.6519182847980005 ) ) ;
#34067=CARTESIAN_POINT ( 'NONE',  ( 19.32507466223246340, 1456.645243537790293, 224.6377563528816950 ) ) ;
#34069=CARTESIAN_POINT ( 'NONE',  ( -26.06749262380980170, 1451.758091925960116, 135.9256846038920230 ) ) ;
#34070=ORIENTED_EDGE ( 'NONE', *, *, #12130, .T. ) ;
#34071=CARTESIAN_POINT ( 'NONE',  ( 16.68183166340000056, 1424.849819094029954, 221.4660109932979992 ) ) ;
#34074=CARTESIAN_POINT ( 'NONE',  ( -1.927277385857209868, 1419.501960165059927, 185.7627030526099929 ) ) ;
#34075=AXIS2_PLACEMENT_3D ( 'NONE', #78187, #2065, #46281 ) ;
#34077=CARTESIAN_POINT ( 'NONE',  ( -3.835404308833623155, 1396.046995657106436, 202.1011854665750036 ) ) ;
#34078=CARTESIAN_POINT ( 'NONE',  ( -22.74821099489519938, 1452.118675354829747, 139.2359698183670105 ) ) ;
#34081=CARTESIAN_POINT ( 'NONE',  ( -0.6098768256049610370, 1408.561131195760026, 270.4290843811310197 ) ) ;
#34082=CARTESIAN_POINT ( 'NONE',  ( 6.582508756332179800, 1418.411819419869744, 233.6284590037290059 ) ) ;
#34084=EDGE_LOOP ( 'NONE', ( #39749, #79301, #93165, #66187, #57367 ) ) ;
#34085=VERTEX_POINT ( 'NONE', #82077 ) ;
#34086=CARTESIAN_POINT ( 'NONE',  ( -23.44508921861510231, 1410.148484811090157, 210.0298535335690246 ) ) ;
#34087=CARTESIAN_POINT ( 'NONE',  ( -4.363122647540000010, 1423.854802298929826, 184.2546043570980032 ) ) ;
#34088=CARTESIAN_POINT ( 'NONE',  ( -11.49747574035130171, 1416.913060341609935, 197.9009878090930101 ) ) ;
#34089=CARTESIAN_POINT ( 'NONE',  ( -45.16578704421618795, 1435.656933826767045, 266.2029088751467611 ) ) ;
#34090=CARTESIAN_POINT ( 'NONE',  ( -20.30416289926380458, 1484.529698969839956, 192.9143954880039757 ) ) ;
#34092=EDGE_CURVE ( 'NONE', #45960, #76272, #52440, .T. ) ;
#34093=CARTESIAN_POINT ( 'NONE',  ( 29.93303073770439582, 1467.353064289500026, 266.6087639478620304 ) ) ;
#34095=CARTESIAN_POINT ( 'NONE',  ( -17.31863478597802697, 1422.547962107037165, 226.6134709424001414 ) ) ;
#34097=ORIENTED_EDGE ( 'NONE', *, *, #87037, .T. ) ;
#34098=CARTESIAN_POINT ( 'NONE',  ( 18.51214429768622693, 1458.740534512576005, 227.6070309199760118 ) ) ;
#34102=ORIENTED_EDGE ( 'NONE', *, *, #83267, .T. ) ;
#34103=CARTESIAN_POINT ( 'NONE',  ( 3.931911118920000447, 1448.296755884660115, 184.2998928590980086 ) ) ;
#34111=CARTESIAN_POINT ( 'NONE',  ( 1.968667276625390095, 1408.981807763489996, 186.9191247717589874 ) ) ;
#34112=CARTESIAN_POINT ( 'NONE',  ( 1.270493918489999929, 1416.663721100529983, 233.2811219237980254 ) ) ;
#34113=CARTESIAN_POINT ( 'NONE',  ( -17.83359347479203905, 1423.458363862109991, 226.0411963962040147 ) ) ;
#34114=CARTESIAN_POINT ( 'NONE',  ( 13.31824321100000041, 1409.378143688529917, 226.7832290943979956 ) ) ;
#34120=VECTOR ( 'NONE', #25906, 1000.000000000000000 ) ;
#34121=CARTESIAN_POINT ( 'NONE',  ( 11.60004869885203682, 1411.254281879943164, 137.0999999980979851 ) ) ;
#34125=B_SPLINE_CURVE_WITH_KNOTS ( 'NONE', 3,
 ( #104373, #105485, #94869, #95974, #79744, #19235, #28776, #71373, #10878, #45050, #79194, #104931, #11431, #43376, #28218, #62405, #96533, #19807, #54013, #64604, #31512, #38263 ),
 .UNSPECIFIED., .F., .F.,
 ( 4, 2, 2, 1, 1, 1, 1, 2, 2, 2, 2, 2, 4 ),
 ( 0.000000000000000000, 0.2500000000000847655, 0.3750000000001300071, 0.4375000000001500466, 0.4687500000001631473, 0.4843750000001671441, 0.4921875000001716960, 0.4960937500001712519, 0.5000000000001707523, 0.7500000000000853762, 0.8125000000000641709, 0.8750000000000429656, 1.000000000000000000 ),
 .UNSPECIFIED. ) ;
#34126=CARTESIAN_POINT ( 'NONE',  ( -34.99794265375160052, 1450.308730971829846, 136.2298232396449862 ) ) ;
#34130=CARTESIAN_POINT ( 'NONE',  ( -3.500000000000000000, 1422.625370988529994, 168.5578661042980286 ) ) ;
#34131=CARTESIAN_POINT ( 'NONE',  ( 11.72722094679999927, 1433.446908946229996, 150.8820538568979828 ) ) ;
#34132=CARTESIAN_POINT ( 'NONE',  ( 12.48077398530000082, 1459.371347868330076, 243.9198229428980085 ) ) ;
#34133=CARTESIAN_POINT ( 'NONE',  ( 12.28605913131140071, 1415.088506334930116, 197.2751500656220287 ) ) ;
#34134=CIRCLE ( 'NONE', #39500, 2.000000000000002220 ) ;
#34135=CARTESIAN_POINT ( 'NONE',  ( -22.53878221424140094, 1411.058442688259902, 212.0450776560099939 ) ) ;
#34139=CARTESIAN_POINT ( 'NONE',  ( -19.01375814760000083, 1486.340012975929994, 189.2527429762979807 ) ) ;
#34142=CARTESIAN_POINT ( 'NONE',  ( 10.63098969396934379, 1398.228131935662532, 216.6347355816575089 ) ) ;
#34143=CARTESIAN_POINT ( 'NONE',  ( -29.45841291127520023, 1509.941770834379895, 211.8256419367419880 ) ) ;
#34144=CARTESIAN_POINT ( 'NONE',  ( 23.43227205659999868, 1410.913138743030004, 212.1033097375579928 ) ) ;
#34145=PLANE ( 'NONE',  #41366 ) ;
#34146=CARTESIAN_POINT ( 'NONE',  ( 26.21349280692992778, 1436.698295471538813, 136.8766113756052221 ) ) ;
#34148=CARTESIAN_POINT ( 'NONE',  ( 21.79083509029999988, 1497.713060387329961, 214.0856487658080027 ) ) ;
#34152=CARTESIAN_POINT ( 'NONE',  ( 0.1759063265243840102, 1476.870715021929982, 182.2288026130389653 ) ) ;
#34153=CARTESIAN_POINT ( 'NONE',  ( -5.370514330159649852, 1422.356910281434239, 139.1416123588654727 ) ) ;
#34155=FACE_OUTER_BOUND ( 'NONE', #25835, .T. ) ;
#34157=CARTESIAN_POINT ( 'NONE',  ( 13.19843678480000015, 1434.900414026109956, 149.6995543751980051 ) ) ;
#34158=CARTESIAN_POINT ( 'NONE',  ( -41.60033908840290451, 1444.718971643000032, 134.0999999983919793 ) ) ;
#34166=CARTESIAN_POINT ( 'NONE',  ( -13.20398174397830005, 1430.333021908660157, 195.5447948587090252 ) ) ;
#34167=DIRECTION ( 'NONE',  ( -0.1402804634201463563, 0.9901118076170130067, 0.000000000000000000 ) ) ;
#34168=CARTESIAN_POINT ( 'NONE',  ( 8.469197029634038643, 1409.208811264400083, 221.4585696155599805 ) ) ;
#34174=CARTESIAN_POINT ( 'NONE',  ( -29.31190787429999745, 1451.889799756029788, 135.2848617097980082 ) ) ;
#34175=CARTESIAN_POINT ( 'NONE',  ( -15.77958100662340080, 1409.472299422209971, 225.4880743202079998 ) ) ;
#34177=ORIENTED_EDGE ( 'NONE', *, *, #86959, .T. ) ;
#34182=CARTESIAN_POINT ( 'NONE',  ( -0.1548099527865300085, 1420.468350699849907, 182.8372881064299804 ) ) ;
#34184=CARTESIAN_POINT ( 'NONE',  ( -11.60004869885203505, 1428.425991026145311, 134.1711281075547788 ) ) ;
#34186=CARTESIAN_POINT ( 'NONE',  ( 19.00883633615545421, 1437.780163653907039, 213.2322572209417899 ) ) ;
#34187=CARTESIAN_POINT ( 'NONE',  ( 1.873062257339999981, 1417.577345317929939, 233.6032974765979873 ) ) ;
#34189=CARTESIAN_POINT ( 'NONE',  ( -23.28153290659989949, 1507.877024493434192, 223.8845470390981802 ) ) ;
#34195=CARTESIAN_POINT ( 'NONE',  ( -2.500000000000000000, 1434.283878676689937, 157.5533472140980109 ) ) ;
#34196=FACE_OUTER_BOUND ( 'NONE', #47572, .T. ) ;
#34199=CARTESIAN_POINT ( 'NONE',  ( -33.93529341107537078, 1435.841716432657222, 135.9421945816383470 ) ) ;
#34202=CARTESIAN_POINT ( 'NONE',  ( -21.12097961670000146, 1430.346877887030132, 198.3664044052980273 ) ) ;
#34203=CARTESIAN_POINT ( 'NONE',  ( -11.06783048073080167, 1426.044759707710000, 103.8947504975569984 ) ) ;
#34204=CARTESIAN_POINT ( 'NONE',  ( 16.85684277289790245, 1410.872046192200060, 191.8747558144809773 ) ) ;
#34207=CARTESIAN_POINT ( 'NONE',  ( 17.11918923422064864, 1509.631155535743119, 184.4835570923741841 ) ) ;
#34208=CARTESIAN_POINT ( 'NONE',  ( 1.520098423109999874, 1489.452917662129948, 187.0062982106979916 ) ) ;
#34209=CARTESIAN_POINT ( 'NONE',  ( -7.132051953269999522, 1405.830933579630027, 267.2558761556979903 ) ) ;
#34210=CARTESIAN_POINT ( 'NONE',  ( 16.35567120235890215, 1509.488510095419770, 233.6167396447019655 ) ) ;
#34213=CARTESIAN_POINT ( 'NONE',  ( -38.63631528028910367, 1439.261520478130024, 136.6606707570919923 ) ) ;
#34214=ORIENTED_EDGE ( 'NONE', *, *, #109828, .T. ) ;
#34215=CARTESIAN_POINT ( 'NONE',  ( 11.36773274011689949, 1396.369100750580174, 213.4700073609069761 ) ) ;
#34217=CARTESIAN_POINT ( 'NONE',  ( -16.63810603980000025, 1458.859429223330153, 229.6331253552980058 ) ) ;
#34221=CARTESIAN_POINT ( 'NONE',  ( -16.68599179819999989, 1461.099982565929849, 230.2790296985980092 ) ) ;
#34235=ORIENTED_EDGE ( 'NONE', *, *, #75460, .T. ) ;
#34236=CARTESIAN_POINT ( 'NONE',  ( 11.75600116617299840, 1426.829850492249989, 145.4901315597400071 ) ) ;
#34238=CARTESIAN_POINT ( 'NONE',  ( 19.76363181259999990, 1497.691518898830054, 228.7599396882980045 ) ) ;
#34240=CARTESIAN_POINT ( 'NONE',  ( -13.35004134540000109, 1415.296882282229944, 221.1257189973979962 ) ) ;
#34242=CARTESIAN_POINT ( 'NONE',  ( -11.35814853775019984, 1432.342270311689845, 151.4015281471440062 ) ) ;
#34246=CARTESIAN_POINT ( 'NONE',  ( -4.869499518229999602, 1422.270630277530017, 184.7950624201980077 ) ) ;
#34249=CARTESIAN_POINT ( 'NONE',  ( -10.01745403176274785, 1410.637555081950040, 188.4336630067121234 ) ) ;
#34251=CARTESIAN_POINT ( 'NONE',  ( 22.63922376101739786, 1413.302736438429747, 206.1995960539140356 ) ) ;
#34253=CARTESIAN_POINT ( 'NONE',  ( -6.754078978114156584, 1519.913060387329779, 184.4732361498326156 ) ) ;
#34254=CARTESIAN_POINT ( 'NONE',  ( -4.649812432218794811, 1423.695263795027358, 184.4549038447098610 ) ) ;
#34256=ORIENTED_EDGE ( 'NONE', *, *, #77742, .F. ) ;
#34258=CARTESIAN_POINT ( 'NONE',  ( 18.27238427227369755, 1424.505937855529965, 223.6578119888600042 ) ) ;
#34260=CARTESIAN_POINT ( 'NONE',  ( -2.902680970014407613, 1484.524336014886785, 183.2878275774386339 ) ) ;
#34264=CARTESIAN_POINT ( 'NONE',  ( 1.323582945269999867, 1489.466620109829819, 186.9612537963979833 ) ) ;
#34266=CARTESIAN_POINT ( 'NONE',  ( -11.16757872979999888, 1425.149737177430097, 145.1863048323980081 ) ) ;
#34273=EDGE_CURVE ( 'NONE', #77021, #55879, #66418, .T. ) ;
#34274=CARTESIAN_POINT ( 'NONE',  ( -19.89091575900000208, 1495.374792094930172, 228.3689221276979993 ) ) ;
#34276=CARTESIAN_POINT ( 'NONE',  ( -16.32629271558399608, 1459.450551812079993, 228.9510548132139718 ) ) ;
#34279=CARTESIAN_POINT ( 'NONE',  ( 21.85509849029999785, 1410.191647020929850, 266.7712709411979972 ) ) ;
#34281=CARTESIAN_POINT ( 'NONE',  ( 24.25229055349999996, 1435.770029208010101, 138.8216067376980050 ) ) ;
#34282=CARTESIAN_POINT ( 'NONE',  ( 18.16373175749999902, 1430.308745069530005, 192.1900383825980043 ) ) ;
#34283=CARTESIAN_POINT ( 'NONE',  ( -0.1466225642774790228, 1507.635109844429962, 237.3673378143610080 ) ) ;
#34284=FACE_OUTER_BOUND ( 'NONE', #1321, .T. ) ;
#34285=DIRECTION ( 'NONE',  ( 0.4258765256105080388, -0.006533365793910755025, 0.9047577024072938068 ) ) ;
#34288=CARTESIAN_POINT ( 'NONE',  ( -13.64317476579999955, 1445.682466854349968, 188.2845503314979965 ) ) ;
#34291=CARTESIAN_POINT ( 'NONE',  ( 4.301461580539999829, 1407.800349814830042, 270.1336327149980434 ) ) ;
#34292=ORIENTED_EDGE ( 'NONE', *, *, #34980, .F. ) ;
#34293=CARTESIAN_POINT ( 'NONE',  ( 1.456838540400960058, 1499.011618624379935, 181.4667026936230059 ) ) ;
#34294=CARTESIAN_POINT ( 'NONE',  ( -13.98332703483129968, 1409.401368927429758, 203.8662359848739811 ) ) ;
#34298=CARTESIAN_POINT ( 'NONE',  ( -21.81807642700000116, 1471.495927914430240, 269.1143084626980340 ) ) ;
#34299=CARTESIAN_POINT ( 'NONE',  ( 1.358935478622729898, 1412.145631141479953, 232.7165187772180275 ) ) ;
#34301=CARTESIAN_POINT ( 'NONE',  ( -24.12916442465748545, 1444.472920415359567, 211.7107983591160405 ) ) ;
#34304=CARTESIAN_POINT ( 'NONE',  ( -3.346415545340000186, 1442.759383208520148, 155.7539078627980018 ) ) ;
#34308=ADVANCED_FACE ( 'NONE', ( #85377 ), #22208, .F. ) ;
#34309=CARTESIAN_POINT ( 'NONE',  ( -22.62661505969999709, 1409.703199196130072, 206.8548854524279932 ) ) ;
#34312=CARTESIAN_POINT ( 'NONE',  ( 14.66127812029999866, 1415.087974639930053, 199.4957085038979869 ) ) ;
#34317=CARTESIAN_POINT ( 'NONE',  ( 0.8251472201360000591, 1438.194204504490017, 150.6035180695979818 ) ) ;
#34322=CARTESIAN_POINT ( 'NONE',  ( -21.99779640679999915, 1409.845345977029865, 211.9582514417379855 ) ) ;
#34324=CARTESIAN_POINT ( 'NONE',  ( 11.70097560617689858, 1426.719468243919891, 141.5896315292509939 ) ) ;
#34329=CARTESIAN_POINT ( 'NONE',  ( -16.56954065640239904, 1507.336002802359872, 224.6960143935069993 ) ) ;
#34330=B_SPLINE_CURVE_WITH_KNOTS ( 'NONE', 5,
 ( #35798, #3326, #11697, #45869, #29054, #95702 ),
 .UNSPECIFIED., .F., .F.,
 ( 6, 6 ),
 ( -1.469182821640000025, -2.166508562106983504E-06 ),
 .UNSPECIFIED. ) ;
#34332=CARTESIAN_POINT ( 'NONE',  ( -9.119309862993969062, 1398.183652844645621, 218.3944131779407201 ) ) ;
#34333=CARTESIAN_POINT ( 'NONE',  ( -3.524418834340278472, 1440.781073485925162, 156.7014001434145598 ) ) ;
#34335=CARTESIAN_POINT ( 'NONE',  ( 1.413944454890000202, 1507.072543608730030, 236.8050756195980284 ) ) ;
#34340=CARTESIAN_POINT ( 'NONE',  ( 11.97251399677129946, 1433.655889273449930, 150.1647575922700071 ) ) ;
#34342=EDGE_LOOP ( 'NONE', ( #58219, #37217, #106253, #67614 ) ) ;
#34343=CARTESIAN_POINT ( 'NONE',  ( -0.0002531825210758750105, 1396.493310238344520, 221.5300458565427562 ) ) ;
#34344=CARTESIAN_POINT ( 'NONE',  ( -21.59613672980000132, 1509.442267788030222, 191.6826760664980043 ) ) ;
#34348=CARTESIAN_POINT ( 'NONE',  ( 2.286265947080000416, 1427.727383903629971, 112.4493539157979995 ) ) ;
#34349=CARTESIAN_POINT ( 'NONE',  ( 18.53962229561609831, 1488.413181566670119, 229.1505926759119802 ) ) ;
#34350=EDGE_CURVE ( 'NONE', #57276, #76827, #9566, .T. ) ;
#34352=CARTESIAN_POINT ( 'NONE',  ( 2.046362623379999857, 1488.173483295229971, 182.0543892500980121 ) ) ;
#34353=CARTESIAN_POINT ( 'NONE',  ( -0.3142747835549999924, 1415.426210663629945, 191.6391921992979803 ) ) ;
#34358=CARTESIAN_POINT ( 'NONE',  ( 13.86388155043169945, 1415.301705643500100, 197.4576564492959960 ) ) ;
#34359=CARTESIAN_POINT ( 'NONE',  ( 11.85132026249999981, 1431.246777428639916, 150.3007239271979927 ) ) ;
#34362=CARTESIAN_POINT ( 'NONE',  ( 14.36662627577019968, 1436.257422054949984, 150.0160098068969887 ) ) ;
#34364=ORIENTED_EDGE ( 'NONE', *, *, #105536, .T. ) ;
#34367=CARTESIAN_POINT ( 'NONE',  ( 13.05599175049793281, 1444.836491748568505, 169.4127969366490731 ) ) ;
#34368=CARTESIAN_POINT ( 'NONE',  ( -2.855376345160000273, 1466.858753905630010, 235.0846608803980189 ) ) ;
#34373=CARTESIAN_POINT ( 'NONE',  ( -18.78398581570814940, 1444.618302659428537, 213.1331773526644611 ) ) ;
#34380=CARTESIAN_POINT ( 'NONE',  ( -18.65451756079999868, 1507.632629717229975, 229.7110761602979778 ) ) ;
#34381=VERTEX_POINT ( 'NONE', #55900 ) ;
#34382=CARTESIAN_POINT ( 'NONE',  ( -2.923521387370000113, 1410.394928919130280, 186.6127609212979905 ) ) ;
#34384=CARTESIAN_POINT ( 'NONE',  ( -11.04992432776889899, 1414.913526854310021, 195.9912987695080346 ) ) ;
#34385=ORIENTED_EDGE ( 'NONE', *, *, #79857, .F. ) ;
#34386=CARTESIAN_POINT ( 'NONE',  ( 23.65786361689999850, 1434.694201751649871, 215.1063102513179786 ) ) ;
#34389=SPHERICAL_SURFACE ( 'NONE', #69628, 2.000000000000000000 ) ;
#34394=CARTESIAN_POINT ( 'NONE',  ( -20.60407645530000309, 1508.351959126529891, 190.1129144765980072 ) ) ;
#34397=EDGE_CURVE ( 'NONE', #65085, #65905, #105732, .T. ) ;
#34398=CARTESIAN_POINT ( 'NONE',  ( 14.55268257189999836, 1410.361135901630178, 191.4983566902979817 ) ) ;
#34399=CARTESIAN_POINT ( 'NONE',  ( -16.74093840945409539, 1486.115613468081847, 187.5028501039167281 ) ) ;
#34403=CARTESIAN_POINT ( 'NONE',  ( 13.60517974880000125, 1473.691213157429956, 264.8398836597979766 ) ) ;
#34404=CARTESIAN_POINT ( 'NONE',  ( 1.610433614691386461, 1452.674093572039055, 183.5081501456340902 ) ) ;
#34406=CARTESIAN_POINT ( 'NONE',  ( -7.334500520190000650, 1507.579365412929974, 235.5537206881979841 ) ) ;
#34407=CARTESIAN_POINT ( 'NONE',  ( -24.04315183079999940, 1445.026065454899936, 213.4541038299180116 ) ) ;
#34408=EDGE_CURVE ( 'NONE', #43746, #49156, #41709, .T. ) ;
#34410=CARTESIAN_POINT ( 'NONE',  ( 17.14579715356120104, 1409.552403581870067, 222.3181863344280202 ) ) ;
#34415=CARTESIAN_POINT ( 'NONE',  ( 0.1075185588789999980, 1406.066315318429815, 269.0456997844980265 ) ) ;
#34416=CIRCLE ( 'NONE', #61237, 2.000000000000000000 ) ;
#34418=CARTESIAN_POINT ( 'NONE',  ( 13.15345997939999911, 1428.696580737029990, 223.2895104518979963 ) ) ;
#34422=CARTESIAN_POINT ( 'NONE',  ( 26.79407919707900021, 1435.433162376700011, 135.2875019197180109 ) ) ;
#34424=CARTESIAN_POINT ( 'NONE',  ( 34.85401832400309274, 1450.338014512889913, 136.2298619501380017 ) ) ;
#34425=CARTESIAN_POINT ( 'NONE',  ( -42.00585553703391639, 1454.281673901052727, 269.0755534770359532 ) ) ;
#34427=CARTESIAN_POINT ( 'NONE',  ( 13.79910387159999807, 1508.398165315730012, 185.5292457990980211 ) ) ;
#34432=CARTESIAN_POINT ( 'NONE',  ( 1.623075365390000080, 1428.602351821930142, 149.4837496357980058 ) ) ;
#34433=EDGE_CURVE ( 'NONE', #63865, #28394, #61771, .T. ) ;
#34435=CARTESIAN_POINT ( 'NONE',  ( 19.57175081105178194, 1452.229599788707219, 144.4156370992074585 ) ) ;
#34436=CARTESIAN_POINT ( 'NONE',  ( 16.33822231007999903, 1488.657264317530007, 188.6886238127860054 ) ) ;
#34437=CARTESIAN_POINT ( 'NONE',  ( 11.44793483447996074, 1425.801405795868959, 139.0695979703967851 ) ) ;
#34438=CARTESIAN_POINT ( 'NONE',  ( -2.370970874524634286, 1427.002265528474027, 134.0999999980980135 ) ) ;
#34440=CARTESIAN_POINT ( 'NONE',  ( -28.83583423950000224, 1509.587522268929888, 209.1203260760459841 ) ) ;
#34443=CARTESIAN_POINT ( 'NONE',  ( 42.85028971309680657, 1440.913025295369835, 270.2009442048760093 ) ) ;
#34444=CARTESIAN_POINT ( 'NONE',  ( -10.59239855707533984, 1451.301507702100480, 152.0626276528745393 ) ) ;
#34446=CARTESIAN_POINT ( 'NONE',  ( 25.31932687029999940, 1435.570944935079979, 136.4448942406980052 ) ) ;
#34448=CARTESIAN_POINT ( 'NONE',  ( 11.90000415720300175, 1434.913060496859998, 147.6452464505769910 ) ) ;
#34449=ORIENTED_EDGE ( 'NONE', *, *, #39255, .T. ) ;
#34450=CARTESIAN_POINT ( 'NONE',  ( -16.44160288201669928, 1409.512366239009907, 225.1669717104299764 ) ) ;
#34452=CARTESIAN_POINT ( 'NONE',  ( 7.435066116149999793, 1441.600846913620217, 149.7516446007980164 ) ) ;
#34453=ORIENTED_EDGE ( 'NONE', *, *, #105016, .F. ) ;
#34455=CARTESIAN_POINT ( 'NONE',  ( 4.219439031349260461, 1446.230224802979819, 182.3842141579679890 ) ) ;
#34457=CARTESIAN_POINT ( 'NONE',  ( 10.90929167140000011, 1426.089277454929970, 92.68786258269780376 ) ) ;
#34459=CARTESIAN_POINT ( 'NONE',  ( 23.55538394579999917, 1409.900238729630018, 209.4988520729140191 ) ) ;
#34460=CARTESIAN_POINT ( 'NONE',  ( 4.202765219874719627, 1425.034743857860121, 185.2477664996769988 ) ) ;
#34465=CARTESIAN_POINT ( 'NONE',  ( 8.482876245789999103, 1508.704763218230028, 182.5447702950980329 ) ) ;
#34470=CARTESIAN_POINT ( 'NONE',  ( -2.776018498009749713E-09, 1414.697267606029982, 245.4362868392339863 ) ) ;
#34473=CARTESIAN_POINT ( 'NONE',  ( -40.71480956220000280, 1443.734648304970051, 137.1148404093979991 ) ) ;
#34475=CARTESIAN_POINT ( 'NONE',  ( -0.4721143188960000292, 1471.791680839530045, 269.8654495172979750 ) ) ;
#34478=CARTESIAN_POINT ( 'NONE',  ( 16.39250384509999847, 1431.113060387329824, 198.8961368102980316 ) ) ;
#34479=CARTESIAN_POINT ( 'NONE',  ( 13.80546151116429954, 1434.979654507460054, 148.5370226032280243 ) ) ;
#34482=CARTESIAN_POINT ( 'NONE',  ( -19.31623058889999811, 1475.513060387329915, 200.7139244924079833 ) ) ;
#34484=CARTESIAN_POINT ( 'NONE',  ( -0.06979922123900890452, 1408.910622944780016, 194.4360052272290034 ) ) ;
#34485=CARTESIAN_POINT ( 'NONE',  ( -12.05032705967369999, 1407.437450256659986, 269.2402808039070123 ) ) ;
#34486=CARTESIAN_POINT ( 'NONE',  ( -14.49936296086660015, 1436.121868349760007, 149.8980290887049875 ) ) ;
#34489=CARTESIAN_POINT ( 'NONE',  ( 13.94587001030000017, 1445.277640235309946, 189.2991415692980013 ) ) ;
#34490=ORIENTED_EDGE ( 'NONE', *, *, #64103, .T. ) ;
#34491=EDGE_LOOP ( 'NONE', ( #18921, #24616, #91686, #57475 ) ) ;
#34492=CARTESIAN_POINT ( 'NONE',  ( 4.724912038846999174, 1422.196582765026051, 184.1782025151506730 ) ) ;
#34494=EDGE_CURVE ( 'NONE', #44794, #41855, #47080, .T. ) ;
#34496=CARTESIAN_POINT ( 'NONE',  ( -18.66657011559999901, 1485.489288798229836, 189.3324219145979725 ) ) ;
#34497=ORIENTED_EDGE ( 'NONE', *, *, #32311, .T. ) ;
#34499=DIRECTION ( 'NONE',  ( -4.137698748469999823E-18, -2.750577543510000101E-14, -1.000000000000000000 ) ) ;
#34501=CARTESIAN_POINT ( 'NONE',  ( -27.17282701799999955, 1509.164027956230029, 203.0634631091180324 ) ) ;
#34502=CARTESIAN_POINT ( 'NONE',  ( -1.527354483230000115, 1467.880741325629970, 230.2836666281979774 ) ) ;
#34504=CARTESIAN_POINT ( 'NONE',  ( -6.825986770030000983, 1409.091027441730148, 196.5037157050980170 ) ) ;
#34506=CARTESIAN_POINT ( 'NONE',  ( 2.149988386126029882E-09, 1405.989059316979819, 266.9611530767110139 ) ) ;
#34509=CARTESIAN_POINT ( 'NONE',  ( 26.28495520090000070, 1469.245429234630137, 210.9605151810879988 ) ) ;
#34510=CARTESIAN_POINT ( 'NONE',  ( 19.59849823883310194, 1467.109269350429940, 224.9849522125649912 ) ) ;
#34511=CARTESIAN_POINT ( 'NONE',  ( -25.02785746449999849, 1436.442580334869945, 137.8071743735980021 ) ) ;
#34514=B_SPLINE_CURVE_WITH_KNOTS ( 'NONE', 5,
 ( #91131, #91681, #32339, #64307, #58100, #109053 ),
 .UNSPECIFIED., .F., .F.,
 ( 6, 6 ),
 ( -7.104449043337727865, 0.000000000000000000 ),
 .UNSPECIFIED. ) ;
#34515=CARTESIAN_POINT ( 'NONE',  ( -15.10917143540000041, 1420.422469564430003, 227.0222420103980028 ) ) ;
#34519=PLANE ( 'NONE',  #31248 ) ;
#34520=CARTESIAN_POINT ( 'NONE',  ( -5.977046268519999650, 1412.833511534230183, 231.6136271241979898 ) ) ;
#34525=CARTESIAN_POINT ( 'NONE',  ( 12.48193344527700077, 1434.439583145440110, 149.7136235699300073 ) ) ;
#34526=CARTESIAN_POINT ( 'NONE',  ( 16.33619008302309794, 1459.305500065469914, 229.1019625438389937 ) ) ;
#34527=CARTESIAN_POINT ( 'NONE',  ( -21.84222827614330242, 1507.845630688500023, 226.4317230014339941 ) ) ;
#34528=CARTESIAN_POINT ( 'NONE',  ( -2.923263677340000033, 1409.521015946229909, 186.8216734875980194 ) ) ;
#34529=DIRECTION ( 'NONE',  ( -3.323949399211515826E-08, -0.03085664264949944391, -0.9995238204287079098 ) ) ;
#34533=DIRECTION ( 'NONE',  ( -0.03489950508427384218, 0.9993908267263977852, -8.612351889057847367E-09 ) ) ;
#34534=CARTESIAN_POINT ( 'NONE',  ( 20.17745194909999995, 1509.606869831929998, 187.6124617494980100 ) ) ;
#34537=CARTESIAN_POINT ( 'NONE',  ( -12.78755503160000018, 1416.844618635429924, 195.3259367831980171 ) ) ;
#34544=CARTESIAN_POINT ( 'NONE',  ( -9788.078716723830439, 2833.596074015639715, 1421.913706742800059 ) ) ;
#34546=FACE_OUTER_BOUND ( 'NONE', #91777, .T. ) ;
#34548=CARTESIAN_POINT ( 'NONE',  ( 18.82708389389999581, 1416.254459046630018, 210.0516237558479986 ) ) ;
#34551=CARTESIAN_POINT ( 'NONE',  ( -21.97938480444670262, 1506.433683733529961, 209.5040264213440082 ) ) ;
#34552=CARTESIAN_POINT ( 'NONE',  ( 41.65366836192780653, 1440.913060353889932, 261.5143753377130338 ) ) ;
#34557=CARTESIAN_POINT ( 'NONE',  ( 1.549551291508020068, 1416.073666489970037, 190.4139934404920211 ) ) ;
#34558=B_SPLINE_CURVE_WITH_KNOTS ( 'NONE', 5,
 ( #38965, #64771, #12124, #54712, #56897, #107837, #88838, #80446, #97778 ),
 .UNSPECIFIED., .F., .F.,
 ( 6, 3, 6 ),
 ( 0.000000000000000000, 0.3174986011340940051, 1.000000000000000000 ),
 .UNSPECIFIED. ) ;
#34559=B_SPLINE_CURVE_WITH_KNOTS ( 'NONE', 3,
 ( #38999, #108425, #55843, #107320, #12711, #46895, #82675, #13788, #64243, #46348, #106222, #80477, #30051, #4327, #5966, #107866, #39570, #63162, #106761, #74293, #20539, #22730, #38457, #73743, #98365, #54743, #13239, #82112, #65344, #99453, #3795, #56932, #14346, #12157, #72107, #40111, #37926, #51272, #66991, #83222, #23298, #93800, #84851, #75393, #92172, #92714, #41221, #49635, #83771, #76473, #102218, #91620, #33908, #7066, #77038, #85404, #42881, #32268, #58035, #33351, #100563, #24935, #75923, #8152, #15991, #109530, #23844, #6513, #31707, #42320, #65891, #110626, #16531, #15444, #32806, #74838, #59687, #50193, #101101, #101647, #100010, #68103, #40666, #108982, #66448, #25497, #84319, #7610, #24401, #58585, #57495 ),
 .UNSPECIFIED., .F., .F.,
 ( 4, 3, 3, 3, 3, 3, 3, 3, 3, 3, 3, 3, 3, 3, 3, 3, 3, 3, 3, 3, 3, 3, 3, 3, 3, 3, 3, 3, 3, 3, 4 ),
 ( 3.477816786180000008, 3.521729306530609893, 3.570087198783100213, 3.634106538065850156, 3.694755914534010088, 3.741217293045549841, 3.763403968410900191, 3.897984528872969978, 4.045194602964830466, 4.230054492803989596, 4.406723692118539759, 4.558577338311470051, 4.583392891433089922, 5.418196481693069444, 5.757360972090920015, 6.611787513787080073, 7.464496660483499468, 8.330048250581310043, 9.169744169958040203, 10.05608535847590090, 10.93306408244489880, 11.79628248831910042, 12.57647286233950013, 13.46759305193459966, 14.34455184101869918, 15.23010248451859994, 16.12090556754780124, 17.01703777043580246, 17.90344418320950126, 18.80443928115469987, 19.70543437909999795 ),
 .UNSPECIFIED. ) ;
#34560=CARTESIAN_POINT ( 'NONE',  ( 25.99851496269999984, 1488.583638219929981, 206.2264607038780184 ) ) ;
#34561=CARTESIAN_POINT ( 'NONE',  ( -27.70707313569999997, 1508.597282338030027, 210.5802476146679680 ) ) ;
#34566=CARTESIAN_POINT ( 'NONE',  ( 13.15471227499809892, 1414.913526845469960, 198.0875664529170024 ) ) ;
#34568=CARTESIAN_POINT ( 'NONE',  ( 7.341327630490000367, 1451.411706688430058, 153.5270054828980051 ) ) ;
#34569=CARTESIAN_POINT ( 'NONE',  ( -27.27513993222922295, 1509.144914828118999, 212.0641667297481945 ) ) ;
#34571=FACE_OUTER_BOUND ( 'NONE', #77602, .T. ) ;
#34572=EDGE_LOOP ( 'NONE', ( #101223, #62614, #19329, #37807 ) ) ;
#34573=CARTESIAN_POINT ( 'NONE',  ( -18.49678403027447970, 1458.777394600179377, 227.6249456275781995 ) ) ;
#34578=VERTEX_POINT ( 'NONE', #49147 ) ;
#34579=CARTESIAN_POINT ( 'NONE',  ( 18.40016863884620335, 1509.233986100049833, 231.0028230578649868 ) ) ;
#34581=CARTESIAN_POINT ( 'NONE',  ( 38.18239218310520044, 1438.793797181449918, 136.6214554205140246 ) ) ;
#34582=CARTESIAN_POINT ( 'NONE',  ( 22.03740498310000007, 1506.809279316830043, 209.0321213382090093 ) ) ;
#34583=CARTESIAN_POINT ( 'NONE',  ( -34.21122884870000291, 1452.338597683630042, 254.6787128983980040 ) ) ;
#34584=EDGE_CURVE ( 'NONE', #18765, #59443, #68509, .T. ) ;
#34588=CARTESIAN_POINT ( 'NONE',  ( 41.65810716170000205, 1443.954329772089977, 135.6863066689980144 ) ) ;
#34590=CARTESIAN_POINT ( 'NONE',  ( 2.251183906690000125, 1409.929084408430072, 185.5254149766979879 ) ) ;
#34591=CARTESIAN_POINT ( 'NONE',  ( 0.3440135400725780057, 1508.975747044360105, 179.3936242082560000 ) ) ;
#34592=CARTESIAN_POINT ( 'NONE',  ( -5.820774585580000604, 1441.874794574320049, 154.7773490368980163 ) ) ;
#34596=CARTESIAN_POINT ( 'NONE',  ( -3.284456177274770017, 1450.616812660400001, 184.8091138726430245 ) ) ;
#34597=CARTESIAN_POINT ( 'NONE',  ( 0.7047506966600000089, 1466.680917148029948, 235.5111193182980003 ) ) ;
#34600=CARTESIAN_POINT ( 'NONE',  ( -42.85030031610000378, 1442.445295568030133, 270.2009491864980077 ) ) ;
#34601=CARTESIAN_POINT ( 'NONE',  ( -23.73562864992240051, 1436.101657882206609, 211.7975321304884062 ) ) ;
#34602=CARTESIAN_POINT ( 'NONE',  ( 16.63506016420000222, 1409.493969489730034, 224.1775087685979884 ) ) ;
#34604=CARTESIAN_POINT ( 'NONE',  ( -2.970495864810880160E-09, 1471.612866569869993, 258.0852669518579887 ) ) ;
#34606=CARTESIAN_POINT ( 'NONE',  ( -1.549353400650000046, 1416.067629296030191, 227.8551223243979962 ) ) ;
#34607=CARTESIAN_POINT ( 'NONE',  ( -9.828586186369999922, 1419.295296778730062, 230.7940941524979905 ) ) ;
#34610=CARTESIAN_POINT ( 'NONE',  ( -0.1353638497925449269, 1486.099632963759177, 181.8223423097216482 ) ) ;
#34612=CARTESIAN_POINT ( 'NONE',  ( -45.83221320203880111, 1439.239226866460058, 266.4138812322049716 ) ) ;
#34613=CARTESIAN_POINT ( 'NONE',  ( -3.083980574099999927, 1426.000842419329956, 185.7246353708979996 ) ) ;
#34622=CARTESIAN_POINT ( 'NONE',  ( -26.80483817892169895, 1451.972128888919997, 135.0832124891520039 ) ) ;
#34626=CARTESIAN_POINT ( 'NONE',  ( 15.80679505899999704, 1506.802866779429905, 193.5570146056979866 ) ) ;
#34627=EDGE_CURVE ( 'NONE', #98127, #48829, #37755, .T. ) ;
#34629=CARTESIAN_POINT ( 'NONE',  ( -22.41760174960000285, 1433.133604864480048, 211.9349560710080027 ) ) ;
#34631=DIRECTION ( 'NONE',  ( -0.3282391760791589785, 0.000000000000000000, -0.9445946449598763284 ) ) ;
#34633=ORIENTED_EDGE ( 'NONE', *, *, #30262, .F. ) ;
#34634=CARTESIAN_POINT ( 'NONE',  ( -1.808643355405459952, 1409.804319575560157, 270.0715077186459894 ) ) ;
#34636=CARTESIAN_POINT ( 'NONE',  ( 12.56618776640000057, 1419.039214449530164, 229.1641305307979906 ) ) ;
#34640=ORIENTED_EDGE ( 'NONE', *, *, #82333, .T. ) ;
#34641=CARTESIAN_POINT ( 'NONE',  ( -23.61214897399189994, 1410.728070274019956, 210.3394959279470129 ) ) ;
#34644=CARTESIAN_POINT ( 'NONE',  ( -2.205156445730000137, 1428.435894572430016, 91.31218443469779800 ) ) ;
#34645=CARTESIAN_POINT ( 'NONE',  ( -18.92589261422770264, 1440.479205312120030, 194.3132821826760050 ) ) ;
#34646=CARTESIAN_POINT ( 'NONE',  ( -21.44238663129999978, 1420.826072400230260, 218.5102530039179953 ) ) ;
#34647=CARTESIAN_POINT ( 'NONE',  ( 35.50728543074449561, 1462.949734127829970, 266.4725766108469998 ) ) ;
#34648=CARTESIAN_POINT ( 'NONE',  ( -2.694550232742050078, 1466.860812160213754, 235.1051272382491106 ) ) ;
#34649=CARTESIAN_POINT ( 'NONE',  ( -16.05250651547230945, 1420.807636012746570, 227.0341330612096158 ) ) ;
#34652=CARTESIAN_POINT ( 'NONE',  ( 18.61165322248807996, 1458.518385769609040, 227.4849388126852148 ) ) ;
#34657=CARTESIAN_POINT ( 'NONE',  ( 26.74463060723959984, 1450.709319562289920, 136.4676450310559801 ) ) ;
#34661=CARTESIAN_POINT ( 'NONE',  ( 18.03239664030000000, 1409.542765553830122, 196.5032867080979884 ) ) ;
#34662=CARTESIAN_POINT ( 'NONE',  ( 13.76936860679999874, 1443.913060387329097, 176.3340081878980641 ) ) ;
#34663=CARTESIAN_POINT ( 'NONE',  ( 6.302973467031479871, 1409.133165070860059, 188.4343998575660066 ) ) ;
#34665=CARTESIAN_POINT ( 'NONE',  ( -23.23380771384215393, 1433.713381843580237, 214.0813135894918560 ) ) ;
#34666=CARTESIAN_POINT ( 'NONE',  ( 0.9766799065800328972, 1451.035295161389968, 182.3741153617290252 ) ) ;
#34669=LINE ( 'NONE', #35224, #51738 ) ;
#34670=ORIENTED_EDGE ( 'NONE', *, *, #67993, .F. ) ;
#34671=CARTESIAN_POINT ( 'NONE',  ( 11.49746945757270034, 1414.913060387399810, 220.3426859905620177 ) ) ;
#34679=CARTESIAN_POINT ( 'NONE',  ( -31.70762145559999468, 1463.873751786229832, 271.1218459616979999 ) ) ;
#34681=CARTESIAN_POINT ( 'NONE',  ( 11.76781850380000094, 1433.613318462829966, 150.8452650320979842 ) ) ;
#34682=DIRECTION ( 'NONE',  ( -0.9999999999901589831, -4.435753632623349643E-06, 7.907321890110700723E-08 ) ) ;
#34683=CARTESIAN_POINT ( 'NONE',  ( 12.03795434198629977, 1414.913057855109855, 197.8276465654620040 ) ) ;
#34688=CARTESIAN_POINT ( 'NONE',  ( -5.874389180599999705, 1486.518516977929949, 182.2223446999980183 ) ) ;
#34689=CARTESIAN_POINT ( 'NONE',  ( 11.91596713793072126, 1398.266359275336981, 214.3189465422430828 ) ) ;
#34690=CARTESIAN_POINT ( 'NONE',  ( -21.82221913530460000, 1509.753632376169890, 231.7352721600289840 ) ) ;
#34692=DIRECTION ( 'NONE',  ( 0.03489949670250328678, 0.9993908270190956511, 0.000000000000000000 ) ) ;
#34693=CARTESIAN_POINT ( 'NONE',  ( 26.30126752569496418, 1436.707550332054780, 136.8509528689714898 ) ) ;
#34695=CARTESIAN_POINT ( 'NONE',  ( 11.28309680436896834, 1434.414735108999821, 151.5611147865129169 ) ) ;
#34701=VERTEX_POINT ( 'NONE', #43498 ) ;
#34703=CARTESIAN_POINT ( 'NONE',  ( -34.00767267269074523, 1444.324653571828776, 154.9192896682974663 ) ) ;
#34704=ADVANCED_FACE ( 'NONE', ( #94996 ), #67938, .F. ) ;
#34712=CARTESIAN_POINT ( 'NONE',  ( -14.74831627590000060, 1414.913060387329779, 216.2126386790480126 ) ) ;
#34717=CARTESIAN_POINT ( 'NONE',  ( -5.370514330159649852, 1422.356910281434239, 139.1416123588654727 ) ) ;
#34721=CARTESIAN_POINT ( 'NONE',  ( 2.689344463419570452, 1464.716346866380036, 236.9361821190090041 ) ) ;
#34724=FACE_OUTER_BOUND ( 'NONE', #29751, .T. ) ;
#34726=CARTESIAN_POINT ( 'NONE',  ( -2.500000000000000000, 1448.894380913990062, 183.1110264324979937 ) ) ;
#34734=CARTESIAN_POINT ( 'NONE',  ( 36.12323184972498069, 1456.485569746546389, 269.5474412128850190 ) ) ;
#34736=CARTESIAN_POINT ( 'NONE',  ( 18.88366234174538860, 1437.295717261725713, 213.5084043479270974 ) ) ;
#34744=CARTESIAN_POINT ( 'NONE',  ( 2.704720143340000327, 1447.053020108410010, 167.4681767528979890 ) ) ;
#34750=CARTESIAN_POINT ( 'NONE',  ( 40.34236413014900080, 1444.188521476819915, 137.0964790503469999 ) ) ;
#34753=CARTESIAN_POINT ( 'NONE',  ( -24.05801048130000197, 1430.354717888529876, 205.3269550452980070 ) ) ;
#34754=CARTESIAN_POINT ( 'NONE',  ( -10.12873630343129960, 1425.173784052110250, 102.3098040917019915 ) ) ;
#34755=CARTESIAN_POINT ( 'NONE',  ( 16.89642274560129920, 1409.876247450909887, 192.5027543463019981 ) ) ;
#34757=EDGE_CURVE ( 'NONE', #86293, #28591, #51038, .T. ) ;
#34758=CARTESIAN_POINT ( 'NONE',  ( 26.93887127448497765, 1509.966274285299505, 195.8255540051888772 ) ) ;
#34759=B_SPLINE_CURVE_WITH_KNOTS ( 'NONE', 3,
 ( #209, #52262, #86387, #95349, #93661, #17499, #34333, #104299, #16942, #68511, #9675, #51696, #85837 ),
 .UNSPECIFIED., .F., .F.,
 ( 4, 2, 2, 1, 2, 2, 4 ),
 ( 0.000000000000000000, 0.2500000000001801892, 0.3750000000003406719, 0.4375000000004209411, 0.4687500000003957390, 0.5000000000003705924, 1.000000000000000000 ),
 .UNSPECIFIED. ) ;
#34760=CARTESIAN_POINT ( 'NONE',  ( -19.70592387159999959, 1434.997135647919777, 208.2149306268859732 ) ) ;
#34762=CARTESIAN_POINT ( 'NONE',  ( 28.35149942427150194, 1508.694958909449952, 209.4206421715829833 ) ) ;
#34765=CARTESIAN_POINT ( 'NONE',  ( -38.73227730840289951, 1439.373716823020004, 136.6705320380260105 ) ) ;
#34767=CARTESIAN_POINT ( 'NONE',  ( 10.99547339623849851, 1397.334305137690080, 216.7175448681140040 ) ) ;
#34769=CARTESIAN_POINT ( 'NONE',  ( -17.64460054589999771, 1459.279091107629938, 228.2703492655979858 ) ) ;
#34772=B_SPLINE_CURVE_WITH_KNOTS ( 'NONE', 3,
 ( #106551, #11944, #20328, #36593, #64025, #96503, #21413, #13019, #54532, #79717, #95949, #55624 ),
 .UNSPECIFIED., .F., .F.,
 ( 4, 2, 1, 1, 2, 2, 4 ),
 ( 0.000000000000000000, 0.2499999999993910982, 0.3749999999990865640, 0.4374999999989341304, 0.4687499999988572474, 0.4999999999987803645, 1.000000000000000000 ),
 .UNSPECIFIED. ) ;
#34773=CIRCLE ( 'NONE', #97280, 40.51314971913410545 ) ;
#34775=CARTESIAN_POINT ( 'NONE',  ( -9.364590633786502138, 1429.570621513040123, 153.1245166651970067 ) ) ;
#34777=FACE_OUTER_BOUND ( 'NONE', #70461, .T. ) ;
#34780=CARTESIAN_POINT ( 'NONE',  ( -13.10038389319999830, 1470.475446589029843, 230.9320392344980064 ) ) ;
#34789=CARTESIAN_POINT ( 'NONE',  ( 11.76802314650979930, 1427.065976753699942, 146.2965458495970097 ) ) ;
#34791=VERTEX_POINT ( 'NONE', #55219 ) ;
#34792=CARTESIAN_POINT ( 'NONE',  ( 10.73506988043325627, 1424.972993549859893, 139.1354236083641922 ) ) ;
#34793=CARTESIAN_POINT ( 'NONE',  ( -11.19477969735920020, 1432.344513997310059, 151.5793346050809873 ) ) ;
#34794=CARTESIAN_POINT ( 'NONE',  ( 9.235801728380000242, 1509.178085974530177, 236.1490528632979817 ) ) ;
#34796=CARTESIAN_POINT ( 'NONE',  ( -5.196096933339999779, 1423.860580957830052, 185.9637380877979922 ) ) ;
#34797=CARTESIAN_POINT ( 'NONE',  ( 6.437126619989999909, 1408.573915340330132, 270.3863109990980433 ) ) ;
#34800=CARTESIAN_POINT ( 'NONE',  ( -15.22113058945292252, 1410.816735285091454, 190.8741554679031651 ) ) ;
#34802=CARTESIAN_POINT ( 'NONE',  ( -15.27240770310000073, 1451.322057353730088, 222.8125034062979921 ) ) ;
#34803=CARTESIAN_POINT ( 'NONE',  ( 17.41558615450000147, 1458.233052838630101, 229.8710874142980174 ) ) ;
#34805=CARTESIAN_POINT ( 'NONE',  ( -5.026496579103560514, 1422.965951282957121, 184.8230535773238046 ) ) ;
#34808=CARTESIAN_POINT ( 'NONE',  ( 0.02089856015480650100, 1507.111761549349922, 237.3522809668369860 ) ) ;
#34810=DIRECTION ( 'NONE',  ( 0.000000000000000000, 1.000000000000000000, 0.000000000000000000 ) ) ;
#34812=CARTESIAN_POINT ( 'NONE',  ( -2.927822177874543907, 1485.046176849765743, 183.1207224758785799 ) ) ;
#34815=ORIENTED_EDGE ( 'NONE', *, *, #31524, .T. ) ;
#34816=CARTESIAN_POINT ( 'NONE',  ( 1.539250766859999953, 1434.996842493070062, 189.4157229410979824 ) ) ;
#34817=CARTESIAN_POINT ( 'NONE',  ( -15.17327376173290077, 1507.614846683550240, 191.8716176117989960 ) ) ;
#34818=CARTESIAN_POINT ( 'NONE',  ( -11.23709411539999969, 1427.780306893930174, 149.8953276417979907 ) ) ;
#34819=CARTESIAN_POINT ( 'NONE',  ( 19.25040279134129761, 1456.938452318830059, 224.7542541199149753 ) ) ;
#34820=FACE_OUTER_BOUND ( 'NONE', #34342, .T. ) ;
#34823=PLANE ( 'NONE',  #64059 ) ;
#34826=CARTESIAN_POINT ( 'NONE',  ( -16.17675210188999912, 1459.146314904164228, 230.7168972899330015 ) ) ;
#34828=CARTESIAN_POINT ( 'NONE',  ( 23.70172896860000122, 1410.698151209229991, 267.2984425158979889 ) ) ;
#34829=CARTESIAN_POINT ( 'NONE',  ( 24.00431267890000342, 1435.335553928009858, 137.4619543163979927 ) ) ;
#34831=CARTESIAN_POINT ( 'NONE',  ( 18.83143426909999718, 1449.734590623980012, 191.7271620068980269 ) ) ;
#34832=CARTESIAN_POINT ( 'NONE',  ( 17.49859608733503435, 1506.366982236113927, 222.3988492512606001 ) ) ;
#34833=CARTESIAN_POINT ( 'NONE',  ( -0.1289163742206849983, 1508.852627678509862, 238.3730907446190201 ) ) ;
#34835=CARTESIAN_POINT ( 'NONE',  ( -1.218484027960000216, 1451.352790356229889, 183.4814141646979806 ) ) ;
#34836=DIRECTION ( 'NONE',  ( 0.9995237784460414554, 0.03085800254233316345, -2.148909692663481157E-07 ) ) ;
#34838=CARTESIAN_POINT ( 'NONE',  ( -13.40733795300000075, 1443.346361125539943, 187.0475323698980219 ) ) ;
#34840=CARTESIAN_POINT ( 'NONE',  ( -31.77787794420000012, 1436.502309427420187, 136.5769674634980220 ) ) ;
#34844=CARTESIAN_POINT ( 'NONE',  ( -14.26819836422360055, 1409.411316853469771, 213.5416273160190030 ) ) ;
#34845=B_SPLINE_SURFACE_WITH_KNOTS ( 'NONE', 5, 5, ( 
 ( #54537, #52866, #86993, #70245, #96508, #20333, #46130, #19213, #3577 ),
 ( #10282, #53416, #44459, #87567, #79174, #36597, #70795, #28196, #104908 ),
 ( #19788, #3029, #37155, #71904, #106020, #105462, #28752, #100354, #40993 ),
 ( #30391, #57284, #39348, #107102, #91412, #29843, #23642, #72964, #6833 ),
 ( #56710, #98143, #4650, #57824, #74619, #40443, #108199, #82461, #81336 ),
 ( #64029, #14689, #56153, #108754, #31487, #32046, #48878, #89751, #74070 ) ),
 .UNSPECIFIED., .F., .F., .F.,
 ( 6, 6 ),
 ( 6, 3, 6 ),
 ( 7.734716563360000130, 13.39941603910000012 ),
 ( -5.551115123129999410E-17, 1.000000000000000000, 2.000000000000000000 ),
 .UNSPECIFIED. ) ;
#34849=CARTESIAN_POINT ( 'NONE',  ( -9.884517834100000400, 1475.002332015830007, 269.0083476225979666 ) ) ;
#34852=CARTESIAN_POINT ( 'NONE',  ( -24.21504902646103119, 1444.549419358813111, 211.4668081895553655 ) ) ;
#34855=CARTESIAN_POINT ( 'NONE',  ( 18.51177196075189713, 1425.457256880149998, 226.0354587072230004 ) ) ;
#34856=B_SPLINE_CURVE_WITH_KNOTS ( 'NONE', 5,
 ( #36676, #97678, #28830, #63028, #45657, #53496 ),
 .UNSPECIFIED., .F., .F.,
 ( 6, 6 ),
 ( 0.000000000000000000, 1.000000000000000000 ),
 .UNSPECIFIED. ) ;
#34857=CARTESIAN_POINT ( 'NONE',  ( -6.661338147749999709E-15, 1443.913060387330006, 155.8032249175980155 ) ) ;
#34858=B_SPLINE_CURVE_WITH_KNOTS ( 'NONE', 3,
 ( #46506, #29672, #63856, #13960 ),
 .UNSPECIFIED., .F., .F.,
 ( 4, 4 ),
 ( -87.06999293020000152, -29.77037676858719806 ),
 .UNSPECIFIED. ) ;
#34862=CARTESIAN_POINT ( 'NONE',  ( -23.60058029740000052, 1410.232510812830014, 207.4740788330479973 ) ) ;
#34863=CARTESIAN_POINT ( 'NONE',  ( 16.96258621739999839, 1415.088016306429836, 208.8510859400770130 ) ) ;
#34866=B_SPLINE_SURFACE_WITH_KNOTS ( 'NONE', 5, 5, ( 
 ( #58259, #101315, #17306, #68329, #100774, #24608, #51501, #86199, #9490, #24065, #25720, #85634, #75066, #34144, #109750, #109216, #25168, #33572, #66671, #94041, #92379, #84542, #67219, #15652, #33029, #83991, #9 ),
 ( #8934, #58802, #16213, #59372, #93483, #42001, #77267, #565, #42545, #7830, #110295, #85085, #67764, #50958, #45878, #79471, #61038, #96264, #69433, #2781, #36901, #61576, #2235, #27955, #71095, #10044, #62707 ),
 ( #78360, #104106, #1117, #105220, #44215, #28508, #1668, #45333, #35247, #96827, #80014, #62138, #20096, #36349, #10609, #53748, #88413, #18418, #95709, #27394, #54289, #11705, #103548, #69991, #43656, #52617, #86755 ),
 ( #87882, #77808, #44778, #18975, #26850, #53171, #35809, #95160, #87313, #78928, #70541, #104658, #19540, #11173, #59725, #110659, #102792, #34509, #388, #42355, #75962, #42923, #67582, #76509, #44026, #86015, #7648 ),
 ( #84358, #110114, #78163, #102256, #93845, #50230, #26650, #32840, #41804, #33386, #59185, #33952, #85442, #58622, #101688, #103348, #68146, #77080, #68685, #17117, #24979, #84897, #51879, #25535, #51305, #92753, #26088 ),
 ( #60278, #93304, #8740, #16566, #94396, #17676, #50760, #9315, #43478, #77622, #69239, #934, #35058, #67033, #60849, #8189, #94974, #86564, #18242, #52437, #9859, #101140, #24434, #16031, #12623, #46801, #97173 ) ),
 .UNSPECIFIED., .F., .F., .F.,
 ( 6, 6 ),
 ( 6, 3, 3, 3, 3, 3, 3, 3, 6 ),
 ( 2.214628065779999933, 99.53245534309999698 ),
 ( 27.66703431970000082, 34.17017219750000123, 36.60162405460000201, 37.81734998310000151, 38.42521294739999860, 39.03307591160000101, 39.44313445259999895, 39.85319299350000222, 40.67331007530000164 ),
 .UNSPECIFIED. ) ;
#34867=CARTESIAN_POINT ( 'NONE',  ( 5.551115123129999164E-15, 1443.913060387330006, 150.8032249175980155 ) ) ;
#34871=CARTESIAN_POINT ( 'NONE',  ( -21.13431233169999857, 1409.651086836630157, 211.8287207610080145 ) ) ;
#34877=CARTESIAN_POINT ( 'NONE',  ( -0.3434805840468270199, 1419.890415353459957, 184.4011449006650025 ) ) ;
#34882=CARTESIAN_POINT ( 'NONE',  ( 2.301262189390000046, 1508.993422234030049, 237.8174349189979750 ) ) ;
#34887=CARTESIAN_POINT ( 'NONE',  ( 11.90437301253190050, 1433.618833607449915, 150.4807851880309784 ) ) ;
#34888=CARTESIAN_POINT ( 'NONE',  ( 26.88198749810000265, 1509.167631437430146, 216.0681759784479823 ) ) ;
#34894=DIRECTION ( 'NONE',  ( -8.600353058048917082E-15, 1.000000000000000000, 0.000000000000000000 ) ) ;
#34895=CARTESIAN_POINT ( 'NONE',  ( 6.742596065479999901, 1428.329919402730184, 101.8807690336980016 ) ) ;
#34896=CARTESIAN_POINT ( 'NONE',  ( 13.95343569979999998, 1507.808995617830078, 232.8046479664980097 ) ) ;
#34897=CARTESIAN_POINT ( 'NONE',  ( 0.6607295372420000090, 1507.643385047829952, 180.9543164539980182 ) ) ;
#34899=LINE ( 'NONE', #10250, #76882 ) ;
#34902=CARTESIAN_POINT ( 'NONE',  ( 35.12295699368850421, 1435.816162438370156, 134.0999999976959884 ) ) ;
#34903=AXIS2_PLACEMENT_3D ( 'NONE', #68408, #7371, #41534 ) ;
#34904=CARTESIAN_POINT ( 'NONE',  ( 11.29532840559999940, 1431.858520139869825, 151.5063415908980176 ) ) ;
#34907=CARTESIAN_POINT ( 'NONE',  ( 13.91387582277720014, 1435.949825113400038, 150.1916920758069978 ) ) ;
#34910=ORIENTED_EDGE ( 'NONE', *, *, #34433, .F. ) ;
#34911=ADVANCED_FACE ( 'NONE', ( #47352 ), #64743, .F. ) ;
#34913=CARTESIAN_POINT ( 'NONE',  ( -1.489041045350000037, 1466.651558513829968, 235.3699858007980197 ) ) ;
#34924=CARTESIAN_POINT ( 'NONE',  ( -1.543833121739990100, 1424.175334750540060, 228.3471663839470125 ) ) ;
#34925=ORIENTED_EDGE ( 'NONE', *, *, #67215, .T. ) ;
#34926=CARTESIAN_POINT ( 'NONE',  ( -12.82273990640000072, 1409.360840331729833, 190.7207006441979900 ) ) ;
#34928=CARTESIAN_POINT ( 'NONE',  ( -7.052967567875161770, 1427.664849047028611, 134.0999999980979851 ) ) ;
#34930=CARTESIAN_POINT ( 'NONE',  ( 22.87026108289999726, 1432.627911869309855, 216.8958265276880297 ) ) ;
#34937=CARTESIAN_POINT ( 'NONE',  ( -20.83047217639999715, 1508.917604325230059, 190.1019414035980049 ) ) ;
#34938=CARTESIAN_POINT ( 'NONE',  ( 29.78122808599999871, 1510.000412735329974, 208.8654317619979963 ) ) ;
#34944=EDGE_CURVE ( 'NONE', #20305, #19532, #19629, .T. ) ;
#34947=CARTESIAN_POINT ( 'NONE',  ( 12.45246947889999944, 1471.374055768729932, 259.9010460380980589 ) ) ;
#34948=EDGE_CURVE ( 'NONE', #18861, #75410, #52185, .T. ) ;
#34949=DIRECTION ( 'NONE',  ( -0.9401064044234715977, -0.2476038136701678993, 0.2342910579129318938 ) ) ;
#34950=CARTESIAN_POINT ( 'NONE',  ( -29.17964204711229925, 1509.932035941090135, 212.3228751013100180 ) ) ;
#34952=CARTESIAN_POINT ( 'NONE',  ( -5.516207685745849965, 1508.892374888589984, 237.2164510697560047 ) ) ;
#34953=CARTESIAN_POINT ( 'NONE',  ( -19.74442643889999971, 1455.875379726729989, 227.8590200344979735 ) ) ;
#34954=DIRECTION ( 'NONE',  ( 1.499379627120000069E-16, 0.000000000000000000, 1.000000000000000000 ) ) ;
#34955=CARTESIAN_POINT ( 'NONE',  ( 17.92730072119849893, 1410.437638468129990, 222.9214644749860099 ) ) ;
#34961=CARTESIAN_POINT ( 'NONE',  ( 29.11003140420000079, 1509.929605083930028, 206.3377952053380113 ) ) ;
#34963=CARTESIAN_POINT ( 'NONE',  ( 13.15366522099999891, 1428.703228679430140, 223.0784815107979853 ) ) ;
#34968=CARTESIAN_POINT ( 'NONE',  ( 27.05706547295939757, 1436.771164537570030, 136.7742348819220126 ) ) ;
#34969=CARTESIAN_POINT ( 'NONE',  ( 35.10515667903409565, 1450.286879874510078, 136.2298007626710046 ) ) ;
#34970=CARTESIAN_POINT ( 'NONE',  ( -41.91367227552535013, 1454.443418938217519, 269.0780518638181888 ) ) ;
#34974=EDGE_CURVE ( 'NONE', #30773, #11858, #58898, .T. ) ;
#34975=CIRCLE ( 'NONE', #77907, 95.87902122902171698 ) ;
#34978=CARTESIAN_POINT ( 'NONE',  ( -3.677837710089999800E-15, 1426.566393376330097, 144.1938086916980239 ) ) ;
#34979=CARTESIAN_POINT ( 'NONE',  ( 13.50143743689999987, 1434.968984401219814, 146.9207468050980196 ) ) ;
#34980=EDGE_CURVE ( 'NONE', #65067, #67251, #65716, .T. ) ;
#34982=CARTESIAN_POINT ( 'NONE',  ( 16.40780854804009792, 1490.854571769470112, 188.6199282104909969 ) ) ;
#34983=CARTESIAN_POINT ( 'NONE',  ( -8.692880859580000054E-10, 1475.561145520330001, 269.2947192204980524 ) ) ;
#34986=CARTESIAN_POINT ( 'NONE',  ( -28.79939865020000056, 1509.589074244230005, 208.7222596598339805 ) ) ;
#34989=CARTESIAN_POINT ( 'NONE',  ( -11.16241964406192366, 1418.574901742673774, 229.3346417604220449 ) ) ;
#34990=CARTESIAN_POINT ( 'NONE',  ( -17.35267690140000241, 1414.988017870030035, 207.7949262546180194 ) ) ;
#34991=CARTESIAN_POINT ( 'NONE',  ( -13.80599379854099951, 1434.979619881170038, 146.4346930281899972 ) ) ;
#34992=CARTESIAN_POINT ( 'NONE',  ( 25.23965222440000034, 1435.378833613199731, 135.6964465882980164 ) ) ;
#34994=DIRECTION ( 'NONE',  ( 0.9822959463214659959, 0.1391731009602450164, 0.1254014426134129889 ) ) ;
#34996=CARTESIAN_POINT ( 'NONE',  ( -17.16958586411000098, 1410.457766366860142, 225.9676320225469794 ) ) ;
#34997=CARTESIAN_POINT ( 'NONE',  ( 7.419509149259999603, 1440.444625599219989, 149.7273825585979807 ) ) ;
#35001=B_SPLINE_CURVE_WITH_KNOTS ( 'NONE', 3,
 ( #2990, #105423, #28714, #87528, #105984, #78568, #55038, #55587, #70757, #4079, #62920, #54497, #46638, #38204 ),
 .UNSPECIFIED., .F., .F.,
 ( 4, 2, 1, 1, 1, 1, 2, 2, 4 ),
 ( 0.000000000000000000, 0.2500000000002161049, 0.3750000000003220202, 0.4375000000003748113, 0.4687500000004317102, 0.4843750000004864997, 0.4921875000005116463, 0.5000000000005367928, 1.000000000000000000 ),
 .UNSPECIFIED. ) ;
#35003=CARTESIAN_POINT ( 'NONE',  ( 10.94214974360000170, 1426.073836398730009, 94.99432300369781501 ) ) ;
#35005=CARTESIAN_POINT ( 'NONE',  ( -0.1147974981524840093, 1507.118024595949919, 237.3465355752350092 ) ) ;
#35006=CARTESIAN_POINT ( 'NONE',  ( -2.515127511734718713, 1421.311320163850723, 184.3934076788736434 ) ) ;
#35009=CARTESIAN_POINT ( 'NONE',  ( 7.817147024559999657, 1507.298328921630173, 182.8873992191979880 ) ) ;
#35010=CARTESIAN_POINT ( 'NONE',  ( 3.686666017499999892, 1448.977420087960127, 184.1966211689980071 ) ) ;
#35016=CARTESIAN_POINT ( 'NONE',  ( -40.27000727579999761, 1443.958079488249950, 137.1320871855979817 ) ) ;
#35019=CARTESIAN_POINT ( 'NONE',  ( -0.9513828761539999679, 1471.786836300230107, 269.8654945467980042 ) ) ;
#35024=CARTESIAN_POINT ( 'NONE',  ( -36.40679663865240201, 1451.403536159749819, 134.6865063755689960 ) ) ;
#35025=B_SPLINE_SURFACE_WITH_KNOTS ( 'NONE', 5, 5, ( 
 ( #89956, #3234, #13230, #4844, #73168, #30606 ),
 ( #37918, #22173, #71562, #72099, #59137, #100555 ),
 ( #15982, #23835, #15435, #93259, #41213, #65881 ),
 ( #75385, #23290, #49627, #108415, #33343, #109522 ),
 ( #32798, #50183, #110617, #76464, #16523, #24927 ),
 ( #33900, #67538, #58027, #74829, #14888, #68095 ),
 ( #49079, #50714, #84844, #74285, #8144, #92162 ),
 ( #84310, #25488, #100002, #24392, #83761, #59679 ),
 ( #58577, #101638, #66982, #42310, #108973, #110067 ) ),
 .UNSPECIFIED., .F., .F., .F.,
 ( 6, 3, 6 ),
 ( 6, 6 ),
 ( 21.34407477379999918, 25.74311937130000061, 30.14216396890000027 ),
 ( 0.000000000000000000, 2.000000000000000000 ),
 .UNSPECIFIED. ) ;
#35026=CARTESIAN_POINT ( 'NONE',  ( -18.88069888589999934, 1519.913060387329779, 196.2596006804980107 ) ) ;
#35028=CARTESIAN_POINT ( 'NONE',  ( 7.143284666917959491, 1409.162509384609848, 195.2043232230670071 ) ) ;
#35029=CARTESIAN_POINT ( 'NONE',  ( -12.08854166899370064, 1407.246857854960126, 268.9879536978270380 ) ) ;
#35030=CARTESIAN_POINT ( 'NONE',  ( -14.14290945506900066, 1435.350905828940085, 149.5435571626070157 ) ) ;
#35032=CARTESIAN_POINT ( 'NONE',  ( -11.86614525289999911, 1432.349253981700031, 150.3971727848980038 ) ) ;
#35033=CARTESIAN_POINT ( 'NONE',  ( 13.24057533709999923, 1444.706717224920112, 187.3823346222980035 ) ) ;
#35036=EDGE_CURVE ( 'NONE', #80080, #99658, #24229, .T. ) ;
#35037=CARTESIAN_POINT ( 'NONE',  ( 5.011594840860459144, 1423.113943537101932, 184.3785993670394987 ) ) ;
#35041=CARTESIAN_POINT ( 'NONE',  ( -8.249097597409999594, 1485.477655575529980, 184.2734846816980223 ) ) ;
#35044=AXIS2_PLACEMENT_3D ( 'NONE', #33910, #347, #24936 ) ;
#35048=CARTESIAN_POINT ( 'NONE',  ( -28.70345826739999850, 1509.590240598730134, 207.9949817522079911 ) ) ;
#35053=B_SPLINE_CURVE_WITH_KNOTS ( 'NONE', 3,
 ( #26691, #53027, #973, #79324, #95562, #94435, #1517, #44066, #35098, #18832 ),
 .UNSPECIFIED., .F., .F.,
 ( 4, 2, 2, 2, 4 ),
 ( 0.000000000000000000, 0.2500000000000000000, 0.5000000000000000000, 0.7500000000000000000, 1.000000000000000000 ),
 .UNSPECIFIED. ) ;
#35054=CARTESIAN_POINT ( 'NONE',  ( -25.74664715480469823, 1449.922850843729975, 208.7294647506780052 ) ) ;
#35055=CARTESIAN_POINT ( 'NONE',  ( -10.72653838659999970, 1445.370122805119991, 185.5580616574980013 ) ) ;
#35056=VERTEX_POINT ( 'NONE', #5900 ) ;
#35058=CARTESIAN_POINT ( 'NONE',  ( 27.70206559570000238, 1508.130759166529742, 212.2772318986179982 ) ) ;
#35060=CARTESIAN_POINT ( 'NONE',  ( -24.06699603970000112, 1435.344051288429910, 136.8276718557980018 ) ) ;
#35062=B_SPLINE_CURVE_WITH_KNOTS ( 'NONE', 3,
 ( #56255, #99331, #41098, #22058, #65767, #24287, #15869, #23736, #15328, #23183, #22605, #13662, #31590, #66337, #74722, #40548, #75277, #39997, #57384, #90946, #109424, #32701, #92056, #66881, #7498, #31037, #91510 ),
 .UNSPECIFIED., .F., .F.,
 ( 4, 2, 2, 1, 1, 1, 1, 2, 2, 2, 2, 1, 1, 1, 2, 2, 4 ),
 ( 0.000000000000000000, 0.06250000000001224021, 0.09375000000001836031, 0.1093750000000226485, 0.1171875000000235367, 0.1210937500000230094, 0.1230468750000218020, 0.1240234375000221212, 0.1250000000000224265, 0.1875000000000156541, 0.2500000000000088818, 0.3749999999999950040, 0.4374999999999895639, 0.4687499999999868994, 0.4843749999999868439, 0.4999999999999867883, 1.000000000000000000 ),
 .UNSPECIFIED. ) ;
#35064=B_SPLINE_CURVE_WITH_KNOTS ( 'NONE', 5,
 ( #96037, #53510, #103885, #62480, #27186, #104994, #69201, #52952, #54075 ),
 .UNSPECIFIED., .F., .F.,
 ( 6, 3, 6 ),
 ( 0.000000000000000000, 0.5333467950542268854, 1.000000000000000000 ),
 .UNSPECIFIED. ) ;
#35067=ADVANCED_FACE ( 'NONE', ( #108357 ), #64266, .F. ) ;
#35070=CARTESIAN_POINT ( 'NONE',  ( -1.873189676845119944, 1451.938853521590090, 184.2960223139319851 ) ) ;
#35071=CARTESIAN_POINT ( 'NONE',  ( -4.146148586359999832, 1410.300477727830184, 232.1600599902980093 ) ) ;
#35073=ADVANCED_FACE ( 'NONE', ( #72984 ), #24963, .T. ) ;
#35077=CARTESIAN_POINT ( 'NONE',  ( 12.44490648448620007, 1434.392432424140225, 149.5192106900200031 ) ) ;
#35078=CARTESIAN_POINT ( 'NONE',  ( 15.33254751237830149, 1488.407451439539955, 231.1339900686130022 ) ) ;
#35079=CARTESIAN_POINT ( 'NONE',  ( -23.80940814504779723, 1509.710483542359952, 225.5335122003920105 ) ) ;
#35080=CARTESIAN_POINT ( 'NONE',  ( -2.242235177520000011, 1409.158574251030132, 187.0303599566979926 ) ) ;
#35082=CARTESIAN_POINT ( 'NONE',  ( 4.240088984218660428, 1441.444059629489857, 162.8289912679279894 ) ) ;
#35085=CARTESIAN_POINT ( 'NONE',  ( 16.42420380379999756, 1507.212883763329955, 193.5443561786979956 ) ) ;
#35090=CARTESIAN_POINT ( 'NONE',  ( -0.7275771281559999526, 1495.113783641829968, 181.2733469408979943 ) ) ;
#35092=CARTESIAN_POINT ( 'NONE',  ( 3.797937935320000236, 1421.119554740329932, 185.2659206367980005 ) ) ;
#35098=CARTESIAN_POINT ( 'NONE',  ( -16.04005855938789793, 1409.473190815148428, 192.8190731777143583 ) ) ;
#35099=CARTESIAN_POINT ( 'NONE',  ( 17.77615777719999812, 1415.140114695929924, 210.2708809818280145 ) ) ;
#35103=DIRECTION ( 'NONE',  ( 0.000000000000000000, 0.000000000000000000, -1.000000000000000000 ) ) ;
#35109=CARTESIAN_POINT ( 'NONE',  ( 24.50139030460000100, 1449.832840726370023, 206.9640024934579969 ) ) ;
#35111=CARTESIAN_POINT ( 'NONE',  ( -24.35760840280000039, 1442.387172707180298, 212.1777659041080142 ) ) ;
#35112=CARTESIAN_POINT ( 'NONE',  ( 7.492276228816673544, 1410.547776690462115, 187.3898987111521706 ) ) ;
#35114=EDGE_CURVE ( 'NONE', #35478, #54360, #55314, .T. ) ;
#35118=VECTOR ( 'NONE', #97170, 1000.000000000000114 ) ;
#35125=CARTESIAN_POINT ( 'NONE',  ( 24.69959934959999970, 1509.552027989230055, 195.6047229538980048 ) ) ;
#35126=VERTEX_POINT ( 'NONE', #36616 ) ;
#35127=CARTESIAN_POINT ( 'NONE',  ( -18.41935412833382202, 1458.939734570434439, 227.7070353066069401 ) ) ;
#35132=CARTESIAN_POINT ( 'NONE',  ( 12.96054471030000066, 1446.716588664140090, 188.5511171461979814 ) ) ;
#35134=CARTESIAN_POINT ( 'NONE',  ( 39.22710209691519623, 1440.047129195570051, 136.7325733605709956 ) ) ;
#35136=CARTESIAN_POINT ( 'NONE',  ( 19.13335938739999875, 1434.810047171419910, 209.3864841450680103 ) ) ;
#35137=CARTESIAN_POINT ( 'NONE',  ( -35.25149193259999691, 1460.997979651529931, 264.2529779472980067 ) ) ;
#35141=CARTESIAN_POINT ( 'NONE',  ( -20.11941513109999846, 1485.685652062829831, 190.9455850217979958 ) ) ;
#35142=CARTESIAN_POINT ( 'NONE',  ( 1.987580315000000208, 1408.982468221330009, 186.9241478344979726 ) ) ;
#35147=CARTESIAN_POINT ( 'NONE',  ( 0.02753318172129999575, 1452.474300612129809, 153.7510498093980118 ) ) ;
#35150=CARTESIAN_POINT ( 'NONE',  ( -18.64618896866739561, 1416.835806635407607, 208.5595417920155512 ) ) ;
#35152=CARTESIAN_POINT ( 'NONE',  ( -43.33646147129999804, 1450.475004575490175, 269.7148345228980020 ) ) ;
#35154=CARTESIAN_POINT ( 'NONE',  ( 17.71298018430000099, 1410.454334487929827, 223.4084641196980101 ) ) ;
#35155=DIRECTION ( 'NONE',  ( 0.4794255386042041711, 0.000000000000000000, 0.8775825618903720926 ) ) ;
#35156=CARTESIAN_POINT ( 'NONE',  ( 4.159508860199999880, 1408.913060387329779, 191.2895657749980103 ) ) ;
#35158=CARTESIAN_POINT ( 'NONE',  ( -1.343523894720000111, 1416.547221147930031, 228.0666963329979922 ) ) ;
#35159=CARTESIAN_POINT ( 'NONE',  ( -5.212293933520000699, 1418.055166734629893, 234.1958690057979879 ) ) ;
#35160=CARTESIAN_POINT ( 'NONE',  ( 23.10442895610000136, 1411.095127645030061, 207.3185325968580059 ) ) ;
#35162=CARTESIAN_POINT ( 'NONE',  ( -45.86418412298019831, 1439.840857331170128, 266.4129133962819651 ) ) ;
#35163=CARTESIAN_POINT ( 'NONE',  ( -3.602258143659999856, 1434.225543709759904, 185.6459190021979850 ) ) ;
#35164=ORIENTED_EDGE ( 'NONE', *, *, #38008, .T. ) ;
#35169=CARTESIAN_POINT ( 'NONE',  ( -5.386823041269999557, 1432.449279870900000, 154.6099110731979920 ) ) ;
#35174=CARTESIAN_POINT ( 'NONE',  ( -26.28577179630749683, 1450.928187855339957, 136.5329518447099986 ) ) ;
#35176=CARTESIAN_POINT ( 'NONE',  ( 19.42898398440000207, 1429.237499567630039, 213.0284083449880086 ) ) ;
#35178=CARTESIAN_POINT ( 'NONE',  ( 14.83581816709999934, 1470.804162801829989, 194.6684007568979666 ) ) ;
#35181=EDGE_CURVE ( 'NONE', #8387, #109101, #96935, .T. ) ;
#35185=CARTESIAN_POINT ( 'NONE',  ( -1.826910925121480123, 1409.229992614159983, 270.3712872650569921 ) ) ;
#35187=CARTESIAN_POINT ( 'NONE',  ( 12.53400550999920071, 1420.773202801019806, 231.1418645745110041 ) ) ;
#35188=CARTESIAN_POINT ( 'NONE',  ( -18.80269612420000058, 1449.648705166280024, 192.8065731388979884 ) ) ;
#35192=ORIENTED_EDGE ( 'NONE', *, *, #65155, .T. ) ;
#35194=CARTESIAN_POINT ( 'NONE',  ( -1.234663454762129797, 1409.459554532440052, 185.7565115510559792 ) ) ;
#35196=CARTESIAN_POINT ( 'NONE',  ( -12.08749531470011718, 1407.203987194673573, 266.9030444376613787 ) ) ;
#35197=CARTESIAN_POINT ( 'NONE',  ( -18.94560849849241535, 1436.391938629627930, 146.5415713983334456 ) ) ;
#35198=CARTESIAN_POINT ( 'NONE',  ( -23.20503365730000311, 1430.784771651529809, 213.5757909921379962 ) ) ;
#35199=CARTESIAN_POINT ( 'NONE',  ( 28.14007468020770020, 1467.874185183969985, 269.3927133897410044 ) ) ;
#35200=CARTESIAN_POINT ( 'NONE',  ( -1.923414284749828562, 1466.968210799180270, 235.2882593390983459 ) ) ;
#35204=CARTESIAN_POINT ( 'NONE',  ( 10.96966286673369950, 1432.359740019160199, 151.7701370213850112 ) ) ;
#35206=CARTESIAN_POINT ( 'NONE',  ( 23.02649207640000029, 1409.822863297029926, 208.4031441088459928 ) ) ;
#35208=CARTESIAN_POINT ( 'NONE',  ( -0.7233576412608461181, 1457.980924837309885, 229.7067188217370131 ) ) ;
#35209=ADVANCED_FACE ( 'NONE', ( #65690 ), #101857, .F. ) ;
#35210=CARTESIAN_POINT ( 'NONE',  ( 26.14323217959369927, 1451.983980635410035, 135.2537540905360061 ) ) ;
#35214=CARTESIAN_POINT ( 'NONE',  ( 18.30580500820000012, 1410.476084872329920, 194.0322744968979976 ) ) ;
#35216=CARTESIAN_POINT ( 'NONE',  ( 2.895653292560566250, 1439.669445174284419, 183.9645025138850372 ) ) ;
#35218=CARTESIAN_POINT ( 'NONE',  ( -18.60031629480377902, 1424.402109664954878, 224.8720212759178878 ) ) ;
#35224=CARTESIAN_POINT ( 'NONE',  ( -9.849896899200842881, 1512.913060387330006, 185.5490084180013923 ) ) ;
#35225=VERTEX_POINT ( 'NONE', #73544 ) ;
#35228=CARTESIAN_POINT ( 'NONE',  ( -0.2839359186375919886, 1408.939684095860002, 231.9819584528090104 ) ) ;
#35229=EDGE_CURVE ( 'NONE', #87953, #30631, #64332, .T. ) ;
#35233=CARTESIAN_POINT ( 'NONE',  ( -9.145222436810001909, 1453.522154064730103, 214.3676144192479853 ) ) ;
#35234=CARTESIAN_POINT ( 'NONE',  ( -1.935345215820309939, 1458.401398452629792, 184.0842910492330304 ) ) ;
#35235=CARTESIAN_POINT ( 'NONE',  ( 11.71656231259999892, 1433.390345078600149, 150.8916009587979943 ) ) ;
#35236=CARTESIAN_POINT ( 'NONE',  ( 19.80583385279999931, 1445.467019039670049, 219.6133835737980178 ) ) ;
#35238=CARTESIAN_POINT ( 'NONE',  ( 12.65294384001390071, 1415.935475482089942, 196.4577491575730050 ) ) ;
#35241=CARTESIAN_POINT ( 'NONE',  ( 22.93376428353750285, 1507.619498552430059, 210.5433103207220142 ) ) ;
#35242=CARTESIAN_POINT ( 'NONE',  ( 23.69434222019999936, 1435.324930578030035, 137.3226534152980207 ) ) ;
#35243=CARTESIAN_POINT ( 'NONE',  ( -7.020681098499999884, 1486.251198431629973, 182.5489229859979901 ) ) ;
#35244=CARTESIAN_POINT ( 'NONE',  ( 0.000000000000000000, 1508.913060387330006, 209.1218459616979999 ) ) ;
#35245=CARTESIAN_POINT ( 'NONE',  ( -7.437115572297779309, 1509.172770186120033, 238.4311077084169881 ) ) ;
#35247=CARTESIAN_POINT ( 'NONE',  ( 24.70281711890000054, 1449.797141322859943, 213.6739267561380018 ) ) ;
#35250=CARTESIAN_POINT ( 'NONE',  ( 26.03716339960346104, 1436.680109442058892, 136.9403589541479107 ) ) ;
#35256=CARTESIAN_POINT ( 'NONE',  ( 0.1629390172021479843, 1484.504367874960053, 181.9008776530140210 ) ) ;
#35257=ORIENTED_EDGE ( 'NONE', *, *, #11938, .F. ) ;
#35258=CARTESIAN_POINT ( 'NONE',  ( 0.000000000000000000, 1442.773887286369927, 126.8032249175980155 ) ) ;
#35261=CARTESIAN_POINT ( 'NONE',  ( -35.14989576446389918, 1451.591923343860117, 134.0999999983660018 ) ) ;
#35265=CARTESIAN_POINT ( 'NONE',  ( 0.4116874139510000585, 1416.851343894929869, 190.6255312621979954 ) ) ;
#35268=CARTESIAN_POINT ( 'NONE',  ( -14.27054084439999926, 1415.934222462129810, 221.2887574511979949 ) ) ;
#35277=CARTESIAN_POINT ( 'NONE',  ( -17.39452685740000248, 1413.991076397230017, 192.1659084337979948 ) ) ;
#35278=DIRECTION ( 'NONE',  ( 1.984846884490000055E-13, 0.000000000000000000, -1.000000000000000000 ) ) ;
#35280=CARTESIAN_POINT ( 'NONE',  ( -15.71169620265270161, 1410.111862918789939, 226.5238431294280019 ) ) ;
#35282=ORIENTED_EDGE ( 'NONE', *, *, #7124, .T. ) ;
#35285=CARTESIAN_POINT ( 'NONE',  ( 26.37059714170000291, 1509.833941931429990, 221.6204849630979936 ) ) ;
#35288=CARTESIAN_POINT ( 'NONE',  ( 39.55840597086309884, 1451.233580783764637, 269.6025367666410375 ) ) ;
#35290=CARTESIAN_POINT ( 'NONE',  ( 19.23317556650448523, 1438.816174030696629, 212.7465897691410817 ) ) ;
#35298=CARTESIAN_POINT ( 'NONE',  ( -13.02211328169330073, 1434.883360788459868, 149.7670459028529990 ) ) ;
#35305=CARTESIAN_POINT ( 'NONE',  ( 40.57811333989999980, 1433.211871387559995, 261.6156834470980357 ) ) ;
#35306=CARTESIAN_POINT ( 'NONE',  ( -25.10029913840000049, 1449.799429884400070, 205.9286887820979928 ) ) ;
#35307=CARTESIAN_POINT ( 'NONE',  ( -11.67404807818740053, 1426.321468137869942, 139.7108783720840108 ) ) ;
#35308=CARTESIAN_POINT ( 'NONE',  ( 16.25665712022090048, 1409.489020141060109, 192.9910857566509890 ) ) ;
#35311=CARTESIAN_POINT ( 'NONE',  ( 28.15539526923029001, 1510.007817771240298, 198.7357687764576895 ) ) ;
#35312=CARTESIAN_POINT ( 'NONE',  ( -19.44845634420000025, 1435.008643399710081, 208.5507817201369960 ) ) ;
#35313=CARTESIAN_POINT ( 'NONE',  ( -43.50118323360000261, 1440.913060407490093, 263.8966221483980235 ) ) ;
#35315=CARTESIAN_POINT ( 'NONE',  ( 31.82246047982030390, 1465.839548924079509, 269.9247166951640224 ) ) ;
#35317=CARTESIAN_POINT ( 'NONE',  ( -38.22481880452640013, 1438.834491510689986, 136.6247642330480119 ) ) ;
#35319=CARTESIAN_POINT ( 'NONE',  ( 10.73158195967269890, 1397.616005728979871, 200.3871790473220074 ) ) ;
#35321=CARTESIAN_POINT ( 'NONE',  ( -17.10148908190000228, 1459.927071089530045, 228.3592279236980005 ) ) ;
#35322=ORIENTED_EDGE ( 'NONE', *, *, #16119, .T. ) ;
#35324=AXIS2_PLACEMENT_3D ( 'NONE', #84669, #58941, #57850 ) ;
#35330=CARTESIAN_POINT ( 'NONE',  ( -12.53380580351000084, 1442.773887400870080, 185.9733686700720057 ) ) ;
#35332=CARTESIAN_POINT ( 'NONE',  ( -9.342819160739999518, 1461.186629906429971, 232.5279129794980122 ) ) ;
#35333=CARTESIAN_POINT ( 'NONE',  ( 0.8412646513084379718, 1420.713512048480197, 182.8900134064909935 ) ) ;
#35338=( BOUNDED_CURVE ( )  B_SPLINE_CURVE ( 3, ( #41654, #67983, #35455, #227 ),
 .UNSPECIFIED., .F., .T. ) 
 B_SPLINE_CURVE_WITH_KNOTS ( ( 4, 4 ),
 ( 5.600235996204509625, 5.892581600017769539 ),
 .UNSPECIFIED. ) 
 CURVE ( )  GEOMETRIC_REPRESENTATION_ITEM ( )  RATIONAL_B_SPLINE_CURVE ( ( 1.000000000000000000, 0.9928905095994882135, 0.9928905095994882135, 1.000000000000000000 ) ) 
 REPRESENTATION_ITEM ( '' )  );
#35341=VERTEX_POINT ( 'NONE', #76280 ) ;
#35342=CARTESIAN_POINT ( 'NONE',  ( 11.83526461542720121, 1430.237649493160006, 149.5707587408450081 ) ) ;
#35344=ORIENTED_EDGE ( 'NONE', *, *, #90309, .F. ) ;
#35347=CARTESIAN_POINT ( 'NONE',  ( -13.51812398686054451, 1443.913060387329324, 169.4008117781592375 ) ) ;
#35350=CARTESIAN_POINT ( 'NONE',  ( -5.116133894400000770, 1420.946959116729886, 186.4728714752979783 ) ) ;
#35351=CARTESIAN_POINT ( 'NONE',  ( 2.316388767259710324, 1408.277175035590062, 270.3918176960409596 ) ) ;
#35352=DIRECTION ( 'NONE',  ( 0.9417419115949053898, -0.3363363969979660806, -9.559255346349042767E-16 ) ) ;
#35357=CARTESIAN_POINT ( 'NONE',  ( 17.96021206210000187, 1457.749394617429971, 229.4559061194979961 ) ) ;
#35358=CARTESIAN_POINT ( 'NONE',  ( 14.72777576890000084, 1453.165958253430063, 195.2129441428980101 ) ) ;
#35361=CARTESIAN_POINT ( 'NONE',  ( 17.72240587385099886, 1414.657222584279907, 224.9178048682000224 ) ) ;
#35365=ADVANCED_FACE ( 'NONE', ( #78490 ), #39693, .T. ) ;
#35367=CARTESIAN_POINT ( 'NONE',  ( -2.946552187109835241, 1485.285160343432153, 182.9853163874463462 ) ) ;
#35368=CARTESIAN_POINT ( 'NONE',  ( 0.000000000000000000, 1512.913060387330006, 209.1218459616979999 ) ) ;
#35373=CARTESIAN_POINT ( 'NONE',  ( -10.93704887400000025, 1430.005839323029932, 151.3915896504979912 ) ) ;
#35374=FACE_OUTER_BOUND ( 'NONE', #48977, .T. ) ;
#35379=CARTESIAN_POINT ( 'NONE',  ( 14.58335259939999951, 1410.403800467930068, 227.7087990198979810 ) ) ;
#35382=CARTESIAN_POINT ( 'NONE',  ( -16.17567356680000046, 1459.146941997929844, 230.7169173512979796 ) ) ;
#35384=CARTESIAN_POINT ( 'NONE',  ( 31.40639260020000023, 1415.744722567929784, 269.1485073036980111 ) ) ;
#35385=B_SPLINE_CURVE_WITH_KNOTS ( 'NONE', 3,
 ( #109284, #83501, #100316, #51023, #75136, #23602, #33643, #16822, #48840, #67839, #82964, #40404, #74581, #49924, #84061, #85158, #84607, #109823, #99750, #7358, #92450, #8444, #76770, #6257, #32568, #15723, #84, #66742, #24678, #100845, #33103, #65634, #41523, #24136, #23040, #58875, #93007, #58326, #57244, #7899, #91373, #42071, #85710, #61111, #78429, #17378, #51577, #69501, #86266, #61645, #94667, #103624, #9005, #77331, #43180, #1184 ),
 .UNSPECIFIED., .F., .F.,
 ( 4, 2, 2, 1, 1, 1, 1, 1, 2, 2, 2, 1, 1, 1, 1, 2, 2, 2, 2, 2, 2, 2, 1, 1, 1, 1, 2, 2, 2, 2, 1, 1, 1, 2, 2, 4 ),
 ( 0.000000000000000000, 0.2500000000126188504, 0.3750000000189228633, 0.4375000000220682916, 0.4687500000236474174, 0.4843750000244362308, 0.4921875000248307486, 0.4960937500250203747, 0.4980468750251229593, 0.5000000000252254884, 0.6250000000316919824, 0.6875000000349166251, 0.7187500000365378838, 0.7343750000373484577, 0.7421875000377536891, 0.7460937500379563048, 0.7500000000381589205, 0.8125000000413759027, 0.8437500000429742908, 0.8750000000445727899, 0.8906250000453606042, 0.8984375000457649474, 0.9023437500459566829, 0.9042968750460645966, 0.9052734375461291005, 0.9057617187961615191, 0.9060058594211788385, 0.9062500000461961580, 0.9218750000388737931, 0.9296875000352123886, 0.9335937500333889583, 0.9355468750324835714, 0.9365234375320303783, 0.9370117187817978976, 0.9375000000315654169, 1.000000000000000000 ),
 .UNSPECIFIED. ) ;
#35387=CARTESIAN_POINT ( 'NONE',  ( 0.5800809713973276160, 1465.108713975482033, 238.1055978074999757 ) ) ;
#35388=CARTESIAN_POINT ( 'NONE',  ( 24.29813646699999907, 1449.724010015529984, 206.4560171053380202 ) ) ;
#35389=CARTESIAN_POINT ( 'NONE',  ( -23.60070384349999983, 1435.435992124709855, 213.5551618677380077 ) ) ;
#35390=DIRECTION ( 'NONE',  ( 0.000000000000000000, -0.8505177418130608347, 0.5259463573989380247 ) ) ;
#35392=CARTESIAN_POINT ( 'NONE',  ( -1.280362373440000034, 1451.774120662730184, 183.7183834658980004 ) ) ;
#35394=CARTESIAN_POINT ( 'NONE',  ( -15.81201443571409904, 1506.433683733589987, 193.8503163142329981 ) ) ;
#35396=CARTESIAN_POINT ( 'NONE',  ( -16.56043081341401901, 1409.526309863062124, 193.4350318160313122 ) ) ;
#35397=CARTESIAN_POINT ( 'NONE',  ( -17.23446452470000168, 1453.313060387329870, 219.9051549417980027 ) ) ;
#35398=CARTESIAN_POINT ( 'NONE',  ( -32.74366364859999834, 1436.969577990789730, 136.5975034958979961 ) ) ;
#35402=CARTESIAN_POINT ( 'NONE',  ( -14.54001393154930000, 1409.420808862239937, 212.5391509058709971 ) ) ;
#35404=CARTESIAN_POINT ( 'NONE',  ( -2.478238621609999637, 1439.208302790359994, 157.7515629680979998 ) ) ;
#35405=CARTESIAN_POINT ( 'NONE',  ( -18.18436572850000132, 1472.598912338130049, 269.3834208221979338 ) ) ;
#35406=DIRECTION ( 'NONE',  ( -0.05326577277506865798, 0.03591581246945392547, 0.9979342723172373031 ) ) ;
#35409=CARTESIAN_POINT ( 'NONE',  ( -24.34971616191185007, 1444.638322005277587, 211.2124739967878213 ) ) ;
#35412=CARTESIAN_POINT ( 'NONE',  ( 17.55069790844339650, 1424.280160729299951, 227.8786989819499809 ) ) ;
#35413=CARTESIAN_POINT ( 'NONE',  ( 20.61376621259999808, 1508.366577482129969, 227.7668722788980062 ) ) ;
#35415=CARTESIAN_POINT ( 'NONE',  ( -3.218260492609999801, 1432.346960983880081, 155.4230413404980027 ) ) ;
#35416=CARTESIAN_POINT ( 'NONE',  ( 2.499999999999999556, 1411.429641636930000, 137.0999999980979851 ) ) ;
#35418=CARTESIAN_POINT ( 'NONE',  ( -7.999195660609999869, 1509.131454673530015, 180.7515949602980072 ) ) ;
#35420=CARTESIAN_POINT ( 'NONE',  ( -23.22374811570000119, 1411.084293947430069, 205.4313518788480053 ) ) ;
#35421=CARTESIAN_POINT ( 'NONE',  ( 16.81460438480000263, 1415.425433635630043, 203.9301085955280257 ) ) ;
#35424=CARTESIAN_POINT ( 'NONE',  ( -4.425709718559999041E-15, 1434.541746329560056, 150.4759714514979976 ) ) ;
#35428=CARTESIAN_POINT ( 'NONE',  ( -22.76038230680000041, 1410.633847100929870, 211.2989740808880015 ) ) ;
#35436=CARTESIAN_POINT ( 'NONE',  ( -7.980985505873261054, 1398.150102696605018, 219.3836182790206237 ) ) ;
#35439=CARTESIAN_POINT ( 'NONE',  ( -19.65671673259999963, 1468.978988229229799, 193.1983232643979704 ) ) ;
#35445=CARTESIAN_POINT ( 'NONE',  ( 11.20527203278069805, 1434.214488751450062, 151.6116235837919817 ) ) ;
#35449=CARTESIAN_POINT ( 'NONE',  ( -21.03123196400000339, 1507.789098030929836, 192.1781279194979959 ) ) ;
#35452=CARTESIAN_POINT ( 'NONE',  ( 13.54190757295939918, 1453.249853630250072, 224.6401645295789820 ) ) ;
#35453=CARTESIAN_POINT ( 'NONE',  ( 17.16377242769999967, 1507.812853982129809, 231.0448963225979924 ) ) ;
#35454=CARTESIAN_POINT ( 'NONE',  ( 12.21796603489999988, 1507.632479711529868, 184.8478369543980193 ) ) ;
#35455=CARTESIAN_POINT ( 'NONE',  ( 10.11864553081269058, 1509.266411275488053, 236.5980910735531779 ) ) ;
#35459=CARTESIAN_POINT ( 'NONE',  ( 38.01446494478440030, 1436.977963747790000, 134.0999999969440069 ) ) ;
#35463=CARTESIAN_POINT ( 'NONE',  ( 13.54853135755140059, 1434.978863808960114, 149.0925490114800027 ) ) ;
#35466=ORIENTED_EDGE ( 'NONE', *, *, #88999, .F. ) ;
#35468=CARTESIAN_POINT ( 'NONE',  ( -1.229676403839999876, 1465.032347023129887, 236.8197607516979986 ) ) ;
#35475=CARTESIAN_POINT ( 'NONE',  ( -0.06018804149849999591, 1508.906897381529916, 238.6255503046979811 ) ) ;
#35478=VERTEX_POINT ( 'NONE', #8505 ) ;
#35479=CARTESIAN_POINT ( 'NONE',  ( 23.27833603578599764, 1440.913060387330006, 232.8848930007430056 ) ) ;
#35480=CARTESIAN_POINT ( 'NONE',  ( -19.58834071409999922, 1508.062712279529933, 229.4587154835980130 ) ) ;
#35481=VERTEX_POINT ( 'NONE', #9072 ) ;
#35483=CARTESIAN_POINT ( 'NONE',  ( -14.50832503429999853, 1410.792323590329943, 190.4765598033980041 ) ) ;
#35484=CARTESIAN_POINT ( 'NONE',  ( -24.38537946479999974, 1441.549228787309858, 211.3644968983080048 ) ) ;
#35486=CARTESIAN_POINT ( 'NONE',  ( 0.0002643472464120411708, 1396.497912824548848, 196.7090272551392616 ) ) ;
#35487=DIRECTION ( 'NONE',  ( -5.145681809797982184E-09, 0.03085823632287491500, -0.9995237712285994780 ) ) ;
#35489=CARTESIAN_POINT ( 'NONE',  ( 15.36997683531480874, 1435.038989812052023, 147.5081740258111722 ) ) ;
#35490=CARTESIAN_POINT ( 'NONE',  ( -26.49915054198219622, 1499.844595131229880, 212.0142546687440301 ) ) ;
#35496=DIRECTION ( 'NONE',  ( -0.7494985254689902066, 0.08460605218640301906, 0.6565773193259429874 ) ) ;
#35497=EDGE_CURVE ( 'NONE', #69002, #64952, #102009, .T. ) ;
#35499=CARTESIAN_POINT ( 'NONE',  ( 28.91076426840000124, 1509.890507619829805, 207.1524129226179980 ) ) ;
#35502=CARTESIAN_POINT ( 'NONE',  ( -15.82940463150903732, 1486.087625934943844, 186.8622631807861012 ) ) ;
#35505=CARTESIAN_POINT ( 'NONE',  ( 42.47353201039999959, 1448.912604704790056, 263.9447844666980245 ) ) ;
#35506=EDGE_CURVE ( 'NONE', #90113, #58583, #88961, .T. ) ;
#35508=CARTESIAN_POINT ( 'NONE',  ( 38.64637139974560398, 1443.913060387190171, 137.1864063390110005 ) ) ;
#35509=CARTESIAN_POINT ( 'NONE',  ( -7.746307814384410406, 1509.115590816079930, 236.8131461681879841 ) ) ;
#35510=CARTESIAN_POINT ( 'NONE',  ( -22.52134604649999972, 1451.600229533030188, 219.4799338534979825 ) ) ;
#35511=CARTESIAN_POINT ( 'NONE',  ( 11.31015084829999928, 1432.869298927259933, 151.5208831616980092 ) ) ;
#35512=CARTESIAN_POINT ( 'NONE',  ( 17.95636871770980036, 1410.547909248580027, 222.9459090208920031 ) ) ;
#35513=CARTESIAN_POINT ( 'NONE',  ( 0.2676492203279999815, 1452.807100928730051, 189.1997072006980147 ) ) ;
#35518=CARTESIAN_POINT ( 'NONE',  ( 0.5592746378849999811, 1405.719121701330096, 267.8539144989980514 ) ) ;
#35519=LINE ( 'NONE', #60753, #73217 ) ;
#35520=CARTESIAN_POINT ( 'NONE',  ( 12.64570686159999902, 1428.691483912829881, 223.9482794350980157 ) ) ;
#35524=CARTESIAN_POINT ( 'NONE',  ( -36.21648822516259969, 1440.913060387389805, 253.2446230051280054 ) ) ;
#35526=CARTESIAN_POINT ( 'NONE',  ( -1.453744412873089864, 1450.692426123599944, 154.2448216411129920 ) ) ;
#35533=CARTESIAN_POINT ( 'NONE',  ( -1.273841231818057862, 1450.738619355563060, 181.8035796647308757 ) ) ;
#35535=CARTESIAN_POINT ( 'NONE',  ( 11.10627834194573538, 1425.149160823644024, 138.4707484690964634 ) ) ;
#35537=CARTESIAN_POINT ( 'NONE',  ( -29.52080282280000034, 1509.954550902929896, 211.0554093484379905 ) ) ;
#35543=CARTESIAN_POINT ( 'NONE',  ( 18.89959486413309975, 1416.839692127159879, 210.6687135792209915 ) ) ;
#35544=CARTESIAN_POINT ( 'NONE',  ( -10.18694299370419998, 1396.268796277229967, 204.7956743315450012 ) ) ;
#35546=CARTESIAN_POINT ( 'NONE',  ( -16.83005542020710266, 1409.747738274599897, 225.5715775287220026 ) ) ;
#35547=CARTESIAN_POINT ( 'NONE',  ( 4.906228319039999342, 1433.447543843880112, 150.0987928807979870 ) ) ;
#35552=CARTESIAN_POINT ( 'NONE',  ( 10.38444639019999904, 1425.403467236129927, 94.99627158069790767 ) ) ;
#35555=CARTESIAN_POINT ( 'NONE',  ( -11.81044603969999862, 1433.053321433509836, 150.5679240076979966 ) ) ;
#35556=CARTESIAN_POINT ( 'NONE',  ( -2.790873196810775614, 1419.912297037458984, 186.1247558487485776 ) ) ;
#35560=CARTESIAN_POINT ( 'NONE',  ( 7.722835720109999080, 1509.114495076129970, 181.4225071154979787 ) ) ;
#35561=CARTESIAN_POINT ( 'NONE',  ( 3.416038303169999679, 1449.507431040339952, 184.0497570492980230 ) ) ;
#35565=ORIENTED_EDGE ( 'NONE', *, *, #4126, .T. ) ;
#35566=CARTESIAN_POINT ( 'NONE',  ( 18.18137294690000161, 1507.608465324829922, 188.5297611294979845 ) ) ;
#35570=CARTESIAN_POINT ( 'NONE',  ( -0.4870700791739999702, 1473.589435998730096, 270.3925729411980114 ) ) ;
#35573=B_SPLINE_CURVE_WITH_KNOTS ( 'NONE', 3,
 ( #60592, #27508, #94712, #102541, #61695, #17988, #26969, #16324, #50525, #86314, #25834, #77919, #1226 ),
 .UNSPECIFIED., .F., .F.,
 ( 4, 2, 2, 1, 2, 2, 4 ),
 ( 0.000000000000000000, 0.2500000000000023870, 0.3750000000000035527, 0.4375000000000029421, 0.4687500000000018319, 0.5000000000000006661, 1.000000000000000000 ),
 .UNSPECIFIED. ) ;
#35577=CARTESIAN_POINT ( 'NONE',  ( -33.93389098834200013, 1451.576030851350197, 135.5842732458419846 ) ) ;
#35578=ADVANCED_FACE ( 'NONE', ( #59495 ), #33934, .T. ) ;
#35580=CARTESIAN_POINT ( 'NONE',  ( -2.500000000000529798, 1448.894380907979894, 155.6080925131469996 ) ) ;
#35582=CARTESIAN_POINT ( 'NONE',  ( 12.63607377350000149, 1408.833611601630082, 216.0564899030879928 ) ) ;
#35583=CARTESIAN_POINT ( 'NONE',  ( -0.7664924707717509778, 1406.506770649930104, 269.4987574733809765 ) ) ;
#35584=CARTESIAN_POINT ( 'NONE',  ( -14.41479079490409987, 1436.126800610740020, 149.9515762605120131 ) ) ;
#35586=CARTESIAN_POINT ( 'NONE',  ( -10.96892109859999920, 1432.312127186730095, 151.7701099962980038 ) ) ;
#35587=CARTESIAN_POINT ( 'NONE',  ( 13.22002162090000077, 1442.920576605979932, 188.2908536790980065 ) ) ;
#35589=VERTEX_POINT ( 'NONE', #108499 ) ;
#35592=CIRCLE ( 'NONE', #96342, 0.5000000000000000000 ) ;
#35595=ORIENTED_EDGE ( 'NONE', *, *, #60421, .F. ) ;
#35597=CARTESIAN_POINT ( 'NONE',  ( 7.388977406289999550, 1415.087797054229895, 224.7253375031980056 ) ) ;
#35599=CARTESIAN_POINT ( 'NONE',  ( -27.59699679970000119, 1509.623160989430062, 202.9201204474879887 ) ) ;
#35600=CARTESIAN_POINT ( 'NONE',  ( -1.514732356010000114, 1507.625766696930214, 232.0393368578980073 ) ) ;
#35601=CARTESIAN_POINT ( 'NONE',  ( 11.41977518000482128, 1433.011620482430772, 151.3551162631975728 ) ) ;
#35608=CARTESIAN_POINT ( 'NONE',  ( 20.07779891821229867, 1477.280519013530011, 225.0994067720200178 ) ) ;
#35609=CARTESIAN_POINT ( 'NONE',  ( -25.36277544819999719, 1435.571748013670003, 136.4218649723979979 ) ) ;
#35614=CARTESIAN_POINT ( 'NONE',  ( -12.98226561589999939, 1414.913060387329779, 219.9156672276980089 ) ) ;
#35617=VERTEX_POINT ( 'NONE', #101733 ) ;
#35618=CARTESIAN_POINT ( 'NONE',  ( 2.500000000000000000, 1434.635760835609972, 157.5644327210980293 ) ) ;
#35619=CARTESIAN_POINT ( 'NONE',  ( 3.018077178498919544, 1440.716223221779728, 157.2134753452489804 ) ) ;
#35625=CARTESIAN_POINT ( 'NONE',  ( 12.20245528595089901, 1434.091338913249956, 149.6907156280659876 ) ) ;
#35627=B_SPLINE_SURFACE_WITH_KNOTS ( 'NONE', 5, 5, ( 
 ( #42139, #34829, #102565, #70136, #42689, #26422 ),
 ( #1247, #52209, #69016, #34281, #86335, #60059 ),
 ( #69574, #103693, #26993, #61182, #18560, #95299 ),
 ( #61721, #95843, #50548, #55510, #54967, #63383 ),
 ( #54427, #45473, #97499, #11305, #106449, #79615 ),
 ( #81231, #2919, #46567, #28087, #88560, #37037 ),
 ( #38136, #4011, #79069, #11843, #96403, #70686 ),
 ( #20767, #89093, #106990, #29732, #98033, #20226 ),
 ( #10751, #38680, #46015, #80145, #96961, #104799 ),
 ( #53885, #44922, #2374, #105353, #36490, #62274 ),
 ( #71231, #3464, #37593, #28644, #71794, #19680 ),
 ( #12380, #105913, #29193, #72318, #88021, #21305 ),
 ( #80701, #62847, #63918, #89638, #12925, #47105 ),
 ( #4547, #72856, #30278, #64471, #19111, #53314 ),
 ( #87456, #65006, #438, #7699, #90176, #33435 ) ),
 .UNSPECIFIED., .F., .F., .F.,
 ( 6, 3, 3, 3, 6 ),
 ( 6, 6 ),
 ( 14.45298335000000023, 21.98568536959999875, 27.70858623979999891, 30.13845758540000119, 37.41853765350000316 ),
 ( 0.000000000000000000, 1.621616996280000000 ),
 .UNSPECIFIED. ) ;
#35628=CARTESIAN_POINT ( 'NONE',  ( 18.15210693040249978, 1469.010815795120152, 228.4209498636830062 ) ) ;
#35629=CARTESIAN_POINT ( 'NONE',  ( -23.50962832835050165, 1509.033178799369807, 224.0176340712529850 ) ) ;
#35630=CARTESIAN_POINT ( 'NONE',  ( -2.431089449619999954, 1409.932888510029898, 186.5211211122979762 ) ) ;
#35631=CARTESIAN_POINT ( 'NONE',  ( 0.05606136413419999381, 1409.080515703730043, 232.6633760207980117 ) ) ;
#35634=CARTESIAN_POINT ( 'NONE',  ( -2.900970950180000063, 1421.449121440929957, 184.2745271147979906 ) ) ;
#35635=CARTESIAN_POINT ( 'NONE',  ( 19.35070455179999982, 1509.010601610729964, 188.1735489204979785 ) ) ;
#35638=CARTESIAN_POINT ( 'NONE',  ( -11.22551998621869807, 1414.913060387399810, 197.5794005584399997 ) ) ;
#35640=ORIENTED_EDGE ( 'NONE', *, *, #47344, .F. ) ;
#35642=CARTESIAN_POINT ( 'NONE',  ( 4.401092509980000678, 1420.174153530429976, 185.7217844323980103 ) ) ;
#35651=CARTESIAN_POINT ( 'NONE',  ( 17.38235991649999690, 1414.983773854429955, 210.5633853152779977 ) ) ;
#35652=CARTESIAN_POINT ( 'NONE',  ( -17.95544320140000139, 1424.506778464429999, 226.1749991304979801 ) ) ;
#35653=CARTESIAN_POINT ( 'NONE',  ( -19.60102139359999995, 1435.996833568079865, 145.7756697456979964 ) ) ;
#35654=CARTESIAN_POINT ( 'NONE',  ( -9.788350359310001636, 1441.600846913620217, 148.8293326998980035 ) ) ;
#35656=CARTESIAN_POINT ( 'NONE',  ( 1.052431931509999918, 1415.163755984130148, 191.3800010946980024 ) ) ;
#35657=CARTESIAN_POINT ( 'NONE',  ( -19.08445480129999794, 1440.913060387330006, 209.8212738029720299 ) ) ;
#35660=CARTESIAN_POINT ( 'NONE',  ( 1.556370309037290012, 1414.996442620790276, 191.7142051069610034 ) ) ;
#35661=CARTESIAN_POINT ( 'NONE',  ( 24.83969286159999967, 1449.817299431849960, 207.3631499707580019 ) ) ;
#35662=ADVANCED_FACE ( 'NONE', ( #59223 ), #8833, .F. ) ;
#35663=CARTESIAN_POINT ( 'NONE',  ( -23.87982329980000173, 1436.855522858850236, 211.6538958347979928 ) ) ;
#35667=B_SPLINE_SURFACE_WITH_KNOTS ( 'NONE', 5, 5, ( 
 ( #32775, #91025, #73709, #15411, #66959, #74802, #24365, #58551, #50157 ),
 ( #110042, #56344, #32234, #5933, #65304, #22694, #40079, #13751, #66414 ),
 ( #107834, #57462, #91588, #14312, #48503, #14863, #52913, #16499, #42843 ),
 ( #59108, #60205, #18172, #44505, #18717, #59654, #87045, #43950, #311 ),
 ( #26576, #101613, #69730, #77005, #17602, #26008, #61333, #78652, #68611 ),
 ( #50688, #60773, #10333, #25459, #9784, #94898, #94324, #103849, #1395 ) ),
 .UNSPECIFIED., .F., .F., .F.,
 ( 6, 6 ),
 ( 6, 3, 6 ),
 ( 25.36855762109999901, 27.09121026449999903 ),
 ( 0.000000000000000000, 1.000000000000000000, 2.000000000000000000 ),
 .UNSPECIFIED. ) ;
#35673=B_SPLINE_CURVE_WITH_KNOTS ( 'NONE', 3,
 ( #77215, #24007, #94535, #32446, #35752, #61529, #105166, #78301, #28457, #70491, #3280, #10551, #71044, #105730 ),
 .UNSPECIFIED., .F., .F.,
 ( 4, 2, 1, 1, 1, 1, 2, 2, 4 ),
 ( 0.000000000000000000, 0.2499999999998150368, 0.3749999999997225553, 0.4374999999996475597, 0.4687499999995786149, 0.4843749999995755062, 0.4921874999995717870, 0.4999999999995680677, 1.000000000000000000 ),
 .UNSPECIFIED. ) ;
#35674=CARTESIAN_POINT ( 'NONE',  ( 16.60876200430000083, 1451.097362684130076, 149.1934168744979843 ) ) ;
#35675=CARTESIAN_POINT ( 'NONE',  ( -0.8265242355799999885, 1408.941923249630008, 187.0792671738979891 ) ) ;
#35676=CARTESIAN_POINT ( 'NONE',  ( 23.19217488219999979, 1509.011520754329922, 193.6160623652979780 ) ) ;
#35678=CARTESIAN_POINT ( 'NONE',  ( -1.547463840030000037, 1414.913060387329779, 225.9340782259980074 ) ) ;
#35682=ORIENTED_EDGE ( 'NONE', *, *, #23915, .F. ) ;
#35683=CARTESIAN_POINT ( 'NONE',  ( 20.30812341819380151, 1509.558769329250026, 230.1713298670660208 ) ) ;
#35685=CARTESIAN_POINT ( 'NONE',  ( 40.17126634324269929, 1442.450104387399733, 136.9828420844469861 ) ) ;
#35687=CARTESIAN_POINT ( 'NONE',  ( -12.45246145670000004, 1471.374038867429817, 259.9010043778980048 ) ) ;
#35688=B_SPLINE_CURVE_WITH_KNOTS ( 'NONE', 4,
 ( #76692, #15113, #49303, #83428, #68877, #24603, #100770, #50954, #75061 ),
 .UNSPECIFIED., .F., .F.,
 ( 5, 4, 5 ),
 ( 0.000000000000000000, 0.9999834295456402344, 1.000000000000000000 ),
 .UNSPECIFIED. ) ;
#35691=CARTESIAN_POINT ( 'NONE',  ( 25.60002290280000281, 1509.583810695030024, 197.6050161354980048 ) ) ;
#35692=CARTESIAN_POINT ( 'NONE',  ( -20.57706974239999909, 1485.807236340330064, 191.5873737050980026 ) ) ;
#35694=CARTESIAN_POINT ( 'NONE',  ( 2.241718320410000409, 1410.369684904329915, 185.5035919006979839 ) ) ;
#35695=CARTESIAN_POINT ( 'NONE',  ( 6.301535050710000085, 1423.297843521130062, 186.2731961210980103 ) ) ;
#35696=CARTESIAN_POINT ( 'NONE',  ( -6.823170074189999212, 1439.352238415810007, 154.2706163447979861 ) ) ;
#35699=CARTESIAN_POINT ( 'NONE',  ( -3.134276369640000226, 1452.365440490629908, 153.7789987939979994 ) ) ;
#35705=CARTESIAN_POINT ( 'NONE',  ( -39.05686162770000180, 1453.566290948429923, 270.0278499002980084 ) ) ;
#35706=CARTESIAN_POINT ( 'NONE',  ( -26.51885021291319688, 1446.534126691539996, 137.5835072909900134 ) ) ;
#35707=CARTESIAN_POINT ( 'NONE',  ( 9.443064477949999258, 1434.540978515130064, 153.1670680800980051 ) ) ;
#35711=CARTESIAN_POINT ( 'NONE',  ( 7.612906430609999830, 1431.113060387329824, 191.6937606090980069 ) ) ;
#35712=CARTESIAN_POINT ( 'NONE',  ( 2.901685312356649948, 1409.503309903549962, 231.2713400696559916 ) ) ;
#35714=CARTESIAN_POINT ( 'NONE',  ( -3.251704830740000052, 1417.670526751729994, 234.4799080884979787 ) ) ;
#35716=CARTESIAN_POINT ( 'NONE',  ( -1.076831829273358521, 1484.840516514630508, 182.1570766342005072 ) ) ;
#35718=CARTESIAN_POINT ( 'NONE',  ( -45.92274223606419525, 1438.266996619100155, 266.6811736395359844 ) ) ;
#35722=CARTESIAN_POINT ( 'NONE',  ( 23.61230825720000226, 1435.322028862560046, 137.2857987807979896 ) ) ;
#35727=CARTESIAN_POINT ( 'NONE',  ( -27.46336423809769656, 1441.403115911309897, 137.3061811715859903 ) ) ;
#35728=CARTESIAN_POINT ( 'NONE',  ( -11.07444842074230174, 1415.954755714380099, 195.9645819946510130 ) ) ;
#35732=CARTESIAN_POINT ( 'NONE',  ( -14.53241430329999773, 1470.815019615729852, 194.7137864531979972 ) ) ;
#35733=CARTESIAN_POINT ( 'NONE',  ( 27.68253994085160130, 1507.989615297080036, 207.6661388942010262 ) ) ;
#35734=CARTESIAN_POINT ( 'NONE',  ( 13.61940320949999972, 1452.819910076330189, 194.9772319796979900 ) ) ;
#35735=EDGE_CURVE ( 'NONE', #57941, #98890, #3912, .T. ) ;
#35736=CARTESIAN_POINT ( 'NONE',  ( 1.804213551060599885, 1410.351307734219972, 232.1928989352460064 ) ) ;
#35737=CARTESIAN_POINT ( 'NONE',  ( -11.47928298387556012, 1425.866406702411268, 139.0912110491933333 ) ) ;
#35738=CARTESIAN_POINT ( 'NONE',  ( -22.98659938915999845, 1452.110350648670192, 138.7940535307059804 ) ) ;
#35742=CARTESIAN_POINT ( 'NONE',  ( -1.222390855309730018, 1409.214342690750073, 270.3713430301190215 ) ) ;
#35744=CARTESIAN_POINT ( 'NONE',  ( 8.888454490430000021, 1417.713827340430043, 230.5629018249979652 ) ) ;
#35750=CARTESIAN_POINT ( 'NONE',  ( -23.77291164573799875, 1410.729768559269814, 210.1269042920389722 ) ) ;
#35751=CARTESIAN_POINT ( 'NONE',  ( -4.653283256210000829, 1425.827074144530116, 186.2156745063980168 ) ) ;
#35752=CARTESIAN_POINT ( 'NONE',  ( -11.33168998458564936, 1437.952585642965687, 152.0540813750432676 ) ) ;
#35755=EDGE_CURVE ( 'NONE', #87953, #104164, #109725, .T. ) ;
#35756=CARTESIAN_POINT ( 'NONE',  ( -20.98880188002820191, 1506.431317093110010, 192.2210660023540072 ) ) ;
#35757=CARTESIAN_POINT ( 'NONE',  ( -17.75051042830000014, 1425.821874560129800, 226.3520932680980025 ) ) ;
#35758=CARTESIAN_POINT ( 'NONE',  ( 36.69248205205470015, 1461.665376385029958, 269.0208840940840105 ) ) ;
#35759=CARTESIAN_POINT ( 'NONE',  ( -8.798117652420820889, 1465.157268619798060, 232.9151898438935575 ) ) ;
#35760=CARTESIAN_POINT ( 'NONE',  ( 8.723378431209999562, 1446.953229722669903, 186.0446995693979773 ) ) ;
#35763=CARTESIAN_POINT ( 'NONE',  ( 19.03319670683364606, 1457.114807116183783, 226.2774458981556052 ) ) ;
#35764=CARTESIAN_POINT ( 'NONE',  ( 1.529023292565329761, 1453.102415013690006, 183.4720393914749934 ) ) ;
#35765=CARTESIAN_POINT ( 'NONE',  ( 22.68092815790000216, 1409.705069317929883, 208.9674978898780182 ) ) ;
#35766=VERTEX_POINT ( 'NONE', #57985 ) ;
#35767=CARTESIAN_POINT ( 'NONE',  ( -0.8815214275217030382, 1457.995828996750106, 229.7940963460050057 ) ) ;
#35769=CARTESIAN_POINT ( 'NONE',  ( 25.44620943400289903, 1452.008651903540112, 135.5281762852589793 ) ) ;
#35770=CARTESIAN_POINT ( 'NONE',  ( -14.26080844802509873, 1456.560644424450174, 195.3871132866240146 ) ) ;
#35773=CARTESIAN_POINT ( 'NONE',  ( 18.15046249250000088, 1410.043460838129931, 194.1297086120979998 ) ) ;
#35774=B_SPLINE_SURFACE_WITH_KNOTS ( 'NONE', 5, 5, ( 
 ( #32174, #59594, #23208, #23759, #50096, #51187, #58493, #50638, #31614 ),
 ( #108881, #91533, #92078, #14811, #92619, #93710, #57408, #57946, #83671 ),
 ( #6427, #24311, #67456, #41122, #65791, #5877, #68012, #66358, #33267 ),
 ( #6968, #15896, #75302, #33820, #109990, #99913, #32725, #48998, #101557 ),
 ( #100477, #16442, #49546, #66905, #24848, #102122, #40021, #74199, #101012 ),
 ( #109445, #84223, #108331, #8066, #83131, #7523, #41681, #25401, #75841 ) ),
 .UNSPECIFIED., .F., .F., .F.,
 ( 6, 6 ),
 ( 6, 3, 6 ),
 ( 0.4666582265040000177, 2.797885342376539963 ),
 ( -1.082960654485929847E-05, 1.000000000000000000, 2.000000000000000000 ),
 .UNSPECIFIED. ) ;
#35776=CARTESIAN_POINT ( 'NONE',  ( 2.962028108840362162, 1439.673284367522001, 184.0494181787074979 ) ) ;
#35777=CARTESIAN_POINT ( 'NONE',  ( 0.3313159878120000013, 1417.263519912130050, 235.9102102634980156 ) ) ;
#35778=CARTESIAN_POINT ( 'NONE',  ( -18.88466409699455539, 1424.778541419677822, 224.4175826655136632 ) ) ;
#35779=CARTESIAN_POINT ( 'NONE',  ( 14.12491358549999987, 1409.406313238730036, 226.3524348291979891 ) ) ;
#35780=CARTESIAN_POINT ( 'NONE',  ( -0.2739194539550000029, 1497.016984061830044, 230.9805001397980107 ) ) ;
#35784=EDGE_LOOP ( 'NONE', ( #52540, #89701, #83693, #54550 ) ) ;
#35788=CARTESIAN_POINT ( 'NONE',  ( 9816.840209715130186, 50.13405481578730161, 1424.308828391600173 ) ) ;
#35790=CARTESIAN_POINT ( 'NONE',  ( -34.38848389989589549, 1450.406366866479857, 136.2345448457099906 ) ) ;
#35792=CARTESIAN_POINT ( 'NONE',  ( -25.52872276659999784, 1450.634754193449908, 248.0989693021979861 ) ) ;
#35796=CARTESIAN_POINT ( 'NONE',  ( 19.00000000000000000, 1442.955095612160221, 209.1218459616979999 ) ) ;
#35798=CARTESIAN_POINT ( 'NONE',  ( -17.99954540876850118, 1410.904693920620048, 195.2564682659330231 ) ) ;
#35799=( BOUNDED_CURVE ( )  B_SPLINE_CURVE ( 3, ( #31089, #75327, #40598, #5901 ),
 .UNSPECIFIED., .F., .F. ) 
 B_SPLINE_CURVE_WITH_KNOTS ( ( 4, 4 ),
 ( 1.441033914288156303, 1.936717213009869099 ),
 .UNSPECIFIED. ) 
 CURVE ( )  GEOMETRIC_REPRESENTATION_ITEM ( )  RATIONAL_B_SPLINE_CURVE ( ( 1.000000000000000000, 0.9796294326414420883, 0.9796294326414420883, 1.000000000000000000 ) ) 
 REPRESENTATION_ITEM ( '' )  );
#35801=AXIS2_PLACEMENT_3D ( 'NONE', #92433, #66182, #100832 ) ;
#35803=CARTESIAN_POINT ( 'NONE',  ( 13.89554995500000167, 1452.733480491630189, 223.3956528723979886 ) ) ;
#35804=EDGE_CURVE ( 'NONE', #43307, #21837, #85926, .T. ) ;
#35805=CARTESIAN_POINT ( 'NONE',  ( -9.618017228990000334, 1486.043860324930165, 183.5224656496979776 ) ) ;
#35807=CARTESIAN_POINT ( 'NONE',  ( -25.97046449806400048, 1509.898002744609812, 192.9853469788230029 ) ) ;
#35809=CARTESIAN_POINT ( 'NONE',  ( 24.95209251429999853, 1469.238639853630048, 215.5966609727680066 ) ) ;
#35816=CARTESIAN_POINT ( 'NONE',  ( 0.1597472590855660013, 1486.419116074489921, 181.8185966615969846 ) ) ;
#35817=SPHERICAL_SURFACE ( 'NONE', #51500, 2.000000000660000055 ) ;
#35820=ADVANCED_FACE ( 'NONE', ( #61867 ), #84880, .F. ) ;
#35826=ORIENTED_EDGE ( 'NONE', *, *, #54205, .T. ) ;
#35835=CARTESIAN_POINT ( 'NONE',  ( 14.72140900422560073, 1409.427143317539958, 211.6119428930840343 ) ) ;
#35838=CARTESIAN_POINT ( 'NONE',  ( -17.51214883540000145, 1417.728543787030048, 192.0614060638979765 ) ) ;
#35841=CARTESIAN_POINT ( 'NONE',  ( 17.22623662315568893, 1443.913060387331598, 162.9225832754749490 ) ) ;
#35845=ORIENTED_EDGE ( 'NONE', *, *, #94018, .T. ) ;
#35847=CARTESIAN_POINT ( 'NONE',  ( 24.90415728650000204, 1509.109212994030031, 220.8332857727979786 ) ) ;
#35851=CARTESIAN_POINT ( 'NONE',  ( 35.04905840024694896, 1457.721304834078865, 269.5321777411671178 ) ) ;
#35853=CARTESIAN_POINT ( 'NONE',  ( 3.412736717740000092, 1396.032235779629900, 220.0203514156980020 ) ) ;
#35854=CARTESIAN_POINT ( 'NONE',  ( 20.18543375162190046, 1451.730034569789950, 209.6998159054799942 ) ) ;
#35858=FACE_OUTER_BOUND ( 'NONE', #4964, .T. ) ;
#35859=CARTESIAN_POINT ( 'NONE',  ( 10.75856251613272718, 1424.957327209176810, 140.6161141926336029 ) ) ;
#35862=CARTESIAN_POINT ( 'NONE',  ( -13.08019506225550010, 1434.911011336890169, 149.7358237173160092 ) ) ;
#35863=LINE ( 'NONE', #10663, #76578 ) ;
#35864=CARTESIAN_POINT ( 'NONE',  ( 44.92382427260000100, 1446.402585538819949, 269.6913831871979710 ) ) ;
#35868=CARTESIAN_POINT ( 'NONE',  ( 40.30319224264979994, 1444.187662185900081, 137.0996438307940082 ) ) ;
#35869=EDGE_LOOP ( 'NONE', ( #31414, #6032, #26353, #8218, #33295 ) ) ;
#35870=CARTESIAN_POINT ( 'NONE',  ( 3.468905163120000072E-10, 1405.830928045030078, 267.2558864325980039 ) ) ;
#35871=CARTESIAN_POINT ( 'NONE',  ( -26.43941341069999851, 1488.684867474930115, 204.4673947574779902 ) ) ;
#35872=CARTESIAN_POINT ( 'NONE',  ( -10.67358497261050054, 1425.014385072390269, 135.2576413182610224 ) ) ;
#35873=CARTESIAN_POINT ( 'NONE',  ( 16.58590676013170295, 1409.592623960390029, 192.7795323272440271 ) ) ;
#35877=CARTESIAN_POINT ( 'NONE',  ( -31.95512683489999617, 1440.913060381139985, 244.1805851169980031 ) ) ;
#35878=CARTESIAN_POINT ( 'NONE',  ( 18.68655961963949963, 1509.584487903890022, 232.0746350300250072 ) ) ;
#35879=CARTESIAN_POINT ( 'NONE',  ( 28.25086641300000068, 1508.135711190629991, 209.3856964555159834 ) ) ;
#35881=DIRECTION ( 'NONE',  ( 0.8234232003240999909, -0.5674277338727967690, -0.000000000000000000 ) ) ;
#35882=ORIENTED_EDGE ( 'NONE', *, *, #18644, .T. ) ;
#35883=CARTESIAN_POINT ( 'NONE',  ( 5.639071283312759419, 1396.170382753050035, 219.3208655836849914 ) ) ;
#35886=CARTESIAN_POINT ( 'NONE',  ( -16.40067627780000237, 1459.015013897929975, 229.6400837563979849 ) ) ;
#35887=ORIENTED_EDGE ( 'NONE', *, *, #18277, .T. ) ;
#35892=CARTESIAN_POINT ( 'NONE',  ( -1.080623904679999914, 1417.487791310030161, 185.0156185439980163 ) ) ;
#35894=ADVANCED_FACE ( 'NONE', ( #47792 ), #101051, .T. ) ;
#35896=CARTESIAN_POINT ( 'NONE',  ( -12.01638156518240130, 1440.881463477919851, 187.8051726210379968 ) ) ;
#35897=CARTESIAN_POINT ( 'NONE',  ( -7.249244512309999777, 1470.477750770629882, 233.8384446450980079 ) ) ;
#35905=CARTESIAN_POINT ( 'NONE',  ( 11.86577998873609907, 1432.313618685340089, 149.9823692228469838 ) ) ;
#35906=CARTESIAN_POINT ( 'NONE',  ( 13.19964874196263338, 1444.708229313989477, 187.3105044755715767 ) ) ;
#35910=CARTESIAN_POINT ( 'NONE',  ( 2.982314100249999989, 1508.959213791230013, 237.3237166239979956 ) ) ;
#35913=CARTESIAN_POINT ( 'NONE',  ( -5.436853854820000720, 1424.722442587329851, 186.3690072748979958 ) ) ;
#35914=CARTESIAN_POINT ( 'NONE',  ( 3.472351607788480177, 1409.306382308760021, 270.3710068956600026 ) ) ;
#35919=CARTESIAN_POINT ( 'NONE',  ( 0.03158484996424502922, 1410.294062402277405, 233.2218019618084099 ) ) ;
#35925=CARTESIAN_POINT ( 'NONE',  ( -5.544570429734849704, 1422.963021390169843, 111.4258773807360114 ) ) ;
#35927=CARTESIAN_POINT ( 'NONE',  ( 26.42714721250000309, 1437.883259618699867, 243.9198229428980085 ) ) ;
#35928=CARTESIAN_POINT ( 'NONE',  ( 13.55396217860879915, 1434.957544704839847, 148.7506959228599897 ) ) ;
#35935=AXIS2_PLACEMENT_3D ( 'NONE', #108776, #40467, #76281 ) ;
#35938=CARTESIAN_POINT ( 'NONE',  ( 19.37133922758618354, 1456.941101056772595, 224.5491805723401626 ) ) ;
#35940=DIRECTION ( 'NONE',  ( 0.7074300732606700892, 0.02470400251916599760, -0.7063514732099990256 ) ) ;
#35944=CARTESIAN_POINT ( 'NONE',  ( 12.50842520650000012, 1415.079606268429870, 228.9876709444980065 ) ) ;
#35946=CARTESIAN_POINT ( 'NONE',  ( -15.69219286469999908, 1459.328416987729952, 229.9957181814980061 ) ) ;
#35948=CARTESIAN_POINT ( 'NONE',  ( 21.96192329710000379, 1409.941828261930141, 267.3321697500979894 ) ) ;
#35950=FACE_OUTER_BOUND ( 'NONE', #4203, .T. ) ;
#35951=CARTESIAN_POINT ( 'NONE',  ( 20.68893471149999996, 1469.156827144430054, 193.1476934458979997 ) ) ;
#35952=CARTESIAN_POINT ( 'NONE',  ( -23.46657084150000117, 1435.066155488599861, 213.1839366923280181 ) ) ;
#35955=CARTESIAN_POINT ( 'NONE',  ( -1.342311606190000006, 1451.734940660029906, 183.7820431827979633 ) ) ;
#35956=CARTESIAN_POINT ( 'NONE',  ( -20.19282075723703684, 1506.569407720561458, 200.1490527362905425 ) ) ;
#35958=CARTESIAN_POINT ( 'NONE',  ( -13.17579405299999884, 1442.542553075959859, 187.8823243441979969 ) ) ;
#35960=CARTESIAN_POINT ( 'NONE',  ( -29.17526201480000125, 1435.517118628549952, 135.6494733468979916 ) ) ;
#35961=CARTESIAN_POINT ( 'NONE',  ( -7.271061757791160929, 1456.602686919181451, 227.6850874585875601 ) ) ;
#35963=CYLINDRICAL_SURFACE ( 'NONE', #43909, 1.000000000000001110 ) ;
#35964=CARTESIAN_POINT ( 'NONE',  ( -14.79665290848370063, 1409.429770892780198, 207.1251313586369918 ) ) ;
#35967=CARTESIAN_POINT ( 'NONE',  ( -45.67178295499999763, 1445.962966203089991, 266.1885921243979851 ) ) ;
#35970=DIRECTION ( 'NONE',  ( 0.7074300732601481734, -0.02470400263378330630, 0.7063514732065131474 ) ) ;
#35972=CARTESIAN_POINT ( 'NONE',  ( 19.02974679407714120, 1457.003061607406380, 225.9956790813866974 ) ) ;
#35975=CARTESIAN_POINT ( 'NONE',  ( 13.74428069839999900, 1415.087818611729972, 219.0809107912880052 ) ) ;
#35976=FACE_OUTER_BOUND ( 'NONE', #49784, .T. ) ;
#35979=CARTESIAN_POINT ( 'NONE',  ( -9.883703466890001010, 1508.498109722830122, 182.1694905005979876 ) ) ;
#35980=CARTESIAN_POINT ( 'NONE',  ( -23.93955323720000194, 1410.670994470229971, 208.0781342075679845 ) ) ;
#35982=CARTESIAN_POINT ( 'NONE',  ( 16.44108920490000258, 1415.931669658029932, 201.4407812804579976 ) ) ;
#35986=EDGE_CURVE ( 'NONE', #65298, #36309, #54042, .T. ) ;
#35991=CARTESIAN_POINT ( 'NONE',  ( 11.90008666459999986, 1434.920851464509951, 147.6452002888979962 ) ) ;
#35996=CARTESIAN_POINT ( 'NONE',  ( 8.178501070643639181, 1441.152429762079919, 153.9860758848200248 ) ) ;
#36000=CARTESIAN_POINT ( 'NONE',  ( -17.41094686896749977, 1485.005976550500236, 188.5081240344379978 ) ) ;
#36001=CARTESIAN_POINT ( 'NONE',  ( -18.93046898119999710, 1449.653411359970050, 193.5799670889979893 ) ) ;
#36006=EDGE_CURVE ( 'NONE', #75020, #69697, #32498, .T. ) ;
#36008=CARTESIAN_POINT ( 'NONE',  ( 11.77041528381420044, 1433.833598648250018, 150.9228460987970095 ) ) ;
#36012=CARTESIAN_POINT ( 'NONE',  ( -22.05719187630000278, 1509.683314500430015, 191.3091005153979722 ) ) ;
#36014=CARTESIAN_POINT ( 'NONE',  ( -0.06574339172959998978, 1508.965708869629907, 179.3766826782980104 ) ) ;
#36015=CARTESIAN_POINT ( 'NONE',  ( 11.89544747750000120, 1434.541746328260160, 147.6465872843980094 ) ) ;
#36019=CARTESIAN_POINT ( 'NONE',  ( -23.84450196390190158, 1452.080391932540124, 136.9869676255979982 ) ) ;
#36021=CARTESIAN_POINT ( 'NONE',  ( -24.59804701143680106, 1444.770899505660054, 210.9018572211569733 ) ) ;
#36023=CARTESIAN_POINT ( 'NONE',  ( 35.92423077391850228, 1436.007692230339899, 134.0999999972619889 ) ) ;
#36028=CARTESIAN_POINT ( 'NONE',  ( 14.43356177019170161, 1436.105945022930200, 149.9343689364710031 ) ) ;
#36034=CARTESIAN_POINT ( 'NONE',  ( -0.7474240596110000023, 1467.090493009529837, 235.5344236438979806 ) ) ;
#36035=CARTESIAN_POINT ( 'NONE',  ( 22.11924855878987728, 1450.910478644122122, 143.0538365109425456 ) ) ;
#36038=EDGE_CURVE ( 'NONE', #59778, #7623, #83041, .T. ) ;
#36039=VECTOR ( 'NONE', #69284, 1000.000000000000114 ) ;
#36040=CARTESIAN_POINT ( 'NONE',  ( -19.07402656877554392, 1442.263495886194960, 210.5458490460772225 ) ) ;
#36043=EDGE_CURVE ( 'NONE', #52385, #45960, #17466, .T. ) ;
#36045=ORIENTED_EDGE ( 'NONE', *, *, #37258, .F. ) ;
#36048=CARTESIAN_POINT ( 'NONE',  ( 32.50672632217259661, 1440.913060387330006, 256.8451983435460306 ) ) ;
#36049=CARTESIAN_POINT ( 'NONE',  ( -17.98937745960000001, 1509.201726663129875, 186.3878134344979856 ) ) ;
#36050=ORIENTED_EDGE ( 'NONE', *, *, #48013, .F. ) ;
#36052=CARTESIAN_POINT ( 'NONE',  ( -14.51206241080000048, 1409.419832773630105, 192.1183054032979953 ) ) ;
#36054=CARTESIAN_POINT ( 'NONE',  ( 0.1595995995380000143, 1486.508831850330125, 181.8147405652979671 ) ) ;
#36056=CARTESIAN_POINT ( 'NONE',  ( 0.0001418537954666921350, 1395.950261259293029, 197.6573513283705665 ) ) ;
#36058=CARTESIAN_POINT ( 'NONE',  ( -26.79413167943010166, 1436.761919080860025, 136.7821860765010058 ) ) ;
#36063=B_SPLINE_CURVE_WITH_KNOTS ( 'NONE', 3,
 ( #96649, #54118, #3162, #38376, #107795, #99373 ),
 .UNSPECIFIED., .F., .F.,
 ( 4, 2, 4 ),
 ( -0.03810055507010769865, -0.01873955902292570239, 0.000000000000000000 ),
 .UNSPECIFIED. ) ;
#36066=CARTESIAN_POINT ( 'NONE',  ( 27.93158904759999928, 1508.017348895330088, 207.9454904019079891 ) ) ;
#36068=CARTESIAN_POINT ( 'NONE',  ( -18.95069757339999938, 1434.818091166690010, 209.0758544139090134 ) ) ;
#36069=CARTESIAN_POINT ( 'NONE',  ( -17.27977277066755946, 1486.136564927255677, 187.9056138646151055 ) ) ;
#36073=CARTESIAN_POINT ( 'NONE',  ( -5.623567758859999945E-10, 1466.838857909629951, 244.5742075746979936 ) ) ;
#36076=CARTESIAN_POINT ( 'NONE',  ( -2.809418260625490049, 1508.990990147629873, 238.3402367501120125 ) ) ;
#36077=CARTESIAN_POINT ( 'NONE',  ( -19.92007499920000058, 1455.402141745330027, 226.0082975429980081 ) ) ;
#36079=CARTESIAN_POINT ( 'NONE',  ( 11.58636795370000172, 1433.009610628010023, 151.1946776810979713 ) ) ;
#36080=CARTESIAN_POINT ( 'NONE',  ( 19.46842866420000107, 1455.664567239729877, 226.2662422576979964 ) ) ;
#36081=CARTESIAN_POINT ( 'NONE',  ( 0.1661831847680000085, 1452.811554597430131, 189.3009787847980192 ) ) ;
#36083=ORIENTED_EDGE ( 'NONE', *, *, #33990, .T. ) ;
#36086=DIRECTION ( 'NONE',  ( 0.000000000000000000, 0.2733307411301343914, -0.9619201141224000828 ) ) ;
#36087=CARTESIAN_POINT ( 'NONE',  ( 30.27492243234960156, 1463.607600769530109, 269.7181436845010580 ) ) ;
#36088=CARTESIAN_POINT ( 'NONE',  ( 5.391625819569999756, 1433.099291512059835, 154.6242831037980068 ) ) ;
#36092=CARTESIAN_POINT ( 'NONE',  ( -36.67895744121949519, 1440.913060387330006, 254.0696615155329994 ) ) ;
#36093=CARTESIAN_POINT ( 'NONE',  ( 34.39105378604129726, 1450.405804220740265, 136.2345510266769963 ) ) ;
#36094=CARTESIAN_POINT ( 'NONE',  ( 2.500574528909250027, 1448.942056006560051, 154.5733147652059927 ) ) ;
#36101=CARTESIAN_POINT ( 'NONE',  ( -8.881784197000000993E-16, 1410.951844103529993, 268.3665355202980436 ) ) ;
#36104=CARTESIAN_POINT ( 'NONE',  ( -0.1078499524459999998, 1475.983410498030025, 267.2349610867980232 ) ) ;
#36109=AXIS2_PLACEMENT_3D ( 'NONE', #12534, #46712, #80842 ) ;
#36110=CARTESIAN_POINT ( 'NONE',  ( -17.83233393729999960, 1415.128105759529944, 207.7695487697079955 ) ) ;
#36112=CARTESIAN_POINT ( 'NONE',  ( 19.00334344017809585, 1416.835288280193936, 210.3100235811058667 ) ) ;
#36113=CARTESIAN_POINT ( 'NONE',  ( -5.573518479978040396, 1396.107691941430176, 199.5941084161559900 ) ) ;
#36116=CARTESIAN_POINT ( 'NONE',  ( -17.22758722712179846, 1410.459222837350126, 225.8949354550800024 ) ) ;
#36117=CARTESIAN_POINT ( 'NONE',  ( 22.28175235382923347, 1509.670458318331612, 227.1137651221278020 ) ) ;
#36118=VERTEX_POINT ( 'NONE', #99824 ) ;
#36122=CARTESIAN_POINT ( 'NONE',  ( 10.00814141210000052, 1425.214601638330123, 94.99987188269780347 ) ) ;
#36124=CARTESIAN_POINT ( 'NONE',  ( 3.156166260290000025, 1466.544008048530031, 236.1241471695980181 ) ) ;
#36129=CARTESIAN_POINT ( 'NONE',  ( -23.55087667009999919, 1411.110693366829764, 210.4794020521279947 ) ) ;
#36130=LINE ( 'NONE', #27720, #23881 ) ;
#36131=CARTESIAN_POINT ( 'NONE',  ( 2.622224098489999822, 1449.049842484869941, 183.1053685486979816 ) ) ;
#36133=CARTESIAN_POINT ( 'NONE',  ( -15.74154698502330163, 1459.394320999469983, 230.7248352790539911 ) ) ;
#36134=ORIENTED_EDGE ( 'NONE', *, *, #13815, .T. ) ;
#36135=EDGE_LOOP ( 'NONE', ( #13683, #88034, #40284, #74189 ) ) ;
#36136=EDGE_CURVE ( 'NONE', #3437, #37815, #101565, .T. ) ;
#36137=CARTESIAN_POINT ( 'NONE',  ( -40.71369779150000312, 1443.851625732439970, 137.1196992376980006 ) ) ;
#36139=CARTESIAN_POINT ( 'NONE',  ( -10.06709464454669956, 1499.964826402849894, 247.9768189705859811 ) ) ;
#36144=EDGE_CURVE ( 'NONE', #77609, #25815, #82943, .T. ) ;
#36145=CARTESIAN_POINT ( 'NONE',  ( -34.91175744441260065, 1450.402292434889887, 136.2167050401169774 ) ) ;
#36146=CARTESIAN_POINT ( 'NONE',  ( -2.500000000000000000, 1448.457353036769973, 161.2531520594690164 ) ) ;
#36147=CARTESIAN_POINT ( 'NONE',  ( 9.510490888398619447, 1396.245174050119886, 214.7739347511380004 ) ) ;
#36148=CARTESIAN_POINT ( 'NONE',  ( 9.336575772837418796, 1408.712768855870081, 198.5035178465510057 ) ) ;
#36149=CARTESIAN_POINT ( 'NONE',  ( -5.339443612929020588, 1406.221089105190003, 266.9497679340149716 ) ) ;
#36150=CARTESIAN_POINT ( 'NONE',  ( -13.76119476942800013, 1434.988040804719958, 148.8304954868820005 ) ) ;
#36152=CARTESIAN_POINT ( 'NONE',  ( 3.709769364390000490, 1425.443954302430029, 185.2607701543980170 ) ) ;
#36153=CARTESIAN_POINT ( 'NONE',  ( 13.37712129999999888, 1445.815448238960016, 188.8332726567979876 ) ) ;
#36154=VERTEX_POINT ( 'NONE', #57320 ) ;
#36162=CARTESIAN_POINT ( 'NONE',  ( 9.839466250099999201, 1415.426091369430196, 224.2613875613980099 ) ) ;
#36165=CARTESIAN_POINT ( 'NONE',  ( -13.70772824027479864, 1507.648153509909889, 184.2587339175119894 ) ) ;
#36167=CARTESIAN_POINT ( 'NONE',  ( 11.21203837860620922, 1433.014098020969641, 151.5746018212971364 ) ) ;
#36170=CARTESIAN_POINT ( 'NONE',  ( -5.999476885900000056, 1410.056533633429808, 231.4736029180979813 ) ) ;
#36171=CARTESIAN_POINT ( 'NONE',  ( -8.921414208959999925, 1447.268111543890200, 186.2693290151980250 ) ) ;
#36173=CARTESIAN_POINT ( 'NONE',  ( -14.58073495223914051, 1436.114484106691634, 149.8442567287235363 ) ) ;
#36176=CARTESIAN_POINT ( 'NONE',  ( 15.62326149577455325, 1506.535970895669379, 224.7081918935420219 ) ) ;
#36177=CARTESIAN_POINT ( 'NONE',  ( -25.34185429560000102, 1436.460898709450021, 137.3540916501980291 ) ) ;
#36179=VECTOR ( 'NONE', #27524, 1000.000000000000000 ) ;
#36181=CARTESIAN_POINT ( 'NONE',  ( 0.008364224685127532796, 1508.450927448398261, 237.9449321159623594 ) ) ;
#36183=CARTESIAN_POINT ( 'NONE',  ( 20.22198891407199994, 1410.979504948318208, 197.8698230559548108 ) ) ;
#36186=CARTESIAN_POINT ( 'NONE',  ( 2.500000000000000000, 1432.484228967709896, 157.4989653737979722 ) ) ;
#36187=CARTESIAN_POINT ( 'NONE',  ( 5.457743877670670152, 1440.715679535709796, 154.7912908120740099 ) ) ;
#36189=ORIENTED_EDGE ( 'NONE', *, *, #32715, .T. ) ;
#36190=DIRECTION ( 'NONE',  ( -7.460783098696655896E-07, -0.9583089388702578093, 0.2857341031112730634 ) ) ;
#36191=LINE ( 'NONE', #21014, #101340 ) ;
#36192=CARTESIAN_POINT ( 'NONE',  ( 12.51168921360669906, 1434.575074074980193, 150.0969845919200054 ) ) ;
#36193=CARTESIAN_POINT ( 'NONE',  ( 13.20134068419620021, 1478.703343677790144, 231.7406313773049931 ) ) ;
#36194=CARTESIAN_POINT ( 'NONE',  ( -24.18231958401429793, 1509.512723376200029, 223.7027743721939999 ) ) ;
#36195=CARTESIAN_POINT ( 'NONE',  ( -1.899659233539999992, 1408.979397949530039, 187.8524191995979891 ) ) ;
#36197=CARTESIAN_POINT ( 'NONE',  ( 0.02480326138201020131, 1420.444607191170007, 182.6734921983770050 ) ) ;
#36199=CARTESIAN_POINT ( 'NONE',  ( -4.319145982190000232, 1421.270721987530123, 186.1375689550980042 ) ) ;
#36202=VERTEX_POINT ( 'NONE', #41030 ) ;
#36203=CARTESIAN_POINT ( 'NONE',  ( -12.78353013627570078, 1416.221314539589912, 196.4153621971449866 ) ) ;
#36207=CARTESIAN_POINT ( 'NONE',  ( 9.275190821709212941, 1436.622319119972872, 152.9610493690184683 ) ) ;
#36212=CARTESIAN_POINT ( 'NONE',  ( 17.35267690140000241, 1414.988017870030035, 210.4487656687780088 ) ) ;
#36213=CARTESIAN_POINT ( 'NONE',  ( -18.54624378429999965, 1425.206167962729978, 225.2666202254980021 ) ) ;
#36214=CARTESIAN_POINT ( 'NONE',  ( -21.38425910549999998, 1436.475178973239963, 143.9724053363979976 ) ) ;
#36215=CARTESIAN_POINT ( 'NONE',  ( -0.5805478584864469660, 1457.956445091640035, 229.5817085807559863 ) ) ;
#36216=CARTESIAN_POINT ( 'NONE',  ( 17.09566487500000065, 1418.986537885430153, 191.5701185073980071 ) ) ;
#36218=CARTESIAN_POINT ( 'NONE',  ( 0.5779700330962650456, 1451.730245120970039, 188.9364029278959833 ) ) ;
#36219=CARTESIAN_POINT ( 'NONE',  ( 11.73811278442431139, 1433.731505864096334, 150.9439206914117619 ) ) ;
#36220=ORIENTED_EDGE ( 'NONE', *, *, #99547, .T. ) ;
#36221=CARTESIAN_POINT ( 'NONE',  ( 1.556453189349229937, 1415.124054205860148, 191.3769848897780150 ) ) ;
#36222=CARTESIAN_POINT ( 'NONE',  ( 23.97240591419999944, 1430.440342350430001, 207.3418792401980113 ) ) ;
#36223=CARTESIAN_POINT ( 'NONE',  ( -11.87682050080051788, 1433.080539119526748, 149.9786770413036265 ) ) ;
#36224=DIRECTION ( 'NONE',  ( -0.9993908270190955401, -0.03489949670250328678, 0.000000000000000000 ) ) ;
#36225=CARTESIAN_POINT ( 'NONE',  ( -18.63433789430000331, 1508.246382728430035, 229.7323350256980063 ) ) ;
#36227=CARTESIAN_POINT ( 'NONE',  ( -22.86388141493510062, 1452.114636054849825, 134.0999999999999943 ) ) ;
#36228=CARTESIAN_POINT ( 'NONE',  ( -18.68121726845560104, 1509.578614484549917, 185.5942095029820109 ) ) ;
#36237=CARTESIAN_POINT ( 'NONE',  ( -18.05523222188424270, 1459.620137051063921, 227.9958600545465970 ) ) ;
#36239=CARTESIAN_POINT ( 'NONE',  ( 20.18524465598390094, 1509.340777616249852, 229.9812346231060189 ) ) ;
#36240=VERTEX_POINT ( 'NONE', #74657 ) ;
#36243=CARTESIAN_POINT ( 'NONE',  ( 18.52260186970000433, 1425.593317732829973, 225.5454236923980034 ) ) ;
#36244=CARTESIAN_POINT ( 'NONE',  ( 13.45445143672208843, 1443.535890046601253, 169.3629104747118959 ) ) ;
#36245=CARTESIAN_POINT ( 'NONE',  ( 12.91599431494240946, 1411.873776468889218, 269.3566367870338922 ) ) ;
#36246=CARTESIAN_POINT ( 'NONE',  ( -40.44435938619999860, 1454.056667761929930, 264.0385842768980069 ) ) ;
#36248=CARTESIAN_POINT ( 'NONE',  ( -11.81090838280000099, 1433.647990716570121, 150.7603589772980115 ) ) ;
#36250=CARTESIAN_POINT ( 'NONE',  ( -20.06661625339999944, 1486.017343259630252, 190.5747571216979850 ) ) ;
#36251=CARTESIAN_POINT ( 'NONE',  ( 11.16746684139999957, 1409.469218647829848, 189.9183212870979958 ) ) ;
#36252=CARTESIAN_POINT ( 'NONE',  ( 5.192738225420000298, 1422.609109026029955, 185.4141380594979864 ) ) ;
#36253=CARTESIAN_POINT ( 'NONE',  ( -7.539474871700000413, 1438.620589098819892, 153.9375992959979840 ) ) ;
#36255=CARTESIAN_POINT ( 'NONE',  ( -2.714057680736050138, 1440.141560261370159, 155.9947301247320013 ) ) ;
#36256=CARTESIAN_POINT ( 'NONE',  ( -6.137775026819999979, 1452.698724561930021, 152.5573369345979984 ) ) ;
#36260=CARTESIAN_POINT ( 'NONE',  ( -38.83547189680000145, 1453.431358638529900, 269.8277507654979672 ) ) ;
#36261=CARTESIAN_POINT ( 'NONE',  ( -24.11880918795291606, 1435.788364753321275, 210.9889112370256044 ) ) ;
#36262=CARTESIAN_POINT ( 'NONE',  ( 6.733046173459999117, 1443.913060387330006, 154.8821828340979891 ) ) ;
#36264=FACE_OUTER_BOUND ( 'NONE', #29989, .T. ) ;
#36265=CARTESIAN_POINT ( 'NONE',  ( 2.923521462801879967, 1410.394928839790055, 231.6309329194170061 ) ) ;
#36266=CARTESIAN_POINT ( 'NONE',  ( -1.556584322539999787, 1415.163755998629995, 226.9904013962980116 ) ) ;
#36267=CARTESIAN_POINT ( 'NONE',  ( -4.185496514609999608, 1416.327449659429931, 232.4314624903980189 ) ) ;
#36269=CARTESIAN_POINT ( 'NONE',  ( -44.07818812065350045, 1430.685783913769910, 266.7420579915649910 ) ) ;
#36270=CARTESIAN_POINT ( 'NONE',  ( -2.695125831749999978, 1436.928758190210146, 184.7684663464980019 ) ) ;
#36273=VERTEX_POINT ( 'NONE', #108793 ) ;
#36276=CARTESIAN_POINT ( 'NONE',  ( -20.61546995249999981, 1508.365016819329867, 190.3615313952979875 ) ) ;
#36277=CARTESIAN_POINT ( 'NONE',  ( -14.19908403099999994, 1410.402768462430004, 190.3287729933980188 ) ) ;
#36282=FACE_OUTER_BOUND ( 'NONE', #19556, .T. ) ;
#36283=CARTESIAN_POINT ( 'NONE',  ( 11.60004869885203682, 1424.919886225515711, 136.4495339943606211 ) ) ;
#36287=ORIENTED_EDGE ( 'NONE', *, *, #72591, .F. ) ;
#36288=CARTESIAN_POINT ( 'NONE',  ( -16.87533949840419822, 1410.935239512470162, 270.3978791998690099 ) ) ;
#36290=CARTESIAN_POINT ( 'NONE',  ( -28.12789902060000102, 1435.479491205339855, 135.2461919473980174 ) ) ;
#36297=CARTESIAN_POINT ( 'NONE',  ( -1.138272880244320051, 1409.887086923559764, 185.4055134639719995 ) ) ;
#36298=CARTESIAN_POINT ( 'NONE',  ( 3.659006180651771967, 1425.028668711506043, 184.9642397768932938 ) ) ;
#36300=CARTESIAN_POINT ( 'NONE',  ( -19.89499272040000122, 1430.791176822330044, 223.1073517981980103 ) ) ;
#36301=CARTESIAN_POINT ( 'NONE',  ( 5.279745845456099929, 1475.319256162549891, 269.4988495444229670 ) ) ;
#36303=CARTESIAN_POINT ( 'NONE',  ( 10.27269517170000057, 1447.035794548080048, 186.9035346276980079 ) ) ;
#36304=( BOUNDED_CURVE ( )  B_SPLINE_CURVE ( 3, ( #58825, #24630, #67244, #86221 ),
 .UNSPECIFIED., .F., .T. ) 
 B_SPLINE_CURVE_WITH_KNOTS ( ( 4, 4 ),
 ( 1.191031352841563917, 1.212284566114525841 ),
 .UNSPECIFIED. ) 
 CURVE ( )  GEOMETRIC_REPRESENTATION_ITEM ( )  RATIONAL_B_SPLINE_CURVE ( ( 1.000000000000000000, 0.9999623587646855327, 0.9999623587646855327, 1.000000000000000000 ) ) 
 REPRESENTATION_ITEM ( '' )  );
#36307=CARTESIAN_POINT ( 'NONE',  ( 19.03110457515579768, 1457.047041246000163, 226.1578386336209974 ) ) ;
#36308=CARTESIAN_POINT ( 'NONE',  ( 1.472146761774899781, 1484.510777100460018, 182.0990331927370107 ) ) ;
#36309=VERTEX_POINT ( 'NONE', #57858 ) ;
#36311=CARTESIAN_POINT ( 'NONE',  ( 26.21478449920509846, 1450.935004627359831, 136.5697675719979713 ) ) ;
#36312=CARTESIAN_POINT ( 'NONE',  ( -15.81201443571409904, 1506.433683733589987, 193.8503163142329981 ) ) ;
#36315=CARTESIAN_POINT ( 'NONE',  ( 17.68757587670000220, 1410.455303309029887, 192.9846075591979968 ) ) ;
#36317=CARTESIAN_POINT ( 'NONE',  ( 2.601738789480323000, 1439.644030142424072, 183.4006585331323720 ) ) ;
#36319=CARTESIAN_POINT ( 'NONE',  ( -23.64337456402409998, 1435.765682558080016, 212.0350035351450231 ) ) ;
#36321=CARTESIAN_POINT ( 'NONE',  ( 29.02628104525710029, 1509.926680456929944, 206.2525988547419900 ) ) ;
#36323=FACE_OUTER_BOUND ( 'NONE', #20511, .T. ) ;
#36324=VERTEX_POINT ( 'NONE', #32639 ) ;
#36327=CARTESIAN_POINT ( 'NONE',  ( -0.5016765698272009910, 1409.762109374920101, 233.0393131857059927 ) ) ;
#36328=ADVANCED_FACE ( 'NONE', ( #15795 ), #4352, .F. ) ;
#36329=CARTESIAN_POINT ( 'NONE',  ( 1232.316865285700032, 2833.596074015789782, -9639.481875267569194 ) ) ;
#36332=EDGE_CURVE ( 'NONE', #46325, #28853, #25358, .T. ) ;
#36334=CARTESIAN_POINT ( 'NONE',  ( -8.518323187880001868, 1460.717990423530182, 243.9198229205979942 ) ) ;
#36335=CARTESIAN_POINT ( 'NONE',  ( 15.79259708711904686, 1474.064254307462761, 266.8744062780497757 ) ) ;
#36337=CARTESIAN_POINT ( 'NONE',  ( 11.87682525570000003, 1433.080808133479877, 149.9786264939980072 ) ) ;
#36340=EDGE_CURVE ( 'NONE', #103319, #47969, #33543, .T. ) ;
#36341=B_SPLINE_SURFACE_WITH_KNOTS ( 'NONE', 5, 1, ( 
 ( #53733, #96253 ),
 ( #55367, #62691 ),
 ( #96813, #29585 ),
 ( #55918, #72183 ),
 ( #98445, #63770 ),
 ( #80002, #44767 ),
 ( #27945, #20084 ),
 ( #81092, #54818 ),
 ( #88943, #87871 ),
 ( #71084, #21714 ),
 ( #11161, #21160 ),
 ( #64323, #104648 ),
 ( #12236, #19528 ),
 ( #78918, #89499 ),
 ( #2224, #72714 ),
 ( #97886, #54277 ),
 ( #45322, #106837 ),
 ( #12792, #88402 ),
 ( #3325, #106302 ),
 ( #3873, #79460 ),
 ( #46970, #37450 ),
 ( #30131, #10596 ),
 ( #11695, #38536 ),
 ( #46425, #36891 ) ),
 .UNSPECIFIED., .F., .F., .F.,
 ( 6, 3, 3, 3, 3, 3, 3, 6 ),
 ( 2, 2 ),
 ( -1.071643382647970112E-05, 1.787098717269999915, 3.575031044529999757, 7.150895699039999442, 35.35713560909999842, 55.42405856439999923, 74.38977909560000512, 84.36278581140000199 ),
 ( 2.018281005271230111, 3.029715956260000009 ),
 .UNSPECIFIED. ) ;
#36344=DIRECTION ( 'NONE',  ( 0.7071067811860475283, 0.000000000000000000, 0.7071067811870476172 ) ) ;
#36345=CARTESIAN_POINT ( 'NONE',  ( 24.09734436609999975, 1435.413501786879806, 137.5049309707980001 ) ) ;
#36346=CARTESIAN_POINT ( 'NONE',  ( -12.16611854289999961, 1486.038279009429971, 184.6517507125980160 ) ) ;
#36347=CARTESIAN_POINT ( 'NONE',  ( 7.982414096761766942, 1398.150145363782258, 198.8611880334231330 ) ) ;
#36349=CARTESIAN_POINT ( 'NONE',  ( 25.18172488799999797, 1449.799985342450100, 212.0110979567280083 ) ) ;
#36351=CARTESIAN_POINT ( 'NONE',  ( -15.46915279469999938, 1508.458298799929935, 231.5778441731980024 ) ) ;
#36353=CARTESIAN_POINT ( 'NONE',  ( 20.04224800140000085, 1476.152569352130058, 225.0639570481980059 ) ) ;
#36354=CARTESIAN_POINT ( 'NONE',  ( 2.499941270706060426, 1419.920042689079992, 110.8944432325759948 ) ) ;
#36355=ADVANCED_FACE ( 'NONE', ( #17452 ), #83061, .T. ) ;
#36357=CARTESIAN_POINT ( 'NONE',  ( 0.1656846011524400197, 1482.872822838080083, 181.9709779989089782 ) ) ;
#36359=VERTEX_POINT ( 'NONE', #21857 ) ;
#36360=CARTESIAN_POINT ( 'NONE',  ( -0.4725090650170000184, 1450.961208915830184, 181.9239884144979840 ) ) ;
#36362=CARTESIAN_POINT ( 'NONE',  ( -20.24816999180000110, 1507.884035326030016, 189.2341655923979999 ) ) ;
#36366=VERTEX_POINT ( 'NONE', #104805 ) ;
#36369=CARTESIAN_POINT ( 'NONE',  ( -16.06428786779999740, 1414.913060387329779, 209.3174441332850222 ) ) ;
#36376=CARTESIAN_POINT ( 'NONE',  ( 10.49013805814599998, 1409.279384075129883, 219.7750123596210017 ) ) ;
#36379=CARTESIAN_POINT ( 'NONE',  ( -18.01683494470000113, 1424.194020404830098, 193.0485151117980251 ) ) ;
#36381=ORIENTED_EDGE ( 'NONE', *, *, #18672, .F. ) ;
#36383=CARTESIAN_POINT ( 'NONE',  ( -0.7133045362011090074, 1467.033258661540003, 237.5733310560259781 ) ) ;
#36384=FACE_OUTER_BOUND ( 'NONE', #8856, .T. ) ;
#36387=CARTESIAN_POINT ( 'NONE',  ( 28.15442102719999795, 1509.896234434229882, 217.4026611133980111 ) ) ;
#36390=CARTESIAN_POINT ( 'NONE',  ( 29.51859446050732316, 1509.963736870992079, 211.6832300364890500 ) ) ;
#36391=CARTESIAN_POINT ( 'NONE',  ( 21.58938658888978779, 1409.666978379882949, 207.8232565829630119 ) ) ;
#36392=CARTESIAN_POINT ( 'NONE',  ( -28.27930516629999858, 1508.150008668130113, 209.2731387451690068 ) ) ;
#36395=CARTESIAN_POINT ( 'NONE',  ( -0.1714601298129999896, 1471.143170311029962, 182.4338783372979833 ) ) ;
#36399=CARTESIAN_POINT ( 'NONE',  ( 6.160531803039999588, 1422.363866332430007, 133.5160842810979887 ) ) ;
#36400=CARTESIAN_POINT ( 'NONE',  ( -0.3821804589910179906, 1506.433683733660018, 187.1424611576989889 ) ) ;
#36402=CARTESIAN_POINT ( 'NONE',  ( 41.46340468307529648, 1444.106639930779920, 136.3851283920170090 ) ) ;
#36404=CARTESIAN_POINT ( 'NONE',  ( 45.67178422140000293, 1440.913060379869876, 266.1886048774979940 ) ) ;
#36405=CARTESIAN_POINT ( 'NONE',  ( -24.95209251639999692, 1469.238639858829856, 202.6470309557579981 ) ) ;
#36406=CARTESIAN_POINT ( 'NONE',  ( -10.78182592408190033, 1425.674068949819912, 99.91377539918158845 ) ) ;
#36407=CARTESIAN_POINT ( 'NONE',  ( 16.22603119529000182, 1409.504885741160024, 192.8289540260319939 ) ) ;
#36410=CARTESIAN_POINT ( 'NONE',  ( -22.15551762850000017, 1489.466917449829907, 208.0059448184480004 ) ) ;
#36411=CARTESIAN_POINT ( 'NONE',  ( -24.64758684779999953, 1426.171069946930174, 240.2509105751980201 ) ) ;
#36413=CARTESIAN_POINT ( 'NONE',  ( 29.15335220830669982, 1509.735908697959758, 209.5818691752959921 ) ) ;
#36415=CARTESIAN_POINT ( 'NONE',  ( 20.59684415428669979, 1507.762623717989982, 227.6602567528719874 ) ) ;
#36419=CARTESIAN_POINT ( 'NONE',  ( 37.77042218360499959, 1442.790213541490175, 137.1073832719119991 ) ) ;
#36421=ORIENTED_EDGE ( 'NONE', *, *, #85304, .F. ) ;
#36424=EDGE_CURVE ( 'NONE', #54363, #67527, #73654, .T. ) ;
#36425=ORIENTED_EDGE ( 'NONE', *, *, #82003, .T. ) ;
#36426=CARTESIAN_POINT ( 'NONE',  ( 13.37406854550570046, 1507.496451373729997, 233.0472692220099873 ) ) ;
#36429=CARTESIAN_POINT ( 'NONE',  ( -11.43754841480000017, 1461.185958034129953, 231.4422348057979946 ) ) ;
#36432=CARTESIAN_POINT ( 'NONE',  ( 0.2576823252080000515, 1419.224537961029910, 184.6439154818979773 ) ) ;
#36437=CARTESIAN_POINT ( 'NONE',  ( 11.86064628478500005, 1431.955178181789961, 149.9690613615080110 ) ) ;
#36441=DIRECTION ( 'NONE',  ( 0.000000000000000000, -1.000000000000000000, 0.000000000000000000 ) ) ;
#36446=CARTESIAN_POINT ( 'NONE',  ( -4.746427511560000312, 1423.669336908029891, 184.8320719503979888 ) ) ;
#36447=CARTESIAN_POINT ( 'NONE',  ( 4.188705820677620650, 1409.351545472750104, 270.3708454374540224 ) ) ;
#36452=CIRCLE ( 'NONE', #86485, 3.994150673153873399 ) ;
#36455=DIRECTION ( 'NONE',  ( 0.000000000000000000, 0.7071067811865474617, 0.7071067811865474617 ) ) ;
#36459=EDGE_LOOP ( 'NONE', ( #87173, #13435, #83509, #63033 ) ) ;
#36460=CARTESIAN_POINT ( 'NONE',  ( 14.73695825489999933, 1419.186926028530252, 255.3819207742980097 ) ) ;
#36465=B_SPLINE_SURFACE_WITH_KNOTS ( 'NONE', 5, 5, ( 
 ( #44788, #78938, #36360, #70551, #104670, #90615, #21734, #73278, #5519 ),
 ( #47531, #29607, #81652, #13339, #89518, #81113, #13895, #107416, #30712 ),
 ( #64898, #99006, #30151, #63258, #63793, #22281, #56484, #4957, #54841 ),
 ( #48081, #4430, #99558, #73842, #82215, #39101, #90056, #39674, #97907 ),
 ( #12256, #46445, #107969, #54298, #31266, #80577, #46989, #3892, #65448 ),
 ( #106324, #64342, #98465, #88965, #38023, #38556, #55386, #72202, #105792 ),
 ( #88427, #21178, #72734, #106860, #37470, #11717, #55937, #45888, #80025 ),
 ( #3346, #97367, #20639, #12809, #71673, #29074, #59251, #74401, #83323 ),
 ( #66006, #84429, #83870, #6067, #14996, #109635, #40220, #93369, #76030 ) ),
 .UNSPECIFIED., .F., .F., .F.,
 ( 6, 3, 6 ),
 ( 6, 3, 6 ),
 ( 1.581906524000000092, 2.897190900920000090, 4.210865504630000089 ),
 ( 0.000000000000000000, 1.000000000000000000, 2.000000000000000000 ),
 .UNSPECIFIED. ) ;
#36469=CARTESIAN_POINT ( 'NONE',  ( -12.81436613661749924, 1447.032455685610103, 185.6742731520540133 ) ) ;
#36472=CARTESIAN_POINT ( 'NONE',  ( 18.18137294690000161, 1507.608465325429734, 188.5297611294979845 ) ) ;
#36473=CARTESIAN_POINT ( 'NONE',  ( -24.22142878869999905, 1443.578504641800009, 212.3984149774479988 ) ) ;
#36478=CARTESIAN_POINT ( 'NONE',  ( 28.12945447419999923, 1510.024089002930168, 194.4010711305979839 ) ) ;
#36479=CIRCLE ( 'NONE', #47207, 95.87929217111340563 ) ;
#36481=CARTESIAN_POINT ( 'NONE',  ( -5.386185223340929973, 1432.347042777500064, 154.6076275972019971 ) ) ;
#36482=CARTESIAN_POINT ( 'NONE',  ( 5.914165527020000646, 1417.414484838129965, 231.4237124127979826 ) ) ;
#36485=CARTESIAN_POINT ( 'NONE',  ( -15.94730198739999949, 1459.284216063530039, 229.6241229289979913 ) ) ;
#36487=CARTESIAN_POINT ( 'NONE',  ( 39.48010127979999595, 1422.408814482829939, 266.8920267569980069 ) ) ;
#36490=CARTESIAN_POINT ( 'NONE',  ( 18.94140730250000004, 1435.974603093500036, 146.3778792160980231 ) ) ;
#36491=CARTESIAN_POINT ( 'NONE',  ( 21.17607668140000143, 1469.155376887830016, 194.0056914575980329 ) ) ;
#36493=CARTESIAN_POINT ( 'NONE',  ( 5.386185205460879644, 1432.347042709529887, 154.6076275981190236 ) ) ;
#36495=CARTESIAN_POINT ( 'NONE',  ( -31.50880186010000017, 1466.258756145929965, 266.5723332967979786 ) ) ;
#36499=CARTESIAN_POINT ( 'NONE',  ( -6.448255163698850545, 1408.606950372470010, 197.2260920424329811 ) ) ;
#36501=CARTESIAN_POINT ( 'NONE',  ( -13.57767673750000093, 1442.998007393829994, 188.1052366738979913 ) ) ;
#36502=CARTESIAN_POINT ( 'NONE',  ( -27.79335146049099947, 1508.202759685119872, 210.4818766450680130 ) ) ;
#36503=CARTESIAN_POINT ( 'NONE',  ( -33.91369295919999871, 1437.010537939619780, 136.5611922338979696 ) ) ;
#36504=CARTESIAN_POINT ( 'NONE',  ( -10.16993673199276671, 1455.367861617207382, 226.0916021546657646 ) ) ;
#36506=FACE_OUTER_BOUND ( 'NONE', #20977, .T. ) ;
#36507=CARTESIAN_POINT ( 'NONE',  ( -14.45571664180179994, 1409.417865136020055, 212.8813991959680152 ) ) ;
#36508=ORIENTED_EDGE ( 'NONE', *, *, #4504, .F. ) ;
#36512=CARTESIAN_POINT ( 'NONE',  ( -31.62532717830000095, 1466.392620420529965, 268.6459143616979759 ) ) ;
#36513=CARTESIAN_POINT ( 'NONE',  ( -17.13990208540000282, 1503.228774872230133, 224.1177471422980148 ) ) ;
#36514=CARTESIAN_POINT ( 'NONE',  ( 0.2707015808795459888, 1419.455472800460029, 184.4597787253470074 ) ) ;
#36519=CARTESIAN_POINT ( 'NONE',  ( 16.60890868733800119, 1423.045925081060204, 227.3707771178220014 ) ) ;
#36520=CARTESIAN_POINT ( 'NONE',  ( 20.61484677210000171, 1508.366076579829951, 227.7402271394979891 ) ) ;
#36521=CARTESIAN_POINT ( 'NONE',  ( 14.29966752569999855, 1463.297110392330069, 223.2977952946979769 ) ) ;
#36525=CARTESIAN_POINT ( 'NONE',  ( -23.07071866700000129, 1409.718707635629926, 208.5793258069899707 ) ) ;
#36526=CARTESIAN_POINT ( 'NONE',  ( 18.05542495199999919, 1416.825784011830137, 208.7596466302789793 ) ) ;
#36527=CARTESIAN_POINT ( 'NONE',  ( -12.60360202350000058, 1416.535385209630022, 194.9281104267980140 ) ) ;
#36529=CARTESIAN_POINT ( 'NONE',  ( 23.01976738670000344, 1409.881403417030015, 211.5932151611179961 ) ) ;
#36530=CARTESIAN_POINT ( 'NONE',  ( -11.95607891459999905, 1433.549464727329905, 149.8823818600980076 ) ) ;
#36535=CARTESIAN_POINT ( 'NONE',  ( -0.1139762647940000123, 1411.657414646530015, 233.3213770427979910 ) ) ;
#36538=CARTESIAN_POINT ( 'NONE',  ( -23.10158782639999941, 1411.031839777530195, 210.9252372482680187 ) ) ;
#36539=AXIS2_PLACEMENT_3D ( 'NONE', #24552, #58740, #5016 ) ;
#36542=CARTESIAN_POINT ( 'NONE',  ( -18.99822365203170094, 1485.804394114710021, 189.5286731071130077 ) ) ;
#36544=CARTESIAN_POINT ( 'NONE',  ( -4.256729589579360429, 1441.274763077670059, 159.9751555247389945 ) ) ;
#36545=VECTOR ( 'NONE', #79500, 1000.000000000000114 ) ;
#36548=ORIENTED_EDGE ( 'NONE', *, *, #25867, .T. ) ;
#36549=CARTESIAN_POINT ( 'NONE',  ( 11.39672343189880088, 1433.938446316660020, 151.4312701205349754 ) ) ;
#36551=ORIENTED_EDGE ( 'NONE', *, *, #91840, .F. ) ;
#36554=CARTESIAN_POINT ( 'NONE',  ( 15.86818584750560035, 1417.144054420810107, 191.3226642558889807 ) ) ;
#36555=CARTESIAN_POINT ( 'NONE',  ( 4.823778297959999684, 1426.859560269130043, 144.1938086916980239 ) ) ;
#36556=DIRECTION ( 'NONE',  ( 1.000000000000000000, 0.000000000000000000, 0.000000000000000000 ) ) ;
#36559=CARTESIAN_POINT ( 'NONE',  ( -24.08412280772440184, 1444.795065662000070, 211.8316922065289987 ) ) ;
#36563=CARTESIAN_POINT ( 'NONE',  ( 13.81908124298479912, 1415.258594621350085, 197.5028968623049934 ) ) ;
#36565=FACE_OUTER_BOUND ( 'NONE', #32153, .T. ) ;
#36566=VERTEX_POINT ( 'NONE', #28511 ) ;
#36567=CARTESIAN_POINT ( 'NONE',  ( 13.51024008597019943, 1434.958051702800049, 149.0116953593919789 ) ) ;
#36580=CARTESIAN_POINT ( 'NONE',  ( 4.223239625950419907, 1446.235523347980006, 167.1961359861499830 ) ) ;
#36586=CARTESIAN_POINT ( 'NONE',  ( 24.64606047185390025, 1440.913060387330006, 237.9243720522470085 ) ) ;
#36588=CARTESIAN_POINT ( 'NONE',  ( -17.69367671410000398, 1508.290913714329918, 186.8003383294980040 ) ) ;
#36589=ORIENTED_EDGE ( 'NONE', *, *, #50187, .F. ) ;
#36591=CARTESIAN_POINT ( 'NONE',  ( -15.18679397699999889, 1410.815794815029903, 190.8549424428979933 ) ) ;
#36593=CARTESIAN_POINT ( 'NONE',  ( -24.38625746622182433, 1440.079494890380602, 212.0144860022579678 ) ) ;
#36594=DIRECTION ( 'NONE',  ( 0.03489949670075159077, -0.9993908270191568244, -1.181473170880211640E-10 ) ) ;
#36595=CARTESIAN_POINT ( 'NONE',  ( -11.06583617882839832, 1414.913527292460003, 196.0153757934279781 ) ) ;
#36596=CARTESIAN_POINT ( 'NONE',  ( 26.07583925208389886, 1441.264734006110075, 138.1452381084750130 ) ) ;
#36597=CARTESIAN_POINT ( 'NONE',  ( -12.06095611880000007, 1433.903655509099963, 149.2721377443980089 ) ) ;
#36598=CARTESIAN_POINT ( 'NONE',  ( 21.17685425119999820, 1435.236150072139935, 141.6298919720979939 ) ) ;
#36599=CARTESIAN_POINT ( 'NONE',  ( 6.115264850039999978, 1465.022781530429938, 233.8169749081980058 ) ) ;
#36601=B_SPLINE_SURFACE_WITH_KNOTS ( 'NONE', 5, 5, ( 
 ( #22076, #90402, #55746, #73640, #81445, #73079, #63598, #46793, #107770 ),
 ( #99348, #80922, #63063, #55192, #88775, #12057, #106660, #29950, #3690 ),
 ( #38351, #64144, #98262, #21531, #18586, #86917, #71264, #10775, #37068 ),
 ( #28673, #69601, #78529, #63412, #52781, #45503, #43820, #19709, #62879 ),
 ( #10209, #44385, #1840, #35975, #37621, #87488, #52235, #44947, #29223 ),
 ( #54454, #9645, #53912, #104277, #97527, #27564, #105385, #79094, #95870 ) ),
 .UNSPECIFIED., .F., .F., .F.,
 ( 6, 6 ),
 ( 6, 3, 6 ),
 ( 39.30566966140000318, 56.26181215439999761 ),
 ( 0.000000000000000000, 1.000000000000000000, 2.000000000000000000 ),
 .UNSPECIFIED. ) ;
#36604=CARTESIAN_POINT ( 'NONE',  ( -26.27875192360060197, 1507.830998981459970, 209.1491001731010044 ) ) ;
#36605=CARTESIAN_POINT ( 'NONE',  ( 27.96976559109999982, 1509.201555290129818, 207.5796322881679998 ) ) ;
#36608=CARTESIAN_POINT ( 'NONE',  ( -18.97219799319119815, 1486.246528605739741, 189.3000344508529906 ) ) ;
#36611=CARTESIAN_POINT ( 'NONE',  ( -0.9518847404100000409, 1415.296882282229944, 227.0497707501980074 ) ) ;
#36612=CARTESIAN_POINT ( 'NONE',  ( 27.24390625040000202, 1454.605078681330042, 244.3119004044979761 ) ) ;
#36613=ADVANCED_FACE ( 'NONE', ( #36905 ), #45338, .F. ) ;
#36616=CARTESIAN_POINT ( 'NONE',  ( 4.363122647530000009, 1416.108409730630001, 162.4768476156980057 ) ) ;
#36617=EDGE_CURVE ( 'NONE', #49524, #38319, #92063, .T. ) ;
#36618=CARTESIAN_POINT ( 'NONE',  ( -18.72510712869999949, 1457.176800226130126, 227.4990798502979885 ) ) ;
#36619=CIRCLE ( 'NONE', #43732, 2.000000000052873261 ) ;
#36621=CARTESIAN_POINT ( 'NONE',  ( 11.86937491419999979, 1432.581104674459993, 149.9818612858980202 ) ) ;
#36622=CARTESIAN_POINT ( 'NONE',  ( 5.360339899599590119, 1422.243068060369978, 144.1383403130810166 ) ) ;
#36627=CARTESIAN_POINT ( 'NONE',  ( 1.328042612950000034, 1406.002643151530037, 266.9604903208979749 ) ) ;
#36631=EDGE_CURVE ( 'NONE', #105296, #98890, #53420, .T. ) ;
#36632=CARTESIAN_POINT ( 'NONE',  ( 6.399316741296109612, 1471.586156901340019, 269.6149390625339493 ) ) ;
#36634=CARTESIAN_POINT ( 'NONE',  ( 5.440910205060000671, 1437.356219380560105, 154.7142170579979847 ) ) ;
#36636=CARTESIAN_POINT ( 'NONE',  ( -39.22252855717829334, 1440.913060397279878, 258.1633042160279388 ) ) ;
#36637=CARTESIAN_POINT ( 'NONE',  ( 37.66833179081890393, 1449.093331502820092, 136.3452658211859898 ) ) ;
#36644=FACE_OUTER_BOUND ( 'NONE', #42901, .T. ) ;
#36647=CARTESIAN_POINT ( 'NONE',  ( -0.5524668390069999990, 1475.317206268129894, 269.4985896541979855 ) ) ;
#36648=DIRECTION ( 'NONE',  ( -0.02952616936612191892, 0.9995640069543085815, 3.638695136259567707E-05 ) ) ;
#36651=LINE ( 'NONE', #38836, #59265 ) ;
#36653=CARTESIAN_POINT ( 'NONE',  ( -17.64235773549999919, 1415.063410501330054, 207.5649593417179801 ) ) ;
#36655=CARTESIAN_POINT ( 'NONE',  ( 26.57374339968509958, 1436.576538602379969, 136.7711906959450232 ) ) ;
#36657=CARTESIAN_POINT ( 'NONE',  ( -8.408055307214409524, 1396.206676148849965, 216.3013428204890261 ) ) ;
#36661=CARTESIAN_POINT ( 'NONE',  ( -16.29312086328269871, 1409.507180582139881, 225.3571590951270025 ) ) ;
#36662=CARTESIAN_POINT ( 'NONE',  ( 11.89544747750000120, 1434.541746328260160, 147.6465872843980094 ) ) ;
#36666=VECTOR ( 'NONE', #43878, 1000.000000000000000 ) ;
#36667=CARTESIAN_POINT ( 'NONE',  ( -11.74015294769649920, 1428.979986577860018, 144.1937977377450011 ) ) ;
#36668=CARTESIAN_POINT ( 'NONE',  ( 10.12215235309999883, 1425.175395598030036, 101.9133589526980046 ) ) ;
#36669=DIRECTION ( 'NONE',  ( -7.229590540988901841E-06, 0.03108153742028734942, -0.9995168522737994943 ) ) ;
#36670=CARTESIAN_POINT ( 'NONE',  ( -16.16285233240872188, 1409.477476458355795, 225.0537141666407592 ) ) ;
#36675=CARTESIAN_POINT ( 'NONE',  ( 6.811012384640000583, 1507.262578865030036, 182.5160571543979984 ) ) ;
#36676=CARTESIAN_POINT ( 'NONE',  ( 0.2612772751870610088, 1416.851343895820037, 190.7759414009450154 ) ) ;
#36682=CARTESIAN_POINT ( 'NONE',  ( -40.71507211770000367, 1443.618860023849948, 137.1015985469979910 ) ) ;
#36683=CARTESIAN_POINT ( 'NONE',  ( -0.2985181081541919967, 1490.954057054879968, 236.6328081109120092 ) ) ;
#36689=CARTESIAN_POINT ( 'NONE',  ( 12.41437396263700066, 1421.386826425689833, 223.7211383651710150 ) ) ;
#36691=CARTESIAN_POINT ( 'NONE',  ( 35.15277841134140147, 1435.727150378580063, 135.4689313601830065 ) ) ;
#36692=CARTESIAN_POINT ( 'NONE',  ( 29.68682906300000113, 1435.534167576209938, 135.1977161657979991 ) ) ;
#36693=CARTESIAN_POINT ( 'NONE',  ( 13.66950429799999966, 1409.390409995830169, 216.6296730155279988 ) ) ;
#36694=CARTESIAN_POINT ( 'NONE',  ( -0.7719351484700760491, 1406.066357371350023, 269.0457477767660066 ) ) ;
#36695=CARTESIAN_POINT ( 'NONE',  ( 40.71369707939999927, 1443.851488934740019, 137.1197025281979904 ) ) ;
#36697=CARTESIAN_POINT ( 'NONE',  ( -11.76903983939999954, 1432.302179094919893, 150.8119321882979875 ) ) ;
#36698=CARTESIAN_POINT ( 'NONE',  ( 13.04724490819999971, 1442.955582623249938, 187.2795607120979753 ) ) ;
#36700=ORIENTED_EDGE ( 'NONE', *, *, #26824, .F. ) ;
#36717=CARTESIAN_POINT ( 'NONE',  ( -5.244631414159999672, 1410.030825445330038, 231.7638218180980232 ) ) ;
#36718=CARTESIAN_POINT ( 'NONE',  ( -12.19576576879999941, 1445.284189276100051, 186.5171162045979827 ) ) ;
#36719=ORIENTED_EDGE ( 'NONE', *, *, #20651, .T. ) ;
#36721=CARTESIAN_POINT ( 'NONE',  ( -24.99421969891459838, 1440.913060486799850, 216.0048573796309768 ) ) ;
#36724=CARTESIAN_POINT ( 'NONE',  ( -25.04882088009999919, 1436.150498452359898, 137.5238809139979992 ) ) ;
#36725=CARTESIAN_POINT ( 'NONE',  ( 34.96986345050569867, 1422.094637478340019, 270.1431711936880333 ) ) ;
#36728=CARTESIAN_POINT ( 'NONE',  ( 0.01932857556553018927, 1507.377889191095164, 237.3808053707595604 ) ) ;
#36734=CARTESIAN_POINT ( 'NONE',  ( 12.27615406349190152, 1509.341753133656539, 182.5553123939410227 ) ) ;
#36735=CARTESIAN_POINT ( 'NONE',  ( -3.618106369209999951, 1415.374423376830009, 232.5614439549979977 ) ) ;
#36737=ORIENTED_EDGE ( 'NONE', *, *, #46016, .F. ) ;
#36741=CARTESIAN_POINT ( 'NONE',  ( 16.37204142619090064, 1469.006598734869840, 229.5670462769519986 ) ) ;
#36743=CARTESIAN_POINT ( 'NONE',  ( -22.70684900021230135, 1509.410791795379964, 226.2783582751810059 ) ) ;
#36744=CARTESIAN_POINT ( 'NONE',  ( -2.825023821920000344, 1409.011712393730022, 187.6092908591980120 ) ) ;
#36745=CARTESIAN_POINT ( 'NONE',  ( -0.3610188369850000356, 1409.865909257629937, 233.1896167169979890 ) ) ;
#36748=CARTESIAN_POINT ( 'NONE',  ( 15.09400015716100008, 1464.825201970499847, 194.8529889085539821 ) ) ;
#36749=CARTESIAN_POINT ( 'NONE',  ( 19.06709222750000166, 1507.978133761729850, 188.5708093027980112 ) ) ;
#36751=EDGE_LOOP ( 'NONE', ( #4776, #49360, #65267, #85096, #41527 ) ) ;
#36752=CARTESIAN_POINT ( 'NONE',  ( -11.48654377540849936, 1414.913057860449953, 197.4148903956670154 ) ) ;
#36756=ADVANCED_FACE ( 'NONE', ( #36506 ), #35963, .T. ) ;
#36763=CARTESIAN_POINT ( 'NONE',  ( 18.08041632129999954, 1415.296882296330068, 210.6774151550479814 ) ) ;
#36765=CARTESIAN_POINT ( 'NONE',  ( -16.07930208289999996, 1436.295294290089942, 148.8862706138980059 ) ) ;
#36767=CARTESIAN_POINT ( 'NONE',  ( -2.446787376320000096, 1432.353341358199941, 150.2884730787980061 ) ) ;
#36768=CARTESIAN_POINT ( 'NONE',  ( 16.16809600799999913, 1413.530257726130003, 191.4342317662980122 ) ) ;
#36770=CARTESIAN_POINT ( 'NONE',  ( 0.5884825575569611056, 1477.920118691090011, 187.7824158287019998 ) ) ;
#36772=VERTEX_POINT ( 'NONE', #63399 ) ;
#36773=CARTESIAN_POINT ( 'NONE',  ( 1.556350644722900078, 1415.152886232740002, 191.3166872668830081 ) ) ;
#36774=CARTESIAN_POINT ( 'NONE',  ( 25.13460091010000141, 1469.176458824629890, 206.2207530469580092 ) ) ;
#36775=CARTESIAN_POINT ( 'NONE',  ( -11.88526718636376067, 1433.193527212150912, 149.9682077723181806 ) ) ;
#36779=CARTESIAN_POINT ( 'NONE',  ( 19.31623058889999811, 1475.513060387329915, 217.5297674309880165 ) ) ;
#36780=CARTESIAN_POINT ( 'NONE',  ( 26.80766065159997069, 1436.328454115282284, 136.7303795916004390 ) ) ;
#36786=CARTESIAN_POINT ( 'NONE',  ( 10.81518794224679958, 1424.921099295370141, 144.1705737284439977 ) ) ;
#36789=CARTESIAN_POINT ( 'NONE',  ( 21.40470761700000324, 1507.840874668130027, 191.1187993005979990 ) ) ;
#36791=FACE_OUTER_BOUND ( 'NONE', #87344, .T. ) ;
#36796=CARTESIAN_POINT ( 'NONE',  ( 18.33918424680000214, 1416.543503932829935, 209.3898435056050005 ) ) ;
#36798=CARTESIAN_POINT ( 'NONE',  ( 12.61676916276099725, 1442.788706415137540, 169.4674284520042988 ) ) ;
#36799=CARTESIAN_POINT ( 'NONE',  ( 35.03707096594791892, 1424.091692757612918, 269.5320251267563094 ) ) ;
#36800=CARTESIAN_POINT ( 'NONE',  ( -1.577671622059999856E-08, 1474.725719134630026, 264.8986983836979903 ) ) ;
#36802=CARTESIAN_POINT ( 'NONE',  ( -11.28694401269999936, 1433.836412287389976, 151.5342276279979785 ) ) ;
#36805=CARTESIAN_POINT ( 'NONE',  ( 11.69034591517040056, 1426.726663316670056, 140.8301495756180088 ) ) ;
#36806=CARTESIAN_POINT ( 'NONE',  ( 5.689812125580000490, 1409.111753005129913, 187.6973877038979879 ) ) ;
#36807=CARTESIAN_POINT ( 'NONE',  ( 6.251976625090000184, 1423.636347555029943, 186.2373219085980054 ) ) ;
#36809=CARTESIAN_POINT ( 'NONE',  ( 9.836119452340000180, 1438.961854673600101, 152.9388124017980317 ) ) ;
#36813=ORIENTED_EDGE ( 'NONE', *, *, #92471, .T. ) ;
#36817=CARTESIAN_POINT ( 'NONE',  ( -42.54899106340000259, 1442.425395630990124, 270.0692087720980226 ) ) ;
#36819=CARTESIAN_POINT ( 'NONE',  ( 3.346415545340000186, 1442.759383208520148, 155.7539078627980018 ) ) ;
#36820=CARTESIAN_POINT ( 'NONE',  ( -15.46960593179999854, 1495.922518723830080, 224.3507688835979934 ) ) ;
#36822=CARTESIAN_POINT ( 'NONE',  ( -11.51310730920000047, 1420.345402828329952, 230.4603701114980083 ) ) ;
#36823=AXIS2_PLACEMENT_3D ( 'NONE', #49419, #9050, #77372 ) ;
#36826=CARTESIAN_POINT ( 'NONE',  ( -45.62046377349849990, 1437.139006798159926, 266.4203617035300340 ) ) ;
#36827=CARTESIAN_POINT ( 'NONE',  ( -2.500000000000000000, 1436.878463555260169, 183.6520988947980015 ) ) ;
#36828=ORIENTED_EDGE ( 'NONE', *, *, #85737, .T. ) ;
#36829=CARTESIAN_POINT ( 'NONE',  ( 24.88936805819999876, 1435.366663778739849, 135.7839653261980004 ) ) ;
#36830=ORIENTED_EDGE ( 'NONE', *, *, #70186, .F. ) ;
#36834=CARTESIAN_POINT ( 'NONE',  ( -12.73441983819999912, 1425.415068379630156, 188.8640771564980128 ) ) ;
#36835=CARTESIAN_POINT ( 'NONE',  ( -27.02393216510709806, 1451.035700111990081, 136.3598584798200193 ) ) ;
#36838=CARTESIAN_POINT ( 'NONE',  ( 3.827327205999999205, 1409.546157813759464, 137.0999999980979851 ) ) ;
#36840=DIRECTION ( 'NONE',  ( 0.7074300732573280959, 0.02470400251971145017, -0.7063514732133270302 ) ) ;
#36843=CARTESIAN_POINT ( 'NONE',  ( -26.80401541404379984, 1414.781986674270001, 270.2830222979230257 ) ) ;
#36845=CARTESIAN_POINT ( 'NONE',  ( -0.7625704858929999164, 1427.674934138829940, 112.4493539157979995 ) ) ;
#36849=EDGE_LOOP ( 'NONE', ( #95781, #76655, #74366, #33588 ) ) ;
#36850=CARTESIAN_POINT ( 'NONE',  ( 45.07050412730048805, 1446.292603878223190, 268.9905583915053171 ) ) ;
#36852=CARTESIAN_POINT ( 'NONE',  ( 3.657938333797013719, 1424.289973031273348, 184.1667673033518895 ) ) ;
#36854=CARTESIAN_POINT ( 'NONE',  ( -18.70785252105190111, 1416.073666489629886, 207.5722946701860110 ) ) ;
#36855=CARTESIAN_POINT ( 'NONE',  ( -19.46569100160000332, 1425.812900638729843, 223.4663329973979842 ) ) ;
#36857=CARTESIAN_POINT ( 'NONE',  ( 5.332756758680099907, 1475.983341725180026, 267.2347467959210121 ) ) ;
#36859=CARTESIAN_POINT ( 'NONE',  ( 5.766269470360000149, 1446.073093314650123, 183.5047901106979964 ) ) ;
#36861=ORIENTED_EDGE ( 'NONE', *, *, #46016, .T. ) ;
#36862=CARTESIAN_POINT ( 'NONE',  ( -14.26333330936780008, 1452.396687514240057, 223.0069981058830137 ) ) ;
#36863=CARTESIAN_POINT ( 'NONE',  ( 1.484957073209509870, 1474.597282977839996, 182.5315330437460091 ) ) ;
#36866=CARTESIAN_POINT ( 'NONE',  ( 25.56660996036589850, 1451.956732796869801, 135.7427434114759990 ) ) ;
#36870=CARTESIAN_POINT ( 'NONE',  ( 17.84430285039999831, 1410.460570803829796, 193.2432472200979987 ) ) ;
#36872=CARTESIAN_POINT ( 'NONE',  ( 16.63042445450000173, 1409.493807611130023, 225.0072295868980063 ) ) ;
#36873=CARTESIAN_POINT ( 'NONE',  ( -19.40238068805140870, 1425.501152276447101, 223.5497471931373923 ) ) ;
#36874=CARTESIAN_POINT ( 'NONE',  ( 0.8680289119235070627, 1450.932674612510027, 182.0391449964180310 ) ) ;
#36875=CARTESIAN_POINT ( 'NONE',  ( 27.68253994085160130, 1507.989615297080036, 207.6661388942010262 ) ) ;
#36877=CARTESIAN_POINT ( 'NONE',  ( 26.20934030730460407, 1446.264570522150279, 137.9472260036899911 ) ) ;
#36883=EDGE_CURVE ( 'NONE', #96481, #660, #33340, .T. ) ;
#36884=CARTESIAN_POINT ( 'NONE',  ( 11040.89558201060572, 2833.596074015790236, -8386.665009981872572 ) ) ;
#36885=CARTESIAN_POINT ( 'NONE',  ( -39.03741743653520047, 1447.683443756730185, 136.5404196528269836 ) ) ;
#36887=CARTESIAN_POINT ( 'NONE',  ( -21.34957048430000270, 1448.971257407479925, 234.3916895749979687 ) ) ;
#36888=CARTESIAN_POINT ( 'NONE',  ( -22.52609268272879817, 1509.699688877640028, 190.9355248210520131 ) ) ;
#36889=CARTESIAN_POINT ( 'NONE',  ( 11.86794208260000083, 1433.007090817639892, 150.2053038657979869 ) ) ;
#36891=CARTESIAN_POINT ( 'NONE',  ( -45.63734427819910167, 1440.913053513229897, 268.9745364329980362 ) ) ;
#36892=CARTESIAN_POINT ( 'NONE',  ( 24.79030299087470013, 1440.913060396060018, 214.6803157916720295 ) ) ;
#36894=CARTESIAN_POINT ( 'NONE',  ( 13.16547634019999968, 1429.085800465429884, 222.6599709325980143 ) ) ;
#36898=CARTESIAN_POINT ( 'NONE',  ( -3.527569048100000160, 1486.518325592330029, 181.8541486797979871 ) ) ;
#36901=CARTESIAN_POINT ( 'NONE',  ( 24.66781776970000095, 1430.359786436929880, 210.6510114860680289 ) ) ;
#36903=CARTESIAN_POINT ( 'NONE',  ( -16.93884357239999972, 1507.634939734329919, 230.1482611379979915 ) ) ;
#36905=FACE_OUTER_BOUND ( 'NONE', #62660, .T. ) ;
#36906=CARTESIAN_POINT ( 'NONE',  ( 5.764290840147539896, 1423.363971970169814, 93.10623776433179444 ) ) ;
#36909=DIRECTION ( 'NONE',  ( 1.000000000000000000, 0.000000000000000000, 0.000000000000000000 ) ) ;
#36911=CARTESIAN_POINT ( 'NONE',  ( -0.9042085446950000049, 1416.833018185029914, 228.0293392571980178 ) ) ;
#36914=CARTESIAN_POINT ( 'NONE',  ( -20.13638283970000131, 1507.886205248129954, 189.0953426691980042 ) ) ;
#36915=CARTESIAN_POINT ( 'NONE',  ( -38.54572101790750338, 1450.058425145499996, 134.0999999982749955 ) ) ;
#36916=ORIENTED_EDGE ( 'NONE', *, *, #2284, .F. ) ;
#36924=CARTESIAN_POINT ( 'NONE',  ( 13.76570265589420039, 1409.393769314739984, 214.9243204603270101 ) ) ;
#36925=CARTESIAN_POINT ( 'NONE',  ( 4.044941532578454790, 1419.921549897504519, 137.0999999980980135 ) ) ;
#36928=CARTESIAN_POINT ( 'NONE',  ( -40.26396455803409680, 1444.186530478750001, 137.1012301494149881 ) ) ;
#36932=ORIENTED_EDGE ( 'NONE', *, *, #21299, .F. ) ;
#36935=CARTESIAN_POINT ( 'NONE',  ( 29.70209480455160289, 1509.984357653646612, 210.2261402311804659 ) ) ;
#36937=CARTESIAN_POINT ( 'NONE',  ( 1.250005296159999890, 1397.324124807030103, 222.0664063312979692 ) ) ;
#36940=CARTESIAN_POINT ( 'NONE',  ( -0.5154891906340001162, 1455.056769859629867, 183.1589657396980044 ) ) ;
#36944=CARTESIAN_POINT ( 'NONE',  ( -13.02075094452810156, 1434.790641786380093, 149.2531060708759867 ) ) ;
#36949=CARTESIAN_POINT ( 'NONE',  ( 41.07185139426759690, 1444.167090557440133, 136.8192919370380025 ) ) ;
#36951=CARTESIAN_POINT ( 'NONE',  ( 6.814834853189999819, 1407.100401533429931, 264.8986986396980114 ) ) ;
#36953=CARTESIAN_POINT ( 'NONE',  ( -26.41621169419999759, 1469.246811866430107, 207.9181783895880073 ) ) ;
#36954=CARTESIAN_POINT ( 'NONE',  ( -10.65149325124349922, 1425.724702697329803, 91.14980580301869395 ) ) ;
#36958=( BOUNDED_CURVE ( )  B_SPLINE_CURVE ( 3, ( #8863, #44152, #25107, #8315 ),
 .UNSPECIFIED., .F., .F. ) 
 B_SPLINE_CURVE_WITH_KNOTS ( ( 4, 4 ),
 ( 5.766256096902659500, 6.404609662640440071 ),
 .UNSPECIFIED. ) 
 CURVE ( )  GEOMETRIC_REPRESENTATION_ITEM ( )  RATIONAL_B_SPLINE_CURVE ( ( 1.000000000000000000, 0.9663293686618639189, 0.9663293686618639189, 1.000000000000000000 ) ) 
 REPRESENTATION_ITEM ( '' )  );
#36959=CARTESIAN_POINT ( 'NONE',  ( -4.026786250540000722, 1408.413060387330006, 137.0999999980979851 ) ) ;
#36960=CARTESIAN_POINT ( 'NONE',  ( -15.89627787769999934, 1415.668893196430190, 250.4785789484980114 ) ) ;
#36961=CARTESIAN_POINT ( 'NONE',  ( 20.30091062346680175, 1509.661473013709838, 230.8308773693809997 ) ) ;
#36963=CARTESIAN_POINT ( 'NONE',  ( -26.31479228349999744, 1435.423696365460046, 135.4819446036979684 ) ) ;
#36964=ADVANCED_FACE ( 'NONE', ( #82909 ), #85106, .T. ) ;
#36965=CARTESIAN_POINT ( 'NONE',  ( 2.738648607395533841, 1448.013770983326594, 154.7581944341845599 ) ) ;
#36966=DIRECTION ( 'NONE',  ( -9.992007221626410836E-16, -0.7071067811865470176, -0.7071067811865480168 ) ) ;
#36972=VERTEX_POINT ( 'NONE', #108664 ) ;
#36976=CARTESIAN_POINT ( 'NONE',  ( -0.2621966296400000118, 1421.807807218729977, 227.6850737390979873 ) ) ;
#36978=CARTESIAN_POINT ( 'NONE',  ( -2.854534533760000325, 1489.061586880230152, 236.0493179470980181 ) ) ;
#36980=EDGE_LOOP ( 'NONE', ( #95214, #78557, #106595, #54488 ) ) ;
#36981=CARTESIAN_POINT ( 'NONE',  ( 45.85445186496249903, 1440.912968281529857, 268.7564834733289558 ) ) ;
#36984=CARTESIAN_POINT ( 'NONE',  ( 13.89849120039999875, 1452.828749846529945, 224.0454814765980132 ) ) ;
#36985=ORIENTED_EDGE ( 'NONE', *, *, #91975, .T. ) ;
#36988=CARTESIAN_POINT ( 'NONE',  ( 11.86362456902309859, 1432.162991587550096, 149.9796059917460127 ) ) ;
#36989=CARTESIAN_POINT ( 'NONE',  ( 13.40902307454580722, 1444.400031499317947, 187.7555987698363538 ) ) ;
#36992=CARTESIAN_POINT ( 'NONE',  ( 5.851689954866730048, 1422.502855755774817, 139.1417834163787575 ) ) ;
#36993=CARTESIAN_POINT ( 'NONE',  ( -13.51702042466202158, 1443.501467202830327, 169.3754641244113373 ) ) ;
#36998=CARTESIAN_POINT ( 'NONE',  ( 16.34988667148460095, 1452.342109763679900, 146.8430469853310001 ) ) ;
#36999=CARTESIAN_POINT ( 'NONE',  ( 3.068142017777439889, 1410.113784448680008, 269.8661674101820154 ) ) ;
#37011=CARTESIAN_POINT ( 'NONE',  ( 37.18025143530000065, 1432.092747987069970, 265.6112251771979800 ) ) ;
#37012=CARTESIAN_POINT ( 'NONE',  ( 13.42933457559999866, 1434.933251406229829, 148.8497112766980308 ) ) ;
#37019=ORIENTED_EDGE ( 'NONE', *, *, #101435, .T. ) ;
#37022=CARTESIAN_POINT ( 'NONE',  ( -11.73653109249999993, 1426.280329148629789, 144.1709412064980143 ) ) ;
#37025=CARTESIAN_POINT ( 'NONE',  ( 18.14165090985069995, 1415.439546991589850, 223.1321341251090189 ) ) ;
#37026=CARTESIAN_POINT ( 'NONE',  ( 5.361911014951845189, 1422.281284793781651, 142.4622902538874314 ) ) ;
#37027=CARTESIAN_POINT ( 'NONE',  ( 27.47350474782500385, 1509.872456313999919, 194.7471083429309999 ) ) ;
#37029=CARTESIAN_POINT ( 'NONE',  ( -8.010413950200000244, 1453.313060387329870, 227.4940039322979999 ) ) ;
#37030=CARTESIAN_POINT ( 'NONE',  ( 15.15971965770000018, 1415.085700719130045, 227.6136599590979870 ) ) ;
#37032=CARTESIAN_POINT ( 'NONE',  ( -16.32411324169200029, 1459.451818037003932, 228.9510944607559964 ) ) ;
#37034=CARTESIAN_POINT ( 'NONE',  ( 39.46828811559999650, 1422.426797802230112, 268.4272099870980242 ) ) ;
#37035=CARTESIAN_POINT ( 'NONE',  ( -19.24864600659999780, 1410.507820697930129, 222.4474005179980054 ) ) ;
#37036=AXIS2_PLACEMENT_3D ( 'NONE', #37561, #64436, #38105 ) ;
#37037=CARTESIAN_POINT ( 'NONE',  ( 21.27861338680000003, 1436.471609301180024, 144.0072822869979916 ) ) ;
#37038=CARTESIAN_POINT ( 'NONE',  ( 21.90978594049999728, 1508.011557042930008, 191.9201679438979795 ) ) ;
#37039=CARTESIAN_POINT ( 'NONE',  ( -16.17519662274699854, 1409.477882727519955, 192.6004389500859872 ) ) ;
#37041=CARTESIAN_POINT ( 'NONE',  ( -0.2153814148640000037, 1475.836819236129941, 266.9611412552980028 ) ) ;
#37043=CARTESIAN_POINT ( 'NONE',  ( -33.91367881351369817, 1435.681798209460112, 135.0664091405390081 ) ) ;
#37044=CARTESIAN_POINT ( 'NONE',  ( -7.626416753354130051, 1407.838202350920028, 198.4036846208539941 ) ) ;
#37045=CARTESIAN_POINT ( 'NONE',  ( -18.20160569639999792, 1416.825421875629900, 205.1678409615580279 ) ) ;
#37046=CARTESIAN_POINT ( 'NONE',  ( -17.60061311809051077, 1410.712255857376476, 193.4350317014313134 ) ) ;
#37047=CARTESIAN_POINT ( 'NONE',  ( -27.88619979645839919, 1508.695391729820130, 210.5767662318619955 ) ) ;
#37049=CARTESIAN_POINT ( 'NONE',  ( -33.92723094509999981, 1436.576986543820112, 136.5095885516980161 ) ) ;
#37050=CARTESIAN_POINT ( 'NONE',  ( -8.145248142631778876, 1456.245062998393223, 227.2183179010753236 ) ) ;
#37053=CARTESIAN_POINT ( 'NONE',  ( -0.3017417235444129764, 1408.923597440540107, 224.1202794661850248 ) ) ;
#37055=VERTEX_POINT ( 'NONE', #101895 ) ;
#37058=CARTESIAN_POINT ( 'NONE',  ( -33.43582158959214468, 1442.831169986189025, 154.5919879262729921 ) ) ;
#37060=CARTESIAN_POINT ( 'NONE',  ( -37.84955692739999478, 1461.864452344229903, 267.2558694692979770 ) ) ;
#37062=CARTESIAN_POINT ( 'NONE',  ( -4.500000000000000000, 1448.210448412289907, 183.1418046154980175 ) ) ;
#37068=CARTESIAN_POINT ( 'NONE',  ( 17.25136325379999747, 1416.823872462129884, 215.4099459140879844 ) ) ;
#37069=CARTESIAN_POINT ( 'NONE',  ( -28.25550469189699854, 1508.223393722109904, 208.8542599017760040 ) ) ;
#37070=CARTESIAN_POINT ( 'NONE',  ( -26.96762182225300108, 1508.002311694569926, 211.4841061306140375 ) ) ;
#37075=CARTESIAN_POINT ( 'NONE',  ( -11.37414570439999828, 1415.063410501330054, 195.5459300842980213 ) ) ;
#37077=CARTESIAN_POINT ( 'NONE',  ( 23.66327964099999903, 1411.099855206130087, 211.3154122771679795 ) ) ;
#37080=CARTESIAN_POINT ( 'NONE',  ( -16.11028175070000046, 1421.340732576330083, 227.0764403262979840 ) ) ;
#37083=CARTESIAN_POINT ( 'NONE',  ( 0.3077026392289999857, 1413.018417486829776, 233.3704243096979951 ) ) ;
#37086=CARTESIAN_POINT ( 'NONE',  ( -22.79695488910000378, 1415.997925189830084, 211.7898339411780171 ) ) ;
#37088=CARTESIAN_POINT ( 'NONE',  ( -1.368198998969730074, 1419.344532540260161, 185.2221260820999760 ) ) ;
#37091=EDGE_CURVE ( 'NONE', #107129, #109428, #58275, .T. ) ;
#37092=CARTESIAN_POINT ( 'NONE',  ( -16.45057082148009897, 1486.105697468709877, 187.2873420190170179 ) ) ;
#37097=ORIENTED_EDGE ( 'NONE', *, *, #6660, .T. ) ;
#37098=B_SPLINE_CURVE_WITH_KNOTS ( 'NONE', 3,
 ( #21273, #44890, #63887, #55482, #89607, #44326, #1783, #95813, #19080, #79040, #30802, #23501, #5052, #81745, #47077, #65537, #47620, #107512, #82860, #99643, #57693, #14545, #4519, #83409, #40307, #48734, #6704, #99096 ),
 .UNSPECIFIED., .F., .F.,
 ( 4, 3, 3, 3, 3, 3, 3, 3, 3, 4 ),
 ( -135.3348859266969839, -117.2219614944759911, -82.53340793120000285, -56.13266858090000255, -37.05188947199999916, -35.60956935775467969, -34.16724924350930337, -32.72651312666420154, -31.25859511619860598, -29.73193251775185786 ),
 .UNSPECIFIED. ) ;
#37099=EDGE_LOOP ( 'NONE', ( #4072, #74777, #87371, #77818, #11449 ) ) ;
#37100=CARTESIAN_POINT ( 'NONE',  ( 28.15885401449999748, 1509.153812686330184, 211.2508761953780265 ) ) ;
#37101=ORIENTED_EDGE ( 'NONE', *, *, #86562, .T. ) ;
#37105=CARTESIAN_POINT ( 'NONE',  ( 15.70001310441050002, 1411.351890569249917, 191.5014854339599992 ) ) ;
#37106=CARTESIAN_POINT ( 'NONE',  ( 15.75924993152980136, 1409.463370494670244, 192.9545979772890121 ) ) ;
#37107=DIRECTION ( 'NONE',  ( -1.000000000000000000, 0.000000000000000000, 0.000000000000000000 ) ) ;
#37108=CARTESIAN_POINT ( 'NONE',  ( -25.36352536740899666, 1450.980594565270167, 137.3053237213029831 ) ) ;
#37110=CARTESIAN_POINT ( 'NONE',  ( 13.52138341930000109, 1409.385237502129939, 227.1744411764980214 ) ) ;
#37113=CARTESIAN_POINT ( 'NONE',  ( 40.55649113733859679, 1439.640597909239887, 134.0999999981079895 ) ) ;
#37116=CARTESIAN_POINT ( 'NONE',  ( -0.5628230732972099304, 1418.319990097900018, 227.8334187985380197 ) ) ;
#37121=ORIENTED_EDGE ( 'NONE', *, *, #70667, .T. ) ;
#37125=CYLINDRICAL_SURFACE ( 'NONE', #70664, 1.500000000000001332 ) ;
#37127=AXIS2_PLACEMENT_3D ( 'NONE', #3870, #46422, #48052 ) ;
#37131=CARTESIAN_POINT ( 'NONE',  ( 11.60004869885203682, 0.000000000000000000, 137.0999999980979851 ) ) ;
#37133=CARTESIAN_POINT ( 'NONE',  ( 4.291176059336820003, 1446.971469614359876, 154.7965853925720126 ) ) ;
#37140=CARTESIAN_POINT ( 'NONE',  ( 31.86551960166520558, 1440.913060387330006, 255.7072771772910187 ) ) ;
#37141=CARTESIAN_POINT ( 'NONE',  ( -16.69460746589999900, 1509.155873805930014, 185.4220695494979907 ) ) ;
#37144=CARTESIAN_POINT ( 'NONE',  ( -13.81938794709999918, 1409.562354991629945, 190.7366003602979845 ) ) ;
#37149=CARTESIAN_POINT ( 'NONE',  ( 22.37294064578369657, 1410.435102231539986, 206.2265387881180061 ) ) ;
#37151=CARTESIAN_POINT ( 'NONE',  ( 27.46336372570400286, 1441.403115843749902, 137.3061811889630235 ) ) ;
#37152=B_SPLINE_CURVE_WITH_KNOTS ( 'NONE', 3,
 ( #18760, #97697, #61925, #20969, #28289, #19313, #79260, #62485, #87091, #29930, #2570, #89298, #12594, #4199, #96605, #87657, #64121, #70886, #19874, #45676, #2011, #54081, #36147, #70331, #79814, #104443, #37248, #27735, #98242, #22055, #90380, #56252, #98793, #83644, #22602, #21512, #56805, #75274, #74173, #100450, #57921, #5290, #13115, #39994, #89843, #90943, #83105, #108301, #30487, #13659, #73057, #23180, #92053, #14229, #55724, #107199, #14787, #91507, #5853, #6399, #40544, #31034, #65216, #49520, #47298, #107751, #23733, #66334, #48973, #74719, #48418, #81422, #99328, #4733, #32146, #108852, #47848, #38876, #6940, #31587, #15325, #65764, #32698, #64676, #41095, #109421, #81982, #39448, #73621, #82561, #99882, #57381, #76921, #100988, #17521, #84743, #102095, #33791, #101530, #109964, #53239, #8040, #87380, #10674, #59569, #24284, #67985, #50611, #110509, #42209, #41657, #44841, #76360, #78995, #2298, #60129, #51162, #25931 ),
 .UNSPECIFIED., .F., .F.,
 ( 4, 3, 3, 3, 3, 3, 3, 3, 3, 3, 3, 3, 3, 3, 3, 3, 3, 3, 3, 3, 3, 3, 3, 3, 3, 3, 3, 3, 3, 3, 3, 3, 3, 3, 3, 3, 3, 3, 3, 4 ),
 ( 0.000000000000000000, 1.208150270900489875, 2.429651893694120268, 3.658664080013049436, 4.894387409778079956, 6.135850761516199903, 7.383699400574919913, 8.633905489600488536, 9.885650277918578865, 10.37921801280000089, 11.62573138507199921, 12.86918051959590059, 14.10827304762559997, 15.34185558769280000, 16.56515402037690166, 17.78190617995440093, 18.98746852701869869, 19.90003809979999971, 21.10030473618510172, 22.30904239636550201, 23.52596673361060198, 24.75067484191579936, 25.98628883277909551, 27.22721929388799822, 28.47521747268259773, 29.42039610570000008, 30.67411275314229968, 31.94530611542449705, 33.20243901502989559, 34.45840916216139505, 35.71192178359849834, 36.99485625054889937, 38.23735636254910020, 39.47464645472779665, 40.70388848455859687, 40.84365965140000299, 42.06598350958260113, 43.28072877285099906, 44.48361342172800192, 45.10384108367830436 ),
 .UNSPECIFIED. ) ;
#37153=B_SPLINE_CURVE_WITH_KNOTS ( 'NONE', 5,
 ( #43986, #78122, #19303, #53504, #29369, #107738, #79803, #88745, #38866, #106091, #99317, #4187, #20408, #71435, #64108 ),
 .UNSPECIFIED., .F., .F.,
 ( 6, 3, 3, 3, 6 ),
 ( 0.000000000000000000, 0.1823333780437425278, 0.5255321158878730747, 0.7212967652657603645, 1.000000000000000000 ),
 .UNSPECIFIED. ) ;
#37155=CARTESIAN_POINT ( 'NONE',  ( -13.19867885639999905, 1434.900411297580149, 148.5640551728980085 ) ) ;
#37156=CARTESIAN_POINT ( 'NONE',  ( 16.10667611295789570, 1435.057002863770549, 146.9490699512605545 ) ) ;
#37157=CARTESIAN_POINT ( 'NONE',  ( 15.69201213754273638, 1410.669748705371148, 191.5225451384409610 ) ) ;
#37159=CIRCLE ( 'NONE', #99697, 2.000006068106865875 ) ;
#37163=FACE_OUTER_BOUND ( 'NONE', #90384, .T. ) ;
#37166=CARTESIAN_POINT ( 'NONE',  ( -21.49889961270000072, 1488.801231227030030, 208.8489735576630153 ) ) ;
#37170=FACE_OUTER_BOUND ( 'NONE', #86771, .T. ) ;
#37171=CARTESIAN_POINT ( 'NONE',  ( 4.804950796049999973, 1465.695272585830025, 240.4142140057979873 ) ) ;
#37175=CARTESIAN_POINT ( 'NONE',  ( -21.38445639540000087, 1453.349625644829985, 224.4824140897979987 ) ) ;
#37177=CARTESIAN_POINT ( 'NONE',  ( 11.58425270890000114, 1432.866135319230125, 151.1952033301980123 ) ) ;
#37178=CARTESIAN_POINT ( 'NONE',  ( 2.500000000000000000, 1419.383414104229814, 144.0748232612980075 ) ) ;
#37183=CARTESIAN_POINT ( 'NONE',  ( 0.8749198469600000250, 1406.783822975030034, 269.6498238079980183 ) ) ;
#37185=VECTOR ( 'NONE', #28130, 1000.000000000000000 ) ;
#37186=EDGE_CURVE ( 'NONE', #72398, #36202, #27482, .T. ) ;
#37188=CARTESIAN_POINT ( 'NONE',  ( 6.659675234235749919, 1473.897714816529970, 270.2927028066139883 ) ) ;
#37190=CARTESIAN_POINT ( 'NONE',  ( 2.478907528220000156, 1433.027990083169925, 157.5361285726980043 ) ) ;
#37191=CARTESIAN_POINT ( 'NONE',  ( 11.60004869885203682, 1424.140514235982437, 136.0100240574817292 ) ) ;
#37192=CARTESIAN_POINT ( 'NONE',  ( -37.15831699375700481, 1440.913060387739961, 254.8961880939840228 ) ) ;
#37194=CARTESIAN_POINT ( 'NONE',  ( -11.86629850686009924, 1432.349867577580198, 149.9824227077560010 ) ) ;
#37196=FACE_OUTER_BOUND ( 'NONE', #30067, .T. ) ;
#37199=ORIENTED_EDGE ( 'NONE', *, *, #48895, .F. ) ;
#37200=CARTESIAN_POINT ( 'NONE',  ( -31.32742178079999462, 1437.308404696490015, 255.3819207742980097 ) ) ;
#37203=CARTESIAN_POINT ( 'NONE',  ( -1.770636241409999867, 1475.812198116930176, 266.9599394754979471 ) ) ;
#37211=CARTESIAN_POINT ( 'NONE',  ( 26.68383462467300049, 1435.975862505480109, 136.4814827833579898 ) ) ;
#37212=CARTESIAN_POINT ( 'NONE',  ( -10.94421840418110037, 1396.295240915489785, 210.8008358220470200 ) ) ;
#37213=CARTESIAN_POINT ( 'NONE',  ( -14.93588953819999965, 1422.319491557630045, 228.4029780258980225 ) ) ;
#37215=CARTESIAN_POINT ( 'NONE',  ( -16.62086504976599954, 1410.867400916760062, 226.5111953344219842 ) ) ;
#37216=CARTESIAN_POINT ( 'NONE',  ( 19.27986066999695680, 1456.016186168368449, 225.1713710279379370 ) ) ;
#37217=ORIENTED_EDGE ( 'NONE', *, *, #36038, .T. ) ;
#37218=CARTESIAN_POINT ( 'NONE',  ( -11.49747572423030029, 1414.913060387329779, 197.9009878255399997 ) ) ;
#37220=CARTESIAN_POINT ( 'NONE',  ( -18.11608073946016617, 1485.171156873887867, 188.9685297383233262 ) ) ;
#37221=CARTESIAN_POINT ( 'NONE',  ( 10.08386706099999941, 1425.185608643229898, 99.60988851169790337 ) ) ;
#37225=CARTESIAN_POINT ( 'NONE',  ( -11.23388613411650105, 1443.913060387330006, 205.3674499604520065 ) ) ;
#37226=AXIS2_PLACEMENT_3D ( 'NONE', #71714, #54339, #47032 ) ;
#37230=CARTESIAN_POINT ( 'NONE',  ( 4.179882439260000027, 1508.490740823229999, 181.1834003096979870 ) ) ;
#37234=CARTESIAN_POINT ( 'NONE',  ( -22.59589169820000265, 1507.700907224229923, 190.9355247910979756 ) ) ;
#37238=CARTESIAN_POINT ( 'NONE',  ( -14.51206241080000048, 1409.419832773630105, 192.1183054032979953 ) ) ;
#37239=CARTESIAN_POINT ( 'NONE',  ( -9.061398245540321028, 1507.228273329460080, 237.0094930597339840 ) ) ;
#37246=CARTESIAN_POINT ( 'NONE',  ( -37.43491952192539429, 1450.745172276120002, 135.6028198332160173 ) ) ;
#37247=CARTESIAN_POINT ( 'NONE',  ( -2.500000000000000000, 1448.210404589970040, 167.6157966154659960 ) ) ;
#37248=CARTESIAN_POINT ( 'NONE',  ( 9.871841148089821161, 1396.257792678529995, 214.1149673374819713 ) ) ;
#37249=CARTESIAN_POINT ( 'NONE',  ( -26.78805561499009968, 1436.761859905399888, 136.7824057165339866 ) ) ;
#37250=CARTESIAN_POINT ( 'NONE',  ( -1.472772997237789872, 1415.954755716330055, 226.2562541087189913 ) ) ;
#37251=CARTESIAN_POINT ( 'NONE',  ( 41.65927937599999353, 1443.915252855300196, 135.6909788338979865 ) ) ;
#37253=CARTESIAN_POINT ( 'NONE',  ( 3.837151314420000237, 1425.396477843930143, 185.3020672648979996 ) ) ;
#37254=CARTESIAN_POINT ( 'NONE',  ( 12.12358720160000125, 1442.555572165430021, 187.1519726473979972 ) ) ;
#37255=VERTEX_POINT ( 'NONE', #18316 ) ;
#37258=EDGE_CURVE ( 'NONE', #64180, #59778, #61469, .T. ) ;
#37264=AXIS2_PLACEMENT_3D ( 'NONE', #22007, #75222, #90898 ) ;
#37266=ORIENTED_EDGE ( 'NONE', *, *, #66601, .F. ) ;
#37275=CARTESIAN_POINT ( 'NONE',  ( -6.440516398849998936, 1409.640628502429990, 231.0932606539979872 ) ) ;
#37279=CARTESIAN_POINT ( 'NONE',  ( 33.12914009259999659, 1451.756166416729911, 134.7383383604980054 ) ) ;
#37280=CARTESIAN_POINT ( 'NONE',  ( -26.31643818619939879, 1440.913060459879944, 223.5219688644119742 ) ) ;
#37282=CARTESIAN_POINT ( 'NONE',  ( 16.61610589626278767, 1423.426877523299481, 227.8835257429488195 ) ) ;
#37284=CARTESIAN_POINT ( 'NONE',  ( 26.02835829290000191, 1413.547636220630011, 269.9886483863980402 ) ) ;
#37285=EDGE_CURVE ( 'NONE', #37407, #93915, #42684, .T. ) ;
#37291=( BOUNDED_SURFACE ( )  B_SPLINE_SURFACE ( 4, 2, ( 
 ( #43211, #50513, #7389, #41554, #67321, #17410, #85741 ),
 ( #84636, #42102, #110398, #33678, #118, #67870, #16855 ),
 ( #42649, #76803, #26952, #1212, #94697, #2331, #61679 ),
 ( #95802, #69534, #53840, #53274, #52167, #36993, #62233 ),
 ( #103655, #27492, #105309, #45428, #71187, #19070, #35347 ) ),
 .UNSPECIFIED., .F., .F., .F. ) 
 B_SPLINE_SURFACE_WITH_KNOTS ( ( 5, 5 ),
 ( 3, 2, 2, 3 ),
 ( 1.967616199060000071, 3.613988937050000239 ),
 ( 11.46118682297159985, 11.46128530315550087, 12.56637061435916003, 12.57442343279650032 ),
 .UNSPECIFIED. ) 
 GEOMETRIC_REPRESENTATION_ITEM ( )  RATIONAL_B_SPLINE_SURFACE ( (
 ( 0.8778316440755170591, 0.8778241674203509648, 0.8778166930676719604, 0.7939440089458740246, 1.000000000000000000, 0.9984984584745990599, 0.9970123125050369683),
 ( 0.8778316440755170591, 0.8778241674203509648, 0.8778166930676719604, 0.7939440089458740246, 1.000000000000000000, 0.9984984584745990599, 0.9970123125050369683),
 ( 0.8778316440755170591, 0.8778241674203509648, 0.8778166930676719604, 0.7939440089458740246, 1.000000000000000000, 0.9984984584745990599, 0.9970123125050369683),
 ( 0.8778316440755170591, 0.8778241674203509648, 0.8778166930676719604, 0.7939440089458740246, 1.000000000000000000, 0.9984984584745990599, 0.9970123125050369683),
 ( 0.8778316440755170591, 0.8778241674203509648, 0.8778166930676719604, 0.7939440089458740246, 1.000000000000000000, 0.9984984584745990599, 0.9970123125050369683) ) ) 
 REPRESENTATION_ITEM ( '' )  SURFACE ( )  );
#37293=ORIENTED_EDGE ( 'NONE', *, *, #48270, .T. ) ;
#37294=CARTESIAN_POINT ( 'NONE',  ( 4.275795800415670200, 1421.906489317239902, 184.1737643678170002 ) ) ;
#37295=CARTESIAN_POINT ( 'NONE',  ( -0.7710674123559999593, 1420.454978029629956, 233.5406515987980072 ) ) ;
#37296=CARTESIAN_POINT ( 'NONE',  ( 5.360168252066184635, 1422.336953262081352, 139.1415641536600276 ) ) ;
#37300=CARTESIAN_POINT ( 'NONE',  ( 10.50998152559020049, 1488.402885203860023, 233.3684635021429870 ) ) ;
#37301=CARTESIAN_POINT ( 'NONE',  ( -20.15451341185540457, 1507.845745166900087, 228.9024278368160026 ) ) ;
#37303=CARTESIAN_POINT ( 'NONE',  ( 0.1764129495400000303, 1409.076774902530133, 232.6426639635980109 ) ) ;
#37304=CARTESIAN_POINT ( 'NONE',  ( -0.04442723591320390381, 1420.445872299549819, 182.6811953437060083 ) ) ;
#37309=ORIENTED_EDGE ( 'NONE', *, *, #52831, .T. ) ;
#37310=CARTESIAN_POINT ( 'NONE',  ( -12.78749341904959991, 1416.842625005220043, 196.1051283137009875 ) ) ;
#37313=CARTESIAN_POINT ( 'NONE',  ( 11.60004869885203327, 1426.466819648586352, 135.9733978570640716 ) ) ;
#37318=CARTESIAN_POINT ( 'NONE',  ( -27.42598290503229919, 1509.711393979569948, 201.1186931426829858 ) ) ;
#37319=CARTESIAN_POINT ( 'NONE',  ( -2.499999992009999783, 1448.405372066850077, 154.5226066568979775 ) ) ;
#37320=CARTESIAN_POINT ( 'NONE',  ( -17.85044820919999964, 1423.477864059130070, 226.0162590187979959 ) ) ;
#37321=CARTESIAN_POINT ( 'NONE',  ( -16.53868516720000059, 1435.074985172869901, 146.6152374475979911 ) ) ;
#37323=CARTESIAN_POINT ( 'NONE',  ( 17.31877846000000076, 1416.204268826130146, 191.9452355195979862 ) ) ;
#37324=CARTESIAN_POINT ( 'NONE',  ( 0.9956485761700990533, 1409.114994398940098, 232.2357569347449839 ) ) ;
#37325=CARTESIAN_POINT ( 'NONE',  ( -18.93888144065705603, 1438.916806179615605, 210.4257881881777053 ) ) ;
#37327=ORIENTED_EDGE ( 'NONE', *, *, #1647, .F. ) ;
#37328=DIRECTION ( 'NONE',  ( 3.740163838737602180E-16, -0.7071067811865475727, -0.7071067811865475727 ) ) ;
#37330=CARTESIAN_POINT ( 'NONE',  ( 11.43185072513739797, 1443.913060387330006, 147.9056598087979921 ) ) ;
#37334=CARTESIAN_POINT ( 'NONE',  ( -18.53418672730000338, 1507.620785846030003, 229.7143111650979961 ) ) ;
#37336=CARTESIAN_POINT ( 'NONE',  ( -17.08684344950000167, 1414.913528139129994, 207.7074066321380030 ) ) ;
#37345=ORIENTED_EDGE ( 'NONE', *, *, #1786, .F. ) ;
#37347=CARTESIAN_POINT ( 'NONE',  ( -0.8266213562413129434, 1417.364321680721559, 235.5374543686832283 ) ) ;
#37348=ORIENTED_EDGE ( 'NONE', *, *, #78052, .T. ) ;
#37349=EDGE_LOOP ( 'NONE', ( #29811, #29080, #75506, #527, #96555, #90999, #47467, #90317, #100578, #12093, #3947, #78139, #8993, #19572, #4956 ) ) ;
#37350=CARTESIAN_POINT ( 'NONE',  ( 18.34590453789999742, 1416.851343897030119, 209.3831232140299790 ) ) ;
#37352=CARTESIAN_POINT ( 'NONE',  ( 13.28748371237506731, 1443.220925009591383, 169.3801757590552768 ) ) ;
#37353=CARTESIAN_POINT ( 'NONE',  ( 36.73277783119023354, 1426.075947637769559, 269.5563403403481288 ) ) ;
#37354=CARTESIAN_POINT ( 'NONE',  ( -32.79493994620000308, 1447.324624203729854, 248.1152222123979811 ) ) ;
#37355=CARTESIAN_POINT ( 'NONE',  ( -20.45323004049999938, 1505.124052112629897, 189.8381095372979814 ) ) ;
#37356=CARTESIAN_POINT ( 'NONE',  ( -11.91180695089999908, 1433.366504895910111, 149.9330032971979847 ) ) ;
#37357=CARTESIAN_POINT ( 'NONE',  ( 27.13474198999999842, 1509.190014491130114, 206.1955381244279693 ) ) ;
#37358=CARTESIAN_POINT ( 'NONE',  ( -18.97220044710000053, 1486.246524106529932, 189.3000240390980196 ) ) ;
#37360=CARTESIAN_POINT ( 'NONE',  ( 12.66769394129999959, 1410.724484346930012, 190.2446672170979980 ) ) ;
#37361=CARTESIAN_POINT ( 'NONE',  ( 5.250757762980000187, 1425.396628029330259, 185.7731830333980270 ) ) ;
#37364=CARTESIAN_POINT ( 'NONE',  ( -17.60627563539999940, 1410.895669412530196, 209.1303365420520208 ) ) ;
#37371=CARTESIAN_POINT ( 'NONE',  ( -20.15863288730000136, 1468.575974982129992, 270.0907409689979772 ) ) ;
#37372=CARTESIAN_POINT ( 'NONE',  ( -23.87637954442272914, 1435.955112056939470, 211.3744525167508641 ) ) ;
#37373=CARTESIAN_POINT ( 'NONE',  ( 4.551914400959999783E-15, 1438.194204504490017, 155.6035180864980134 ) ) ;
#37378=CARTESIAN_POINT ( 'NONE',  ( -12.25907712989999965, 1420.080780804629740, 228.9648508334979908 ) ) ;
#37381=CARTESIAN_POINT ( 'NONE',  ( -45.11974237219880735, 1434.479238661079989, 266.4358854948999920 ) ) ;
#37387=CARTESIAN_POINT ( 'NONE',  ( 11.60004869885203860, 1428.965959225140750, 137.0999999980979851 ) ) ;
#37388=CARTESIAN_POINT ( 'NONE',  ( -15.21150735940000054, 1425.420275960830168, 190.1564087504980023 ) ) ;
#37389=AXIS2_PLACEMENT_3D ( 'NONE', #40265, #82273, #74448 ) ;
#37390=EDGE_CURVE ( 'NONE', #99485, #59125, #106483, .T. ) ;
#37394=CARTESIAN_POINT ( 'NONE',  ( -14.45760366698473476, 1416.831922872548603, 221.3918072960863128 ) ) ;
#37396=AXIS2_PLACEMENT_3D ( 'NONE', #94209, #67949, #68496 ) ;
#37401=CARTESIAN_POINT ( 'NONE',  ( -17.06173606976129875, 1410.334726962669947, 270.2383762330159698 ) ) ;
#37403=CARTESIAN_POINT ( 'NONE',  ( -2.329729395510000245, 1427.373795049630189, 123.0297916884979941 ) ) ;
#37404=FACE_OUTER_BOUND ( 'NONE', #27426, .T. ) ;
#37406=ORIENTED_EDGE ( 'NONE', *, *, #65961, .F. ) ;
#37407=VERTEX_POINT ( 'NONE', #17189 ) ;
#37408=CARTESIAN_POINT ( 'NONE',  ( 42.05250925581326271, 1454.198947671722181, 269.0743982858291474 ) ) ;
#37410=CARTESIAN_POINT ( 'NONE',  ( 3.628297850329112340, 1424.511231154813004, 184.4969362830124169 ) ) ;
#37411=CARTESIAN_POINT ( 'NONE',  ( -2.295166956463912555, 1406.025797069441978, 266.9593544920077761 ) ) ;
#37415=CARTESIAN_POINT ( 'NONE',  ( -23.64337587120000350, 1435.765690983199875, 212.0349968398180067 ) ) ;
#37417=CARTESIAN_POINT ( 'NONE',  ( 22.61120763781960008, 1471.946618767329937, 268.2742167358389906 ) ) ;
#37418=CARTESIAN_POINT ( 'NONE',  ( 12.15086845379999936, 1416.067629296030191, 223.4638310076980190 ) ) ;
#37422=ORIENTED_EDGE ( 'NONE', *, *, #98140, .T. ) ;
#37424=CARTESIAN_POINT ( 'NONE',  ( 1.471210503239640088, 1485.356266705550070, 182.0621681642270175 ) ) ;
#37426=CARTESIAN_POINT ( 'NONE',  ( 7.178570183835717877, 1456.617266911955539, 227.6511887398625618 ) ) ;
#37427=CARTESIAN_POINT ( 'NONE',  ( -18.89905695062199698, 1416.828039266840278, 207.5749027128360069 ) ) ;
#37428=CARTESIAN_POINT ( 'NONE',  ( -23.10251492229999926, 1410.654477831930080, 210.9078341742080056 ) ) ;
#37431=CARTESIAN_POINT ( 'NONE',  ( 21.12232554610000079, 1409.814838513229915, 201.9876924679279853 ) ) ;
#37432=CARTESIAN_POINT ( 'NONE',  ( -2.500000000000000000, 1447.900699890634087, 170.5263301012278703 ) ) ;
#37433=CARTESIAN_POINT ( 'NONE',  ( -25.45241361353140164, 1455.866316869260118, 210.5319270057530048 ) ) ;
#37435=CARTESIAN_POINT ( 'NONE',  ( 0.5698001572631269385, 1450.893161896769925, 181.2939298055520112 ) ) ;
#37437=CARTESIAN_POINT ( 'NONE',  ( 2.500000000000000000, 1439.336914142910018, 160.7446215807900103 ) ) ;
#37444=CARTESIAN_POINT ( 'NONE',  ( -11113.05219664940705, 50.13405481578727318, 8751.225064238135019 ) ) ;
#37445=CARTESIAN_POINT ( 'NONE',  ( -38.21397471328810269, 1448.627478676439978, 136.4064453422460303 ) ) ;
#37447=CARTESIAN_POINT ( 'NONE',  ( -6.850948850460000017, 1456.378850171129898, 224.8635561661979807 ) ) ;
#37448=CARTESIAN_POINT ( 'NONE',  ( -2.643034510968909956, 1464.878779939289871, 184.1462389150400156 ) ) ;
#37449=CARTESIAN_POINT ( 'NONE',  ( 11.42365759299999972, 1433.140261693259845, 151.3530816855979992 ) ) ;
#37450=CARTESIAN_POINT ( 'NONE',  ( -45.39783323183259967, 1444.747477121759857, 268.9810394864909995 ) ) ;
#37455=CARTESIAN_POINT ( 'NONE',  ( 22.84654337450259831, 1507.483738429069717, 210.0129884701899812 ) ) ;
#37457=CARTESIAN_POINT ( 'NONE',  ( -19.36230209990018025, 1485.611961570589528, 189.8635189068809268 ) ) ;
#37459=CARTESIAN_POINT ( 'NONE',  ( 2.376090132089999862, 1482.817598545530018, 234.9716043272979960 ) ) ;
#37460=AXIS2_PLACEMENT_3D ( 'NONE', #86172, #96232, #103513 ) ;
#37462=CARTESIAN_POINT ( 'NONE',  ( -15.36975367949999871, 1507.878415112629909, 231.4074980585979802 ) ) ;
#37465=CARTESIAN_POINT ( 'NONE',  ( 5.555191409685329873, 1422.974801224869907, 110.9492657717959929 ) ) ;
#37467=CARTESIAN_POINT ( 'NONE',  ( 1.422559892400000026, 1466.356769739329820, 235.0198037906980062 ) ) ;
#37469=EDGE_LOOP ( 'NONE', ( #16287, #101346, #84185, #25871 ) ) ;
#37470=CARTESIAN_POINT ( 'NONE',  ( -1.107844858910000063, 1451.282733439329832, 183.1474623122980177 ) ) ;
#37472=CARTESIAN_POINT ( 'NONE',  ( -25.78156655170059608, 1509.813372604039841, 223.1298223243570078 ) ) ;
#37482=CARTESIAN_POINT ( 'NONE',  ( 23.55007129670912036, 1410.927094386046747, 207.7715154849149144 ) ) ;
#37485=CARTESIAN_POINT ( 'NONE',  ( 12.85129650592379846, 1409.361837545100116, 216.7469526318749899 ) ) ;
#37488=CARTESIAN_POINT ( 'NONE',  ( -18.41416944129999678, 1437.064010179910156, 192.2764675452979759 ) ) ;
#37489=CARTESIAN_POINT ( 'NONE',  ( 24.02863916850529691, 1507.902931906480035, 195.9323055859989893 ) ) ;
#37492=ORIENTED_EDGE ( 'NONE', *, *, #106736, .F. ) ;
#37494=CARTESIAN_POINT ( 'NONE',  ( -11.53151684693130008, 1415.184612914939862, 195.3895478472830121 ) ) ;
#37495=FACE_OUTER_BOUND ( 'NONE', #2851, .T. ) ;
#37496=CARTESIAN_POINT ( 'NONE',  ( 31.15391034571117146, 1461.365240553406920, 269.4835205282784045 ) ) ;
#37498=CARTESIAN_POINT ( 'NONE',  ( 3.911218387687235953, 1414.913060387329779, 224.8752140912787354 ) ) ;
#37500=CARTESIAN_POINT ( 'NONE',  ( -1.197234916440000019, 1467.463882650130017, 182.9502258106980150 ) ) ;
#37502=CARTESIAN_POINT ( 'NONE',  ( -26.76690114070098758, 1436.758409284090476, 136.7827424958600204 ) ) ;
#37505=CARTESIAN_POINT ( 'NONE',  ( -12.96903165645690059, 1434.787792369200133, 149.4958389638820222 ) ) ;
#37507=B_SPLINE_SURFACE_WITH_KNOTS ( 'NONE', 4, 5, ( 
 ( #33857, #69712, #68048, #837, #8648, #59632 ),
 ( #85924, #41713, #9227, #77533, #101596, #110572 ),
 ( #7559, #75873, #15933, #42825, #59088, #8101 ),
 ( #43385, #50136, #25990, #17022, #93210, #16479 ),
 ( #35520, #102695, #103832, #52352, #34418, #34963 ) ),
 .UNSPECIFIED., .F., .F., .F.,
 ( 5, 5 ),
 ( 6, 6 ),
 ( 6.734755223250000533, 23.51228018150000310 ),
 ( -2.775557561569999727E-17, 1.000000000000000000 ),
 .UNSPECIFIED. ) ;
#37508=CARTESIAN_POINT ( 'NONE',  ( 1.341974321609999743, 1416.832348283729971, 190.1632194751979910 ) ) ;
#37510=CARTESIAN_POINT ( 'NONE',  ( -16.22971081790149839, 1485.231972063210151, 229.4479590017650139 ) ) ;
#37511=CARTESIAN_POINT ( 'NONE',  ( 41.63873300600299387, 1444.030015486870070, 135.9017893062919882 ) ) ;
#37512=ORIENTED_EDGE ( 'NONE', *, *, #38968, .F. ) ;
#37514=CARTESIAN_POINT ( 'NONE',  ( 7.132053334199999206, 1405.830928060730230, 267.2558864130979828 ) ) ;
#37515=CARTESIAN_POINT ( 'NONE',  ( -26.91706399349999757, 1488.687396145830007, 206.2930393126480055 ) ) ;
#37516=CARTESIAN_POINT ( 'NONE',  ( -10.04958432075110153, 1425.197681561259969, 97.53048915649959838 ) ) ;
#37517=CARTESIAN_POINT ( 'NONE',  ( -0.7038401922759969231, 1507.336008941910222, 231.8508856179180100 ) ) ;
#37519=AXIS2_PLACEMENT_3D ( 'NONE', #48077, #46985, #30147 ) ;
#37520=CARTESIAN_POINT ( 'NONE',  ( -5.038677021079999818, 1414.987262864929789, 244.5742075775979743 ) ) ;
#37522=ADVANCED_FACE ( 'NONE', ( #21068 ), #56211, .T. ) ;
#37524=CARTESIAN_POINT ( 'NONE',  ( 32.73687869649999982, 1451.769863600429971, 134.7502305315980209 ) ) ;
#37526=CARTESIAN_POINT ( 'NONE',  ( -2.500000000000000000, 1429.342233201230101, 157.2075084771979903 ) ) ;
#37528=CARTESIAN_POINT ( 'NONE',  ( 5.943024939599999001, 1509.160954526729938, 238.4862494313980221 ) ) ;
#37531=CARTESIAN_POINT ( 'NONE',  ( -10.56484691688378597, 1423.845928272108267, 137.4577028072829421 ) ) ;
#37532=CARTESIAN_POINT ( 'NONE',  ( -22.81024108693009822, 1409.709601909520188, 208.9207945697700097 ) ) ;
#37536=CARTESIAN_POINT ( 'NONE',  ( 4.500000000000000000, 1425.929641636930000, 183.3886486283980162 ) ) ;
#37537=CARTESIAN_POINT ( 'NONE',  ( 4.219439073160000220, 1441.595895977600094, 127.8666744532979891 ) ) ;
#37538=CARTESIAN_POINT ( 'NONE',  ( -1.976821269320000019, 1489.062954066330121, 236.2429157177979846 ) ) ;
#37539=CARTESIAN_POINT ( 'NONE',  ( 5.409864550977149911, 1440.893826613949841, 154.8143284419219867 ) ) ;
#37541=CARTESIAN_POINT ( 'NONE',  ( 11.73643181629999965, 1426.280401702730160, 144.1638243103979846 ) ) ;
#37542=CARTESIAN_POINT ( 'NONE',  ( -12.02797161415869986, 1415.088136167450102, 221.1177398843049957 ) ) ;
#37543=CARTESIAN_POINT ( 'NONE',  ( 14.91364890520000053, 1485.710536188930064, 225.0739173850980137 ) ) ;
#37547=CARTESIAN_POINT ( 'NONE',  ( 11.83309251696740105, 1430.099177678210026, 149.5098043249829800 ) ) ;
#37550=FACE_OUTER_BOUND ( 'NONE', #31966, .T. ) ;
#37557=CARTESIAN_POINT ( 'NONE',  ( 20.52137544053379870, 1452.196438165939981, 142.6117432215559973 ) ) ;
#37559=CARTESIAN_POINT ( 'NONE',  ( 1.438079373956610008, 1409.221132550520224, 270.3713132426580046 ) ) ;
#37561=CARTESIAN_POINT ( 'NONE',  ( 5.402232622379999017E-16, 1413.913060387330006, 209.1218459616979999 ) ) ;
#37564=CARTESIAN_POINT ( 'NONE',  ( 15.89248692530000007, 1471.309462467230105, 194.8090275957980282 ) ) ;
#37566=CARTESIAN_POINT ( 'NONE',  ( 17.98175490010330080, 1423.057749139549969, 225.1621279517349876 ) ) ;
#37569=CARTESIAN_POINT ( 'NONE',  ( 17.87874083579999862, 1415.075539390429867, 265.6112251771979800 ) ) ;
#37570=VECTOR ( 'NONE', #89988, 1000.000000000000000 ) ;
#37574=CARTESIAN_POINT ( 'NONE',  ( 39.26193983301609336, 1423.042221552809906, 269.8021829593399730 ) ) ;
#37579=CARTESIAN_POINT ( 'NONE',  ( -0.8280578839340340114, 1450.871635902641628, 154.2446588023700542 ) ) ;
#37581=CARTESIAN_POINT ( 'NONE',  ( -10.45459916649999954, 1441.816060358160030, 186.8492846416980058 ) ) ;
#37582=CARTESIAN_POINT ( 'NONE',  ( 6.560537731721620247, 1509.222499095490093, 179.2361269201259972 ) ) ;
#37584=CARTESIAN_POINT ( 'NONE',  ( -14.59882275830000076, 1475.513060387329915, 223.7206687204979971 ) ) ;
#37585=CARTESIAN_POINT ( 'NONE',  ( 16.58222327440000399, 1412.750976071529976, 226.6462158149980155 ) ) ;
#37590=CARTESIAN_POINT ( 'NONE',  ( 45.57495757519999557, 1434.881052582139773, 268.2238934247979500 ) ) ;
#37591=CARTESIAN_POINT ( 'NONE',  ( -18.39324904740000122, 1410.479025241530053, 224.0575692145980042 ) ) ;
#37592=B_SPLINE_CURVE_WITH_KNOTS ( 'NONE', 5,
 ( #68748, #102851, #94451, #80988, #98331, #73142, #55812, #30580, #90478 ),
 .UNSPECIFIED., .F., .F.,
 ( 6, 3, 6 ),
 ( 0.000000000000000000, 0.5447623589902206298, 1.000000000000000000 ),
 .UNSPECIFIED. ) ;
#37593=CARTESIAN_POINT ( 'NONE',  ( 17.61383487560000205, 1435.259801188919937, 146.8137243960979959 ) ) ;
#37594=CARTESIAN_POINT ( 'NONE',  ( 22.47117279520000110, 1488.581167089130076, 194.6265784292980072 ) ) ;
#37595=CARTESIAN_POINT ( 'NONE',  ( 29.67496808539234365, 1509.980355513194809, 207.9080589769481833 ) ) ;
#37597=CARTESIAN_POINT ( 'NONE',  ( -21.85618413279999572, 1471.634021946630128, 266.7712522008980613 ) ) ;
#37599=CARTESIAN_POINT ( 'NONE',  ( -39.85331543310000058, 1441.120390181860103, 136.8371630922980273 ) ) ;
#37600=CARTESIAN_POINT ( 'NONE',  ( -8.971317772902260401, 1408.181544129620079, 199.2698409955270051 ) ) ;
#37601=CARTESIAN_POINT ( 'NONE',  ( -12.58432885909999932, 1415.426210663629945, 196.9819687637979939 ) ) ;
#37603=CARTESIAN_POINT ( 'NONE',  ( -12.88966618989999979, 1442.875255404869904, 186.4032537866980022 ) ) ;
#37606=CARTESIAN_POINT ( 'NONE',  ( -27.70478114339999820, 1435.630643383260121, 136.1390072790979957 ) ) ;
#37610=CARTESIAN_POINT ( 'NONE',  ( -6.697668172239800377, 1409.146948113720100, 222.5083809332480200 ) ) ;
#37611=CARTESIAN_POINT ( 'NONE',  ( 13.10742788021580019, 1414.941152333586842, 197.9471227725614426 ) ) ;
#37613=CARTESIAN_POINT ( 'NONE',  ( -4.065119941006720694, 1421.084427985996399, 137.4065821739406772 ) ) ;
#37614=CARTESIAN_POINT ( 'NONE',  ( -37.54399022510000350, 1461.570446756029924, 266.4251594875980231 ) ) ;
#37617=CARTESIAN_POINT ( 'NONE',  ( -26.88792329530000202, 1508.603612637529977, 212.0174590681980078 ) ) ;
#37621=CARTESIAN_POINT ( 'NONE',  ( 14.17095083369999919, 1415.425644477329797, 219.3842840303979926 ) ) ;
#37622=CARTESIAN_POINT ( 'NONE',  ( 15.30965536770000135, 1495.931236920830088, 224.3053488962979998 ) ) ;
#37631=CARTESIAN_POINT ( 'NONE',  ( 22.50003437009999629, 1409.698778901130254, 210.1517532643880202 ) ) ;
#37635=CARTESIAN_POINT ( 'NONE',  ( -16.57624646909999910, 1421.408089520330122, 226.9966418715980012 ) ) ;
#37636=CARTESIAN_POINT ( 'NONE',  ( -11.87490713740000103, 1433.006767100669776, 150.3951466367980174 ) ) ;
#37637=CARTESIAN_POINT ( 'NONE',  ( -11.68514080771860009, 1426.730168479550002, 140.4580954921360103 ) ) ;
#37638=CARTESIAN_POINT ( 'NONE',  ( 0.3110986828880000221, 1414.379630184029793, 233.4276179574980006 ) ) ;
#37639=DIRECTION ( 'NONE',  ( -0.9999999999532290795, -9.321873569642529338E-06, 2.577697155618075134E-06 ) ) ;
#37645=CARTESIAN_POINT ( 'NONE',  ( -23.74108753817469974, 1436.296634041249945, 212.5883363871789982 ) ) ;
#37646=CARTESIAN_POINT ( 'NONE',  ( -15.48464347335860047, 1485.614289314720054, 187.1168877932479973 ) ) ;
#37649=CARTESIAN_POINT ( 'NONE',  ( -4.283857371189049523, 1440.956241081810049, 155.9231041381889895 ) ) ;
#37651=ORIENTED_EDGE ( 'NONE', *, *, #63800, .F. ) ;
#37653=CARTESIAN_POINT ( 'NONE',  ( 27.96002538619999811, 1508.622315501829917, 211.1985762216579872 ) ) ;
#37657=CARTESIAN_POINT ( 'NONE',  ( 1.580871945720000005, 1426.963505220229990, 133.6118001900980232 ) ) ;
#37659=CARTESIAN_POINT ( 'NONE',  ( 11.97724519069999971, 1441.600846913620217, 147.6096801420980000 ) ) ;
#37660=CARTESIAN_POINT ( 'NONE',  ( -25.30806138896770108, 1450.980851669160074, 137.3985563705309971 ) ) ;
#37662=CARTESIAN_POINT ( 'NONE',  ( 5.842743512439999343, 1410.494458809630032, 231.1215182491980045 ) ) ;
#37666=CARTESIAN_POINT ( 'NONE',  ( 41.66177311458239529, 1443.657316189979838, 134.0999999982009854 ) ) ;
#37674=EDGE_LOOP ( 'NONE', ( #63298, #107422, #52880, #93333 ) ) ;
#37678=CARTESIAN_POINT ( 'NONE',  ( 13.00130910693166975, 1451.219797464038720, 150.9319667301929826 ) ) ;
#37681=CARTESIAN_POINT ( 'NONE',  ( -17.63885398217787781, 1447.971996929747547, 217.7157177369595047 ) ) ;
#37684=CARTESIAN_POINT ( 'NONE',  ( 3.456073863659999912, 1414.971339025629959, 192.2203226080980016 ) ) ;
#37688=ORIENTED_EDGE ( 'NONE', *, *, #104411, .F. ) ;
#37689=CARTESIAN_POINT ( 'NONE',  ( 28.96304334425650140, 1440.913060387330006, 249.8538069052020205 ) ) ;
#37692=ORIENTED_EDGE ( 'NONE', *, *, #94421, .T. ) ;
#37694=CARTESIAN_POINT ( 'NONE',  ( -14.04326434459999895, 1410.776247947130059, 190.2283950358979894 ) ) ;
#37697=DIRECTION ( 'NONE',  ( -0.01245851141472737768, -0.0004350606870917433900, -0.9999222950887373118 ) ) ;
#37698=CARTESIAN_POINT ( 'NONE',  ( 22.08732799627270182, 1410.055779663399790, 206.2710209263929926 ) ) ;
#37699=B_SPLINE_CURVE_WITH_KNOTS ( 'NONE', 3,
 ( #52251, #67952, #93115, #61224, #16385, #95338 ),
 .UNSPECIFIED., .F., .F.,
 ( 4, 2, 4 ),
 ( 9.026196891026570071E-07, 0.4991090056710880130, 0.9980282895626380046 ),
 .UNSPECIFIED. ) ;
#37701=CARTESIAN_POINT ( 'NONE',  ( 2.149988386126029882E-09, 1405.989059316979819, 266.9611530767110139 ) ) ;
#37705=CARTESIAN_POINT ( 'NONE',  ( 7.749473586019999694, 1464.901857590230065, 233.2267652364979824 ) ) ;
#37710=CARTESIAN_POINT ( 'NONE',  ( 18.33920247187146302, 1446.399485069377306, 215.8072429957955478 ) ) ;
#37712=CARTESIAN_POINT ( 'NONE',  ( -18.84387474539999729, 1434.822844257510042, 209.4888865856029838 ) ) ;
#37718=CARTESIAN_POINT ( 'NONE',  ( 23.86131649859999726, 1453.015588120629900, 232.0003380056980120 ) ) ;
#37719=CARTESIAN_POINT ( 'NONE',  ( -11.77007789369999990, 1432.382129548040211, 150.8117526338979815 ) ) ;
#37722=CARTESIAN_POINT ( 'NONE',  ( -18.63567686369149712, 1430.070544426440165, 209.4876081949650199 ) ) ;
#37723=CARTESIAN_POINT ( 'NONE',  ( -20.55070256179999788, 1444.800646429470135, 223.1595721194979944 ) ) ;
#37724=DIRECTION ( 'NONE',  ( -0.3390050494209005394, -0.7071067811868606556, -0.6205445805634677292 ) ) ;
#37725=CARTESIAN_POINT ( 'NONE',  ( 0.04704307171739999932, 1470.812340169630033, 188.5971280676980086 ) ) ;
#37729=CARTESIAN_POINT ( 'NONE',  ( 2.101979435200000079, 1406.024670839530017, 266.9594151837979439 ) ) ;
#37733=CARTESIAN_POINT ( 'NONE',  ( 41.13051483880099113, 1450.960394653560115, 270.0519150180469978 ) ) ;
#37736=CARTESIAN_POINT ( 'NONE',  ( 11.60004869885203682, 1422.941111951575749, 135.6422307863141157 ) ) ;
#37739=CARTESIAN_POINT ( 'NONE',  ( -18.18137283769999968, 1507.608465321030053, 229.7139307937979993 ) ) ;
#37740=CARTESIAN_POINT ( 'NONE',  ( 2.295797454685203576, 1449.787077434956245, 154.4026079438378929 ) ) ;
#37743=CARTESIAN_POINT ( 'NONE',  ( -1.438891081339280120, 1452.191228260170192, 183.8587004481619829 ) ) ;
#37745=CARTESIAN_POINT ( 'NONE',  ( 25.91590772989999891, 1441.261220175949802, 138.4451201509980365 ) ) ;
#37748=ORIENTED_EDGE ( 'NONE', *, *, #102772, .F. ) ;
#37749=CARTESIAN_POINT ( 'NONE',  ( -11.47403709489999990, 1414.639208232530109, 262.6648722511980054 ) ) ;
#37750=ADVANCED_FACE ( 'NONE', ( #95469 ), #10349, .T. ) ;
#37754=CARTESIAN_POINT ( 'NONE',  ( -0.5564123471769999441, 1475.757529860029990, 269.0455876596980147 ) ) ;
#37755=B_SPLINE_CURVE_WITH_KNOTS ( 'NONE', 3,
 ( #18815, #95542, #53009, #86587 ),
 .UNSPECIFIED., .F., .F.,
 ( 4, 4 ),
 ( 0.000000000000000000, 1.000000000000000000 ),
 .UNSPECIFIED. ) ;
#37757=CARTESIAN_POINT ( 'NONE',  ( -28.09993212570000054, 1509.169756167430023, 210.4944500219079941 ) ) ;
#37758=CARTESIAN_POINT ( 'NONE',  ( -3.989402217979193033, 1448.297716895625172, 185.0737791360926963 ) ) ;
#37762=CARTESIAN_POINT ( 'NONE',  ( 26.80191237839250107, 1435.454312953110048, 135.5610332147589929 ) ) ;
#37763=CARTESIAN_POINT ( 'NONE',  ( -6.646217445733189955, 1396.145151416729959, 217.9435964253609939 ) ) ;
#37766=CARTESIAN_POINT ( 'NONE',  ( -15.22947800210000047, 1422.122175526829778, 227.7536867804980147 ) ) ;
#37767=CARTESIAN_POINT ( 'NONE',  ( 11.86716023049999968, 1432.353341358199941, 147.6509521729980179 ) ) ;
#37769=CARTESIAN_POINT ( 'NONE',  ( 1.804213693440000155, 1410.351307743929965, 232.1928990402979878 ) ) ;
#37773=CARTESIAN_POINT ( 'NONE',  ( 10.62480271660000142, 1425.043747535729835, 132.2061233091980057 ) ) ;
#37782=CARTESIAN_POINT ( 'NONE',  ( 1.716045945209999868, 1509.007693206030126, 179.5167849949980052 ) ) ;
#37785=ADVANCED_FACE ( 'NONE', ( #3642 ), #108067, .T. ) ;
#37788=ORIENTED_EDGE ( 'NONE', *, *, #67787, .F. ) ;
#37790=CARTESIAN_POINT ( 'NONE',  ( -7.738809642880000617, 1396.243216920830037, 200.0727852474580004 ) ) ;
#37791=CARTESIAN_POINT ( 'NONE',  ( -4.163739766079999960, 1409.058461383930080, 188.2538941213980195 ) ) ;
#37792=CARTESIAN_POINT ( 'NONE',  ( 12.54268436849999979, 1408.913060387329779, 223.0428732173979824 ) ) ;
#37795=CARTESIAN_POINT ( 'NONE',  ( -1.365172581131870011, 1416.963969358779877, 185.3230370589230063 ) ) ;
#37796=CARTESIAN_POINT ( 'NONE',  ( 1.914833391339999968, 1429.772458808630063, 184.5724300327979961 ) ) ;
#37797=CARTESIAN_POINT ( 'NONE',  ( -41.12450279298050049, 1446.742067430790030, 135.7069966715910141 ) ) ;
#37798=B_SPLINE_CURVE_WITH_KNOTS ( 'NONE', 5,
 ( #47735, #75695, #6272, #14107, #81869, #15200 ),
 .UNSPECIFIED., .F., .F.,
 ( 6, 6 ),
 ( -1.510872622183800029, -4.733984335647534181E-07 ),
 .UNSPECIFIED. ) ;
#37799=CARTESIAN_POINT ( 'NONE',  ( -2.500000000000079936, 1448.853500281970128, 156.0591697921909997 ) ) ;
#37800=CARTESIAN_POINT ( 'NONE',  ( 29.16088018400000337, 1435.515811254470009, 135.2139231482979937 ) ) ;
#37801=CARTESIAN_POINT ( 'NONE',  ( 0.9044596846589999517, 1416.819756528429934, 190.2149403000979930 ) ) ;
#37802=CARTESIAN_POINT ( 'NONE',  ( -3.816632885168049771, 1406.173185440710085, 269.0404319194170171 ) ) ;
#37803=CARTESIAN_POINT ( 'NONE',  ( 40.27186280670000684, 1443.842024488900051, 137.1351532911979803 ) ) ;
#37806=CARTESIAN_POINT ( 'NONE',  ( 12.71388170200000189, 1442.799400843799958, 186.7083504157980087 ) ) ;
#37807=ORIENTED_EDGE ( 'NONE', *, *, #54309, .T. ) ;
#37808=ORIENTED_EDGE ( 'NONE', *, *, #6645, .T. ) ;
#37810=CARTESIAN_POINT ( 'NONE',  ( -15.46700374319999938, 1461.188231601529878, 228.6959067671980108 ) ) ;
#37815=VERTEX_POINT ( 'NONE', #48941 ) ;
#37816=CARTESIAN_POINT ( 'NONE',  ( -2.953089928408080045, 1509.083816246680044, 179.3119815030040058 ) ) ;
#37820=CARTESIAN_POINT ( 'NONE',  ( 2.763736212470000009, 1415.425644477229980, 226.3988609140980088 ) ) ;
#37824=CARTESIAN_POINT ( 'NONE',  ( -3.576202738689999716, 1409.205377980830008, 231.7680162657979963 ) ) ;
#37825=CARTESIAN_POINT ( 'NONE',  ( -3.679272716979999913, 1453.313060387329870, 189.6495746351980074 ) ) ;
#37826=ORIENTED_EDGE ( 'NONE', *, *, #97509, .T. ) ;
#37827=CARTESIAN_POINT ( 'NONE',  ( -14.11276137784757978, 1435.081324051009688, 149.0356280077207032 ) ) ;
#37828=CARTESIAN_POINT ( 'NONE',  ( -26.54480924795199925, 1440.913060445639985, 224.6644947001300068 ) ) ;
#37830=DIRECTION ( 'NONE',  ( 0.000000000000000000, 0.000000000000000000, 1.000000000000000000 ) ) ;
#37831=EDGE_CURVE ( 'NONE', #23724, #3072, #54798, .T. ) ;
#37833=CARTESIAN_POINT ( 'NONE',  ( 41.55348321080259666, 1432.499391167679960, 270.0571128646830061 ) ) ;
#37836=CARTESIAN_POINT ( 'NONE',  ( 23.29389168950000411, 1409.986405036029964, 208.3140838675509769 ) ) ;
#37839=CARTESIAN_POINT ( 'NONE',  ( 20.72660872792978282, 1410.996521324362220, 199.1611606857948686 ) ) ;
#37841=EDGE_LOOP ( 'NONE', ( #1207, #637, #70066, #73191 ) ) ;
#37842=CARTESIAN_POINT ( 'NONE',  ( -4.291175242752039765, 1446.971469842819943, 154.7965863647420122 ) ) ;
#37843=CARTESIAN_POINT ( 'NONE',  ( -6.008305668000000210, 1417.906421182329950, 231.8399811658979957 ) ) ;
#37850=CARTESIAN_POINT ( 'NONE',  ( -7.105427357599999217E-15, 1432.413060387330006, 146.1721969590979882 ) ) ;
#37853=CARTESIAN_POINT ( 'NONE',  ( -0.1796713856869999737, 1410.302588876229947, 233.2312010261979935 ) ) ;
#37854=CARTESIAN_POINT ( 'NONE',  ( 0.1601811252895079807, 1420.470269613179880, 182.7389971891749951 ) ) ;
#37857=CARTESIAN_POINT ( 'NONE',  ( 19.56461708790000031, 1509.492094473429916, 187.5226862208980094 ) ) ;
#37864=CARTESIAN_POINT ( 'NONE',  ( 10.37096375755954192, 1396.275222422115121, 201.1218459616979999 ) ) ;
#37866=CARTESIAN_POINT ( 'NONE',  ( 10.68507717228444243, 1434.716557689225283, 152.0058149931969353 ) ) ;
#37868=PRODUCT_DEFINITION_CONTEXT ( 'detailed design', #64909, 'design' ) ;
#37870=CARTESIAN_POINT ( 'NONE',  ( 16.81342751137891511, 1421.939823536384210, 226.9481537518386176 ) ) ;
#37871=CARTESIAN_POINT ( 'NONE',  ( 6.313072733930000346, 1422.316561012229840, 186.3238498068980107 ) ) ;
#37872=CARTESIAN_POINT ( 'NONE',  ( -18.15573960440000434, 1424.737936287830053, 225.8718214486980003 ) ) ;
#37875=CARTESIAN_POINT ( 'NONE',  ( -7.320561577120000329, 1432.353341358199941, 149.5448088695980005 ) ) ;
#37876=CARTESIAN_POINT ( 'NONE',  ( 18.34036076829999828, 1488.313847894929722, 189.1254428722979810 ) ) ;
#37878=CARTESIAN_POINT ( 'NONE',  ( -16.64494502007340770, 1432.422161184578044, 218.5249863156588219 ) ) ;
#37880=ORIENTED_EDGE ( 'NONE', *, *, #61044, .F. ) ;
#37883=CARTESIAN_POINT ( 'NONE',  ( 11.76640019110000068, 1437.123680669209989, 147.7210023317979903 ) ) ;
#37885=CARTESIAN_POINT ( 'NONE',  ( -24.52306583130000206, 1436.926870631639986, 210.6343607071179918 ) ) ;
#37888=CARTESIAN_POINT ( 'NONE',  ( -2.986444372602363728, 1425.988535542772979, 185.4516627005385772 ) ) ;
#37889=CARTESIAN_POINT ( 'NONE',  ( 12.44994833213096008, 1435.748311113976797, 150.9813188435746270 ) ) ;
#37890=CARTESIAN_POINT ( 'NONE',  ( -17.11050544143609997, 1414.913527275050001, 207.5943401297909929 ) ) ;
#37899=CARTESIAN_POINT ( 'NONE',  ( 21.02378441960000188, 1508.374119905930002, 190.5095349432980072 ) ) ;
#37907=CARTESIAN_POINT ( 'NONE',  ( 12.90411285433943611, 1442.893553763067530, 169.4358074260771332 ) ) ;
#37908=CARTESIAN_POINT ( 'NONE',  ( 31.13322700354939343, 1420.444298374236496, 269.4832979485171904 ) ) ;
#37909=CARTESIAN_POINT ( 'NONE',  ( -25.42953938249999979, 1453.762068279829919, 238.1443916851980305 ) ) ;
#37910=CARTESIAN_POINT ( 'NONE',  ( -19.98650548909999713, 1487.993256480629952, 190.6491142766980147 ) ) ;
#37911=CARTESIAN_POINT ( 'NONE',  ( -11.92631326350000087, 1433.455531743929896, 150.1111345919979954 ) ) ;
#37912=TOROIDAL_SURFACE ( 'NONE', #30540, 24.00000000000000000, 1.000000000000000000 ) ;
#37913=CARTESIAN_POINT ( 'NONE',  ( 27.48210477259999962, 1509.872756633229983, 199.3218240744180036 ) ) ;
#37914=CARTESIAN_POINT ( 'NONE',  ( -19.20165183970000200, 1486.139761766429956, 189.5810907390980162 ) ) ;
#37917=CARTESIAN_POINT ( 'NONE',  ( 4.540052872590000455, 1421.340300729830005, 185.5158982254980060 ) ) ;
#37918=CARTESIAN_POINT ( 'NONE',  ( -24.40996130410000120, 1440.626642977380016, 212.0145020556379905 ) ) ;
#37923=CARTESIAN_POINT ( 'NONE',  ( 1.895454726076929561E-09, 1410.564254227580022, 257.2398119582219920 ) ) ;
#37925=ORIENTED_EDGE ( 'NONE', *, *, #12860, .T. ) ;
#37926=CARTESIAN_POINT ( 'NONE',  ( -11.85748657036189968, 1431.735414931930109, 149.9492757270899972 ) ) ;
#37928=CARTESIAN_POINT ( 'NONE',  ( -8.322172262500000528, 1473.608514543630008, 270.1222559170979594 ) ) ;
#37929=CARTESIAN_POINT ( 'NONE',  ( -23.86106795586941942, 1435.967792748258717, 211.4074662604529067 ) ) ;
#37931=CARTESIAN_POINT ( 'NONE',  ( -15.05666906759999968, 1495.930445535429953, 224.5094625774979988 ) ) ;
#37934=CARTESIAN_POINT ( 'NONE',  ( 0.2099472870183970163, 1452.743325152459875, 183.2501930988930212 ) ) ;
#37935=CARTESIAN_POINT ( 'NONE',  ( -13.37979245520000049, 1421.464012522729945, 229.5728339053979994 ) ) ;
#37939=CARTESIAN_POINT ( 'NONE',  ( -44.41403626570249941, 1432.254696578300127, 268.8004549980919933 ) ) ;
#37940=ORIENTED_EDGE ( 'NONE', *, *, #39428, .T. ) ;
#37941=CARTESIAN_POINT ( 'NONE',  ( -3.536775676796930501, 1494.955962957219981, 181.4953438780639772 ) ) ;
#37942=EDGE_LOOP ( 'NONE', ( #43692, #65750, #38346, #65202, #107720, #19301 ) ) ;
#37943=ORIENTED_EDGE ( 'NONE', *, *, #88228, .T. ) ;
#37946=CARTESIAN_POINT ( 'NONE',  ( 17.05103420828933380, 1409.778319746613079, 224.8086557538146906 ) ) ;
#37947=CARTESIAN_POINT ( 'NONE',  ( -2.665104874070000296, 1425.412186680530112, 185.9059251853979902 ) ) ;
#37949=CARTESIAN_POINT ( 'NONE',  ( -27.02656364750020401, 1451.901091008129924, 135.4178927912169854 ) ) ;
#37953=DIRECTION ( 'NONE',  ( -0.3363363969988524271, -0.9417419115945887542, 0.000000000000000000 ) ) ;
#37955=ORIENTED_EDGE ( 'NONE', *, *, #26212, .F. ) ;
#37956=CARTESIAN_POINT ( 'NONE',  ( -9.584254063140670965, 1410.554478348119801, 270.0755687917119872 ) ) ;
#37957=CARTESIAN_POINT ( 'NONE',  ( -2.286265947080000416, 1427.727383903629971, 112.4493539157979995 ) ) ;
#37960=ORIENTED_EDGE ( 'NONE', *, *, #69222, .T. ) ;
#37962=CARTESIAN_POINT ( 'NONE',  ( 44.74112653917228499, 1447.656416290266407, 268.9998424599907025 ) ) ;
#37964=CARTESIAN_POINT ( 'NONE',  ( -14.22053218827930188, 1436.255562567059997, 150.1050894581620128 ) ) ;
#37965=CARTESIAN_POINT ( 'NONE',  ( -0.3255694447470000030, 1486.004385721930021, 181.7846486939979798 ) ) ;
#37966=CARTESIAN_POINT ( 'NONE',  ( -21.76163504101332080, 1506.366982243313487, 212.1069626703776407 ) ) ;
#37967=CARTESIAN_POINT ( 'NONE',  ( 5.391625819569999756, 1433.099291512059835, 154.6242831037980068 ) ) ;
#37968=CARTESIAN_POINT ( 'NONE',  ( 15.86141264426099973, 1474.310288337290103, 267.4439829464420200 ) ) ;
#37969=CARTESIAN_POINT ( 'NONE',  ( 11.20854081390000090, 1414.996444526030018, 222.5314265605980211 ) ) ;
#37970=CARTESIAN_POINT ( 'NONE',  ( 7.678837752449999776, 1445.740092221990153, 183.5513996952979880 ) ) ;
#37973=CARTESIAN_POINT ( 'NONE',  ( -38.81202641437909762, 1436.797832205920031, 135.3761633872119887 ) ) ;
#37974=CARTESIAN_POINT ( 'NONE',  ( -21.36341525586438550, 1454.134263472093608, 222.4395773065823789 ) ) ;
#37978=CARTESIAN_POINT ( 'NONE',  ( 25.28734891721619960, 1450.982973813519720, 137.4270881049000081 ) ) ;
#37981=CARTESIAN_POINT ( 'NONE',  ( 18.47322038440000114, 1409.558159458129921, 197.4202168127980030 ) ) ;
#37982=CARTESIAN_POINT ( 'NONE',  ( 22.91694143579999832, 1410.643289488730034, 207.1553313229279922 ) ) ;
#37983=CARTESIAN_POINT ( 'NONE',  ( -26.56555459097119964, 1481.927937259539931, 210.5566609482799834 ) ) ;
#37985=CARTESIAN_POINT ( 'NONE',  ( 0.6813382182996269298, 1451.459142117649890, 182.8216330104679912 ) ) ;
#37986=B_SPLINE_CURVE_WITH_KNOTS ( 'NONE', 3,
 ( #40336, #56051, #5650, #91295, #62990, #90178 ),
 .UNSPECIFIED., .F., .F.,
 ( 4, 2, 4 ),
 ( 0.000000000000000000, 0.5000395032561160136, 1.000267919028009933 ),
 .UNSPECIFIED. ) ;
#37992=DIRECTION ( 'NONE',  ( 0.03084238745359989264, -0.9990097612528838766, 0.03206624483187858754 ) ) ;
#37993=CARTESIAN_POINT ( 'NONE',  ( 2.500000000000000000, 1439.114301455650093, 157.7261946041980138 ) ) ;
#37994=CARTESIAN_POINT ( 'NONE',  ( -9.236170142511459957, 1423.625851892860055, 144.1551608696729829 ) ) ;
#37995=CARTESIAN_POINT ( 'NONE',  ( -36.08318819676349420, 1449.986793179470169, 136.2470111316459906 ) ) ;
#37996=CARTESIAN_POINT ( 'NONE',  ( 10.85733419331820393, 1424.789793182321318, 138.1870230799576404 ) ) ;
#37998=CARTESIAN_POINT ( 'NONE',  ( -2.898404794048390354, 1484.263598554799955, 183.3162688752209704 ) ) ;
#38002=CARTESIAN_POINT ( 'NONE',  ( 25.01304800111659787, 1440.913060398049993, 216.1348349641639857 ) ) ;
#38008=EDGE_CURVE ( 'NONE', #28026, #22756, #66109, .T. ) ;
#38013=ADVANCED_FACE ( 'NONE', ( #7740 ), #39208, .T. ) ;
#38015=CARTESIAN_POINT ( 'NONE',  ( -12.04996996890000105, 1508.335006800029987, 233.7287155051980108 ) ) ;
#38018=CARTESIAN_POINT ( 'NONE',  ( 5.372875771976799442, 1422.387436188309948, 137.8049185903410319 ) ) ;
#38020=CARTESIAN_POINT ( 'NONE',  ( 1.551201541590000232, 1466.314669792330051, 234.8893240182980264 ) ) ;
#38023=CARTESIAN_POINT ( 'NONE',  ( -1.019439684479999997, 1451.327316323330024, 183.0760546737980121 ) ) ;
#38026=CARTESIAN_POINT ( 'NONE',  ( -16.63478241967279914, 1414.913060387399810, 207.7445871609179733 ) ) ;
#38029=EDGE_LOOP ( 'NONE', ( #101276, #2727, #7516, #50935 ) ) ;
#38031=DIRECTION ( 'NONE',  ( 0.8495773475194792201, -0.1203693149516160271, 0.5135460627829260272 ) ) ;
#38033=CARTESIAN_POINT ( 'NONE',  ( -11.60004869885202972, 1426.698742266320096, 134.5125406510034338 ) ) ;
#38035=CARTESIAN_POINT ( 'NONE',  ( 21.21789656210188468, 1509.702941487444605, 188.2403193419460479 ) ) ;
#38036=CARTESIAN_POINT ( 'NONE',  ( 14.91913257496040046, 1409.434047977000091, 208.5473241550759838 ) ) ;
#38039=EDGE_CURVE ( 'NONE', #39681, #42334, #99971, .T. ) ;
#38040=CARTESIAN_POINT ( 'NONE',  ( -18.23663199019999936, 1440.788381478219890, 191.4112727536980003 ) ) ;
#38043=EDGE_LOOP ( 'NONE', ( #22182, #18120, #81674, #50813 ) ) ;
#38044=VERTEX_POINT ( 'NONE', #101784 ) ;
#38045=B_SPLINE_CURVE_WITH_KNOTS ( 'NONE', 3,
 ( #58231, #34113, #68303, #94015, #17279, #31907, #100222, #23502, #15088, #49281, #6705, #40860, #92355, #15627, #10578, #61551, #35218, #2205, #69404, #9467, #69960, #1640, #70516, #62110, #77240, #104631, #35778, #43632, #27369, #1092, #77782, #95684, #87853, #53716, #2753, #36873, #102953, #104074, #53145, #52593, #88385, #71067, #78328, #27928, #62674, #18950, #96234, #87283, #103515, #86727, #54259, #43080, #26254, #10018, #44749, #17835, #68851, #26819, #86174, #94560, #61006, #11142, #105189, #541, #95132, #45302, #34665, #52038, #36319 ),
 .UNSPECIFIED., .F., .F.,
 ( 4, 2, 2, 2, 2, 2, 1, 1, 2, 2, 2, 2, 1, 1, 2, 2, 2, 2, 1, 1, 2, 2, 2, 1, 2, 2, 2, 1, 1, 1, 2, 2, 2, 2, 1, 1, 1, 1, 1, 2, 2, 4 ),
 ( 0.000000000000000000, 0.03124999999976661724, 0.04687499999965134140, 0.06249999999953606555, 0.07812499999942078277, 0.08593749999936303730, 0.08984374999934520434, 0.09179687499932684402, 0.09277343749930819228, 0.09374999999928952665, 0.1093749999990587252, 0.1171874999989445804, 0.1210937499988954391, 0.1230468749988719857, 0.1240234374988613553, 0.1249999999988507110, 0.1562499999987173038, 0.1718749999986504684, 0.1796874999986185217, 0.1835937499986117216, 0.1855468749986193822, 0.1874999999986270149, 0.2187499999986969867, 0.2343749999987318755, 0.2421874999987381205, 0.2499999999987443378, 0.3749999999989568900, 0.4374999999990732968, 0.4687499999991417421, 0.4843749999991775468, 0.4921874999991939781, 0.4999999999992104094, 0.6249999999994299005, 0.6874999999995489164, 0.7187499999996067590, 0.7343749999996357358, 0.7421874999996502797, 0.7460937499996576072, 0.7480468749996712630, 0.7490234374996782574, 0.7499999999996851408, 1.000000000000000000 ),
 .UNSPECIFIED. ) ;
#38048=CARTESIAN_POINT ( 'NONE',  ( -11.26466626661590098, 1415.020374543960088, 195.6559317589140221 ) ) ;
#38049=CARTESIAN_POINT ( 'NONE',  ( -11.93818408299999945, 1433.480074519959999, 149.8972116839979947 ) ) ;
#38050=CARTESIAN_POINT ( 'NONE',  ( 3.111006074948589777E-10, 1465.532046810729980, 239.7303713660589892 ) ) ;
#38051=CARTESIAN_POINT ( 'NONE',  ( -20.16694168119990138, 1493.837731802399958, 190.7961038711720221 ) ) ;
#38052=CARTESIAN_POINT ( 'NONE',  ( 2.546717553650000188, 1397.067799814130012, 221.7839619645980065 ) ) ;
#38054=CARTESIAN_POINT ( 'NONE',  ( -18.97219799319119815, 1486.246528605739741, 189.3000344508529906 ) ) ;
#38058=CARTESIAN_POINT ( 'NONE',  ( -13.62986346476509958, 1435.068496676610039, 149.3976263793470025 ) ) ;
#38060=CARTESIAN_POINT ( 'NONE',  ( 0.9044594075830000302, 1416.819760216229952, 190.2149401804979902 ) ) ;
#38063=B_SPLINE_CURVE_WITH_KNOTS ( 'NONE', 5,
 ( #7833, #78362, #42002, #110298, #85636, #59374 ),
 .UNSPECIFIED., .F., .F.,
 ( 6, 6 ),
 ( 0.000000000000000000, 11.48858425020000240 ),
 .UNSPECIFIED. ) ;
#38064=ORIENTED_EDGE ( 'NONE', *, *, #39759, .F. ) ;
#38065=CARTESIAN_POINT ( 'NONE',  ( 29.79081509879999601, 1435.029579668840142, 240.1465591088980034 ) ) ;
#38066=CARTESIAN_POINT ( 'NONE',  ( -25.27895407679999806, 1469.239702726530140, 203.5787248714279940 ) ) ;
#38067=CARTESIAN_POINT ( 'NONE',  ( -2.550919205790000088, 1504.648467973429888, 180.9569263682979852 ) ) ;
#38068=CARTESIAN_POINT ( 'NONE',  ( 2.509110313610579488E-14, 1423.297483101070156, 232.1344543676479759 ) ) ;
#38070=CARTESIAN_POINT ( 'NONE',  ( -15.47923624559999922, 1416.261629426230002, 248.5133305101979886 ) ) ;
#38072=CARTESIAN_POINT ( 'NONE',  ( 0.8426039787746957277, 1415.538311208945288, 233.2356076681966783 ) ) ;
#38073=FACE_OUTER_BOUND ( 'NONE', #88113, .T. ) ;
#38074=EDGE_LOOP ( 'NONE', ( #74038, #1132, #65431 ) ) ;
#38075=CARTESIAN_POINT ( 'NONE',  ( -2.500000000000000000, 1432.112068525799941, 157.4891847571979895 ) ) ;
#38077=DIRECTION ( 'NONE',  ( 0.1838871638018280408, 0.9727212700611359564, -0.1414172611797089030 ) ) ;
#38081=CARTESIAN_POINT ( 'NONE',  ( -23.71385237390180123, 1410.153949763399851, 208.7056816592929920 ) ) ;
#38086=CARTESIAN_POINT ( 'NONE',  ( -0.4938443966799999640, 1470.488522285229919, 235.7260322168980053 ) ) ;
#38088=VERTEX_POINT ( 'NONE', #59277 ) ;
#38089=CARTESIAN_POINT ( 'NONE',  ( 11.43729524049999924, 1425.481262536329950, 144.1593964291980114 ) ) ;
#38090=CARTESIAN_POINT ( 'NONE',  ( -13.01671764799590036, 1416.842625005220043, 221.9093393807470136 ) ) ;
#38091=CARTESIAN_POINT ( 'NONE',  ( 13.40854346959999965, 1452.823344015929933, 224.6980477592980208 ) ) ;
#38095=CARTESIAN_POINT ( 'NONE',  ( 13.51730467772499722, 1443.864691789369090, 188.0480164084754904 ) ) ;
#38100=CARTESIAN_POINT ( 'NONE',  ( 12.71039585379999970, 1507.471771701229954, 233.3404624238980034 ) ) ;
#38102=CARTESIAN_POINT ( 'NONE',  ( 14.55389011864330051, 1452.404827345299964, 148.1692795786860017 ) ) ;
#38105=DIRECTION ( 'NONE',  ( 0.000000000000000000, 0.000000000000000000, -1.000000000000000000 ) ) ;
#38107=CARTESIAN_POINT ( 'NONE',  ( 0.03486440002950671330, 1409.388410587884891, 232.8483323310555591 ) ) ;
#38109=DIRECTION ( 'NONE',  ( -0.000000000000000000, -0.000000000000000000, 1.000000000000000000 ) ) ;
#38111=CARTESIAN_POINT ( 'NONE',  ( -24.30503083389229602, 1508.888284146479918, 222.4513817739089916 ) ) ;
#38114=CARTESIAN_POINT ( 'NONE',  ( 7.553102826339999964, 1423.481562109630204, 234.3916895958979865 ) ) ;
#38118=CARTESIAN_POINT ( 'NONE',  ( 43.03456162790020301, 1428.697681977020011, 269.7258210693699993 ) ) ;
#38123=CARTESIAN_POINT ( 'NONE',  ( -1.074557793710971598, 1450.811636816389637, 154.2492438910815622 ) ) ;
#38128=CARTESIAN_POINT ( 'NONE',  ( 18.75982378228949798, 1509.568167869620083, 185.1556198730530127 ) ) ;
#38130=CARTESIAN_POINT ( 'NONE',  ( 12.01847341019976589, 1433.726575741404076, 149.8323943637946059 ) ) ;
#38131=CARTESIAN_POINT ( 'NONE',  ( 15.32255284400000050, 1419.766531890930082, 227.7483529289979742 ) ) ;
#38134=CARTESIAN_POINT ( 'NONE',  ( 41.00899597450000300, 1425.451880489129962, 269.1035016206980117 ) ) ;
#38135=CARTESIAN_POINT ( 'NONE',  ( -18.21389191229999938, 1409.549103508730013, 222.3583561910980109 ) ) ;
#38136=CARTESIAN_POINT ( 'NONE',  ( 19.62004841539999944, 1435.182524171729938, 143.5804541147979876 ) ) ;
#38137=CARTESIAN_POINT ( 'NONE',  ( 25.45525579099999902, 1488.577326412729917, 202.6760865476379934 ) ) ;
#38138=CARTESIAN_POINT ( 'NONE',  ( 24.57285633690000282, 1439.622216053659940, 213.1838506830980009 ) ) ;
#38139=ADVANCED_FACE ( 'NONE', ( #15565 ), #66106, .F. ) ;
#38140=CARTESIAN_POINT ( 'NONE',  ( -0.3382973561789999750, 1475.836249162829972, 266.9611136385980217 ) ) ;
#38142=CARTESIAN_POINT ( 'NONE',  ( -39.20985834264440228, 1439.158936599190156, 136.6284022834660163 ) ) ;
#38143=CARTESIAN_POINT ( 'NONE',  ( 0.2084417785648140231, 1458.224878346390142, 183.0292437909860155 ) ) ;
#38144=CARTESIAN_POINT ( 'NONE',  ( -13.84827599230330009, 1408.877987748370060, 207.9041386013730346 ) ) ;
#38148=ADVANCED_FACE ( 'NONE', ( #70323 ), #43437, .F. ) ;
#38149=CARTESIAN_POINT ( 'NONE',  ( -27.78647954532239694, 1508.087771980839989, 210.4724892245600074 ) ) ;
#38150=CARTESIAN_POINT ( 'NONE',  ( -4.291175242752039765, 1446.971469842819943, 154.7965863647420122 ) ) ;
#38151=CARTESIAN_POINT ( 'NONE',  ( -26.80765817130000173, 1436.328495614390022, 136.7303568460980046 ) ) ;
#38152=CARTESIAN_POINT ( 'NONE',  ( 2.871913733999305940, 1466.359209332784530, 234.1530941677849569 ) ) ;
#38155=FACE_OUTER_BOUND ( 'NONE', #39321, .T. ) ;
#38158=CARTESIAN_POINT ( 'NONE',  ( 15.41405264505409889, 1509.425107283729858, 233.4982122163600309 ) ) ;
#38159=CARTESIAN_POINT ( 'NONE',  ( -29.78098341020000106, 1466.870135787829895, 269.3614920601979748 ) ) ;
#38160=CARTESIAN_POINT ( 'NONE',  ( -16.72308823676789657, 1489.783577386040179, 223.6951472220740129 ) ) ;
#38161=CARTESIAN_POINT ( 'NONE',  ( 18.64672481370000057, 1416.851343898729965, 209.6839434896789669 ) ) ;
#38162=CARTESIAN_POINT ( 'NONE',  ( -27.13474158619999699, 1509.190014537030038, 212.0481536874080177 ) ) ;
#38166=CARTESIAN_POINT ( 'NONE',  ( 20.59686811859999978, 1507.763399985229853, 227.6863920494979823 ) ) ;
#38167=CARTESIAN_POINT ( 'NONE',  ( -29.68037260229820262, 1509.976800595009991, 208.5710708581900121 ) ) ;
#38169=CARTESIAN_POINT ( 'NONE',  ( 0.5019399832390400995, 1413.804834606910163, 184.9224728268669935 ) ) ;
#38170=VERTEX_POINT ( 'NONE', #78687 ) ;
#38171=CARTESIAN_POINT ( 'NONE',  ( -12.37364323390000109, 1509.415518769829987, 181.8814867841980174 ) ) ;
#38173=EDGE_CURVE ( 'NONE', #98691, #2271, #54716, .T. ) ;
#38175=CARTESIAN_POINT ( 'NONE',  ( -12.15086845379999936, 1416.067629296030191, 194.7798609157979968 ) ) ;
#38177=CARTESIAN_POINT ( 'NONE',  ( 22.07912570460000268, 1409.684080446629878, 211.6989830675280189 ) ) ;
#38180=CARTESIAN_POINT ( 'NONE',  ( -15.81258200789999790, 1421.897701213729988, 227.3576972447979756 ) ) ;
#38181=CARTESIAN_POINT ( 'NONE',  ( -11.30563979010000075, 1432.585777830499865, 151.5215853277979932 ) ) ;
#38186=CARTESIAN_POINT ( 'NONE',  ( -1.435685682569999955, 1417.080663547029872, 233.9312154598979987 ) ) ;
#38189=CARTESIAN_POINT ( 'NONE',  ( -18.38030196201400202, 1485.844866795689995, 189.0206862885210057 ) ) ;
#38196=CARTESIAN_POINT ( 'NONE',  ( 28.07231212390000152, 1508.101920094730076, 210.4687657402579930 ) ) ;
#38197=ORIENTED_EDGE ( 'NONE', *, *, #38357, .T. ) ;
#38199=DIRECTION ( 'NONE',  ( -0.7122454525621805255, 0.000000000000000000, -0.7019304917899598095 ) ) ;
#38200=CARTESIAN_POINT ( 'NONE',  ( 15.96313815125649782, 1420.408442670840031, 191.2218829645730125 ) ) ;
#38201=CARTESIAN_POINT ( 'NONE',  ( 20.34226454299999887, 1454.597587043530211, 225.1509561457980340 ) ) ;
#38202=DIRECTION ( 'NONE',  ( 0.000000000000000000, 0.000000000000000000, 1.000000000000000000 ) ) ;
#38203=CARTESIAN_POINT ( 'NONE',  ( -25.12509679820039921, 1451.311955931910006, 137.4238367825970215 ) ) ;
#38204=CARTESIAN_POINT ( 'NONE',  ( 12.84239221398829933, 1435.935692713660046, 150.8114773724069835 ) ) ;
#38205=CARTESIAN_POINT ( 'NONE',  ( 5.852848188970000365, 1410.053989038129885, 231.0988934593979991 ) ) ;
#38207=( NAMED_UNIT ( * ) SI_UNIT ( $, .STERADIAN. ) SOLID_ANGLE_UNIT ( ) );
#38208=CARTESIAN_POINT ( 'NONE',  ( 40.27155789680160325, 1448.225093240230080, 134.0999999982899737 ) ) ;
#38210=ORIENTED_EDGE ( 'NONE', *, *, #40056, .F. ) ;
#38212=CARTESIAN_POINT ( 'NONE',  ( -15.68560764121220252, 1410.853875961199947, 226.7268370761429992 ) ) ;
#38214=ORIENTED_EDGE ( 'NONE', *, *, #17330, .F. ) ;
#38216=AXIS2_PLACEMENT_3D ( 'NONE', #15725, #39867, #98665 ) ;
#38217=CARTESIAN_POINT ( 'NONE',  ( 9.847354017823224837, 1410.631711604590237, 229.8729602667554559 ) ) ;
#38218=CARTESIAN_POINT ( 'NONE',  ( 0.000000000000000000, 1402.754281879943164, 135.5999999980979851 ) ) ;
#38219=CARTESIAN_POINT ( 'NONE',  ( 3.388329910033260006, 1451.546035976184839, 153.9285079010525124 ) ) ;
#38221=CARTESIAN_POINT ( 'NONE',  ( -17.50616331224802735, 1448.242994606246612, 218.0980532679095063 ) ) ;
#38225=CARTESIAN_POINT ( 'NONE',  ( 1.546874264509999986, 1416.828040557830036, 190.2227689706980129 ) ) ;
#38229=ORIENTED_EDGE ( 'NONE', *, *, #15751, .T. ) ;
#38230=CARTESIAN_POINT ( 'NONE',  ( 25.94212426325589860, 1440.913060387330006, 242.0455472739620006 ) ) ;
#38231=FACE_OUTER_BOUND ( 'NONE', #23340, .T. ) ;
#38232=ORIENTED_EDGE ( 'NONE', *, *, #3811, .F. ) ;
#38234=CARTESIAN_POINT ( 'NONE',  ( -16.14044004459999826, 1410.408804127830081, 191.4391529896979876 ) ) ;
#38236=CARTESIAN_POINT ( 'NONE',  ( -24.39250185919999936, 1440.969627941150065, 211.3361222571480198 ) ) ;
#38239=AXIS2_PLACEMENT_3D ( 'NONE', #71161, #72795, #38077 ) ;
#38240=CARTESIAN_POINT ( 'NONE',  ( 13.46831950203149830, 1436.161406562190223, 150.5249638017590144 ) ) ;
#38241=CARTESIAN_POINT ( 'NONE',  ( 3.757756526780000161, 1406.106055978829772, 266.9554538344980301 ) ) ;
#38244=CARTESIAN_POINT ( 'NONE',  ( 6.226325556679999984, 1465.716049800030078, 233.5720425652980055 ) ) ;
#38245=CARTESIAN_POINT ( 'NONE',  ( 2.121334001142850118E-11, 1407.752913430750141, 267.9039250724300132 ) ) ;
#38249=CARTESIAN_POINT ( 'NONE',  ( 19.18867383189600417, 1443.582650154266503, 213.4775594393471749 ) ) ;
#38252=CARTESIAN_POINT ( 'NONE',  ( -21.39582113410000019, 1488.805759879029893, 208.9522497871160169 ) ) ;
#38259=CARTESIAN_POINT ( 'NONE',  ( -26.09830977477409775, 1509.824433447099864, 222.5363761071970146 ) ) ;
#38260=CARTESIAN_POINT ( 'NONE',  ( -0.4599427841477299883, 1508.922901691350035, 238.6016026774880174 ) ) ;
#38262=CARTESIAN_POINT ( 'NONE',  ( 12.76595157039999862, 1446.243769161290174, 188.3984060521979984 ) ) ;
#38263=CARTESIAN_POINT ( 'NONE',  ( -24.08426305480000451, 1411.115211393229856, 208.6111285346999864 ) ) ;
#38264=CARTESIAN_POINT ( 'NONE',  ( 12.98226713004290112, 1414.913060387349788, 198.3280232619060257 ) ) ;
#38268=CARTESIAN_POINT ( 'NONE',  ( 2.776430554999999689, 1405.810978695030144, 267.5339349680979808 ) ) ;
#38270=B_SPLINE_CURVE_WITH_KNOTS ( 'NONE', 3,
 ( #81780, #96406, #89096, #54970, #71233, #28089, #88562, #19682, #56052, #106451, #106992, #29734, #11846, #63920, #98589, #36493 ),
 .UNSPECIFIED., .F., .F.,
 ( 4, 2, 2, 2, 2, 2, 2, 4 ),
 ( 8.544639080107319913E-08, 0.4101168854422549970, 0.8109689984529260265, 1.212505501424880006, 1.416242740394599853, 1.518121827656090161, 1.569055395889600080, 1.620000854487389841 ),
 .UNSPECIFIED. ) ;
#38272=CARTESIAN_POINT ( 'NONE',  ( 6.690595718171389983, 1474.175196074600080, 270.1377304235489873 ) ) ;
#38275=CARTESIAN_POINT ( 'NONE',  ( 11.60004869885879231, 1423.657548013328096, 137.0691450735224350 ) ) ;
#38278=CARTESIAN_POINT ( 'NONE',  ( -1.636727350584959773, 1450.664746045244556, 183.2094855785913978 ) ) ;
#38279=CARTESIAN_POINT ( 'NONE',  ( 2.431405075025240059, 1449.537433731769852, 154.7921670947710027 ) ) ;
#38280=CARTESIAN_POINT ( 'NONE',  ( -13.69065454899539880, 1415.152886233429854, 220.6114883211280073 ) ) ;
#38283=CARTESIAN_POINT ( 'NONE',  ( -30.40113726520000270, 1433.623945462319853, 255.3819207682979595 ) ) ;
#38285=CARTESIAN_POINT ( 'NONE',  ( 4.269304843480000500, 1441.143128249819938, 158.1185154358979901 ) ) ;
#38286=CARTESIAN_POINT ( 'NONE',  ( -0.2126388994629999918, 1475.048161703429969, 269.6500587019980344 ) ) ;
#38287=CARTESIAN_POINT ( 'NONE',  ( -28.53738135360000072, 1451.916516915729972, 134.8736009463979997 ) ) ;
#38289=CARTESIAN_POINT ( 'NONE',  ( -2.976586033138599596, 1448.268719613186704, 184.4363391144643458 ) ) ;
#38296=CARTESIAN_POINT ( 'NONE',  ( -5.980973321690750133, 1396.121920580289952, 218.4025002956929882 ) ) ;
#38298=CARTESIAN_POINT ( 'NONE',  ( -15.35996473989999878, 1420.804668691529969, 227.0340416244980020 ) ) ;
#38299=CARTESIAN_POINT ( 'NONE',  ( 19.28298846601172301, 1455.999974110760149, 225.1882103107009243 ) ) ;
#38300=ORIENTED_EDGE ( 'NONE', *, *, #3790, .F. ) ;
#38302=CARTESIAN_POINT ( 'NONE',  ( 2.923521583079999875, 1410.394928893030283, 231.6309338985980162 ) ) ;
#38304=CARTESIAN_POINT ( 'NONE',  ( 10.97118381930000020, 1425.274992001930059, 132.2037382631980051 ) ) ;
#38306=CARTESIAN_POINT ( 'NONE',  ( -5426.659192927121694, 54.07981494722833560, 8449.939230966660034 ) ) ;
#38307=B_SPLINE_CURVE_WITH_KNOTS ( 'NONE', 3,
 ( #26007, #855, #9243, #8118, #110041, #60772, #25458, #94896, #18171, #34982, #34436, #52368, #43949, #67509, #17039, #76435, #24364, #84284, #42285, #60204, #110588, #102713, #78092, #94323, #85369, #8664, #1394, #101067, #66958, #59106, #85940, #92678, #15954, #33874, #101612, #50155, #16498, #68065, #42842, #7577 ),
 .UNSPECIFIED., .F., .F.,
 ( 4, 3, 3, 3, 3, 3, 3, 3, 3, 3, 3, 3, 3, 4 ),
 ( -168.5477118249999933, -162.5507363268910126, -153.8407794596359963, -144.7791047296130102, -135.4369637970760039, -125.4361478828139980, -114.7710760797919960, -103.0116084759360007, -88.20793680898479749, -73.11625194994489618, -61.36907839288639366, -50.68835095691321158, -40.67933903265419815, -31.15146013443029460 ),
 .UNSPECIFIED. ) ;
#38308=CARTESIAN_POINT ( 'NONE',  ( -12.45478753333599720, 1442.762691980110048, 151.6226032058479802 ) ) ;
#38309=ADVANCED_FACE ( 'NONE', ( #110628 ), #99106, .T. ) ;
#38313=CARTESIAN_POINT ( 'NONE',  ( 7.327188678030000624, 1507.874256059229992, 182.6136352915980297 ) ) ;
#38318=ORIENTED_EDGE ( 'NONE', *, *, #110279, .T. ) ;
#38319=VERTEX_POINT ( 'NONE', #106093 ) ;
#38320=PLANE ( 'NONE',  #98028 ) ;
#38321=CARTESIAN_POINT ( 'NONE',  ( 2.925327306374799985, 1410.322647625880109, 231.6260571398940158 ) ) ;
#38322=CARTESIAN_POINT ( 'NONE',  ( -1.396725214890000011, 1415.041103191730144, 226.7314491796980178 ) ) ;
#38324=CARTESIAN_POINT ( 'NONE',  ( 0.000000000000000000, 1452.913060387330006, 179.9625354400980086 ) ) ;
#38327=CARTESIAN_POINT ( 'NONE',  ( 17.09102838100000099, 1413.530045447530028, 226.3661571205980181 ) ) ;
#38328=CARTESIAN_POINT ( 'NONE',  ( 2.020974489129999885, 1410.305613295530065, 185.4468934685980059 ) ) ;
#38329=CARTESIAN_POINT ( 'NONE',  ( -41.11424902454939456, 1444.666461503340088, 136.8180534356220051 ) ) ;
#38330=CARTESIAN_POINT ( 'NONE',  ( 40.66801799462539435, 1442.602446576360080, 136.9833458737259946 ) ) ;
#38332=CARTESIAN_POINT ( 'NONE',  ( 33.27874934317770084, 1436.988425504300039, 136.5809431225799813 ) ) ;
#38333=CARTESIAN_POINT ( 'NONE',  ( 11.28006282179999964, 1430.719829126430113, 151.3394816934979872 ) ) ;
#38334=CARTESIAN_POINT ( 'NONE',  ( 41.14066506200000362, 1444.183247956199921, 136.8991343562979921 ) ) ;
#38336=CARTESIAN_POINT ( 'NONE',  ( 4.055275498809999490, 1423.964747713630231, 184.0972450836979988 ) ) ;
#38337=CARTESIAN_POINT ( 'NONE',  ( 11.78238132140000083, 1440.882651473599935, 188.1224434270980055 ) ) ;
#38339=ORIENTED_EDGE ( 'NONE', *, *, #91995, .T. ) ;
#38342=CARTESIAN_POINT ( 'NONE',  ( -13.89782283490000125, 1452.807100928030195, 194.8455099693979662 ) ) ;
#38346=ORIENTED_EDGE ( 'NONE', *, *, #53726, .F. ) ;
#38347=CARTESIAN_POINT ( 'NONE',  ( -14.32724710653639910, 1509.467756537190098, 183.0197988060039904 ) ) ;
#38349=EDGE_CURVE ( 'NONE', #68340, #41530, #88747, .T. ) ;
#38351=CARTESIAN_POINT ( 'NONE',  ( 15.44258166179999847, 1414.913060387329779, 214.5365335479179976 ) ) ;
#38356=CARTESIAN_POINT ( 'NONE',  ( -35.04400506982609187, 1424.099278616513175, 269.5321162145484095 ) ) ;
#38357=EDGE_CURVE ( 'NONE', #109512, #17927, #1073, .T. ) ;
#38358=CARTESIAN_POINT ( 'NONE',  ( -11.16950626350000064, 1409.469289622230008, 228.3240238616979809 ) ) ;
#38361=CARTESIAN_POINT ( 'NONE',  ( 2.500000000000000000, 1419.446092955830181, 146.1320802672979937 ) ) ;
#38362=CARTESIAN_POINT ( 'NONE',  ( -30.52556887503000027, 1440.913060387399810, 239.9851491244249928 ) ) ;
#38366=CARTESIAN_POINT ( 'NONE',  ( 24.89781524799989754, 1415.678878148830108, 269.9191937554660399 ) ) ;
#38371=CARTESIAN_POINT ( 'NONE',  ( 23.16826695290000160, 1409.827445977929756, 208.5989265901500005 ) ) ;
#38372=CARTESIAN_POINT ( 'NONE',  ( -8.113694374351904770, 1425.905879024222713, 225.6960958089561586 ) ) ;
#38376=CARTESIAN_POINT ( 'NONE',  ( 0.2403276022373450060, 1424.313268885149910, 227.5210991795279938 ) ) ;
#38377=CARTESIAN_POINT ( 'NONE',  ( -3.616492858290000001, 1417.910832933829852, 232.6758466721979914 ) ) ;
#38378=EDGE_CURVE ( 'NONE', #79432, #53095, #19854, .T. ) ;
#38383=CARTESIAN_POINT ( 'NONE',  ( 0.7830886349010000025, 1415.510552653030118, 233.2794445565979800 ) ) ;
#38385=CARTESIAN_POINT ( 'NONE',  ( -20.37003372361249731, 1507.842576381340223, 228.6074795959160042 ) ) ;
#38394=ORIENTED_EDGE ( 'NONE', *, *, #94108, .F. ) ;
#38397=VERTEX_POINT ( 'NONE', #63036 ) ;
#38399=AXIS2_PLACEMENT_3D ( 'NONE', #85147, #86808, #52124 ) ;
#38400=CARTESIAN_POINT ( 'NONE',  ( 22.59589508572869931, 1507.700907081449941, 227.3081682119560014 ) ) ;
#38403=CARTESIAN_POINT ( 'NONE',  ( -26.85483190386980112, 1509.266232500709975, 201.3403652348490311 ) ) ;
#38404=CARTESIAN_POINT ( 'NONE',  ( -2.499999987950000335, 1447.625363425740034, 167.4763715217980007 ) ) ;
#38405=CARTESIAN_POINT ( 'NONE',  ( -19.81884662830000110, 1427.029209586630259, 224.1944963751980140 ) ) ;
#38407=CARTESIAN_POINT ( 'NONE',  ( -9.675350337739999418, 1433.447543843880112, 148.7453054530979841 ) ) ;
#38408=CARTESIAN_POINT ( 'NONE',  ( 16.97760447559999974, 1508.233635190930045, 188.0201034282980004 ) ) ;
#38410=CARTESIAN_POINT ( 'NONE',  ( -18.49741831292255512, 1436.683225729171227, 212.7525086259309433 ) ) ;
#38415=CARTESIAN_POINT ( 'NONE',  ( 11.72470770320000000, 1437.821967610810134, 147.7443706334980220 ) ) ;
#38420=CARTESIAN_POINT ( 'NONE',  ( -13.15646098871717129, 1443.074065570369839, 186.7349259480803596 ) ) ;
#38422=CARTESIAN_POINT ( 'NONE',  ( -17.09240173490840320, 1414.913527292460003, 207.6788998298750073 ) ) ;
#38432=ORIENTED_EDGE ( 'NONE', *, *, #82993, .F. ) ;
#38433=EDGE_LOOP ( 'NONE', ( #75544, #105477, #36548, #31265 ) ) ;
#38435=CARTESIAN_POINT ( 'NONE',  ( 13.37406854560000014, 1507.496451373729997, 233.0472692219979933 ) ) ;
#38437=CARTESIAN_POINT ( 'NONE',  ( 30.75249563405095898, 1420.147177030162538, 269.4790404245597983 ) ) ;
#38438=CARTESIAN_POINT ( 'NONE',  ( -36.81312677009999845, 1440.913060384420078, 254.5659337159979998 ) ) ;
#38439=AXIS2_PLACEMENT_3D ( 'NONE', #32447, #17812, #101262 ) ;
#38441=CARTESIAN_POINT ( 'NONE',  ( -11.69527910600000098, 1433.555496640800129, 150.9724154829980023 ) ) ;
#38444=CARTESIAN_POINT ( 'NONE',  ( -19.02744254319999939, 1485.647624488630072, 189.5786657373980120 ) ) ;
#38446=EDGE_CURVE ( 'NONE', #24977, #47969, #49231, .T. ) ;
#38447=CARTESIAN_POINT ( 'NONE',  ( -26.71905419379999813, 1436.374501372160012, 136.7391346277979949 ) ) ;
#38450=CARTESIAN_POINT ( 'NONE',  ( -4.500000000000000000, 1417.575542696430148, 161.0097146498980010 ) ) ;
#38454=CARTESIAN_POINT ( 'NONE',  ( 7.642515834685991225E-10, 1410.900380117609984, 256.4109302437369706 ) ) ;
#38455=ORIENTED_EDGE ( 'NONE', *, *, #72762, .T. ) ;
#38456=ORIENTED_EDGE ( 'NONE', *, *, #2511, .T. ) ;
#38457=CARTESIAN_POINT ( 'NONE',  ( -11.86244099381709916, 1432.080345950339961, 149.9764139188839920 ) ) ;
#38460=CARTESIAN_POINT ( 'NONE',  ( -33.45710699309999825, 1460.809384530529996, 270.1367558008980154 ) ) ;
#38461=CARTESIAN_POINT ( 'NONE',  ( 3.156166260290000025, 1466.544008048530031, 236.1241471695980181 ) ) ;
#38464=EDGE_CURVE ( 'NONE', #85608, #69919, #23810, .T. ) ;
#38465=CARTESIAN_POINT ( 'NONE',  ( 0.2142980244695730230, 1452.886707787869909, 183.2554660003850131 ) ) ;
#38466=CARTESIAN_POINT ( 'NONE',  ( -14.49383156030000031, 1422.099018230730053, 229.4564958546980051 ) ) ;
#38470=CARTESIAN_POINT ( 'NONE',  ( -27.50738397533670110, 1412.571463151949956, 268.1607314479759907 ) ) ;
#38473=ORIENTED_EDGE ( 'NONE', *, *, #105036, .T. ) ;
#38474=ORIENTED_EDGE ( 'NONE', *, *, #59764, .T. ) ;
#38476=CARTESIAN_POINT ( 'NONE',  ( 4.631508481766313245, 1423.709513865996996, 183.8663217726549135 ) ) ;
#38478=CARTESIAN_POINT ( 'NONE',  ( -15.45655017849999879, 1440.435998840410093, 189.5583962537980085 ) ) ;
#38480=ORIENTED_EDGE ( 'NONE', *, *, #71313, .T. ) ;
#38488=CARTESIAN_POINT ( 'NONE',  ( -9.898755429526129745, 1408.724963430380058, 270.2742877825459686 ) ) ;
#38489=CARTESIAN_POINT ( 'NONE',  ( 1.610281973209999908E-15, 1427.674934138829940, 112.4493539157979995 ) ) ;
#38493=ORIENTED_EDGE ( 'NONE', *, *, #62702, .F. ) ;
#38494=CARTESIAN_POINT ( 'NONE',  ( 42.36757903333897701, 1453.626821642604227, 269.0658443221472567 ) ) ;
#38495=EDGE_CURVE ( 'NONE', #43234, #105296, #33259, .T. ) ;
#38497=CARTESIAN_POINT ( 'NONE',  ( -13.39012931902800041, 1436.134316771910107, 150.5611366713399946 ) ) ;
#38498=CARTESIAN_POINT ( 'NONE',  ( -0.03399551901351580141, 1409.332672981930045, 185.4489178702069978 ) ) ;
#38500=ADVANCED_FACE ( 'NONE', ( #109414 ), #92010, .T. ) ;
#38501=CARTESIAN_POINT ( 'NONE',  ( -20.62320340999438528, 1506.569407725107112, 217.0556035612084713 ) ) ;
#38502=CARTESIAN_POINT ( 'NONE',  ( -18.38268101079999894, 1430.797810259230118, 225.7446671720980191 ) ) ;
#38503=CARTESIAN_POINT ( 'NONE',  ( 15.74277789255459936, 1473.851709889820086, 269.2139740697160164 ) ) ;
#38504=CARTESIAN_POINT ( 'NONE',  ( 12.72284891840000043, 1416.311719779230089, 222.6852781584979653 ) ) ;
#38508=CARTESIAN_POINT ( 'NONE',  ( -33.91369111065759512, 1435.681798630919957, 135.0584844183200346 ) ) ;
#38509=CARTESIAN_POINT ( 'NONE',  ( -23.92444880932286111, 1445.948748625923145, 213.1725788544748923 ) ) ;
#38511=CARTESIAN_POINT ( 'NONE',  ( 7.411925917899073291, 1456.536940314574167, 227.5735638817602364 ) ) ;
#38513=CARTESIAN_POINT ( 'NONE',  ( -4.108880503800459216, 1440.120469803585365, 185.4247791707405497 ) ) ;
#38515=CARTESIAN_POINT ( 'NONE',  ( 20.70465513139999914, 1409.636082885830092, 202.1075812846079884 ) ) ;
#38517=CARTESIAN_POINT ( 'NONE',  ( 15.94345642359999715, 1409.469818154030008, 225.2684697977979909 ) ) ;
#38521=CARTESIAN_POINT ( 'NONE',  ( 4.253135465434060514, 1441.316943195099839, 160.6080137006729842 ) ) ;
#38522=CARTESIAN_POINT ( 'NONE',  ( 2.500000000000000000, 1439.604493174409981, 166.9187913666470138 ) ) ;
#38529=CARTESIAN_POINT ( 'NONE',  ( -8.492687501607809608, 1424.222007390339968, 101.6998641355710049 ) ) ;
#38531=CARTESIAN_POINT ( 'NONE',  ( -40.01985023196169777, 1445.652369265400011, 136.8565960713379752 ) ) ;
#38534=CARTESIAN_POINT ( 'NONE',  ( -2.379356867398829678, 1477.797235972689805, 183.4954656640089752 ) ) ;
#38536=CARTESIAN_POINT ( 'NONE',  ( -45.63734462135529668, 1442.192498193280016, 268.9745364237319905 ) ) ;
#38537=B_SPLINE_SURFACE_WITH_KNOTS ( 'NONE', 4, 5, ( 
 ( #39360, #21971, #39913, #56163, #72975, #108212 ),
 ( #47766, #81901, #5207, #74083, #65680, #73534 ),
 ( #82472, #100367, #107670, #5770, #65130, #31500 ),
 ( #99798, #23092, #91425, #74631, #108766, #32059 ),
 ( #49430, #23653, #57835, #91962, #83552, #6845 ) ),
 .UNSPECIFIED., .F., .F., .F.,
 ( 5, 5 ),
 ( 6, 6 ),
 ( 4.842510457999999574, 5.115712977159999397 ),
 ( 0.000000000000000000, 2.000000000000000000 ),
 .UNSPECIFIED. ) ;
#38538=CARTESIAN_POINT ( 'NONE',  ( 28.16386307796540223, 1440.913060387279984, 231.8139636807940178 ) ) ;
#38545=CARTESIAN_POINT ( 'NONE',  ( -11.86716023049999968, 1432.353341358199941, 147.6509521729980179 ) ) ;
#38547=CARTESIAN_POINT ( 'NONE',  ( -17.04970511980000225, 1508.515036612230006, 230.3270150111979717 ) ) ;
#38551=CARTESIAN_POINT ( 'NONE',  ( -15.57748978299999898, 1507.212883763329955, 192.6976421578980023 ) ) ;
#38553=CARTESIAN_POINT ( 'NONE',  ( 1.908739326689999904, 1465.060976646429935, 235.3867066285980059 ) ) ;
#38554=CARTESIAN_POINT ( 'NONE',  ( -41.65674268029999894, 1443.992461967939789, 135.6790812281979868 ) ) ;
#38555=VERTEX_POINT ( 'NONE', #69080 ) ;
#38556=CARTESIAN_POINT ( 'NONE',  ( -1.027621871790000085, 1451.767504252629806, 183.3788275550980131 ) ) ;
#38559=CARTESIAN_POINT ( 'NONE',  ( -18.24633262864339756, 1416.842625005220043, 208.9597599549800009 ) ) ;
#38560=ORIENTED_EDGE ( 'NONE', *, *, #19408, .T. ) ;
#38572=CARTESIAN_POINT ( 'NONE',  ( 18.02574752529999813, 1424.482706161330043, 224.6196056148980063 ) ) ;
#38573=CARTESIAN_POINT ( 'NONE',  ( 1.166167165090000069, 1418.953384179930026, 184.8577940441979877 ) ) ;
#38574=CARTESIAN_POINT ( 'NONE',  ( -18.41452686919999593, 1437.075586301560179, 192.6723155837979959 ) ) ;
#38576=CARTESIAN_POINT ( 'NONE',  ( -2.427038242517200128, 1449.569853069620194, 183.3138490965509959 ) ) ;
#38577=ORIENTED_EDGE ( 'NONE', *, *, #17886, .T. ) ;
#38579=( BOUNDED_CURVE ( )  B_SPLINE_CURVE ( 3, ( #13603, #39937, #23115, #56746 ),
 .UNSPECIFIED., .F., .F. ) 
 B_SPLINE_CURVE_WITH_KNOTS ( ( 4, 4 ),
 ( 1.307301600140529985, 1.688785180142575060 ),
 .UNSPECIFIED. ) 
 CURVE ( )  GEOMETRIC_REPRESENTATION_ITEM ( )  RATIONAL_B_SPLINE_CURVE ( ( 1.000000000000000000, 0.9879092475434242404, 0.9879092475434242404, 1.000000000000000000 ) ) 
 REPRESENTATION_ITEM ( '' )  );
#38581=CARTESIAN_POINT ( 'NONE',  ( -11.34486004996399977, 1415.059973085260026, 195.5756060859239938 ) ) ;
#38582=CARTESIAN_POINT ( 'NONE',  ( -11.97808853149999919, 1435.413056357760070, 151.1931547270979763 ) ) ;
#38584=CARTESIAN_POINT ( 'NONE',  ( -6.119344404807989421E-10, 1468.772255180760112, 250.5908485024660024 ) ) ;
#38587=CARTESIAN_POINT ( 'NONE',  ( -1.793335950739999962, 1419.496365638530051, 185.6406336190979971 ) ) ;
#38588=CARTESIAN_POINT ( 'NONE',  ( -0.1926035411919999885, 1484.826485890729828, 181.8486164389979933 ) ) ;
#38591=ADVANCED_FACE ( 'NONE', ( #79130 ), #90158, .F. ) ;
#38595=CARTESIAN_POINT ( 'NONE',  ( 11.27110984222679946, 1434.117046727379829, 151.5594388631620006 ) ) ;
#38596=CARTESIAN_POINT ( 'NONE',  ( -13.95840997858960009, 1435.352809884700264, 149.6697649492990081 ) ) ;
#38598=CARTESIAN_POINT ( 'NONE',  ( 20.92457304854260158, 1409.643762579499935, 205.0061533375680085 ) ) ;
#38600=CARTESIAN_POINT ( 'NONE',  ( -16.70268422512909723, 1500.167277360910020, 229.9148981415720243 ) ) ;
#38602=EDGE_LOOP ( 'NONE', ( #41762, #69786, #15339 ) ) ;
#38603=CARTESIAN_POINT ( 'NONE',  ( 32.03901053599999926, 1430.123112397830027, 250.0966427502979741 ) ) ;
#38604=CYLINDRICAL_SURFACE ( 'NONE', #93996, 2.000000000000000000 ) ;
#38605=CARTESIAN_POINT ( 'NONE',  ( 0.4635522705379999664, 1504.645434567829852, 181.0404501616980042 ) ) ;
#38607=CARTESIAN_POINT ( 'NONE',  ( -17.84692918829999897, 1410.032953027829990, 195.3924022816980255 ) ) ;
#38608=CARTESIAN_POINT ( 'NONE',  ( 1.861700016370000164E-09, 1407.650947845630071, 270.1377426662980383 ) ) ;
#38609=CARTESIAN_POINT ( 'NONE',  ( -23.75152772239999877, 1432.714080072660181, 220.8246967967979799 ) ) ;
#38613=CARTESIAN_POINT ( 'NONE',  ( 30.24133951009999777, 1451.857592286530007, 135.2575210613979948 ) ) ;
#38617=EDGE_CURVE ( 'NONE', #100495, #34701, #81521, .T. ) ;
#38618=CARTESIAN_POINT ( 'NONE',  ( 2.905289237559999904, 1509.014515323130126, 238.4132587644979822 ) ) ;
#38620=ORIENTED_EDGE ( 'NONE', *, *, #4133, .F. ) ;
#38622=CARTESIAN_POINT ( 'NONE',  ( -23.91153463986099936, 1410.421621703130086, 208.6572241185120049 ) ) ;
#38628=CARTESIAN_POINT ( 'NONE',  ( -4.375055004340000053, 1479.770299212029840, 235.2382511805980130 ) ) ;
#38632=CARTESIAN_POINT ( 'NONE',  ( 11.15480544429999910, 1425.160630053029990, 144.1619436902979885 ) ) ;
#38633=CARTESIAN_POINT ( 'NONE',  ( -12.16511160556770044, 1414.971513442450032, 220.6991975209760142 ) ) ;
#38636=ORIENTED_EDGE ( 'NONE', *, *, #2908, .F. ) ;
#38638=CARTESIAN_POINT ( 'NONE',  ( 13.27015362366167217, 1443.199215167730699, 187.6658312763560446 ) ) ;
#38643=CARTESIAN_POINT ( 'NONE',  ( -4.363122647530000009, 1409.354802298930053, 146.1721969590979882 ) ) ;
#38645=CARTESIAN_POINT ( 'NONE',  ( -4.459046139639999851, 1425.240413237929943, 186.1432435763979925 ) ) ;
#38650=CARTESIAN_POINT ( 'NONE',  ( -10.97268961956110012, 1432.538086023540245, 151.7700193388709806 ) ) ;
#38651=CARTESIAN_POINT ( 'NONE',  ( 0.03704823030615916196, 1409.672459229776450, 233.0526395660594972 ) ) ;
#38659=CARTESIAN_POINT ( 'NONE',  ( 17.24149055319999846, 1434.891998881070094, 209.1218459616979999 ) ) ;
#38660=CARTESIAN_POINT ( 'NONE',  ( -0.04714347637158690374, 1424.289205137260069, 227.6285544301180153 ) ) ;
#38663=ADVANCED_FACE ( 'NONE', ( #82954 ), #67021, .F. ) ;
#38668=CARTESIAN_POINT ( 'NONE',  ( -1.661536740469999884, 1441.600846913620217, 150.6803463261979914 ) ) ;
#38669=CARTESIAN_POINT ( 'NONE',  ( -13.79565920049999939, 1416.830001024129842, 221.9088573472979817 ) ) ;
#38675=CARTESIAN_POINT ( 'NONE',  ( 15.98031816559999996, 1422.108692535729915, 227.4722591969980101 ) ) ;
#38678=CARTESIAN_POINT ( 'NONE',  ( 45.66301396820000491, 1436.924929342960013, 268.7619381858979750 ) ) ;
#38679=CARTESIAN_POINT ( 'NONE',  ( -19.06484846609999906, 1410.501627938029969, 222.8115755776980222 ) ) ;
#38680=CARTESIAN_POINT ( 'NONE',  ( 18.47698316009999786, 1435.143056706319840, 145.4054505043980043 ) ) ;
#38681=CARTESIAN_POINT ( 'NONE',  ( -0.7130142950260000001, 1416.844618646229947, 227.9191939115979721 ) ) ;
#38683=CARTESIAN_POINT ( 'NONE',  ( -15.94338848148980148, 1409.469815784339971, 192.9752912694130202 ) ) ;
#38684=CARTESIAN_POINT ( 'NONE',  ( 12.61618830369999955, 1416.831305870130109, 223.3237475159979795 ) ) ;
#38686=CARTESIAN_POINT ( 'NONE',  ( -36.72317469411459712, 1436.720746570669917, 136.2687545549769936 ) ) ;
#38687=CARTESIAN_POINT ( 'NONE',  ( 0.2120850959947599979, 1456.177984629059893, 183.1170619906590105 ) ) ;
#38688=CARTESIAN_POINT ( 'NONE',  ( -8.260959520976138393, 1408.154429929020125, 220.0006158248199881 ) ) ;
#38692=CARTESIAN_POINT ( 'NONE',  ( 12.40435961620000072, 1434.419950087150255, 147.6244959444979941 ) ) ;
#38693=CARTESIAN_POINT ( 'NONE',  ( -39.18506236317279701, 1437.902641090850011, 134.0999999975949777 ) ) ;
#38698=CARTESIAN_POINT ( 'NONE',  ( -9.025147011466630786, 1409.228225465760033, 221.0552217307139813 ) ) ;
#38701=CARTESIAN_POINT ( 'NONE',  ( 14.46831308334499866, 1508.704177307590044, 232.8351181552330047 ) ) ;
#38702=CARTESIAN_POINT ( 'NONE',  ( 31.94087964542345048, 1416.502482517117869, 269.3169482426198442 ) ) ;
#38709=CARTESIAN_POINT ( 'NONE',  ( -28.46393112459029950, 1508.969040165770139, 208.7960455483320175 ) ) ;
#38711=CARTESIAN_POINT ( 'NONE',  ( 2.745142294599053567, 1419.769955103634175, 137.0999999980979567 ) ) ;
#38715=CARTESIAN_POINT ( 'NONE',  ( 5.191014570674193251, 1422.191164659828701, 138.4291919130531880 ) ) ;
#38719=B_SPLINE_CURVE_WITH_KNOTS ( 'NONE', 3,
 ( #9361, #102841, #60324, #43525 ),
 .UNSPECIFIED., .F., .F.,
 ( 4, 4 ),
 ( 5.115887024574549358, 6.089794067229999719 ),
 .UNSPECIFIED. ) ;
#38720=CARTESIAN_POINT ( 'NONE',  ( 20.90914698570000141, 1409.807713502029856, 217.2189215442579950 ) ) ;
#38721=FACE_OUTER_BOUND ( 'NONE', #107334, .T. ) ;
#38723=CARTESIAN_POINT ( 'NONE',  ( -17.86815066140000141, 1424.407639920930023, 228.2372701936979809 ) ) ;
#38727=AXIS2_PLACEMENT_3D ( 'NONE', #57795, #49381, #40411 ) ;
#38730=CARTESIAN_POINT ( 'NONE',  ( -1.831354244299999934, 1416.588294615730092, 233.3593385782979794 ) ) ;
#38733=CARTESIAN_POINT ( 'NONE',  ( -10.33648297811009975, 1485.164656460750166, 184.8983750646000033 ) ) ;
#38736=CARTESIAN_POINT ( 'NONE',  ( 18.89905511659999959, 1416.828040475729949, 210.6687957193779823 ) ) ;
#38739=ORIENTED_EDGE ( 'NONE', *, *, #59080, .F. ) ;
#38740=CARTESIAN_POINT ( 'NONE',  ( 27.46146691510000082, 1508.600904575230061, 213.3784942867079906 ) ) ;
#38742=CARTESIAN_POINT ( 'NONE',  ( 3.214223995087363672, 1507.157967210614061, 181.4588691370872482 ) ) ;
#38744=CARTESIAN_POINT ( 'NONE',  ( 15.94629373821300078, 1419.829628885949887, 191.2397526529200036 ) ) ;
#38745=CARTESIAN_POINT ( 'NONE',  ( 20.89213389120000031, 1453.805113726430136, 224.2163675376980052 ) ) ;
#38747=ADVANCED_FACE ( 'NONE', ( #15039 ), #38604, .F. ) ;
#38748=CARTESIAN_POINT ( 'NONE',  ( -24.31234282530909852, 1452.048309861259895, 136.6059775254549891 ) ) ;
#38750=CARTESIAN_POINT ( 'NONE',  ( 12.52086369699999935, 1410.723690760830095, 228.7769307124980003 ) ) ;
#38754=B_SPLINE_CURVE_WITH_KNOTS ( 'NONE', 3,
 ( #99652, #99104, #57147, #66103, #38660, #40314 ),
 .UNSPECIFIED., .F., .F.,
 ( 4, 2, 4 ),
 ( -0.03264310120058740161, -0.01583012587366310064, -2.621721704315627122E-08 ),
 .UNSPECIFIED. ) ;
#38755=CARTESIAN_POINT ( 'NONE',  ( 41.59656558032850171, 1442.666623284490015, 134.0999999980969903 ) ) ;
#38756=CARTESIAN_POINT ( 'NONE',  ( -40.10831975841819741, 1442.142396374759983, 136.9487569356429901 ) ) ;
#38758=CARTESIAN_POINT ( 'NONE',  ( 14.55552041736240021, 1435.948062197440095, 149.7943142905429852 ) ) ;
#38764=CARTESIAN_POINT ( 'NONE',  ( -0.07105538368350000633, 1451.175970991930171, 182.5309677413980012 ) ) ;
#38768=CARTESIAN_POINT ( 'NONE',  ( -16.20118746261578835, 1450.456937708418309, 221.2434354958739675 ) ) ;
#38771=CARTESIAN_POINT ( 'NONE',  ( 28.13497766429999913, 1508.084884363030142, 208.3112646548739804 ) ) ;
#38772=CARTESIAN_POINT ( 'NONE',  ( 8.218608085730000568, 1415.425433635630043, 193.5610124803980057 ) ) ;
#38774=ORIENTED_EDGE ( 'NONE', *, *, #29579, .F. ) ;
#38778=CARTESIAN_POINT ( 'NONE',  ( 35.59427720072490331, 1440.913060387330006, 261.7132250683009715 ) ) ;
#38779=CARTESIAN_POINT ( 'NONE',  ( 19.03110457520000054, 1457.047041247629977, 226.1578386330979811 ) ) ;
#38781=CARTESIAN_POINT ( 'NONE',  ( -0.1198308412573760029, 1451.168734167799812, 182.5321973637160227 ) ) ;
#38784=CARTESIAN_POINT ( 'NONE',  ( -24.49718675060000095, 1441.226578766219973, 211.0033545095979832 ) ) ;
#38785=CARTESIAN_POINT ( 'NONE',  ( 22.46374799362600072, 1410.651871220149815, 206.2118963477199998 ) ) ;
#38789=CARTESIAN_POINT ( 'NONE',  ( 11.40383981496231591, 1425.336178278838133, 144.1583008349757336 ) ) ;
#38790=CARTESIAN_POINT ( 'NONE',  ( 4.627533690799999988, 1466.419777224029986, 233.9118733120979812 ) ) ;
#38791=CARTESIAN_POINT ( 'NONE',  ( 0.1205199568272290050, 1457.838980749249913, 229.0211416662100135 ) ) ;
#38793=EDGE_CURVE ( 'NONE', #758, #75410, #31735, .T. ) ;
#38795=CARTESIAN_POINT ( 'NONE',  ( -22.71594008370638562, 1409.706314096660435, 209.0156538452060317 ) ) ;
#38805=CARTESIAN_POINT ( 'NONE',  ( 24.36881673870000142, 1444.160329039040107, 213.3381660858680107 ) ) ;
#38806=CARTESIAN_POINT ( 'NONE',  ( -11.76319757070000094, 1431.851246079359953, 150.7944596534980235 ) ) ;
#38810=CARTESIAN_POINT ( 'NONE',  ( 12.22832369420000020, 1445.155617767419926, 186.6170932793979773 ) ) ;
#38811=CARTESIAN_POINT ( 'NONE',  ( -19.46735787119999728, 1444.804550784760067, 225.1090302134979879 ) ) ;
#38812=CARTESIAN_POINT ( 'NONE',  ( 5.386599516782380803, 1432.386091107299762, 154.6080078439310057 ) ) ;
#38814=CARTESIAN_POINT ( 'NONE',  ( -1.622337697689999914, 1484.281053948429872, 182.6410747883979866 ) ) ;
#38815=EDGE_LOOP ( 'NONE', ( #41394, #47198, #33048, #30592 ) ) ;
#38817=CARTESIAN_POINT ( 'NONE',  ( 0.8877057929439999828, 1405.849110591630051, 267.2346354947979989 ) ) ;
#38820=CARTESIAN_POINT ( 'NONE',  ( 22.96977252851270990, 1432.194948239369296, 216.1620617374289850 ) ) ;
#38824=CARTESIAN_POINT ( 'NONE',  ( -1.179291431074050100, 1450.813351930680028, 155.3354871613740045 ) ) ;
#38825=CARTESIAN_POINT ( 'NONE',  ( -1.624815496279135241, 1451.579047725773080, 184.0101596272184565 ) ) ;
#38826=CARTESIAN_POINT ( 'NONE',  ( 2.496316844175979544, 1449.223786328959932, 155.0643092729569901 ) ) ;
#38827=CARTESIAN_POINT ( 'NONE',  ( -13.94822761416910240, 1415.393085341430151, 220.8713811350969820 ) ) ;
#38829=CARTESIAN_POINT ( 'NONE',  ( -28.52406122560000057, 1430.067484667830058, 255.3819207682979595 ) ) ;
#38832=CARTESIAN_POINT ( 'NONE',  ( 2.499999926920000171, 1440.210289421680045, 168.7266379278979969 ) ) ;
#38833=CARTESIAN_POINT ( 'NONE',  ( -6.209676061589999740, 1475.800420687429778, 267.8376408680979921 ) ) ;
#38834=DIRECTION ( 'NONE',  ( -0.7067700363771036720, 0.03085824620770448792, -0.7067700363771036720 ) ) ;
#38836=CARTESIAN_POINT ( 'NONE',  ( 6.232532001854651504, 1405.413060387330006, 220.5304192662728440 ) ) ;
#38840=CARTESIAN_POINT ( 'NONE',  ( -24.61293950550089704, 1444.770188684140066, 210.8869336946189890 ) ) ;
#38843=CARTESIAN_POINT ( 'NONE',  ( -10.72715585175719966, 1396.287660924140027, 211.8461252756880242 ) ) ;
#38844=B_SPLINE_CURVE_WITH_KNOTS ( 'NONE', 3,
 ( #59656, #37611, #45492, #60775 ),
 .UNSPECIFIED., .F., .F.,
 ( 4, 4 ),
 ( 0.000000000000000000, 1.000000000000000000 ),
 .UNSPECIFIED. ) ;
#38846=CARTESIAN_POINT ( 'NONE',  ( 19.29701624502764190, 1455.937115892289057, 225.2550683788775814 ) ) ;
#38851=CARTESIAN_POINT ( 'NONE',  ( 10.52899685699999921, 1425.090219727929934, 126.2876617244979798 ) ) ;
#38859=CARTESIAN_POINT ( 'NONE',  ( 2.336427541990000023, 1507.413612230230001, 181.2610990600980188 ) ) ;
#38863=CARTESIAN_POINT ( 'NONE',  ( 17.22670715777832839, 1410.879751196339157, 192.2060273682096749 ) ) ;
#38866=CARTESIAN_POINT ( 'NONE',  ( -14.45727104390000051, 1444.967096565130078, 188.7843282767979929 ) ) ;
#38867=CARTESIAN_POINT ( 'NONE',  ( 2.871070354779960088, 1409.266853455240152, 231.0074625432760058 ) ) ;
#38868=CARTESIAN_POINT ( 'NONE',  ( -1.159637561150000051, 1415.063410489829948, 226.6648382762980134 ) ) ;
#38869=CARTESIAN_POINT ( 'NONE',  ( -0.0001401872352955277768, 1395.950288251542815, 220.5864547455709044 ) ) ;
#38870=CARTESIAN_POINT ( 'NONE',  ( -14.28311008799576065, 1434.994877684804578, 148.2389552663005077 ) ) ;
#38873=CARTESIAN_POINT ( 'NONE',  ( 16.74784213730000104, 1413.534413880030115, 226.5806976118979890 ) ) ;
#38874=CARTESIAN_POINT ( 'NONE',  ( 14.16563741459999903, 1410.295047179630046, 191.3811060272979887 ) ) ;
#38876=CARTESIAN_POINT ( 'NONE',  ( 8.445405620969070881, 1396.207980526650090, 201.9858892368549732 ) ) ;
#38877=CARTESIAN_POINT ( 'NONE',  ( -39.61513715173970240, 1439.514898078000215, 136.6561437647560240 ) ) ;
#38878=CARTESIAN_POINT ( 'NONE',  ( 10.81519956410000027, 1424.921090988229935, 144.1714224093980192 ) ) ;
#38879=CARTESIAN_POINT ( 'NONE',  ( 41.48884051969999831, 1443.959437935279993, 136.5760756673980154 ) ) ;
#38880=ORIENTED_EDGE ( 'NONE', *, *, #35506, .T. ) ;
#38881=CARTESIAN_POINT ( 'NONE',  ( 3.842196749729999805, 1424.768327057229953, 185.0917902076980113 ) ) ;
#38882=CARTESIAN_POINT ( 'NONE',  ( 1.857330175695710350, 1450.366835696837143, 181.8689242810781366 ) ) ;
#38885=CARTESIAN_POINT ( 'NONE',  ( -17.95163359629999533, 1488.038499059930018, 229.1097482272980130 ) ) ;
#38893=CARTESIAN_POINT ( 'NONE',  ( -8.942586000020730452, 1509.338997363079898, 180.2808501620069990 ) ) ;
#38896=CARTESIAN_POINT ( 'NONE',  ( -15.42462372342430932, 1461.099982565929849, 228.7269502612183771 ) ) ;
#38898=ORIENTED_EDGE ( 'NONE', *, *, #30443, .F. ) ;
#38901=CARTESIAN_POINT ( 'NONE',  ( -35.14253230574213660, 1424.207438634963864, 269.5334840037577351 ) ) ;
#38902=CARTESIAN_POINT ( 'NONE',  ( -1.637939388229999960, 1410.349266066630207, 232.9014652880979952 ) ) ;
#38903=CARTESIAN_POINT ( 'NONE',  ( -10.78330898009999927, 1453.313060387329870, 191.8873814369979982 ) ) ;
#38906=CARTESIAN_POINT ( 'NONE',  ( -35.38730834711080320, 1440.913060388089889, 251.6904557940889902 ) ) ;
#38908=CARTESIAN_POINT ( 'NONE',  ( -0.3690490828443839799, 1465.421766398420004, 236.2943576644740062 ) ) ;
#38909=CARTESIAN_POINT ( 'NONE',  ( 15.30542547920000018, 1410.181902236829728, 270.3573229405980101 ) ) ;
#38913=CARTESIAN_POINT ( 'NONE',  ( 23.05752159060000039, 1409.824208518830119, 208.4404237973319880 ) ) ;
#38916=CIRCLE ( 'NONE', #46164, 7.975189853890007896 ) ;
#38919=CARTESIAN_POINT ( 'NONE',  ( 4.267709349675449459, 1420.674582551029971, 185.5795260963529927 ) ) ;
#38920=CARTESIAN_POINT ( 'NONE',  ( -8.480871446589999252, 1420.439733004030131, 230.9234419115979904 ) ) ;
#38921=( BOUNDED_SURFACE ( )  B_SPLINE_SURFACE ( 3, 2, ( 
 ( #100369, #23654, #93058 ),
 ( #91963, #14701, #49973 ),
 ( #6846, #39915, #15239 ),
 ( #75185, #41007, #32619 ),
 ( #24191, #58378, #65131 ),
 ( #109874, #92504, #49431 ),
 ( #84109, #7409, #41574 ),
 ( #58927, #67342, #74084 ),
 ( #101440, #24730, #108213 ),
 ( #16332, #7954, #73535 ),
 ( #31501, #107671, #30956 ),
 ( #91426, #48890, #83018 ) ),
 .UNSPECIFIED., .F., .F., .F. ) 
 B_SPLINE_SURFACE_WITH_KNOTS ( ( 4, 2, 2, 2, 2, 4 ),
 ( 3, 3 ),
 ( -4.818654156246715559E-13, 0.0004428215754125967830, 0.0008856431513070589815, 0.001328464727201521126, 0.001549875515148752252, 0.001771286303095983379 ),
 ( 0.000000000000000000, 1.000000000000000000 ),
 .UNSPECIFIED. ) 
 GEOMETRIC_REPRESENTATION_ITEM ( )  RATIONAL_B_SPLINE_SURFACE ( (
 ( 1.000000000000000000, 0.8676549166461677842, 1.000000000000000000),
 ( 1.000000000000000000, 0.8796972043940699537, 1.000000000000000000),
 ( 1.000000000000000000, 0.8923052904408216301, 1.000000000000000000),
 ( 1.000000000000000000, 0.9171311462241392709, 1.000000000000000000),
 ( 1.000000000000000000, 0.9293640644949126006, 1.000000000000000000),
 ( 1.000000000000000000, 0.9509457646758097127, 1.000000000000000000),
 ( 1.000000000000000000, 0.9602070476915617325, 1.000000000000000000),
 ( 1.000000000000000000, 0.9693527540417160582, 1.000000000000000000),
 ( 1.000000000000000000, 0.9716220080584853092, 1.000000000000000000),
 ( 1.000000000000000000, 0.9742788806458316797, 1.000000000000000000),
 ( 1.000000000000000000, 0.9746510992719278343, 1.000000000000000000),
 ( 1.000000000000000000, 0.9740160527066915597, 1.000000000000000000) ) ) 
 REPRESENTATION_ITEM ( '' )  SURFACE ( )  );
#38922=CARTESIAN_POINT ( 'NONE',  ( 10.49818696109023186, 1422.381269827019423, 137.0999999980981272 ) ) ;
#38923=ORIENTED_EDGE ( 'NONE', *, *, #6278, .T. ) ;
#38926=CARTESIAN_POINT ( 'NONE',  ( 0.9892016712189999339, 1417.304970919730067, 235.7878985900979956 ) ) ;
#38930=FACE_OUTER_BOUND ( 'NONE', #92111, .T. ) ;
#38932=CARTESIAN_POINT ( 'NONE',  ( 18.06717587838990013, 1416.826860677879949, 208.8995450462120118 ) ) ;
#38933=DIRECTION ( 'NONE',  ( 0.000000000000000000, 0.000000000000000000, -1.000000000000000000 ) ) ;
#38935=VERTEX_POINT ( 'NONE', #55253 ) ;
#38937=CARTESIAN_POINT ( 'NONE',  ( 29.22958591724099975, 1509.933780020319773, 206.4713313096740137 ) ) ;
#38938=ORIENTED_EDGE ( 'NONE', *, *, #15873, .F. ) ;
#38940=CARTESIAN_POINT ( 'NONE',  ( 20.46232921600000054, 1454.237003251030046, 223.5521112539979924 ) ) ;
#38941=CARTESIAN_POINT ( 'NONE',  ( 8.057909095891742979, 1438.036219788864173, 153.6519697238730942 ) ) ;
#38944=CARTESIAN_POINT ( 'NONE',  ( -27.24127397847530219, 1509.605191577599953, 201.1898831551650062 ) ) ;
#38945=CARTESIAN_POINT ( 'NONE',  ( -10.10004869885203682, 1411.254281879943164, 135.5999999980979851 ) ) ;
#38946=CARTESIAN_POINT ( 'NONE',  ( -19.15018216310000199, 1426.147315663830113, 224.7566274145979719 ) ) ;
#38947=CARTESIAN_POINT ( 'NONE',  ( -31.74245818353665172, 1465.468252347056250, 269.3210959786474064 ) ) ;
#38950=B_SPLINE_CURVE_WITH_KNOTS ( 'NONE', 4,
 ( #96377, #96936, #53859, #29711, #45448 ),
 .UNSPECIFIED., .F., .F.,
 ( 5, 5 ),
 ( 0.000000000000000000, 1.000000000000000000 ),
 .UNSPECIFIED. ) ;
#38952=CARTESIAN_POINT ( 'NONE',  ( -18.31626795570251076, 1436.062568559702640, 213.5329773601903298 ) ) ;
#38961=CARTESIAN_POINT ( 'NONE',  ( 1.469130622283230103, 1487.271942394239886, 181.9786426215879942 ) ) ;
#38963=CARTESIAN_POINT ( 'NONE',  ( -12.92553196027594176, 1442.905430701026944, 186.4482871715469514 ) ) ;
#38965=CARTESIAN_POINT ( 'NONE',  ( -8.313145311751080513, 1507.316772571419961, 235.1568484389069909 ) ) ;
#38968=EDGE_CURVE ( 'NONE', #7623, #94000, #65417, .T. ) ;
#38969=FACE_OUTER_BOUND ( 'NONE', #64404, .T. ) ;
#38977=ORIENTED_EDGE ( 'NONE', *, *, #84249, .T. ) ;
#38979=CARTESIAN_POINT ( 'NONE',  ( 18.05542472024740164, 1416.825783990419950, 208.7596433786079899 ) ) ;
#38982=CARTESIAN_POINT ( 'NONE',  ( 38.80991273106157280, 1429.204819279143976, 269.5897298496287817 ) ) ;
#38983=CARTESIAN_POINT ( 'NONE',  ( -31.18244400280000050, 1447.044067085910001, 244.2061907774979943 ) ) ;
#38984=CARTESIAN_POINT ( 'NONE',  ( -20.14249648099999845, 1499.094827274529962, 189.7136622036979929 ) ) ;
#38986=CARTESIAN_POINT ( 'NONE',  ( -11.21637391500000192, 1433.532588004509989, 151.5878911200980212 ) ) ;
#38988=CARTESIAN_POINT ( 'NONE',  ( -19.52948423790000021, 1485.515647422730126, 190.0633780688980039 ) ) ;
#38991=CARTESIAN_POINT ( 'NONE',  ( 8.778727692719998643, 1440.670317412140093, 153.7060891647979872 ) ) ;
#38992=CARTESIAN_POINT ( 'NONE',  ( 13.13254582842679774, 1428.645359689489851, 223.2771978780310178 ) ) ;
#38996=CARTESIAN_POINT ( 'NONE',  ( 5.267020990686269920E-09, 1406.060656444949927, 266.8269676183700199 ) ) ;
#38999=CARTESIAN_POINT ( 'NONE',  ( -11.86610048948770135, 1432.336024750160050, 149.9824232984959735 ) ) ;
#39001=CARTESIAN_POINT ( 'NONE',  ( -24.89782654780000115, 1466.147263882030074, 269.9192101110980389 ) ) ;
#39002=CARTESIAN_POINT ( 'NONE',  ( 13.08557583159999993, 1509.198239579430037, 234.3544144791979988 ) ) ;
#39003=CARTESIAN_POINT ( 'NONE',  ( 9.421550853199999409, 1433.443826258700028, 153.1575888881980063 ) ) ;
#39005=CARTESIAN_POINT ( 'NONE',  ( 0.2165510715247410123, 1452.950780108749996, 183.2553406918169969 ) ) ;
#39006=CARTESIAN_POINT ( 'NONE',  ( -9.849896899200842881, 1519.913060387329779, 185.5490084180013923 ) ) ;
#39010=CARTESIAN_POINT ( 'NONE',  ( -41.85400445561560190, 1426.437045596680036, 268.8779146404949643 ) ) ;
#39013=ORIENTED_EDGE ( 'NONE', *, *, #17992, .T. ) ;
#39016=CARTESIAN_POINT ( 'NONE',  ( 17.11714618744286653, 1444.740067931808881, 162.7561046190442369 ) ) ;
#39020=CARTESIAN_POINT ( 'NONE',  ( -13.16389777740000078, 1440.431676128409890, 188.3426591800980248 ) ) ;
#39021=CARTESIAN_POINT ( 'NONE',  ( -15.90881031062220075, 1461.182782413890209, 228.4097491243460070 ) ) ;
#39022=ORIENTED_EDGE ( 'NONE', *, *, #107501, .T. ) ;
#39025=ADVANCED_FACE ( 'NONE', ( #21050 ), #7091, .T. ) ;
#39028=CARTESIAN_POINT ( 'NONE',  ( -39.91390632348250023, 1425.727616005299978, 270.2554194705400050 ) ) ;
#39030=CARTESIAN_POINT ( 'NONE',  ( -2.403335121230000038, 1396.180591763030179, 197.3371931114980100 ) ) ;
#39032=EDGE_LOOP ( 'NONE', ( #30173, #105285, #12396, #24556 ) ) ;
#39037=CARTESIAN_POINT ( 'NONE',  ( -0.03715205675588980488, 1409.647736300129964, 185.2081566933059946 ) ) ;
#39042=CARTESIAN_POINT ( 'NONE',  ( 12.78690713350000152, 1416.828040475229955, 222.7042044314979989 ) ) ;
#39047=CARTESIAN_POINT ( 'NONE',  ( -33.91369104902859988, 1451.728768199629940, 135.6928041595160153 ) ) ;
#39048=CARTESIAN_POINT ( 'NONE',  ( -23.50051618060902570, 1448.308771251206053, 215.7218330829513775 ) ) ;
#39049=B_SPLINE_CURVE_WITH_KNOTS ( 'NONE', 5,
 ( #8736, #27215, #384, #35054, #69797, #7644 ),
 .UNSPECIFIED., .F., .F.,
 ( 6, 6 ),
 ( -167.9874969530119984, -30.64195154390000653 ),
 .UNSPECIFIED. ) ;
#39051=CARTESIAN_POINT ( 'NONE',  ( 9.531827753298708572, 1455.676400814010321, 226.7632778638479465 ) ) ;
#39052=CARTESIAN_POINT ( 'NONE',  ( 24.84980271777819993, 1451.808520470279973, 136.8918982205989892 ) ) ;
#39053=CARTESIAN_POINT ( 'NONE',  ( 13.46339118210000052, 1415.263254644529979, 197.1639476829979856 ) ) ;
#39054=CARTESIAN_POINT ( 'NONE',  ( -11.68639022133180028, 1416.948096802419968, 211.2488954177810001 ) ) ;
#39055=CARTESIAN_POINT ( 'NONE',  ( 19.75836274200000275, 1410.963915033830062, 196.8094767124980251 ) ) ;
#39056=B_SPLINE_CURVE_WITH_KNOTS ( 'NONE', 3,
 ( #42759, #36021, #44426, #60127, #76920, #53382, #1316, #1884, #43864, #10818, #86958, #68529, #78569, #25375, #9696, #44988, #16960, #85857, #36559, #70211, #52829, #27609 ),
 .UNSPECIFIED., .F., .F.,
 ( 4, 3, 3, 3, 3, 3, 3, 4 ),
 ( -2.000000000000000000, -1.902662651915229874, -1.582520240992760119, -1.259666668549479951, -0.9395862512417130219, -0.6254581966034109541, -0.3129536411610209790, 0.000000000000000000 ),
 .UNSPECIFIED. ) ;
#39057=CARTESIAN_POINT ( 'NONE',  ( 16.66094735740000132, 1410.867388120730084, 226.5061907895980085 ) ) ;
#39060=CARTESIAN_POINT ( 'NONE',  ( 22.36671582959205651, 1452.044573827695331, 219.5114896727811811 ) ) ;
#39062=CARTESIAN_POINT ( 'NONE',  ( 2.500000000000000000, 1439.615672362369878, 170.5246407131980106 ) ) ;
#39067=B_SPLINE_SURFACE_WITH_KNOTS ( 'NONE', 5, 5, ( 
 ( #50360, #65503, #49249, #22896, #99612, #91774, #48701, #75557, #100717 ),
 ( #41939, #101254, #74458, #16157, #75004, #39731, #109154, #100185, #84486 ),
 ( #92323, #57105, #7773, #83372, #22343, #23999, #24553, #108023, #32438 ),
 ( #6117, #109691, #31872, #108586, #110233, #23468, #15052, #14511, #90671 ),
 ( #6673, #40826, #82825, #64950, #99064, #56543, #57662, #66614, #48144 ),
 ( #15594, #83930, #82283, #7232, #41392, #32967, #60974, #68820, #511 ),
 ( #34636, #61522, #26786, #59315, #60410, #50896, #95099, #35187, #1060 ),
 ( #10543, #94528, #18365, #95650, #67708, #110789, #85026, #8867, #17802 ),
 ( #25111, #35744, #76637, #77751, #52003, #18917, #102921, #43600, #85570 ),
 ( #43051, #52560, #69931, #104044, #8319, #44717, #69372, #78869, #53115 ),
 ( #26221, #86693, #42480, #77208, #33507, #101817, #103481, #93427, #34082 ),
 ( #86143, #16696, #9436, #9987, #25664, #68275, #102382, #44157, #78293 ),
 ( #87252, #59857, #93981, #17247, #51440, #1607, #27336, #70483, #55875 ),
 ( #71602, #88357, #20035, #12187, #4360, #11646, #19480, #105723, #29006 ),
 ( #53682, #106255, #13271, #87824, #46380, #3273, #47462, #29541, #80512 ) ),
 .UNSPECIFIED., .F., .F., .F.,
 ( 6, 3, 3, 3, 6 ),
 ( 6, 3, 6 ),
 ( 71.01177471054140256, 77.03401477149999721, 87.95300694690000398, 98.87199912229999654, 105.5884550614849928 ),
 ( 0.000000000000000000, 1.000000000000000000, 2.000579642670969882 ),
 .UNSPECIFIED. ) ;
#39068=CARTESIAN_POINT ( 'NONE',  ( -44.50818758269999620, 1445.910501413080055, 269.6919245774980141 ) ) ;
#39069=CIRCLE ( 'NONE', #6955, 5.133097426430088817 ) ;
#39070=CARTESIAN_POINT ( 'NONE',  ( -3.609371144360000283, 1448.978751989720195, 184.9854825331979953 ) ) ;
#39073=CARTESIAN_POINT ( 'NONE',  ( -40.26396455803409680, 1444.186530478750001, 137.1012301494149881 ) ) ;
#39074=CARTESIAN_POINT ( 'NONE',  ( 11.60004869885203682, 1425.898600695503546, 137.5181336713743292 ) ) ;
#39075=CARTESIAN_POINT ( 'NONE',  ( -4.500000000000000000, 1425.929641636930000, 127.2892455880980123 ) ) ;
#39076=CARTESIAN_POINT ( 'NONE',  ( -2.500000000000000000, 1419.454841297830171, 146.2312480424980095 ) ) ;
#39079=CARTESIAN_POINT ( 'NONE',  ( 32.01195192442499859, 1440.913060383300035, 244.1429064951479972 ) ) ;
#39085=CARTESIAN_POINT ( 'NONE',  ( 45.67177343720949523, 1440.913060382069943, 266.1885934449759930 ) ) ;
#39089=CARTESIAN_POINT ( 'NONE',  ( 15.08448175589999884, 1409.953164874830009, 191.7150831455979869 ) ) ;
#39094=EDGE_CURVE ( 'NONE', #5500, #52165, #83910, .T. ) ;
#39095=CARTESIAN_POINT ( 'NONE',  ( -13.41982536019999905, 1453.154034701130058, 193.5350393489979979 ) ) ;
#39097=CARTESIAN_POINT ( 'NONE',  ( 1.394897302499999991, 1465.720900699230015, 235.3343340621979962 ) ) ;
#39101=CARTESIAN_POINT ( 'NONE',  ( -0.6413067440629999227, 1451.969509408830163, 183.1830565138979807 ) ) ;
#39105=CARTESIAN_POINT ( 'NONE',  ( -18.09118544614330304, 1416.225364278609959, 209.0355310070899861 ) ) ;
#39106=ORIENTED_EDGE ( 'NONE', *, *, #22963, .T. ) ;
#39112=CARTESIAN_POINT ( 'NONE',  ( -6.754078978114156584, 1512.913060387330006, 184.4732361498326156 ) ) ;
#39113=EDGE_CURVE ( 'NONE', #36273, #104141, #54602, .T. ) ;
#39116=CARTESIAN_POINT ( 'NONE',  ( 13.31407495111609940, 1409.377998129700018, 202.3408434151739925 ) ) ;
#39117=CARTESIAN_POINT ( 'NONE',  ( 18.80463393750000023, 1425.801073282529842, 225.6039001781980176 ) ) ;
#39119=CARTESIAN_POINT ( 'NONE',  ( -18.52955747089999861, 1440.801523186710028, 192.1682810942980097 ) ) ;
#39120=CARTESIAN_POINT ( 'NONE',  ( 11.86550948949999906, 1432.301448183290177, 150.3971867778979856 ) ) ;
#39121=AXIS2_PLACEMENT_3D ( 'NONE', #82591, #15358, #22637 ) ;
#39122=CARTESIAN_POINT ( 'NONE',  ( -4.038223998531310421, 1450.278802180569983, 185.0006718053259647 ) ) ;
#39124=ORIENTED_EDGE ( 'NONE', *, *, #60421, .T. ) ;
#39126=EDGE_CURVE ( 'NONE', #73912, #8321, #94617, .T. ) ;
#39127=CARTESIAN_POINT ( 'NONE',  ( -2.499989269620250809, 1419.524750234567819, 137.1000002976804808 ) ) ;
#39128=CARTESIAN_POINT ( 'NONE',  ( -11.96704581050000016, 1433.884959444120113, 150.6597764172979907 ) ) ;
#39129=CARTESIAN_POINT ( 'NONE',  ( 29.75012120190000076, 1509.993914123429931, 209.6841247587719863 ) ) ;
#39130=CARTESIAN_POINT ( 'NONE',  ( -20.02005738860690087, 1489.080029727439978, 190.9336551125319943 ) ) ;
#39137=CARTESIAN_POINT ( 'NONE',  ( -18.64672481365220236, 1416.851343896850040, 208.5597484336410048 ) ) ;
#39138=EDGE_CURVE ( 'NONE', #89175, #97581, #52947, .T. ) ;
#39139=B_SPLINE_CURVE_WITH_KNOTS ( 'NONE', 5,
 ( #70913, #23210, #74202, #106670, #13142, #38361, #99358, #4761, #29959, #107781, #100479, #47326, #66360, #22632, #47877, #64707, #57948, #56281, #14260, #81456, #23761 ),
 .UNSPECIFIED., .F., .F.,
 ( 6, 3, 3, 3, 3, 3, 6 ),
 ( 122.5631238770533997, 122.5666549750004037, 128.3589772970003082, 134.1528038510001863, 139.9378092970001148, 146.0761118390000206, 146.2079031070000212 ),
 .UNSPECIFIED. ) ;
#39142=CARTESIAN_POINT ( 'NONE',  ( 2.590873905056420234, 1407.641759256400064, 222.0240870714810058 ) ) ;
#39143=CIRCLE ( 'NONE', #101718, 1.000000000000000000 ) ;
#39144=CARTESIAN_POINT ( 'NONE',  ( -13.84691416458350055, 1435.860713939990092, 150.1842040648199941 ) ) ;
#39146=CARTESIAN_POINT ( 'NONE',  ( 6.840648518365643582, 1425.417253097355342, 226.3025326348858073 ) ) ;
#39148=AXIS2_PLACEMENT_3D ( 'NONE', #17131, #78742, #36190 ) ;
#39152=CARTESIAN_POINT ( 'NONE',  ( 27.24390624950000372, 1427.221042094929999, 244.3119003951980233 ) ) ;
#39155=CARTESIAN_POINT ( 'NONE',  ( -1.045121690502980094, 1507.562507687170182, 232.0280612577400063 ) ) ;
#39156=CARTESIAN_POINT ( 'NONE',  ( 21.76163503289691903, 1506.366982240506104, 206.1367291981587186 ) ) ;
#39157=CARTESIAN_POINT ( 'NONE',  ( -29.14244551250000015, 1435.145987499609873, 238.0755264353980181 ) ) ;
#39159=CARTESIAN_POINT ( 'NONE',  ( -0.4878038053971470167, 1452.896025903080044, 152.5254486361209842 ) ) ;
#39160=CARTESIAN_POINT ( 'NONE',  ( 28.26596675839999762, 1451.065831357529987, 136.3389790085980167 ) ) ;
#39161=ORIENTED_EDGE ( 'NONE', *, *, #79640, .T. ) ;
#39162=CARTESIAN_POINT ( 'NONE',  ( 11.07444841881259912, 1415.954755716080172, 222.2791099274719784 ) ) ;
#39163=CARTESIAN_POINT ( 'NONE',  ( -24.41186848580399982, 1440.913060429360030, 212.0284777848129920 ) ) ;
#39164=CARTESIAN_POINT ( 'NONE',  ( 8.917823571280001360, 1509.304539168530027, 237.8784254626980044 ) ) ;
#39167=CARTESIAN_POINT ( 'NONE',  ( -10.23170511530682525, 1422.701956246408599, 137.1234386916033827 ) ) ;
#39168=CARTESIAN_POINT ( 'NONE',  ( -23.92933769846699832, 1410.421755315850078, 208.7355662265979959 ) ) ;
#39171=AXIS2_PLACEMENT_3D ( 'NONE', #22213, #5441, #90540 ) ;
#39173=CARTESIAN_POINT ( 'NONE',  ( -4.395186754550000074, 1489.059423926730005, 235.6527567464979995 ) ) ;
#39177=CARTESIAN_POINT ( 'NONE',  ( 45.67158849016559685, 1441.839016858149989, 266.1883947468940050 ) ) ;
#39178=CARTESIAN_POINT ( 'NONE',  ( -11.70695556590979969, 1414.913057860449953, 220.6083897370939724 ) ) ;
#39180=CARTESIAN_POINT ( 'NONE',  ( -0.1035703829190000036, 1420.452886222830102, 182.7051921315980110 ) ) ;
#39184=CARTESIAN_POINT ( 'NONE',  ( 12.64536475901971890, 1442.792007884521581, 186.5960024392706487 ) ) ;
#39189=CARTESIAN_POINT ( 'NONE',  ( 0.4863421998530879642, 1418.702335047680208, 184.7127968358159933 ) ) ;
#39191=CARTESIAN_POINT ( 'NONE',  ( 8.160491664018758584, 1452.628089738999961, 151.2681714364080108 ) ) ;
#39196=CARTESIAN_POINT ( 'NONE',  ( 0.01602020491292198423, 1408.960543678336762, 232.1618151973992497 ) ) ;
#39197=CARTESIAN_POINT ( 'NONE',  ( -13.54609157666829944, 1434.953585316950011, 148.7557093113670135 ) ) ;
#39200=ADVANCED_FACE ( 'NONE', ( #54670 ), #76879, .F. ) ;
#39201=CARTESIAN_POINT ( 'NONE',  ( -24.83471925681290315, 1509.481687055530074, 222.6988703109550158 ) ) ;
#39204=CARTESIAN_POINT ( 'NONE',  ( 11.40468314536590100, 1414.972329067380088, 222.2791104303979921 ) ) ;
#39208=B_SPLINE_SURFACE_WITH_KNOTS ( 'NONE', 5, 3, ( 
 ( #50328, #67124, #76058, #110201 ),
 ( #32934, #24523, #110756, #49217 ),
 ( #101224, #83343, #108551, #31841 ),
 ( #74973, #15019, #58712, #50858 ),
 ( #92845, #33475, #57627, #49765 ),
 ( #74424, #83896, #66026, #67677 ) ),
 .UNSPECIFIED., .F., .F., .F.,
 ( 6, 6 ),
 ( 4, 4 ),
 ( 0.000000000000000000, 11.48858425020000062 ),
 ( 37.69911184309999896, 40.20365518519999881 ),
 .UNSPECIFIED. ) ;
#39212=ORIENTED_EDGE ( 'NONE', *, *, #48928, .T. ) ;
#39214=CARTESIAN_POINT ( 'NONE',  ( -2.455820327400000114, 1434.541746329560056, 150.3615916412979914 ) ) ;
#39217=CARTESIAN_POINT ( 'NONE',  ( -14.00898869779999956, 1416.833018181429907, 221.8520907042980070 ) ) ;
#39218=CARTESIAN_POINT ( 'NONE',  ( 11.70028423970000020, 1433.720629087699990, 151.0079596410979832 ) ) ;
#39220=CARTESIAN_POINT ( 'NONE',  ( 13.01671764799699993, 1416.842625005220043, 196.3343525426479914 ) ) ;
#39221=B_SPLINE_CURVE_WITH_KNOTS ( 'NONE', 5,
 ( #38736, #63980, #12977, #20279, #98642, #21364, #89696, #55572, #47160 ),
 .UNSPECIFIED., .F., .F.,
 ( 6, 3, 6 ),
 ( 0.7655572723410000169, 2.316155491860000026, 3.835724788519999429 ),
 .UNSPECIFIED. ) ;
#39223=CARTESIAN_POINT ( 'NONE',  ( 2.921915679247010011, 1414.085076703340064, 231.7960692163919703 ) ) ;
#39224=CARTESIAN_POINT ( 'NONE',  ( -12.86224528119999988, 1519.913060387329779, 228.0025448475979886 ) ) ;
#39225=CARTESIAN_POINT ( 'NONE',  ( 16.45032630069999868, 1417.430338871630056, 226.9554082569979983 ) ) ;
#39228=CARTESIAN_POINT ( 'NONE',  ( -19.07843485409999928, 1410.941104706429996, 222.8264070888980086 ) ) ;
#39231=CARTESIAN_POINT ( 'NONE',  ( 19.79807428129999991, 1508.018205000529861, 188.8464914106980075 ) ) ;
#39232=CARTESIAN_POINT ( 'NONE',  ( -25.24617298109999908, 1450.838013018590118, 137.6080363986979762 ) ) ;
#39236=EDGE_CURVE ( 'NONE', #61659, #34791, #27791, .T. ) ;
#39239=CARTESIAN_POINT ( 'NONE',  ( -9.435157404909999102, 1414.913060387329779, 222.1292708042979882 ) ) ;
#39240=CARTESIAN_POINT ( 'NONE',  ( 0.2100116478871839887, 1457.341752983120159, 183.0671337708849933 ) ) ;
#39241=CARTESIAN_POINT ( 'NONE',  ( -14.17767550720000003, 1409.408155725629967, 203.0979980328280021 ) ) ;
#39244=EDGE_CURVE ( 'NONE', #77737, #70841, #47825, .T. ) ;
#39245=CARTESIAN_POINT ( 'NONE',  ( -8.178500771994089646, 1441.152429774469965, 153.9860759686779943 ) ) ;
#39246=CARTESIAN_POINT ( 'NONE',  ( 12.40410385870000098, 1434.420076928460048, 149.1896426101980069 ) ) ;
#39247=DIRECTION ( 'NONE',  ( -2.473221764039894783E-17, 0.000000000000000000, -1.000000000000000000 ) ) ;
#39249=ORIENTED_EDGE ( 'NONE', *, *, #35506, .F. ) ;
#39254=CARTESIAN_POINT ( 'NONE',  ( -0.5038386193489999831, 1452.963758663529916, 183.2902632327979973 ) ) ;
#39255=EDGE_CURVE ( 'NONE', #101013, #105289, #95848, .T. ) ;
#39256=CARTESIAN_POINT ( 'NONE',  ( 0.1681681984989999989, 1420.016189442530049, 171.1670476502980023 ) ) ;
#39257=CARTESIAN_POINT ( 'NONE',  ( 44.74173090250090468, 1434.085289301948251, 268.9999157369318823 ) ) ;
#39259=CARTESIAN_POINT ( 'NONE',  ( -19.73881298686153229, 1499.102984487484946, 189.2247233355559501 ) ) ;
#39265=CARTESIAN_POINT ( 'NONE',  ( -27.03405988099999746, 1451.512678451430020, 136.1495578053979614 ) ) ;
#39266=EDGE_CURVE ( 'NONE', #55879, #109101, #10552, .T. ) ;
#39269=CARTESIAN_POINT ( 'NONE',  ( -16.33510206972449907, 1410.578254075250015, 226.6050706015539902 ) ) ;
#39270=CARTESIAN_POINT ( 'NONE',  ( 0.5133626083067620582, 1410.311097044259895, 185.0719925509139898 ) ) ;
#39271=ORIENTED_EDGE ( 'NONE', *, *, #51179, .F. ) ;
#39272=CARTESIAN_POINT ( 'NONE',  ( -12.00508716839999934, 1508.989785511929995, 182.7232473457980007 ) ) ;
#39276=CARTESIAN_POINT ( 'NONE',  ( -0.1980063625633159963, 1419.359867767670039, 184.4979803712249975 ) ) ;
#39279=CARTESIAN_POINT ( 'NONE',  ( 19.54316991260000336, 1410.091339499530022, 220.4324682491979956 ) ) ;
#39280=CARTESIAN_POINT ( 'NONE',  ( -1.804128457859720092, 1410.345740199939883, 186.0509510551849814 ) ) ;
#39282=CARTESIAN_POINT ( 'NONE',  ( -18.14246331760000075, 1424.695492789029913, 227.8876255367979979 ) ) ;
#39284=CARTESIAN_POINT ( 'NONE',  ( 16.63178568020000014, 1409.493855139530069, 223.7919630844980077 ) ) ;
#39292=CARTESIAN_POINT ( 'NONE',  ( -11.57752524527410110, 1486.021447801480008, 184.4692410163380032 ) ) ;
#39293=ORIENTED_EDGE ( 'NONE', *, *, #65928, .F. ) ;
#39296=CARTESIAN_POINT ( 'NONE',  ( -4.234119969708030951, 1441.492840331990010, 163.8906307119239898 ) ) ;
#39298=EDGE_LOOP ( 'NONE', ( #22862, #89108, #6361, #53623 ) ) ;
#39300=CARTESIAN_POINT ( 'NONE',  ( 28.70345850190000192, 1509.590240593130147, 210.2487084362280143 ) ) ;
#39301=ORIENTED_EDGE ( 'NONE', *, *, #105536, .F. ) ;
#39304=CARTESIAN_POINT ( 'NONE',  ( -11.39350426579230025, 1425.508008078089915, 141.1901541546949943 ) ) ;
#39305=CARTESIAN_POINT ( 'NONE',  ( 1.152385366779999920, 1508.177879779530031, 180.8347444588980011 ) ) ;
#39308=CARTESIAN_POINT ( 'NONE',  ( -24.14079447473799789, 1452.054257227049902, 136.9211370085970145 ) ) ;
#39309=B_SPLINE_CURVE_WITH_KNOTS ( 'NONE', 5,
 ( #36875, #86178, #10582, #95687, #69408, #36321 ),
 .UNSPECIFIED., .F., .F.,
 ( 6, 6 ),
 ( 0.000000000000000000, 1.000000000000000000 ),
 .UNSPECIFIED. ) ;
#39310=CARTESIAN_POINT ( 'NONE',  ( -11.73645620750000163, 1426.280382981230105, 144.1655706660979774 ) ) ;
#39315=CARTESIAN_POINT ( 'NONE',  ( 36.53452253882689860, 1451.194196174300032, 134.0999999986999853 ) ) ;
#39316=CARTESIAN_POINT ( 'NONE',  ( -40.26434707082469799, 1443.230809785309930, 137.0716638627269788 ) ) ;
#39317=CARTESIAN_POINT ( 'NONE',  ( 13.95068308120620060, 1435.004429209999898, 148.7713137966129864 ) ) ;
#39321=EDGE_LOOP ( 'NONE', ( #72411, #67173, #97037, #103076, #90432, #65110 ) ) ;
#39324=CARTESIAN_POINT ( 'NONE',  ( 0.09653062418259999999, 1451.692067920030013, 183.0365772874980053 ) ) ;
#39328=CARTESIAN_POINT ( 'NONE',  ( -26.35475552313950232, 1507.985742420310089, 201.5462045797129917 ) ) ;
#39330=CARTESIAN_POINT ( 'NONE',  ( -9277.788495362316098, 2833.746317950420689, 5939.014819763676314 ) ) ;
#39331=CARTESIAN_POINT ( 'NONE',  ( -10613.67162176269994, 54.28084076250828360, 5061.882847083795241 ) ) ;
#39332=CARTESIAN_POINT ( 'NONE',  ( 11.80290349340000056, 1415.088016306429836, 196.9360299734980231 ) ) ;
#39339=CARTESIAN_POINT ( 'NONE',  ( 19.65890388680000100, 1477.381973150129852, 226.7576334579979971 ) ) ;
#39340=ORIENTED_EDGE ( 'NONE', *, *, #72907, .F. ) ;
#39342=CARTESIAN_POINT ( 'NONE',  ( -16.31589243200000183, 1410.414964140629991, 191.5459822045979763 ) ) ;
#39347=CARTESIAN_POINT ( 'NONE',  ( -2.158139092959999950, 1508.640225114429995, 180.2987574298980178 ) ) ;
#39348=CARTESIAN_POINT ( 'NONE',  ( -13.19883015649999969, 1434.900409594529947, 147.8554851810979756 ) ) ;
#39350=CARTESIAN_POINT ( 'NONE',  ( 16.58228743579999787, 1460.774766522529944, 229.0346157100979951 ) ) ;
#39351=CARTESIAN_POINT ( 'NONE',  ( -11.60004869885203682, 1423.973206102585664, 135.9381536973014590 ) ) ;
#39354=B_SPLINE_SURFACE_WITH_KNOTS ( 'NONE', 5, 5, ( 
 ( #97314, #97854, #20583, #12201, #46396, #29021, #105174, #69944, #20051 ),
 ( #106270, #62094, #36859, #87839, #79427, #11127, #87266, #80527, #2738 ),
 ( #37970, #29556, #62658, #63741, #96780, #54245, #88371, #21129, #27351 ),
 ( #11661, #10560, #78309, #45837, #86708, #1624, #35760, #104058, #3288 ),
 ( #61535, #78884, #79970, #95665, #44734, #27912, #2190, #36303, #70499 ),
 ( #104616, #73224, #73789, #90560, #13839, #31209, #23353, #65943, #100067 ) ),
 .UNSPECIFIED., .F., .F., .F.,
 ( 6, 6 ),
 ( 6, 3, 6 ),
 ( 9.202839167560000533, 20.64174078209999763 ),
 ( 0.000000000000000000, 1.000000000000000000, 2.000000000000000000 ),
 .UNSPECIFIED. ) ;
#39356=CARTESIAN_POINT ( 'NONE',  ( -0.08725294298748798028, 1486.463441972811779, 181.7930006954420037 ) ) ;
#39360=CARTESIAN_POINT ( 'NONE',  ( 18.70459388869999628, 1509.566239198929907, 186.5372755795979742 ) ) ;
#39367=CARTESIAN_POINT ( 'NONE',  ( -11.29610511779999982, 1431.916778257889973, 151.5105990156980056 ) ) ;
#39370=CARTESIAN_POINT ( 'NONE',  ( 27.01856162345059786, 1451.963899306131680, 135.0861192397252069 ) ) ;
#39373=B_SPLINE_CURVE_WITH_KNOTS ( 'NONE', 3,
 ( #26548, #100619, #59617, #14954 ),
 .UNSPECIFIED., .F., .F.,
 ( 4, 4 ),
 ( 0.000000000000000000, 1.000000000000000000 ),
 .UNSPECIFIED. ) ;
#39374=CARTESIAN_POINT ( 'NONE',  ( -21.23607560820000018, 1470.084651651229933, 224.2120819598980006 ) ) ;
#39375=CARTESIAN_POINT ( 'NONE',  ( -9.482852257741408053, 1424.109967149583326, 139.1406704986484044 ) ) ;
#39379=CARTESIAN_POINT ( 'NONE',  ( 3.757756526780000161, 1406.106055978829772, 266.9554538344980301 ) ) ;
#39382=CARTESIAN_POINT ( 'NONE',  ( 21.09445956586550608, 1428.283637055626286, 219.6230929203899507 ) ) ;
#39385=CARTESIAN_POINT ( 'NONE',  ( 11.73709356406289928, 1426.695943121369965, 144.1748013758129900 ) ) ;
#39387=CARTESIAN_POINT ( 'NONE',  ( -2.441038202540000146, 1449.508741061479896, 155.6080925163979884 ) ) ;
#39388=CARTESIAN_POINT ( 'NONE',  ( -11.95968169409999859, 1446.500037956690221, 187.4450202269979968 ) ) ;
#39390=CARTESIAN_POINT ( 'NONE',  ( -19.88407671807765809, 1485.200176455136216, 190.7915739009804099 ) ) ;
#39394=CARTESIAN_POINT ( 'NONE',  ( -23.42675388609999843, 1438.250513045190246, 234.3916895488980003 ) ) ;
#39397=CARTESIAN_POINT ( 'NONE',  ( -4.969071879919999546, 1475.566901209930165, 269.0361176487980401 ) ) ;
#39398=FACE_OUTER_BOUND ( 'NONE', #105044, .T. ) ;
#39400=CARTESIAN_POINT ( 'NONE',  ( -8.636908121861750942, 1486.516023803749704, 183.0083597854972766 ) ) ;
#39404=CARTESIAN_POINT ( 'NONE',  ( 12.26355851476349912, 1416.702560753930129, 223.5733017519110035 ) ) ;
#39408=CARTESIAN_POINT ( 'NONE',  ( 24.69959627108774924, 1509.552018375699618, 195.6047270735438701 ) ) ;
#39409=CARTESIAN_POINT ( 'NONE',  ( -17.57263694559999934, 1409.691668941730086, 195.6049344922980140 ) ) ;
#39410=CARTESIAN_POINT ( 'NONE',  ( -15.81192270634400288, 1421.036774565764063, 227.0412074172699874 ) ) ;
#39411=CARTESIAN_POINT ( 'NONE',  ( 19.59345072173944757, 1455.474483766830417, 225.8838923643688474 ) ) ;
#39412=ORIENTED_EDGE ( 'NONE', *, *, #33553, .F. ) ;
#39413=DIRECTION ( 'NONE',  ( 0.000000000000000000, 0.000000000000000000, -1.000000000000000000 ) ) ;
#39428=EDGE_CURVE ( 'NONE', #57302, #44714, #24983, .T. ) ;
#39433=CARTESIAN_POINT ( 'NONE',  ( -11.96158875949999967, 1396.389701308929943, 207.5433552565580158 ) ) ;
#39434=CARTESIAN_POINT ( 'NONE',  ( -22.33897111659999979, 1410.187224098330034, 212.0108098173379858 ) ) ;
#39436=CARTESIAN_POINT ( 'NONE',  ( -1.441539353560000070, 1414.983773854429955, 226.5042058782979666 ) ) ;
#39437=CARTESIAN_POINT ( 'NONE',  ( -13.51164583954868448, 1444.016856206453213, 169.3518408349974322 ) ) ;
#39438=CARTESIAN_POINT ( 'NONE',  ( -26.37683243140000044, 1508.582706621130228, 201.5299903364179954 ) ) ;
#39441=CARTESIAN_POINT ( 'NONE',  ( 17.26703884499999830, 1419.032847617429979, 226.5196259762979878 ) ) ;
#39446=CARTESIAN_POINT ( 'NONE',  ( -41.56522242718469329, 1445.106110315470005, 135.9524270544380045 ) ) ;
#39448=CARTESIAN_POINT ( 'NONE',  ( 6.447394074667360364, 1396.138208400039957, 200.1593900886609845 ) ) ;
#39449=CARTESIAN_POINT ( 'NONE',  ( 1.138464810440000141, 1416.254459047329874, 190.2411719155979881 ) ) ;
#39450=CARTESIAN_POINT ( 'NONE',  ( 11.43741207009999883, 1425.481177415629872, 144.1677667564979970 ) ) ;
#39452=VERTEX_POINT ( 'NONE', #97623 ) ;
#39453=CARTESIAN_POINT ( 'NONE',  ( 3.713785113579999742, 1424.815349392029930, 185.0498344327979794 ) ) ;
#39460=DIRECTION ( 'NONE',  ( 0.000000000000000000, 0.000000000000000000, 1.000000000000000000 ) ) ;
#39466=CARTESIAN_POINT ( 'NONE',  ( 2.500000000000000000, 1448.482477207059901, 160.8482066586829831 ) ) ;
#39468=FACE_OUTER_BOUND ( 'NONE', #20516, .T. ) ;
#39470=VERTEX_POINT ( 'NONE', #13033 ) ;
#39472=CIRCLE ( 'NONE', #105584, 451.3741471861067680 ) ;
#39475=CARTESIAN_POINT ( 'NONE',  ( -35.60174245805101378, 1424.724877476223128, 269.5399423230903722 ) ) ;
#39476=CARTESIAN_POINT ( 'NONE',  ( -1.069820623280000049, 1408.950419346429953, 232.0160439753980199 ) ) ;
#39479=CARTESIAN_POINT ( 'NONE',  ( -0.01305586186176959859, 1452.917665869470056, 183.2406260983729851 ) ) ;
#39480=CARTESIAN_POINT ( 'NONE',  ( -33.74865851176389953, 1440.913060389799966, 248.3065938399680022 ) ) ;
#39482=CARTESIAN_POINT ( 'NONE',  ( -0.6059102731196839287, 1465.006891891870055, 237.7143419758519940 ) ) ;
#39483=CARTESIAN_POINT ( 'NONE',  ( 10.53025398842429894, 1410.959292425960030, 269.8740791142779472 ) ) ;
#39487=CARTESIAN_POINT ( 'NONE',  ( 23.30720214069999940, 1409.831584714629798, 208.9977026400509885 ) ) ;
#39492=CARTESIAN_POINT ( 'NONE',  ( 4.207967578379720130, 1420.996416529009821, 185.4063400840479972 ) ) ;
#39493=CARTESIAN_POINT ( 'NONE',  ( 0.1277302730189999735, 1419.774434123929950, 184.3736332935979760 ) ) ;
#39496=ORIENTED_EDGE ( 'NONE', *, *, #61029, .T. ) ;
#39498=CARTESIAN_POINT ( 'NONE',  ( 18.79647803339999967, 1416.822694190429729, 209.8352280844500228 ) ) ;
#39499=CARTESIAN_POINT ( 'NONE',  ( 0.3099421919009999749, 1416.442944220429808, 233.6989699818980171 ) ) ;
#39500=AXIS2_PLACEMENT_3D ( 'NONE', #100650, #58131, #25039 ) ;
#39501=CARTESIAN_POINT ( 'NONE',  ( -21.63548603055769703, 1509.707618109219993, 229.5065455109210006 ) ) ;
#39510=ORIENTED_EDGE ( 'NONE', *, *, #97190, .F. ) ;
#39514=CARTESIAN_POINT ( 'NONE',  ( -0.2751659205230000405, 1506.798305149130101, 231.4088083078979992 ) ) ;
#39515=CARTESIAN_POINT ( 'NONE',  ( 21.15356505109999929, 1453.179070293830137, 222.9746448834980015 ) ) ;
#39516=CARTESIAN_POINT ( 'NONE',  ( 6.026450563690831430, 1440.073360909948860, 154.5831774296489129 ) ) ;
#39519=CARTESIAN_POINT ( 'NONE',  ( -26.56916871408720127, 1508.840664607660074, 201.4539126542630072 ) ) ;
#39522=CARTESIAN_POINT ( 'NONE',  ( -19.05596984009999773, 1425.010854422730063, 224.1379177625979935 ) ) ;
#39523=CARTESIAN_POINT ( 'NONE',  ( -23.61227025210000008, 1435.322036687620084, 137.2858276859979867 ) ) ;
#39525=CARTESIAN_POINT ( 'NONE',  ( 19.64045971950000080, 1507.861171870530143, 188.7866432982980029 ) ) ;
#39527=CARTESIAN_POINT ( 'NONE',  ( -15.89197043703675583, 1469.153657686127644, 269.3685434817093665 ) ) ;
#39531=CARTESIAN_POINT ( 'NONE',  ( 11.87227031139999944, 1435.412617320299887, 147.6610825172980128 ) ) ;
#39533=CARTESIAN_POINT ( 'NONE',  ( -12.54268436849999979, 1408.913060387329779, 221.6645303301980050 ) ) ;
#39534=CARTESIAN_POINT ( 'NONE',  ( 1.468394784813899845, 1487.955722966210033, 181.9488289805979946 ) ) ;
#39535=CARTESIAN_POINT ( 'NONE',  ( -15.43159309022804493, 1451.439643999777445, 222.6302084244509842 ) ) ;
#39536=CARTESIAN_POINT ( 'NONE',  ( -13.19336125707238061, 1444.715447408086675, 186.5675026392735276 ) ) ;
#39537=LINE ( 'NONE', #99418, #80673 ) ;
#39539=CARTESIAN_POINT ( 'NONE',  ( -3.835404308833623155, 1405.413060387330006, 202.1011854665750036 ) ) ;
#39544=DIRECTION ( 'NONE',  ( -0.3363363969979658030, -0.9417419115949056119, 0.000000000000000000 ) ) ;
#39554=CARTESIAN_POINT ( 'NONE',  ( 4.634283904179999078E-09, 1465.695272584029908, 240.4142140037979800 ) ) ;
#39556=CARTESIAN_POINT ( 'NONE',  ( -11.31301446079999984, 1433.586356650280095, 151.4935912186979863 ) ) ;
#39558=CARTESIAN_POINT ( 'NONE',  ( 11.69439630328679947, 1426.723912090049907, 141.1194945047550107 ) ) ;
#39560=FACE_OUTER_BOUND ( 'NONE', #104710, .T. ) ;
#39567=CARTESIAN_POINT ( 'NONE',  ( -1.430581255003579772E-09, 1413.383262237239933, 249.6119133123739857 ) ) ;
#39569=ORIENTED_EDGE ( 'NONE', *, *, #836, .T. ) ;
#39570=CARTESIAN_POINT ( 'NONE',  ( -11.86398566780919950, 1432.188216858459782, 149.9803512562860135 ) ) ;
#39572=CARTESIAN_POINT ( 'NONE',  ( -3.400296248400000110, 1471.337052564629857, 269.3361249056980000 ) ) ;
#39573=CARTESIAN_POINT ( 'NONE',  ( -1.555569193359999991, 1415.296882296330068, 227.2022622829979639 ) ) ;
#39577=CARTESIAN_POINT ( 'NONE',  ( 35.89837063142969953, 1451.292665198759778, 135.5646561065310038 ) ) ;
#39583=CARTESIAN_POINT ( 'NONE',  ( -42.26673233833929544, 1426.182016276979994, 267.7309908727469860 ) ) ;
#39585=CARTESIAN_POINT ( 'NONE',  ( -24.89775034519999863, 1442.835538705840008, 210.5176537872779932 ) ) ;
#39589=AXIS2_PLACEMENT_3D ( 'NONE', #79221, #98197, #55133 ) ;
#39591=CARTESIAN_POINT ( 'NONE',  ( 41.11865450958669754, 1444.162607370569958, 136.7833858997449852 ) ) ;
#39593=CARTESIAN_POINT ( 'NONE',  ( -15.72029972270000009, 1440.436594279349947, 189.7121662737980046 ) ) ;
#39594=CARTESIAN_POINT ( 'NONE',  ( -2.133905332862266135, 1450.047792930902915, 182.8895505775221295 ) ) ;
#39596=CARTESIAN_POINT ( 'NONE',  ( 10.10004869885203682, 1411.254281879943164, 135.5999999980979851 ) ) ;
#39597=( BOUNDED_CURVE ( )  B_SPLINE_CURVE ( 3, ( #36165, #79279, #75985, #26111 ),
 .UNSPECIFIED., .F., .T. ) 
 B_SPLINE_CURVE_WITH_KNOTS ( ( 4, 4 ),
 ( 1.424829929282025898, 1.707080582674059821 ),
 .UNSPECIFIED. ) 
 CURVE ( )  GEOMETRIC_REPRESENTATION_ITEM ( )  RATIONAL_B_SPLINE_CURVE ( ( 1.000000000000000000, 0.9933722251124278424, 0.9933722251124278424, 1.000000000000000000 ) ) 
 REPRESENTATION_ITEM ( '' )  );
#39599=VECTOR ( 'NONE', #46133, 1000.000000000000114 ) ;
#39603=CARTESIAN_POINT ( 'NONE',  ( -44.93140264801330375, 1435.581069431369997, 269.6837702837809729 ) ) ;
#39605=CARTESIAN_POINT ( 'NONE',  ( -1.171291564450000156, 1396.015411382230013, 197.4876103079979828 ) ) ;
#39609=CARTESIAN_POINT ( 'NONE',  ( 0.3350112074000000106, 1452.978120002730066, 183.2691759946980028 ) ) ;
#39610=CARTESIAN_POINT ( 'NONE',  ( 27.49569038830730605, 1468.273487270390888, 269.4050666718689513 ) ) ;
#39612=CARTESIAN_POINT ( 'NONE',  ( -2.500000000000000000, 1419.414122305159026, 142.6947176393313441 ) ) ;
#39613=CARTESIAN_POINT ( 'NONE',  ( -0.03584877448754099361, 1410.017694336640034, 185.0604024924950011 ) ) ;
#39616=DIRECTION ( 'NONE',  ( -2.274506543718548102E-15, -0.7071067811865474617, -0.7071067811865474617 ) ) ;
#39617=CARTESIAN_POINT ( 'NONE',  ( -0.2694122078740051607, 1452.981479858197417, 183.2530805312008511 ) ) ;
#39618=CARTESIAN_POINT ( 'NONE',  ( 4.363122647530000009, 1407.471318475732687, 137.0999999980979851 ) ) ;
#39619=CARTESIAN_POINT ( 'NONE',  ( 4.283856666023710069, 1440.956247486469920, 155.9231014612180104 ) ) ;
#39621=VERTEX_POINT ( 'NONE', #14147 ) ;
#39624=CARTESIAN_POINT ( 'NONE',  ( -38.81202643698959776, 1450.612734567539974, 134.7398511103019985 ) ) ;
#39626=CARTESIAN_POINT ( 'NONE',  ( -23.37010607166610043, 1448.870807780643645, 216.3500970213881089 ) ) ;
#39627=ORIENTED_EDGE ( 'NONE', *, *, #108252, .F. ) ;
#39628=CARTESIAN_POINT ( 'NONE',  ( 9.265501621498845708, 1455.798605834726004, 226.8760981150780935 ) ) ;
#39630=CARTESIAN_POINT ( 'NONE',  ( 13.47470376080000065, 1415.128105756529976, 197.4143262845979905 ) ) ;
#39633=CARTESIAN_POINT ( 'NONE',  ( 17.50305786550000064, 1410.885931832129927, 225.6206267369979912 ) ) ;
#39635=CARTESIAN_POINT ( 'NONE',  ( 13.89869200000000049, 1452.835253893030085, 223.8385666725980059 ) ) ;
#39636=CARTESIAN_POINT ( 'NONE',  ( 4.247012561190310009, 1441.378048274870025, 161.6132208113730258 ) ) ;
#39640=ORIENTED_EDGE ( 'NONE', *, *, #106213, .T. ) ;
#39643=CARTESIAN_POINT ( 'NONE',  ( -41.12099125829999480, 1454.819569115930108, 269.7572481037980197 ) ) ;
#39644=CARTESIAN_POINT ( 'NONE',  ( -11.71997758781537868, 1414.913060387329779, 220.1971170300299434 ) ) ;
#39645=CARTESIAN_POINT ( 'NONE',  ( -3.047791110882830168, 1421.605825503799906, 133.5222801187929917 ) ) ;
#39648=CARTESIAN_POINT ( 'NONE',  ( 2.095694667039108339, 1417.379259930220314, 233.2286282754426168 ) ) ;
#39649=CARTESIAN_POINT ( 'NONE',  ( -2.500000000000000000, 1432.180584051779761, 157.4911758378979982 ) ) ;
#39652=CARTESIAN_POINT ( 'NONE',  ( 28.49669390769100374, 1440.913060387309997, 233.1064013253619862 ) ) ;
#39655=CARTESIAN_POINT ( 'NONE',  ( 13.21447417100000088, 1422.962187270429922, 221.8217804547979881 ) ) ;
#39656=VERTEX_POINT ( 'NONE', #108767 ) ;
#39659=CARTESIAN_POINT ( 'NONE',  ( 13.51610093808350221, 1442.913060377700731, 150.6358704321319237 ) ) ;
#39662=CARTESIAN_POINT ( 'NONE',  ( -0.5085492386525418684, 1408.930820210946422, 186.5021863892519320 ) ) ;
#39665=CARTESIAN_POINT ( 'NONE',  ( -17.73406580063780069, 1423.343214054229975, 226.1884525926029994 ) ) ;
#39668=CARTESIAN_POINT ( 'NONE',  ( -16.09728575562460051, 1496.785509464440111, 224.3774119518249961 ) ) ;
#39669=CARTESIAN_POINT ( 'NONE',  ( -15.03004244010000079, 1489.480617680229898, 193.2534437250980091 ) ) ;
#39671=CARTESIAN_POINT ( 'NONE',  ( 2.219216292930000112, 1464.733825611330076, 235.9342693422979949 ) ) ;
#39673=ORIENTED_EDGE ( 'NONE', *, *, #84652, .T. ) ;
#39674=CARTESIAN_POINT ( 'NONE',  ( -0.7219500573439999735, 1452.548174062430007, 183.3754457303979848 ) ) ;
#39681=VERTEX_POINT ( 'NONE', #6310 ) ;
#39684=CARTESIAN_POINT ( 'NONE',  ( -11.60004869884828338, 1426.501519354271977, 135.6460154492365575 ) ) ;
#39686=CARTESIAN_POINT ( 'NONE',  ( 2.745142294599053567, 1419.769955103634175, 137.0999999980979567 ) ) ;
#39687=B_SPLINE_CURVE_WITH_KNOTS ( 'NONE', 3,
 ( #5637, #75058, #14566, #57162, #82879, #82337, #40326, #31925, #81223, #4538, #91829, #66118, #22393 ),
 .UNSPECIFIED., .F., .F.,
 ( 4, 3, 3, 3, 4 ),
 ( -6.921059206559499799, -6.378283243919759649, -5.323661303994230209, -4.287854170524850517, -3.271576390819999958 ),
 .UNSPECIFIED. ) ;
#39688=CARTESIAN_POINT ( 'NONE',  ( 10.34831838578470098, 1409.274431628310140, 198.3247425477780155 ) ) ;
#39689=CARTESIAN_POINT ( 'NONE',  ( 18.52259794967000062, 1425.592554617246151, 225.5483412146120088 ) ) ;
#39691=CARTESIAN_POINT ( 'NONE',  ( -19.91456662359999896, 1485.663097783829926, 191.2402015274980158 ) ) ;
#39692=CARTESIAN_POINT ( 'NONE',  ( 11.76903984429999994, 1432.302179532869786, 150.8119321890980018 ) ) ;
#39693=TOROIDAL_SURFACE ( 'NONE', #61159, 25.96906897330000064, 0.5000000000000000000 ) ;
#39694=CARTESIAN_POINT ( 'NONE',  ( -3.615177284590409990, 1449.532947440919997, 184.9113150316539986 ) ) ;
#39697=CARTESIAN_POINT ( 'NONE',  ( -7.826748708962336210, 1427.837793894468859, 134.0999999980979851 ) ) ;
#39701=CARTESIAN_POINT ( 'NONE',  ( -20.23330171276339939, 1495.987187365530190, 190.7338839421090313 ) ) ;
#39704=CARTESIAN_POINT ( 'NONE',  ( -0.1904153588180000078, 1483.383698146929873, 181.9103537380979958 ) ) ;
#39706=CARTESIAN_POINT ( 'NONE',  ( -46.04570283003550202, 1440.250595516199837, 266.6772069938360232 ) ) ;
#39707=CARTESIAN_POINT ( 'NONE',  ( -19.80431309490000302, 1426.801393628430105, 224.9940485357979867 ) ) ;
#39708=CARTESIAN_POINT ( 'NONE',  ( -22.39107471859139764, 1501.813592682170110, 208.5249304223659976 ) ) ;
#39713=CARTESIAN_POINT ( 'NONE',  ( 3.897533513563200103, 1407.987765282759938, 221.8195319916089829 ) ) ;
#39714=CARTESIAN_POINT ( 'NONE',  ( -14.08841074084159928, 1436.255549608840056, 150.1863611090900008 ) ) ;
#39715=SURFACE_SIDE_STYLE ('',( #66042 ) ) ;
#39716=CARTESIAN_POINT ( 'NONE',  ( 2.977092784659999936, 1421.750417338729903, 122.8790358596979928 ) ) ;
#39719=CARTESIAN_POINT ( 'NONE',  ( 33.66409354169999801, 1434.352089750400182, 250.0355534229980492 ) ) ;
#39720=CARTESIAN_POINT ( 'NONE',  ( -27.66125109240000057, 1508.130528727329875, 205.7926023901279677 ) ) ;
#39721=CARTESIAN_POINT ( 'NONE',  ( 0.4840505593630000103, 1486.443749368729868, 181.8234518676980258 ) ) ;
#39722=CARTESIAN_POINT ( 'NONE',  ( -17.06941237829999736, 1409.674943312830010, 194.0661809782980072 ) ) ;
#39724=CARTESIAN_POINT ( 'NONE',  ( -21.29137176940000131, 1428.105725915830135, 225.2483481452979959 ) ) ;
#39726=CARTESIAN_POINT ( 'NONE',  ( -2.967187434369539911, 1452.809443918890111, 152.3758103778500015 ) ) ;
#39727=CARTESIAN_POINT ( 'NONE',  ( 27.44739306059999961, 1451.807595801730031, 135.7772701328979963 ) ) ;
#39728=ORIENTED_EDGE ( 'NONE', *, *, #52842, .T. ) ;
#39731=CARTESIAN_POINT ( 'NONE',  ( 16.34718949245090158, 1423.188823444010040, 228.3968466436469953 ) ) ;
#39732=CARTESIAN_POINT ( 'NONE',  ( 17.33645362950000290, 1414.996442546130083, 210.3925741896480304 ) ) ;
#39736=CARTESIAN_POINT ( 'NONE',  ( -22.87714078023959985, 1409.721603508060070, 209.3742144960980056 ) ) ;
#39738=CARTESIAN_POINT ( 'NONE',  ( -0.1620123092989999847, 1416.817366565030170, 227.3670020742980284 ) ) ;
#39740=CARTESIAN_POINT ( 'NONE',  ( -1.545769114060000060, 1507.641667498930019, 237.1363977266979930 ) ) ;
#39744=CARTESIAN_POINT ( 'NONE',  ( 43.12262697494430341, 1452.630018548870112, 266.2617581945530105 ) ) ;
#39745=ADVANCED_FACE ( 'NONE', ( #66249 ), #38921, .T. ) ;
#39746=CARTESIAN_POINT ( 'NONE',  ( -12.87305953236479894, 1416.529254608160045, 221.9220372573969939 ) ) ;
#39749=ORIENTED_EDGE ( 'NONE', *, *, #17863, .F. ) ;
#39751=EDGE_CURVE ( 'NONE', #99599, #52697, #30365, .T. ) ;
#39753=CARTESIAN_POINT ( 'NONE',  ( 13.48661114156805496, 1443.650664694040188, 188.0188052989198582 ) ) ;
#39754=ORIENTED_EDGE ( 'NONE', *, *, #17320, .F. ) ;
#39755=ORIENTED_EDGE ( 'NONE', *, *, #90583, .F. ) ;
#39759=EDGE_CURVE ( 'NONE', #23029, #97372, #83139, .T. ) ;
#39761=CARTESIAN_POINT ( 'NONE',  ( 2.865104109652619524, 1452.813008747159756, 152.3914803971919980 ) ) ;
#39764=CARTESIAN_POINT ( 'NONE',  ( 19.02174849391997924, 1456.743990138540767, 225.7168055990159985 ) ) ;
#39766=FACE_OUTER_BOUND ( 'NONE', #20039, .T. ) ;
#39767=CARTESIAN_POINT ( 'NONE',  ( -13.63839190360340048, 1434.968068183459991, 148.6805963842519986 ) ) ;
#39768=CARTESIAN_POINT ( 'NONE',  ( 16.06975285769999928, 1489.474306033529956, 194.0919983873980073 ) ) ;
#39770=CARTESIAN_POINT ( 'NONE',  ( -24.04775057459589860, 1508.134858764150067, 222.3238671512500275 ) ) ;
#39771=CARTESIAN_POINT ( 'NONE',  ( 9.559188306630000298, 1428.004395111430085, 145.6094494780980142 ) ) ;
#39775=CARTESIAN_POINT ( 'NONE',  ( -3.274320305756030160E-16, 1450.913060387229962, 154.2476693630359819 ) ) ;
#39785=CARTESIAN_POINT ( 'NONE',  ( 11.92647681149999883, 1433.523782385620052, 150.2359986513980061 ) ) ;
#39786=CARTESIAN_POINT ( 'NONE',  ( 12.15345567070000143, 1468.554006627229910, 265.6112251771979800 ) ) ;
#39787=CARTESIAN_POINT ( 'NONE',  ( -22.86388144358860330, 1435.295931049460023, 134.1000000049170069 ) ) ;
#39792=CARTESIAN_POINT ( 'NONE',  ( 14.90141943649999945, 1419.765491606529849, 227.9873096972980022 ) ) ;
#39793=CARTESIAN_POINT ( 'NONE',  ( 0.5359454300520634096, 1410.309919237011854, 233.1502810298127883 ) ) ;
#39795=CARTESIAN_POINT ( 'NONE',  ( -18.08242730619999605, 1410.468575122029733, 224.5973926771980018 ) ) ;
#39799=CARTESIAN_POINT ( 'NONE',  ( -17.13435691658580140, 1410.007868545600104, 192.3884277009809978 ) ) ;
#39802=CARTESIAN_POINT ( 'NONE',  ( -10.96946876072200006, 1432.347663854339999, 151.7701362700559855 ) ) ;
#39803=CARTESIAN_POINT ( 'NONE',  ( -8.469419501860000921, 1416.216252248530054, 225.1067773946980139 ) ) ;
#39804=CARTESIAN_POINT ( 'NONE',  ( 0.2169929020791310226, 1453.438874170419922, 183.2345656878090097 ) ) ;
#39805=CARTESIAN_POINT ( 'NONE',  ( -9.740725139009999367, 1409.193360974830057, 198.3895369463979819 ) ) ;
#39806=CARTESIAN_POINT ( 'NONE',  ( -12.18581598819999989, 1415.088016306429836, 197.3189424682980189 ) ) ;
#39807=CARTESIAN_POINT ( 'NONE',  ( -28.44549777152819914, 1509.607982451979979, 211.0864871972310084 ) ) ;
#39808=CARTESIAN_POINT ( 'NONE',  ( 13.50119150350000119, 1434.968975554210147, 147.9458048916980033 ) ) ;
#39809=CARTESIAN_POINT ( 'NONE',  ( -35.52558520677190046, 1435.900183204640143, 134.0999999974749812 ) ) ;
#39810=CARTESIAN_POINT ( 'NONE',  ( 8.765894577279999211, 1440.430470941899785, 186.4520186125980103 ) ) ;
#39811=ORIENTED_EDGE ( 'NONE', *, *, #109532, .T. ) ;
#39816=CARTESIAN_POINT ( 'NONE',  ( -1.033934541210000058, 1452.678099303230056, 183.5143811305979966 ) ) ;
#39819=CARTESIAN_POINT ( 'NONE',  ( -19.90347714819266400, 1504.417445143046052, 189.0711003657198148 ) ) ;
#39821=CARTESIAN_POINT ( 'NONE',  ( 2.500000000000000000, 1425.929641631630147, 183.3886485112979869 ) ) ;
#39825=CARTESIAN_POINT ( 'NONE',  ( -28.53735979761090036, 1509.098833409579811, 208.7800982448970046 ) ) ;
#39826=CARTESIAN_POINT ( 'NONE',  ( -15.81239850789610202, 1409.465374018880084, 225.3821397894910206 ) ) ;
#39834=CARTESIAN_POINT ( 'NONE',  ( 0.2860585402580000380, 1466.760278681229920, 235.6133694232979963 ) ) ;
#39835=CARTESIAN_POINT ( 'NONE',  ( 20.46412024869999868, 1410.988662584130225, 219.2699858747980102 ) ) ;
#39836=CARTESIAN_POINT ( 'NONE',  ( -2.418217451635309878, 1419.517398164420001, 186.0902754504199947 ) ) ;
#39838=CARTESIAN_POINT ( 'NONE',  ( -16.07129795299999842, 1423.037556925630042, 229.0666284455979849 ) ) ;
#39841=CARTESIAN_POINT ( 'NONE',  ( 24.98278806157259879, 1430.498769693610029, 208.7705283626380037 ) ) ;
#39843=CARTESIAN_POINT ( 'NONE',  ( 10.22570915140000025, 1431.113060387329824, 225.5143498067979806 ) ) ;
#39844=CARTESIAN_POINT ( 'NONE',  ( -23.45859897689999940, 1430.822343046630067, 211.7813861080580011 ) ) ;
#39846=ADVANCED_FACE ( 'NONE', ( #53295 ), #82136, .F. ) ;
#39851=CARTESIAN_POINT ( 'NONE',  ( -4.221362096953909848, 1441.596168439879875, 170.5366494805969921 ) ) ;
#39853=ORIENTED_EDGE ( 'NONE', *, *, #36136, .F. ) ;
#39856=EDGE_LOOP ( 'NONE', ( #58781, #8908, #62370, #77585, #9239 ) ) ;
#39859=CARTESIAN_POINT ( 'NONE',  ( -11.63960718312326748, 1425.863102008939904, 144.3731951731623440 ) ) ;
#39860=CARTESIAN_POINT ( 'NONE',  ( 15.94106684230400184, 1410.432583999669760, 191.5989877904739842 ) ) ;
#39866=CARTESIAN_POINT ( 'NONE',  ( 34.54825073197359586, 1451.683981886209949, 134.0999999981819713 ) ) ;
#39867=DIRECTION ( 'NONE',  ( 0.3363363969979660806, 0.9417419115949053898, 0.000000000000000000 ) ) ;
#39870=CARTESIAN_POINT ( 'NONE',  ( -3.666694481987490040, 1509.114858341099989, 179.5219341129400163 ) ) ;
#39873=CARTESIAN_POINT ( 'NONE',  ( 5.485270235611575451, 1410.482254480975371, 231.1776710310072644 ) ) ;
#39876=CARTESIAN_POINT ( 'NONE',  ( 0.1718821611349999889, 1452.986277132529949, 183.2483320761980110 ) ) ;
#39878=CARTESIAN_POINT ( 'NONE',  ( -2.500000000000000000, 1439.624608411989811, 169.5728731851750126 ) ) ;
#39880=CARTESIAN_POINT ( 'NONE',  ( 33.91369111058539687, 1451.728768197430099, 135.0591089875200055 ) ) ;
#39882=EDGE_CURVE ( 'NONE', #110373, #5142, #16914, .T. ) ;
#39883=CARTESIAN_POINT ( 'NONE',  ( 26.05603448480000139, 1437.546877748950010, 137.0232845100980228 ) ) ;
#39884=CARTESIAN_POINT ( 'NONE',  ( 12.13987719790000064, 1415.426210663629945, 196.5375171025980023 ) ) ;
#39890=CARTESIAN_POINT ( 'NONE',  ( 39.99774708740250162, 1440.913060387330006, 267.3729947719869529 ) ) ;
#39891=CARTESIAN_POINT ( 'NONE',  ( -0.0002224978450532523575, 1452.169907037069606, 153.8711149815915462 ) ) ;
#39893=CARTESIAN_POINT ( 'NONE',  ( -0.01304300853801059965, 1452.999749671699874, 183.2385070597169943 ) ) ;
#39897=CARTESIAN_POINT ( 'NONE',  ( -12.79518584150000038, 1426.055539333530078, 222.4327048618980029 ) ) ;
#39898=CARTESIAN_POINT ( 'NONE',  ( -20.32975018110188259, 1508.870389951621746, 229.0186712996133735 ) ) ;
#39899=CARTESIAN_POINT ( 'NONE',  ( 45.48702082709758798, 1436.948629695928048, 266.1936686269212942 ) ) ;
#39903=CARTESIAN_POINT ( 'NONE',  ( 12.71492891619999988, 1463.042985206030153, 231.2054259453979910 ) ) ;
#39904=CARTESIAN_POINT ( 'NONE',  ( -23.54657453824519919, 1420.952714651539964, 210.9134052879049648 ) ) ;
#39905=DIRECTION ( 'NONE',  ( 0.000000000000000000, -0.9990482215818579093, -0.04361938736533144123 ) ) ;
#39908=EDGE_CURVE ( 'NONE', #110254, #54705, #93822, .T. ) ;
#39911=CARTESIAN_POINT ( 'NONE',  ( 17.43217232700621722, 1448.245005021945417, 217.7414174091619259 ) ) ;
#39913=CARTESIAN_POINT ( 'NONE',  ( 18.64061438810000126, 1509.327891197830013, 187.7640544359979913 ) ) ;
#39915=CARTESIAN_POINT ( 'NONE',  ( -11.60004869884502732, 1425.372347710274653, 138.1236363301591439 ) ) ;
#39917=ORIENTED_EDGE ( 'NONE', *, *, #26110, .F. ) ;
#39919=CARTESIAN_POINT ( 'NONE',  ( 25.66618467929999881, 1444.303020621219957, 221.6515381826980047 ) ) ;
#39920=CARTESIAN_POINT ( 'NONE',  ( -11.84270513390000090, 1430.621905942929970, 150.1494318102980117 ) ) ;
#39923=CARTESIAN_POINT ( 'NONE',  ( -5.329063471891149685E-15, 1428.868807534159941, 155.3340205489109849 ) ) ;
#39926=CARTESIAN_POINT ( 'NONE',  ( 12.84295322920000082, 1444.979964823190130, 186.6187016747979897 ) ) ;
#39927=CARTESIAN_POINT ( 'NONE',  ( -18.38271312340000208, 1444.809750369289759, 226.8202415501980056 ) ) ;
#39929=CARTESIAN_POINT ( 'NONE',  ( -2.496620389599999879, 1485.857485423129901, 182.3495326893979893 ) ) ;
#39932=CARTESIAN_POINT ( 'NONE',  ( 9.769670128800001407, 1407.519369601530116, 269.6204844436979897 ) ) ;
#39933=EDGE_CURVE ( 'NONE', #81697, #9577, #45074, .T. ) ;
#39934=CARTESIAN_POINT ( 'NONE',  ( 0.5238745688090000741, 1409.870337461830104, 185.0929766115979760 ) ) ;
#39935=CARTESIAN_POINT ( 'NONE',  ( 17.66554091740000132, 1410.882309102730005, 192.9158045799980243 ) ) ;
#39936=CARTESIAN_POINT ( 'NONE',  ( 21.71754518174779491, 1429.404468804660610, 218.5691086971039283 ) ) ;
#39937=CARTESIAN_POINT ( 'NONE',  ( 15.82489611782290240, 1509.465677942714137, 184.1612054350828203 ) ) ;
#39938=CARTESIAN_POINT ( 'NONE',  ( -0.5021741993441900531, 1413.729074630699870, 233.3179678917850026 ) ) ;
#39940=CARTESIAN_POINT ( 'NONE',  ( -2.307020840992839883, 1449.832034867059974, 154.5197370804639831 ) ) ;
#39941=CARTESIAN_POINT ( 'NONE',  ( -12.42428048090000026, 1445.297595047380128, 186.7045969743979867 ) ) ;
#39942=CARTESIAN_POINT ( 'NONE',  ( 1.462738438227520144, 1450.687750484019944, 155.0630772167459952 ) ) ;
#39943=CARTESIAN_POINT ( 'NONE',  ( -14.20217057992160115, 1415.778512723650010, 221.1297441146029712 ) ) ;
#39945=CARTESIAN_POINT ( 'NONE',  ( -7.991890656415680638, 1409.192143358779958, 196.4723718539459867 ) ) ;
#39946=CARTESIAN_POINT ( 'NONE',  ( 10.72994439777698439, 1424.980258667470935, 138.6335552007459455 ) ) ;
#39947=CARTESIAN_POINT ( 'NONE',  ( 3.696739103780000146, 1440.987872693469853, 157.0266763811980013 ) ) ;
#39948=CARTESIAN_POINT ( 'NONE',  ( -4.933848679039999574, 1475.129223611229918, 269.4903295208979443 ) ) ;
#39949=CARTESIAN_POINT ( 'NONE',  ( -4.235648567922631003, 1446.341758401669949, 163.6974501593520017 ) ) ;
#39951=CARTESIAN_POINT ( 'NONE',  ( -14.91306988694542923, 1486.499853230188137, 185.9738472613629199 ) ) ;
#39954=CARTESIAN_POINT ( 'NONE',  ( -17.60627216660330063, 1410.895669502700230, 193.4350316886979897 ) ) ;
#39957=CARTESIAN_POINT ( 'NONE',  ( 25.78167222729700114, 1509.813387082529971, 195.1140727163279962 ) ) ;
#39958=CARTESIAN_POINT ( 'NONE',  ( -19.22980863180000100, 1409.584580101929987, 199.6886479387179918 ) ) ;
#39959=CARTESIAN_POINT ( 'NONE',  ( 2.500000000000000000, 1448.210448409899982, 182.3842139592889851 ) ) ;
#39962=CARTESIAN_POINT ( 'NONE',  ( -2.297865873822824145, 1410.371582420674713, 232.7246199332096239 ) ) ;
#39965=CARTESIAN_POINT ( 'NONE',  ( 11.72669663920000005, 1426.286371213729808, 143.4670320514979949 ) ) ;
#39968=CARTESIAN_POINT ( 'NONE',  ( 10.94233749380000020, 1409.295175233830150, 190.2941314834980062 ) ) ;
#39974=CARTESIAN_POINT ( 'NONE',  ( -14.94707557629999961, 1464.413060387330006, 223.3779789887979916 ) ) ;
#39978=CARTESIAN_POINT ( 'NONE',  ( 20.00897032557049826, 1508.357423559000154, 229.1242640148969940 ) ) ;
#39980=VERTEX_POINT ( 'NONE', #73387 ) ;
#39981=ORIENTED_EDGE ( 'NONE', *, *, #55052, .F. ) ;
#39982=CARTESIAN_POINT ( 'NONE',  ( -12.38667194039999941, 1397.378208682429886, 212.8773238670779904 ) ) ;
#39983=CARTESIAN_POINT ( 'NONE',  ( -21.12354134859999988, 1409.814880802030075, 216.2513170893979861 ) ) ;
#39984=ORIENTED_EDGE ( 'NONE', *, *, #28880, .F. ) ;
#39985=CARTESIAN_POINT ( 'NONE',  ( -12.64444544987818020, 1445.030967319847377, 169.4649881375822247 ) ) ;
#39986=CARTESIAN_POINT ( 'NONE',  ( 22.47005530878909241, 1509.697731202374825, 228.0526691234717873 ) ) ;
#39991=CARTESIAN_POINT ( 'NONE',  ( 9.052748310100000140, 1449.229322941700048, 186.1672263551980109 ) ) ;
#39993=CARTESIAN_POINT ( 'NONE',  ( 44.70565337623089874, 1440.913053082580063, 269.9105772721819676 ) ) ;
#39994=CARTESIAN_POINT ( 'NONE',  ( 11.04255400179049929, 1396.298674870250125, 209.9401464633739920 ) ) ;
#39995=CARTESIAN_POINT ( 'NONE',  ( 14.36283523568019937, 1416.196255300799976, 196.9494022668550031 ) ) ;
#39996=CARTESIAN_POINT ( 'NONE',  ( 11.83663831039999970, 1430.188662621430012, 150.0176914616980071 ) ) ;
#39997=CARTESIAN_POINT ( 'NONE',  ( 6.917574163163576095, 1509.156500478879025, 180.5619989194156005 ) ) ;
#39999=CARTESIAN_POINT ( 'NONE',  ( 13.00321027915850003, 1435.856774820759711, 150.7051697245010189 ) ) ;
#40001=ORIENTED_EDGE ( 'NONE', *, *, #16691, .F. ) ;
#40004=CARTESIAN_POINT ( 'NONE',  ( -15.42294715779999947, 1459.506347036930038, 230.2271999085980099 ) ) ;
#40009=ORIENTED_EDGE ( 'NONE', *, *, #34584, .F. ) ;
#40011=CARTESIAN_POINT ( 'NONE',  ( 2.500000000000000000, 1448.563435859630090, 159.6568317789180185 ) ) ;
#40018=CARTESIAN_POINT ( 'NONE',  ( -19.01751557161993134, 1413.711985803739708, 269.3842094040881534 ) ) ;
#40020=EDGE_CURVE ( 'NONE', #72991, #80364, #106393, .T. ) ;
#40021=CARTESIAN_POINT ( 'NONE',  ( 0.2033579075311599815, 1416.218865267220053, 227.1056941053959974 ) ) ;
#40023=CARTESIAN_POINT ( 'NONE',  ( 24.65284846710000011, 1440.998862877870124, 212.5088464049680113 ) ) ;
#40024=CARTESIAN_POINT ( 'NONE',  ( -32.33429779520879777, 1440.913060389619886, 244.9699471617589950 ) ) ;
#40026=FACE_OUTER_BOUND ( 'NONE', #102767, .T. ) ;
#40028=CARTESIAN_POINT ( 'NONE',  ( 14.76285304363459794, 1412.136382785999785, 269.6387137786039716 ) ) ;
#40031=CARTESIAN_POINT ( 'NONE',  ( 23.94662184079999889, 1410.398902072829969, 209.3165411815660093 ) ) ;
#40032=CARTESIAN_POINT ( 'NONE',  ( 0.02095502431091895990, 1507.112669616160019, 237.3523204869388792 ) ) ;
#40034=CARTESIAN_POINT ( 'NONE',  ( -11.60004869885203682, 1425.456763142306272, 136.9372401164825703 ) ) ;
#40037=CARTESIAN_POINT ( 'NONE',  ( 15.09682228229999978, 1409.610690924630035, 192.0685155598980032 ) ) ;
#40042=CARTESIAN_POINT ( 'NONE',  ( 17.60627508980000044, 1410.895669370830092, 224.8086596393980017 ) ) ;
#40048=CARTESIAN_POINT ( 'NONE',  ( -11.87823649874709986, 1433.207008023099888, 147.6493504979379736 ) ) ;
#40052=CARTESIAN_POINT ( 'NONE',  ( -27.01380866140000236, 1450.681584507220123, 136.4483241423979791 ) ) ;
#40056=EDGE_CURVE ( 'NONE', #11858, #44698, #100413, .T. ) ;
#40058=ORIENTED_EDGE ( 'NONE', *, *, #16119, .F. ) ;
#40059=CARTESIAN_POINT ( 'NONE',  ( 0.2288628776169999990, 1457.825816290129751, 228.9826145029980182 ) ) ;
#40061=CARTESIAN_POINT ( 'NONE',  ( 23.90525189569999753, 1446.959187819619956, 216.4132176579479960 ) ) ;
#40062=CARTESIAN_POINT ( 'NONE',  ( 8.952338953416104417, 1437.015053605790399, 153.1552784082401786 ) ) ;
#40066=CARTESIAN_POINT ( 'NONE',  ( 15.23801107490102247, 1420.745564912765531, 227.8424191170523443 ) ) ;
#40067=CARTESIAN_POINT ( 'NONE',  ( 6.251976625090000184, 1423.636347555029943, 186.2373219085980054 ) ) ;
#40068=CARTESIAN_POINT ( 'NONE',  ( -18.82070097289999921, 1425.548023863429989, 224.8286763900980247 ) ) ;
#40071=CARTESIAN_POINT ( 'NONE',  ( 17.47858465850000087, 1445.355796517389990, 190.5483357571979752 ) ) ;
#40073=CARTESIAN_POINT ( 'NONE',  ( -29.82992791574873337, 1462.373732266217303, 269.4690031617170121 ) ) ;
#40074=ORIENTED_EDGE ( 'NONE', *, *, #105782, .F. ) ;
#40076=CARTESIAN_POINT ( 'NONE',  ( -39.43000968072596635, 1423.549647405266114, 269.1442499132564876 ) ) ;
#40079=CARTESIAN_POINT ( 'NONE',  ( -0.1544391217869999777, 1417.354636897429828, 235.2106466983979942 ) ) ;
#40080=CARTESIAN_POINT ( 'NONE',  ( -12.88287017495675180, 1442.882806527179127, 186.3955768649811944 ) ) ;
#40082=CARTESIAN_POINT ( 'NONE',  ( 4.500000000000000000, 1425.929641636930000, 183.3886486283980162 ) ) ;
#40084=CARTESIAN_POINT ( 'NONE',  ( -2.372055168030982930, 1415.656490859390487, 232.9357013292204215 ) ) ;
#40086=CARTESIAN_POINT ( 'NONE',  ( 18.80464302510000252, 1425.801049065629968, 225.6039134470979945 ) ) ;
#40087=CARTESIAN_POINT ( 'NONE',  ( -12.77015161775204177, 1442.833871923525749, 169.4527266999588733 ) ) ;
#40088=CARTESIAN_POINT ( 'NONE',  ( -15.09681984919999920, 1409.610690840030202, 226.1751760239980058 ) ) ;
#40089=ORIENTED_EDGE ( 'NONE', *, *, #23541, .F. ) ;
#40094=CARTESIAN_POINT ( 'NONE',  ( 16.67301258007090325, 1414.971349104640012, 208.8753071508930077 ) ) ;
#40099=CARTESIAN_POINT ( 'NONE',  ( -11.87899302940000013, 1433.117272603449919, 149.9761280929979819 ) ) ;
#40101=CARTESIAN_POINT ( 'NONE',  ( 17.41346973679999977, 1410.020394403929913, 224.1775087769979962 ) ) ;
#40102=CARTESIAN_POINT ( 'NONE',  ( -25.85694180069999959, 1436.522598591890073, 136.9096217434980360 ) ) ;
#40103=CARTESIAN_POINT ( 'NONE',  ( -14.68424190075857894, 1429.954736308614429, 222.0400034816578057 ) ) ;
#40105=CARTESIAN_POINT ( 'NONE',  ( 1.324218434260000077, 1452.129555781629961, 183.4093038337979920 ) ) ;
#40107=CARTESIAN_POINT ( 'NONE',  ( -20.41791317763336622, 1509.743963675110081, 231.1018990513161668 ) ) ;
#40108=CARTESIAN_POINT ( 'NONE',  ( -1.656929189209940043E-09, 1413.545274745300048, 249.1207792992729821 ) ) ;
#40109=EDGE_LOOP ( 'NONE', ( #106403, #70070, #86429, #53246 ) ) ;
#40111=CARTESIAN_POINT ( 'NONE',  ( -11.85755111573270071, 1431.739894570919887, 149.9497684120179883 ) ) ;
#40113=CARTESIAN_POINT ( 'NONE',  ( -7.240565274249999739, 1470.982841272730184, 269.3413375565979777 ) ) ;
#40116=FACE_OUTER_BOUND ( 'NONE', #948, .T. ) ;
#40117=CARTESIAN_POINT ( 'NONE',  ( 0.2487136076107180072, 1451.379526256489953, 182.5560867144160113 ) ) ;
#40122=CARTESIAN_POINT ( 'NONE',  ( -39.51545107973109339, 1423.010726206650133, 266.3651880554039622 ) ) ;
#40127=VECTOR ( 'NONE', #107494, 1000.000000000000000 ) ;
#40132=CARTESIAN_POINT ( 'NONE',  ( -2.500000000000000000, 1434.141256042250006, 183.7754221751980026 ) ) ;
#40135=CARTESIAN_POINT ( 'NONE',  ( -16.72084742370000043, 1440.439203200979819, 190.3227648696979770 ) ) ;
#40137=CARTESIAN_POINT ( 'NONE',  ( -2.129012891770579508, 1450.054690635432507, 182.8874644828513283 ) ) ;
#40140=CARTESIAN_POINT ( 'NONE',  ( -26.21200917470000036, 1435.609253055569980, 136.1127715238980045 ) ) ;
#40145=CARTESIAN_POINT ( 'NONE',  ( 45.63712937690380755, 1440.913060387330006, 268.9747523971630017 ) ) ;
#40146=CARTESIAN_POINT ( 'NONE',  ( 0.06764684832619999311, 1408.848989329930191, 194.7501694690980116 ) ) ;
#40148=CARTESIAN_POINT ( 'NONE',  ( -3.586209743369999980, 1396.221085749330086, 197.6373087627979714 ) ) ;
#40160=CARTESIAN_POINT ( 'NONE',  ( 5.436747755899999923, 1437.112761795790220, 154.7095357218980212 ) ) ;
#40161=EDGE_CURVE ( 'NONE', #83258, #1325, #4113, .T. ) ;
#40162=CARTESIAN_POINT ( 'NONE',  ( -14.76761537580000017, 1430.144808017329979, 221.9970169696979667 ) ) ;
#40163=CARTESIAN_POINT ( 'NONE',  ( 18.80463395749418609, 1425.801070877558004, 225.6039093632070376 ) ) ;
#40168=CARTESIAN_POINT ( 'NONE',  ( -11.15268071913589942, 1425.700850061899928, 101.7510819996820004 ) ) ;
#40170=CARTESIAN_POINT ( 'NONE',  ( -19.36207330082412881, 1457.403296974644263, 226.2910419354238343 ) ) ;
#40173=CARTESIAN_POINT ( 'NONE',  ( -24.41826286173580840, 1509.769384798847341, 225.6085766216700677 ) ) ;
#40175=CARTESIAN_POINT ( 'NONE',  ( -4.141637188104014378, 1439.809767520328933, 185.4878219303663229 ) ) ;
#40177=CARTESIAN_POINT ( 'NONE',  ( 11.58478124470000026, 1415.063410489829948, 222.3466023727980030 ) ) ;
#40178=CARTESIAN_POINT ( 'NONE',  ( 1.530052826864370052, 1452.704406626560058, 183.4894965714629791 ) ) ;
#40180=CARTESIAN_POINT ( 'NONE',  ( 24.29980230545161746, 1445.714648955952498, 214.3234337815786716 ) ) ;
#40184=ORIENTED_EDGE ( 'NONE', *, *, #94649, .F. ) ;
#40186=DIRECTION ( 'NONE',  ( 0.9995237695669298983, 0.03085829012780005876, 1.050424002118616340E-06 ) ) ;
#40188=CARTESIAN_POINT ( 'NONE',  ( 1.132427485120000064E-14, 1421.588970873729977, 90.97065375769790307 ) ) ;
#40191=CARTESIAN_POINT ( 'NONE',  ( -0.04898095367366699787, 1508.952069630370033, 179.4017721621569876 ) ) ;
#40194=CARTESIAN_POINT ( 'NONE',  ( 18.02093535799999913, 1424.326836137830014, 225.1991050518980160 ) ) ;
#40196=CARTESIAN_POINT ( 'NONE',  ( 5.157704406284129827E-09, 1406.911841301380036, 222.1218459627310153 ) ) ;
#40197=CARTESIAN_POINT ( 'NONE',  ( 34.82401208279389948, 1440.913060385709969, 250.5797988201090050 ) ) ;
#40200=CARTESIAN_POINT ( 'NONE',  ( 12.93261679809999976, 1416.825245919230156, 221.7399671197980240 ) ) ;
#40203=AXIS2_PLACEMENT_3D ( 'NONE', #97317, #9453, #20587 ) ;
#40205=CARTESIAN_POINT ( 'NONE',  ( -1.514738108749209999, 1507.606285622480073, 232.0384771855580084 ) ) ;
#40208=CARTESIAN_POINT ( 'NONE',  ( -13.01671764799590036, 1416.842625005220043, 221.9093393807470136 ) ) ;
#40211=CARTESIAN_POINT ( 'NONE',  ( -17.52327301342160126, 1415.836208884639973, 225.9446061863119724 ) ) ;
#40214=CARTESIAN_POINT ( 'NONE',  ( -15.93370838064100248, 1491.571823434650014, 224.2164500899540087 ) ) ;
#40215=CARTESIAN_POINT ( 'NONE',  ( -251.6678281593879944, 1855.626960278319984, 173.9672998193020135 ) ) ;
#40219=ORIENTED_EDGE ( 'NONE', *, *, #31563, .F. ) ;
#40220=CARTESIAN_POINT ( 'NONE',  ( -1.304523669740000225, 1451.773061479729904, 183.6942222515980063 ) ) ;
#40224=ORIENTED_EDGE ( 'NONE', *, *, #33002, .T. ) ;
#40227=CARTESIAN_POINT ( 'NONE',  ( -11.63679813930000151, 1439.363771630820111, 147.7934734181980048 ) ) ;
#40228=CARTESIAN_POINT ( 'NONE',  ( 11.89193436271280113, 1434.276600485830159, 147.6498533937430011 ) ) ;
#40233=DIRECTION ( 'NONE',  ( 0.000000000000000000, 0.000000000000000000, 1.000000000000000000 ) ) ;
#40234=CARTESIAN_POINT ( 'NONE',  ( 18.28846457996500163, 1425.324642923450028, 225.4724497386589803 ) ) ;
#40237=CARTESIAN_POINT ( 'NONE',  ( 10.96941897920000031, 1432.344069363209883, 151.7701285250979879 ) ) ;
#40238=CARTESIAN_POINT ( 'NONE',  ( -2.545475536568049701, 1449.267405237600087, 183.6438597093680016 ) ) ;
#40239=EDGE_LOOP ( 'NONE', ( #1766, #82991, #108841, #46116 ) ) ;
#40241=CARTESIAN_POINT ( 'NONE',  ( 2.512783080302469774, 1509.132906964770200, 239.1218459480490139 ) ) ;
#40242=CARTESIAN_POINT ( 'NONE',  ( 19.07243531070609777, 1456.493896479490104, 226.7047778378099849 ) ) ;
#40244=CARTESIAN_POINT ( 'NONE',  ( -12.12002620680000042, 1433.961363555340085, 150.1912452130979716 ) ) ;
#40245=CARTESIAN_POINT ( 'NONE',  ( 8.296490667357130383E-11, 1466.080307989299854, 241.7690657028170165 ) ) ;
#40246=CARTESIAN_POINT ( 'NONE',  ( -20.25904020392970040, 1496.820878093550164, 190.7097365830209981 ) ) ;
#40248=DIRECTION ( 'NONE',  ( -0.6906235817280228506, 0.2466512791305629781, 0.6798545541984799545 ) ) ;
#40249=CIRCLE ( 'NONE', #92129, 30.00000000000000000 ) ;
#40250=CARTESIAN_POINT ( 'NONE',  ( -0.5453392599249999861, 1476.674368370930097, 182.2373881275980239 ) ) ;
#40252=CARTESIAN_POINT ( 'NONE',  ( -46.16777166034429314, 1440.913065320969963, 266.9714496862470128 ) ) ;
#40254=CARTESIAN_POINT ( 'NONE',  ( -20.18543317628819977, 1451.730021516360011, 208.5438760233379867 ) ) ;
#40256=CARTESIAN_POINT ( 'NONE',  ( 6.244762012776079452, 1407.784308379980075, 220.5925233722940106 ) ) ;
#40258=B_SPLINE_SURFACE_WITH_KNOTS ( 'NONE', 5, 5, ( 
 ( #107897, #98395, #40146, #56967, #74329, #91099, #14377, #48570, #17671 ),
 ( #24429, #41797, #44022, #383, #84892, #69234, #51300, #94391, #16561 ),
 ( #85437, #8735, #67028, #101683, #59179, #24973, #7643, #76505, #75957 ),
 ( #25530, #78158, #42918, #103343, #17112, #26645, #43472, #77617, #33946 ),
 ( #51873, #77074, #110109, #93299, #33381, #102787, #60843, #59720, #101135 ),
 ( #86009, #60273, #34504, #50755, #8184, #929, #1470, #93840, #84352 ) ),
 .UNSPECIFIED., .F., .F., .F.,
 ( 6, 6 ),
 ( 6, 3, 6 ),
 ( 52.45005585730000064, 62.38124646570000209 ),
 ( 0.000000000000000000, 1.000000000000000000, 2.000000000000000000 ),
 .UNSPECIFIED. ) ;
#40261=ORIENTED_EDGE ( 'NONE', *, *, #104271, .T. ) ;
#40262=CARTESIAN_POINT ( 'NONE',  ( 39.40331993399999533, 1435.955742673169880, 259.1105269787980205 ) ) ;
#40263=CARTESIAN_POINT ( 'NONE',  ( -27.70206559600000062, 1508.130759164429946, 205.9664600262279919 ) ) ;
#40264=CARTESIAN_POINT ( 'NONE',  ( -0.5320368101529999727, 1499.383640133830113, 181.1599537584980055 ) ) ;
#40265=CARTESIAN_POINT ( 'NONE',  ( 4.363122647530000009, 1432.413060387330006, 146.1721969590979882 ) ) ;
#40267=CARTESIAN_POINT ( 'NONE',  ( -18.28167441760000145, 1423.284962468630056, 231.7606941460979897 ) ) ;
#40269=CARTESIAN_POINT ( 'NONE',  ( -21.70213619864250276, 1452.155205091640028, 140.9573533261639966 ) ) ;
#40271=CARTESIAN_POINT ( 'NONE',  ( -5.360340255521029995, 1422.242729809129969, 144.1582390553999744 ) ) ;
#40276=ORIENTED_EDGE ( 'NONE', *, *, #16149, .F. ) ;
#40278=CARTESIAN_POINT ( 'NONE',  ( -23.90704851129999753, 1410.421101986430131, 209.5356727241129988 ) ) ;
#40279=ORIENTED_EDGE ( 'NONE', *, *, #56320, .F. ) ;
#40283=CARTESIAN_POINT ( 'NONE',  ( -22.25208704810000171, 1415.845517319630062, 214.9433210100679901 ) ) ;
#40284=ORIENTED_EDGE ( 'NONE', *, *, #29579, .T. ) ;
#40286=CARTESIAN_POINT ( 'NONE',  ( 45.19053312608840400, 1446.052362190220265, 268.9873881031790006 ) ) ;
#40289=CARTESIAN_POINT ( 'NONE',  ( -0.02608006148170000094, 1419.743832528429948, 184.3822973806979917 ) ) ;
#40292=CARTESIAN_POINT ( 'NONE',  ( 12.53380745427929988, 1442.773887455719887, 186.4115735415020083 ) ) ;
#40294=CARTESIAN_POINT ( 'NONE',  ( 12.96698787743724424, 1442.929322678499602, 187.1422095272347121 ) ) ;
#40297=CARTESIAN_POINT ( 'NONE',  ( 3.932773640260000203, 1448.980696606500032, 184.2693352687979882 ) ) ;
#40298=CARTESIAN_POINT ( 'NONE',  ( 26.83637367288270070, 1451.055154343129971, 136.3626532266509628 ) ) ;
#40301=CARTESIAN_POINT ( 'NONE',  ( 3.605245751538479926, 1452.787162431489833, 152.2996838318599941 ) ) ;
#40306=CARTESIAN_POINT ( 'NONE',  ( 2.902343876856320115, 1466.632250330839952, 234.1422825383600070 ) ) ;
#40307=CARTESIAN_POINT ( 'NONE',  ( -16.69647987924599875, 1411.957873142359858, 191.7070286008739970 ) ) ;
#40309=CARTESIAN_POINT ( 'NONE',  ( 2.801329332423560636, 1440.706061933215551, 170.5311005724319955 ) ) ;
#40310=CARTESIAN_POINT ( 'NONE',  ( -24.03880222912709996, 1508.063415561920237, 222.3187217912339975 ) ) ;
#40311=CARTESIAN_POINT ( 'NONE',  ( 0.1681681984982243971, 1405.973120458232188, 137.0999999980979851 ) ) ;
#40313=CARTESIAN_POINT ( 'NONE',  ( 9.562842933049999772, 1427.428384358229778, 219.6133831119979902 ) ) ;
#40314=CARTESIAN_POINT ( 'NONE',  ( 3.203789175851970288E-09, 1424.294192408320214, 227.6053815985079893 ) ) ;
#40320=ORIENTED_EDGE ( 'NONE', *, *, #25538, .T. ) ;
#40322=CARTESIAN_POINT ( 'NONE',  ( -1.650293394300000216, 1438.194204504490017, 150.5634062101979964 ) ) ;
#40326=CARTESIAN_POINT ( 'NONE',  ( 0.8608076301245028983, 1450.861566175740109, 181.3854559141449840 ) ) ;
#40328=CARTESIAN_POINT ( 'NONE',  ( 0.6301902189002333010, 1467.066691292220639, 235.5390148699710835 ) ) ;
#40330=CARTESIAN_POINT ( 'NONE',  ( 0.1681674884180490159, 1420.473121907760060, 182.7464979049940155 ) ) ;
#40331=CARTESIAN_POINT ( 'NONE',  ( 11.41285014610000026, 1422.099025052029901, 229.8069411653980012 ) ) ;
#40332=CARTESIAN_POINT ( 'NONE',  ( 13.02322703161950024, 1416.825784015089994, 221.6328457863429833 ) ) ;
#40334=CARTESIAN_POINT ( 'NONE',  ( -16.81208394469999945, 1409.500151295429987, 223.9875056278980026 ) ) ;
#40336=CARTESIAN_POINT ( 'NONE',  ( 27.69925877688100258, 1441.434395746940027, 137.3015763641899980 ) ) ;
#40337=CARTESIAN_POINT ( 'NONE',  ( -17.40901011393470199, 1410.017888045460040, 193.0747045748870221 ) ) ;
#40338=CARTESIAN_POINT ( 'NONE',  ( 1.192550336225690098E-06, 1408.657067415270149, 195.1347666596020076 ) ) ;
#40341=CARTESIAN_POINT ( 'NONE',  ( -1.160956870409999953, 1414.971439108430104, 226.6888194207980121 ) ) ;
#40342=CARTESIAN_POINT ( 'NONE',  ( 0.1701966656071439987, 1480.214123346120232, 182.0851929733079828 ) ) ;
#40344=ORIENTED_EDGE ( 'NONE', *, *, #55584, .T. ) ;
#40345=CARTESIAN_POINT ( 'NONE',  ( -24.49842486978874945, 1451.934881895486114, 137.2711189102183198 ) ) ;
#40347=CARTESIAN_POINT ( 'NONE',  ( 12.91297502169999944, 1434.774370803509782, 149.0259275850980032 ) ) ;
#40348=CARTESIAN_POINT ( 'NONE',  ( -40.21460569546650277, 1439.107902997820020, 134.0999999981339954 ) ) ;
#40349=CARTESIAN_POINT ( 'NONE',  ( 3.846235792629999928, 1440.870317293109792, 184.3772602386979997 ) ) ;
#40352=DIRECTION ( 'NONE',  ( 0.7071067802247986700, -0.01693885153322989556, 0.7069038666387766900 ) ) ;
#40355=CARTESIAN_POINT ( 'NONE',  ( 18.63567692469789705, 1430.070545818819937, 208.7560837280540227 ) ) ;
#40356=CARTESIAN_POINT ( 'NONE',  ( 36.28172795142912577, 1420.161297467323493, 269.2207334997069665 ) ) ;
#40357=CARTESIAN_POINT ( 'NONE',  ( 21.04915883790000208, 1471.323284331829882, 209.7080812325230283 ) ) ;
#40362=CARTESIAN_POINT ( 'NONE',  ( -26.81029715973576444, 1436.081135210529737, 136.5370857271699663 ) ) ;
#40364=CARTESIAN_POINT ( 'NONE',  ( -29.47598808667450143, 1509.906165461940191, 208.6054833806550164 ) ) ;
#40365=CARTESIAN_POINT ( 'NONE',  ( -16.01078298560119961, 1409.497709431180056, 225.5354710659109969 ) ) ;
#40372=CARTESIAN_POINT ( 'NONE',  ( 23.95042262499999808, 1509.749427575030040, 225.5182035443980055 ) ) ;
#40375=CARTESIAN_POINT ( 'NONE',  ( 0.8662027080590000150, 1465.087949259730067, 238.0466396433980094 ) ) ;
#40376=EDGE_CURVE ( 'NONE', #94371, #87953, #101144, .T. ) ;
#40377=CARTESIAN_POINT ( 'NONE',  ( 18.87422689890000171, 1410.495332323530192, 221.7757844262980029 ) ) ;
#40378=CARTESIAN_POINT ( 'NONE',  ( -2.189223485552659998, 1414.936483310510084, 186.1778520092960036 ) ) ;
#40379=ADVANCED_FACE ( 'NONE', ( #34820 ), #50538, .F. ) ;
#40380=CARTESIAN_POINT ( 'NONE',  ( -17.73407118999999810, 1423.343216095329808, 226.1884512641980223 ) ) ;
#40382=CARTESIAN_POINT ( 'NONE',  ( 24.05147185178290314, 1411.090383835510011, 208.4115470962599943 ) ) ;
#40384=CARTESIAN_POINT ( 'NONE',  ( 7.326859461719999800, 1453.313060387329870, 227.7771414719979930 ) ) ;
#40387=CARTESIAN_POINT ( 'NONE',  ( -5.490999923311999709, 1485.816407977019935, 182.9198330246910018 ) ) ;
#40389=CARTESIAN_POINT ( 'NONE',  ( -4.221515794169249602, 1441.604558287980126, 168.7334682647589830 ) ) ;
#40391=ORIENTED_EDGE ( 'NONE', *, *, #15820, .T. ) ;
#40395=CARTESIAN_POINT ( 'NONE',  ( 1.448679645196929933, 1507.129709964000085, 181.1126013477120011 ) ) ;
#40397=CARTESIAN_POINT ( 'NONE',  ( -21.30585458279999855, 1410.903636193130069, 200.5893642190180231 ) ) ;
#40398=CARTESIAN_POINT ( 'NONE',  ( 2.205156445730000137, 1428.435894572430016, 91.31218443469779800 ) ) ;
#40399=CARTESIAN_POINT ( 'NONE',  ( 16.42012968119449923, 1410.579620556590044, 191.6756617717020106 ) ) ;
#40401=CARTESIAN_POINT ( 'NONE',  ( 41.52362570818139886, 1442.051313831599828, 135.5055742887579981 ) ) ;
#40404=CARTESIAN_POINT ( 'NONE',  ( 11.47334203980808276, 1464.061491388687273, 231.7760070827772552 ) ) ;
#40409=CYLINDRICAL_SURFACE ( 'NONE', #9592, 1.436538049339996181 ) ;
#40411=DIRECTION ( 'NONE',  ( 0.000000000000000000, 0.000000000000000000, -1.000000000000000000 ) ) ;
#40415=CARTESIAN_POINT ( 'NONE',  ( -17.59268554400000184, 1410.455475221230017, 194.0661810319979850 ) ) ;
#40416=CARTESIAN_POINT ( 'NONE',  ( 0.02280772265270000071, 1450.912263924099989, 181.2411195727979702 ) ) ;
#40417=CARTESIAN_POINT ( 'NONE',  ( -3.236612797780000328, 1484.261208539930067, 183.3592960838980161 ) ) ;
#40420=B_SPLINE_CURVE_WITH_KNOTS ( 'NONE', 3,
 ( #78701, #42333, #2014, #77598 ),
 .UNSPECIFIED., .F., .F.,
 ( 4, 4 ),
 ( 0.000000000000000000, 1.000000000000000000 ),
 .UNSPECIFIED. ) ;
#40421=B_SPLINE_CURVE_WITH_KNOTS ( 'NONE', 3,
 ( #32275, #92720, #7073, #59153 ),
 .UNSPECIFIED., .F., .F.,
 ( 4, 4 ),
 ( -47.20273799956279959, -29.43575841650000058 ),
 .UNSPECIFIED. ) ;
#40423=CARTESIAN_POINT ( 'NONE',  ( 33.91369114129039986, 1435.681798693210112, 134.7402661674759941 ) ) ;
#40426=CARTESIAN_POINT ( 'NONE',  ( 33.98103710425687041, 1443.913060387329324, 154.9319925572100942 ) ) ;
#40428=ORIENTED_EDGE ( 'NONE', *, *, #33855, .F. ) ;
#40431=ORIENTED_EDGE ( 'NONE', *, *, #68566, .F. ) ;
#40432=CARTESIAN_POINT ( 'NONE',  ( 41.55687132039510345, 1440.913060387330006, 269.1110027756790259 ) ) ;
#40433=CARTESIAN_POINT ( 'NONE',  ( -0.0002577169993026165776, 1452.568168760216622, 153.5123052302506892 ) ) ;
#40435=CARTESIAN_POINT ( 'NONE',  ( -0.3202584381410000236, 1451.681415889429900, 183.0549383082980057 ) ) ;
#40436=ADVANCED_FACE ( 'NONE', ( #33705 ), #50019, .F. ) ;
#40437=CARTESIAN_POINT ( 'NONE',  ( -15.35486504390000029, 1409.449264088030077, 192.1003565319979884 ) ) ;
#40440=CARTESIAN_POINT ( 'NONE',  ( -4.474042835350000580, 1420.726059067829965, 186.3567251020980109 ) ) ;
#40442=CARTESIAN_POINT ( 'NONE',  ( 7.054183505060000137, 1406.398142208129912, 266.9413180379979735 ) ) ;
#40443=CARTESIAN_POINT ( 'NONE',  ( -12.06132760070000032, 1433.903324594730066, 147.1502524840979902 ) ) ;
#40444=CARTESIAN_POINT ( 'NONE',  ( 26.86204993032690069, 1508.007394616730153, 206.2315948942269870 ) ) ;
#40445=CARTESIAN_POINT ( 'NONE',  ( 16.31715900080000026, 1460.257358923430047, 229.2418418610980098 ) ) ;
#40446=CARTESIAN_POINT ( 'NONE',  ( -10.75958976553603819, 1424.480348114876506, 137.8583268508966739 ) ) ;
#40450=CARTESIAN_POINT ( 'NONE',  ( 20.50000000000000000, 1442.773887286369927, 169.0968414572980123 ) ) ;
#40451=CARTESIAN_POINT ( 'NONE',  ( -0.1001984567280549965, 1508.308975277190029, 180.4408595641159820 ) ) ;
#40454=B_SPLINE_CURVE_WITH_KNOTS ( 'NONE', 3,
 ( #10353, #101217, #86511, #109650, #61900, #16113, #96017 ),
 .UNSPECIFIED., .F., .F.,
 ( 4, 3, 4 ),
 ( -20.59614224704469976, -18.01294953900849904, -15.04010021667880004 ),
 .UNSPECIFIED. ) ;
#40458=EDGE_LOOP ( 'NONE', ( #101412, #105868, #74292, #27885, #38300, #59500 ) ) ;
#40462=CARTESIAN_POINT ( 'NONE',  ( -11.29829825160000034, 1432.080963479299953, 151.5184116568979960 ) ) ;
#40465=CARTESIAN_POINT ( 'NONE',  ( 6.305024129259999555, 1422.156209412130011, 144.1468801376980196 ) ) ;
#40466=B_SPLINE_CURVE_WITH_KNOTS ( 'NONE', 3,
 ( #103026, #59966, #52658, #25767, #35290, #95200, #17351, #93527, #94638, #34186, #84583, #75657, #8980, #61085, #34736, #69476, #52109, #50459, #41497, #26896, #110341, #18461, #109797, #7874, #42042, #26323, #25210, #17913, #33613, #67266, #7333, #67810, #77308, #94081, #101924, #43151, #51546, #102478, #33075, #76194, #59415, #606, #24648, #101358, #103596, #86239, #58850, #92982, #16796, #16256, #51000, #85131, #8418, #85683 ),
 .UNSPECIFIED., .F., .F.,
 ( 4, 2, 2, 1, 1, 1, 1, 1, 2, 2, 2, 2, 1, 1, 1, 1, 1, 2, 2, 2, 2, 1, 1, 1, 1, 1, 2, 2, 2, 2, 1, 1, 1, 2, 2, 4 ),
 ( 0.000000000000000000, 0.1250000000035015324, 0.1875000000052515492, 0.2187500000061264882, 0.2343750000065650818, 0.2421875000067657546, 0.2460937500068673678, 0.2480468750069194372, 0.2490234375069441952, 0.2500000000069689809, 0.3750000000063240524, 0.4375000000060016991, 0.4687500000058259508, 0.4843750000057260863, 0.4921875000056777916, 0.4960937500056679661, 0.4980468750056630256, 0.4990234375056590843, 0.5000000000056551430, 0.6250000000030080383, 0.6875000000016828761, 0.7187500000010204060, 0.7343750000006781242, 0.7421875000004977130, 0.7460937500003983480, 0.7480468750003566036, 0.7490234375003448353, 0.7500000000003329559, 0.8125000000003542722, 0.8437500000003754774, 0.8593750000003955725, 0.8671875000003966827, 0.8710937500003971268, 0.8730468750003963496, 0.8750000000003955725, 1.000000000000000000 ),
 .UNSPECIFIED. ) ;
#40467=DIRECTION ( 'NONE',  ( 0.000000000000000000, 1.000000000000000000, 0.000000000000000000 ) ) ;
#40468=CARTESIAN_POINT ( 'NONE',  ( 12.44069282309999913, 1446.394401557849960, 188.1775352768979701 ) ) ;
#40470=CARTESIAN_POINT ( 'NONE',  ( -20.21251411980000157, 1470.087779964230094, 225.9614712067979951 ) ) ;
#40475=CARTESIAN_POINT ( 'NONE',  ( 3.744464175900000136, 1406.377798150230092, 269.2893938024980116 ) ) ;
#40476=EDGE_CURVE ( 'NONE', #96461, #48130, #69066, .T. ) ;
#40477=CARTESIAN_POINT ( 'NONE',  ( 0.08329622130249998702, 1408.915969163729869, 186.0161422112979892 ) ) ;
#40478=DIRECTION ( 'NONE',  ( -0.1141463326676888657, -0.5076720045192847364, -0.8539553563072771469 ) ) ;
#40480=VECTOR ( 'NONE', #99015, 1000.000000000000114 ) ;
#40481=CARTESIAN_POINT ( 'NONE',  ( 22.78255286321940076, 1431.711273479132842, 216.5513474728326457 ) ) ;
#40483=CARTESIAN_POINT ( 'NONE',  ( 26.63183758487663155, 1507.995768146901355, 215.9641994103228058 ) ) ;
#40484=LINE ( 'NONE', #50554, #12092 ) ;
#40485=CARTESIAN_POINT ( 'NONE',  ( -1.174890917327530149, 1450.814461561099961, 154.7899053676320023 ) ) ;
#40486=CARTESIAN_POINT ( 'NONE',  ( -1.556661572576635955, 1451.024750845122753, 183.5973180285813271 ) ) ;
#40487=CARTESIAN_POINT ( 'NONE',  ( -17.49001816009999999, 1408.913060387329779, 212.4168409189479974 ) ) ;
#40490=CARTESIAN_POINT ( 'NONE',  ( -10.13264865422269878, 1409.266900275340049, 198.1207111944070220 ) ) ;
#40491=CARTESIAN_POINT ( 'NONE',  ( 20.46625090740818109, 1507.818616722226807, 228.4183586287386447 ) ) ;
#40492=CARTESIAN_POINT ( 'NONE',  ( 3.116763890020000094, 1441.234358967379876, 170.5448746976979919 ) ) ;
#40493=CARTESIAN_POINT ( 'NONE',  ( -1.779266724299999991, 1476.084642096830066, 267.8527211508980486 ) ) ;
#40494=CARTESIAN_POINT ( 'NONE',  ( -11.19904275380046599, 1425.025785267508354, 138.1878544111817462 ) ) ;
#40495=CARTESIAN_POINT ( 'NONE',  ( -17.60627216660330063, 1410.895669502700230, 193.4350316886979897 ) ) ;
#40496=EDGE_CURVE ( 'NONE', #69919, #44698, #102773, .T. ) ;
#40501=CARTESIAN_POINT ( 'NONE',  ( 2.760778564396810353, 1409.009468899150079, 230.1977509304229841 ) ) ;
#40504=EDGE_CURVE ( 'NONE', #77737, #22920, #28632, .T. ) ;
#40505=CARTESIAN_POINT ( 'NONE',  ( -22.38836670029999709, 1410.616270142430039, 203.1479786175279969 ) ) ;
#40508=CARTESIAN_POINT ( 'NONE',  ( -3.298498094659999769, 1407.650947899530138, 270.1377426963979929 ) ) ;
#40509=ORIENTED_EDGE ( 'NONE', *, *, #83167, .F. ) ;
#40513=DIRECTION ( 'NONE',  ( -0.7067700363771036720, 0.03085824620770448792, -0.7067700363771036720 ) ) ;
#40521=CARTESIAN_POINT ( 'NONE',  ( -9.534219445089998857, 1428.030197386430018, 144.1938086916980239 ) ) ;
#40525=CARTESIAN_POINT ( 'NONE',  ( 20.85715114138509918, 1508.960603666100042, 227.8108728366430000 ) ) ;
#40529=EDGE_LOOP ( 'NONE', ( #103987, #42079, #31117, #82167, #50797 ) ) ;
#40530=ORIENTED_EDGE ( 'NONE', *, *, #83719, .F. ) ;
#40531=CARTESIAN_POINT ( 'NONE',  ( 11.85650668279999920, 1434.045051391929974, 150.8704278162979904 ) ) ;
#40532=CARTESIAN_POINT ( 'NONE',  ( -7.937424474279999309, 1397.838828921930144, 219.9794736354980103 ) ) ;
#40533=CARTESIAN_POINT ( 'NONE',  ( -19.24584652619999758, 1409.749709703130065, 221.2367099497979837 ) ) ;
#40535=CARTESIAN_POINT ( 'NONE',  ( -13.31737298010640380, 1444.561816739103051, 169.3769464296262299 ) ) ;
#40536=CARTESIAN_POINT ( 'NONE',  ( 22.33114268944675018, 1509.698422332540986, 228.3716627733444113 ) ) ;
#40539=CARTESIAN_POINT ( 'NONE',  ( 17.85825448869999832, 1419.057470054430041, 225.0456301946979920 ) ) ;
#40541=CARTESIAN_POINT ( 'NONE',  ( 14.44949573220000083, 1468.697490635830036, 188.3306200720979859 ) ) ;
#40542=CARTESIAN_POINT ( 'NONE',  ( -7.191821496720000262, 1414.913060387229962, 194.0837811316980037 ) ) ;
#40544=CARTESIAN_POINT ( 'NONE',  ( 10.54395425458129942, 1396.281263384510112, 205.7609669223470235 ) ) ;
#40545=EDGE_CURVE ( 'NONE', #89981, #12260, #39687, .T. ) ;
#40546=CARTESIAN_POINT ( 'NONE',  ( 1.149035020129999918, 1415.140114695929924, 191.3456881844979875 ) ) ;
#40547=CARTESIAN_POINT ( 'NONE',  ( 11.22829442119999932, 1427.193422228129975, 149.5441094775980275 ) ) ;
#40548=CARTESIAN_POINT ( 'NONE',  ( 7.515087040108598515, 1509.176409119497976, 180.7408218922122387 ) ) ;
#40550=CARTESIAN_POINT ( 'NONE',  ( 12.96456176665079951, 1434.782329531799860, 149.4767548373170030 ) ) ;
#40553=VERTEX_POINT ( 'NONE', #39787 ) ;
#40554=CARTESIAN_POINT ( 'NONE',  ( -18.04049389182639729, 1478.103586370280027, 228.8030285101139896 ) ) ;
#40555=CARTESIAN_POINT ( 'NONE',  ( -4.153219689960000238, 1466.619231579529924, 234.7255339115979780 ) ) ;
#40556=CARTESIAN_POINT ( 'NONE',  ( -12.78671360849999772, 1416.817366564930126, 196.1060123485979716 ) ) ;
#40560=ORIENTED_EDGE ( 'NONE', *, *, #3535, .F. ) ;
#40562=CARTESIAN_POINT ( 'NONE',  ( 2.500000000000000000, 1448.335387686779995, 163.4889113519770092 ) ) ;
#40564=( BOUNDED_SURFACE ( )  B_SPLINE_SURFACE ( 4, 2, ( 
 ( #85054, #51467, #77237, #34662, #68847, #104628, #52035, #76668, #86171, #27925, #103512 ),
 ( #25691, #95129, #26251, #60439, #94557, #104071, #9464, #17832, #43629, #52590, #77778 ),
 ( #61548, #1089, #26816, #61003, #18391, #86723, #44185, #95680, #53142, #87280, #10575 ),
 ( #78896, #44746, #79982, #12776, #96231, #54257, #64304, #88383, #45299, #3301, #2751 ),
 ( #106818, #11673, #96793, #79439, #46407, #89481, #88926, #98424, #63751, #28479, #97865 ) ),
 .UNSPECIFIED., .F., .T., .F. ) 
 B_SPLINE_SURFACE_WITH_KNOTS ( ( 5, 5 ),
 ( 3, 2, 2, 2, 2, 3 ),
 ( 3.613988937050000239, 5.260361675040000407 ),
 ( 5.178099995975939507, 6.283185307179590673, 7.853981633974480125, 9.424777960769379348, 10.99557428756429900, 11.46128530315550087 ),
 .UNSPECIFIED. ) 
 GEOMETRIC_REPRESENTATION_ITEM ( )  RATIONAL_B_SPLINE_SURFACE ( (
 ( 0.8778166930676709612, 0.7939440089458740246, 1.000000000000000000, 0.7071067811865480168, 1.000000000000000000, 0.7071067811865480168, 1.000000000000000000, 0.7071067811865480168, 1.000000000000000000, 0.9131627722406729930, 0.8778166930676709612),
 ( 0.8778166930676709612, 0.7939440089458740246, 1.000000000000000000, 0.7071067811865480168, 1.000000000000000000, 0.7071067811865480168, 1.000000000000000000, 0.7071067811865480168, 1.000000000000000000, 0.9131627722406729930, 0.8778166930676709612),
 ( 0.8778166930676709612, 0.7939440089458740246, 1.000000000000000000, 0.7071067811865480168, 1.000000000000000000, 0.7071067811865480168, 1.000000000000000000, 0.7071067811865480168, 1.000000000000000000, 0.9131627722406729930, 0.8778166930676709612),
 ( 0.8778166930676709612, 0.7939440089458740246, 1.000000000000000000, 0.7071067811865480168, 1.000000000000000000, 0.7071067811865480168, 1.000000000000000000, 0.7071067811865480168, 1.000000000000000000, 0.9131627722406729930, 0.8778166930676709612),
 ( 0.8778166930676709612, 0.7939440089458740246, 1.000000000000000000, 0.7071067811865480168, 1.000000000000000000, 0.7071067811865480168, 1.000000000000000000, 0.7071067811865480168, 1.000000000000000000, 0.9131627722406729930, 0.8778166930676709612) ) ) 
 REPRESENTATION_ITEM ( '' )  SURFACE ( )  );
#40569=CARTESIAN_POINT ( 'NONE',  ( -21.02506738559999988, 1509.639958407829909, 229.8460882628980073 ) ) ;
#40570=CARTESIAN_POINT ( 'NONE',  ( -36.12168399312893996, 1425.338662683803022, 269.5474266120900779 ) ) ;
#40575=CARTESIAN_POINT ( 'NONE',  ( -28.98124970245649834, 1440.913060387189944, 234.8964103687889917 ) ) ;
#40577=PLANE ( 'NONE',  #39121 ) ;
#40579=CARTESIAN_POINT ( 'NONE',  ( 8.021036561768740469, 1410.327436765469884, 270.0743298054680395 ) ) ;
#40581=CARTESIAN_POINT ( 'NONE',  ( 23.31374782499999654, 1409.831799812029885, 209.2655790302239893 ) ) ;
#40588=ADVANCED_FACE ( 'NONE', ( #6722 ), #33010, .F. ) ;
#40589=CARTESIAN_POINT ( 'NONE',  ( 0.04809717934580000354, 1420.202363427830051, 183.9005163246980032 ) ) ;
#40590=CARTESIAN_POINT ( 'NONE',  ( -3.482404828285579956, 1485.996524617339901, 182.2044860649310181 ) ) ;
#40592=ORIENTED_EDGE ( 'NONE', *, *, #11355, .T. ) ;
#40594=CARTESIAN_POINT ( 'NONE',  ( 18.89924256150000303, 1416.831925117730179, 210.6687426732179631 ) ) ;
#40597=CARTESIAN_POINT ( 'NONE',  ( -18.18137283769999968, 1507.608465321030053, 229.7139307937979993 ) ) ;
#40598=CARTESIAN_POINT ( 'NONE',  ( -4.925559152112373162, 1409.085064703106355, 194.7584071229671849 ) ) ;
#40600=LINE ( 'NONE', #90994, #30809 ) ;
#40604=CARTESIAN_POINT ( 'NONE',  ( -25.66452594925480923, 1450.796198851616282, 137.0023867642745188 ) ) ;
#40606=ORIENTED_EDGE ( 'NONE', *, *, #11781, .F. ) ;
#40609=CARTESIAN_POINT ( 'NONE',  ( 0.2329173765010000285, 1487.216803758130027, 230.2681330600980232 ) ) ;
#40611=FACE_OUTER_BOUND ( 'NONE', #85509, .T. ) ;
#40615=CARTESIAN_POINT ( 'NONE',  ( 7.013597998606249107, 1416.776616305703783, 231.0639749510152399 ) ) ;
#40617=CARTESIAN_POINT ( 'NONE',  ( 40.18841066169029830, 1444.887014588840202, 136.9828721817030157 ) ) ;
#40618=CARTESIAN_POINT ( 'NONE',  ( -19.34668267510000206, 1426.404838512529977, 224.4165203646980160 ) ) ;
#40619=CARTESIAN_POINT ( 'NONE',  ( -24.71654799220000243, 1435.786941262089840, 137.7886789613979772 ) ) ;
#40621=CARTESIAN_POINT ( 'NONE',  ( 12.86159104559999911, 1509.362197043529932, 182.9546168079979793 ) ) ;
#40623=CARTESIAN_POINT ( 'NONE',  ( -27.62462018541545916, 1463.884133562258057, 269.4472085826375292 ) ) ;
#40625=CARTESIAN_POINT ( 'NONE',  ( -4.196074440480000121E-15, 1430.453334911130241, 150.3332009510979788 ) ) ;
#40627=CARTESIAN_POINT ( 'NONE',  ( -43.11111256194765673, 1429.682096741483065, 269.0454486936832268 ) ) ;
#40630=CARTESIAN_POINT ( 'NONE',  ( -15.24610303002120659, 1451.631057024628035, 222.8112762265741651 ) ) ;
#40632=CARTESIAN_POINT ( 'NONE',  ( -13.51709569822251922, 1443.869434758233183, 187.1393552450566915 ) ) ;
#40635=CARTESIAN_POINT ( 'NONE',  ( -1.649050658508506073, 1415.557147993468789, 233.1206746122759341 ) ) ;
#40638=CARTESIAN_POINT ( 'NONE',  ( -12.77345823270095870, 1442.835097972180620, 169.4523692618799657 ) ) ;
#40639=CARTESIAN_POINT ( 'NONE',  ( -15.08447935729999934, 1409.953164787530113, 226.5286084827979778 ) ) ;
#40640=ORIENTED_EDGE ( 'NONE', *, *, #80072, .T. ) ;
#40641=CARTESIAN_POINT ( 'NONE',  ( 0.4068402808920000280, 1415.948532224930204, 190.9215044426980228 ) ) ;
#40642=EDGE_CURVE ( 'NONE', #92171, #15354, #34330, .T. ) ;
#40643=CARTESIAN_POINT ( 'NONE',  ( 21.46027241321153411, 1509.101876359112566, 226.4434528296256417 ) ) ;
#40646=CARTESIAN_POINT ( 'NONE',  ( 18.15372975567069957, 1416.529254608160045, 209.1733715860090115 ) ) ;
#40649=CARTESIAN_POINT ( 'NONE',  ( -3.935524436840000195, 1461.184553958630204, 220.7697451388980028 ) ) ;
#40650=CARTESIAN_POINT ( 'NONE',  ( -20.60158592759999863, 1507.916213491630060, 190.0723952602979807 ) ) ;
#40651=CARTESIAN_POINT ( 'NONE',  ( -11.87922033200000094, 1433.121278621640158, 150.0748730425980000 ) ) ;
#40652=EDGE_CURVE ( 'NONE', #19628, #5604, #109111, .T. ) ;
#40655=CARTESIAN_POINT ( 'NONE',  ( 25.03647985883640104, 1433.346993170209998, 209.5640697471909846 ) ) ;
#40656=CARTESIAN_POINT ( 'NONE',  ( -26.25026149509999840, 1438.546304523360050, 137.1341921698980002 ) ) ;
#40657=CARTESIAN_POINT ( 'NONE',  ( -14.58270751444020341, 1429.861807585111592, 222.1210857218158878 ) ) ;
#40659=CARTESIAN_POINT ( 'NONE',  ( 2.675979268209999873, 1451.712890839929969, 183.7935420642980091 ) ) ;
#40661=EDGE_CURVE ( 'NONE', #31602, #2577, #101183, .T. ) ;
#40662=CARTESIAN_POINT ( 'NONE',  ( -27.53680538714794324, 1509.986730036300969, 197.2170476805838177 ) ) ;
#40665=ORIENTED_EDGE ( 'NONE', *, *, #79491, .T. ) ;
#40666=CARTESIAN_POINT ( 'NONE',  ( -11.75633636577309993, 1426.832617176000213, 145.5136197768400166 ) ) ;
#40668=CARTESIAN_POINT ( 'NONE',  ( -5.035691841070000230, 1473.968067415529958, 270.1320510969979978 ) ) ;
#40671=CARTESIAN_POINT ( 'NONE',  ( 36.52315179513340127, 1449.845863385239909, 136.2557797426800050 ) ) ;
#40677=CARTESIAN_POINT ( 'NONE',  ( -42.10743620715810209, 1426.274024488540135, 266.8069455525510421 ) ) ;
#40678=ORIENTED_EDGE ( 'NONE', *, *, #47219, .T. ) ;
#40679=CARTESIAN_POINT ( 'NONE',  ( -2.109056957580000002, 1421.166295015029846, 183.8085771866980167 ) ) ;
#40680=EDGE_CURVE ( 'NONE', #64662, #4923, #82535, .T. ) ;
#40685=CARTESIAN_POINT ( 'NONE',  ( 4.640563141391067958, 1423.702541937380602, 183.8770172325440058 ) ) ;
#40689=CARTESIAN_POINT ( 'NONE',  ( -14.43289921072090110, 1509.539432542180066, 182.8218189571549885 ) ) ;
#40690=CARTESIAN_POINT ( 'NONE',  ( -7.546903754000000575, 1440.426785413330208, 186.1739043644979859 ) ) ;
#40692=CARTESIAN_POINT ( 'NONE',  ( -15.46699364564850043, 1461.188218472669860, 228.6959131744210083 ) ) ;
#40694=CARTESIAN_POINT ( 'NONE',  ( -26.80188213010000098, 1435.454224975739862, 135.5604543457980071 ) ) ;
#40698=( BOUNDED_CURVE ( )  B_SPLINE_CURVE ( 3, ( #29332, #79763, #87608, #3071 ),
 .UNSPECIFIED., .F., .T. ) 
 B_SPLINE_CURVE_WITH_KNOTS ( ( 4, 4 ),
 ( 1.650548988561060026, 1.665073080160537788 ),
 .UNSPECIFIED. ) 
 CURVE ( )  GEOMETRIC_REPRESENTATION_ITEM ( )  RATIONAL_B_SPLINE_CURVE ( ( 1.000000000000000000, 0.9999824209741901004, 0.9999824209741901004, 1.000000000000000000 ) ) 
 REPRESENTATION_ITEM ( '' )  );
#40699=CARTESIAN_POINT ( 'NONE',  ( -39.37395162027389972, 1426.108969844229932, 270.3385322152020649 ) ) ;
#40701=CARTESIAN_POINT ( 'NONE',  ( -6.170313877949999970, 1397.182081567729938, 197.8857380414980014 ) ) ;
#40702=CARTESIAN_POINT ( 'NONE',  ( -38.20494153861119457, 1442.993962785479880, 137.1161392804889942 ) ) ;
#40705=DIRECTION ( 'NONE',  ( 0.000000000000000000, 0.000000000000000000, 1.000000000000000000 ) ) ;
#40706=CARTESIAN_POINT ( 'NONE',  ( 3.902542035141590038, 1426.015650130040058, 185.2953857556300079 ) ) ;
#40708=CARTESIAN_POINT ( 'NONE',  ( -23.85803262429999805, 1435.336726310830045, 137.1743639523980107 ) ) ;
#40709=CARTESIAN_POINT ( 'NONE',  ( 0.1595995995380000143, 1486.508831850330125, 181.8147405652979671 ) ) ;
#40715=CARTESIAN_POINT ( 'NONE',  ( -13.15726447020000123, 1414.996442546230128, 220.4820293380979876 ) ) ;
#40724=CARTESIAN_POINT ( 'NONE',  ( 12.91446205857219987, 1435.737941321880044, 150.7125339207690047 ) ) ;
#40725=CARTESIAN_POINT ( 'NONE',  ( 13.61423569610000150, 1415.579607672129896, 196.7893798472979938 ) ) ;
#40726=CARTESIAN_POINT ( 'NONE',  ( 16.31200673029999848, 1449.547814607470173, 190.3222646265980131 ) ) ;
#40727=CARTESIAN_POINT ( 'NONE',  ( 25.61534012080000267, 1452.018571213930045, 135.1702111959979788 ) ) ;
#40730=CARTESIAN_POINT ( 'NONE',  ( -0.1166470026081705552, 1506.491018783253367, 187.0913018223803874 ) ) ;
#40731=CARTESIAN_POINT ( 'NONE',  ( 24.45342579656801618, 1444.690443231116660, 213.7192692780448908 ) ) ;
#40733=CARTESIAN_POINT ( 'NONE',  ( 33.91369110979999846, 1435.681798629080049, 135.0664268281979901 ) ) ;
#40737=CARTESIAN_POINT ( 'NONE',  ( -12.78723768810000117, 1416.835809767730098, 195.5393901623979787 ) ) ;
#40738=CARTESIAN_POINT ( 'NONE',  ( 16.19087789078229989, 1409.478458302130093, 193.2334102746530107 ) ) ;
#40739=CARTESIAN_POINT ( 'NONE',  ( 1.781954896769999852, 1421.049472850429993, 183.1039533116980067 ) ) ;
#40744=CARTESIAN_POINT ( 'NONE',  ( 18.83207817909999804, 1416.311719782429918, 210.6697760117079952 ) ) ;
#40747=CARTESIAN_POINT ( 'NONE',  ( 36.52292854368440800, 1440.913060387340010, 253.7928692754369706 ) ) ;
#40749=CARTESIAN_POINT ( 'NONE',  ( -21.31355172039999957, 1471.299568758130135, 207.5959159578679873 ) ) ;
#40751=ORIENTED_EDGE ( 'NONE', *, *, #13050, .F. ) ;
#40752=ORIENTED_EDGE ( 'NONE', *, *, #109197, .F. ) ;
#40755=B_SPLINE_CURVE_WITH_KNOTS ( 'NONE', 5,
 ( #62401, #19230, #61850, #45045, #79190, #2496, #106035, #54553, #97628 ),
 .UNSPECIFIED., .F., .F.,
 ( 6, 3, 6 ),
 ( 0.000000000000000000, 0.5828366913979391439, 1.000000000000000000 ),
 .UNSPECIFIED. ) ;
#40758=AXIS2_PLACEMENT_3D ( 'NONE', #70960, #2640, #35103 ) ;
#40759=CARTESIAN_POINT ( 'NONE',  ( -12.61823209568500026, 1416.826860677879949, 222.0544590270410197 ) ) ;
#40762=DIRECTION ( 'NONE',  ( 0.9417419115949053898, -0.3363363969979660806, 9.559255346349054600E-15 ) ) ;
#40765=CARTESIAN_POINT ( 'NONE',  ( -15.10740574596529839, 1465.251597859479944, 223.4038671133249920 ) ) ;
#40766=CARTESIAN_POINT ( 'NONE',  ( 24.95756467220000019, 1451.613974107930062, 137.4741664119979987 ) ) ;
#40777=ORIENTED_EDGE ( 'NONE', *, *, #62192, .T. ) ;
#40779=CARTESIAN_POINT ( 'NONE',  ( 35.62940004342829781, 1437.304582500250262, 136.5355437598550168 ) ) ;
#40781=CARTESIAN_POINT ( 'NONE',  ( 1.802301219090000073, 1409.910657985330090, 232.1755723407979985 ) ) ;
#40787=CARTESIAN_POINT ( 'NONE',  ( 13.00319530123149825, 1409.367141973109938, 201.7590943873260017 ) ) ;
#40788=DIRECTION ( 'NONE',  ( -1.000000000000000000, 0.000000000000000000, 0.000000000000000000 ) ) ;
#40791=CARTESIAN_POINT ( 'NONE',  ( 11.30198679499999947, 1432.355652606810054, 151.5220046058980188 ) ) ;
#40793=CARTESIAN_POINT ( 'NONE',  ( -3.369446259835010338, 1448.970159117820003, 184.7951506743999914 ) ) ;
#40796=CARTESIAN_POINT ( 'NONE',  ( 19.00954907529469651, 1456.857281488789795, 226.5573691136240200 ) ) ;
#40797=CARTESIAN_POINT ( 'NONE',  ( -12.81107806870000054, 1435.505600523229759, 150.7241902968979730 ) ) ;
#40800=CARTESIAN_POINT ( 'NONE',  ( 2.688586027246119947, 1509.006950727750109, 238.2845013960090057 ) ) ;
#40801=LINE ( 'NONE', #38587, #13883 ) ;
#40804=CARTESIAN_POINT ( 'NONE',  ( -46.05254598119929454, 1440.698150564019898, 266.6769892118650205 ) ) ;
#40808=AXIS2_PLACEMENT_3D ( 'NONE', #37234, #52942, #103299 ) ;
#40809=CARTESIAN_POINT ( 'NONE',  ( 4.398715393588610745, 1409.066666913600102, 223.5593897730840069 ) ) ;
#40810=EDGE_CURVE ( 'NONE', #8175, #75798, #60709, .T. ) ;
#40811=CARTESIAN_POINT ( 'NONE',  ( 5.684698448500000723, 1422.983443193229959, 101.6537298026979954 ) ) ;
#40813=ORIENTED_EDGE ( 'NONE', *, *, #69666, .T. ) ;
#40814=CARTESIAN_POINT ( 'NONE',  ( 29.63060611060000227, 1437.055399740629809, 238.0637397513980034 ) ) ;
#40815=CARTESIAN_POINT ( 'NONE',  ( -1.462006285199999978, 1452.693442003630025, 183.1060772031979980 ) ) ;
#40817=EDGE_CURVE ( 'NONE', #86466, #23487, #4765, .T. ) ;
#40819=CARTESIAN_POINT ( 'NONE',  ( -26.57890459470000266, 1440.913060377039983, 225.2395996604980155 ) ) ;
#40821=CARTESIAN_POINT ( 'NONE',  ( 0.7186111224017516230, 1415.502631355655922, 233.2905737576144247 ) ) ;
#40822=CARTESIAN_POINT ( 'NONE',  ( 29.24087330780000116, 1451.891771913630237, 134.8528131887979953 ) ) ;
#40823=ORIENTED_EDGE ( 'NONE', *, *, #29742, .T. ) ;
#40824=DIRECTION ( 'NONE',  ( -0.8304244096547924725, -0.2476038119107163427, -0.4990868182759106708 ) ) ;
#40826=CARTESIAN_POINT ( 'NONE',  ( 14.52431039145089997, 1420.570648330259928, 228.2522164977820296 ) ) ;
#40829=ORIENTED_EDGE ( 'NONE', *, *, #5717, .F. ) ;
#40832=CARTESIAN_POINT ( 'NONE',  ( -22.82803524321889910, 1409.710179317919938, 209.0907902649259995 ) ) ;
#40833=ORIENTED_EDGE ( 'NONE', *, *, #78317, .F. ) ;
#40839=CARTESIAN_POINT ( 'NONE',  ( -15.47717805819999981, 1507.633541959229888, 231.3088780856980122 ) ) ;
#40840=CARTESIAN_POINT ( 'NONE',  ( -19.15216164439999957, 1415.854273250330152, 223.1450478733979992 ) ) ;
#40842=AXIS2_PLACEMENT_3D ( 'NONE', #62251, #10160, #78477 ) ;
#40843=CARTESIAN_POINT ( 'NONE',  ( 46.15276881562959943, 1443.753714320680047, 267.5938072023989776 ) ) ;
#40845=CARTESIAN_POINT ( 'NONE',  ( 0.1379860871630000096, 1419.157121733429904, 184.6437352945980024 ) ) ;
#40848=CARTESIAN_POINT ( 'NONE',  ( 18.75615393743843029, 1458.159782462800649, 227.2589280249185606 ) ) ;
#40851=CARTESIAN_POINT ( 'NONE',  ( 2.500000005229999989, 1448.233542440780184, 182.8968085845980056 ) ) ;
#40852=CARTESIAN_POINT ( 'NONE',  ( 26.85709460237750079, 1451.975207230750129, 134.9160983460150192 ) ) ;
#40858=CARTESIAN_POINT ( 'NONE',  ( 2.151766400366240006, 1408.988201725800081, 186.9699580838769748 ) ) ;
#40859=CARTESIAN_POINT ( 'NONE',  ( -13.46701286011549925, 1434.939967867589985, 148.8194410816790025 ) ) ;
#40860=CARTESIAN_POINT ( 'NONE',  ( -18.54538606469993312, 1424.331165113354700, 224.9582236530350769 ) ) ;
#40861=CARTESIAN_POINT ( 'NONE',  ( 3.497150990277209104, 1441.358042536442326, 170.5351636937986370 ) ) ;
#40864=DIRECTION ( 'NONE',  ( -0.9417419115949662300, -0.2378257470769920556, 0.2378257470769920556 ) ) ;
#40865=EDGE_LOOP ( 'NONE', ( #3832, #49651, #2740, #6531 ) ) ;
#40870=( BOUNDED_CURVE ( )  B_SPLINE_CURVE ( 3, ( #105239, #80034, #44797, #86220 ),
 .UNSPECIFIED., .F., .F. ) 
 B_SPLINE_CURVE_WITH_KNOTS ( ( 4, 4 ),
 ( 6.207195670891930028, 6.514798957309980487 ),
 .UNSPECIFIED. ) 
 CURVE ( )  GEOMETRIC_REPRESENTATION_ITEM ( )  RATIONAL_B_SPLINE_CURVE ( ( 1.000000000000000000, 0.9921305491659986320, 0.9921305491659986320, 1.000000000000000000 ) ) 
 REPRESENTATION_ITEM ( '' )  );
#40873=CARTESIAN_POINT ( 'NONE',  ( 13.06210717429999946, 1418.073220907129780, 221.6712522191980099 ) ) ;
#40874=CARTESIAN_POINT ( 'NONE',  ( -40.73184307449999864, 1440.913060387330006, 268.3665355201979992 ) ) ;
#40876=CARTESIAN_POINT ( 'NONE',  ( 11.87454696380000030, 1433.566416203000017, 150.5469651275980141 ) ) ;
#40877=CARTESIAN_POINT ( 'NONE',  ( 38.34143788450000301, 1440.913060387330006, 265.6112250856980381 ) ) ;
#40878=CARTESIAN_POINT ( 'NONE',  ( 13.15726442949999964, 1415.948532224930204, 196.5399405751979884 ) ) ;
#40882=CARTESIAN_POINT ( 'NONE',  ( 12.78749341904959991, 1416.842625005220043, 222.1385636096939891 ) ) ;
#40884=CARTESIAN_POINT ( 'NONE',  ( -17.48419695489999981, 1410.887768726630156, 225.6235195252980077 ) ) ;
#40885=CARTESIAN_POINT ( 'NONE',  ( -0.5620977654159999837, 1416.851343902729923, 227.7685710129979952 ) ) ;
#40886=CARTESIAN_POINT ( 'NONE',  ( -7.083943808717527268, 1442.001743124033055, 184.0116861733216069 ) ) ;
#40887=CARTESIAN_POINT ( 'NONE',  ( -17.06446529402930068, 1409.673968815769967, 193.1470206694820035 ) ) ;
#40891=FACE_OUTER_BOUND ( 'NONE', #95171, .T. ) ;
#40893=CARTESIAN_POINT ( 'NONE',  ( 0.2059318620510010023, 1459.640043076150050, 182.9685224155400078 ) ) ;
#40894=CARTESIAN_POINT ( 'NONE',  ( -10.79382269979189957, 1414.913060387349788, 196.1395788316550011 ) ) ;
#40896=CARTESIAN_POINT ( 'NONE',  ( -20.22153155800000235, 1444.740067931809790, 161.9155394238979966 ) ) ;
#40897=CARTESIAN_POINT ( 'NONE',  ( -29.06644740117960168, 1509.916355021930030, 211.6311731943499979 ) ) ;
#40898=CARTESIAN_POINT ( 'NONE',  ( 13.80518339569999853, 1434.979590798060144, 149.4781242251980302 ) ) ;
#40899=CARTESIAN_POINT ( 'NONE',  ( -41.49772933732800340, 1445.334750750280136, 134.0999999984909721 ) ) ;
#40901=VERTEX_POINT ( 'NONE', #28924 ) ;
#40909=AXIS2_PLACEMENT_3D ( 'NONE', #38461, #106225, #53645 ) ;
#40912=CARTESIAN_POINT ( 'NONE',  ( 21.02608924029999926, 1456.853724928630072, 225.6706377209980303 ) ) ;
#40918=CARTESIAN_POINT ( 'NONE',  ( -33.93392600300000339, 1451.271752324530098, 135.9465290377980011 ) ) ;
#40919=CARTESIAN_POINT ( 'NONE',  ( -16.78004044744790235, 1410.586458347280086, 226.3834300362210001 ) ) ;
#40924=AXIS2_PLACEMENT_3D ( 'NONE', #20606, #45859, #79992 ) ;
#40926=CARTESIAN_POINT ( 'NONE',  ( -20.78416915826518618, 1410.998464924520249, 218.9268079218183232 ) ) ;
#40928=CARTESIAN_POINT ( 'NONE',  ( -0.2146684641345620037, 1419.294041481389968, 184.5302216556299868 ) ) ;
#40929=B_SPLINE_CURVE_WITH_KNOTS ( 'NONE', 3,
 ( #25657, #2714, #94521, #87816, #45265, #36283, #70475, #77744, #11104, #51433, #17795, #103473, #18358, #52552 ),
 .UNSPECIFIED., .F., .F.,
 ( 4, 2, 2, 2, 2, 2, 4 ),
 ( 0.000000000000000000, 0.0005413989221883810064, 0.001082797844376762013, 0.002165595688753024425, 0.002706994610941156065, 0.003248393533129286404, 0.004331191377505529301 ),
 .UNSPECIFIED. ) ;
#40930=ADVANCED_FACE ( 'NONE', ( #44072 ), #48188, .F. ) ;
#40931=CARTESIAN_POINT ( 'NONE',  ( 22.84636239139999603, 1410.205970967429948, 213.3090871733579661 ) ) ;
#40932=CARTESIAN_POINT ( 'NONE',  ( -22.52564151159999639, 1509.699673122230024, 190.3321270482979912 ) ) ;
#40933=CARTESIAN_POINT ( 'NONE',  ( -17.05725733019999879, 1423.778776128129948, 228.3108127086979948 ) ) ;
#40937=CARTESIAN_POINT ( 'NONE',  ( 13.22806383159999832, 1431.113060387329824, 223.7296695649979767 ) ) ;
#40940=AXIS2_PLACEMENT_3D ( 'NONE', #82985, #40975, #6276 ) ;
#40941=CARTESIAN_POINT ( 'NONE',  ( -5.424805956284839858, 1485.524231091950014, 183.2664633616439858 ) ) ;
#40942=ORIENTED_EDGE ( 'NONE', *, *, #61029, .F. ) ;
#40944=CARTESIAN_POINT ( 'NONE',  ( -4.221749840679269283, 1441.602648943890017, 169.9194788150119848 ) ) ;
#40947=CARTESIAN_POINT ( 'NONE',  ( -16.67802482740000158, 1423.369746731130135, 229.1820141820979870 ) ) ;
#40951=CARTESIAN_POINT ( 'NONE',  ( -11.15802834450066960, 1425.158734329488198, 144.3721351036122940 ) ) ;
#40952=CARTESIAN_POINT ( 'NONE',  ( 15.77332111128689895, 1410.712355435420022, 191.5214290250879685 ) ) ;
#40954=CARTESIAN_POINT ( 'NONE',  ( 39.14754442216379715, 1437.687579504329960, 135.1140516034500081 ) ) ;
#40958=CARTESIAN_POINT ( 'NONE',  ( 39.62133910696010020, 1449.056109088829999, 134.0999999980940061 ) ) ;
#40959=CARTESIAN_POINT ( 'NONE',  ( -25.50058789191978903, 1507.958244999422959, 219.0382223049803372 ) ) ;
#40965=CARTESIAN_POINT ( 'NONE',  ( 2.500000000000000000, 1411.429641636930000, 126.8043280305979863 ) ) ;
#40967=CARTESIAN_POINT ( 'NONE',  ( 0.1012992125219999984, 1452.346416936929927, 183.2694984107980076 ) ) ;
#40968=CARTESIAN_POINT ( 'NONE',  ( -3.226026720880000198, 1485.996674929329856, 182.1725539718979974 ) ) ;
#40969=CARTESIAN_POINT ( 'NONE',  ( -2.500000000000000000, 1439.466623781370117, 162.9904194795870183 ) ) ;
#40971=CIRCLE ( 'NONE', #103547, 1.638701816490922836 ) ;
#40974=CARTESIAN_POINT ( 'NONE',  ( 2.215029529077919612, 1421.204142362009861, 183.2132787965950058 ) ) ;
#40975=DIRECTION ( 'NONE',  ( -0.3363363969981477131, 0.6659120918162938496, -0.6659120918162938496 ) ) ;
#40978=ORIENTED_EDGE ( 'NONE', *, *, #67475, .F. ) ;
#40984=CARTESIAN_POINT ( 'NONE',  ( 18.93563805549999657, 1457.027062798830002, 226.9364425294979810 ) ) ;
#40986=CARTESIAN_POINT ( 'NONE',  ( -13.76900370180000088, 1415.553739807329976, 221.3900038008980005 ) ) ;
#40993=CARTESIAN_POINT ( 'NONE',  ( -11.87539561500000040, 1433.006908915509939, 148.5636847365980202 ) ) ;
#40994=CARTESIAN_POINT ( 'NONE',  ( -16.08458092929999950, 1496.377567048629999, 224.3648175664979760 ) ) ;
#40995=CARTESIAN_POINT ( 'NONE',  ( 12.57364047979999810, 1461.601951568030017, 232.5174476254979652 ) ) ;
#40997=CARTESIAN_POINT ( 'NONE',  ( -4.832904859673011977, 1422.320778277333375, 184.7689124830623086 ) ) ;
#41001=CARTESIAN_POINT ( 'NONE',  ( 19.26683521067225868, 1456.110280151028292, 225.0772932314519892 ) ) ;
#41002=CARTESIAN_POINT ( 'NONE',  ( 19.05195134132430113, 1485.012485562190022, 228.6148904062209795 ) ) ;
#41007=CARTESIAN_POINT ( 'NONE',  ( -11.60004869885885981, 1425.580039266544873, 138.3016037470954984 ) ) ;
#41012=CARTESIAN_POINT ( 'NONE',  ( -11.56293446569999972, 1431.298376297659843, 151.1185897447979869 ) ) ;
#41013=DIRECTION ( 'NONE',  ( 0.001339522651315419892, 0.9999644786255611484, 0.008321488218843280452 ) ) ;
#41015=CARTESIAN_POINT ( 'NONE',  ( 11.76196303810490029, 1425.587148917709783, 146.3422016857230119 ) ) ;
#41018=CARTESIAN_POINT ( 'NONE',  ( -19.12494372069999926, 1470.092089012029874, 227.6083304972979988 ) ) ;
#41024=CARTESIAN_POINT ( 'NONE',  ( 7.089205951499999436, 1406.122960630329999, 267.8325111671979926 ) ) ;
#41025=CARTESIAN_POINT ( 'NONE',  ( 0.04535681774329999860, 1409.423586797529879, 185.2161043470979678 ) ) ;
#41027=CARTESIAN_POINT ( 'NONE',  ( 24.41839517916415403, 1437.873015353542996, 212.8347989158633027 ) ) ;
#41030=CARTESIAN_POINT ( 'NONE',  ( 1.546943247107299912, 1416.828039266790029, 190.2227890105679933 ) ) ;
#41034=CARTESIAN_POINT ( 'NONE',  ( -12.76211179859999945, 1446.342786738940049, 187.8166300136979885 ) ) ;
#41035=CARTESIAN_POINT ( 'NONE',  ( 1.971747376402030127, 1450.333125966990110, 155.0636711809370070 ) ) ;
#41038=B_SPLINE_CURVE_WITH_KNOTS ( 'NONE', 5,
 ( #62435, #4160, #96561, #105514, #38287, #19833, #72469, #98194, #54038, #106599, #29884, #1969 ),
 .UNSPECIFIED., .F., .F.,
 ( 6, 3, 3, 6 ),
 ( 0.000000000000000000, 0.1840082528089916347, 0.5520247584167143895, 1.000000000000000000 ),
 .UNSPECIFIED. ) ;
#41039=CARTESIAN_POINT ( 'NONE',  ( -6.509745615790000883, 1426.468882645629947, 219.6133833021979740 ) ) ;
#41040=B_SPLINE_SURFACE_WITH_KNOTS ( 'NONE', 4, 5, ( 
 ( #110563, #18147, #69139, #102687, #93736, #17014 ),
 ( #103243, #95975, #25982, #103824, #94299, #51777 ),
 ( #85915, #52342, #70265, #1942, #36080, #104374 ),
 ( #27670, #3601, #90315, #70820, #88693, #72449 ),
 ( #29865, #79195, #72989, #11432, #56176, #4140 ) ),
 .UNSPECIFIED., .F., .F., .F.,
 ( 5, 5 ),
 ( 6, 6 ),
 ( 83.28839604430000065, 84.04303036039999597 ),
 ( 0.000000000000000000, 2.000000000000000000 ),
 .UNSPECIFIED. ) ;
#41041=CARTESIAN_POINT ( 'NONE',  ( 10.88304335850896010, 1425.085735208080905, 138.6335396438064436 ) ) ;
#41043=CARTESIAN_POINT ( 'NONE',  ( -2.755319248979999802, 1475.501610869329852, 269.2919052328979888 ) ) ;
#41044=CARTESIAN_POINT ( 'NONE',  ( -4.224262963665889714, 1446.243947084759839, 166.7663216723609878 ) ) ;
#41046=CARTESIAN_POINT ( 'NONE',  ( 18.21301937251889669, 1417.703604459479948, 223.2038275229089948 ) ) ;
#41049=CARTESIAN_POINT ( 'NONE',  ( -11.97827956719999776, 1441.604408666619975, 150.7817505876979851 ) ) ;
#41051=CARTESIAN_POINT ( 'NONE',  ( -25.55722864341189648, 1470.062555774519979, 211.0468171208650006 ) ) ;
#41052=DIRECTION ( 'NONE',  ( -0.000000000000000000, 1.000000000000000000, 0.000000000000000000 ) ) ;
#41053=CARTESIAN_POINT ( 'NONE',  ( -46.16777962713913297, 1440.913025796686270, 266.9714940337735811 ) ) ;
#41054=CARTESIAN_POINT ( 'NONE',  ( -22.22003955790000163, 1410.184095304630091, 203.2211024675479791 ) ) ;
#41056=CARTESIAN_POINT ( 'NONE',  ( -15.08006399635999983, 1422.394886018492116, 228.4054473227839992 ) ) ;
#41060=B_SPLINE_SURFACE_WITH_KNOTS ( 'NONE', 5, 5, ( 
 ( #18146, #69704, #77525, #69138, #62976, #18690 ),
 ( #826, #86462, #95427, #87590, #43919, #3051 ),
 ( #36621, #9755, #2500, #88143, #45602, #78066 ),
 ( #70264, #70819, #20353, #1369, #78626, #52887 ),
 ( #54558, #103242, #87015, #37177, #35511, #103823 ),
 ( #26552, #88692, #1941, #36079, #60746, #27123 ) ),
 .UNSPECIFIED., .F., .F., .F.,
 ( 6, 6 ),
 ( 6, 6 ),
 ( 2.161187085849999967, 3.155691482920000013 ),
 ( 0.000000000000000000, 2.242653719299999793 ),
 .UNSPECIFIED. ) ;
#41061=CARTESIAN_POINT ( 'NONE',  ( -4.500000000000000000, 1448.210448412289907, 183.1418046154980175 ) ) ;
#41065=CARTESIAN_POINT ( 'NONE',  ( 11.61671915839999869, 1425.877048038330031, 142.7663299324979960 ) ) ;
#41070=CARTESIAN_POINT ( 'NONE',  ( 27.13948228459569734, 1449.857009993160091, 136.5864004438930124 ) ) ;
#41071=CARTESIAN_POINT ( 'NONE',  ( -0.06764669157372509012, 1408.848989335589977, 223.4935224539250100 ) ) ;
#41074=CARTESIAN_POINT ( 'NONE',  ( -7.214502255410000231, 1427.316505021429975, 144.1938086916980239 ) ) ;
#41078=VECTOR ( 'NONE', #21152, 1000.000000000000000 ) ;
#41079=CARTESIAN_POINT ( 'NONE',  ( 22.02982242722629991, 1509.705750766509937, 228.9645431730439782 ) ) ;
#41083=CARTESIAN_POINT ( 'NONE',  ( 11.97707002367110007, 1433.612440445840093, 149.8647669520520083 ) ) ;
#41084=CARTESIAN_POINT ( 'NONE',  ( -9.880256809820002317, 1396.317500971430036, 216.0574990009879741 ) ) ;
#41085=CARTESIAN_POINT ( 'NONE',  ( -21.13431007490000013, 1409.651086757829944, 211.8287213018879811 ) ) ;
#41086=ORIENTED_EDGE ( 'NONE', *, *, #47972, .T. ) ;
#41087=CARTESIAN_POINT ( 'NONE',  ( -12.92812670435129796, 1444.919964772552021, 169.4323874481358700 ) ) ;
#41088=CARTESIAN_POINT ( 'NONE',  ( 22.14096540611513575, 1509.702029783286889, 228.7416374943908579 ) ) ;
#41091=CARTESIAN_POINT ( 'NONE',  ( 18.02093535799999913, 1424.326836137830014, 225.1991050518980160 ) ) ;
#41092=CARTESIAN_POINT ( 'NONE',  ( 2.889876570069999762, 1449.237408619179860, 183.9651879290979934 ) ) ;
#41095=CARTESIAN_POINT ( 'NONE',  ( 7.090230613856629560, 1396.160656768040099, 200.6535277794220065 ) ) ;
#41096=CARTESIAN_POINT ( 'NONE',  ( 1.226570660889999997, 1415.553739809529816, 190.6686965949980106 ) ) ;
#41097=CARTESIAN_POINT ( 'NONE',  ( 11.30181802809999958, 1432.344320995729731, 151.5221848940979896 ) ) ;
#41098=CARTESIAN_POINT ( 'NONE',  ( 8.900197448897545272, 1509.223855520506504, 181.2015886599364762 ) ) ;
#41100=CARTESIAN_POINT ( 'NONE',  ( 13.38600686010279972, 1434.923461442529970, 148.9942416261320091 ) ) ;
#41105=CARTESIAN_POINT ( 'NONE',  ( -19.93329733863729913, 1507.860201379970022, 229.2059767788809950 ) ) ;
#41106=CARTESIAN_POINT ( 'NONE',  ( -5.374569443010000391, 1464.404629604329784, 236.8301565885979869 ) ) ;
#41111=ORIENTED_EDGE ( 'NONE', *, *, #19397, .T. ) ;
#41119=FACE_OUTER_BOUND ( 'NONE', #29830, .T. ) ;
#41120=CARTESIAN_POINT ( 'NONE',  ( -2.923263438819999838, 1409.521015953330107, 186.8216762074980011 ) ) ;
#41121=CARTESIAN_POINT ( 'NONE',  ( -0.3331912114570000361, 1408.924695680830155, 232.1910260989980088 ) ) ;
#41122=CARTESIAN_POINT ( 'NONE',  ( -0.5835301444350500244, 1415.089118586289942, 226.3143562410230061 ) ) ;
#41124=CARTESIAN_POINT ( 'NONE',  ( 19.10224170140000410, 1426.438701496329941, 223.3166183795979975 ) ) ;
#41127=CARTESIAN_POINT ( 'NONE',  ( -0.4080517659392200458, 1465.111786428190044, 238.1138255402620132 ) ) ;
#41128=CARTESIAN_POINT ( 'NONE',  ( 7.559855552100000153, 1408.395244667930001, 270.2818740095979706 ) ) ;
#41130=CARTESIAN_POINT ( 'NONE',  ( 22.71503220009999779, 1409.706269051729805, 209.0936436305159987 ) ) ;
#41134=ADVANCED_FACE ( 'NONE', ( #47377 ), #109918, .F. ) ;
#41138=CARTESIAN_POINT ( 'NONE',  ( 0.2324887852820000100, 1420.496092096330131, 182.7590697851979940 ) ) ;
#41140=ADVANCED_FACE ( 'NONE', ( #33866 ), #31183, .F. ) ;
#41142=EDGE_LOOP ( 'NONE', ( #63336, #44314, #16029, #75373 ) ) ;
#41147=EDGE_CURVE ( 'NONE', #35589, #41404, #10125, .T. ) ;
#41148=CARTESIAN_POINT ( 'NONE',  ( -38.61942532600000533, 1444.188087375399846, 137.1592399812980148 ) ) ;
#41153=CARTESIAN_POINT ( 'NONE',  ( -23.84859116899999876, 1446.062256459500077, 214.1355555763180121 ) ) ;
#41154=CARTESIAN_POINT ( 'NONE',  ( 0.8957613442250700331, 1452.912621291000050, 183.3566031976109798 ) ) ;
#41155=ADVANCED_FACE ( 'NONE', ( #19685 ), #16920, .F. ) ;
#41164=CARTESIAN_POINT ( 'NONE',  ( -0.04665562252469999949, 1457.821573612329985, 229.0784639932980156 ) ) ;
#41165=CARTESIAN_POINT ( 'NONE',  ( 22.77748398619999648, 1450.072706315450205, 219.0539608951079913 ) ) ;
#41167=CARTESIAN_POINT ( 'NONE',  ( 11.60004869885203682, 0.000000000000000000, 134.0999999980979851 ) ) ;
#41168=EDGE_CURVE ( 'NONE', #100091, #79464, #86278, .T. ) ;
#41169=CARTESIAN_POINT ( 'NONE',  ( 26.26611707621578873, 1450.753935678440257, 136.6023704354048220 ) ) ;
#41171=CARTESIAN_POINT ( 'NONE',  ( 29.68682906300000113, 1435.534167576209938, 135.1977161657979991 ) ) ;
#41172=CARTESIAN_POINT ( 'NONE',  ( 38.15215272849530237, 1448.684869598680052, 136.3987171033640209 ) ) ;
#41173=CARTESIAN_POINT ( 'NONE',  ( 20.00077711682029857, 1506.539416727767502, 218.4579560628022818 ) ) ;
#41176=CARTESIAN_POINT ( 'NONE',  ( -17.45221183250000152, 1413.296611998330036, 225.8619397856980129 ) ) ;
#41179=CARTESIAN_POINT ( 'NONE',  ( -29.80092322115732983, 1462.394957644986334, 269.4686990303187599 ) ) ;
#41182=CARTESIAN_POINT ( 'NONE',  ( 4.144681717681806710, 1507.117986406631189, 186.7896738910754380 ) ) ;
#41185=DIRECTION ( 'NONE',  ( 0.9098001251504946874, -0.3556210061633369723, 0.2140033463558929649 ) ) ;
#41187=CARTESIAN_POINT ( 'NONE',  ( -0.8265242355799999885, 1408.941923249630008, 187.0792671738979891 ) ) ;
#41188=CARTESIAN_POINT ( 'NONE',  ( -12.95896253566151834, 1444.901424241698123, 186.2279615641708972 ) ) ;
#41189=B_SPLINE_SURFACE_WITH_KNOTS ( 'NONE', 3, 5, ( 
 ( #93880, #59215, #92238, #77111, #34537, #16597 ),
 ( #101722, #7681, #110143, #41837, #83838, #42952 ),
 ( #68719, #419, #85472, #42385, #102824, #40737 ),
 ( #94427, #76540, #17703, #51907, #75993, #17146 ) ),
 .UNSPECIFIED., .F., .F., .F.,
 ( 4, 4 ),
 ( 6, 6 ),
 ( 5.479561955080000324, 5.505632800979999963 ),
 ( 0.000000000000000000, 1.000000000000000000 ),
 .UNSPECIFIED. ) ;
#41193=CARTESIAN_POINT ( 'NONE',  ( -4.193705225835856254, 1415.995780155225248, 232.4011042397820859 ) ) ;
#41194=CARTESIAN_POINT ( 'NONE',  ( 17.74176952027255183, 1410.893628039027362, 223.3341983228125400 ) ) ;
#41195=CARTESIAN_POINT ( 'NONE',  ( 25.28186086219999851, 1435.386619864120121, 135.7772238486980143 ) ) ;
#41196=CARTESIAN_POINT ( 'NONE',  ( -12.94642120436389554, 1442.917301946143425, 169.4295745761914702 ) ) ;
#41197=CARTESIAN_POINT ( 'NONE',  ( 18.01510524478549868, 1424.528298123270133, 225.6033285300410114 ) ) ;
#41200=CARTESIAN_POINT ( 'NONE',  ( 0.2612772523340000097, 1416.851343897030119, 190.7759414237980025 ) ) ;
#41204=CARTESIAN_POINT ( 'NONE',  ( 18.10358820054819873, 1416.830086716310007, 209.0369172249700114 ) ) ;
#41209=CARTESIAN_POINT ( 'NONE',  ( -11.46499703930000003, 1433.136224980220049, 151.2988949122980102 ) ) ;
#41213=CARTESIAN_POINT ( 'NONE',  ( -24.65468602429999834, 1440.334300524250011, 210.6770184181980028 ) ) ;
#41214=SPHERICAL_SURFACE ( 'NONE', #53364, 2.000000000000000000 ) ;
#41215=CARTESIAN_POINT ( 'NONE',  ( 1.610950544670000095, 1451.193671323529998, 183.0676007769979776 ) ) ;
#41217=CARTESIAN_POINT ( 'NONE',  ( -27.81626572861782520, 1509.996270472295009, 197.8821087052356518 ) ) ;
#41218=CARTESIAN_POINT ( 'NONE',  ( -2.747389875506000363E-09, 1415.237975642199899, 243.5845164730120018 ) ) ;
#41221=CARTESIAN_POINT ( 'NONE',  ( -11.83934983080530046, 1430.503885545030016, 149.6717847768150023 ) ) ;
#41224=CARTESIAN_POINT ( 'NONE',  ( -5.377271149169999376, 1473.660644874129957, 270.2871877486979884 ) ) ;
#41225=CARTESIAN_POINT ( 'NONE',  ( -1.549353400650000046, 1416.067629296030191, 227.8551223243979962 ) ) ;
#41228=CARTESIAN_POINT ( 'NONE',  ( 39.85254359737009366, 1448.755683825020014, 135.8476807215540134 ) ) ;
#41229=CARTESIAN_POINT ( 'NONE',  ( 15.29461995089999959, 1453.313060387329870, 195.2084026670979995 ) ) ;
#41234=CARTESIAN_POINT ( 'NONE',  ( -12.14973932564840098, 1406.923408263400006, 267.7908327071809822 ) ) ;
#41238=EDGE_LOOP ( 'NONE', ( #60448, #45842, #45688, #82971, #30050 ) ) ;
#41241=CARTESIAN_POINT ( 'NONE',  ( 4.952140499603463475, 1422.530607013576628, 184.3907845083923007 ) ) ;
#41245=CARTESIAN_POINT ( 'NONE',  ( -19.45227738350000024, 1485.491809083029921, 189.8902479364980138 ) ) ;
#41246=VECTOR ( 'NONE', #74669, 1000.000000000000000 ) ;
#41247=CARTESIAN_POINT ( 'NONE',  ( -17.88319679657989880, 1498.319102843910059, 229.4271407816139856 ) ) ;
#41250=B_SPLINE_CURVE_WITH_KNOTS ( 'NONE', 3,
 ( #36058, #10856, #95404, #80811, #20881, #104352, #97067 ),
 .UNSPECIFIED., .F., .F.,
 ( 4, 3, 4 ),
 ( 5.821231011620000118, 13.81665860822499781, 14.11476443669999981 ),
 .UNSPECIFIED. ) ;
#41253=CARTESIAN_POINT ( 'NONE',  ( -0.7264217198650000373, 1457.949969450530034, 229.7272997097979896 ) ) ;
#41255=CARTESIAN_POINT ( 'NONE',  ( -44.43459082169709973, 1440.913052735869996, 270.0922309517229678 ) ) ;
#41260=CARTESIAN_POINT ( 'NONE',  ( -11.86654302293240093, 1432.368244302329913, 149.9823801698750003 ) ) ;
#41263=CARTESIAN_POINT ( 'NONE',  ( -24.91674476280000050, 1436.144616349540001, 137.7434857531980015 ) ) ;
#41265=CARTESIAN_POINT ( 'NONE',  ( -24.36140358970000008, 1441.380331911939948, 211.7116804488580044 ) ) ;
#41270=CARTESIAN_POINT ( 'NONE',  ( -13.13054719229040046, 1414.913526854310021, 220.1717702895670072 ) ) ;
#41271=EDGE_CURVE ( 'NONE', #71251, #80762, #42526, .T. ) ;
#41273=ORIENTED_EDGE ( 'NONE', *, *, #2427, .T. ) ;
#41274=CARTESIAN_POINT ( 'NONE',  ( -2.485061398530379773, 1451.956239371870197, 184.6525714882409943 ) ) ;
#41275=FACE_OUTER_BOUND ( 'NONE', #23471, .T. ) ;
#41276=CARTESIAN_POINT ( 'NONE',  ( -19.62068968046267514, 1457.036717113561963, 225.8553759409991244 ) ) ;
#41279=AXIS2_PLACEMENT_3D ( 'NONE', #17717, #77664, #25026 ) ;
#41280=EDGE_CURVE ( 'NONE', #5427, #43546, #825, .T. ) ;
#41282=CARTESIAN_POINT ( 'NONE',  ( -4.117520247412672418, 1441.433507593749027, 184.2698927454183035 ) ) ;
#41286=DIRECTION ( 'NONE',  ( -1.065814103640000080E-14, -1.000000000000000000, -2.775557561560010037E-16 ) ) ;
#41290=CARTESIAN_POINT ( 'NONE',  ( 41.20351478744365181, 1440.849789031605269, 135.3869887111343076 ) ) ;
#41291=CARTESIAN_POINT ( 'NONE',  ( 15.94345596297699963, 1409.469818137940138, 225.2684692625209948 ) ) ;
#41294=CARTESIAN_POINT ( 'NONE',  ( -12.78776258890000150, 1416.851343897030119, 195.9645815389980044 ) ) ;
#41296=CARTESIAN_POINT ( 'NONE',  ( 1.506876827590000190, 1419.080345689929800, 184.9340756889980071 ) ) ;
#41297=EDGE_CURVE ( 'NONE', #19483, #9730, #97012, .T. ) ;
#41300=B_SPLINE_CURVE_WITH_KNOTS ( 'NONE', 5,
 ( #17668, #102249, #101132, #102785, #110106, #24427 ),
 .UNSPECIFIED., .F., .F.,
 ( 6, 6 ),
 ( 0.000000000000000000, 1.000000000000000000 ),
 .UNSPECIFIED. ) ;
#41304=CARTESIAN_POINT ( 'NONE',  ( 17.66103185136753595, 1423.256579349406593, 226.2635097096822960 ) ) ;
#41305=CARTESIAN_POINT ( 'NONE',  ( 18.34194392892833392, 1425.469024528380032, 224.8862135115603564 ) ) ;
#41307=CARTESIAN_POINT ( 'NONE',  ( 43.48089572550729542, 1440.913060357599988, 263.7552761525859637 ) ) ;
#41316=CARTESIAN_POINT ( 'NONE',  ( -19.67975695282724402, 1485.238170136274221, 190.3376061193639828 ) ) ;
#41319=CARTESIAN_POINT ( 'NONE',  ( 9.314155605375137981, 1440.512919951834874, 186.6528570261106665 ) ) ;
#41320=ADVANCED_FACE ( 'NONE', ( #87051 ), #98201, .F. ) ;
#41321=CIRCLE ( 'NONE', #32366, 1.848467280504758614 ) ;
#41326=CARTESIAN_POINT ( 'NONE',  ( -14.46927441969999961, 1471.316885393030134, 193.6194182199980105 ) ) ;
#41327=CARTESIAN_POINT ( 'NONE',  ( -26.92366826496267151, 1508.479997278783912, 212.0212860892887647 ) ) ;
#41328=CARTESIAN_POINT ( 'NONE',  ( -10.98084453577630093, 1433.016921785290151, 151.7694248368179899 ) ) ;
#41331=ORIENTED_EDGE ( 'NONE', *, *, #97715, .T. ) ;
#41336=ORIENTED_EDGE ( 'NONE', *, *, #70277, .F. ) ;
#41337=AXIS2_PLACEMENT_3D ( 'NONE', #77657, #20479, #18279 ) ;
#41341=CARTESIAN_POINT ( 'NONE',  ( 1.443308927659999963, 1409.130619246129982, 231.7887507488979963 ) ) ;
#41351=CARTESIAN_POINT ( 'NONE',  ( 18.12087390759399952, 1425.009392209530006, 225.3858863835779971 ) ) ;
#41354=CARTESIAN_POINT ( 'NONE',  ( -2.708033116823189701, 1440.599352780370054, 162.2211373591810002 ) ) ;
#41355=CARTESIAN_POINT ( 'NONE',  ( -2.167054049770140267, 1450.334844765639900, 183.7367558523040145 ) ) ;
#41358=CARTESIAN_POINT ( 'NONE',  ( 18.86441005807279936, 1457.254199909039926, 227.0288101415989956 ) ) ;
#41359=CYLINDRICAL_SURFACE ( 'NONE', #76893, 26.99999999999999289 ) ;
#41362=CARTESIAN_POINT ( 'NONE',  ( -5.634996128403319327E-09, 1475.539493321410191, 266.4014118970719665 ) ) ;
#41363=CARTESIAN_POINT ( 'NONE',  ( -19.92782875493840322, 1486.092669036620009, 191.0199231053420021 ) ) ;
#41366=AXIS2_PLACEMENT_3D ( 'NONE', #25723, #103549, #68330 ) ;
#41367=( BOUNDED_CURVE ( )  B_SPLINE_CURVE ( 3, ( #57296, #3586, #56720, #72972 ),
 .UNSPECIFIED., .F., .T. ) 
 B_SPLINE_CURVE_WITH_KNOTS ( ( 4, 4 ),
 ( 4.711836388641210682, 5.211837385119190813 ),
 .UNSPECIFIED. ) 
 CURVE ( )  GEOMETRIC_REPRESENTATION_ITEM ( )  RATIONAL_B_SPLINE_CURVE ( ( 1.000000000000000000, 0.9792748656294838483, 0.9792748656294838483, 1.000000000000000000 ) ) 
 REPRESENTATION_ITEM ( '' )  );
#41368=CARTESIAN_POINT ( 'NONE',  ( -1.027602790635403940, 1484.904666167705045, 182.1256391034334001 ) ) ;
#41375=CARTESIAN_POINT ( 'NONE',  ( 6.972733162820000885, 1409.156553594830029, 222.0127823373979936 ) ) ;
#41378=CIRCLE ( 'NONE', #98587, 39.03564169359999170 ) ;
#41379=CARTESIAN_POINT ( 'NONE',  ( -26.23819217370180112, 1451.260861365519986, 136.3865425181880084 ) ) ;
#41381=CARTESIAN_POINT ( 'NONE',  ( -1.492328960440000234E-08, 1421.349368237830049, 217.1428156467079873 ) ) ;
#41383=CARTESIAN_POINT ( 'NONE',  ( -17.59268554400000184, 1410.455475221230017, 194.0661810319979850 ) ) ;
#41388=CARTESIAN_POINT ( 'NONE',  ( 0.2174505330332355268, 1415.406392250408317, 233.4370360999116087 ) ) ;
#41389=CARTESIAN_POINT ( 'NONE',  ( -11.60004869885203682, 1428.983126981193436, 134.0999999980979851 ) ) ;
#41390=ORIENTED_EDGE ( 'NONE', *, *, #94644, .F. ) ;
#41392=CARTESIAN_POINT ( 'NONE',  ( 13.07195414875639905, 1420.782728793139995, 229.6046982246629966 ) ) ;
#41394=ORIENTED_EDGE ( 'NONE', *, *, #39244, .T. ) ;
#41395=ORIENTED_EDGE ( 'NONE', *, *, #109532, .F. ) ;
#41397=CARTESIAN_POINT ( 'NONE',  ( -24.14721334009210096, 1411.115368492089829, 209.1440074703779999 ) ) ;
#41400=CARTESIAN_POINT ( 'NONE',  ( -44.91577693743988675, 1434.529242213127191, 266.2100843130238559 ) ) ;
#41402=CARTESIAN_POINT ( 'NONE',  ( -16.67592638840000063, 1498.345628701330043, 229.8334741389980138 ) ) ;
#41404=VERTEX_POINT ( 'NONE', #31546 ) ;
#41405=CARTESIAN_POINT ( 'NONE',  ( 44.41064987292289601, 1449.900485654209888, 266.4579286601659760 ) ) ;
#41407=FACE_OUTER_BOUND ( 'NONE', #27481, .T. ) ;
#41409=CIRCLE ( 'NONE', #272, 39.03564169359999170 ) ;
#41411=CARTESIAN_POINT ( 'NONE',  ( 18.74615377336336763, 1458.186127939198286, 227.2766744674128461 ) ) ;
#41413=SPHERICAL_SURFACE ( 'NONE', #110546, 2.000000000000000000 ) ;
#41414=ORIENTED_EDGE ( 'NONE', *, *, #97715, .F. ) ;
#41415=CARTESIAN_POINT ( 'NONE',  ( 2.664669577620000229, 1448.940583421350084, 183.3789499996979941 ) ) ;
#41417=CARTESIAN_POINT ( 'NONE',  ( 26.61928075775020019, 1451.917450893630075, 135.4298136244730131 ) ) ;
#41419=CARTESIAN_POINT ( 'NONE',  ( 3.363656671351779703, 1452.795598908070133, 152.3302338689809687 ) ) ;
#41422=CARTESIAN_POINT ( 'NONE',  ( 22.29596073799999800, 1409.691652492829917, 210.9314411838980163 ) ) ;
#41424=CARTESIAN_POINT ( 'NONE',  ( 1.791777137004639808, 1408.975630623710003, 186.8710971495229956 ) ) ;
#41427=CARTESIAN_POINT ( 'NONE',  ( 4.220605471363215067, 1441.596061467261961, 170.5366720304299974 ) ) ;
#41428=EDGE_CURVE ( 'NONE', #8770, #49915, #376, .T. ) ;
#41432=CARTESIAN_POINT ( 'NONE',  ( 12.25440271872080089, 1415.429375168339902, 221.8382653057779805 ) ) ;
#41433=CARTESIAN_POINT ( 'NONE',  ( 11.58617225630350056, 1432.339219477939878, 151.0669298090909933 ) ) ;
#41434=CARTESIAN_POINT ( 'NONE',  ( -14.35518320136639936, 1509.483853104240097, 182.9676327163749932 ) ) ;
#41441=CARTESIAN_POINT ( 'NONE',  ( -30.40113726820000295, 1448.202175313850148, 255.3819207742980097 ) ) ;
#41444=CARTESIAN_POINT ( 'NONE',  ( 40.73184307449999864, 1440.913060387330006, 268.3665355201979992 ) ) ;
#41446=CARTESIAN_POINT ( 'NONE',  ( -15.97231422325309858, 1420.661169593619888, 229.0305620570229905 ) ) ;
#41450=DIRECTION ( 'NONE',  ( 0.03489949670250328678, 0.9993908270190956511, 0.000000000000000000 ) ) ;
#41451=CARTESIAN_POINT ( 'NONE',  ( -16.28816891670000189, 1409.481855779529951, 224.8535106610980279 ) ) ;
#41453=VECTOR ( 'NONE', #43387, 1000.000000000000000 ) ;
#41456=CARTESIAN_POINT ( 'NONE',  ( -17.60613511254510044, 1410.891461967290070, 193.0293542103540005 ) ) ;
#41457=CARTESIAN_POINT ( 'NONE',  ( 1.352725010051470031E-06, 1408.141559141799917, 195.7211362560979921 ) ) ;
#41461=CARTESIAN_POINT ( 'NONE',  ( -1.546872636329999828, 1416.828040559629926, 228.0209234244979655 ) ) ;
#41463=VECTOR ( 'NONE', #7742, 1000.000000000000000 ) ;
#41464=CARTESIAN_POINT ( 'NONE',  ( 0.1725211256299399865, 1478.850466436460010, 182.1437687294350098 ) ) ;
#41468=CARTESIAN_POINT ( 'NONE',  ( -27.48389906189999721, 1443.913060387330006, 168.8435737885979790 ) ) ;
#41469=CARTESIAN_POINT ( 'NONE',  ( -6.291725117431780312, 1441.035272557219969, 154.5485622712799909 ) ) ;
#41470=CARTESIAN_POINT ( 'NONE',  ( 11.94102939159999899, 1433.615517387009959, 149.9804957290979814 ) ) ;
#41471=CARTESIAN_POINT ( 'NONE',  ( -41.31139259188770296, 1441.358669517780072, 134.0999999980719792 ) ) ;
#41481=CARTESIAN_POINT ( 'NONE',  ( 2.987353644710000200, 1434.208463618870155, 184.4752811826979837 ) ) ;
#41485=EDGE_LOOP ( 'NONE', ( #22059, #7698, #67923, #58334 ) ) ;
#41486=CARTESIAN_POINT ( 'NONE',  ( -28.55763293120000057, 1451.763088273230096, 135.7446055613980036 ) ) ;
#41488=CARTESIAN_POINT ( 'NONE',  ( -15.73449429231209962, 1409.488492326539927, 225.5890253965289958 ) ) ;
#41492=CARTESIAN_POINT ( 'NONE',  ( -19.18702366623263345, 1410.944745777546132, 222.6092016983794508 ) ) ;
#41495=CARTESIAN_POINT ( 'NONE',  ( -5.205339500303640676, 1440.970228300089957, 155.0076768945519916 ) ) ;
#41497=CARTESIAN_POINT ( 'NONE',  ( 18.23339910126861696, 1435.524963833022184, 214.8813641882896661 ) ) ;
#41501=CARTESIAN_POINT ( 'NONE',  ( 22.65255995593916793, 1509.725411181612344, 190.0317360007398406 ) ) ;
#41505=CARTESIAN_POINT ( 'NONE',  ( 4.283011301580000207, 1446.850650613710059, 156.0811442086979923 ) ) ;
#41507=CARTESIAN_POINT ( 'NONE',  ( 14.20204665139999989, 1416.837080243330092, 196.5054414751979834 ) ) ;
#41513=CARTESIAN_POINT ( 'NONE',  ( -22.14280421120000142, 1430.347761830729951, 200.3259973920780226 ) ) ;
#41514=CARTESIAN_POINT ( 'NONE',  ( -11.73643846425350112, 1426.280394569859936, 144.1643001077410133 ) ) ;
#41515=CARTESIAN_POINT ( 'NONE',  ( 16.02348580795440114, 1409.472571313510116, 192.9354709474999936 ) ) ;
#41517=CARTESIAN_POINT ( 'NONE',  ( 41.00233898590440162, 1442.023813499529979, 136.7354043627939859 ) ) ;
#41522=CARTESIAN_POINT ( 'NONE',  ( -2.233190733192939703, 1509.062325976219881, 179.3893463272050042 ) ) ;
#41523=CARTESIAN_POINT ( 'NONE',  ( 16.95828785292910368, 1460.444661627857840, 228.7722236097744712 ) ) ;
#41526=CARTESIAN_POINT ( 'NONE',  ( -33.91369265678890343, 1437.010538859309918, 136.5611844326260211 ) ) ;
#41527=ORIENTED_EDGE ( 'NONE', *, *, #73558, .T. ) ;
#41530=VERTEX_POINT ( 'NONE', #93639 ) ;
#41534=DIRECTION ( 'NONE',  ( -1.000000000000000000, 0.000000000000000000, 0.000000000000000000 ) ) ;
#41538=CARTESIAN_POINT ( 'NONE',  ( 11.75889809420000098, 1441.171049811090143, 188.0932782936979777 ) ) ;
#41539=CARTESIAN_POINT ( 'NONE',  ( 36.37832876739999932, 1435.767865857460265, 134.0999984849980251 ) ) ;
#41548=ORIENTED_EDGE ( 'NONE', *, *, #15873, .T. ) ;
#41549=CARTESIAN_POINT ( 'NONE',  ( 11.75361422675159950, 1426.796514659970171, 145.3264244949029944 ) ) ;
#41551=EDGE_LOOP ( 'NONE', ( #79559, #94833, #10523, #46031 ) ) ;
#41552=CARTESIAN_POINT ( 'NONE',  ( -13.97021087459999933, 1416.254459046630018, 221.7771524697980112 ) ) ;
#41553=ADVANCED_FACE ( 'NONE', ( #51123 ), #110829, .T. ) ;
#41554=CARTESIAN_POINT ( 'NONE',  ( -12.29654148988069373, 1442.773887286368335, 164.4841150006940325 ) ) ;
#41556=B_SPLINE_CURVE_WITH_KNOTS ( 'NONE', 5,
 ( #56030, #64447, #81210, #91816, #56581, #81754 ),
 .UNSPECIFIED., .F., .F.,
 ( 6, 6 ),
 ( 0.000000000000000000, 1.000000000000000000 ),
 .UNSPECIFIED. ) ;
#41558=CARTESIAN_POINT ( 'NONE',  ( -12.97083089140000034, 1419.897565124330185, 222.0283718032980005 ) ) ;
#41561=CARTESIAN_POINT ( 'NONE',  ( -10.07044770968007086, 1410.639375716134509, 188.4534418757513663 ) ) ;
#41563=CARTESIAN_POINT ( 'NONE',  ( 25.17408349516659882, 1470.080148438860078, 206.2206069998139810 ) ) ;
#41564=CARTESIAN_POINT ( 'NONE',  ( 14.06063856439999959, 1462.621720260530083, 230.5467405163980175 ) ) ;
#41565=CARTESIAN_POINT ( 'NONE',  ( -1.748115639427892942, 1451.913200175966722, 184.1800637472881021 ) ) ;
#41566=DIRECTION ( 'NONE',  ( 0.7067700363771036720, 0.03085824620770448445, -0.7067700363771035610 ) ) ;
#41569=CARTESIAN_POINT ( 'NONE',  ( 18.05238084035439883, 1424.492099674600013, 224.2916874381059813 ) ) ;
#41573=CARTESIAN_POINT ( 'NONE',  ( -2.923257245691396555, 1484.976779218816773, 183.1526432644509725 ) ) ;
#41574=CARTESIAN_POINT ( 'NONE',  ( -11.60004869885203682, 1426.385955719393905, 138.5855947434999962 ) ) ;
#41577=CARTESIAN_POINT ( 'NONE',  ( 0.5988589531109999031, 1507.637957906029897, 186.4745305517980114 ) ) ;
#41580=CARTESIAN_POINT ( 'NONE',  ( -11.18028693329999967, 1425.314180641229996, 146.2031382805980115 ) ) ;
#41586=CARTESIAN_POINT ( 'NONE',  ( -21.25027440960000291, 1495.370426451130015, 226.3512016020980013 ) ) ;
#41589=ORIENTED_EDGE ( 'NONE', *, *, #109763, .T. ) ;
#41591=CARTESIAN_POINT ( 'NONE',  ( 4.991045909560000382, 1405.947371129429939, 267.5267951891979692 ) ) ;
#41593=CARTESIAN_POINT ( 'NONE',  ( 19.25987197789999783, 1430.303363230129889, 194.0063009370979898 ) ) ;
#41596=CARTESIAN_POINT ( 'NONE',  ( -1.514430937639999808, 1450.835264095519960, 183.4743802333980227 ) ) ;
#41598=CARTESIAN_POINT ( 'NONE',  ( 15.44143521737569991, 1490.297619048229990, 194.0665802802050166 ) ) ;
#41600=CARTESIAN_POINT ( 'NONE',  ( -12.89353471100000093, 1445.498271942709835, 187.5282893900980241 ) ) ;
#41601=CARTESIAN_POINT ( 'NONE',  ( 18.89959486413309975, 1416.839692127159879, 210.6687135792209915 ) ) ;
#41603=CARTESIAN_POINT ( 'NONE',  ( 7.595213675750000171, 1408.121098801730113, 270.1248737335980081 ) ) ;
#41604=CARTESIAN_POINT ( 'NONE',  ( 1.449210345413849854, 1506.595259686350118, 181.1359157415290042 ) ) ;
#41605=CARTESIAN_POINT ( 'NONE',  ( -9.145222436720001014, 1428.303966710330087, 214.3676144197979738 ) ) ;
#41608=CARTESIAN_POINT ( 'NONE',  ( -9.935412840599997963, 1475.334996326929968, 267.8131885700980206 ) ) ;
#41609=CARTESIAN_POINT ( 'NONE',  ( 11.36018337630000019, 1414.996442546230128, 222.2791104318980047 ) ) ;
#41610=CARTESIAN_POINT ( 'NONE',  ( -22.52564151159999639, 1509.699673122230024, 190.3321270482979912 ) ) ;
#41611=CARTESIAN_POINT ( 'NONE',  ( -19.34729233231120205, 1486.470064436709890, 189.5887045964369975 ) ) ;
#41614=CARTESIAN_POINT ( 'NONE',  ( -6.510459374210000760, 1435.947057077009958, 154.7340827710979738 ) ) ;
#41617=FACE_OUTER_BOUND ( 'NONE', #77147, .T. ) ;
#41618=CARTESIAN_POINT ( 'NONE',  ( -19.54165211589999629, 1410.091287196029953, 197.8089316916980067 ) ) ;
#41622=CARTESIAN_POINT ( 'NONE',  ( -1.300519565079999921E-15, 1440.444625599219989, 150.6821045058979962 ) ) ;
#41626=CARTESIAN_POINT ( 'NONE',  ( 11.42701431400000089, 1425.487255414029960, 143.4621352013980129 ) ) ;
#41628=CARTESIAN_POINT ( 'NONE',  ( 11.73351217698500015, 1426.698186165599964, 143.9179939085790068 ) ) ;
#41629=SPHERICAL_SURFACE ( 'NONE', #23581, 2.000000000550000046 ) ;
#41632=CARTESIAN_POINT ( 'NONE',  ( -17.15874760866699944, 1507.620489300740019, 224.4056177524859947 ) ) ;
#41635=CARTESIAN_POINT ( 'NONE',  ( -9.559188306630000298, 1428.004395111430085, 145.6094494780980142 ) ) ;
#41639=FACE_OUTER_BOUND ( 'NONE', #88917, .T. ) ;
#41642=ORIENTED_EDGE ( 'NONE', *, *, #32901, .F. ) ;
#41643=CARTESIAN_POINT ( 'NONE',  ( 12.02044816154730178, 1433.916076607059949, 150.4036537052579945 ) ) ;
#41644=CARTESIAN_POINT ( 'NONE',  ( -7.930219352209999073, 1398.148604353429846, 219.9854233436979882 ) ) ;
#41647=CARTESIAN_POINT ( 'NONE',  ( -25.61067805310000267, 1508.555235019130123, 199.5030921420180050 ) ) ;
#41650=CARTESIAN_POINT ( 'NONE',  ( -14.32200080931659869, 1509.463657562170056, 183.0292320648689781 ) ) ;
#41651=CARTESIAN_POINT ( 'NONE',  ( 10.70473176346070154, 1498.104840791710103, 233.7592016339740155 ) ) ;
#41652=B_SPLINE_CURVE_WITH_KNOTS ( 'NONE', 3,
 ( #103161, #77983, #9126, #200 ),
 .UNSPECIFIED., .F., .F.,
 ( 4, 4 ),
 ( 0.000000000000000000, 1.000000000000000000 ),
 .UNSPECIFIED. ) ;
#41653=CARTESIAN_POINT ( 'NONE',  ( 15.28119998530000068, 1449.230982227970117, 190.0712285711979916 ) ) ;
#41654=CARTESIAN_POINT ( 'NONE',  ( 3.048828143997139861, 1509.019527812190063, 237.9289388395170306 ) ) ;
#41657=CARTESIAN_POINT ( 'NONE',  ( 1.435225544770050154, 1395.963179567740099, 198.2036689045829974 ) ) ;
#41658=CARTESIAN_POINT ( 'NONE',  ( 0.9667867126429999791, 1415.996778984329922, 190.4114842333980278 ) ) ;
#41659=CARTESIAN_POINT ( 'NONE',  ( 11.56574130529999955, 1431.513070563570182, 151.1467947063979977 ) ) ;
#41662=CARTESIAN_POINT ( 'NONE',  ( 13.04027018280589978, 1434.994425313320107, 149.9717208830880111 ) ) ;
#41665=CARTESIAN_POINT ( 'NONE',  ( 13.13752534233263347, 1444.768944423229641, 169.4002553938786946 ) ) ;
#41666=CARTESIAN_POINT ( 'NONE',  ( -11.13364320589999856, 1462.223842109729958, 233.3656537020980011 ) ) ;
#41667=CARTESIAN_POINT ( 'NONE',  ( -4.219439073160000220, 1446.230224797059918, 170.2811368938980081 ) ) ;
#41670=ORIENTED_EDGE ( 'NONE', *, *, #20821, .F. ) ;
#41672=CARTESIAN_POINT ( 'NONE',  ( -1.797631911580000130, 1415.838340813430023, 185.8046423929979767 ) ) ;
#41674=EDGE_LOOP ( 'NONE', ( #40391, #36381, #63799, #68893 ) ) ;
#41679=CARTESIAN_POINT ( 'NONE',  ( -12.26976426819999944, 1410.715041853229877, 189.3560318399979963 ) ) ;
#41681=CARTESIAN_POINT ( 'NONE',  ( 0.3551244063982409993, 1416.218047878440075, 227.0926723912329805 ) ) ;
#41682=VERTEX_POINT ( 'NONE', #35416 ) ;
#41683=CARTESIAN_POINT ( 'NONE',  ( 23.64707162479999880, 1434.553497323629927, 214.9047861787279885 ) ) ;
#41685=CARTESIAN_POINT ( 'NONE',  ( 3.156166260290000025, 1466.544008048530031, 236.1241471695980181 ) ) ;
#41687=CARTESIAN_POINT ( 'NONE',  ( 15.04635084860490046, 1411.118372808829918, 270.3649387868580334 ) ) ;
#41689=CARTESIAN_POINT ( 'NONE',  ( 23.98506269609999819, 1411.113951130829946, 208.3864704457530195 ) ) ;
#41695=CARTESIAN_POINT ( 'NONE',  ( 2.685928792098830620, 1419.763152350967857, 137.0999999980978430 ) ) ;
#41699=CARTESIAN_POINT ( 'NONE',  ( 36.92076361760000225, 1453.101244315629856, 259.2255047987979992 ) ) ;
#41702=CARTESIAN_POINT ( 'NONE',  ( -5.483186321339999836, 1439.280902240999922, 154.7474923763980144 ) ) ;
#41709=B_SPLINE_CURVE_WITH_KNOTS ( 'NONE', 5,
 ( #55345, #56439, #73234, #81611, #29032, #30107 ),
 .UNSPECIFIED., .F., .F.,
 ( 6, 6 ),
 ( 0.000000000000000000, 11.48858425020000240 ),
 .UNSPECIFIED. ) ;
#41712=CARTESIAN_POINT ( 'NONE',  ( -27.03405935060176901, 1451.816840469728959, 135.7882905775978770 ) ) ;
#41713=CARTESIAN_POINT ( 'NONE',  ( 12.55018658110000196, 1419.800154493929995, 223.5686081623980215 ) ) ;
#41714=CARTESIAN_POINT ( 'NONE',  ( 38.61927353243170558, 1444.188088105049928, 137.1592452208769828 ) ) ;
#41715=CARTESIAN_POINT ( 'NONE',  ( -5.851191224163104110, 1425.133440372593213, 186.4975237928585443 ) ) ;
#41717=CARTESIAN_POINT ( 'NONE',  ( -24.15153490410000359, 1438.063247892820073, 212.1983423404379892 ) ) ;
#41718=B_SPLINE_CURVE_WITH_KNOTS ( 'NONE', 5,
 ( #18566, #52216, #53893, #96412, #95852, #87467 ),
 .UNSPECIFIED., .F., .F.,
 ( 6, 6 ),
 ( -1.452596962060000108, -1.327391353722617851E-06 ),
 .UNSPECIFIED. ) ;
#41719=CARTESIAN_POINT ( 'NONE',  ( 27.34169570636690239, 1435.928060154659988, 136.5046493440970039 ) ) ;
#41720=CARTESIAN_POINT ( 'NONE',  ( 40.12924064502020371, 1445.213485489899995, 136.9285573339909945 ) ) ;
#41721=CARTESIAN_POINT ( 'NONE',  ( 16.68563273243293210, 1506.380977035248861, 223.4251768443501760 ) ) ;
#41722=PLANE ( 'NONE',  #109310 ) ;
#41724=CARTESIAN_POINT ( 'NONE',  ( 10.95491197589999999, 1509.295614343230227, 182.0238867766980206 ) ) ;
#41726=CARTESIAN_POINT ( 'NONE',  ( -38.63865849408829689, 1452.914171151027176, 269.5870376815316831 ) ) ;
#41727=EDGE_LOOP ( 'NONE', ( #48183, #99906, #88110, #13476 ) ) ;
#41734=CARTESIAN_POINT ( 'NONE',  ( -0.1681681984989999989, 1405.973120458222411, 137.0999999980979851 ) ) ;
#41737=CARTESIAN_POINT ( 'NONE',  ( -10.99560576475330542, 1418.486348324287064, 229.4293017187473538 ) ) ;
#41738=CARTESIAN_POINT ( 'NONE',  ( -20.54020145117927498, 1450.964032953651895, 144.9884247554932415 ) ) ;
#41740=CARTESIAN_POINT ( 'NONE',  ( 25.00561208829999771, 1436.149542637609784, 137.5831833732979987 ) ) ;
#41743=CARTESIAN_POINT ( 'NONE',  ( -0.3142797416910570463, 1415.426207913209964, 191.6391945173240003 ) ) ;
#41747=CARTESIAN_POINT ( 'NONE',  ( 7.135682362486938324, 1445.817047258000457, 183.2676370014899589 ) ) ;
#41748=CARTESIAN_POINT ( 'NONE',  ( 12.87691439960000039, 1507.477875213329980, 233.2689574170979938 ) ) ;
#41750=CARTESIAN_POINT ( 'NONE',  ( -22.53808385540000003, 1454.461372222829823, 231.7546718361979856 ) ) ;
#41752=CARTESIAN_POINT ( 'NONE',  ( 4.396219768207910050, 1425.786877246529912, 185.4645489200509871 ) ) ;
#41754=CARTESIAN_POINT ( 'NONE',  ( -2.558108261982198428, 1420.763624677371809, 185.5735512640813170 ) ) ;
#41756=CARTESIAN_POINT ( 'NONE',  ( -14.63475337105202101, 1429.908932556607169, 222.0813138987385287 ) ) ;
#41760=CARTESIAN_POINT ( 'NONE',  ( -24.55563515408854158, 1509.884957629476048, 191.8160791308368402 ) ) ;
#41762=ORIENTED_EDGE ( 'NONE', *, *, #13293, .T. ) ;
#41763=ORIENTED_EDGE ( 'NONE', *, *, #73976, .T. ) ;
#41768=CARTESIAN_POINT ( 'NONE',  ( -5.165175409120000616, 1471.356177552630015, 269.6177996896980176 ) ) ;
#41769=CARTESIAN_POINT ( 'NONE',  ( 12.08137332695765842, 1433.867263877792993, 147.5406663739968565 ) ) ;
#41771=CARTESIAN_POINT ( 'NONE',  ( 14.60782360329999996, 1431.113060387329824, 195.8937821300980033 ) ) ;
#41774=EDGE_CURVE ( 'NONE', #77110, #5392, #76975, .T. ) ;
#41776=CARTESIAN_POINT ( 'NONE',  ( -17.83228018670000026, 1408.913060387329779, 204.9623371014980080 ) ) ;
#41779=CARTESIAN_POINT ( 'NONE',  ( -20.53126236479100086, 1409.661581851170013, 266.7933185538669818 ) ) ;
#41780=CARTESIAN_POINT ( 'NONE',  ( -13.68913941687680058, 1435.559263906229944, 150.0920709695850235 ) ) ;
#41781=EDGE_LOOP ( 'NONE', ( #66220, #98644, #44873, #53943 ) ) ;
#41783=VERTEX_POINT ( 'NONE', #43277 ) ;
#41785=CARTESIAN_POINT ( 'NONE',  ( -21.97938480444670262, 1506.433683733529961, 209.5040264213440082 ) ) ;
#41788=CARTESIAN_POINT ( 'NONE',  ( -17.09529087520000346, 1470.470234692029862, 189.0510684403979837 ) ) ;
#41789=CARTESIAN_POINT ( 'NONE',  ( -17.09199761692149977, 1498.340372574690036, 229.5617320311440039 ) ) ;
#41791=LINE ( 'NONE', #18229, #1037 ) ;
#41792=EDGE_CURVE ( 'NONE', #4103, #108385, #1705, .T. ) ;
#41797=CARTESIAN_POINT ( 'NONE',  ( -1.398741533879999999, 1408.961905518030107, 194.4353072542980101 ) ) ;
#41800=CARTESIAN_POINT ( 'NONE',  ( 15.31956813402619666, 1506.436298853404651, 193.3531772691010815 ) ) ;
#41804=CARTESIAN_POINT ( 'NONE',  ( 26.43941340970000198, 1488.684867473429904, 213.7762971690580116 ) ) ;
#41807=CARTESIAN_POINT ( 'NONE',  ( 19.91508182626240142, 1477.278815843640132, 225.3081590611470233 ) ) ;
#41808=CARTESIAN_POINT ( 'NONE',  ( -11.49747572423030029, 1414.913060387329779, 197.9009878255399997 ) ) ;
#41809=CARTESIAN_POINT ( 'NONE',  ( -24.64589136669999903, 1442.596336934359897, 210.7637021778280086 ) ) ;
#41813=CARTESIAN_POINT ( 'NONE',  ( 5.500900010980000587, 1439.900099495240056, 154.7565255832979858 ) ) ;
#41814=FACE_OUTER_BOUND ( 'NONE', #62257, .T. ) ;
#41815=CARTESIAN_POINT ( 'NONE',  ( 3.831162495979924643, 1440.893596831928335, 156.3803834073238477 ) ) ;
#41817=ORIENTED_EDGE ( 'NONE', *, *, #76661, .T. ) ;
#41818=CARTESIAN_POINT ( 'NONE',  ( -38.81202645930000017, 1436.797832437210218, 134.0999985825980332 ) ) ;
#41820=CARTESIAN_POINT ( 'NONE',  ( -19.86778455305866942, 1456.672304896796277, 225.4249518172526052 ) ) ;
#41821=ORIENTED_EDGE ( 'NONE', *, *, #90435, .T. ) ;
#41825=FACE_OUTER_BOUND ( 'NONE', #58214, .T. ) ;
#41827=AXIS2_PLACEMENT_3D ( 'NONE', #7101, #48571, #22216 ) ;
#41828=CARTESIAN_POINT ( 'NONE',  ( 2.451271202390000070, 1433.447543843880112, 150.3250444719979839 ) ) ;
#41830=FACE_OUTER_BOUND ( 'NONE', #26947, .T. ) ;
#41831=CARTESIAN_POINT ( 'NONE',  ( 4.223051414464590536, 1441.592138948940146, 167.3011229986659885 ) ) ;
#41833=DIRECTION ( 'NONE',  ( 0.000000000000000000, -1.000000000000000000, -2.312964634635740689E-15 ) ) ;
#41834=CARTESIAN_POINT ( 'NONE',  ( 20.84366507899999732, 1509.634592532730039, 188.2028936218980277 ) ) ;
#41837=CARTESIAN_POINT ( 'NONE',  ( -12.73024483699999898, 1416.833018152729892, 195.1128574262980067 ) ) ;
#41846=CARTESIAN_POINT ( 'NONE',  ( 1.807048120887469578, 1416.685803381123378, 232.7081437053816728 ) ) ;
#41847=CARTESIAN_POINT ( 'NONE',  ( 17.70041754922767296, 1423.341415640119749, 226.2080326948689901 ) ) ;
#41848=CARTESIAN_POINT ( 'NONE',  ( 18.45217032144871894, 1425.619926260229931, 224.9274540208776330 ) ) ;
#41850=CARTESIAN_POINT ( 'NONE',  ( 43.27085592825979887, 1440.913060356199821, 263.5081753078439988 ) ) ;
#41852=CARTESIAN_POINT ( 'NONE',  ( 0.000000000000000000, 1519.913060387329779, 233.4018459616980010 ) ) ;
#41855=VERTEX_POINT ( 'NONE', #21881 ) ;
#41856=B_SPLINE_CURVE_WITH_KNOTS ( 'NONE', 3,
 ( #68067, #93762, #102179, #33875, #33315, #102714, #67510, #51802, #24900, #9244, #35535, #27148, #93232, #17040, #51237, #85370, #52369, #85942, #34437, #84819, #69163 ),
 .UNSPECIFIED., .F., .F.,
 ( 4, 2, 1, 1, 1, 2, 2, 2, 2, 2, 2, 4 ),
 ( 0.000000000000000000, 1.207358997277241904E-05, 2.414717994554483807E-05, 4.829435989153836644E-05, 9.658871978357142722E-05, 0.0001931774395680907182, 0.0003863548791367152433, 0.0007727097582739642393, 0.001159064637411213235, 0.001352242076979837679, 0.001448830796764309387, 0.001545419516548780878 ),
 .UNSPECIFIED. ) ;
#41858=EDGE_CURVE ( 'NONE', #70574, #98399, #64886, .T. ) ;
#41859=CARTESIAN_POINT ( 'NONE',  ( 17.22354464511785821, 1410.184082523955794, 192.5759529289406942 ) ) ;
#41860=CARTESIAN_POINT ( 'NONE',  ( -24.34268787264259970, 1442.549328851149994, 212.2035684885649687 ) ) ;
#41861=CARTESIAN_POINT ( 'NONE',  ( 2.273290303349758457, 1410.370752790504412, 185.5123687935691237 ) ) ;
#41863=CARTESIAN_POINT ( 'NONE',  ( 16.19492410460000187, 1409.478599598930032, 217.9908631324380224 ) ) ;
#41864=CARTESIAN_POINT ( 'NONE',  ( 18.49631469930000094, 1416.851343894929869, 209.5335333753989744 ) ) ;
#41868=CARTESIAN_POINT ( 'NONE',  ( 22.80545758519999922, 1450.887189432959758, 142.4385674641980017 ) ) ;
#41869=( BOUNDED_CURVE ( )  B_SPLINE_CURVE ( 3, ( #32571, #91376, #82967, #6261 ),
 .UNSPECIFIED., .F., .F. ) 
 B_SPLINE_CURVE_WITH_KNOTS ( ( 4, 4 ),
 ( 4.704954595420359986, 5.211301734500129790 ),
 .UNSPECIFIED. ) 
 CURVE ( )  GEOMETRIC_REPRESENTATION_ITEM ( )  RATIONAL_B_SPLINE_CURVE ( ( 1.000000000000000000, 0.9787482600944612532, 0.9787482600944612532, 1.000000000000000000 ) ) 
 REPRESENTATION_ITEM ( '' )  );
#41874=CARTESIAN_POINT ( 'NONE',  ( -15.13342374508840038, 1507.606285602760181, 191.8462590464540085 ) ) ;
#41879=ORIENTED_EDGE ( 'NONE', *, *, #95879, .T. ) ;
#41882=CARTESIAN_POINT ( 'NONE',  ( 36.34707484411779888, 1437.575034581910131, 136.5422136037309713 ) ) ;
#41885=CIRCLE ( 'NONE', #36539, 10.00000000000000000 ) ;
#41889=CARTESIAN_POINT ( 'NONE',  ( -0.4299350982835939416, 1451.092099702937730, 182.2245401379511520 ) ) ;
#41890=CARTESIAN_POINT ( 'NONE',  ( 18.95790016943493939, 1509.575089211102750, 186.6267876694127779 ) ) ;
#41892=EDGE_CURVE ( 'NONE', #55821, #57154, #90207, .T. ) ;
#41893=CARTESIAN_POINT ( 'NONE',  ( 3.022804847239999759, 1409.018619058630065, 186.7640392999980179 ) ) ;
#41896=CARTESIAN_POINT ( 'NONE',  ( -4.222336330638260193, 1441.606005989779987, 166.9080596108109944 ) ) ;
#41898=CARTESIAN_POINT ( 'NONE',  ( -25.16854656449999794, 1451.224506337529874, 137.5711276817980320 ) ) ;
#41904=CARTESIAN_POINT ( 'NONE',  ( 19.46939419728449749, 1455.727202090050014, 226.4972727368899825 ) ) ;
#41909=CARTESIAN_POINT ( 'NONE',  ( -1.032992184830370031E-08, 1474.676908767299892, 264.7279807803609515 ) ) ;
#41911=CARTESIAN_POINT ( 'NONE',  ( -0.7133824534919999127, 1416.822690122329959, 227.9183239597979878 ) ) ;
#41917=CARTESIAN_POINT ( 'NONE',  ( -45.59497939955269885, 1438.873046339160055, 266.1906450788720235 ) ) ;
#41920=ADVANCED_FACE ( 'NONE', ( #109648 ), #73441, .T. ) ;
#41923=B_SPLINE_CURVE_WITH_KNOTS ( 'NONE', 3,
 ( #48621, #100104, #99532, #24478, #74923, #101182, #67078, #32354, #6045, #82753, #13314, #14424, #107395, #49169, #90037, #73256, #22816, #40196 ),
 .UNSPECIFIED., .F., .F.,
 ( 4, 2, 2, 2, 2, 2, 2, 2, 4 ),
 ( 0.000000000000000000, 0.07958679019459939663, 0.1577458466451709951, 0.2359250078159189912, 0.2750922612652370036, 0.2946660706215870063, 0.3044518104690189797, 0.3144120845289309907, 0.3151965516711889848 ),
 .UNSPECIFIED. ) ;
#41924=CARTESIAN_POINT ( 'NONE',  ( -27.69925886641940238, 1441.434395751479997, 137.3015763626259798 ) ) ;
#41926=EDGE_CURVE ( 'NONE', #58564, #71251, #15462, .T. ) ;
#41927=CARTESIAN_POINT ( 'NONE',  ( -26.16688589682070187, 1451.542564073259882, 136.1869649791260315 ) ) ;
#41929=CARTESIAN_POINT ( 'NONE',  ( 25.15583052850000101, 1439.261431119660074, 217.2951522780279845 ) ) ;
#41931=CARTESIAN_POINT ( 'NONE',  ( 15.51935361379999989, 1506.809279316930088, 193.4756025686980081 ) ) ;
#41934=CARTESIAN_POINT ( 'NONE',  ( -12.93678125246493771, 1396.364822743412560, 207.0732903518876924 ) ) ;
#41935=CARTESIAN_POINT ( 'NONE',  ( -13.58235846979999906, 1416.828040475229955, 221.9087530951979659 ) ) ;
#41938=CARTESIAN_POINT ( 'NONE',  ( -4.767656242956440416, 1410.583764236560228, 269.3374945991810137 ) ) ;
#41939=CARTESIAN_POINT ( 'NONE',  ( 16.63147820130039989, 1421.790408391879964, 227.0569735401810192 ) ) ;
#41943=EDGE_CURVE ( 'NONE', #5163, #68079, #58337, .T. ) ;
#41944=CARTESIAN_POINT ( 'NONE',  ( -24.02381549939999772, 1410.732491813230126, 209.5701859032720051 ) ) ;
#41946=DIRECTION ( 'NONE',  ( -1.000000000000000000, 0.000000000000000000, 0.000000000000000000 ) ) ;
#41947=CARTESIAN_POINT ( 'NONE',  ( -11.16223122930000144, 1428.970455832429934, 101.8807690336980016 ) ) ;
#41950=CARTESIAN_POINT ( 'NONE',  ( -1.581402563589999977, 1498.352608146529974, 236.7257605069980002 ) ) ;
#41951=CARTESIAN_POINT ( 'NONE',  ( -17.57163213930000012, 1410.882994532030125, 225.4813515594979947 ) ) ;
#41952=CARTESIAN_POINT ( 'NONE',  ( 45.59504749288019809, 1442.766519910440138, 268.9761053574069933 ) ) ;
#41953=CARTESIAN_POINT ( 'NONE',  ( -0.5656601614563600000, 1424.194575819369902, 228.0927458373740251 ) ) ;
#41954=CARTESIAN_POINT ( 'NONE',  ( -16.13553931567702193, 1420.899259742274353, 227.0324294037215225 ) ) ;
#41957=CARTESIAN_POINT ( 'NONE',  ( -11.14671771210699980, 1434.019356486030119, 151.6529807626459956 ) ) ;
#41961=CARTESIAN_POINT ( 'NONE',  ( 3.932342930579999507, 1448.638726228580026, 184.2846140409980364 ) ) ;
#41967=B_SPLINE_SURFACE_WITH_KNOTS ( 'NONE', 5, 5, ( 
 ( #24604, #59368, #93478, #68325, #66668, #75614 ),
 ( #5, #109747, #58798, #7286, #34139, #24062 ),
 ( #6178, #58256, #84538, #15648, #59918, #74513 ),
 ( #92376, #94038, #100246, #15114, #49304, #83429 ),
 ( #16209, #6726, #49854, #50413, #96260, #102979 ),
 ( #62135, #86195, #51497, #77805, #105216, #9487 ),
 ( #86751, #36346, #104102, #10041, #19535, #2230 ),
 ( #18415, #35805, #70538, #1664, #1114, #61035 ),
 ( #62703, #53743, #104655, #35243, #10603, #27952 ),
 ( #69429, #87878, #87310, #11169, #45329, #34688 ),
 ( #69985, #26277, #44774, #103544, #79468, #60467 ),
 ( #96822, #85630, #68878, #2778, #28504, #36898 ) ),
 .UNSPECIFIED., .F., .F., .F.,
 ( 6, 3, 3, 6 ),
 ( 6, 6 ),
 ( 6.182282359980000308, 12.54225916440000077, 24.91223976350000058, 34.19375089779999399 ),
 ( 0.1502731719950000100, 0.6000000000009999557 ),
 .UNSPECIFIED. ) ;
#41970=CARTESIAN_POINT ( 'NONE',  ( 1.748432842252070074, 1408.974117007579935, 186.8594775301320112 ) ) ;
#41971=CARTESIAN_POINT ( 'NONE',  ( 1.009298393719999964, 1415.944724089230021, 233.1672510863979824 ) ) ;
#41973=DIRECTION ( 'NONE',  ( -0.4438071788273494356, -0.8961223063964589564, 0.000000000000000000 ) ) ;
#41976=CARTESIAN_POINT ( 'NONE',  ( 13.87806392702616698, 1421.462115117653866, 230.8073813634572105 ) ) ;
#41979=AXIS2_PLACEMENT_3D ( 'NONE', #9783, #17601, #51236 ) ;
#41980=CARTESIAN_POINT ( 'NONE',  ( 11.83148343547229864, 1432.336211092349913, 150.3814746356140120 ) ) ;
#41982=EDGE_CURVE ( 'NONE', #27781, #72991, #20824, .T. ) ;
#41988=CARTESIAN_POINT ( 'NONE',  ( -38.34143788450000301, 1445.301772818269910, 265.6112251771979800 ) ) ;
#41989=CARTESIAN_POINT ( 'NONE',  ( -21.53951952428644745, 1509.203566254688440, 191.7343637106751828 ) ) ;
#41990=CARTESIAN_POINT ( 'NONE',  ( 11.92439245019999916, 1433.423794087070064, 149.9160333479979954 ) ) ;
#41991=CARTESIAN_POINT ( 'NONE',  ( 14.35418281399999962, 1450.996202460929908, 214.3676144200779845 ) ) ;
#41995=CARTESIAN_POINT ( 'NONE',  ( 2.760778564396810353, 1409.009468899150079, 230.1977509304229841 ) ) ;
#41999=DIRECTION ( 'NONE',  ( -5.612627869608440548E-17, -0.03489949670197409898, 0.9993908270191140808 ) ) ;
#42000=CARTESIAN_POINT ( 'NONE',  ( -17.38481315180000308, 1410.884446742730233, 225.7833460420979748 ) ) ;
#42001=CARTESIAN_POINT ( 'NONE',  ( 23.00452548930000063, 1430.350017905930144, 215.8863230596679728 ) ) ;
#42002=CARTESIAN_POINT ( 'NONE',  ( 4.703965987320000013E-16, 1428.579607037230062, 149.5143047311979672 ) ) ;
#42008=CARTESIAN_POINT ( 'NONE',  ( 0.1703894054731670271, 1480.100913143119897, 182.0900560439260119 ) ) ;
#42009=CARTESIAN_POINT ( 'NONE',  ( -10.80134480061109947, 1441.261220175989820, 153.0805715986579969 ) ) ;
#42011=CARTESIAN_POINT ( 'NONE',  ( -13.31869796660000027, 1444.740067931809790, 169.3753098992980028 ) ) ;
#42013=FACE_OUTER_BOUND ( 'NONE', #72012, .T. ) ;
#42015=CARTESIAN_POINT ( 'NONE',  ( -40.44958274777649621, 1439.458628679120011, 134.0999999981179940 ) ) ;
#42017=ORIENTED_EDGE ( 'NONE', *, *, #41428, .T. ) ;
#42019=AXIS2_PLACEMENT_3D ( 'NONE', #93433, #67714, #41946 ) ;
#42021=CARTESIAN_POINT ( 'NONE',  ( -15.03806458159999870, 1414.913060387229962, 216.3136682808679723 ) ) ;
#42023=EDGE_CURVE ( 'NONE', #47384, #84894, #87695, .T. ) ;
#42025=CARTESIAN_POINT ( 'NONE',  ( -12.78776258889159934, 1416.851343895820037, 195.9645815067300134 ) ) ;
#42027=DIRECTION ( 'NONE',  ( -0.3892484888175452573, 0.9211327884476036010, 0.000000000000000000 ) ) ;
#42031=VERTEX_POINT ( 'NONE', #7729 ) ;
#42032=CARTESIAN_POINT ( 'NONE',  ( -28.55009876189999574, 1451.915930383729801, 135.3068286921980246 ) ) ;
#42033=CARTESIAN_POINT ( 'NONE',  ( -15.79838181210750214, 1409.567131171960000, 225.8770295224450138 ) ) ;
#42034=FACE_OUTER_BOUND ( 'NONE', #20938, .T. ) ;
#42037=CARTESIAN_POINT ( 'NONE',  ( -21.64610633839767573, 1411.027676083505639, 216.2671881281004005 ) ) ;
#42041=CARTESIAN_POINT ( 'NONE',  ( 38.90111251957022631, 1452.461926335832231, 269.5912703700630573 ) ) ;
#42042=CARTESIAN_POINT ( 'NONE',  ( 17.94471134571137583, 1434.902817273550909, 215.4479691263156553 ) ) ;
#42047=CARTESIAN_POINT ( 'NONE',  ( 10.78330898009999927, 1453.313060387329870, 226.3563104863980016 ) ) ;
#42051=LINE ( 'NONE', #110348, #8977 ) ;
#42054=CARTESIAN_POINT ( 'NONE',  ( 14.45760372910000058, 1416.831925117829996, 196.8518845416979843 ) ) ;
#42056=ORIENTED_EDGE ( 'NONE', *, *, #70015, .T. ) ;
#42057=ADVANCED_FACE ( 'NONE', ( #19991 ), #21283, .F. ) ;
#42061=CARTESIAN_POINT ( 'NONE',  ( -25.36027075149999988, 1449.801358176479880, 206.9464496238279878 ) ) ;
#42062=CARTESIAN_POINT ( 'NONE',  ( -11.13172969966639947, 1426.040969812840103, 108.4495695014479963 ) ) ;
#42063=AXIS2_PLACEMENT_3D ( 'NONE', #70545, #71667, #72197 ) ;
#42064=CARTESIAN_POINT ( 'NONE',  ( 16.29451049919999761, 1409.859978110029942, 192.0605078528979845 ) ) ;
#42066=CARTESIAN_POINT ( 'NONE',  ( 18.29376482344865451, 1509.671222653318864, 185.3449578346911437 ) ) ;
#42067=CARTESIAN_POINT ( 'NONE',  ( 1.562525333773240543, 1450.589639673192551, 181.7027468294939183 ) ) ;
#42071=CARTESIAN_POINT ( 'NONE',  ( 17.11588712847992610, 1460.309517847519601, 228.6647148658520337 ) ) ;
#42079=ORIENTED_EDGE ( 'NONE', *, *, #15951, .T. ) ;
#42081=CARTESIAN_POINT ( 'NONE',  ( -29.67498122965860929, 1509.980309120330958, 210.3356156768038261 ) ) ;
#42088=CARTESIAN_POINT ( 'NONE',  ( 33.91369117179520032, 1451.728768195329849, 134.4205496120819987 ) ) ;
#42090=CIRCLE ( 'NONE', #49289, 1.560060070890045836 ) ;
#42091=CARTESIAN_POINT ( 'NONE',  ( 26.48466844540000054, 1437.480003640949917, 136.8777945664980109 ) ) ;
#42094=ORIENTED_EDGE ( 'NONE', *, *, #19568, .F. ) ;
#42098=CARTESIAN_POINT ( 'NONE',  ( 11.78445004594039958, 1427.574272142750033, 147.3232557260809870 ) ) ;
#42099=CARTESIAN_POINT ( 'NONE',  ( 20.08410857819999862, 1507.858969061830066, 229.0550880116979897 ) ) ;
#42101=CARTESIAN_POINT ( 'NONE',  ( -13.79555462530000121, 1416.822690122329959, 221.9085254461979844 ) ) ;
#42102=CARTESIAN_POINT ( 'NONE',  ( -16.90776107416510143, 1442.831169986189479, 162.4346387413914385 ) ) ;
#42106=CARTESIAN_POINT ( 'NONE',  ( 21.47248244664589834, 1409.703582322209968, 206.3643650589729930 ) ) ;
#42107=CARTESIAN_POINT ( 'NONE',  ( -8.085907062746878537, 1446.678893608761427, 154.0132172026529531 ) ) ;
#42109=CARTESIAN_POINT ( 'NONE',  ( -7.854300036778085747, 1410.563322333322276, 187.7028744996234764 ) ) ;
#42111=CARTESIAN_POINT ( 'NONE',  ( -15.58140587179999947, 1473.850404518229880, 223.6693376217980074 ) ) ;
#42115=B_SPLINE_SURFACE_WITH_KNOTS ( 'NONE', 5, 5, ( 
 ( #8207, #15498, #8761, #77101, #42373, #43497, #50253, #42942, #77641, #409, #50781, #51896, #92227, #84382, #34526, #60297, #94414, #953, #67600, #101159, #33405, #92775, #17692, #66513 ),
 ( #83826, #58095, #7126, #7668, #101709, #75455, #25001, #27785, #70935, #61418, #78746, #69821, #28340, #36741, #79304, #61974, #62535, #96088, #19364, #53567, #35628, #52456, #10992, #94994 ),
 ( #87712, #44045, #19925, #2616, #2061, #105051, #36193, #70377, #18262, #104494, #79858, #69258, #78184, #1495, #96656, #53008, #45164, #103939, #86586, #54125, #88252, #11545, #45720, #27237 ),
 ( #3168, #9877, #87142, #10432, #37300, #71493, #95541, #26669, #35078, #103366, #18813, #44603, #60868, #110504, #7490, #9692, #50064, #8035, #8585, #34349, #16957, #43860, #25371, #59017 ),
 ( #59563, #94809, #86404, #60123, #41651, #17516, #78007, #16412, #33784, #25926, #68526, #224, #767, #76356, #51158, #50606, #69084, #43317, #9153, #76916, #103185, #102625, #94241, #51715 ),
 ( #85854, #75807, #101525, #92587, #77465, #1313, #34896, #85285, #42754, #26488, #58459, #35453, #84738, #60683, #18084, #52279, #67981, #67426, #24813, #69641, #93144, #24278, #42205, #15858 ) ),
 .UNSPECIFIED., .F., .F., .F.,
 ( 6, 6 ),
 ( 6, 3, 3, 3, 3, 3, 3, 6 ),
 ( 50.65640425731359642, 99.21450639910000291 ),
 ( 27.66900091189999955, 34.04388441780000107, 36.53848016469999749, 37.78577803820000014, 38.40942697490000057, 39.03307591160000101, 39.72592191760000446, 40.41939032376900087 ),
 .UNSPECIFIED. ) ;
#42116=CARTESIAN_POINT ( 'NONE',  ( -2.499950827471990156, 1420.113971994240046, 91.17141353883751265 ) ) ;
#42117=ORIENTED_EDGE ( 'NONE', *, *, #108440, .T. ) ;
#42121=CARTESIAN_POINT ( 'NONE',  ( -2.975995255039647791, 1485.562730373825843, 182.7647656639549893 ) ) ;
#42125=CARTESIAN_POINT ( 'NONE',  ( 1.121218210719999941, 1416.837080253930026, 190.1583376728979999 ) ) ;
#42127=CARTESIAN_POINT ( 'NONE',  ( -11.70642185290000015, 1427.901906309730066, 149.0556982179979855 ) ) ;
#42128=CARTESIAN_POINT ( 'NONE',  ( -10.89398335968819609, 1427.232626390989253, 149.7228750583091426 ) ) ;
#42129=CARTESIAN_POINT ( 'NONE',  ( -5.672962389570000319, 1441.121347655589943, 185.4629166390980117 ) ) ;
#42130=CARTESIAN_POINT ( 'NONE',  ( 16.74268639634610167, 1509.497727879889908, 233.3777497809320209 ) ) ;
#42132=CARTESIAN_POINT ( 'NONE',  ( 0.2751658889820000065, 1506.798305107329952, 186.8348836488979998 ) ) ;
#42133=CARTESIAN_POINT ( 'NONE',  ( -21.53048477309999953, 1495.369685639130012, 225.8950395148980022 ) ) ;
#42135=CARTESIAN_POINT ( 'NONE',  ( -16.12914238563999803, 1459.079501637530029, 229.9877974799539970 ) ) ;
#42138=CARTESIAN_POINT ( 'NONE',  ( 31.50789225850000008, 1415.566663160229837, 266.5723572024979831 ) ) ;
#42139=CARTESIAN_POINT ( 'NONE',  ( 23.61230825720000226, 1435.322028862560046, 137.2857987807979896 ) ) ;
#42140=CARTESIAN_POINT ( 'NONE',  ( 18.72836455420000235, 1430.305649525229910, 193.0986251508980160 ) ) ;
#42141=CARTESIAN_POINT ( 'NONE',  ( -0.03116252646638100615, 1508.849096702560018, 238.3754306579919842 ) ) ;
#42144=CARTESIAN_POINT ( 'NONE',  ( -1.418593301179999822, 1450.896267606680112, 183.3515803373980191 ) ) ;
#42145=CARTESIAN_POINT ( 'NONE',  ( 6.415419946120000105, 1464.066614333030202, 235.9991510476980068 ) ) ;
#42147=CARTESIAN_POINT ( 'NONE',  ( -13.52632321789999992, 1443.506831778320247, 187.5835459910979921 ) ) ;
#42149=B_SPLINE_SURFACE_WITH_KNOTS ( 'NONE', 5, 5, ( 
 ( #12871, #37532, #73343, #12317, #105288, #45408, #38081, #38622, #90120, #47051, #46507, #20704 ),
 ( #63857, #47591, #54900, #62780, #72258, #96894, #106388, #39168, #89579, #11247, #20165, #21240 ),
 ( #79548, #81175, #4491, #106927, #29673, #30215, #72800, #64406, #88492, #81715, #107477, #30775 ),
 ( #66620, #33511, #75009, #108591, #50364, #109159, #24004, #15057, #32972, #108028, #99617, #31325 ),
 ( #32443, #40832, #65508, #23474, #56548, #82288, #91237, #58200, #22902, #83377, #6678, #41397 ),
 ( #75562, #76099, #48150, #57667, #109697, #101259, #31878, #7778, #92328, #57110, #14516, #48706 ),
 ( #82830, #6122, #49256, #83936, #84490, #90676, #15599, #40278, #41944, #13961, #100722, #5586 ),
 ( #74463, #66066, #39736, #67161, #100190, #91779, #49804, #24557, #7237, #58745, #92884, #110237 ),
 ( #16161, #67712, #22347, #73902, #17253, #60979, #76641, #59319, #35750, #77213, #25669, #103487 ),
 ( #110793, #26791, #516, #42485, #85575, #17807, #34086, #26226, #85031, #9992, #86148, #95104 ),
 ( #18370, #87257, #94533, #10549, #69377, #93431, #53120, #44162, #34641, #51445, #52008, #68825 ),
 ( #104049, #102926, #8323, #9441, #50900, #8872, #44722, #52565, #2180, #68279, #1065, #60416 ) ),
 .UNSPECIFIED., .F., .F., .F.,
 ( 6, 3, 3, 6 ),
 ( 6, 3, 3, 6 ),
 ( 6.280178283895380353, 6.736940245399999583, 7.650418229669999626, 8.353136552314619934 ),
 ( -2.296936462289909714E-05, 0.3577959157660000056, 1.028223679459999929, 1.454028915480000128 ),
 .UNSPECIFIED. ) ;
#42150=CARTESIAN_POINT ( 'NONE',  ( -13.40958089250450058, 1414.996442620860080, 220.3303868550709694 ) ) ;
#42156=CARTESIAN_POINT ( 'NONE',  ( -7.003472331669999384, 1474.927564370629852, 269.4815203934979877 ) ) ;
#42159=CARTESIAN_POINT ( 'NONE',  ( -24.14549998876145764, 1444.489244581972571, 211.6571596010163034 ) ) ;
#42161=CARTESIAN_POINT ( 'NONE',  ( -14.88313348660000024, 1507.431571772529878, 226.1823695288979934 ) ) ;
#42162=CARTESIAN_POINT ( 'NONE',  ( -3.329166574300000292, 1441.604926038239910, 155.7074624611979914 ) ) ;
#42165=CARTESIAN_POINT ( 'NONE',  ( -14.94140562103229897, 1495.722860151610121, 224.6009365516689797 ) ) ;
#42166=AXIS2_PLACEMENT_3D ( 'NONE', #29071, #45885, #80022 ) ;
#42167=CARTESIAN_POINT ( 'NONE',  ( -21.71184628989999865, 1409.671254766829861, 205.3856355629080213 ) ) ;
#42171=CARTESIAN_POINT ( 'NONE',  ( 2.853106639830000072E-11, 1406.768167790330153, 269.6447283206980501 ) ) ;
#42173=CARTESIAN_POINT ( 'NONE',  ( 1.669693912109999845, 1443.913060387330006, 150.7596247526980164 ) ) ;
#42176=AXIS2_PLACEMENT_3D ( 'NONE', #57140, #14546, #48179 ) ;
#42178=CARTESIAN_POINT ( 'NONE',  ( 2.500000000000000000, 1419.524771318244348, 137.0999999980979851 ) ) ;
#42180=CARTESIAN_POINT ( 'NONE',  ( 11.70815223902249969, 1426.714662349520040, 142.1026649480299966 ) ) ;
#42184=CARTESIAN_POINT ( 'NONE',  ( -0.02192817098988990299, 1407.539782047199878, 222.1835171467989767 ) ) ;
#42191=CARTESIAN_POINT ( 'NONE',  ( 20.49662116624929808, 1508.357926176179944, 228.4036846774660034 ) ) ;
#42193=ORIENTED_EDGE ( 'NONE', *, *, #14490, .T. ) ;
#42194=EDGE_CURVE ( 'NONE', #54705, #86845, #81109, .T. ) ;
#42196=CARTESIAN_POINT ( 'NONE',  ( 11.94807789040000046, 1434.016817471380136, 150.6813232005980012 ) ) ;
#42197=CARTESIAN_POINT ( 'NONE',  ( 0.02816728215279999670, 1396.454734798429854, 221.5795905766979956 ) ) ;
#42204=CARTESIAN_POINT ( 'NONE',  ( -14.10445144186040167, 1509.241981962429918, 183.4385781783369964 ) ) ;
#42205=CARTESIAN_POINT ( 'NONE',  ( 19.83834310884089902, 1507.818237620550008, 229.2329726552200100 ) ) ;
#42206=CARTESIAN_POINT ( 'NONE',  ( 6.468572857769999906, 1468.699776068629944, 184.1927265961979856 ) ) ;
#42207=CARTESIAN_POINT ( 'NONE',  ( -4.912413666740000018, 1414.913060387329779, 193.3950669238979856 ) ) ;
#42209=CARTESIAN_POINT ( 'NONE',  ( 1.694385804820909946, 1395.972229643439960, 198.2391840958000273 ) ) ;
#42210=CARTESIAN_POINT ( 'NONE',  ( 1.499137190340000148, 1414.988017874730076, 191.7262494343979995 ) ) ;
#42211=CARTESIAN_POINT ( 'NONE',  ( 11.29663592990000076, 1431.956444431130194, 151.5122984544979943 ) ) ;
#42213=ORIENTED_EDGE ( 'NONE', *, *, #108576, .T. ) ;
#42214=CARTESIAN_POINT ( 'NONE',  ( 13.48799209720280068, 1435.249280822409901, 149.8908522090940210 ) ) ;
#42217=CARTESIAN_POINT ( 'NONE',  ( 13.15321365204082937, 1444.754408317047137, 169.3979468993565547 ) ) ;
#42218=CARTESIAN_POINT ( 'NONE',  ( -4.160884814660000153, 1464.635754290229897, 236.0840284009980223 ) ) ;
#42219=CARTESIAN_POINT ( 'NONE',  ( 27.70127829715709922, 1509.880410340700564, 198.6376133113687388 ) ) ;
#42227=B_SPLINE_CURVE_WITH_KNOTS ( 'NONE', 3,
 ( #91930, #76788, #105, #15202, #32027, #32587, #49393, #83521, #100863, #60006, #6815, #40974, #94127, #109301, #108736, #79018, #70080, #10695, #71173, #53826, #69522, #68967, #104193, #70624, #87965, #2319, #85727, #35333, #44867, #53261, #11254 ),
 .UNSPECIFIED., .F., .F.,
 ( 4, 3, 3, 3, 3, 3, 3, 3, 3, 3, 4 ),
 ( -9.981901822019999315, -7.493366175190000256, -7.462945440909900086, -7.082627746929741619, -6.854993841720989245, -6.664003371819999799, -6.519631016808869362, -5.825253142550000263, -5.772861621891269834, -4.972392862104999978, -4.119532581659999693 ),
 .UNSPECIFIED. ) ;
#42231=ORIENTED_EDGE ( 'NONE', *, *, #88087, .T. ) ;
#42233=CARTESIAN_POINT ( 'NONE',  ( -19.65556552330000173, 1509.582207740129888, 230.9700502577980217 ) ) ;
#42234=CARTESIAN_POINT ( 'NONE',  ( -5.821460640849999812, 1409.620882950629948, 187.3298282121979810 ) ) ;
#42238=CARTESIAN_POINT ( 'NONE',  ( 24.42325426270000222, 1438.217997540760052, 213.0745112425780121 ) ) ;
#42239=DIRECTION ( 'NONE',  ( 0.03450791125932765879, 0.9994044208155703490, 8.783400807868103433E-05 ) ) ;
#42240=CARTESIAN_POINT ( 'NONE',  ( 13.80599381087229993, 1434.979619881599774, 146.4346930152470065 ) ) ;
#42249=CARTESIAN_POINT ( 'NONE',  ( 31.70762145559999468, 1417.952368988429953, 271.1218459616979999 ) ) ;
#42250=CARTESIAN_POINT ( 'NONE',  ( 14.52033014849999759, 1409.926738468830081, 191.6835547760979921 ) ) ;
#42255=CARTESIAN_POINT ( 'NONE',  ( 27.90885394509999884, 1457.406260637129890, 250.2249407756980020 ) ) ;
#42257=CARTESIAN_POINT ( 'NONE',  ( -8.076961596850001257, 1418.814380367629838, 233.3636024205979993 ) ) ;
#42266=CARTESIAN_POINT ( 'NONE',  ( 0.1071766512309999947, 1406.264975254330011, 269.2947192205979832 ) ) ;
#42267=CARTESIAN_POINT ( 'NONE',  ( -0.04693436202600000107, 1467.618576924229956, 229.5068687307980042 ) ) ;
#42268=CARTESIAN_POINT ( 'NONE',  ( 24.60632226619999940, 1440.982747020230136, 212.6699546725280072 ) ) ;
#42269=CARTESIAN_POINT ( 'NONE',  ( 37.90967934912709580, 1445.000095422539971, 137.0440870150370074 ) ) ;
#42272=CARTESIAN_POINT ( 'NONE',  ( 15.32734268939944933, 1420.809437254912609, 227.7941278867960762 ) ) ;
#42273=CARTESIAN_POINT ( 'NONE',  ( 32.65728749220649973, 1435.637725527470138, 135.5426019811650065 ) ) ;
#42274=CARTESIAN_POINT ( 'NONE',  ( 39.40243926798699903, 1447.114675383599888, 136.6257780722449979 ) ) ;
#42282=CARTESIAN_POINT ( 'NONE',  ( -44.12252941662215022, 1432.101884911245406, 269.0173719654496836 ) ) ;
#42283=VERTEX_POINT ( 'NONE', #90498 ) ;
#42285=CARTESIAN_POINT ( 'NONE',  ( 15.73707872690769882, 1469.695642903600174, 189.2816229824940137 ) ) ;
#42286=FACE_OUTER_BOUND ( 'NONE', #55227, .T. ) ;
#42288=CARTESIAN_POINT ( 'NONE',  ( 19.60089115691128470, 1455.490215338870485, 226.0492849636472954 ) ) ;
#42291=CARTESIAN_POINT ( 'NONE',  ( -13.93937700741352792, 1420.276149642025757, 227.5832580472266216 ) ) ;
#42294=CARTESIAN_POINT ( 'NONE',  ( 25.32380175889999663, 1435.401097828169895, 135.8572049329980018 ) ) ;
#42295=CARTESIAN_POINT ( 'NONE',  ( -10.70803624744210047, 1396.286993253289893, 206.3112538434370151 ) ) ;
#42296=ORIENTED_EDGE ( 'NONE', *, *, #41774, .T. ) ;
#42297=CARTESIAN_POINT ( 'NONE',  ( 0.8770414022313379743, 1414.913057846380070, 192.4603704288240067 ) ) ;
#42298=CARTESIAN_POINT ( 'NONE',  ( 21.03615327617330166, 1508.023275217195760, 226.0759873548938117 ) ) ;
#42299=ORIENTED_EDGE ( 'NONE', *, *, #3636, .F. ) ;
#42303=DIRECTION ( 'NONE',  ( -0.9899229090099358475, 3.338231922391333496E-06, 0.1416073239848933130 ) ) ;
#42304=CARTESIAN_POINT ( 'NONE',  ( -17.23416124950000139, 1457.524421634029977, 225.2691253537979890 ) ) ;
#42306=CARTESIAN_POINT ( 'NONE',  ( 4.330481386014059630, 1425.574591470910036, 185.4354870873890206 ) ) ;
#42310=CARTESIAN_POINT ( 'NONE',  ( -24.23130728210000129, 1437.896947393770006, 211.0914040829580074 ) ) ;
#42311=FACE_OUTER_BOUND ( 'NONE', #24686, .T. ) ;
#42312=FACE_OUTER_BOUND ( 'NONE', #89524, .T. ) ;
#42314=CARTESIAN_POINT ( 'NONE',  ( -23.34220398524906770, 1509.843709858650982, 228.0495150535502091 ) ) ;
#42316=CARTESIAN_POINT ( 'NONE',  ( -2.713960167710639967E-10, 1417.262443616730025, 235.9145977375980010 ) ) ;
#42320=CARTESIAN_POINT ( 'NONE',  ( -11.78715034128589956, 1427.678896089820000, 147.4800145233820103 ) ) ;
#42327=EDGE_CURVE ( 'NONE', #101819, #95045, #4314, .T. ) ;
#42328=DIRECTION ( 'NONE',  ( 1.000000000000000000, 0.000000000000000000, 0.000000000000000000 ) ) ;
#42329=CARTESIAN_POINT ( 'NONE',  ( -22.93376428353440488, 1507.619498552430059, 207.7003816026530103 ) ) ;
#42332=CARTESIAN_POINT ( 'NONE',  ( -20.49050045394660202, 1409.815506645270034, 269.1358135908449754 ) ) ;
#42333=CARTESIAN_POINT ( 'NONE',  ( -11.07188855570740138, 1414.941240495252941, 195.8493003954075391 ) ) ;
#42334=VERTEX_POINT ( 'NONE', #99439 ) ;
#42336=CARTESIAN_POINT ( 'NONE',  ( 13.81179073420000059, 1445.166753938590091, 189.1769591503979768 ) ) ;
#42339=CARTESIAN_POINT ( 'NONE',  ( 4.571912029077168427, 1422.069887020605847, 184.0289291679942494 ) ) ;
#42343=CYLINDRICAL_SURFACE ( 'NONE', #7269, 1.000000000000001110 ) ;
#42344=ORIENTED_EDGE ( 'NONE', *, *, #95973, .F. ) ;
#42345=CARTESIAN_POINT ( 'NONE',  ( -10.83195828220730839, 1414.913060387329779, 196.7927967275896890 ) ) ;
#42347=CARTESIAN_POINT ( 'NONE',  ( -28.68932943090000265, 1509.915949688529963, 202.5637259519879763 ) ) ;
#42348=CARTESIAN_POINT ( 'NONE',  ( -0.9111207389620000763, 1467.881514926830050, 230.2715671425980020 ) ) ;
#42351=CARTESIAN_POINT ( 'NONE',  ( -13.70772824027479864, 1507.648153509909889, 184.2587339175119894 ) ) ;
#42355=CARTESIAN_POINT ( 'NONE',  ( 26.35247771890000124, 1469.246089662630084, 210.6409091504179969 ) ) ;
#42358=CARTESIAN_POINT ( 'NONE',  ( -13.03231315604520191, 1436.015888718699898, 150.7292108121390299 ) ) ;
#42361=AXIS2_PLACEMENT_3D ( 'NONE', #65567, #15656, #31938 ) ;
#42362=CARTESIAN_POINT ( 'NONE',  ( -14.61893924920000032, 1413.173045456330101, 226.8392015079979842 ) ) ;
#42365=EDGE_LOOP ( 'NONE', ( #105690, #53679, #82467, #91534 ) ) ;
#42367=CARTESIAN_POINT ( 'NONE',  ( -1.387083595259999802, 1410.307627408429880, 232.9611065579980220 ) ) ;
#42368=CARTESIAN_POINT ( 'NONE',  ( -19.74923653411236657, 1456.849059588098953, 225.6335635741733370 ) ) ;
#42369=ORIENTED_EDGE ( 'NONE', *, *, #86662, .F. ) ;
#42372=CARTESIAN_POINT ( 'NONE',  ( 12.80510718569220074, 1435.062306801080240, 150.3516382532390026 ) ) ;
#42373=CARTESIAN_POINT ( 'NONE',  ( 9.922165068644240193, 1459.297038473970133, 232.1972491097930060 ) ) ;
#42375=CARTESIAN_POINT ( 'NONE',  ( 2.493947715939999643, 1442.756953654919926, 150.6345094620980092 ) ) ;
#42380=FACE_OUTER_BOUND ( 'NONE', #213, .T. ) ;
#42381=CARTESIAN_POINT ( 'NONE',  ( 20.10853051189999974, 1509.039643803929948, 188.6705484871980048 ) ) ;
#42383=AXIS2_PLACEMENT_3D ( 'NONE', #82034, #5339, #100498 ) ;
#42385=CARTESIAN_POINT ( 'NONE',  ( -12.72996574539999948, 1416.826388498530150, 195.1129838194979982 ) ) ;
#42391=CARTESIAN_POINT ( 'NONE',  ( 11081.89558200929423, 2833.596074015641989, 8724.858692895628337 ) ) ;
#42394=CARTESIAN_POINT ( 'NONE',  ( 18.89905511659999959, 1416.828040475729949, 210.6687957193779823 ) ) ;
#42399=CARTESIAN_POINT ( 'NONE',  ( 43.89935492036580200, 1440.913060360979898, 264.2399530293329803 ) ) ;
#42403=CARTESIAN_POINT ( 'NONE',  ( 0.5620975284970839425, 1416.851343896850040, 190.4751211475700075 ) ) ;
#42406=CARTESIAN_POINT ( 'NONE',  ( 1.547340046859259965, 1416.576002133120028, 190.2496894819780096 ) ) ;
#42407=CARTESIAN_POINT ( 'NONE',  ( 16.78578239015438811, 1409.668514543772062, 192.8593785157384275 ) ) ;
#42408=CIRCLE ( 'NONE', #105013, 1.999999999999973577 ) ;
#42409=CARTESIAN_POINT ( 'NONE',  ( -24.41180956639999877, 1441.164382444379953, 212.0429753022879993 ) ) ;
#42411=CARTESIAN_POINT ( 'NONE',  ( -3.024617817738020076, 1425.990483723350280, 185.4946073275085894 ) ) ;
#42416=CARTESIAN_POINT ( 'NONE',  ( 7.330937150280000481, 1451.832881924430239, 153.4313473593979893 ) ) ;
#42417=DIRECTION ( 'NONE',  ( 0.9417419115949053898, -0.3363363969979660806, 5.735553207809421716E-15 ) ) ;
#42419=CARTESIAN_POINT ( 'NONE',  ( 23.57479768189999803, 1509.037294151330116, 194.3365427184980092 ) ) ;
#42423=CARTESIAN_POINT ( 'NONE',  ( -20.01979917808080245, 1409.612167179720018, 217.0233986995509952 ) ) ;
#42424=EDGE_LOOP ( 'NONE', ( #98364, #51169, #65370, #44592 ) ) ;
#42425=EDGE_LOOP ( 'NONE', ( #96463, #63593, #106626, #45679, #4264 ) ) ;
#42426=CARTESIAN_POINT ( 'NONE',  ( 19.76863720275370184, 1508.335761315370064, 229.3107344876569869 ) ) ;
#42428=CARTESIAN_POINT ( 'NONE',  ( 39.89315444343499450, 1441.403880509019928, 136.8692038438520058 ) ) ;
#42429=CARTESIAN_POINT ( 'NONE',  ( 0.1681681984989999989, 1432.413060387330006, 146.1721969590979882 ) ) ;
#42435=CARTESIAN_POINT ( 'NONE',  ( -12.81082785388507794, 1435.922453314257382, 150.8250786316239953 ) ) ;
#42437=CARTESIAN_POINT ( 'NONE',  ( 4.817021387869999671, 1409.081274480830189, 187.8331875977980019 ) ) ;
#42438=CARTESIAN_POINT ( 'NONE',  ( 4.660105491930000454, 1423.711922466630085, 183.8926758387979703 ) ) ;
#42440=CARTESIAN_POINT ( 'NONE',  ( -2.500000000250119925, 1440.023260367290050, 162.2535809969560034 ) ) ;
#42442=CARTESIAN_POINT ( 'NONE',  ( -22.21719680079999648, 1451.325171265629933, 143.2349378059979870 ) ) ;
#42443=CARTESIAN_POINT ( 'NONE',  ( 0.7566313362349998961, 1467.043555274730124, 235.5078946572979817 ) ) ;
#42447=CARTESIAN_POINT ( 'NONE',  ( 22.12758967943027244, 1506.606278686416999, 209.2169694191676967 ) ) ;
#42448=CARTESIAN_POINT ( 'NONE',  ( 16.77073029129999782, 1488.221064575230002, 188.9956101863979825 ) ) ;
#42449=CARTESIAN_POINT ( 'NONE',  ( -1.782192625468050338E-12, 1470.276122712049983, 254.7521491344949993 ) ) ;
#42450=CARTESIAN_POINT ( 'NONE',  ( 15.85112983123188357, 1436.286788543214243, 149.0859302454996111 ) ) ;
#42451=CARTESIAN_POINT ( 'NONE',  ( -0.6414547015529999952, 1416.067629290630066, 227.6224876852980117 ) ) ;
#42453=CARTESIAN_POINT ( 'NONE',  ( -5.007571308570000213, 1417.958038874930025, 233.5392730366980061 ) ) ;
#42456=CARTESIAN_POINT ( 'NONE',  ( -0.1563126519980407303, 1486.071014054024317, 181.8244914540917421 ) ) ;
#42458=CARTESIAN_POINT ( 'NONE',  ( -45.94107864437709310, 1438.459200226280245, 266.6805786380390373 ) ) ;
#42463=CARTESIAN_POINT ( 'NONE',  ( -2.478828574380000038, 1434.283354135890022, 157.5745121407980207 ) ) ;
#42464=VECTOR ( 'NONE', #47788, 1000.000000000000114 ) ;
#42467=CARTESIAN_POINT ( 'NONE',  ( -26.75494362287030015, 1450.708015636789924, 136.4629296848829938 ) ) ;
#42468=EDGE_LOOP ( 'NONE', ( #69237, #16443, #93073, #74060, #37121, #104197 ) ) ;
#42469=CARTESIAN_POINT ( 'NONE',  ( 7.882974896040000345, 1421.108448708030210, 221.4185163294980327 ) ) ;
#42471=CARTESIAN_POINT ( 'NONE',  ( 14.83720918809999922, 1488.813684183029864, 193.9548961439979848 ) ) ;
#42472=CARTESIAN_POINT ( 'NONE',  ( -2.510232470973990271, 1419.517688769939923, 186.1000036307290202 ) ) ;
#42473=B_SPLINE_CURVE_WITH_KNOTS ( 'NONE', 5,
 ( #562, #71092, #8930, #27392, #52614, #43653, #43103, #77263, #26847, #95156, #94584, #17864 ),
 .UNSPECIFIED., .F., .F.,
 ( 6, 3, 3, 6 ),
 ( 0.000000000000000000, 0.3740180191949237787, 0.7913393397332487700, 1.000000000000000000 ),
 .UNSPECIFIED. ) ;
#42479=CARTESIAN_POINT ( 'NONE',  ( -2.992362202849540243, 1410.309682308740094, 269.6157897731519597 ) ) ;
#42480=CARTESIAN_POINT ( 'NONE',  ( 6.324577195401869467, 1417.249146248230090, 231.3662450834670210 ) ) ;
#42482=ORIENTED_EDGE ( 'NONE', *, *, #48536, .F. ) ;
#42484=B_SPLINE_CURVE_WITH_KNOTS ( 'NONE', 5,
 ( #49386, #40415, #16290, #58336, #57257, #66208 ),
 .UNSPECIFIED., .F., .F.,
 ( 6, 6 ),
 ( 0.000000000000000000, 1.000000000000000000 ),
 .UNSPECIFIED. ) ;
#42485=CARTESIAN_POINT ( 'NONE',  ( -22.87778797449940171, 1409.742461299279967, 209.5888460124660071 ) ) ;
#42488=CARTESIAN_POINT ( 'NONE',  ( 16.42371624802357744, 1409.486589196651948, 222.7146196853670972 ) ) ;
#42489=VECTOR ( 'NONE', #23380, 1000.000000000000000 ) ;
#42490=CARTESIAN_POINT ( 'NONE',  ( -45.62084243191078770, 1439.252524108265561, 266.1900039064981343 ) ) ;
#42491=CARTESIAN_POINT ( 'NONE',  ( -20.37302944780879699, 1486.732096115899822, 192.8446084916569987 ) ) ;
#42493=CARTESIAN_POINT ( 'NONE',  ( 39.23058051887299769, 1459.489499153630049, 266.8982678320860487 ) ) ;
#42495=CARTESIAN_POINT ( 'NONE',  ( -17.25240610853359513, 1422.435072564651591, 226.6616450818354735 ) ) ;
#42498=CARTESIAN_POINT ( 'NONE',  ( 18.67276003095157932, 1458.371783447332291, 227.3962319617383230 ) ) ;
#42502=CARTESIAN_POINT ( 'NONE',  ( 3.439931081349999697, 1448.290196152649969, 184.1542931849980107 ) ) ;
#42509=CARTESIAN_POINT ( 'NONE',  ( 0.7136616831755410173, 1408.937982002440094, 186.5967116053269876 ) ) ;
#42510=CARTESIAN_POINT ( 'NONE',  ( 1.363624045170000132, 1415.765549035329968, 232.8698710209980050 ) ) ;
#42517=CARTESIAN_POINT ( 'NONE',  ( 12.78749341904959991, 1416.842625005220043, 222.1385636096939891 ) ) ;
#42518=B_SPLINE_SURFACE_WITH_KNOTS ( 'NONE', 5, 5, ( 
 ( #106573, #3595, #37719, #28770, #62971, #88687 ),
 ( #46695, #80825, #21435, #44476, #4668, #57842 ),
 ( #100900, #109342, #66799, #56169, #81908, #57305 ),
 ( #48896, #99804, #108772, #91431, #99249, #83023 ),
 ( #55646, #32066, #89767, #100374, #40462, #5213 ),
 ( #98717, #30409, #64598, #47774, #39367, #74637 ),
 ( #66256, #6315, #38806, #21977, #47226, #108218 ),
 ( #72981, #5778, #32624, #90307, #75191, #31506 ),
 ( #49436, #91969, #30961, #41012, #14707, #13587 ),
 ( #23659, #15244, #73541, #83558, #82478, #6851 ),
 ( #13038, #90865, #81352, #107676, #107119, #65686 ),
 ( #65136, #39920, #22527, #56728, #14153, #48339 ),
 ( #74089, #23099, #33703, #69562, #85769, #35373 ),
 ( #688, #103109, #93064, #24735, #52195, #8502 ),
 ( #60046, #94724, #75735, #102551, #18002, #76277 ),
 ( #102006, #9068, #110425, #43237, #26410, #77385 ),
 ( #58383, #67898, #24197, #33159, #94164, #50536 ),
 ( #1236, #84115, #86324, #51632, #34818, #16881 ),
 ( #85211, #25290, #42127, #59492, #69005, #9608 ),
 ( #60602, #93602, #92509, #77929, #15776, #58932 ),
 ( #25844, #16337, #49978, #42674, #51085, #76831 ),
 ( #17434, #67348, #7414, #43779, #41580, #109879 ),
 ( #84661, #145, #101445, #7960, #34266, #68448 ),
 ( #11829, #37022, #80130, #20213, #52742, #70123 ) ),
 .UNSPECIFIED., .F., .F., .F.,
 ( 6, 3, 3, 3, 3, 3, 3, 6 ),
 ( 6, 6 ),
 ( 3.408434289659999727, 3.762248994509999722, 4.579389332449999905, 5.750344375240000083, 7.455049017759999508, 9.159753660279999821, 12.56916294530000044, 19.70543437909999795 ),
 ( 0.000000000000000000, 2.208859368739999773 ),
 .UNSPECIFIED. ) ;
#42519=CARTESIAN_POINT ( 'NONE',  ( 11.85318847787639918, 1432.336023879089907, 150.2214167536129992 ) ) ;
#42526=( BOUNDED_CURVE ( )  B_SPLINE_CURVE ( 3, ( #81520, #73146, #41194, #8672 ),
 .UNSPECIFIED., .F., .T. ) 
 B_SPLINE_CURVE_WITH_KNOTS ( ( 4, 4 ),
 ( 2.628864438368395007, 3.267182934356360313 ),
 .UNSPECIFIED. ) 
 CURVE ( )  GEOMETRIC_REPRESENTATION_ITEM ( )  RATIONAL_B_SPLINE_CURVE ( ( 1.000000000000000000, 0.9663330366853500886, 0.9663330366853500886, 1.000000000000000000 ) ) 
 REPRESENTATION_ITEM ( '' )  );
#42527=CARTESIAN_POINT ( 'NONE',  ( -34.26800564901520119, 1450.417484578289987, 136.2368926780540050 ) ) ;
#42533=CARTESIAN_POINT ( 'NONE',  ( 11.65871887359999981, 1433.573214819259874, 151.0439516045979929 ) ) ;
#42534=CARTESIAN_POINT ( 'NONE',  ( 25.65427092719999891, 1447.057116126670053, 243.9198229650980068 ) ) ;
#42535=CARTESIAN_POINT ( 'NONE',  ( 12.16511160558169991, 1414.971513442450032, 197.5444944024079916 ) ) ;
#42540=EDGE_CURVE ( 'NONE', #98568, #52837, #107622, .T. ) ;
#42541=CARTESIAN_POINT ( 'NONE',  ( 22.12673984907599944, 1409.685743169220132, 208.3470065775269973 ) ) ;
#42543=CARTESIAN_POINT ( 'NONE',  ( 2.641403850869999737, 1466.630502951829840, 234.1756239694980195 ) ) ;
#42544=VECTOR ( 'NONE', #45231, 1000.000000000000000 ) ;
#42545=CARTESIAN_POINT ( 'NONE',  ( 23.83044711719999853, 1430.353408614430009, 213.6317407082179898 ) ) ;
#42547=CARTESIAN_POINT ( 'NONE',  ( -8.878767216129999085, 1509.223113770430018, 236.7286233840980003 ) ) ;
#42549=CARTESIAN_POINT ( 'NONE',  ( 16.37061378800000000, 1453.313060387329870, 220.2891823736979973 ) ) ;
#42554=CARTESIAN_POINT ( 'NONE',  ( 0.1826399099826500061, 1472.956896255519951, 182.3968825522989903 ) ) ;
#42557=CARTESIAN_POINT ( 'NONE',  ( -18.57285056714472304, 1444.740067931808881, 161.9794701184628991 ) ) ;
#42558=CARTESIAN_POINT ( 'NONE',  ( -5.839375756963000264, 1441.004146652379859, 154.6877192777659786 ) ) ;
#42560=CARTESIAN_POINT ( 'NONE',  ( -41.42406817617050052, 1441.754257788219775, 134.0999999980809889 ) ) ;
#42566=CARTESIAN_POINT ( 'NONE',  ( -15.86930209750000031, 1414.913060387329779, 211.6478204561080076 ) ) ;
#42572=CARTESIAN_POINT ( 'NONE',  ( 22.95908931529999819, 1507.624001450029937, 210.4418640519579924 ) ) ;
#42580=CARTESIAN_POINT ( 'NONE',  ( -30.95328360879999963, 1451.678783263429978, 135.6739097202980133 ) ) ;
#42581=CARTESIAN_POINT ( 'NONE',  ( 12.53676446056794624, 1442.773887286370382, 169.5333422587208645 ) ) ;
#42582=CARTESIAN_POINT ( 'NONE',  ( 10.11781796957937551, 1428.435797280887527, 137.0999999980966777 ) ) ;
#42588=CARTESIAN_POINT ( 'NONE',  ( 41.02245392713034988, 1447.677742136113920, 269.6289972548281071 ) ) ;
#42589=CARTESIAN_POINT ( 'NONE',  ( 14.35695837613839032, 1409.414416421430587, 192.9647261027294007 ) ) ;
#42590=CARTESIAN_POINT ( 'NONE',  ( 5.343479918049999888, 1396.099658817830004, 218.7752541424879951 ) ) ;
#42598=CARTESIAN_POINT ( 'NONE',  ( 2.499999987519999856, 1448.405371708940038, 154.5226066912979945 ) ) ;
#42599=CARTESIAN_POINT ( 'NONE',  ( -2.500000000000000000, 1436.625622233000058, 157.6304333937980005 ) ) ;
#42601=CONICAL_SURFACE ( 'NONE', #87293, 21.50000000000000355, 0.3430239404209998177 ) ;
#42606=ORIENTED_EDGE ( 'NONE', *, *, #11363, .F. ) ;
#42609=CARTESIAN_POINT ( 'NONE',  ( -23.00452549200000263, 1430.350017918430012, 202.3573688689379821 ) ) ;
#42610=CARTESIAN_POINT ( 'NONE',  ( -10.81738549768889968, 1425.668387765759917, 102.3030755685860100 ) ) ;
#42611=CARTESIAN_POINT ( 'NONE',  ( 16.62869176917200065, 1409.868729623830177, 192.2451677454709795 ) ) ;
#42613=CARTESIAN_POINT ( 'NONE',  ( 29.04764039190411395, 1510.038300840001739, 201.6228361755694323 ) ) ;
#42615=CARTESIAN_POINT ( 'NONE',  ( 1.539252401269999959, 1434.992946304420002, 189.4158960071980005 ) ) ;
#42620=CARTESIAN_POINT ( 'NONE',  ( -15.97230738210199696, 1420.722887419069821, 227.0315163971459924 ) ) ;
#42622=CARTESIAN_POINT ( 'NONE',  ( 10.02107572612820086, 1396.322385283019912, 216.0185856081670011 ) ) ;
#42624=CARTESIAN_POINT ( 'NONE',  ( -16.38659414299999639, 1458.929922077130186, 229.9995173766979804 ) ) ;
#42626=ORIENTED_EDGE ( 'NONE', *, *, #61044, .T. ) ;
#42628=CARTESIAN_POINT ( 'NONE',  ( 8.770757543469729952E-15, 1422.771842310740112, 151.0941926623779921 ) ) ;
#42634=CARTESIAN_POINT ( 'NONE',  ( 12.20923102414920436, 1507.046626258653760, 228.0865972342955956 ) ) ;
#42638=CARTESIAN_POINT ( 'NONE',  ( 33.98103710425687041, 1443.501467202839649, 154.9319925572100942 ) ) ;
#42644=CARTESIAN_POINT ( 'NONE',  ( 11.76080740273470049, 1426.908826233330046, 145.8170930824429945 ) ) ;
#42645=ADVANCED_FACE ( 'NONE', ( #100527 ), #47261, .F. ) ;
#42646=CARTESIAN_POINT ( 'NONE',  ( 20.33516419129999875, 1507.859939371830023, 228.7622698018979861 ) ) ;
#42648=CARTESIAN_POINT ( 'NONE',  ( -14.00875078090000159, 1416.819756528429934, 221.8514975898980026 ) ) ;
#42649=CARTESIAN_POINT ( 'NONE',  ( -17.11778670694504711, 1443.086052842848176, 162.7557629363845990 ) ) ;
#42652=CARTESIAN_POINT ( 'NONE',  ( -4.983945999730000409, 1425.062923145830155, 186.2539488382980153 ) ) ;
#42654=CARTESIAN_POINT ( 'NONE',  ( -5.465287381910192366, 1446.862131887090982, 154.6411839201834937 ) ) ;
#42658=CARTESIAN_POINT ( 'NONE',  ( -16.83556428340000011, 1507.627023023630045, 224.6625388484980022 ) ) ;
#42661=CARTESIAN_POINT ( 'NONE',  ( -4.688107345455859054, 1423.663410245182149, 184.4846934393623599 ) ) ;
#42662=CARTESIAN_POINT ( 'NONE',  ( 0.1562295902064984587, 1410.302064435142938, 185.0131410921949850 ) ) ;
#42664=CARTESIAN_POINT ( 'NONE',  ( 18.03753337733320095, 1424.489286807229973, 224.3984010197989960 ) ) ;
#42666=EDGE_CURVE ( 'NONE', #12743, #103816, #74207, .T. ) ;
#42667=CARTESIAN_POINT ( 'NONE',  ( -2.928324112734959517, 1485.053537356824791, 183.1171725139605542 ) ) ;
#42668=CARTESIAN_POINT ( 'NONE',  ( -9.176206605676330024E-06, 1406.768156800490033, 269.6447221830679837 ) ) ;
#42671=CARTESIAN_POINT ( 'NONE',  ( 0.5862352712159999424, 1471.323284329630042, 188.0726871234980138 ) ) ;
#42673=EDGE_CURVE ( 'NONE', #69390, #73043, #28775, .T. ) ;
#42674=CARTESIAN_POINT ( 'NONE',  ( -11.47389391070000109, 1425.951597195029990, 147.0448823332980055 ) ) ;
#42676=CARTESIAN_POINT ( 'NONE',  ( 29.31378126858938060, 1450.601291961854031, 136.3806914572924143 ) ) ;
#42681=CARTESIAN_POINT ( 'NONE',  ( -20.75531091540000261, 1495.371774238330090, 227.1192881343980048 ) ) ;
#42684=B_SPLINE_CURVE_WITH_KNOTS ( 'NONE', 5,
 ( #1006, #36243, #70431, #27845, #62026, #9385 ),
 .UNSPECIFIED., .F., .F.,
 ( 6, 6 ),
 ( 0.000000000000000000, 1.000000000000000000 ),
 .UNSPECIFIED. ) ;
#42687=MECHANICAL_DESIGN_GEOMETRIC_PRESENTATION_REPRESENTATION('',(#74907),#53492);
#42688=CARTESIAN_POINT ( 'NONE',  ( 30.23511527080000150, 1414.232503506630110, 267.4627318704980325 ) ) ;
#42689=CARTESIAN_POINT ( 'NONE',  ( 24.92728913490000053, 1436.178271453029993, 137.8894200858980241 ) ) ;
#42691=CARTESIAN_POINT ( 'NONE',  ( 20.31340460420000227, 1449.728792434289971, 194.1812982889979935 ) ) ;
#42692=ADVANCED_FACE ( 'NONE', ( #36644 ), #30256, .F. ) ;
#42695=CARTESIAN_POINT ( 'NONE',  ( 20.22029059781747407, 1426.889228552814757, 220.9842331285456964 ) ) ;
#42697=CARTESIAN_POINT ( 'NONE',  ( -0.5042624802195529998, 1509.595895645290057, 205.5688950569590077 ) ) ;
#42698=CARTESIAN_POINT ( 'NONE',  ( 15.95383384960000228, 1506.798305107329952, 193.5571554442980187 ) ) ;
#42700=CARTESIAN_POINT ( 'NONE',  ( -13.51374722289999930, 1445.514830763570217, 188.1418749665980101 ) ) ;
#42703=CARTESIAN_POINT ( 'NONE',  ( 10.97762738470000166, 1408.611869070129842, 270.1116084948980074 ) ) ;
#42705=CARTESIAN_POINT ( 'NONE',  ( 1.453362474727719844, 1502.444710984339963, 181.3169649662810059 ) ) ;
#42706=CARTESIAN_POINT ( 'NONE',  ( -14.48215298470269907, 1409.418788313440018, 205.4675657464059952 ) ) ;
#42710=CARTESIAN_POINT ( 'NONE',  ( -9.929189165030001263, 1475.283055377529990, 268.4433786484979692 ) ) ;
#42715=CARTESIAN_POINT ( 'NONE',  ( -24.38621446027962847, 1444.659099962498203, 211.1570028031310073 ) ) ;
#42717=CARTESIAN_POINT ( 'NONE',  ( -24.20882859423510070, 1435.739118765830199, 210.8967395777180229 ) ) ;
#42718=CARTESIAN_POINT ( 'NONE',  ( -11.94206337009999963, 1438.199233188169956, 150.9847479746979957 ) ) ;
#42722=CARTESIAN_POINT ( 'NONE',  ( -23.19328137029999937, 1410.218139083129927, 206.0158621637780243 ) ) ;
#42726=CARTESIAN_POINT ( 'NONE',  ( 2.446787376320000096, 1432.353341358199941, 150.2884730787980061 ) ) ;
#42729=CARTESIAN_POINT ( 'NONE',  ( -3.549608351769999892, 1507.276797637930031, 180.9704965309979912 ) ) ;
#42732=CARTESIAN_POINT ( 'NONE',  ( 11.69897705284829925, 1426.720814411340143, 141.4468014655840022 ) ) ;
#42736=CARTESIAN_POINT ( 'NONE',  ( -16.71438865490179992, 1507.439213204299904, 224.6678772092570000 ) ) ;
#42738=CARTESIAN_POINT ( 'NONE',  ( -4.376213210466648462, 1398.043588354321628, 221.3632903160299463 ) ) ;
#42739=CARTESIAN_POINT ( 'NONE',  ( 0.000000000000000000, 1405.413060387330006, 209.1218459616979999 ) ) ;
#42741=CARTESIAN_POINT ( 'NONE',  ( -17.60568779080000112, 1410.876629449830034, 194.3219271762980043 ) ) ;
#42746=CARTESIAN_POINT ( 'NONE',  ( 11.94927061825729986, 1433.750257499170175, 150.4505018609179956 ) ) ;
#42751=DIRECTION ( 'NONE',  ( -0.1041548977914050628, 0.000000000000000000, 0.9945610877497982338 ) ) ;
#42753=CARTESIAN_POINT ( 'NONE',  ( -0.1613635983459999756, 1507.107001919430104, 180.9028748717980193 ) ) ;
#42754=CARTESIAN_POINT ( 'NONE',  ( 15.90103281899999921, 1507.811112176129882, 231.7872566220979991 ) ) ;
#42755=B_SPLINE_CURVE_WITH_KNOTS ( 'NONE', 3,
 ( #63831, #39708, #97943, #55420, #65483, #6099, #40254, #23446, #88998, #39137 ),
 .UNSPECIFIED., .F., .F.,
 ( 4, 3, 3, 4 ),
 ( -157.4421957120000002, -134.5125376663179964, -78.90079083566818952, -29.52656374254129901 ),
 .UNSPECIFIED. ) ;
#42757=CARTESIAN_POINT ( 'NONE',  ( 4.322182879569999692, 1488.170148571130085, 182.6105505137979890 ) ) ;
#42758=CARTESIAN_POINT ( 'NONE',  ( -0.3621993314249999929, 1416.825784011830137, 191.0664210096979900 ) ) ;
#42759=CARTESIAN_POINT ( 'NONE',  ( -24.61293950550089704, 1444.770188684140066, 210.8869336946189890 ) ) ;
#42760=B_SPLINE_SURFACE_WITH_KNOTS ( 'NONE', 5, 5, ( 
 ( #40692, #72656, #39021, #22207, #63720, #97831 ),
 ( #47997, #106784, #12737, #21109, #55311, #67569 ),
 ( #25521, #8727, #84344, #23867, #76497, #58062 ),
 ( #102243, #75419, #83796, #49663, #84879, #50218 ),
 ( #109557, #24423, #41789, #7090, #93825, #41247 ),
 ( #32828, #59712, #75948, #109009, #110099, #67020 ) ),
 .UNSPECIFIED., .F., .F., .F.,
 ( 6, 6 ),
 ( 6, 6 ),
 ( 19.14974397187629762, 84.90069406665540441 ),
 ( -1.908382372295470058E-05, 2.000000000000000000 ),
 .UNSPECIFIED. ) ;
#42762=CARTESIAN_POINT ( 'NONE',  ( 1.600048698852036821, 1401.254281879943164, 134.0999999980979851 ) ) ;
#42763=CARTESIAN_POINT ( 'NONE',  ( 11.85851232169999925, 1431.806521938459809, 149.9579072722980015 ) ) ;
#42765=ORIENTED_EDGE ( 'NONE', *, *, #45962, .F. ) ;
#42766=CARTESIAN_POINT ( 'NONE',  ( 14.11666836576459971, 1435.826325603770101, 149.9982859278159992 ) ) ;
#42769=CARTESIAN_POINT ( 'NONE',  ( 13.17549261770877678, 1444.733027075352084, 169.3947134178655460 ) ) ;
#42770=CARTESIAN_POINT ( 'NONE',  ( -4.035063157659999789, 1465.902341356430043, 234.8124638711979912 ) ) ;
#42775=CARTESIAN_POINT ( 'NONE',  ( -18.89211047122036646, 1444.064104411348126, 212.4334844116814338 ) ) ;
#42779=ORIENTED_EDGE ( 'NONE', *, *, #70417, .T. ) ;
#42781=ORIENTED_EDGE ( 'NONE', *, *, #72916, .F. ) ;
#42784=CARTESIAN_POINT ( 'NONE',  ( -19.08918019649999920, 1507.695924774130162, 229.6553491538980154 ) ) ;
#42786=CARTESIAN_POINT ( 'NONE',  ( -12.62875319149999953, 1409.354066166529719, 191.1165109835980047 ) ) ;
#42790=CARTESIAN_POINT ( 'NONE',  ( 18.27965585589999975, 1424.887530935629911, 223.6444487664979874 ) ) ;
#42799=CARTESIAN_POINT ( 'NONE',  ( -22.45507226509999654, 1509.697208789830029, 190.1127326308979946 ) ) ;
#42807=CARTESIAN_POINT ( 'NONE',  ( 29.81190406250000180, 1458.385319745129891, 254.8364781926979958 ) ) ;
#42808=EDGE_CURVE ( 'NONE', #32688, #28487, #78142, .T. ) ;
#42809=DIRECTION ( 'NONE',  ( 0.2020450509758154878, -0.9583089383565609465, -0.2020439953131532573 ) ) ;
#42811=CARTESIAN_POINT ( 'NONE',  ( -2.573904878592180090, 1507.948512224160140, 237.1221455541720218 ) ) ;
#42814=ADVANCED_FACE ( 'NONE', ( #38155 ), #25887, .F. ) ;
#42815=LINE ( 'NONE', #76976, #92964 ) ;
#42816=CARTESIAN_POINT ( 'NONE',  ( 17.87007737865920021, 1410.277280938980084, 222.8748137377850185 ) ) ;
#42821=CARTESIAN_POINT ( 'NONE',  ( 0.2158683024189999855, 1405.842952038429985, 267.2349487601980513 ) ) ;
#42822=CARTESIAN_POINT ( 'NONE',  ( 27.78452736639999898, 1508.000976259829940, 207.7754990609180084 ) ) ;
#42825=CARTESIAN_POINT ( 'NONE',  ( 12.91403689499999885, 1422.765650913930131, 223.3157943658980287 ) ) ;
#42829=CARTESIAN_POINT ( 'NONE',  ( 27.33348089620090349, 1436.347956869720065, 136.7123816897339736 ) ) ;
#42830=CARTESIAN_POINT ( 'NONE',  ( 35.60247521962389783, 1450.154959175330077, 136.2349793190689979 ) ) ;
#42833=CARTESIAN_POINT ( 'NONE',  ( 11.97166819159999918, 1507.754052776729850, 184.6972969620979939 ) ) ;
#42837=ORIENTED_EDGE ( 'NONE', *, *, #37091, .F. ) ;
#42839=CARTESIAN_POINT ( 'NONE',  ( -29.75208676439999778, 1419.160608152730219, 268.3665355201979992 ) ) ;
#42840=CARTESIAN_POINT ( 'NONE',  ( 12.06139631399999956, 1433.903263441289710, 146.7588256667980033 ) ) ;
#42842=CARTESIAN_POINT ( 'NONE',  ( 13.93255354277440006, 1413.006837750429895, 191.0564263268389880 ) ) ;
#42843=CARTESIAN_POINT ( 'NONE',  ( -0.3602478992429999916, 1417.265131029429995, 235.9082177996980079 ) ) ;
#42846=CARTESIAN_POINT ( 'NONE',  ( -12.75438347776878523, 1444.998130645058609, 185.9525006451713409 ) ) ;
#42850=CARTESIAN_POINT ( 'NONE',  ( 3.931910744533549718, 1448.296755838050103, 184.2998928686550073 ) ) ;
#42854=CARTESIAN_POINT ( 'NONE',  ( -17.98384814369800111, 1416.218865267220053, 209.3252038692039889 ) ) ;
#42855=CARTESIAN_POINT ( 'NONE',  ( 25.19713807460000154, 1435.377389496489741, 135.6160520644979783 ) ) ;
#42857=CARTESIAN_POINT ( 'NONE',  ( -13.43242319806410734, 1443.480650712422175, 169.3649796478555913 ) ) ;
#42860=CARTESIAN_POINT ( 'NONE',  ( 0.04548916784448110012, 1416.835419214280137, 190.9576572557899965 ) ) ;
#42861=CARTESIAN_POINT ( 'NONE',  ( 21.60872085536062315, 1509.279327547744060, 226.5667642667719690 ) ) ;
#42863=ORIENTED_EDGE ( 'NONE', *, *, #95913, .T. ) ;
#42865=CARTESIAN_POINT ( 'NONE',  ( 0.000000000000000000, 1508.913060387330006, 224.7618459619980058 ) ) ;
#42866=CARTESIAN_POINT ( 'NONE',  ( 10.96395988120000098, 1426.065921947929837, 96.53120952369779673 ) ) ;
#42868=CARTESIAN_POINT ( 'NONE',  ( 21.85421336060000286, 1409.676226334529929, 212.4289253482880042 ) ) ;
#42869=CARTESIAN_POINT ( 'NONE',  ( -0.06958495686334870145, 1507.116651890610001, 237.3500246953010162 ) ) ;
#42871=CIRCLE ( 'NONE', #84014, 40.01690241379998980 ) ;
#42872=CARTESIAN_POINT ( 'NONE',  ( -2.534203887357130203, 1421.318133204249989, 184.2270941939309807 ) ) ;
#42875=CARTESIAN_POINT ( 'NONE',  ( -23.96695290484002427, 1411.114064708981914, 209.9397034195345100 ) ) ;
#42876=CARTESIAN_POINT ( 'NONE',  ( 3.225138584909999828, 1449.296389503839919, 183.9159307004979951 ) ) ;
#42879=VERTEX_POINT ( 'NONE', #9510 ) ;
#42881=CARTESIAN_POINT ( 'NONE',  ( -11.81668901717160125, 1429.106002162380037, 148.9487562432439915 ) ) ;
#42883=CARTESIAN_POINT ( 'NONE',  ( -0.4703851458920000339, 1471.586156922030113, 269.6149382613980379 ) ) ;
#42884=CARTESIAN_POINT ( 'NONE',  ( 13.80599381087229993, 1434.979619881599774, 146.4346930152470065 ) ) ;
#42886=VECTOR ( 'NONE', #42417, 1000.000000000000114 ) ;
#42889=CARTESIAN_POINT ( 'NONE',  ( 22.38213208939999888, 1410.189388605130034, 206.5142564081580190 ) ) ;
#42890=DIRECTION ( 'NONE',  ( 0.000000000000000000, 0.000000000000000000, 1.000000000000000000 ) ) ;
#42891=CARTESIAN_POINT ( 'NONE',  ( -21.79083509029999988, 1497.713060387329961, 204.1580431575879686 ) ) ;
#42893=CARTESIAN_POINT ( 'NONE',  ( 13.39711660771139989, 1407.758611748120074, 204.6035603181729812 ) ) ;
#42894=CARTESIAN_POINT ( 'NONE',  ( -20.64341172155089765, 1409.395087195580118, 268.3019762121069789 ) ) ;
#42895=CARTESIAN_POINT ( 'NONE',  ( -14.27116635546209977, 1435.344418236619958, 149.4515510706479802 ) ) ;
#42897=FACE_OUTER_BOUND ( 'NONE', #49526, .T. ) ;
#42898=CARTESIAN_POINT ( 'NONE',  ( 14.26589412800000112, 1443.159997941379970, 189.6457918547979773 ) ) ;
#42899=B_SPLINE_SURFACE_WITH_KNOTS ( 'NONE', 5, 5, ( 
 ( #47119, #107558, #30293, #40349, #106462, #54982 ),
 ( #72332, #31397, #108661, #108101, #89652, #107005 ),
 ( #29746, #82905, #55525, #12938, #21865, #56064 ),
 ( #90191, #13475, #57186, #5662, #99138, #39810 ),
 ( #73970, #47665, #12395, #89107, #65577, #56618 ),
 ( #81792, #99689, #5095, #21321, #73422, #91310 ) ),
 .UNSPECIFIED., .F., .F., .F.,
 ( 6, 6 ),
 ( 6, 6 ),
 ( 9.044683945550000104, 20.53336383379999930 ),
 ( 0.000000000000000000, 2.000000000000000000 ),
 .UNSPECIFIED. ) ;
#42901=EDGE_LOOP ( 'NONE', ( #85514, #90817, #96340, #11793, #54458, #77297, #86160, #40224, #26679, #514, #26571 ) ) ;
#42905=CARTESIAN_POINT ( 'NONE',  ( -17.36067012530000042, 1485.486309981630029, 188.4584240454980204 ) ) ;
#42907=B_SPLINE_SURFACE_WITH_KNOTS ( 'NONE', 5, 5, ( 
 ( #88989, #98490, #73306, #87918, #12833, #12277 ),
 ( #79509, #100688, #100150, #22309, #74425, #58713 ),
 ( #64919, #66584, #99032, #56512, #109660, #23971 ),
 ( #108552, #49218, #31842, #109122, #15020, #92846 ),
 ( #90639, #66027, #6641, #32936, #13920, #22865 ),
 ( #84455, #41358, #23435, #48107, #58166, #7741 ),
 ( #16124, #57629, #107992, #49766, #91198, #101225 ),
 ( #83897, #40796, #40242, #91744, #30737, #82247 ),
 ( #5546, #57071, #75526, #107441, #41904, #14478 ) ),
 .UNSPECIFIED., .F., .F., .F.,
 ( 6, 3, 6 ),
 ( 6, 6 ),
 ( 1.978931347950330100, 6.366800399639999775, 10.01893279935279857 ),
 ( -0.02042752934279919858, 2.000000000000000000 ),
 .UNSPECIFIED. ) ;
#42910=CARTESIAN_POINT ( 'NONE',  ( -5.360253346836620025, 1422.908173213679902, 148.1968392030750294 ) ) ;
#42913=B_SPLINE_CURVE_WITH_KNOTS ( 'NONE', 3,
 ( #66093, #101286, #66644, #84514, #58229, #100745, #16185, #83961, #110819, #25140, #94013, #49279, #58774, #110262, #109721, #34663, #50927, #539, #24031, #76669, #68301, #7261, #75590, #24581, #8345, #40858, #32998, #100220, #23500, #101847, #57692, #75034, #59344, #67185, #92353, #91807, #15086, #34111, #15625, #92912, #93453, #83408, #109185, #16724, #49831, #6703, #32470, #41424, #50386, #7803, #41970, #43078, #102410, #76122, #33538, #67738, #85055, #25692, #42509, #59889, #17277, #51468, #85600, #8901 ),
 .UNSPECIFIED., .F., .F.,
 ( 4, 3, 3, 3, 3, 3, 3, 3, 3, 3, 3, 3, 3, 3, 3, 3, 3, 3, 3, 3, 3, 4 ),
 ( -26.25736392449690015, -24.17957599523969847, -21.70254519240599933, -19.22146160226090217, -16.73813815629290147, -15.82759752639899986, -13.34013828998019946, -11.64113835685350118, -9.942138423719999452, -9.890507822196667576, -9.830620131415628293, -9.764989817940161743, -9.692984518980310327, -9.605203300184257387, -9.521724663411312406, -9.450162862300381050, -9.387712128909072362, -9.328012329869999064, -8.803020716547550251, -8.080332690346452296, -7.533520025769998796, -7.218912042999999557 ),
 .UNSPECIFIED. ) ;
#42914=CARTESIAN_POINT ( 'NONE',  ( -28.13477487810000000, 1508.112005706330137, 208.1343964124890249 ) ) ;
#42915=B_SPLINE_SURFACE_WITH_KNOTS ( 'NONE', 4, 5, ( 
 ( #106398, #37541, #71176, #38089, #62789, #71743 ),
 ( #79560, #81182, #105860, #105297, #38632, #4498 ),
 ( #46514, #29683, #106938, #96904, #21804, #55460 ),
 ( #28588, #45417, #72264, #56004, #3962, #3411 ),
 ( #54372, #73352, #97447, #80648, #2860, #90128 ) ),
 .UNSPECIFIED., .F., .F., .F.,
 ( 5, 5 ),
 ( 6, 6 ),
 ( 21.65831097310000075, 21.66873975040000033 ),
 ( 0.000000000000000000, 2.175433359549999945 ),
 .UNSPECIFIED. ) ;
#42916=CARTESIAN_POINT ( 'NONE',  ( -0.5884397385249999779, 1477.829042423129977, 230.4572567998980048 ) ) ;
#42918=CARTESIAN_POINT ( 'NONE',  ( -4.214983652439999950, 1408.999356326429961, 195.2850467926979832 ) ) ;
#42919=CARTESIAN_POINT ( 'NONE',  ( -11.90005276459999983, 1409.328619386830042, 226.7881247709979959 ) ) ;
#42920=CARTESIAN_POINT ( 'NONE',  ( 15.83141032767047385, 1506.691119431293828, 193.5604645770621062 ) ) ;
#42921=ORIENTED_EDGE ( 'NONE', *, *, #43617, .F. ) ;
#42922=CARTESIAN_POINT ( 'NONE',  ( -23.83721392209670142, 1411.098975797860021, 210.1927897357339816 ) ) ;
#42923=CARTESIAN_POINT ( 'NONE',  ( 26.41621169419999759, 1469.246811861230071, 210.3255135326479888 ) ) ;
#42925=CARTESIAN_POINT ( 'NONE',  ( 19.02723184334069728, 1456.923419417749983, 225.4092703561889834 ) ) ;
#42926=CARTESIAN_POINT ( 'NONE',  ( -24.38719517939999903, 1435.532251698759865, 137.4549481994980056 ) ) ;
#42934=CARTESIAN_POINT ( 'NONE',  ( 0.000000000000000000, 0.000000000000000000, 137.0999999980979851 ) ) ;
#42935=CARTESIAN_POINT ( 'NONE',  ( -3.094201202990000343, 1410.302849984529985, 232.4943490077980073 ) ) ;
#42940=CARTESIAN_POINT ( 'NONE',  ( 12.11768918586579957, 1435.396653826159991, 151.1061025449240276 ) ) ;
#42941=ADVANCED_FACE ( 'NONE', ( #585 ), #76873, .T. ) ;
#42942=CARTESIAN_POINT ( 'NONE',  ( 13.59057177484809920, 1459.300748119509990, 230.6113061433740086 ) ) ;
#42943=CARTESIAN_POINT ( 'NONE',  ( -23.56173385978110346, 1508.473166743119918, 223.3827176401680106 ) ) ;
#42945=CYLINDRICAL_SURFACE ( 'NONE', #109227, 1.000000000000001110 ) ;
#42948=CARTESIAN_POINT ( 'NONE',  ( -3.268819354880000194, 1420.886035747430014, 185.9708108249980114 ) ) ;
#42949=CARTESIAN_POINT ( 'NONE',  ( 19.86733751369999723, 1508.094164472129933, 189.0003703628979963 ) ) ;
#42952=CARTESIAN_POINT ( 'NONE',  ( -12.78752278169999812, 1416.843576337130116, 195.5392800409980225 ) ) ;
#42963=CARTESIAN_POINT ( 'NONE',  ( 18.94857910520000033, 1416.535385209630022, 210.2462401506180072 ) ) ;
#42964=CARTESIAN_POINT ( 'NONE',  ( 19.77969251879999746, 1507.818093401829856, 229.2755605921979907 ) ) ;
#42965=CARTESIAN_POINT ( 'NONE',  ( -3.206876023519999563, 1419.434649146130141, 184.2270935464979971 ) ) ;
#42967=CARTESIAN_POINT ( 'NONE',  ( 14.45783227242900004, 1416.839692127189892, 196.8516148535319985 ) ) ;
#42968=CARTESIAN_POINT ( 'NONE',  ( 40.67904025323289829, 1440.913060359499923, 260.2254464820850330 ) ) ;
#42971=CARTESIAN_POINT ( 'NONE',  ( 10.94841652689837197, 1430.808938732566503, 151.6571754023756569 ) ) ;
#42973=CARTESIAN_POINT ( 'NONE',  ( 1.547206249379240006, 1416.640375553360172, 190.2404263963619826 ) ) ;
#42974=CARTESIAN_POINT ( 'NONE',  ( 23.10158937639999976, 1411.031839729830153, 207.3184562272780056 ) ) ;
#42975=DIRECTION ( 'NONE',  ( 1.000000000000000000, 0.000000000000000000, 0.000000000000000000 ) ) ;
#42976=CARTESIAN_POINT ( 'NONE',  ( -28.77213282419999985, 1509.917805404529872, 211.3774502118079965 ) ) ;
#42978=CARTESIAN_POINT ( 'NONE',  ( -3.945206105667222740, 1426.016427470225381, 186.0654355582702806 ) ) ;
#42984=CARTESIAN_POINT ( 'NONE',  ( -27.33695648125489441, 1509.220068158296499, 212.0715281516864081 ) ) ;
#42985=CARTESIAN_POINT ( 'NONE',  ( -22.57319772750419773, 1409.701314710050156, 209.4509374963450057 ) ) ;
#42989=CARTESIAN_POINT ( 'NONE',  ( -17.45699404409595346, 1460.525946869913014, 228.2422679384081619 ) ) ;
#42992=CARTESIAN_POINT ( 'NONE',  ( -18.13442287810000053, 1409.546328388530128, 221.5845444630980126 ) ) ;
#42995=CARTESIAN_POINT ( 'NONE',  ( 20.31327811046839926, 1509.661823207899943, 230.8228138406879850 ) ) ;
#42997=CARTESIAN_POINT ( 'NONE',  ( 39.45646300420639818, 1440.433025902419786, 136.7700313797910212 ) ) ;
#42998=CARTESIAN_POINT ( 'NONE',  ( 21.39582113410000019, 1488.805759879729976, 209.2914421362780217 ) ) ;
#43001=MECHANICAL_DESIGN_GEOMETRIC_PRESENTATION_REPRESENTATION('',(#48608),#100463);
#43004=CARTESIAN_POINT ( 'NONE',  ( -12.36580673073694925, 1435.688790776224323, 151.0188895871725094 ) ) ;
#43005=CARTESIAN_POINT ( 'NONE',  ( -21.10757296110000070, 1485.953501962929977, 191.9491461224980071 ) ) ;
#43006=CARTESIAN_POINT ( 'NONE',  ( 3.145295632899999916, 1409.190415107630088, 186.3419696091980029 ) ) ;
#43009=CARTESIAN_POINT ( 'NONE',  ( 11.04138766019999984, 1437.532134242359916, 152.0929085511980077 ) ) ;
#43011=AXIS2_PLACEMENT_3D ( 'NONE', #28664, #45493, #71253 ) ;
#43013=CARTESIAN_POINT ( 'NONE',  ( 1.280930038209999955, 1465.268052754130167, 235.9623018578980123 ) ) ;
#43016=CARTESIAN_POINT ( 'NONE',  ( -40.40963026859999729, 1454.388582061129910, 270.2497097010980269 ) ) ;
#43019=CARTESIAN_POINT ( 'NONE',  ( 15.13342375178309851, 1507.606285622089899, 226.3974328904010065 ) ) ;
#43020=CARTESIAN_POINT ( 'NONE',  ( -4.628375330620350073E-09, 1471.965220085929786, 258.9142969561589780 ) ) ;
#43023=CARTESIAN_POINT ( 'NONE',  ( -10.01338583650000125, 1417.954340053530132, 229.9952712016979888 ) ) ;
#43028=CARTESIAN_POINT ( 'NONE',  ( -45.86255884625870038, 1437.690697618850209, 266.6831300263739877 ) ) ;
#43038=CARTESIAN_POINT ( 'NONE',  ( -25.44898708460110015, 1451.960713826190158, 135.8021707696539977 ) ) ;
#43040=CARTESIAN_POINT ( 'NONE',  ( 28.07850873120000301, 1440.913060381239802, 231.9053043630979971 ) ) ;
#43045=CARTESIAN_POINT ( 'NONE',  ( -23.04921901674742202, 1449.613099141845169, 219.4632572153743411 ) ) ;
#43047=CARTESIAN_POINT ( 'NONE',  ( 4.220605471363215067, 1441.596061467261961, 170.5366720304299974 ) ) ;
#43050=CARTESIAN_POINT ( 'NONE',  ( -1.867263997642370166, 1407.952308472890081, 270.2921350646259953 ) ) ;
#43051=CARTESIAN_POINT ( 'NONE',  ( 8.033834871089998941, 1417.062815916630143, 230.8059444928980213 ) ) ;
#43052=CARTESIAN_POINT ( 'NONE',  ( -0.4986843622567649348, 1508.982343520079894, 238.8510830230749775 ) ) ;
#43057=CARTESIAN_POINT ( 'NONE',  ( -0.6901598988031059090, 1408.937161423990119, 186.3200950031190075 ) ) ;
#43058=CARTESIAN_POINT ( 'NONE',  ( -2.368833328420000051, 1427.018531676430030, 133.6118001900980232 ) ) ;
#43059=CARTESIAN_POINT ( 'NONE',  ( -20.77546492954260060, 1499.605258637040151, 192.4370125005800105 ) ) ;
#43060=CARTESIAN_POINT ( 'NONE',  ( -20.65311841410000326, 1420.828459663129934, 220.4668751674979887 ) ) ;
#43061=CARTESIAN_POINT ( 'NONE',  ( 39.11478698586859082, 1459.396654483650082, 266.6203158930860013 ) ) ;
#43063=DIRECTION ( 'NONE',  ( -0.9995237709234254808, 0.03085824620771311644, -1.986952269380852068E-13 ) ) ;
#43066=CARTESIAN_POINT ( 'NONE',  ( 18.30869780503379118, 1459.158508961783355, 227.8104749284805450 ) ) ;
#43069=ORIENTED_EDGE ( 'NONE', *, *, #21376, .F. ) ;
#43070=CARTESIAN_POINT ( 'NONE',  ( -0.9613100514576319311, 1458.000292018469736, 229.8256281850430014 ) ) ;
#43071=CARTESIAN_POINT ( 'NONE',  ( 25.65001819901760172, 1452.017406081909940, 135.2459253483869759 ) ) ;
#43072=B_SPLINE_SURFACE_WITH_KNOTS ( 'NONE', 5, 4, ( 
 ( #110376, #33655, #93561, #5731, #74042 ),
 ( #26362, #34775, #60557, #104186, #77342 ),
 ( #69513, #2312, #9563, #44296, #103063 ),
 ( #60000, #644, #78439, #94119, #42628 ),
 ( #94678, #9018, #86832, #96339, #17391 ),
 ( #17949, #25802, #68960, #1194, #51588 ) ),
 .UNSPECIFIED., .F., .F., .F.,
 ( 6, 6 ),
 ( 5, 5 ),
 ( -1.876035874425760076E-05, 11.48858425020000062 ),
 ( 25.78146411700000229, 39.23969207129999859 ),
 .UNSPECIFIED. ) ;
#43076=CARTESIAN_POINT ( 'NONE',  ( 18.68627176030000214, 1410.927968804830016, 194.6744492970979934 ) ) ;
#43078=CARTESIAN_POINT ( 'NONE',  ( 1.734150443606229830, 1408.973618255220117, 186.8556639801219887 ) ) ;
#43079=CARTESIAN_POINT ( 'NONE',  ( 2.395751473290000266, 1417.680330609130124, 234.5234243683980253 ) ) ;
#43080=CARTESIAN_POINT ( 'NONE',  ( -21.56194541866146608, 1429.229356591500391, 219.1470650008878067 ) ) ;
#43081=CARTESIAN_POINT ( 'NONE',  ( 2.760778564396810353, 1409.009468899150079, 230.1977509304229841 ) ) ;
#43082=CARTESIAN_POINT ( 'NONE',  ( -0.004856263471414200630, 1508.953874411239894, 179.4326758686540018 ) ) ;
#43087=CARTESIAN_POINT ( 'NONE',  ( 11.84451615446399941, 1432.336085895850147, 150.3016814953629989 ) ) ;
#43091=CARTESIAN_POINT ( 'NONE',  ( -35.80287825771539900, 1450.088642008699935, 136.2393403088510127 ) ) ;
#43095=CARTESIAN_POINT ( 'NONE',  ( -21.07223475955725434, 1508.254227182171917, 192.1325232464991757 ) ) ;
#43096=CARTESIAN_POINT ( 'NONE',  ( 11.88608296559999999, 1433.201875827699951, 150.0808573810979851 ) ) ;
#43097=CARTESIAN_POINT ( 'NONE',  ( 1.998401444330000344E-15, 1456.909266848530024, 224.8635561844979804 ) ) ;
#43103=CARTESIAN_POINT ( 'NONE',  ( 22.68092815790000216, 1409.705069317929883, 208.9674978898780182 ) ) ;
#43105=DIRECTION ( 'NONE',  ( 0.000000000000000000, 0.000000000000000000, -1.000000000000000000 ) ) ;
#43106=CARTESIAN_POINT ( 'NONE',  ( -29.58054436722819958, 1509.946035758800008, 208.7921511973499662 ) ) ;
#43109=CARTESIAN_POINT ( 'NONE',  ( 0.000000000000000000, 1508.913060387330006, 209.1218459616979999 ) ) ;
#43110=CARTESIAN_POINT ( 'NONE',  ( -8.767938172670000085, 1509.161953616930077, 236.4477657171979956 ) ) ;
#43112=CARTESIAN_POINT ( 'NONE',  ( 17.20730882039999798, 1475.513060387329915, 220.8541519961979986 ) ) ;
#43116=CARTESIAN_POINT ( 'NONE',  ( 0.1614806029945209942, 1485.376953580510190, 181.8633822554020014 ) ) ;
#43121=CARTESIAN_POINT ( 'NONE',  ( -17.22592475669603473, 1443.913060387329097, 162.9227486557985003 ) ) ;
#43122=CARTESIAN_POINT ( 'NONE',  ( 11.94106625650000097, 1433.615480207630071, 149.7888360282980216 ) ) ;
#43123=CARTESIAN_POINT ( 'NONE',  ( -35.94635777402429966, 1451.396212934329924, 134.0999999986040052 ) ) ;
#43125=VERTEX_POINT ( 'NONE', #3902 ) ;
#43126=DIRECTION ( 'NONE',  ( 0.000000000000000000, 1.000000000000000000, 0.000000000000000000 ) ) ;
#43128=CARTESIAN_POINT ( 'NONE',  ( -14.38361700439999957, 1416.219761280730154, 221.3510334114980083 ) ) ;
#43139=ORIENTED_EDGE ( 'NONE', *, *, #62202, .T. ) ;
#43141=CARTESIAN_POINT ( 'NONE',  ( -15.73521006790659982, 1409.471155031050102, 225.4906514931829804 ) ) ;
#43146=CARTESIAN_POINT ( 'NONE',  ( 22.37845227239999701, 1507.839484417730091, 224.3727521372980220 ) ) ;
#43149=CARTESIAN_POINT ( 'NONE',  ( 35.14304713054083606, 1457.618104024274999, 269.5334826510517701 ) ) ;
#43151=CARTESIAN_POINT ( 'NONE',  ( 16.20831509755612032, 1432.093373871191261, 218.3923509098792124 ) ) ;
#43153=CARTESIAN_POINT ( 'NONE',  ( 1.448737595259999900, 1416.464314113729870, 232.8152744311979916 ) ) ;
#43155=CARTESIAN_POINT ( 'NONE',  ( -21.33188487129976352, 1507.840678936435324, 227.2305665397985308 ) ) ;
#43159=CARTESIAN_POINT ( 'NONE',  ( 3.657345069180000241, 1446.327858677260110, 165.9157416560979925 ) ) ;
#43164=ORIENTED_EDGE ( 'NONE', *, *, #55584, .F. ) ;
#43166=EDGE_LOOP ( 'NONE', ( #30234, #108332, #83033, #64551, #83246 ) ) ;
#43168=EDGE_CURVE ( 'NONE', #81409, #5765, #51049, .T. ) ;
#43169=CARTESIAN_POINT ( 'NONE',  ( -24.62246550749999940, 1430.359249636930144, 207.4018885027879833 ) ) ;
#43170=CARTESIAN_POINT ( 'NONE',  ( -11.08641866761180061, 1425.203475087560037, 139.7057191062969821 ) ) ;
#43171=CARTESIAN_POINT ( 'NONE',  ( 16.11138931009760000, 1409.475610048200224, 192.9913841948230129 ) ) ;
#43172=EDGE_CURVE ( 'NONE', #91492, #52184, #46998, .T. ) ;
#43174=CARTESIAN_POINT ( 'NONE',  ( 28.97550801065250781, 1510.035835560405985, 201.3478078290377198 ) ) ;
#43175=EDGE_CURVE ( 'NONE', #31041, #90450, #62298, .T. ) ;
#43176=CARTESIAN_POINT ( 'NONE',  ( -20.56164794690000264, 1453.151875980330033, 207.7900157754679924 ) ) ;
#43177=CARTESIAN_POINT ( 'NONE',  ( -43.50118324600000363, 1438.239418340559951, 263.8966221458980499 ) ) ;
#43180=CARTESIAN_POINT ( 'NONE',  ( 18.07609654799121301, 1459.453657016485749, 227.9871296375955581 ) ) ;
#43182=CARTESIAN_POINT ( 'NONE',  ( -37.21137227029399952, 1438.039346661569880, 136.5665973368240032 ) ) ;
#43184=CARTESIAN_POINT ( 'NONE',  ( 8.869149785548881226, 1397.558652790959968, 219.0168133846440242 ) ) ;
#43186=CARTESIAN_POINT ( 'NONE',  ( -16.78608357809999774, 1458.775951820630098, 230.6691475833980007 ) ) ;
#43190=DIRECTION ( 'NONE',  ( 0.6670494068259388287, 0.5110419776299538475, 0.5421080943439499089 ) ) ;
#43195=CARTESIAN_POINT ( 'NONE',  ( -1.568400560060000171, 1461.197012475930023, 235.1144211530979931 ) ) ;
#43201=ORIENTED_EDGE ( 'NONE', *, *, #43940, .F. ) ;
#43206=CARTESIAN_POINT ( 'NONE',  ( 11.80565717473840159, 1428.511365933469961, 148.4624678142999983 ) ) ;
#43208=CARTESIAN_POINT ( 'NONE',  ( 19.88163472539999788, 1487.529703934430245, 227.8197638940980028 ) ) ;
#43210=CARTESIAN_POINT ( 'NONE',  ( -1.463277806657410141, 1481.197952492230115, 182.6166260140540203 ) ) ;
#43211=CARTESIAN_POINT ( 'NONE',  ( -16.68533971102617741, 1442.773887286371291, 162.0931267225411148 ) ) ;
#43212=CARTESIAN_POINT ( 'NONE',  ( 6.925614559599999609, 1507.258869698729995, 235.3367835963979928 ) ) ;
#43215=CARTESIAN_POINT ( 'NONE',  ( -5.374640472830000348, 1422.289355296129997, 186.1135859276980113 ) ) ;
#43218=EDGE_CURVE ( 'NONE', #87081, #93372, #2020, .T. ) ;
#43221=CARTESIAN_POINT ( 'NONE',  ( -15.78501546999999938, 1473.845615658229917, 223.6172981401979882 ) ) ;
#43222=CARTESIAN_POINT ( 'NONE',  ( 17.87824514789999952, 1457.869968850630130, 229.1928660837979805 ) ) ;
#43224=CARTESIAN_POINT ( 'NONE',  ( 15.57943184246149926, 1507.275788652510073, 225.6169562388830059 ) ) ;
#43226=CARTESIAN_POINT ( 'NONE',  ( -5.796746189644780500, 1423.410246674609880, 91.23000440890038476 ) ) ;
#43229=CARTESIAN_POINT ( 'NONE',  ( 18.06216501867849900, 1424.493447207169993, 224.2377043503520042 ) ) ;
#43231=CARTESIAN_POINT ( 'NONE',  ( -2.944200527638781928, 1485.258749652005463, 183.0025506695369870 ) ) ;
#43234=VERTEX_POINT ( 'NONE', #101767 ) ;
#43235=CARTESIAN_POINT ( 'NONE',  ( 0.9156123318609999950, 1507.627022993330229, 186.2283749853979771 ) ) ;
#43236=CARTESIAN_POINT ( 'NONE',  ( -12.59650064061658981, 1416.818673809773827, 194.8446894363833906 ) ) ;
#43237=CARTESIAN_POINT ( 'NONE',  ( -11.53336845399999966, 1429.132254792629965, 150.3949716609980101 ) ) ;
#43238=CYLINDRICAL_SURFACE ( 'NONE', #18232, 13.00000000000000355 ) ;
#43240=CARTESIAN_POINT ( 'NONE',  ( 16.90776328024010056, 1509.516719368900112, 233.6187669235270050 ) ) ;
#43243=CARTESIAN_POINT ( 'NONE',  ( 13.85654454600000030, 1410.401893713229811, 228.0973156211979926 ) ) ;
#43248=CARTESIAN_POINT ( 'NONE',  ( 30.02767535379999941, 1414.536195395429786, 266.6069031101980045 ) ) ;
#43249=LINE ( 'NONE', #51646, #55407 ) ;
#43250=CARTESIAN_POINT ( 'NONE',  ( 17.96041831760000207, 1430.310057063830072, 191.8733975052979872 ) ) ;
#43251=CARTESIAN_POINT ( 'NONE',  ( 7.204249177822559247, 1506.516057208486473, 229.9648155173111945 ) ) ;
#43254=CARTESIAN_POINT ( 'NONE',  ( -1.503967762139999831, 1452.143910241330104, 183.9258428494979682 ) ) ;
#43257=CARTESIAN_POINT ( 'NONE',  ( -13.28024027740000079, 1444.654401305939928, 186.6935413929979859 ) ) ;
#43259=CARTESIAN_POINT ( 'NONE',  ( 4.095224926770001161, 1416.176064121729951, 162.4091932246979866 ) ) ;
#43263=CARTESIAN_POINT ( 'NONE',  ( -13.31148314272640043, 1409.377907621740178, 202.3438456377509738 ) ) ;
#43268=CARTESIAN_POINT ( 'NONE',  ( -23.65409152669999671, 1471.025497520530052, 267.0034733968980163 ) ) ;
#43271=EDGE_CURVE ( 'NONE', #33967, #7065, #82098, .T. ) ;
#43275=CYLINDRICAL_SURFACE ( 'NONE', #47909, 1.000000000000001110 ) ;
#43276=CARTESIAN_POINT ( 'NONE',  ( 11.26466625542379951, 1415.020374538979922, 222.5877601533069878 ) ) ;
#43277=CARTESIAN_POINT ( 'NONE',  ( 1.556370309037290012, 1414.996442620790276, 191.7142051069610034 ) ) ;
#43279=CARTESIAN_POINT ( 'NONE',  ( -1.581901184577762409, 1426.946688134061105, 137.0999999980979567 ) ) ;
#43280=CARTESIAN_POINT ( 'NONE',  ( -21.87473849839999929, 1409.676943088129974, 205.8784099853780276 ) ) ;
#43281=CARTESIAN_POINT ( 'NONE',  ( 16.47341461499999937, 1414.971287085330005, 206.4938333208580161 ) ) ;
#43285=B_SPLINE_CURVE_WITH_KNOTS ( 'NONE', 5,
 ( #40733, #93330, #16058, #16593, #75989, #74363, #58649, #41290, #65962, #84390, #6583, #25010 ),
 .UNSPECIFIED., .F., .F.,
 ( 6, 3, 3, 6 ),
 ( 0.000000000000000000, 0.4382291140948913477, 0.7277099922235745755, 1.000000000000000000 ),
 .UNSPECIFIED. ) ;
#43287=CARTESIAN_POINT ( 'NONE',  ( 1.657615632539999773, 1440.444625599219989, 150.6406752848980091 ) ) ;
#43291=CARTESIAN_POINT ( 'NONE',  ( -22.43804543029999721, 1409.696614199630176, 210.2088496164680009 ) ) ;
#43293=CARTESIAN_POINT ( 'NONE',  ( 11.73043893254989989, 1426.700124572799950, 143.6977314769600014 ) ) ;
#43297=CARTESIAN_POINT ( 'NONE',  ( -0.3400762940194579920, 1420.320061791650005, 183.9482503623439982 ) ) ;
#43299=CARTESIAN_POINT ( 'NONE',  ( 2.522951803030079727E-08, 1397.914279477030050, 222.1218461579910297 ) ) ;
#43300=CARTESIAN_POINT ( 'NONE',  ( 0.4558763517165467793, 1414.913060387330006, 193.0031710580974504 ) ) ;
#43301=CARTESIAN_POINT ( 'NONE',  ( -18.32982102970000327, 1430.286950519430093, 194.1997649584980081 ) ) ;
#43304=CARTESIAN_POINT ( 'NONE',  ( 40.96767724775679653, 1447.290420510560125, 135.1833091849670154 ) ) ;
#43307=VERTEX_POINT ( 'NONE', #97792 ) ;
#43308=CARTESIAN_POINT ( 'NONE',  ( 11.42758288567859992, 1434.038670268820169, 151.4105907050079907 ) ) ;
#43309=CARTESIAN_POINT ( 'NONE',  ( 26.35467955869999912, 1507.985761560129959, 216.6977068428279836 ) ) ;
#43311=CARTESIAN_POINT ( 'NONE',  ( -0.0002568563788362631089, 1396.632929649832704, 221.6694727126995303 ) ) ;
#43316=CARTESIAN_POINT ( 'NONE',  ( 2.244413413239999766, 1428.081157166129969, 101.8807690336980016 ) ) ;
#43317=CARTESIAN_POINT ( 'NONE',  ( 18.40075938393449917, 1498.113744106350168, 229.7466415152620129 ) ) ;
#43320=B_SPLINE_CURVE_WITH_KNOTS ( 'NONE', 3,
 ( #7271, #24591, #58238, #25701 ),
 .UNSPECIFIED., .F., .F.,
 ( 4, 4 ),
 ( 0.000000000000000000, 1.000000000000000000 ),
 .UNSPECIFIED. ) ;
#43321=CARTESIAN_POINT ( 'NONE',  ( 5.737348681029999398, 1507.636265651229905, 182.1362798208980109 ) ) ;
#43322=CARTESIAN_POINT ( 'NONE',  ( -0.2707600216260000470, 1415.088016306429836, 192.1592597442979979 ) ) ;
#43325=CARTESIAN_POINT ( 'NONE',  ( 14.30888197748840085, 1416.029511585970113, 197.0047464494140286 ) ) ;
#43326=CARTESIAN_POINT ( 'NONE',  ( 11.75825615539999980, 1431.471826025599967, 150.7534513679979966 ) ) ;
#43329=CARTESIAN_POINT ( 'NONE',  ( 13.86183822248450070, 1435.004851280240018, 148.8463810403530090 ) ) ;
#43333=EDGE_CURVE ( 'NONE', #1304, #7623, #3307, .T. ) ;
#43334=CARTESIAN_POINT ( 'NONE',  ( 12.98442612396902796, 1444.885683142492098, 169.4237764324444697 ) ) ;
#43335=CARTESIAN_POINT ( 'NONE',  ( -0.6059034394429999582, 1465.006891022829905, 237.7143252328980054 ) ) ;
#43340=CARTESIAN_POINT ( 'NONE',  ( -18.98444801177922514, 1443.378814963748482, 211.6381416663761001 ) ) ;
#43345=ORIENTED_EDGE ( 'NONE', *, *, #5496, .F. ) ;
#43347=CARTESIAN_POINT ( 'NONE',  ( -19.63615623729999982, 1508.568590186330084, 229.6083364675979794 ) ) ;
#43349=CARTESIAN_POINT ( 'NONE',  ( -10.72453240200000124, 1409.287569311029984, 189.7722108729980164 ) ) ;
#43351=CARTESIAN_POINT ( 'NONE',  ( -9.380124768717641004, 1428.163396101657781, 134.0999999980979851 ) ) ;
#43353=CARTESIAN_POINT ( 'NONE',  ( 21.88686710819999703, 1430.321349793229956, 220.0073909120980034 ) ) ;
#43357=CARTESIAN_POINT ( 'NONE',  ( 8.886207544592329199, 1432.346591521910113, 153.1913203755599966 ) ) ;
#43359=B_SPLINE_CURVE_WITH_KNOTS ( 'NONE', 5,
 ( #97762, #29451, #5921, #81498, #20483, #40067, #54693, #37871, #88819, #12105, #55795, #72056 ),
 .UNSPECIFIED., .F., .F.,
 ( 6, 3, 3, 6 ),
 ( 0.000000000000000000, 0.3179072520873084673, 0.5558626742919888786, 1.000000000000000000 ),
 .UNSPECIFIED. ) ;
#43363=CARTESIAN_POINT ( 'NONE',  ( -20.50902834189999879, 1508.364533681130069, 189.6819253274979928 ) ) ;
#43366=CARTESIAN_POINT ( 'NONE',  ( 14.22405166870000137, 1409.409775216930029, 192.8963038564980081 ) ) ;
#43367=CARTESIAN_POINT ( 'NONE',  ( -18.45994912253222253, 1486.199205235777072, 188.8535768566627269 ) ) ;
#43369=VERTEX_POINT ( 'NONE', #85817 ) ;
#43371=CARTESIAN_POINT ( 'NONE',  ( 32.18003819369999974, 1459.550832481329962, 259.4131166698980451 ) ) ;
#43372=CARTESIAN_POINT ( 'NONE',  ( 3.674421735066214278, 1450.449123075120724, 184.1280417905258560 ) ) ;
#43374=CARTESIAN_POINT ( 'NONE',  ( -5.283213344790979704, 1507.787234078490201, 236.3252226269889888 ) ) ;
#43375=CARTESIAN_POINT ( 'NONE',  ( -23.68747534799999954, 1447.176912900409889, 214.7820647780980039 ) ) ;
#43376=CARTESIAN_POINT ( 'NONE',  ( -22.30075843119631429, 1411.051997994482235, 202.8314164432181030 ) ) ;
#43377=CARTESIAN_POINT ( 'NONE',  ( 17.05553375226330104, 1409.525490177569964, 222.2504613337279977 ) ) ;
#43383=VECTOR ( 'NONE', #109612, 1000.000000000000000 ) ;
#43385=CARTESIAN_POINT ( 'NONE',  ( 12.55190973179999858, 1425.728534340630176, 223.8561624606980160 ) ) ;
#43386=CARTESIAN_POINT ( 'NONE',  ( 5.477776093029999238, 1439.067881875560033, 154.7441050454979745 ) ) ;
#43387=DIRECTION ( 'NONE',  ( 0.000000000000000000, 0.000000000000000000, -1.000000000000000000 ) ) ;
#43389=CARTESIAN_POINT ( 'NONE',  ( 33.30038288836900051, 1436.135148397250077, 136.3179756724720164 ) ) ;
#43390=CARTESIAN_POINT ( 'NONE',  ( 36.46770289711280100, 1449.819842309009800, 136.2622417282709932 ) ) ;
#43391=CARTESIAN_POINT ( 'NONE',  ( -45.63713141301216325, 1443.374874937930372, 268.9747502902704355 ) ) ;
#43397=CARTESIAN_POINT ( 'NONE',  ( -36.99165393039999827, 1427.133824787629919, 268.3665355199980240 ) ) ;
#43398=CARTESIAN_POINT ( 'NONE',  ( 11.87977127189999926, 1433.311038246140015, 146.7587715624979978 ) ) ;
#43402=DIRECTION ( 'NONE',  ( 0.7074300732573280959, 0.02470400251971149874, -0.7063514732133270302 ) ) ;
#43409=CARTESIAN_POINT ( 'NONE',  ( -37.90967934872600154, 1445.000095422659797, 137.0440870150139858 ) ) ;
#43411=CARTESIAN_POINT ( 'NONE',  ( -16.78845670593169714, 1414.971513442450032, 208.7062368472520006 ) ) ;
#43412=CARTESIAN_POINT ( 'NONE',  ( 24.40199393649999848, 1435.349635217629839, 136.1409814179979776 ) ) ;
#43413=CARTESIAN_POINT ( 'NONE',  ( -13.40387510366765866, 1443.414769640762870, 169.3677538767024089 ) ) ;
#43415=ADVANCED_FACE ( 'NONE', ( #69608 ), #8913, .T. ) ;
#43416=CARTESIAN_POINT ( 'NONE',  ( -16.16280329491559797, 1409.477474777709858, 225.0536677993360115 ) ) ;
#43420=LINE ( 'NONE', #69745, #23315 ) ;
#43425=CARTESIAN_POINT ( 'NONE',  ( -11.80982523969999853, 1433.007417310889878, 150.5682162921980023 ) ) ;
#43429=CARTESIAN_POINT ( 'NONE',  ( -24.15268595891001979, 1411.115258066103024, 209.2894665055660823 ) ) ;
#43430=CARTESIAN_POINT ( 'NONE',  ( 2.491648406910000002, 1449.120029875969976, 182.5880893073980076 ) ) ;
#43433=ORIENTED_EDGE ( 'NONE', *, *, #78864, .F. ) ;
#43434=ORIENTED_EDGE ( 'NONE', *, *, #86959, .F. ) ;
#43435=CARTESIAN_POINT ( 'NONE',  ( -40.70885756149999679, 1444.085015817089925, 137.1037827856980016 ) ) ;
#43437=CYLINDRICAL_SURFACE ( 'NONE', #49342, 2.000000000000001776 ) ;
#43439=CARTESIAN_POINT ( 'NONE',  ( -3.520666757299999894, 1486.235012026530057, 181.9081341745979898 ) ) ;
#43443=CARTESIAN_POINT ( 'NONE',  ( 21.74754144930000166, 1409.672501264029961, 207.1047251593579972 ) ) ;
#43445=CARTESIAN_POINT ( 'NONE',  ( -22.94032544519359718, 1507.620489270479993, 207.7960379221760263 ) ) ;
#43447=CARTESIAN_POINT ( 'NONE',  ( 14.46065478178650032, 1409.241212025219966, 204.2271823003410134 ) ) ;
#43448=CARTESIAN_POINT ( 'NONE',  ( -8.363319336106780355, 1406.549798397139966, 266.9339146100829794 ) ) ;
#43450=CARTESIAN_POINT ( 'NONE',  ( -14.40366254822449932, 1435.998939573110192, 149.9111377689429787 ) ) ;
#43451=ORIENTED_EDGE ( 'NONE', *, *, #104822, .T. ) ;
#43452=CARTESIAN_POINT ( 'NONE',  ( -11.86584295870000183, 1432.318020648750007, 149.9824182359980114 ) ) ;
#43453=CARTESIAN_POINT ( 'NONE',  ( 13.44142854779999929, 1443.469795417129944, 187.9564574482980106 ) ) ;
#43460=CARTESIAN_POINT ( 'NONE',  ( -13.52062872760000012, 1485.480753740029968, 186.3238177837980061 ) ) ;
#43467=B_SPLINE_CURVE_WITH_KNOTS ( 'NONE', 3,
 ( #99047, #23985, #58727, #22327, #92308, #74440, #13383, #47570, #81695, #39146, #91214, #73322, #7758 ),
 .UNSPECIFIED., .F., .F.,
 ( 4, 2, 1, 1, 1, 2, 2, 4 ),
 ( 0.000000000000000000, 0.2499999999999759082, 0.3749999999999673039, 0.4374999999999629741, 0.4687499999999663602, 0.4843749999999606426, 0.4999999999999549249, 1.000000000000000000 ),
 .UNSPECIFIED. ) ;
#43468=CARTESIAN_POINT ( 'NONE',  ( -27.71749578960000093, 1508.609859370430058, 205.9131467889379792 ) ) ;
#43472=CARTESIAN_POINT ( 'NONE',  ( -3.870783063939999380, 1407.691700113030038, 196.5444094325980302 ) ) ;
#43473=CARTESIAN_POINT ( 'NONE',  ( -13.04207607270000047, 1409.368499719529837, 225.9431834757980084 ) ) ;
#43474=CARTESIAN_POINT ( 'NONE',  ( -1.438891081339280120, 1452.191228260170192, 183.8587004481619829 ) ) ;
#43475=VERTEX_POINT ( 'NONE', #22439 ) ;
#43476=EDGE_CURVE ( 'NONE', #80494, #86711, #104842, .T. ) ;
#43478=CARTESIAN_POINT ( 'NONE',  ( 27.30475511630000085, 1508.128822474129947, 213.8345258920280116 ) ) ;
#43479=CARTESIAN_POINT ( 'NONE',  ( 19.96891611054200055, 1487.423520469470077, 226.6552576108419998 ) ) ;
#43480=CARTESIAN_POINT ( 'NONE',  ( -25.50352605559999830, 1436.178832785409895, 137.0488846515980015 ) ) ;
#43481=APPLICATION_CONTEXT ( 'automotive_design' ) ;
#43485=CARTESIAN_POINT ( 'NONE',  ( -14.79571947709999868, 1410.747178383630171, 226.7235372410980005 ) ) ;
#43490=DIRECTION ( 'NONE',  ( -2.191843104705535248E-06, -0.9999999999950412999, 2.261297895848575335E-06 ) ) ;
#43496=CARTESIAN_POINT ( 'NONE',  ( 12.05521173712990013, 1435.480315805250029, 151.1576910952140054 ) ) ;
#43497=CARTESIAN_POINT ( 'NONE',  ( 12.09098897718920007, 1459.298984292019895, 231.2999770925069924 ) ) ;
#43498=CARTESIAN_POINT ( 'NONE',  ( 1.742626220133139947, 1466.605724716640225, 234.7106070719929960 ) ) ;
#43499=CARTESIAN_POINT ( 'NONE',  ( -2.883410139480000023, 1409.181735915330137, 187.1726403038979925 ) ) ;
#43501=CARTESIAN_POINT ( 'NONE',  ( 4.233744409028489919, 1441.501406244219879, 164.0921308226519955 ) ) ;
#43503=CARTESIAN_POINT ( 'NONE',  ( -3.910864687060000122, 1421.809797752930081, 185.0240497693979762 ) ) ;
#43504=CARTESIAN_POINT ( 'NONE',  ( 20.49660127010000110, 1509.524916156329937, 188.2007677697980057 ) ) ;
#43507=CARTESIAN_POINT ( 'NONE',  ( -12.86122366611309964, 1416.830086716310007, 196.3807296669870084 ) ) ;
#43508=DIRECTION ( 'NONE',  ( -1.000000000000000000, 0.000000000000000000, 0.000000000000000000 ) ) ;
#43514=UNCERTAINTY_MEASURE_WITH_UNIT (LENGTH_MEASURE( 1.000000000000000082E-05 ), #45546, 'distance_accuracy_value', 'NONE');
#43515=CARTESIAN_POINT ( 'NONE',  ( -2.826458050128489941, 1435.843485468609970, 222.4962428573750230 ) ) ;
#43519=CARTESIAN_POINT ( 'NONE',  ( -3.148243355340000438, 1447.343022729889981, 154.4222316151980010 ) ) ;
#43520=CARTESIAN_POINT ( 'NONE',  ( 19.18343150420380994, 1507.776529595233569, 229.7058341636958971 ) ) ;
#43522=CARTESIAN_POINT ( 'NONE',  ( -27.43355922089999765, 1507.980920696130170, 210.8261541407979962 ) ) ;
#43523=CARTESIAN_POINT ( 'NONE',  ( 17.38341196999999738, 1410.833858183129905, 192.4620098003979933 ) ) ;
#43525=CARTESIAN_POINT ( 'NONE',  ( -3.054816033052110136, 1485.996906143959905, 182.1538611115439892 ) ) ;
#43527=ORIENTED_EDGE ( 'NONE', *, *, #109539, .F. ) ;
#43529=CARTESIAN_POINT ( 'NONE',  ( 26.10596347299999920, 1488.578367652129828, 206.7493494209179801 ) ) ;
#43530=CARTESIAN_POINT ( 'NONE',  ( -27.92328169199999977, 1509.198544188530150, 210.7148123472180146 ) ) ;
#43537=CARTESIAN_POINT ( 'NONE',  ( 21.07905887619999774, 1451.363990295029907, 144.5323817167979996 ) ) ;
#43538=CARTESIAN_POINT ( 'NONE',  ( 3.835404308833624043, 1396.046995657106436, 216.1425064568209677 ) ) ;
#43540=PLANE ( 'NONE',  #53287 ) ;
#43544=CARTESIAN_POINT ( 'NONE',  ( 20.40137755018059806, 1509.563325793020113, 230.2999756913229987 ) ) ;
#43546=VERTEX_POINT ( 'NONE', #89676 ) ;
#43547=CARTESIAN_POINT ( 'NONE',  ( 12.59782697949999886, 1446.921545761879770, 188.3055334180980083 ) ) ;
#43550=CARTESIAN_POINT ( 'NONE',  ( 18.06710007320000244, 1416.825245919329973, 208.8994639621759859 ) ) ;
#43551=CARTESIAN_POINT ( 'NONE',  ( -27.41410062850000173, 1466.213783604629953, 262.1295771318979746 ) ) ;
#43556=CARTESIAN_POINT ( 'NONE',  ( 2.214595992090000021, 1409.158101833729916, 186.0729899510980090 ) ) ;
#43557=CARTESIAN_POINT ( 'NONE',  ( 12.78776258891489981, 1416.851343896290018, 222.2791104166909975 ) ) ;
#43558=CARTESIAN_POINT ( 'NONE',  ( -8.251909913180000444, 1439.861448988760003, 153.7181667749979965 ) ) ;
#43559=CARTESIAN_POINT ( 'NONE',  ( 11.39453196610000063, 1435.362097760900042, 151.5417152564980086 ) ) ;
#43561=CARTESIAN_POINT ( 'NONE',  ( -23.70762051470000031, 1451.657018865829968, 140.3727388198980179 ) ) ;
#43562=CARTESIAN_POINT ( 'NONE',  ( 0.1446574667840000161, 1466.770087014230057, 235.6259499557980064 ) ) ;
#43563=ORIENTED_EDGE ( 'NONE', *, *, #60673, .T. ) ;
#43566=CARTESIAN_POINT ( 'NONE',  ( -43.35450150260000157, 1444.057287291979947, 270.3367522392980504 ) ) ;
#43568=CARTESIAN_POINT ( 'NONE',  ( 3.240637488290000423, 1434.541222282480021, 155.4779008716980115 ) ) ;
#43570=CARTESIAN_POINT ( 'NONE',  ( 11.73230603450000054, 1475.513060387329915, 191.9145371412979841 ) ) ;
#43573=CARTESIAN_POINT ( 'NONE',  ( -1.121465867070000177, 1416.819756528530206, 228.0845568296979877 ) ) ;
#43574=CARTESIAN_POINT ( 'NONE',  ( -2.999143295649999708, 1416.435214488830070, 232.8852738930980024 ) ) ;
#43576=CARTESIAN_POINT ( 'NONE',  ( -0.9196686337267430122, 1485.046405773928882, 182.0632183934076807 ) ) ;
#43578=CARTESIAN_POINT ( 'NONE',  ( -45.55790118172819803, 1438.878221330320002, 268.9770245028310001 ) ) ;
#43579=CARTESIAN_POINT ( 'NONE',  ( -4.150360165000000379, 1431.492714444460034, 185.8659833644979926 ) ) ;
#43584=DIRECTION ( 'NONE',  ( 0.1402804634202828582, -0.9901118076169937998, 0.000000000000000000 ) ) ;
#43585=CARTESIAN_POINT ( 'NONE',  ( -26.75392516979539792, 1441.320991203599988, 137.5422828455679962 ) ) ;
#43587=CARTESIAN_POINT ( 'NONE',  ( -25.79053548221810388, 1451.562458167700015, 136.3675287681099917 ) ) ;
#43590=CARTESIAN_POINT ( 'NONE',  ( -15.08937679799999998, 1488.812149332929721, 194.1581390134980154 ) ) ;
#43592=CARTESIAN_POINT ( 'NONE',  ( 13.72746433319999859, 1452.819461535329992, 195.0715466040980175 ) ) ;
#43595=CARTESIAN_POINT ( 'NONE',  ( -23.43613533817220329, 1452.094652507430055, 137.8989582699280163 ) ) ;
#43598=CARTESIAN_POINT ( 'NONE',  ( -0.5924040333921269941, 1410.239981589289982, 269.6149254805689566 ) ) ;
#43600=CARTESIAN_POINT ( 'NONE',  ( 8.991145853091611073, 1419.232555150580083, 232.5600238179060000 ) ) ;
#43606=CARTESIAN_POINT ( 'NONE',  ( -0.2484258432390819560, 1408.921735608980043, 186.5246867112969937 ) ) ;
#43607=CARTESIAN_POINT ( 'NONE',  ( 3.827327165375219664, 1424.046157828239984, 183.3886487722830054 ) ) ;
#43608=CARTESIAN_POINT ( 'NONE',  ( -11.44291537990000052, 1428.994970000029980, 123.0297916884979941 ) ) ;
#43610=CARTESIAN_POINT ( 'NONE',  ( -20.94637264616769556, 1505.073634949130110, 192.2640080708209780 ) ) ;
#43611=CARTESIAN_POINT ( 'NONE',  ( -19.18810533770000148, 1425.814069711829916, 223.9739304577979908 ) ) ;
#43612=CARTESIAN_POINT ( 'NONE',  ( 38.95530193960379961, 1459.246772374329794, 268.9606472942739970 ) ) ;
#43614=CARTESIAN_POINT ( 'NONE',  ( -4.019478480316913682, 1466.624674277336908, 234.7461397303189869 ) ) ;
#43617=EDGE_CURVE ( 'NONE', #26609, #98841, #34027, .T. ) ;
#43619=CARTESIAN_POINT ( 'NONE',  ( -14.03764155707720107, 1452.555513769060099, 223.0320990030590167 ) ) ;
#43621=CARTESIAN_POINT ( 'NONE',  ( 23.71139080889999917, 1410.394892077029908, 208.2669468599999902 ) ) ;
#43623=CARTESIAN_POINT ( 'NONE',  ( -0.5805478584864469660, 1457.956445091640035, 229.5817085807559863 ) ) ;
#43624=CARTESIAN_POINT ( 'NONE',  ( 25.09476263457070289, 1451.973863162750149, 136.0431116258349959 ) ) ;
#43628=CARTESIAN_POINT ( 'NONE',  ( 17.53538859780000081, 1410.022483724830181, 193.0866497752979853 ) ) ;
#43629=CARTESIAN_POINT ( 'NONE',  ( 20.24673233129999872, 1444.324653571829913, 162.1129423953979938 ) ) ;
#43632=CARTESIAN_POINT ( 'NONE',  ( -18.99019980698101051, 1424.920940954418484, 224.2460923394500867 ) ) ;
#43633=CARTESIAN_POINT ( 'NONE',  ( 0.9973831003862488886, 1450.902295810800069, 182.0851543307630038 ) ) ;
#43634=CARTESIAN_POINT ( 'NONE',  ( 18.77802067605560055, 1476.445422708370188, 228.3675973292809829 ) ) ;
#43637=CARTESIAN_POINT ( 'NONE',  ( 11.57735155927789883, 1414.971513442450032, 221.2869575672650058 ) ) ;
#43638=CARTESIAN_POINT ( 'NONE',  ( 11.65870934109939938, 1432.338283370469981, 150.9211944259870108 ) ) ;
#43639=SPHERICAL_SURFACE ( 'NONE', #67798, 2.000000000000000000 ) ;
#43642=DIRECTION ( 'NONE',  ( 0.6456624059335341892, -0.004098122786874927245, -0.7636119845535058737 ) ) ;
#43643=CARTESIAN_POINT ( 'NONE',  ( -11.06589456340000055, 1457.157324861229881, 234.3916895958979865 ) ) ;
#43645=CARTESIAN_POINT ( 'NONE',  ( 11.46353857769999962, 1433.470779071320067, 151.3229031972979897 ) ) ;
#43646=CARTESIAN_POINT ( 'NONE',  ( 14.97660096209999914, 1451.660971648529767, 219.6133834379979817 ) ) ;
#43647=CARTESIAN_POINT ( 'NONE',  ( 12.57270521885200054, 1416.218865267220053, 196.2615492320400108 ) ) ;
#43648=( BOUNDED_CURVE ( )  B_SPLINE_CURVE ( 3, ( #61286, #105460, #62954, #52864 ),
 .UNSPECIFIED., .F., .T. ) 
 B_SPLINE_CURVE_WITH_KNOTS ( ( 4, 4 ),
 ( 6.031750469185639396, 6.430154089112100735 ),
 .UNSPECIFIED. ) 
 CURVE ( )  GEOMETRIC_REPRESENTATION_ITEM ( )  RATIONAL_B_SPLINE_CURVE ( ( 1.000000000000000000, 0.9868165610007129107, 0.9868165610007129107, 1.000000000000000000 ) ) 
 REPRESENTATION_ITEM ( '' )  );
#43653=CARTESIAN_POINT ( 'NONE',  ( 22.69544225309999774, 1409.705575941829920, 209.0104250642420141 ) ) ;
#43654=CARTESIAN_POINT ( 'NONE',  ( 9.382156933674025368, 1398.191381926702661, 200.1155936601079190 ) ) ;
#43655=CARTESIAN_POINT ( 'NONE',  ( 1.742626186960000156, 1466.605724540429947, 234.7106070974979843 ) ) ;
#43656=CARTESIAN_POINT ( 'NONE',  ( 25.71796661899999847, 1449.805629472589999, 209.6503985265360086 ) ) ;
#43666=ORIENTED_EDGE ( 'NONE', *, *, #9075, .T. ) ;
#43667=CARTESIAN_POINT ( 'NONE',  ( 16.37730527473435060, 1414.913060387329779, 210.1804486578982676 ) ) ;
#43668=B_SPLINE_CURVE_WITH_KNOTS ( 'NONE', 5,
 ( #1826, #29208, #78515, #71809, #79081, #96975 ),
 .UNSPECIFIED., .F., .F.,
 ( 6, 6 ),
 ( 0.000000000000000000, 1.000000000000000000 ),
 .UNSPECIFIED. ) ;
#43671=CARTESIAN_POINT ( 'NONE',  ( -36.14177852645050137, 1451.331926750479852, 134.0999999986410103 ) ) ;
#43673=VERTEX_POINT ( 'NONE', #33070 ) ;
#43674=B_SPLINE_SURFACE_WITH_KNOTS ( 'NONE', 5, 5, ( 
 ( #31596, #13124, #64685, #48981, #47308, #65774 ),
 ( #22064, #81431, #99891, #23189, #91515, #12604 ),
 ( #64130, #98251, #83114, #6408, #40554, #89308 ),
 ( #46782, #90390, #80913, #21521, #55733, #38885 ),
 ( #73066, #6948, #83654, #66887, #57929, #92061 ),
 ( #49529, #41105, #25940, #92601, #16427, #109973 ) ),
 .UNSPECIFIED., .F., .F., .F.,
 ( 6, 6 ),
 ( 6, 6 ),
 ( 37.80270741440000393, 108.0413671919999956 ),
 ( -3.367982578744440036E-05, 2.000002141449999993 ),
 .UNSPECIFIED. ) ;
#43677=CARTESIAN_POINT ( 'NONE',  ( -13.49734247349999983, 1415.088275290130014, 220.8629234729979771 ) ) ;
#43678=CARTESIAN_POINT ( 'NONE',  ( 11.59870872757815086, 1426.255586768791318, 138.4426008133268908 ) ) ;
#43681=PLANE ( 'NONE',  #19089 ) ;
#43685=CARTESIAN_POINT ( 'NONE',  ( -17.59962683420000218, 1413.995480048929949, 192.5357147007979961 ) ) ;
#43688=CARTESIAN_POINT ( 'NONE',  ( 12.94068535313422430, 1442.831169986190616, 169.4787936161906430 ) ) ;
#43689=CARTESIAN_POINT ( 'NONE',  ( 3.028503249993359958, 1440.533662647540041, 157.2362874162160153 ) ) ;
#43692=ORIENTED_EDGE ( 'NONE', *, *, #4362, .T. ) ;
#43693=CARTESIAN_POINT ( 'NONE',  ( 26.35476029009999976, 1507.985741737729995, 216.6974866551179844 ) ) ;
#43696=CARTESIAN_POINT ( 'NONE',  ( 37.04966271671443678, 1455.306136334554367, 269.5612861309130039 ) ) ;
#43698=CARTESIAN_POINT ( 'NONE',  ( 6.220301990569999440, 1397.477102019330232, 220.4683151594979904 ) ) ;
#43705=CARTESIAN_POINT ( 'NONE',  ( 4.225063846580001226, 1446.249084106590090, 165.9135352184979979 ) ) ;
#43706=B_SPLINE_SURFACE_WITH_KNOTS ( 'NONE', 5, 5, ( 
 ( #21517, #23185, #57386, #40550, #57926, #41662, #33247, #102102, #74177, #108307, #100993, #31592 ),
 ( #59029, #65769, #92058, #15330, #24289, #50074, #99887, #5858, #84748, #24824, #39999, #91512 ),
 ( #14792, #58470, #67437, #48978, #32703, #82566, #83650, #75818, #92597, #83110, #6404, #74724 ),
 ( #109426, #109970, #108857, #49525, #8046, #32151, #66339, #101535, #93154, #16423, #15871, #84203 ),
 ( #7500, #100455, #23738, #66883, #50616, #33796, #42214, #110514, #76365, #6945, #25382, #90948 ),
 ( #14234, #41100, #67990, #75279, #48423, #70218, #59574, #94252, #51729, #17526, #60133, #44997 ),
 ( #93688, #18095, #36567, #35463, #61802, #16968, #27077, #778, #70765, #34907, #78576, #52289 ),
 ( #85295, #95375, #8594, #61260, #44432, #68538, #77477, #86414, #42766, #76926, #51167, #9704 ),
 ( #85864, #103194, #26499, #10825, #235, #69093, #95923, #104876, #1891, #60695, #94818, #34362 ),
 ( #102636, #104322, #79141, #43329, #9165, #25937, #69653, #27616, #1322, #2451, #36028, #43872 ),
 ( #78015, #103774, #18639, #52838, #86965, #10256, #19184, #53388, #87537, #19758, #30357, #97038 ),
 ( #81307, #53960, #98667, #39317, #29812, #21929, #80780, #64549, #106525, #38758, #46647, #71875 ) ),
 .UNSPECIFIED., .F., .F., .F.,
 ( 6, 3, 3, 6 ),
 ( 6, 3, 3, 6 ),
 ( 5.812567949725580441, 6.561021380799999747, 7.569428689259999565, 8.073660213293690546 ),
 ( -6.147585442244000271E-05, 0.3720032648969999745, 1.117748131209999940, 1.738394476804420163 ),
 .UNSPECIFIED. ) ;
#43708=CARTESIAN_POINT ( 'NONE',  ( 13.79565896120000090, 1416.830000968330069, 196.3348345146980023 ) ) ;
#43714=CARTESIAN_POINT ( 'NONE',  ( 18.32011816680000038, 1412.375214688430106, 259.8063374112979886 ) ) ;
#43715=CARTESIAN_POINT ( 'NONE',  ( -18.41411252810000221, 1430.349328007529948, 194.3797768215980000 ) ) ;
#43716=CARTESIAN_POINT ( 'NONE',  ( -10.76776797470689928, 1424.951090220029982, 141.1922884968350047 ) ) ;
#43717=CARTESIAN_POINT ( 'NONE',  ( 16.32525169496349804, 1409.508281775810019, 192.9210035046159817 ) ) ;
#43719=CARTESIAN_POINT ( 'NONE',  ( 27.87530505112587775, 1509.998252036734357, 198.0047724899852994 ) ) ;
#43720=CARTESIAN_POINT ( 'NONE',  ( -22.16059216520000419, 1489.466620110029908, 207.7982630164780176 ) ) ;
#43722=CARTESIAN_POINT ( 'NONE',  ( 29.68037260111940157, 1509.976800593680082, 209.6726210628699789 ) ) ;
#43723=EDGE_CURVE ( 'NONE', #11508, #13046, #65879, .T. ) ;
#43725=CARTESIAN_POINT ( 'NONE',  ( -37.68692244320210705, 1438.373698044699950, 136.5893188863019816 ) ) ;
#43727=CARTESIAN_POINT ( 'NONE',  ( 8.217383325229510760, 1396.379639214240115, 218.2416968472290080 ) ) ;
#43729=CARTESIAN_POINT ( 'NONE',  ( -16.41679994470000281, 1458.914834253029994, 230.3641776037980264 ) ) ;
#43731=EDGE_LOOP ( 'NONE', ( #16809, #46175, #20720, #39013 ) ) ;
#43732=AXIS2_PLACEMENT_3D ( 'NONE', #33964, #75974, #23356 ) ;
#43733=CARTESIAN_POINT ( 'NONE',  ( -29.24937076371160671, 1509.934532405178516, 211.7291565801588149 ) ) ;
#43739=CARTESIAN_POINT ( 'NONE',  ( -12.30608628080000067, 1442.741623762909967, 186.5150421474980078 ) ) ;
#43741=CARTESIAN_POINT ( 'NONE',  ( 28.45107529421216697, 1509.906593692594470, 206.0415051226699177 ) ) ;
#43742=LINE ( 'NONE', #10131, #6364 ) ;
#43746=VERTEX_POINT ( 'NONE', #14058 ) ;
#43750=CARTESIAN_POINT ( 'NONE',  ( 11.74655472833119951, 1426.725573876949966, 144.8372549033489918 ) ) ;
#43755=CARTESIAN_POINT ( 'NONE',  ( 5.190825549110000381, 1509.094328009829951, 237.6860785186979967 ) ) ;
#43757=CARTESIAN_POINT ( 'NONE',  ( -5.755370776679999523, 1424.283853029129887, 186.4664930395979923 ) ) ;
#43758=CARTESIAN_POINT ( 'NONE',  ( 4.112859965242409821, 1410.383928704729897, 269.6166979547700180 ) ) ;
#43759=LINE ( 'NONE', #77911, #110347 ) ;
#43768=CARTESIAN_POINT ( 'NONE',  ( -2.499957258650039815, 1419.547118819750267, 136.6619867572729845 ) ) ;
#43770=CARTESIAN_POINT ( 'NONE',  ( 18.11762544937269936, 1424.498479437349943, 224.0223624214009988 ) ) ;
#43772=CARTESIAN_POINT ( 'NONE',  ( -2.898163115812544710, 1484.340737685897466, 183.3113270340765837 ) ) ;
#43778=CARTESIAN_POINT ( 'NONE',  ( -24.42830362399999800, 1444.284632803539807, 211.0503697367179825 ) ) ;
#43779=CARTESIAN_POINT ( 'NONE',  ( -11.46173801930000025, 1425.627560988929872, 146.1134360337979956 ) ) ;
#43782=CARTESIAN_POINT ( 'NONE',  ( 27.01382310970000233, 1451.969724731730139, 134.9184576876980088 ) ) ;
#43785=CARTESIAN_POINT ( 'NONE',  ( 14.00845289490000134, 1415.082769112230153, 228.2443160964980109 ) ) ;
#43787=CARTESIAN_POINT ( 'NONE',  ( -15.90941686800000099, 1459.206357706029848, 229.9918337653980132 ) ) ;
#43789=CARTESIAN_POINT ( 'NONE',  ( 29.91696786530000196, 1414.743747860729854, 269.1810462695979709 ) ) ;
#43791=CARTESIAN_POINT ( 'NONE',  ( 18.77981283949999991, 1430.305403855530130, 193.1839142650980250 ) ) ;
#43792=CARTESIAN_POINT ( 'NONE',  ( -20.93923811180000172, 1428.771874825830082, 221.3173514296979931 ) ) ;
#43795=CARTESIAN_POINT ( 'NONE',  ( 5.360207926212690488, 1422.242713656610022, 144.1549664376839814 ) ) ;
#43796=CARTESIAN_POINT ( 'NONE',  ( -1.708753861699999987, 1450.488287334239885, 182.5123027767980091 ) ) ;
#43798=CARTESIAN_POINT ( 'NONE',  ( -15.99522875749999962, 1414.971279908829956, 203.4402680263180230 ) ) ;
#43799=CARTESIAN_POINT ( 'NONE',  ( -13.19176083819999867, 1443.059844678469972, 186.7785638985979801 ) ) ;
#43800=ADVANCED_FACE ( 'NONE', ( #109253 ), #59903, .F. ) ;
#43803=CARTESIAN_POINT ( 'NONE',  ( -33.53719164820000032, 1436.564435420739983, 136.5219720490979967 ) ) ;
#43805=VERTEX_POINT ( 'NONE', #61080 ) ;
#43807=CARTESIAN_POINT ( 'NONE',  ( -14.68124966667719988, 1409.425740922790055, 211.8641606095099803 ) ) ;
#43808=B_SPLINE_SURFACE_WITH_KNOTS ( 'NONE', 2, 5, ( 
 ( #82720, #31756, #49686, #83269, #23352, #40715 ),
 ( #110123, #32320, #66503, #41270, #109580, #32851 ),
 ( #67042, #67591, #35614, #96078, #33961, #17124 ) ),
 .UNSPECIFIED., .F., .F., .F.,
 ( 3, 3 ),
 ( 6, 6 ),
 ( 1.399803019519999969, 2.016961153520000050 ),
 ( 0.000000000000000000, 1.000000000000000000 ),
 .UNSPECIFIED. ) ;
#43811=CARTESIAN_POINT ( 'NONE',  ( -38.50379591154272418, 1443.086052842849085, 136.9552667236205821 ) ) ;
#43812=CARTESIAN_POINT ( 'NONE',  ( -7.090184954099999715, 1475.703047307030147, 267.8325052247980125 ) ) ;
#43816=CARTESIAN_POINT ( 'NONE',  ( 18.16574811487310015, 1421.104903170840089, 223.5180812899619980 ) ) ;
#43818=FACE_OUTER_BOUND ( 'NONE', #4502, .T. ) ;
#43819=CARTESIAN_POINT ( 'NONE',  ( 17.30469233084960123, 1424.057501815570049, 228.1010343377980121 ) ) ;
#43820=CARTESIAN_POINT ( 'NONE',  ( 15.98493104980000190, 1416.216252248729916, 217.5912660269380012 ) ) ;
#43821=CARTESIAN_POINT ( 'NONE',  ( -11.89522282729999958, 1434.541161981840105, 151.0452005854980086 ) ) ;
#43826=CARTESIAN_POINT ( 'NONE',  ( -23.16614514220000132, 1409.886532898030055, 207.1837266853979997 ) ) ;
#43827=CARTESIAN_POINT ( 'NONE',  ( 12.70717284289999860, 1414.913060387329779, 197.8159508449980137 ) ) ;
#43830=B_SPLINE_SURFACE_WITH_KNOTS ( 'NONE', 5, 3, ( 
 ( #22951, #90723, #22389, #98571 ),
 ( #64994, #81218, #21840, #72304 ),
 ( #98019, #57156, #38668, #91281 ),
 ( #56037, #73392, #14561, #82875 ),
 ( #6168, #106976, #40322, #30264 ),
 ( #74504, #90164, #30817, #13445 ),
 ( #47636, #81764, #5067, #39214 ),
 ( #16200, #8362, #33557, #66659 ),
 ( #109202, #16739, #15640, #84530 ) ),
 .UNSPECIFIED., .F., .F., .F.,
 ( 6, 3, 6 ),
 ( 4, 4 ),
 ( 0.000000000000000000, 5.782490304330000441, 11.25975508159999983 ),
 ( 37.69911184309999896, 40.20365518519999881 ),
 .UNSPECIFIED. ) ;
#43831=CARTESIAN_POINT ( 'NONE',  ( 0.8307690413430001142, 1441.600846913440137, 150.7224806086979640 ) ) ;
#43836=CARTESIAN_POINT ( 'NONE',  ( -22.74352257909999864, 1409.874439094229956, 210.5210124972680035 ) ) ;
#43842=CARTESIAN_POINT ( 'NONE',  ( -0.8668663496707069704, 1420.136354665399949, 184.5670725461910138 ) ) ;
#43846=CARTESIAN_POINT ( 'NONE',  ( 2.324758082599999831, 1508.994242728630070, 237.7951232945979996 ) ) ;
#43852=CARTESIAN_POINT ( 'NONE',  ( 11.16030059240809891, 1434.071225047799999, 151.6430048918290083 ) ) ;
#43854=CARTESIAN_POINT ( 'NONE',  ( -0.0002548899671389549728, 1396.374106340500475, 221.3992528296966213 ) ) ;
#43856=CARTESIAN_POINT ( 'NONE',  ( -21.23228437720000272, 1508.977225839029870, 191.9851283159979971 ) ) ;
#43858=CARTESIAN_POINT ( 'NONE',  ( 16.59201921935060042, 1441.947058765370002, 190.5569223725519805 ) ) ;
#43859=CARTESIAN_POINT ( 'NONE',  ( 11.01124415049999961, 1428.984115384829920, 91.31218443469779800 ) ) ;
#43860=CARTESIAN_POINT ( 'NONE',  ( 18.99471019034560015, 1488.414476589019841, 228.8317491358870086 ) ) ;
#43862=CARTESIAN_POINT ( 'NONE',  ( 13.86663486569999826, 1507.632686203329968, 185.8229747852979870 ) ) ;
#43863=CARTESIAN_POINT ( 'NONE',  ( -2.859824010850000153, 1416.824060884929850, 191.2754762073979862 ) ) ;
#43864=CARTESIAN_POINT ( 'NONE',  ( -24.35354770432089921, 1444.782666551750026, 211.2047157338469958 ) ) ;
#43867=CARTESIAN_POINT ( 'NONE',  ( 13.43786152523319899, 1415.007830323630060, 197.8851484046579969 ) ) ;
#43872=CARTESIAN_POINT ( 'NONE',  ( 14.44259369381050107, 1436.255177350019949, 149.9682632730880130 ) ) ;
#43874=VERTEX_POINT ( 'NONE', #104693 ) ;
#43875=EDGE_LOOP ( 'NONE', ( #64128, #31796, #108957, #102909 ) ) ;
#43877=CARTESIAN_POINT ( 'NONE',  ( -2.751894522449999769, 1465.785413735030033, 235.3217997380980080 ) ) ;
#43878=DIRECTION ( 'NONE',  ( 0.000000000000000000, 0.000000000000000000, 1.000000000000000000 ) ) ;
#43881=CARTESIAN_POINT ( 'NONE',  ( -18.97929560748146827, 1443.421918779768930, 211.6863114044098211 ) ) ;
#43883=CARTESIAN_POINT ( 'NONE',  ( 4.242807150219759293, 1446.407532295220108, 162.3334345628060191 ) ) ;
#43884=CARTESIAN_POINT ( 'NONE',  ( 0.6603057237680000080, 1507.898464389029868, 237.4637152757979948 ) ) ;
#43888=CARTESIAN_POINT ( 'NONE',  ( 23.03224585666420055, 1440.913060387330006, 231.8929951805789926 ) ) ;
#43889=CARTESIAN_POINT ( 'NONE',  ( -19.06717646990000148, 1508.525021831829918, 229.8525292550980055 ) ) ;
#43890=ORIENTED_EDGE ( 'NONE', *, *, #106127, .T. ) ;
#43892=CARTESIAN_POINT ( 'NONE',  ( -14.33997081240000071, 1409.413823202629828, 191.5153657412979840 ) ) ;
#43893=CARTESIAN_POINT ( 'NONE',  ( -24.49087403330000257, 1441.667334617299957, 211.0234093942380014 ) ) ;
#43896=CARTESIAN_POINT ( 'NONE',  ( 0.0002635607284424891939, 1396.409786001411021, 196.8022392320345375 ) ) ;
#43897=CARTESIAN_POINT ( 'NONE',  ( -11.89384099105951087, 1433.284007347989927, 147.6487936648496770 ) ) ;
#43906=CARTESIAN_POINT ( 'NONE',  ( -20.86054011819999943, 1508.959477709930070, 190.3575368045979985 ) ) ;
#43909=AXIS2_PLACEMENT_3D ( 'NONE', #104813, #87475, #27553 ) ;
#43910=CARTESIAN_POINT ( 'NONE',  ( 14.80326726320000041, 1409.939845482530018, 191.7219674997980121 ) ) ;
#43914=CARTESIAN_POINT ( 'NONE',  ( 40.57815444089999346, 1448.614255965100028, 261.6157397843979879 ) ) ;
#43917=CARTESIAN_POINT ( 'NONE',  ( -2.626137216361650317, 1508.420410720970040, 237.4127342639979759 ) ) ;
#43918=CARTESIAN_POINT ( 'NONE',  ( -22.15139830520000075, 1451.884836738830245, 222.5180298456980097 ) ) ;
#43919=CARTESIAN_POINT ( 'NONE',  ( 11.30340088569999857, 1432.444851987580023, 151.5218631127980018 ) ) ;
#43920=CARTESIAN_POINT ( 'NONE',  ( 17.32269403890969883, 1409.630503568620043, 222.4515702929919883 ) ) ;
#43921=CARTESIAN_POINT ( 'NONE',  ( 0.2751658889820000065, 1506.798305107329952, 186.8348836488979998 ) ) ;
#43923=VERTEX_POINT ( 'NONE', #30176 ) ;
#43925=EDGE_CURVE ( 'NONE', #55354, #6757, #10038, .T. ) ;
#43926=CARTESIAN_POINT ( 'NONE',  ( 0.3342173453870000421, 1406.778501198230060, 269.6500372471979858 ) ) ;
#43927=CARTESIAN_POINT ( 'NONE',  ( 28.70471845000000144, 1509.915451243230109, 206.7904320628580024 ) ) ;
#43929=EDGE_CURVE ( 'NONE', #7138, #57302, #64813, .T. ) ;
#43930=CARTESIAN_POINT ( 'NONE',  ( -4.927642603766289224E-06, 1473.264982651129912, 270.4290828326839460 ) ) ;
#43931=CARTESIAN_POINT ( 'NONE',  ( 2.478804629799999937, 1434.635234717510002, 157.5856215605979855 ) ) ;
#43934=ADVANCED_FACE ( 'NONE', ( #29634 ), #42907, .F. ) ;
#43935=CARTESIAN_POINT ( 'NONE',  ( -39.59018362911489675, 1440.913060399770075, 258.6997408151970603 ) ) ;
#43936=CARTESIAN_POINT ( 'NONE',  ( -26.41481021949999786, 1448.998476365520219, 136.8839732230979962 ) ) ;
#43940=EDGE_CURVE ( 'NONE', #59669, #99476, #103422, .T. ) ;
#43942=VECTOR ( 'NONE', #65371, 1000.000000000000000 ) ;
#43943=DIRECTION ( 'NONE',  ( -0.3363363969981663093, -0.6659120918162475533, 0.6659120918163308200 ) ) ;
#43945=CARTESIAN_POINT ( 'NONE',  ( 2.431412526649999961, 1428.647745098929818, 149.4227846719979880 ) ) ;
#43946=CARTESIAN_POINT ( 'NONE',  ( 12.91337836679999995, 1434.774321454559868, 146.9205881264979894 ) ) ;
#43949=CARTESIAN_POINT ( 'NONE',  ( 16.19903696008579885, 1484.264179847840069, 188.8259855492240149 ) ) ;
#43950=CARTESIAN_POINT ( 'NONE',  ( -0.4915625660039999456, 1417.355248640930085, 235.5475657494979771 ) ) ;
#43958=CARTESIAN_POINT ( 'NONE',  ( 26.67084063728509591, 1435.736201010440254, 136.2273027514239914 ) ) ;
#43959=CARTESIAN_POINT ( 'NONE',  ( -9.581540676829499503, 1396.247655162970204, 203.5967411505729956 ) ) ;
#43961=EDGE_CURVE ( 'NONE', #79464, #88339, #1030, .T. ) ;
#43963=CARTESIAN_POINT ( 'NONE',  ( 2.482344662330000062, 1440.444625599219989, 150.5580151863979950 ) ) ;
#43965=VERTEX_POINT ( 'NONE', #50859 ) ;
#43968=EDGE_CURVE ( 'NONE', #1945, #47514, #19339, .T. ) ;
#43969=CARTESIAN_POINT ( 'NONE',  ( 11.03848064059999956, 1426.925978087529984, 93.46471121569780394 ) ) ;
#43973=CARTESIAN_POINT ( 'NONE',  ( 0.02089856015480650100, 1507.111761549349922, 237.3522809668369860 ) ) ;
#43980=ADVANCED_BREP_SHAPE_REPRESENTATION ( '', ( #45166, #21632 ), #91264 ) ;
#43984=ORIENTED_EDGE ( 'NONE', *, *, #107533, .T. ) ;
#43986=CARTESIAN_POINT ( 'NONE',  ( -12.01638156518240130, 1440.881463477919851, 187.8051726210379968 ) ) ;
#43989=CARTESIAN_POINT ( 'NONE',  ( -1.462229769779999966, 1473.574695470329971, 270.3922974155980228 ) ) ;
#43991=CARTESIAN_POINT ( 'NONE',  ( -0.5927006846649999217, 1486.019493224930102, 182.0006702160980012 ) ) ;
#43995=B_SPLINE_SURFACE_WITH_KNOTS ( 'NONE', 5, 5, ( 
 ( #79369, #86648, #94485, #69885, #26176, #103435 ),
 ( #78814, #88315, #17757, #87209, #78250, #11609 ),
 ( #10501, #19436, #95607, #53636, #60929, #62036 ),
 ( #87780, #468, #11060, #96159, #26741, #52517 ),
 ( #18326, #69327, #2129, #105117, #45230, #44673 ),
 ( #1018, #60363, #43558, #68777, #18874, #36253 ),
 ( #51960, #1564, #9943, #104561, #95059, #35696 ),
 ( #9395, #86102, #44115, #77708, #19996, #2684 ),
 ( #77166, #104001, #34592, #27298, #102878, #61479 ) ),
 .UNSPECIFIED., .F., .F., .F.,
 ( 6, 3, 6 ),
 ( 6, 6 ),
 ( 6.014757930710000089, 12.35992132620000028, 20.20875810949999973 ),
 ( -8.881784197010000791E-16, 10.00000000000000000 ),
 .UNSPECIFIED. ) ;
#43996=CARTESIAN_POINT ( 'NONE',  ( -2.500000000000000000, 1448.251506100900087, 165.7051602490600146 ) ) ;
#43998=CARTESIAN_POINT ( 'NONE',  ( 13.56949689579999863, 1407.458599673630033, 211.9076660747180085 ) ) ;
#43999=CARTESIAN_POINT ( 'NONE',  ( -5.276338247293970163, 1406.998453906240002, 269.6412759965049872 ) ) ;
#44000=CARTESIAN_POINT ( 'NONE',  ( -14.59287591719009924, 1436.244828798179924, 149.8708817315680051 ) ) ;
#44002=CARTESIAN_POINT ( 'NONE',  ( -11.86607074870000034, 1432.333944652370064, 149.9824168324979894 ) ) ;
#44003=CARTESIAN_POINT ( 'NONE',  ( 13.21847508789999992, 1443.021094946160019, 188.0964758581980050 ) ) ;
#44010=EDGE_CURVE ( 'NONE', #69312, #55354, #65444, .T. ) ;
#44012=ORIENTED_EDGE ( 'NONE', *, *, #1741, .F. ) ;
#44016=CARTESIAN_POINT ( 'NONE',  ( 7.090792818829999788, 1414.913060387329779, 223.8701622068980157 ) ) ;
#44018=CARTESIAN_POINT ( 'NONE',  ( -29.51517718210000041, 1509.962164600430015, 206.4717076456580003 ) ) ;
#44022=CARTESIAN_POINT ( 'NONE',  ( -1.369507862000000076, 1408.899449949929931, 194.7487734720979802 ) ) ;
#44024=CARTESIAN_POINT ( 'NONE',  ( -7.412346052360000215, 1445.966532708270051, 184.7546665820979968 ) ) ;
#44026=CARTESIAN_POINT ( 'NONE',  ( 26.57328462079999909, 1469.248969691330103, 209.5010851783610235 ) ) ;
#44027=CARTESIAN_POINT ( 'NONE',  ( 19.34119489396760017, 1467.092958138930044, 225.7365580626360213 ) ) ;
#44029=CARTESIAN_POINT ( 'NONE',  ( -24.99442991419999771, 1435.370276030620062, 135.8317735983980015 ) ) ;
#44032=CARTESIAN_POINT ( 'NONE',  ( -14.06572158429999853, 1410.763503225130080, 226.9651548780980193 ) ) ;
#44034=CARTESIAN_POINT ( 'NONE',  ( -11.60004869885203682, 1423.462184080423640, 135.7647354700178255 ) ) ;
#44037=CARTESIAN_POINT ( 'NONE',  ( -1.910768082022130221, 1451.940451724439981, 184.3264785220040096 ) ) ;
#44038=CARTESIAN_POINT ( 'NONE',  ( -11.44752262699999790, 1410.292588858030058, 228.7853414855979963 ) ) ;
#44044=CARTESIAN_POINT ( 'NONE',  ( 12.31419433885969994, 1434.254980775230024, 149.8258268142650138 ) ) ;
#44045=CARTESIAN_POINT ( 'NONE',  ( 4.528451146867410237, 1478.701329350719789, 234.4837791156560058 ) ) ;
#44046=CARTESIAN_POINT ( 'NONE',  ( -22.82526493734260242, 1509.659686721229946, 227.0554986310429797 ) ) ;
#44047=EDGE_CURVE ( 'NONE', #93939, #80118, #8691, .T. ) ;
#44048=FACE_OUTER_BOUND ( 'NONE', #17580, .T. ) ;
#44049=CARTESIAN_POINT ( 'NONE',  ( 0.3074360972340000053, 1409.850187049029955, 233.1714481110979875 ) ) ;
#44050=CARTESIAN_POINT ( 'NONE',  ( -0.1562598024478560055, 1420.468994851849857, 182.7540538292380177 ) ) ;
#44052=CARTESIAN_POINT ( 'NONE',  ( -3.613094777869999774, 1419.785023685729811, 186.2978470366979877 ) ) ;
#44053=CARTESIAN_POINT ( 'NONE',  ( 20.16473730159999889, 1508.103700731429853, 189.3367716560979943 ) ) ;
#44054=CARTESIAN_POINT ( 'NONE',  ( 18.27965585607352494, 1424.887530935828636, 223.6444487662844267 ) ) ;
#44055=ORIENTED_EDGE ( 'NONE', *, *, #21255, .T. ) ;
#44056=CARTESIAN_POINT ( 'NONE',  ( -12.93261306534080113, 1416.826860677879949, 196.5036138660090046 ) ) ;
#44057=CARTESIAN_POINT ( 'NONE',  ( -11.63188697299999852, 1495.113783641430018, 182.9907808364980042 ) ) ;
#44059=CARTESIAN_POINT ( 'NONE',  ( 3.784406612299999750, 1421.548653729329999, 184.8121101002980140 ) ) ;
#44066=CARTESIAN_POINT ( 'NONE',  ( -16.13536806862473227, 1409.511687815599998, 192.6629801062032072 ) ) ;
#44067=CARTESIAN_POINT ( 'NONE',  ( 17.36801834879999973, 1414.983773852829927, 210.5058389443579756 ) ) ;
#44068=CARTESIAN_POINT ( 'NONE',  ( -8.907440304760756433, 1432.353341358200169, 149.1004941874240330 ) ) ;
#44072=FACE_OUTER_BOUND ( 'NONE', #71583, .T. ) ;
#44074=CARTESIAN_POINT ( 'NONE',  ( -26.79413167943010166, 1436.761919080860025, 136.7821860765010058 ) ) ;
#44075=CARTESIAN_POINT ( 'NONE',  ( 11.58615099567862572, 1433.820869185889478, 151.2068889330676598 ) ) ;
#44076=ORIENTED_EDGE ( 'NONE', *, *, #72781, .F. ) ;
#44077=CARTESIAN_POINT ( 'NONE',  ( 0.8911620065751310049, 1507.483750996730123, 186.2752927782370023 ) ) ;
#44079=EDGE_CURVE ( 'NONE', #21233, #7608, #55473, .T. ) ;
#44080=CARTESIAN_POINT ( 'NONE',  ( -23.84094907769999949, 1436.644390274100260, 212.4895236289980005 ) ) ;
#44082=CARTESIAN_POINT ( 'NONE',  ( -3.819952067502766280, 1426.014366150848446, 186.0245215687357359 ) ) ;
#44088=CARTESIAN_POINT ( 'NONE',  ( 13.36059443969999982, 1414.988015881329829, 197.8813518256980046 ) ) ;
#44091=CARTESIAN_POINT ( 'NONE',  ( -15.71383117100744897, 1506.606278695164519, 224.7011522283434033 ) ) ;
#44094=EDGE_LOOP ( 'NONE', ( #7776, #96896, #60013, #58818 ) ) ;
#44095=CARTESIAN_POINT ( 'NONE',  ( -1.547463840030000037, 1414.913060387329779, 225.9340782259980074 ) ) ;
#44097=DIRECTION ( 'NONE',  ( -1.049689422327477382E-06, 0.03085829058775882774, 0.9995237695527303678 ) ) ;
#44098=ORIENTED_EDGE ( 'NONE', *, *, #96325, .F. ) ;
#44100=CARTESIAN_POINT ( 'NONE',  ( 20.04661031711670205, 1509.276535231649859, 229.7844010504510095 ) ) ;
#44102=CARTESIAN_POINT ( 'NONE',  ( 38.03973805443759915, 1438.663203083320013, 136.6110655224219954 ) ) ;
#44104=CARTESIAN_POINT ( 'NONE',  ( 15.89205235460757315, 1412.672487590961282, 269.3685437928070883 ) ) ;
#44105=CARTESIAN_POINT ( 'NONE',  ( -42.46017262339999832, 1454.582918749130158, 266.3334795814980112 ) ) ;
#44106=EDGE_CURVE ( 'NONE', #59255, #6406, #71353, .T. ) ;
#44109=B_SPLINE_CURVE_WITH_KNOTS ( 'NONE', 5,
 ( #22690, #98874, #45752, #56339, #13747, #3752 ),
 .UNSPECIFIED., .F., .F.,
 ( 6, 6 ),
 ( 14.91778147325059933, 22.01924661119420890 ),
 .UNSPECIFIED. ) ;
#44111=CARTESIAN_POINT ( 'NONE',  ( -11.29932808600985972, 1434.474993683731782, 151.5487048912618206 ) ) ;
#44113=CARTESIAN_POINT ( 'NONE',  ( 2.025968481520000086, 1408.983808766029824, 186.4771966811979951 ) ) ;
#44114=CARTESIAN_POINT ( 'NONE',  ( 4.714441181029999761, 1423.953913941430073, 185.0673980490979886 ) ) ;
#44115=CARTESIAN_POINT ( 'NONE',  ( -6.686616183240000844, 1441.247408104989972, 154.4574209342979998 ) ) ;
#44119=CARTESIAN_POINT ( 'NONE',  ( 0.004285590335689999815, 1452.913210043329855, 152.9533009523979956 ) ) ;
#44124=CARTESIAN_POINT ( 'NONE',  ( -44.50818758269999620, 1445.910501413080055, 269.6919245774980141 ) ) ;
#44126=CARTESIAN_POINT ( 'NONE',  ( 9.587366264599999965, 1440.450814879359996, 153.1449006345979740 ) ) ;
#44127=DIRECTION ( 'NONE',  ( 0.000000000000000000, 0.000000000000000000, -1.000000000000000000 ) ) ;
#44129=CARTESIAN_POINT ( 'NONE',  ( 2.801091625889360337, 1409.037716335049936, 230.4781056456209853 ) ) ;
#44131=CARTESIAN_POINT ( 'NONE',  ( -4.245035385839999620, 1415.991794987329968, 232.3966682199979914 ) ) ;
#44132=B_SPLINE_CURVE_WITH_KNOTS ( 'NONE', 5,
 ( #55229, #22118, #48481, #31649, #46832, #38937 ),
 .UNSPECIFIED., .F., .F.,
 ( 6, 6 ),
 ( -2.000000000000000000, -9.120498578596425432E-09 ),
 .UNSPECIFIED. ) ;
#44133=CARTESIAN_POINT ( 'NONE',  ( -1.229877626282320779, 1484.645096144196486, 182.2669562530408598 ) ) ;
#44135=CARTESIAN_POINT ( 'NONE',  ( -46.00986170831419741, 1439.835802669839950, 268.4966223753010581 ) ) ;
#44139=EDGE_LOOP ( 'NONE', ( #59855, #51605, #16347, #42094 ) ) ;
#44142=CARTESIAN_POINT ( 'NONE',  ( -27.22940015632950050, 1441.374094644329944, 137.3495836813739857 ) ) ;
#44144=VECTOR ( 'NONE', #64077, 1000.000000000000227 ) ;
#44146=VERTEX_POINT ( 'NONE', #72111 ) ;
#44148=CARTESIAN_POINT ( 'NONE',  ( -14.45750500688560081, 1416.828039245989885, 221.3916439204320170 ) ) ;
#44149=CARTESIAN_POINT ( 'NONE',  ( 15.95383384960000228, 1506.798305107329952, 193.5571554442980187 ) ) ;
#44151=CARTESIAN_POINT ( 'NONE',  ( -11.58491445499556072, 1426.183919005333564, 138.6952712166350352 ) ) ;
#44152=CARTESIAN_POINT ( 'NONE',  ( -17.60611312488026670, 1410.890515041045774, 194.4989067822270101 ) ) ;
#44155=CARTESIAN_POINT ( 'NONE',  ( -6.865870934037390683, 1408.020560016030004, 270.1275732224370358 ) ) ;
#44157=CARTESIAN_POINT ( 'NONE',  ( 4.872266624350030106, 1418.137296580060138, 233.6603738433760213 ) ) ;
#44162=CARTESIAN_POINT ( 'NONE',  ( -23.52688643275999780, 1410.415118700949961, 210.2554788044750183 ) ) ;
#44163=CARTESIAN_POINT ( 'NONE',  ( -4.193899600139999961, 1425.337788341129908, 186.1504193666980029 ) ) ;
#44165=CARTESIAN_POINT ( 'NONE',  ( 0.0001408309371566590163, 1408.913070111550269, 186.4658721391990071 ) ) ;
#44167=CARTESIAN_POINT ( 'NONE',  ( -19.25467140439389624, 1450.982098615540281, 193.9791526570050166 ) ) ;
#44168=CARTESIAN_POINT ( 'NONE',  ( -19.73265327440000050, 1425.811828412130126, 222.9530360735979855 ) ) ;
#44169=CARTESIAN_POINT ( 'NONE',  ( 30.03031303698100274, 1467.498499503609992, 266.8645947477900222 ) ) ;
#44172=( BOUNDED_CURVE ( )  B_SPLINE_CURVE ( 3, ( #103025, #42589, #16255, #76742 ),
 .UNSPECIFIED., .F., .T. ) 
 B_SPLINE_CURVE_WITH_KNOTS ( ( 4, 4 ),
 ( 1.704095840793119931, 2.349013555596815017 ),
 .UNSPECIFIED. ) 
 CURVE ( )  GEOMETRIC_REPRESENTATION_ITEM ( )  RATIONAL_B_SPLINE_CURVE ( ( 1.000000000000000000, 0.9656393833455322318, 0.9656393833455322318, 1.000000000000000000 ) ) 
 REPRESENTATION_ITEM ( '' )  );
#44175=CARTESIAN_POINT ( 'NONE',  ( 23.59369949126165622, 1411.097251101419033, 211.5720139885703190 ) ) ;
#44176=CARTESIAN_POINT ( 'NONE',  ( 1.501870405408500142, 1464.999530953469957, 182.9509895119559815 ) ) ;
#44177=CARTESIAN_POINT ( 'NONE',  ( 22.77443950849999865, 1409.708263161830018, 208.9272941533559731 ) ) ;
#44178=ORIENTED_EDGE ( 'NONE', *, *, #69455, .T. ) ;
#44180=CARTESIAN_POINT ( 'NONE',  ( 25.91250833790000030, 1451.849349898129958, 135.8364949240979911 ) ) ;
#44181=CARTESIAN_POINT ( 'NONE',  ( -22.43804543029999721, 1409.696614199630176, 210.2088496164680009 ) ) ;
#44184=CARTESIAN_POINT ( 'NONE',  ( 17.37384703899999749, 1410.444760247230079, 192.4767873331980184 ) ) ;
#44185=CARTESIAN_POINT ( 'NONE',  ( 27.68130203340000151, 1444.740067931809790, 168.8183730152979933 ) ) ;
#44186=CARTESIAN_POINT ( 'NONE',  ( 1.665296718610000060, 1417.520169485130054, 234.6989198356980069 ) ) ;
#44188=CARTESIAN_POINT ( 'NONE',  ( 1.127302894264770039, 1450.859558279620160, 182.1360551162379977 ) ) ;
#44194=ORIENTED_EDGE ( 'NONE', *, *, #97844, .T. ) ;
#44197=B_SPLINE_CURVE_WITH_KNOTS ( 'NONE', 3,
 ( #23899, #49145, #23362, #91125, #40173, #84381, #59203, #68166, #57552, #92226, #93321, #110131, #101707, #49695, #91675, #14948, #66512, #100615, #16583, #83824 ),
 .UNSPECIFIED., .F., .F.,
 ( 4, 2, 1, 2, 2, 1, 1, 1, 1, 1, 2, 2, 4 ),
 ( 0.000000000000000000, 0.2500000000002167155, 0.3750000000003254064, 0.4375000000003794187, 0.5000000000004334311, 0.6250000000005402345, 0.6875000000005936363, 0.7187500000006207257, 0.7343750000006342704, 0.7421875000006368239, 0.7460937500006337153, 0.7500000000006307177, 1.000000000000000000 ),
 .UNSPECIFIED. ) ;
#44198=DIRECTION ( 'NONE',  ( 0.000000000000000000, 1.000000000000000000, 0.000000000000000000 ) ) ;
#44203=CARTESIAN_POINT ( 'NONE',  ( -18.57221552470000248, 1447.675799122940134, 219.6133833292979887 ) ) ;
#44205=CARTESIAN_POINT ( 'NONE',  ( 11.89943377740000052, 1433.335282505560144, 150.1709607732979919 ) ) ;
#44207=CARTESIAN_POINT ( 'NONE',  ( 3.114882401749999641, 1454.846680951630105, 214.3676144197979738 ) ) ;
#44208=CARTESIAN_POINT ( 'NONE',  ( 26.33767527485199977, 1440.913060395190087, 223.6248100573809836 ) ) ;
#44211=CARTESIAN_POINT ( 'NONE',  ( 24.97896770994293547, 1436.441713528391574, 137.9167425154915918 ) ) ;
#44214=CARTESIAN_POINT ( 'NONE',  ( -25.47742517682650032, 1509.802751679349967, 193.2942475626609848 ) ) ;
#44215=CARTESIAN_POINT ( 'NONE',  ( 22.97761738710000046, 1449.791915361709925, 218.1846805547179997 ) ) ;
#44219=CARTESIAN_POINT ( 'NONE',  ( -41.62601876731983452, 1442.681032278104794, 135.5698701779593023 ) ) ;
#44224=CARTESIAN_POINT ( 'NONE',  ( 0.1670098483671519918, 1482.089753829420033, 182.0046196815349901 ) ) ;
#44225=B_SPLINE_CURVE_WITH_KNOTS ( 'NONE', 3,
 ( #4477, #45393, #3389, #5008, #62196, #106372, #39155, #79532, #29660, #37517, #2835, #71720 ),
 .UNSPECIFIED., .F., .F.,
 ( 4, 2, 2, 2, 2, 4 ),
 ( -0.1123552150373909875, -0.09789198304339560841, -0.08346217084110789386, -0.05408911861973839802, -0.02844403185827369673, -2.821858199469895467E-07 ),
 .UNSPECIFIED. ) ;
#44228=CARTESIAN_POINT ( 'NONE',  ( -0.7130990469979998636, 1416.837309316629899, 227.9189225404980164 ) ) ;
#44230=CARTESIAN_POINT ( 'NONE',  ( 5.386185205460879644, 1432.347042709529887, 154.6076275981190236 ) ) ;
#44236=CARTESIAN_POINT ( 'NONE',  ( -15.60349157319999769, 1415.087797054229895, 216.5108232632080103 ) ) ;
#44237=CARTESIAN_POINT ( 'NONE',  ( -8.991629940588330427, 1509.227055023859975, 237.0095830223739881 ) ) ;
#44238=CARTESIAN_POINT ( 'NONE',  ( 22.57319362359999815, 1409.701316935530031, 208.7927549349429910 ) ) ;
#44242=CARTESIAN_POINT ( 'NONE',  ( 14.66484709975379985, 1409.425168132260069, 211.9475575867689940 ) ) ;
#44246=CARTESIAN_POINT ( 'NONE',  ( -17.36186237040000080, 1412.953349025430043, 192.1948984129979863 ) ) ;
#44251=EDGE_LOOP ( 'NONE', ( #38977, #32973, #10328, #100053 ) ) ;
#44257=DIRECTION ( 'NONE',  ( 0.000000000000000000, -1.000000000000000000, 0.000000000000000000 ) ) ;
#44258=CARTESIAN_POINT ( 'NONE',  ( 32.58707754757925557, 1460.160100176146443, 269.5002707768942400 ) ) ;
#44260=CARTESIAN_POINT ( 'NONE',  ( -28.04656858090000071, 1508.051246290529889, 210.1181873726100093 ) ) ;
#44270=CARTESIAN_POINT ( 'NONE',  ( -15.68560764121220252, 1410.853875961199947, 226.7268370761429992 ) ) ;
#44274=CARTESIAN_POINT ( 'NONE',  ( -33.92723111727409702, 1435.682240498233568, 135.5030908501479985 ) ) ;
#44277=CARTESIAN_POINT ( 'NONE',  ( -25.75587219220000179, 1449.806259877490220, 208.7857563948580264 ) ) ;
#44278=CARTESIAN_POINT ( 'NONE',  ( -11.24451365029999828, 1426.879224447430033, 108.4514502916979950 ) ) ;
#44279=CARTESIAN_POINT ( 'NONE',  ( 17.20497987027239972, 1410.737466176999988, 192.2100592557800098 ) ) ;
#44281=CARTESIAN_POINT ( 'NONE',  ( 15.70278030267772351, 1509.582838606658015, 183.5495200154611837 ) ) ;
#44282=CARTESIAN_POINT ( 'NONE',  ( -21.99073835760000151, 1489.474306033830089, 208.3865218840309979 ) ) ;
#44283=CARTESIAN_POINT ( 'NONE',  ( -33.60183515869999837, 1438.777037856849802, 248.0844435640979668 ) ) ;
#44284=CARTESIAN_POINT ( 'NONE',  ( 17.06289018075510100, 1509.516276409990041, 233.1776295764580027 ) ) ;
#44285=CARTESIAN_POINT ( 'NONE',  ( 28.75826058055400125, 1509.399771093630079, 209.5084960995969823 ) ) ;
#44287=CARTESIAN_POINT ( 'NONE',  ( 30.80316622530000004, 1451.837341253830118, 134.8070091183980139 ) ) ;
#44288=ORIENTED_EDGE ( 'NONE', *, *, #29464, .F. ) ;
#44289=CARTESIAN_POINT ( 'NONE',  ( 5.776208867308529449, 1396.296062051389981, 219.5799282863600013 ) ) ;
#44291=CARTESIAN_POINT ( 'NONE',  ( -17.93598132460000016, 1458.546043109529819, 228.2699785320980084 ) ) ;
#44294=CIRCLE ( 'NONE', #58601, 0.5869955059086555682 ) ;
#44296=CARTESIAN_POINT ( 'NONE',  ( -3.181555658762940109, 1425.362665593959946, 153.9433765262999998 ) ) ;
#44298=CARTESIAN_POINT ( 'NONE',  ( 0.5133923723890000401, 1410.300673476330076, 185.0724364044980348 ) ) ;
#44301=CARTESIAN_POINT ( 'NONE',  ( -0.02516806119179999801, 1415.404723302029879, 233.4400559027980080 ) ) ;
#44302=CARTESIAN_POINT ( 'NONE',  ( 27.23667244607642601, 1509.093166509125922, 206.1841183845450587 ) ) ;
#44310=CARTESIAN_POINT ( 'NONE',  ( 11.84842883606899910, 1431.111952647210046, 149.8465606311750093 ) ) ;
#44314=ORIENTED_EDGE ( 'NONE', *, *, #109775, .T. ) ;
#44315=CARTESIAN_POINT ( 'NONE',  ( -1.459250905673769916, 1476.185953128230267, 182.8314277312189802 ) ) ;
#44317=FACE_OUTER_BOUND ( 'NONE', #109151, .T. ) ;
#44319=CARTESIAN_POINT ( 'NONE',  ( -5.549327278860000767, 1424.136432490230163, 186.3245620642980214 ) ) ;
#44320=CARTESIAN_POINT ( 'NONE',  ( 3.437535550059239942, 1409.880280454960257, 270.0719098211940263 ) ) ;
#44326=CARTESIAN_POINT ( 'NONE',  ( -18.13339771048960003, 1456.359500463610175, 190.4520856073839923 ) ) ;
#44331=CARTESIAN_POINT ( 'NONE',  ( 17.85481329854330212, 1418.946007097159963, 225.0424457944430117 ) ) ;
#44332=CARTESIAN_POINT ( 'NONE',  ( -5.792969890798230992, 1423.404851848579938, 91.44995330505670950 ) ) ;
#44334=CARTESIAN_POINT ( 'NONE',  ( 40.73184307449999864, 1436.263014496900041, 268.3665355202980436 ) ) ;
#44342=CARTESIAN_POINT ( 'NONE',  ( -24.63624201280000037, 1442.774873945370018, 210.7765137803880009 ) ) ;
#44344=CARTESIAN_POINT ( 'NONE',  ( -10.95935098528551244, 1431.615009654569576, 151.7698559583776330 ) ) ;
#44346=DIRECTION ( 'NONE',  ( 0.08330058266261865241, -0.04363816413316890658, 0.9955685428734450948 ) ) ;
#44350=CARTESIAN_POINT ( 'NONE',  ( 9.315195566419999906, 1415.075089874329933, 230.3176940828979866 ) ) ;
#44353=CARTESIAN_POINT ( 'NONE',  ( -16.68599179869999816, 1461.161699058230170, 228.2799821568980008 ) ) ;
#44355=CARTESIAN_POINT ( 'NONE',  ( 36.00838277309999569, 1418.547366844530188, 267.3063737350979636 ) ) ;
#44358=CARTESIAN_POINT ( 'NONE',  ( 23.93712380200000212, 1508.007210533329953, 195.6926836911979990 ) ) ;
#44359=CARTESIAN_POINT ( 'NONE',  ( -23.03512223430000105, 1433.464687408990130, 215.3644030352079994 ) ) ;
#44360=EDGE_CURVE ( 'NONE', #75410, #94873, #58045, .T. ) ;
#44364=CARTESIAN_POINT ( 'NONE',  ( -16.68563267514501192, 1506.380977038190167, 194.8185150136861807 ) ) ;
#44366=CARTESIAN_POINT ( 'NONE',  ( -12.84783018959999978, 1441.405291080990082, 188.1530445986979885 ) ) ;
#44371=VERTEX_POINT ( 'NONE', #4857 ) ;
#44373=CARTESIAN_POINT ( 'NONE',  ( -14.69536968390760023, 1409.426234004640037, 206.4567448585879959 ) ) ;
#44378=CARTESIAN_POINT ( 'NONE',  ( -41.92232120730000133, 1455.764491110230210, 269.0823108244979949 ) ) ;
#44380=CARTESIAN_POINT ( 'NONE',  ( 0.1600851318103049814, 1420.194783999099855, 183.7319659859389844 ) ) ;
#44381=CARTESIAN_POINT ( 'NONE',  ( -24.09814616333339998, 1444.255785637029931, 212.5772553280679915 ) ) ;
#44384=LINE ( 'NONE', #2946, #30070 ) ;
#44385=CARTESIAN_POINT ( 'NONE',  ( 13.25708502300000013, 1414.913060387329779, 218.7345124127879785 ) ) ;
#44387=CARTESIAN_POINT ( 'NONE',  ( 15.56483135290000064, 1506.802866805429858, 224.9286410369979876 ) ) ;
#44390=CARTESIAN_POINT ( 'NONE',  ( -10.28933532049999933, 1509.343598223630124, 180.9832471055979966 ) ) ;
#44392=CARTESIAN_POINT ( 'NONE',  ( -23.42828032239999914, 1409.895749727629891, 208.2087021844820072 ) ) ;
#44393=CARTESIAN_POINT ( 'NONE',  ( 15.86930212090000047, 1414.913060387329779, 206.5958717475980109 ) ) ;
#44396=CARTESIAN_POINT ( 'NONE',  ( 3.920879176457659820, 1439.701872010520219, 184.6839060028229937 ) ) ;
#44408=CIRCLE ( 'NONE', #73091, 2.000000000000000000 ) ;
#44409=CARTESIAN_POINT ( 'NONE',  ( -18.08515272772859817, 1485.385435469039976, 188.9366095778659940 ) ) ;
#44410=CARTESIAN_POINT ( 'NONE',  ( 1.427799582350000041, 1507.072958340530022, 236.7919270625980346 ) ) ;
#44414=VERTEX_POINT ( 'NONE', #108428 ) ;
#44416=CARTESIAN_POINT ( 'NONE',  ( 11.89956535492810019, 1433.601946136900096, 150.4842440392990000 ) ) ;
#44421=CARTESIAN_POINT ( 'NONE',  ( 17.93144346440610093, 1487.353935485449938, 189.1550781922330202 ) ) ;
#44422=CARTESIAN_POINT ( 'NONE',  ( 11.74015320060000001, 1428.979986575930070, 144.1938086916980239 ) ) ;
#44424=CARTESIAN_POINT ( 'NONE',  ( -0.3393288214439999506, 1507.645777512030008, 180.8011794364980176 ) ) ;
#44426=CARTESIAN_POINT ( 'NONE',  ( -24.58339591430969762, 1444.771579268069900, 210.9170101329549993 ) ) ;
#44428=CARTESIAN_POINT ( 'NONE',  ( 14.14026437185819951, 1415.666200591919960, 197.1771109711220049 ) ) ;
#44432=CARTESIAN_POINT ( 'NONE',  ( 13.80425961236019994, 1435.071252090369853, 149.2278468116170131 ) ) ;
#44434=ORIENTED_EDGE ( 'NONE', *, *, #87037, .F. ) ;
#44438=CARTESIAN_POINT ( 'NONE',  ( -2.896739157130000297, 1464.852796890729905, 236.4445922117980103 ) ) ;
#44444=CARTESIAN_POINT ( 'NONE',  ( 4.222016814108400240, 1446.225616327549915, 168.0534523820770119 ) ) ;
#44445=B_SPLINE_CURVE_WITH_KNOTS ( 'NONE', 3,
 ( #16915, #9104, #1270, #84694, #52231, #42715, #33739, #35409, #9641, #76868, #51670, #17469, #58965, #34852, #69597, #95320, #103715, #93098, #181, #60082, #42159, #34301, #102040, #25327, #59523, #85243, #68483, #94198, #10205, #16370, #85807, #44381 ),
 .UNSPECIFIED., .F., .F.,
 ( 4, 2, 2, 1, 1, 2, 2, 2, 2, 1, 1, 2, 2, 2, 2, 2, 2, 4 ),
 ( 0.000000000000000000, 0.1249999999980515863, 0.1874999999970757558, 0.2187499999965558106, 0.2343749999963441188, 0.2421874999961906305, 0.2499999999960371699, 0.3749999999951986185, 0.4374999999947972729, 0.4687499999946139750, 0.4843749999945410889, 0.4921874999944861329, 0.4999999999944311213, 0.6249999999958106844, 0.6874999999965263342, 0.7187499999969048092, 0.7499999999972831732, 1.000000000000000000 ),
 .UNSPECIFIED. ) ;
#44450=CARTESIAN_POINT ( 'NONE',  ( 24.07817550441599863, 1440.913060387330006, 235.9284644500330046 ) ) ;
#44451=CARTESIAN_POINT ( 'NONE',  ( -19.81193674840000085, 1509.671936380629859, 186.7489041350980017 ) ) ;
#44454=CARTESIAN_POINT ( 'NONE',  ( -14.12627676950000044, 1409.406360842129970, 191.9008118980979987 ) ) ;
#44455=CARTESIAN_POINT ( 'NONE',  ( -24.63623744410000072, 1442.774865482090036, 210.7765178920280107 ) ) ;
#44459=CARTESIAN_POINT ( 'NONE',  ( -13.19852776819999995, 1434.900412999929813, 149.2724498062979990 ) ) ;
#44460=CARTESIAN_POINT ( 'NONE',  ( 19.62004841539999944, 1435.182524171729938, 143.5804541147979876 ) ) ;
#44473=VERTEX_POINT ( 'NONE', #15447 ) ;
#44474=PLANE ( 'NONE',  #33437 ) ;
#44475=CARTESIAN_POINT ( 'NONE',  ( 5.301749024639999419, 1468.084175537029978, 248.5896189578980113 ) ) ;
#44476=CARTESIAN_POINT ( 'NONE',  ( -11.57648288090000044, 1432.337770414690112, 151.1968906810979831 ) ) ;
#44478=CARTESIAN_POINT ( 'NONE',  ( -7.489162529773470744, 1508.654039492000038, 236.0717299073370157 ) ) ;
#44479=CARTESIAN_POINT ( 'NONE',  ( -19.04969050960000132, 1456.540524118229996, 228.2072777489979956 ) ) ;
#44481=CARTESIAN_POINT ( 'NONE',  ( 17.45016910582259939, 1409.714858682069917, 222.5484171803500146 ) ) ;
#44482=CARTESIAN_POINT ( 'NONE',  ( -0.08793211890650000362, 1470.815019615130041, 188.6578406787979816 ) ) ;
#44488=CARTESIAN_POINT ( 'NONE',  ( -4.500000000000000000, 1418.913060387330006, 172.2701767054979882 ) ) ;
#44489=CARTESIAN_POINT ( 'NONE',  ( 19.76075415080629938, 1471.422017333550230, 270.0618168504850019 ) ) ;
#44491=CARTESIAN_POINT ( 'NONE',  ( -23.91014234936227467, 1436.885471179933802, 212.4210152180790772 ) ) ;
#44494=CARTESIAN_POINT ( 'NONE',  ( -39.77527677378599691, 1440.913060401030179, 258.9675477506260108 ) ) ;
#44495=CARTESIAN_POINT ( 'NONE',  ( 35.35472037963140224, 1450.224566512450110, 136.2317276167839850 ) ) ;
#44502=CARTESIAN_POINT ( 'NONE',  ( 3.452230076589999808, 1448.972367684420078, 184.0844731014979914 ) ) ;
#44505=CARTESIAN_POINT ( 'NONE',  ( -0.2975168056209999690, 1416.438871972429979, 233.7075449661979860 ) ) ;
#44511=CARTESIAN_POINT ( 'NONE',  ( -18.83207817909999804, 1416.311719782429918, 207.5739159116880046 ) ) ;
#44513=CARTESIAN_POINT ( 'NONE',  ( 26.46121328487780033, 1436.564390249430062, 136.7873533364920036 ) ) ;
#44514=CARTESIAN_POINT ( 'NONE',  ( -9.446360030840120103, 1396.242934550719838, 203.3640226473000041 ) ) ;
#44515=ORIENTED_EDGE ( 'NONE', *, *, #36006, .F. ) ;
#44516=( BOUNDED_CURVE ( )  B_SPLINE_CURVE ( 3, ( #13460, #40886, #108088, #71388 ),
 .UNSPECIFIED., .F., .T. ) 
 B_SPLINE_CURVE_WITH_KNOTS ( ( 4, 4 ),
 ( 2.021799836360349989, 2.259315975108074692 ),
 .UNSPECIFIED. ) 
 CURVE ( )  GEOMETRIC_REPRESENTATION_ITEM ( )  RATIONAL_B_SPLINE_CURVE ( ( 1.000000000000000000, 0.9953043629482734023, 0.9953043629482734023, 1.000000000000000000 ) ) 
 REPRESENTATION_ITEM ( '' )  );
#44517=CARTESIAN_POINT ( 'NONE',  ( -16.17741046092470114, 1409.477982791400109, 225.0323175894529868 ) ) ;
#44518=CARTESIAN_POINT ( 'NONE',  ( 9.740283752330000766, 1438.194204504490017, 148.7998369308980102 ) ) ;
#44519=ORIENTED_EDGE ( 'NONE', *, *, #68243, .F. ) ;
#44523=CARTESIAN_POINT ( 'NONE',  ( 10.65150121880000178, 1425.724714984030015, 91.14980631569790148 ) ) ;
#44524=DIRECTION ( 'NONE',  ( 3.164571201028890223E-15, -1.000000000000000000, 0.000000000000000000 ) ) ;
#44527=EDGE_CURVE ( 'NONE', #78872, #46325, #31455, .T. ) ;
#44532=CARTESIAN_POINT ( 'NONE',  ( -24.16126736702833000, 1411.115437147818739, 208.9405857977035339 ) ) ;
#44537=VERTEX_POINT ( 'NONE', #30618 ) ;
#44538=ORIENTED_EDGE ( 'NONE', *, *, #99547, .F. ) ;
#44539=CARTESIAN_POINT ( 'NONE',  ( -41.65668282690000268, 1444.004026777709896, 136.1262226100980115 ) ) ;
#44541=CARTESIAN_POINT ( 'NONE',  ( -0.2658355946003779779, 1507.129453219969946, 237.3293658036959926 ) ) ;
#44542=CARTESIAN_POINT ( 'NONE',  ( -0.4896151268140000457, 1473.897694200829847, 270.2927087789979623 ) ) ;
#44544=CARTESIAN_POINT ( 'NONE',  ( -2.790497053790000237, 1486.234749837029995, 181.8136913017980021 ) ) ;
#44548=CARTESIAN_POINT ( 'NONE',  ( -2.500000000000000000, 1448.415523929209940, 161.9475238664840049 ) ) ;
#44549=CARTESIAN_POINT ( 'NONE',  ( -12.95793659252135654, 1435.633131908374480, 150.6734405774689662 ) ) ;
#44550=CARTESIAN_POINT ( 'NONE',  ( 3.114442184824649740, 1407.350062395909845, 196.1192100924239980 ) ) ;
#44551=CARTESIAN_POINT ( 'NONE',  ( 5.471684509034499571E-05, 1406.265030819799904, 269.2947838974420165 ) ) ;
#44552=CARTESIAN_POINT ( 'NONE',  ( -14.33374980507880103, 1435.338667551370008, 149.4045105969410088 ) ) ;
#44555=CARTESIAN_POINT ( 'NONE',  ( 13.28694838949999912, 1443.173555058169995, 187.6984227527979954 ) ) ;
#44557=ORIENTED_EDGE ( 'NONE', *, *, #28541, .F. ) ;
#44565=ADVANCED_FACE ( 'NONE', ( #82678 ), #31710, .T. ) ;
#44568=CARTESIAN_POINT ( 'NONE',  ( 7.723895006289999365, 1416.216596894629902, 225.6857186377980042 ) ) ;
#44571=EDGE_CURVE ( 'NONE', #575, #4737, #91556, .T. ) ;
#44576=DIRECTION ( 'NONE',  ( 0.000000000000000000, -1.000000000000000000, 0.000000000000000000 ) ) ;
#44577=CARTESIAN_POINT ( 'NONE',  ( -6.153079222899999756, 1409.127930650229928, 230.3577016067980026 ) ) ;
#44578=CARTESIAN_POINT ( 'NONE',  ( -5.805250577859999872, 1446.068923017249972, 184.0668530776979992 ) ) ;
#44581=CARTESIAN_POINT ( 'NONE',  ( -25.11643266749259595, 1440.913060493619923, 216.7860662917659909 ) ) ;
#44584=CARTESIAN_POINT ( 'NONE',  ( -24.93438155140000134, 1435.649195298570248, 136.9390313255980232 ) ) ;
#44590=CARTESIAN_POINT ( 'NONE',  ( 21.19090038262594433, 1411.012220291270069, 200.4862705368239233 ) ) ;
#44592=ORIENTED_EDGE ( 'NONE', *, *, #56916, .T. ) ;
#44594=CARTESIAN_POINT ( 'NONE',  ( 3.008618833319030017, 1440.893622201600010, 157.1951523134509898 ) ) ;
#44597=VERTEX_POINT ( 'NONE', #85978 ) ;
#44599=CIRCLE ( 'NONE', #30265, 2.000000000000000000 ) ;
#44601=CARTESIAN_POINT ( 'NONE',  ( 12.32076549412740007, 1434.285059378609958, 149.9228593313019644 ) ) ;
#44602=B_SPLINE_SURFACE_WITH_KNOTS ( 'NONE', 5, 5, ( 
 ( #49272, #68296, #83399, #58222, #76662, #7796, #16717, #58767, #50918, #110812, #102404, #110256 ),
 ( #40852, #33531, #83955, #50380, #109178, #25686, #32463, #7255, #59880, #100739, #67732, #75027 ),
 ( #92346, #94006, #17271, #51462, #66084, #109715, #66638, #57685, #16178, #40298, #74482, #108609 ),
 ( #15618, #49825, #31898, #23493, #41417, #75583, #32990, #67179, #92905, #9458, #533, #34657 ),
 ( #102944, #60434, #79434, #35210, #69952, #52583, #69396, #104066, #68841, #20058, #53707, #17825 ),
 ( #62102, #43071, #87275, #26810, #85594, #44180, #52028, #53137, #10569, #78891, #36311, #86717 ),
 ( #10009, #87846, #86166, #35769, #36866, #26246, #77772, #18386, #45294, #2745, #104623, #60997 ),
 ( #94552, #11134, #8892, #27360, #43624, #71059, #105182, #78318, #77231, #1083, #61543, #95673 ),
 ( #103507, #18942, #70507, #1632, #28473, #62667, #95123, #44741, #2197, #27919, #96788, #96226 ),
 ( #19503, #12772, #11668, #79977, #29563, #80536, #39052, #65401, #97321, #55343, #89476, #72160 ),
 ( #105745, #56437, #13846, #73232, #88378, #46949, #29029, #55898, #98965, #31219, #37978, #107375 ),
 ( #99507, #22239, #20591, #81069, #30670, #45844, #90016, #106277, #54252, #4384, #54790, #21691 ) ),
 .UNSPECIFIED., .F., .F., .F.,
 ( 6, 3, 3, 6 ),
 ( 6, 3, 3, 6 ),
 ( 13.03551675900000006, 13.93909308159999938, 15.74624572679999979, 17.56257963661519739 ),
 ( -0.0002656258151532139909, 0.3080049601120000147, 0.9240148803369999664, 1.597676193965150038 ),
 .UNSPECIFIED. ) ;
#44603=CARTESIAN_POINT ( 'NONE',  ( 16.55300517245429859, 1488.409285182970052, 230.4335696866129979 ) ) ;
#44605=CARTESIAN_POINT ( 'NONE',  ( -23.90590786130449885, 1509.492427560550141, 224.2268974937140058 ) ) ;
#44608=CARTESIAN_POINT ( 'NONE',  ( -2.775557561559999991E-17, 1408.913060387329779, 231.7748916200980034 ) ) ;
#44609=CARTESIAN_POINT ( 'NONE',  ( 2.961376673209999755, 1417.751980673930120, 234.4067280231980135 ) ) ;
#44611=CARTESIAN_POINT ( 'NONE',  ( -2.829338567090000200, 1421.191772942729813, 185.4464042013979963 ) ) ;
#44612=CARTESIAN_POINT ( 'NONE',  ( 18.84923899389999846, 1508.518338803630058, 188.3455786348980041 ) ) ;
#44613=EDGE_LOOP ( 'NONE', ( #20537, #8595, #80911, #21288, #107300 ) ) ;
#44615=CARTESIAN_POINT ( 'NONE',  ( -19.92228370630000001, 1485.913060387229962, 190.2096421728979863 ) ) ;
#44619=CARTESIAN_POINT ( 'NONE',  ( 4.363122647530000009, 1421.971318475729959, 183.8271342376980044 ) ) ;
#44621=CARTESIAN_POINT ( 'NONE',  ( 10.20727470078544030, 1435.399071415931758, 152.3495190223391091 ) ) ;
#44626=DIRECTION ( 'NONE',  ( 1.000000000000000000, 0.000000000000000000, 0.000000000000000000 ) ) ;
#44627=CARTESIAN_POINT ( 'NONE',  ( 17.62728127150000290, 1415.048591094029916, 210.5990483032680061 ) ) ;
#44628=CARTESIAN_POINT ( 'NONE',  ( -18.26675077970000061, 1424.840336371829835, 227.6848321215980206 ) ) ;
#44629=CARTESIAN_POINT ( 'NONE',  ( -15.90533261240000051, 1435.486427895659972, 148.6044062959979897 ) ) ;
#44630=CARTESIAN_POINT ( 'NONE',  ( -0.5987183604784179769, 1507.212886163649955, 231.7504617458309895 ) ) ;
#44631=CARTESIAN_POINT ( 'NONE',  ( 16.24504166639999880, 1416.217127671729941, 191.3512804590980068 ) ) ;
#44633=CARTESIAN_POINT ( 'NONE',  ( -19.02402554036360627, 1439.750327254491367, 209.9292271237399916 ) ) ;
#44634=CARTESIAN_POINT ( 'NONE',  ( 10.82295897259685269, 1424.914574748641826, 144.7906534265950143 ) ) ;
#44635=ORIENTED_EDGE ( 'NONE', *, *, #9671, .T. ) ;
#44636=CARTESIAN_POINT ( 'NONE',  ( 0.6474875409317040198, 1507.275794996420018, 186.4417145385390029 ) ) ;
#44637=CARTESIAN_POINT ( 'NONE',  ( -9792.142915468795763, 50.28429875023824280, -1105.735995892511028 ) ) ;
#44641=CARTESIAN_POINT ( 'NONE',  ( -3.522208045919057451, 1426.008235538924737, 185.8885408405282931 ) ) ;
#44643=DIRECTION ( 'NONE',  ( -0.9901118076173108795, 0.1402804634180439824, 0.000000000000000000 ) ) ;
#44652=CARTESIAN_POINT ( 'NONE',  ( 24.04921614290000065, 1508.500197933130039, 195.9136757570979910 ) ) ;
#44653=ORIENTED_EDGE ( 'NONE', *, *, #71279, .F. ) ;
#44654=CARTESIAN_POINT ( 'NONE',  ( -1.326919697740000181, 1414.988015876829877, 226.4745228867980131 ) ) ;
#44657=CARTESIAN_POINT ( 'NONE',  ( 20.06110565012859936, 1509.143991300649986, 229.7914472179430163 ) ) ;
#44659=ORIENTED_EDGE ( 'NONE', *, *, #25237, .T. ) ;
#44660=CARTESIAN_POINT ( 'NONE',  ( 19.47176263695120113, 1508.319487713160015, 229.5268495768910100 ) ) ;
#44662=CARTESIAN_POINT ( 'NONE',  ( 13.40432466244523013, 1443.415710732174603, 169.3677059354045866 ) ) ;
#44663=CARTESIAN_POINT ( 'NONE',  ( 18.84387474539999729, 1434.822844257309953, 208.7548053377890085 ) ) ;
#44664=CARTESIAN_POINT ( 'NONE',  ( -13.01666421170000021, 1472.524044086929962, 262.4458738597979846 ) ) ;
#44665=B_SPLINE_CURVE_WITH_KNOTS ( 'NONE', 3,
 ( #85498, #103972, #86072, #27269, #42978, #76565, #27827, #77137, #86618, #44082, #9368, #78221, #95576, #18846, #16623, #77675, #10468, #44641, #78784, #2097, #62007, #50819, #34009, #102306, #84951, #68203, #8242, #42411, #59784, #37888, #87749, #88835, #80986, #106186, #28375, #88285, #70970, #13202, #3756 ),
 .UNSPECIFIED., .F., .F.,
 ( 4, 2, 2, 1, 1, 2, 2, 2, 2, 1, 1, 2, 2, 2, 2, 2, 1, 1, 1, 2, 2, 2, 4 ),
 ( 0.000000000000000000, 0.06249999999957017716, 0.09374999999935659800, 0.1093749999992551653, 0.1171874999992067318, 0.1210937499991825289, 0.1249999999991583122, 0.1874999999988822830, 0.2187499999987529697, 0.2343749999986922405, 0.2421874999986679544, 0.2460937499986559640, 0.2499999999986439736, 0.3749999999982069343, 0.4374999999979756748, 0.4687499999978566589, 0.4843749999978096965, 0.4921874999977803866, 0.4960937499977566834, 0.4980468749977415288, 0.4999999999977263743, 0.7499999999988631316, 1.000000000000000000 ),
 .UNSPECIFIED. ) ;
#44669=CARTESIAN_POINT ( 'NONE',  ( 27.59998756409999743, 1509.654128750629980, 206.1402511112580100 ) ) ;
#44671=CARTESIAN_POINT ( 'NONE',  ( 6.506310070979999693, 1410.514241582030081, 186.9556225147979944 ) ) ;
#44672=CARTESIAN_POINT ( 'NONE',  ( 5.554866099599999885, 1421.644415044730067, 186.0588715001979949 ) ) ;
#44673=CARTESIAN_POINT ( 'NONE',  ( -8.766760704440001106, 1437.289887460749924, 153.2969298518980281 ) ) ;
#44674=CARTESIAN_POINT ( 'NONE',  ( 10.43358995060000005, 1436.699218567949856, 152.2773048147980148 ) ) ;
#44676=CARTESIAN_POINT ( 'NONE',  ( 19.03110457515579768, 1457.047041246000163, 226.1578386336209974 ) ) ;
#44681=CARTESIAN_POINT ( 'NONE',  ( -44.13011771299999708, 1440.913068107089885, 270.2165841919979812 ) ) ;
#44682=CARTESIAN_POINT ( 'NONE',  ( -23.93711277806432847, 1435.908512379617378, 211.2583651232883710 ) ) ;
#44683=CARTESIAN_POINT ( 'NONE',  ( 17.11609659350000001, 1409.675656910730140, 223.5180517379979790 ) ) ;
#44685=VECTOR ( 'NONE', #43402, 1000.000000000000000 ) ;
#44688=DIRECTION ( 'NONE',  ( 0.3363363969981477131, -0.6659120918162938496, 0.6659120918162938496 ) ) ;
#44689=CARTESIAN_POINT ( 'NONE',  ( 2.279486851180000162, 1508.935250639130118, 237.8394454172980090 ) ) ;
#44690=CARTESIAN_POINT ( 'NONE',  ( -7.702505263429999971, 1417.009600301830005, 231.0840807062979820 ) ) ;
#44693=CARTESIAN_POINT ( 'NONE',  ( -44.58457768240119634, 1432.195838635359905, 268.5431226110130183 ) ) ;
#44698=VERTEX_POINT ( 'NONE', #12584 ) ;
#44702=DIRECTION ( 'NONE',  ( 0.000000000000000000, 0.000000000000000000, 1.000000000000000000 ) ) ;
#44705=FACE_OUTER_BOUND ( 'NONE', #71394, .T. ) ;
#44707=CARTESIAN_POINT ( 'NONE',  ( 12.74111566449999877, 1416.823634022829992, 196.2610674185980031 ) ) ;
#44711=EDGE_CURVE ( 'NONE', #32822, #95978, #108294, .T. ) ;
#44714=VERTEX_POINT ( 'NONE', #108844 ) ;
#44715=CARTESIAN_POINT ( 'NONE',  ( -23.40572486892139992, 1412.384539677990233, 270.0161358559570317 ) ) ;
#44717=CARTESIAN_POINT ( 'NONE',  ( 7.889072528545669094, 1418.815176736690091, 232.2028265587920259 ) ) ;
#44722=CARTESIAN_POINT ( 'NONE',  ( -23.30090455988580089, 1410.145525358959958, 210.1953146085759840 ) ) ;
#44724=CARTESIAN_POINT ( 'NONE',  ( -0.3188903335409049578, 1408.924196283109950, 186.5730539788620206 ) ) ;
#44727=CARTESIAN_POINT ( 'NONE',  ( -20.53128328073639253, 1409.661528479226718, 266.7934139810452621 ) ) ;
#44731=CARTESIAN_POINT ( 'NONE',  ( -18.75133052940000411, 1415.856152504829879, 223.8867772891979939 ) ) ;
#44732=CARTESIAN_POINT ( 'NONE',  ( 5.341581777923300578, 1476.076623253339903, 267.5369962912580490 ) ) ;
#44734=CARTESIAN_POINT ( 'NONE',  ( 10.37306595179999924, 1445.891253827790251, 186.4156611468980032 ) ) ;
#44736=VERTEX_POINT ( 'NONE', #57912 ) ;
#44737=CARTESIAN_POINT ( 'NONE',  ( -14.14968278069630081, 1452.475144026350108, 223.0094203056700053 ) ) ;
#44738=CARTESIAN_POINT ( 'NONE',  ( 1.481821286034419982, 1476.734267533799994, 182.4382444874360090 ) ) ;
#44739=VERTEX_POINT ( 'NONE', #29922 ) ;
#44741=CARTESIAN_POINT ( 'NONE',  ( 25.20984846640109822, 1451.589895632459957, 136.8724018194579912 ) ) ;
#44742=CARTESIAN_POINT ( 'NONE',  ( 14.20165756390000134, 1416.819756528530206, 196.5061806366979908 ) ) ;
#44745=CARTESIAN_POINT ( 'NONE',  ( 18.79898005950000339, 1410.492675419430043, 194.9234042622980212 ) ) ;
#44746=CARTESIAN_POINT ( 'NONE',  ( 12.73318793669440829, 1444.994950788470533, 164.6858276811441328 ) ) ;
#44747=CARTESIAN_POINT ( 'NONE',  ( 2.603541569773797359, 1439.644274085440657, 183.4060696333851865 ) ) ;
#44748=CARTESIAN_POINT ( 'NONE',  ( 0.4773158509259999849, 1416.462031948630056, 233.6651878465979735 ) ) ;
#44749=CARTESIAN_POINT ( 'NONE',  ( -22.07883734336632742, 1430.373802828663202, 217.8216703382841501 ) ) ;
#44751=DIRECTION ( 'NONE',  ( -1.000000000000000000, 0.000000000000000000, 0.000000000000000000 ) ) ;
#44759=CARTESIAN_POINT ( 'NONE',  ( -0.4465890250242970372, 1409.330979278389805, 232.7383886707189902 ) ) ;
#44763=CARTESIAN_POINT ( 'NONE',  ( -13.84930592310000108, 1450.388901282120059, 209.1218459616979999 ) ) ;
#44765=CARTESIAN_POINT ( 'NONE',  ( -2.908753373654089813, 1451.958507811900063, 184.7558797852969690 ) ) ;
#44766=CARTESIAN_POINT ( 'NONE',  ( 11.87694622159999902, 1433.083833627729973, 150.0917096319979862 ) ) ;
#44767=CARTESIAN_POINT ( 'NONE',  ( -2.115953714250000228, 1475.022810911229953, 269.6431591146979940 ) ) ;
#44769=CARTESIAN_POINT ( 'NONE',  ( 26.79041820568939869, 1440.913060391970021, 225.8523074638320054 ) ) ;
#44771=EDGE_LOOP ( 'NONE', ( #17546, #59741, #8870, #3013, #48775 ) ) ;
#44772=CARTESIAN_POINT ( 'NONE',  ( 0.1681681984989999989, 1418.913060387330006, 172.2701767054979882 ) ) ;
#44774=CARTESIAN_POINT ( 'NONE',  ( -4.682538493039999139, 1486.134978737730080, 182.1338541308979870 ) ) ;
#44775=CARTESIAN_POINT ( 'NONE',  ( 7.975931650403921935, 1398.149953820521660, 198.8561492682118228 ) ) ;
#44776=CARTESIAN_POINT ( 'NONE',  ( -15.07933690175220143, 1509.452906090019951, 236.3415195119960117 ) ) ;
#44778=CARTESIAN_POINT ( 'NONE',  ( 21.80621299799999946, 1469.235547599130086, 222.1300559395980088 ) ) ;
#44780=CARTESIAN_POINT ( 'NONE',  ( -8.365380114920000665, 1508.201457570829916, 235.3635179348979989 ) ) ;
#44782=CARTESIAN_POINT ( 'NONE',  ( 20.66053749647389992, 1495.927313020109750, 225.6903912862549930 ) ) ;
#44783=CARTESIAN_POINT ( 'NONE',  ( 10.45855884280000048, 1409.218564510729720, 219.7594970117980040 ) ) ;
#44785=CARTESIAN_POINT ( 'NONE',  ( 0.1674239622419670115, 1481.845507357109909, 182.0151124697109992 ) ) ;
#44787=ORIENTED_EDGE ( 'NONE', *, *, #54326, .F. ) ;
#44788=CARTESIAN_POINT ( 'NONE',  ( -0.5697963391879999895, 1450.893162800530263, 181.2886238165980046 ) ) ;
#44794=VERTEX_POINT ( 'NONE', #66326 ) ;
#44797=CARTESIAN_POINT ( 'NONE',  ( 27.33789150208756524, 1509.867720594859293, 198.5752084302989147 ) ) ;
#44802=CARTESIAN_POINT ( 'NONE',  ( 12.21909990819059999, 1409.339760750069900, 217.7291232207390124 ) ) ;
#44805=CARTESIAN_POINT ( 'NONE',  ( -17.56738044160000101, 1412.957744255030093, 192.5650100598980146 ) ) ;
#44807=ORIENTED_EDGE ( 'NONE', *, *, #43175, .T. ) ;
#44812=ORIENTED_EDGE ( 'NONE', *, *, #82003, .F. ) ;
#44813=B_SPLINE_CURVE_WITH_KNOTS ( 'NONE', 3,
 ( #69685, #3580, #21963, #38791, #89754, #74623 ),
 .UNSPECIFIED., .F., .F.,
 ( 4, 2, 4 ),
 ( -0.03892040104653909927, -0.01978009174228249900, -5.188642626663408919E-09 ),
 .UNSPECIFIED. ) ;
#44814=CARTESIAN_POINT ( 'NONE',  ( 24.72376531809999989, 1509.776433298830170, 223.3047247638980082 ) ) ;
#44816=CARTESIAN_POINT ( 'NONE',  ( -11.17933822150000012, 1434.140065272970105, 151.6287470207980164 ) ) ;
#44817=AXIS2_PLACEMENT_3D ( 'NONE', #86749, #36344, #78922 ) ;
#44819=CARTESIAN_POINT ( 'NONE',  ( 35.05450822442378467, 1457.715342177672028, 269.5322532702526246 ) ) ;
#44821=CARTESIAN_POINT ( 'NONE',  ( 4.717917756090000303, 1396.259829913929934, 220.1600754375980102 ) ) ;
#44822=CARTESIAN_POINT ( 'NONE',  ( 2.715010028530000064, 1417.669881552329798, 234.6652376653979957 ) ) ;
#44824=CARTESIAN_POINT ( 'NONE',  ( -1.182076869679999920, 1452.180487653529781, 183.6023549528979686 ) ) ;
#44826=CARTESIAN_POINT ( 'NONE',  ( -26.47803665465272260, 1436.726639266544453, 136.8122681834409207 ) ) ;
#44829=CARTESIAN_POINT ( 'NONE',  ( -13.02114638533239876, 1434.814403427030129, 149.4658423292819975 ) ) ;
#44830=CARTESIAN_POINT ( 'NONE',  ( -1.154631945609999823E-14, 1421.542806690330053, 144.1893924737979944 ) ) ;
#44831=CARTESIAN_POINT ( 'NONE',  ( -0.3757451851924459851, 1473.184910198040143, 188.5980016707920299 ) ) ;
#44833=CARTESIAN_POINT ( 'NONE',  ( 40.38134792428180475, 1444.189104679979891, 137.0917438250710063 ) ) ;
#44835=CARTESIAN_POINT ( 'NONE',  ( 43.50119000050000295, 1440.913060359109977, 263.8966302655979916 ) ) ;
#44836=CARTESIAN_POINT ( 'NONE',  ( -26.39526639180000345, 1469.246565964829870, 207.8134133741079950 ) ) ;
#44837=CARTESIAN_POINT ( 'NONE',  ( -10.96674589548630152, 1426.064964913880203, 96.72801120346360904 ) ) ;
#44838=CARTESIAN_POINT ( 'NONE',  ( 16.68432847059190038, 1409.595862666960102, 192.9240629956530029 ) ) ;
#44841=CARTESIAN_POINT ( 'NONE',  ( 1.175130270553210066, 1395.954096840620196, 198.1774300419000099 ) ) ;
#44843=DIRECTION ( 'NONE',  ( 1.733298337313369794E-15, -0.8730714504182227609, -0.4875922912276409171 ) ) ;
#44844=CARTESIAN_POINT ( 'NONE',  ( -25.82475784780000083, 1425.523015327230041, 244.3435519318979914 ) ) ;
#44846=CARTESIAN_POINT ( 'NONE',  ( 28.53735979763590080, 1509.098833403789740, 209.4635936774309926 ) ) ;
#44849=CARTESIAN_POINT ( 'NONE',  ( 33.52142403570000084, 1451.742483455429920, 134.7272099485979879 ) ) ;
#44850=ORIENTED_EDGE ( 'NONE', *, *, #25595, .F. ) ;
#44851=CARTESIAN_POINT ( 'NONE',  ( 3.515651971320000069, 1396.218664545030151, 197.1791320925980244 ) ) ;
#44853=EDGE_CURVE ( 'NONE', #59125, #61195, #62387, .T. ) ;
#44854=CARTESIAN_POINT ( 'NONE',  ( -16.51558990230000035, 1459.313172484830147, 228.9821122170980061 ) ) ;
#44855=ORIENTED_EDGE ( 'NONE', *, *, #58388, .F. ) ;
#44856=ORIENTED_EDGE ( 'NONE', *, *, #72941, .T. ) ;
#44864=CARTESIAN_POINT ( 'NONE',  ( -19.46624395007912156, 1486.378570646362505, 189.7119165574182205 ) ) ;
#44866=CARTESIAN_POINT ( 'NONE',  ( 27.33695563809355633, 1509.220067111051776, 206.1721638638696561 ) ) ;
#44867=CARTESIAN_POINT ( 'NONE',  ( 0.6444153132796710537, 1420.643208713479908, 182.8466803230259927 ) ) ;
#44870=FACE_OUTER_BOUND ( 'NONE', #19044, .T. ) ;
#44873=ORIENTED_EDGE ( 'NONE', *, *, #45205, .F. ) ;
#44874=CARTESIAN_POINT ( 'NONE',  ( 11.86350184823050036, 1432.154420217069855, 149.9793174209499966 ) ) ;
#44876=DIRECTION ( 'NONE',  ( 0.000000000000000000, 0.000000000000000000, -1.000000000000000000 ) ) ;
#44878=CARTESIAN_POINT ( 'NONE',  ( -15.56469051740000076, 1506.798305107229908, 193.1680121121979994 ) ) ;
#44880=CARTESIAN_POINT ( 'NONE',  ( -11.90008666459999986, 1434.920851464509951, 147.6452002888979962 ) ) ;
#44883=CARTESIAN_POINT ( 'NONE',  ( -4.593646130120000670, 1423.772470591829915, 184.4006771823979989 ) ) ;
#44884=CARTESIAN_POINT ( 'NONE',  ( 1.469863004249710059, 1407.943267555710008, 270.2923612881479585 ) ) ;
#44890=CARTESIAN_POINT ( 'NONE',  ( -18.93088166866530031, 1481.225508140669945, 189.7381378927790081 ) ) ;
#44897=CARTESIAN_POINT ( 'NONE',  ( 36.06124927020000115, 1436.776486031050126, 262.6648722463980334 ) ) ;
#44898=CARTESIAN_POINT ( 'NONE',  ( 13.72150112095459917, 1434.975563626920120, 148.6100187623320039 ) ) ;
#44900=AXIS2_PLACEMENT_3D ( 'NONE', #85520, #57613, #109106 ) ;
#44903=CARTESIAN_POINT ( 'NONE',  ( 11.79348306668460111, 1408.364582718329984, 270.1182552284680014 ) ) ;
#44908=CARTESIAN_POINT ( 'NONE',  ( -24.09704111839999996, 1443.988162845919987, 212.1154897055279775 ) ) ;
#44913=CARTESIAN_POINT ( 'NONE',  ( 6.588559639229999654, 1509.276047527829860, 179.0991342149980028 ) ) ;
#44915=CARTESIAN_POINT ( 'NONE',  ( -11.16733641199999916, 1453.313060387329870, 225.4924597496980141 ) ) ;
#44916=CARTESIAN_POINT ( 'NONE',  ( 14.66309662039999928, 1412.744218893529933, 227.7783495036979957 ) ) ;
#44920=CARTESIAN_POINT ( 'NONE',  ( 41.33291310559999943, 1425.226874449430170, 266.5540610868980025 ) ) ;
#44922=CARTESIAN_POINT ( 'NONE',  ( 18.25065742789999845, 1435.135490642300056, 145.6248056324979814 ) ) ;
#44923=CARTESIAN_POINT ( 'NONE',  ( 20.60562827940000119, 1469.157082743329966, 193.0059214098980078 ) ) ;
#44924=CARTESIAN_POINT ( 'NONE',  ( -22.49610135040000003, 1431.913548303140033, 217.2868528580380030 ) ) ;
#44926=CARTESIAN_POINT ( 'NONE',  ( -0.8855859651640000108, 1475.830651730830141, 266.9608409856979847 ) ) ;
#44928=CARTESIAN_POINT ( 'NONE',  ( -41.66467407060099504, 1443.190448348939981, 136.0675278794840040 ) ) ;
#44931=CARTESIAN_POINT ( 'NONE',  ( -12.31367500480000032, 1442.688057702260039, 186.5150438736980050 ) ) ;
#44932=CARTESIAN_POINT ( 'NONE',  ( -27.80059196791649967, 1508.274126421260007, 210.4902684585850068 ) ) ;
#44937=CARTESIAN_POINT ( 'NONE',  ( -14.92887067431809989, 1409.434388038909901, 209.5123278269470006 ) ) ;
#44939=CARTESIAN_POINT ( 'NONE',  ( -5.371114210517032639, 1422.361293165692587, 138.9481839148339759 ) ) ;
#44940=CARTESIAN_POINT ( 'NONE',  ( -44.47031950239999532, 1451.019422310730079, 266.2216427720979937 ) ) ;
#44942=CARTESIAN_POINT ( 'NONE',  ( 0.4823992292522150116, 1418.714218680099975, 184.7113719357920161 ) ) ;
#44943=CARTESIAN_POINT ( 'NONE',  ( -22.57318049250000058, 1409.701333220029937, 209.4509250479570142 ) ) ;
#44946=CARTESIAN_POINT ( 'NONE',  ( 16.94821773669399789, 1422.804739068089930, 226.9354301654539938 ) ) ;
#44947=CARTESIAN_POINT ( 'NONE',  ( 14.63039435740000016, 1416.519106787730152, 219.7110180114979983 ) ) ;
#44948=CARTESIAN_POINT ( 'NONE',  ( 15.48562912010000048, 1495.933122566730162, 224.0697311691979792 ) ) ;
#44954=CARTESIAN_POINT ( 'NONE',  ( 17.63393959649999942, 1415.931784856029935, 206.2978456718479947 ) ) ;
#44955=CARTESIAN_POINT ( 'NONE',  ( -12.26979136719999985, 1416.828040475729949, 194.6643372668980021 ) ) ;
#44957=CARTESIAN_POINT ( 'NONE',  ( 23.77260840609999804, 1411.103764635429798, 210.9084169415280030 ) ) ;
#44960=CARTESIAN_POINT ( 'NONE',  ( -15.49281651649999958, 1421.632445824929846, 227.2929371620980135 ) ) ;
#44961=CARTESIAN_POINT ( 'NONE',  ( -11.58425284650000009, 1432.866144662169972, 151.1952032978979901 ) ) ;
#44963=CARTESIAN_POINT ( 'NONE',  ( 0.3007953952340000070, 1410.295994791430076, 233.2561088422980049 ) ) ;
#44966=CARTESIAN_POINT ( 'NONE',  ( -22.52609268272879817, 1509.699688877640028, 190.9355248210520131 ) ) ;
#44967=CARTESIAN_POINT ( 'NONE',  ( -0.8004569503022459509, 1420.698947351120069, 183.5197807342519809 ) ) ;
#44970=CARTESIAN_POINT ( 'NONE',  ( -18.59208672289999953, 1425.224709566930187, 227.1497469740980080 ) ) ;
#44971=CARTESIAN_POINT ( 'NONE',  ( -14.71962813352180000, 1485.852042466279954, 186.4453625732280102 ) ) ;
#44977=CARTESIAN_POINT ( 'NONE',  ( 11.40351120802290019, 1433.961723248389944, 151.4265909395499818 ) ) ;
#44979=ORIENTED_EDGE ( 'NONE', *, *, #63202, .F. ) ;
#44981=CARTESIAN_POINT ( 'NONE',  ( 1.547463840030000037, 1414.913060387329779, 192.3096136973980208 ) ) ;
#44982=CARTESIAN_POINT ( 'NONE',  ( 15.98819541800289912, 1421.269252389829944, 191.1953072301890018 ) ) ;
#44983=CARTESIAN_POINT ( 'NONE',  ( 0.1578430167310000132, 1507.631289506030271, 180.9061429542980193 ) ) ;
#44986=CARTESIAN_POINT ( 'NONE',  ( 2.829025757189999712, 1488.172259156529890, 182.2276165502979950 ) ) ;
#44988=CARTESIAN_POINT ( 'NONE',  ( -24.14169241750170158, 1444.792590611489913, 211.6367681704030019 ) ) ;
#44989=EDGE_CURVE ( 'NONE', #61631, #50836, #89207, .T. ) ;
#44991=CARTESIAN_POINT ( 'NONE',  ( 34.31734398635919803, 1435.703512753839959, 134.0999999980490145 ) ) ;
#44993=CIRCLE ( 'NONE', #58289, 28.41070217520000440 ) ;
#44997=CARTESIAN_POINT ( 'NONE',  ( 13.74453438472139943, 1436.216212073029965, 150.3798774187329741 ) ) ;
#45000=ORIENTED_EDGE ( 'NONE', *, *, #107812, .F. ) ;
#45016=CARTESIAN_POINT ( 'NONE',  ( 23.97023455779339685, 1440.913060387330006, 235.5343584298519772 ) ) ;
#45017=CARTESIAN_POINT ( 'NONE',  ( -14.12785558649999906, 1509.345507846829832, 183.3895937959979676 ) ) ;
#45019=CARTESIAN_POINT ( 'NONE',  ( 25.58350377144139998, 1449.893453280530139, 137.3546802799529871 ) ) ;
#45021=CARTESIAN_POINT ( 'NONE',  ( -13.41649805129999962, 1409.381574823129995, 191.5176180624980020 ) ) ;
#45023=CARTESIAN_POINT ( 'NONE',  ( -24.36523717070000217, 1440.927836225630017, 211.6868765465779916 ) ) ;
#45027=CARTESIAN_POINT ( 'NONE',  ( -12.48454216434870645, 1434.418201845518297, 147.3004665988038084 ) ) ;
#45029=CARTESIAN_POINT ( 'NONE',  ( 13.80546151116429954, 1434.979654507460054, 148.5370226032280243 ) ) ;
#45030=FACE_OUTER_BOUND ( 'NONE', #110421, .T. ) ;
#45036=CARTESIAN_POINT ( 'NONE',  ( 28.27930517080000072, 1508.150008669530052, 208.9705538469389978 ) ) ;
#45042=EDGE_LOOP ( 'NONE', ( #51149, #103951, #8677, #19458 ) ) ;
#45043=CARTESIAN_POINT ( 'NONE',  ( -1.270728281904929924, 1414.996443537369942, 226.4582996361970118 ) ) ;
#45044=CARTESIAN_POINT ( 'NONE',  ( 21.39592531770000150, 1453.782470550929929, 225.7912808434980150 ) ) ;
#45045=CARTESIAN_POINT ( 'NONE',  ( -18.32069918539999875, 1457.567609363029987, 229.9399091793980006 ) ) ;
#45046=CARTESIAN_POINT ( 'NONE',  ( -11.81707110430000007, 1430.266231075130008, 147.2485970657980090 ) ) ;
#45047=CARTESIAN_POINT ( 'NONE',  ( -6.844637409469999767, 1507.263724706429912, 235.7154609632979714 ) ) ;
#45048=CARTESIAN_POINT ( 'NONE',  ( -18.97274404719999907, 1457.324312373629937, 226.8825690747979991 ) ) ;
#45050=CARTESIAN_POINT ( 'NONE',  ( -21.70628021907349137, 1411.031453783015195, 201.5216881071951605 ) ) ;
#45051=CARTESIAN_POINT ( 'NONE',  ( 5.360351092102419557, 1422.243568082540150, 144.1133778792190014 ) ) ;
#45052=CARTESIAN_POINT ( 'NONE',  ( 0.1642147860209999810, 1434.814457747790129, 190.0887174017979930 ) ) ;
#45056=CARTESIAN_POINT ( 'NONE',  ( 0.7780697151959999891, 1405.754330040730110, 267.5369108394980344 ) ) ;
#45058=B_SPLINE_CURVE_WITH_KNOTS ( 'NONE', 3,
 ( #107933, #6026, #31773, #31225, #40730, #13854, #48037, #57003, #49151, #72698, #92231 ),
 .UNSPECIFIED., .F., .F.,
 ( 4, 2, 1, 2, 2, 4 ),
 ( 0.000000000000000000, 0.2499999999999520939, 0.3749999999999407696, 0.4375000000000707212, 0.5000000000002006173, 1.000000000000000000 ),
 .UNSPECIFIED. ) ;
#45059=CARTESIAN_POINT ( 'NONE',  ( 42.00606667534940186, 1451.376206482430007, 270.3372530110870002 ) ) ;
#45060=CARTESIAN_POINT ( 'NONE',  ( 2.478410607399999854, 1438.230131886350136, 157.7118229332980093 ) ) ;
#45061=CARTESIAN_POINT ( 'NONE',  ( -40.27780736350000268, 1444.639155820560063, 137.0225327466980048 ) ) ;
#45064=CARTESIAN_POINT ( 'NONE',  ( -26.57078163029999729, 1448.091204785469927, 137.0346892529979925 ) ) ;
#45065=CARTESIAN_POINT ( 'NONE',  ( 0.5717981366250000086, 1450.893092756410169, 154.2461502948980012 ) ) ;
#45066=DIRECTION ( 'NONE',  ( 0.9952216675636860188, -0.01326783003108352073, 0.09673570746121909480 ) ) ;
#45067=CARTESIAN_POINT ( 'NONE',  ( 0.5718102594343560385, 1450.893092333070172, 154.2421351020080067 ) ) ;
#45069=CARTESIAN_POINT ( 'NONE',  ( 19.58711162175621823, 1488.292444595022744, 189.9646409983099602 ) ) ;
#45072=CARTESIAN_POINT ( 'NONE',  ( -1.612803906969698220, 1450.558055974748413, 182.3143092148731341 ) ) ;
#45074=B_SPLINE_CURVE_WITH_KNOTS ( 'NONE', 4,
 ( #14557, #91821, #108629, #75603, #83973 ),
 .UNSPECIFIED., .F., .F.,
 ( 5, 5 ),
 ( 8.673617379884035472E-19, 0.009483690916888026790 ),
 .UNSPECIFIED. ) ;
#45075=CARTESIAN_POINT ( 'NONE',  ( -0.8824136083850000478, 1475.554964337430192, 269.2944284116979929 ) ) ;
#45078=CARTESIAN_POINT ( 'NONE',  ( -3.730224799879785724, 1448.293533855142186, 184.9867838729743994 ) ) ;
#45081=CARTESIAN_POINT ( 'NONE',  ( -18.62061618460000290, 1416.021639796329964, 208.3328397087159942 ) ) ;
#45083=CARTESIAN_POINT ( 'NONE',  ( 26.61008156381389966, 1435.426649381249945, 135.3751932008159713 ) ) ;
#45084=CARTESIAN_POINT ( 'NONE',  ( -7.669900437163190254, 1396.180899213449948, 217.0741413368000110 ) ) ;
#45085=B_SPLINE_CURVE_WITH_KNOTS ( 'NONE', 5,
 ( #98204, #74681, #108814, #39408, #65177, #39957 ),
 .UNSPECIFIED., .F., .F.,
 ( 6, 6 ),
 ( 0.000000000000000000, 1.000000000000000000 ),
 .UNSPECIFIED. ) ;
#45087=CARTESIAN_POINT ( 'NONE',  ( -14.94295326230000143, 1421.973613342230010, 227.7489465375979876 ) ) ;
#45088=CARTESIAN_POINT ( 'NONE',  ( -16.68455712722449746, 1409.595976310660035, 225.3198650213400072 ) ) ;
#45089=CARTESIAN_POINT ( 'NONE',  ( 4.978523888090000682, 1441.600846913620217, 150.3430135618980046 ) ) ;
#45092=CARTESIAN_POINT ( 'NONE',  ( 1.984536219169999782, 1410.356878570029949, 232.0128186513979927 ) ) ;
#45093=CARTESIAN_POINT ( 'NONE',  ( -16.69612950000000140, 1484.879939360330127, 188.0702094165980043 ) ) ;
#45094=CARTESIAN_POINT ( 'NONE',  ( 10.77722223709999838, 1425.675087937729813, 99.60349438569788560 ) ) ;
#45098=CARTESIAN_POINT ( 'NONE',  ( -12.53380498098199602, 1442.773887284840612, 205.2015002797237173 ) ) ;
#45111=CARTESIAN_POINT ( 'NONE',  ( -13.80541478530910027, 1434.979604282769969, 148.5370187744020143 ) ) ;
#45113=CARTESIAN_POINT ( 'NONE',  ( -1.188215600249533876, 1410.329429340306433, 185.4357503969870891 ) ) ;
#45117=CARTESIAN_POINT ( 'NONE',  ( -2.500000000000000000, 1448.385612528629963, 162.4910655934610020 ) ) ;
#45118=CARTESIAN_POINT ( 'NONE',  ( 33.91369110979999846, 1435.681798629080049, 135.0664268281979901 ) ) ;
#45119=CARTESIAN_POINT ( 'NONE',  ( 13.57063579770000139, 1407.765491483530013, 211.9101277129380207 ) ) ;
#45120=CARTESIAN_POINT ( 'NONE',  ( -6.094615587868089435, 1406.362613768930032, 269.0310553213910225 ) ) ;
#45123=CARTESIAN_POINT ( 'NONE',  ( -11.76924708169999967, 1432.318127236120063, 150.8119212263979989 ) ) ;
#45124=CARTESIAN_POINT ( 'NONE',  ( 12.38749917709999870, 1442.753158610539913, 186.6620494205980094 ) ) ;
#45135=CARTESIAN_POINT ( 'NONE',  ( 11.45335004989999916, 1414.913060387329779, 222.0967534668980079 ) ) ;
#45139=CARTESIAN_POINT ( 'NONE',  ( -41.27401914175700881, 1435.068058891863529, 269.6337388993341051 ) ) ;
#45141=CARTESIAN_POINT ( 'NONE',  ( -3.714969551469999853, 1409.978796437530036, 232.2880016815979900 ) ) ;
#45142=CARTESIAN_POINT ( 'NONE',  ( -12.53380499169999851, 1445.052233488290085, 185.6742736857979992 ) ) ;
#45144=CARTESIAN_POINT ( 'NONE',  ( -4.363122561674769528, 1421.971318449149976, 184.5104913919989826 ) ) ;
#45148=CARTESIAN_POINT ( 'NONE',  ( -25.36428637739999914, 1436.617909526469930, 137.3808187117979855 ) ) ;
#45149=CARTESIAN_POINT ( 'NONE',  ( 43.06395268920530128, 1431.911435351959881, 270.2257575559060001 ) ) ;
#45153=CARTESIAN_POINT ( 'NONE',  ( 0.01445514656653382191, 1507.861152181168563, 237.5326258831030657 ) ) ;
#45155=CARTESIAN_POINT ( 'NONE',  ( 22.35774114936210566, 1411.052082638657112, 204.9822757281434349 ) ) ;
#45159=CARTESIAN_POINT ( 'NONE',  ( -4.150225335050000020, 1415.373311228230023, 232.3889413475980064 ) ) ;
#45161=VERTEX_POINT ( 'NONE', #48685 ) ;
#45164=CARTESIAN_POINT ( 'NONE',  ( 17.43470154943939932, 1478.709718884490030, 229.3935422930289860 ) ) ;
#45165=CARTESIAN_POINT ( 'NONE',  ( -23.81112428631299593, 1508.486698750989945, 222.8584575549710109 ) ) ;
#45166=MANIFOLD_SOLID_BREP ( 'Stock-MAS-682-1', #53918 ) ;
#45169=CARTESIAN_POINT ( 'NONE',  ( -0.1344824551021089887, 1420.462349845229937, 182.7339235605570025 ) ) ;
#45171=CARTESIAN_POINT ( 'NONE',  ( 16.25496458785010034, 1501.813617903470004, 193.7110474371100111 ) ) ;
#45172=CARTESIAN_POINT ( 'NONE',  ( 18.93308395989999937, 1509.362410549930246, 187.5217593452979941 ) ) ;
#45174=VERTEX_POINT ( 'NONE', #21043 ) ;
#45175=CARTESIAN_POINT ( 'NONE',  ( -12.33030208333440036, 1415.427621830080170, 196.6186630558540003 ) ) ;
#45176=CARTESIAN_POINT ( 'NONE',  ( -11.71447269829999982, 1499.713794938330011, 182.8078852171979918 ) ) ;
#45177=ORIENTED_EDGE ( 'NONE', *, *, #109197, .T. ) ;
#45179=CARTESIAN_POINT ( 'NONE',  ( 1.546867617820790075, 1416.839692126689897, 190.2222510973109877 ) ) ;
#45183=DIRECTION ( 'NONE',  ( 0.000000000000000000, 1.000000000000000000, 0.000000000000000000 ) ) ;
#45184=CARTESIAN_POINT ( 'NONE',  ( 17.60960321790000194, 1415.041103191630100, 210.5185711766079919 ) ) ;
#45185=CARTESIAN_POINT ( 'NONE',  ( -17.84085719520000168, 1424.376552934430038, 226.3470615041979670 ) ) ;
#45186=CARTESIAN_POINT ( 'NONE',  ( -22.37341732390000004, 1435.279001492649968, 139.8076879873979976 ) ) ;
#45188=CARTESIAN_POINT ( 'NONE',  ( 17.67008274869999696, 1428.766651565430038, 191.5438197617980052 ) ) ;
#45190=CARTESIAN_POINT ( 'NONE',  ( 0.5931383417482081200, 1491.015063307030005, 187.2060224152310184 ) ) ;
#45193=CARTESIAN_POINT ( 'NONE',  ( 1.556574321196450006, 1415.089996090870045, 191.4482120491740034 ) ) ;
#45194=CARTESIAN_POINT ( 'NONE',  ( 26.03031014660000153, 1488.581978119829955, 206.4905525074180161 ) ) ;
#45195=CARTESIAN_POINT ( 'NONE',  ( -24.08776747539999974, 1437.704999045569821, 212.2548087022379661 ) ) ;
#45197=CARTESIAN_POINT ( 'NONE',  ( -18.60392326990000100, 1508.243836138129836, 229.7334999568980152 ) ) ;
#45199=CARTESIAN_POINT ( 'NONE',  ( 20.65321958619999876, 1453.313060387329870, 210.0984853413359872 ) ) ;
#45205=EDGE_CURVE ( 'NONE', #45774, #24662, #39143, .T. ) ;
#45206=EDGE_CURVE ( 'NONE', #35617, #28394, #104666, .T. ) ;
#45209=CARTESIAN_POINT ( 'NONE',  ( 15.05358515032119904, 1410.831827804430077, 191.5175411757069810 ) ) ;
#45210=CARTESIAN_POINT ( 'NONE',  ( 21.39772588749999827, 1509.704957013630064, 188.4542805408979973 ) ) ;
#45212=CARTESIAN_POINT ( 'NONE',  ( -18.47236838445734719, 1458.829591624305749, 227.6520860182954777 ) ) ;
#45215=CARTESIAN_POINT ( 'NONE',  ( 20.28959732197790089, 1509.463221166710127, 230.1365879813909885 ) ) ;
#45221=CARTESIAN_POINT ( 'NONE',  ( 12.54031924683600430, 1442.774810235321866, 169.4746789495621897 ) ) ;
#45222=CARTESIAN_POINT ( 'NONE',  ( 21.20812184460000083, 1488.814055420830073, 208.7429176965079876 ) ) ;
#45223=CARTESIAN_POINT ( 'NONE',  ( 4.206714493999999137E-09, 1470.400760097329794, 255.2684105280980020 ) ) ;
#45225=CARTESIAN_POINT ( 'NONE',  ( -11.94180911519999988, 1433.516160569599833, 150.0911335117980059 ) ) ;
#45226=CARTESIAN_POINT ( 'NONE',  ( 24.04911891789999956, 1508.500175175629920, 195.9134722914980102 ) ) ;
#45227=CARTESIAN_POINT ( 'NONE',  ( 4.363122647530000009, 1421.971318475729959, 178.0486554715980105 ) ) ;
#45230=CARTESIAN_POINT ( 'NONE',  ( -9.012265790579998992, 1437.710537571299938, 153.1651550408980142 ) ) ;
#45231=DIRECTION ( 'NONE',  ( -0.000000000000000000, 1.000000000000000000, 0.000000000000000000 ) ) ;
#45236=CARTESIAN_POINT ( 'NONE',  ( -2.713960167710639967E-10, 1417.262443616730025, 235.9145977375980010 ) ) ;
#45237=B_SPLINE_CURVE_WITH_KNOTS ( 'NONE', 3,
 ( #92705, #6503, #5958, #66439, #91611, #7602, #40657, #41756, #75915, #40103, #57486, #53494, #87639 ),
 .UNSPECIFIED., .F., .F.,
 ( 4, 2, 2, 1, 2, 2, 4 ),
 ( 0.000000000000000000, 0.2499999999999987232, 0.4999999999999974465, 0.6250000000000086597, 0.6875000000000129896, 0.7500000000000173195, 1.000000000000000000 ),
 .UNSPECIFIED. ) ;
#45239=CARTESIAN_POINT ( 'NONE',  ( -34.89169900679999614, 1462.401046348830278, 269.8669090264980355 ) ) ;
#45240=EDGE_CURVE ( 'NONE', #85608, #38935, #13745, .T. ) ;
#45242=CARTESIAN_POINT ( 'NONE',  ( 6.550315845290000521E-15, 1440.444625599219989, 155.6821044880979912 ) ) ;
#45244=CARTESIAN_POINT ( 'NONE',  ( 0.9786431567949999133, 1497.713060387329961, 186.5280767325980094 ) ) ;
#45245=CARTESIAN_POINT ( 'NONE',  ( 2.823995551231429868, 1409.082596969919905, 230.6442242877770070 ) ) ;
#45246=CARTESIAN_POINT ( 'NONE',  ( 1.164704066880000166, 1507.351178548329926, 237.0483094473980259 ) ) ;
#45247=CARTESIAN_POINT ( 'NONE',  ( -11.35628460690000097, 1419.578172898530056, 229.5089160734980283 ) ) ;
#45251=CARTESIAN_POINT ( 'NONE',  ( -44.26911428083240452, 1430.613050725120047, 267.6606138304829869 ) ) ;
#45254=ORIENTED_EDGE ( 'NONE', *, *, #51620, .F. ) ;
#45260=CARTESIAN_POINT ( 'NONE',  ( 16.19492570339999915, 1409.478599654730033, 224.8086529783979870 ) ) ;
#45261=CARTESIAN_POINT ( 'NONE',  ( -7.311252174589999875, 1425.409830198830150, 186.8070320980980057 ) ) ;
#45262=ORIENTED_EDGE ( 'NONE', *, *, #6835, .F. ) ;
#45264=CARTESIAN_POINT ( 'NONE',  ( 13.15607067970000088, 1416.813004075630033, 196.3352670360980312 ) ) ;
#45265=CARTESIAN_POINT ( 'NONE',  ( 11.60004869885203682, 1425.327753716559073, 136.8073925826587356 ) ) ;
#45271=CARTESIAN_POINT ( 'NONE',  ( -9.540560617780160513, 1410.806727061010179, 269.8726498066840236 ) ) ;
#45273=CARTESIAN_POINT ( 'NONE',  ( -0.8041763403130000043, 1426.566393376330097, 144.1938086916980239 ) ) ;
#45277=ORIENTED_EDGE ( 'NONE', *, *, #20160, .F. ) ;
#45278=CARTESIAN_POINT ( 'NONE',  ( 33.30246916720928851, 1464.284855331462268, 269.2880880758933699 ) ) ;
#45280=CARTESIAN_POINT ( 'NONE',  ( 3.627035553931058143, 1424.689726282432957, 184.6936925814563040 ) ) ;
#45282=CARTESIAN_POINT ( 'NONE',  ( -17.80515869325809675, 1415.152886231989896, 207.5654953169710097 ) ) ;
#45283=CARTESIAN_POINT ( 'NONE',  ( -19.30882480040000004, 1420.833581750830035, 223.3059896308980115 ) ) ;
#45286=CARTESIAN_POINT ( 'NONE',  ( -17.36858564312840869, 1422.635098520762767, 226.5745447126183763 ) ) ;
#45289=CARTESIAN_POINT ( 'NONE',  ( 19.44016575157431603, 1410.953682894560870, 220.9327019326229333 ) ) ;
#45290=CARTESIAN_POINT ( 'NONE',  ( 1.472587025414080042, 1484.115384728570234, 182.1162732876320263 ) ) ;
#45291=ORIENTED_EDGE ( 'NONE', *, *, #30216, .T. ) ;
#45294=CARTESIAN_POINT ( 'NONE',  ( 25.98086901942570037, 1451.279931479090010, 136.5097477484009971 ) ) ;
#45298=CARTESIAN_POINT ( 'NONE',  ( 16.65035232609999838, 1409.494503502829957, 193.9825473880979985 ) ) ;
#45299=CARTESIAN_POINT ( 'NONE',  ( 20.17294526779999941, 1444.994950788469851, 161.5349527656980229 ) ) ;
#45300=FACE_OUTER_BOUND ( 'NONE', #4108, .T. ) ;
#45301=CARTESIAN_POINT ( 'NONE',  ( 0.1391290138140000021, 1415.759273717029828, 233.4531323245979877 ) ) ;
#45302=CARTESIAN_POINT ( 'NONE',  ( -22.83227036410434252, 1432.448231568467236, 215.4813152793481095 ) ) ;
#45303=B_SPLINE_CURVE_WITH_KNOTS ( 'NONE', 3,
 ( #74155, #38863, #4719, #29365, #47284, #20405 ),
 .UNSPECIFIED., .F., .F.,
 ( 4, 2, 4 ),
 ( 0.000000000000000000, 0.5000000000000000000, 1.000000000000000000 ),
 .UNSPECIFIED. ) ;
#45304=CARTESIAN_POINT ( 'NONE',  ( 0.3611859533326580163, 1452.655354317530055, 183.2864753396520143 ) ) ;
#45305=ADVANCED_FACE ( 'NONE', ( #2678 ), #45450, .T. ) ;
#45307=EDGE_CURVE ( 'NONE', #9799, #102747, #60629, .T. ) ;
#45311=CARTESIAN_POINT ( 'NONE',  ( 11.73700276120000119, 1426.696009609230032, 144.1682878315979792 ) ) ;
#45312=B_SPLINE_SURFACE_WITH_KNOTS ( 'NONE', 5, 5, ( 
 ( #103347, #68145, #9314, #101139, #42922, #24433 ),
 ( #68684, #59184, #59724, #17116, #94395, #102255 ),
 ( #92752, #16030, #60848, #25534, #76508, #50759 ),
 ( #18241, #110658, #50229, #51304, #7647, #93303 ),
 ( #387, #75961, #33385, #8739, #33951, #67581 ),
 ( #77079, #86014, #77621, #85441, #71472, #10410 ) ),
 .UNSPECIFIED., .F., .F., .F.,
 ( 6, 6 ),
 ( 6, 6 ),
 ( 30.60719516609999857, 168.0115522031930197 ),
 ( -0.001304583034726280013, 2.000849590660000121 ),
 .UNSPECIFIED. ) ;
#45313=CARTESIAN_POINT ( 'NONE',  ( -0.2682795917991919743, 1457.891717849350016, 229.2666142623699841 ) ) ;
#45315=CARTESIAN_POINT ( 'NONE',  ( 8561.628222780833312, 50.13405481578727318, 11261.64903810669421 ) ) ;
#45316=CARTESIAN_POINT ( 'NONE',  ( -37.84132625714809706, 1448.955271367279920, 136.3629971985199916 ) ) ;
#45318=CARTESIAN_POINT ( 'NONE',  ( -25.65427091389999958, 1447.057116126660048, 243.9198229428980085 ) ) ;
#45319=EDGE_CURVE ( 'NONE', #101369, #107891, #24480, .T. ) ;
#45320=CARTESIAN_POINT ( 'NONE',  ( 0.1681681984989999989, 1413.717199569329750, 164.8680577770979880 ) ) ;
#45321=CARTESIAN_POINT ( 'NONE',  ( 11.79467674799999877, 1433.007546473260163, 150.6262850383980094 ) ) ;
#45322=CARTESIAN_POINT ( 'NONE',  ( -38.67644254896129752, 1458.284314194199851, 269.8062628433829673 ) ) ;
#45323=CARTESIAN_POINT ( 'NONE',  ( 27.58375870893669912, 1440.913060388060103, 229.4262493117180099 ) ) ;
#45326=EDGE_LOOP ( 'NONE', ( #24125, #107093, #73791, #40978 ) ) ;
#45328=CARTESIAN_POINT ( 'NONE',  ( 15.23086226699999912, 1495.985335716230111, 224.7399028826979759 ) ) ;
#45329=CARTESIAN_POINT ( 'NONE',  ( -5.873126364289999124, 1486.384359668930074, 182.2278923802979875 ) ) ;
#45333=CARTESIAN_POINT ( 'NONE',  ( 24.41209542509999864, 1449.795792320089959, 214.5721300427080109 ) ) ;
#45335=DIRECTION ( 'NONE',  ( -0.1831271638493041642, -0.06610684103802308420, -0.9808640718409884496 ) ) ;
#45338=SPHERICAL_SURFACE ( 'NONE', #42063, 1.999998248449999849 ) ;
#45339=CARTESIAN_POINT ( 'NONE',  ( 1.704989397879402180, 1417.527060573706422, 233.7744594592636815 ) ) ;
#45342=ADVANCED_FACE ( 'NONE', ( #55150 ), #104011, .F. ) ;
#45344=ORIENTED_EDGE ( 'NONE', *, *, #14146, .T. ) ;
#45345=CARTESIAN_POINT ( 'NONE',  ( -12.29654148988069373, 1445.052233488290085, 164.4841150006940325 ) ) ;
#45347=CARTESIAN_POINT ( 'NONE',  ( -28.34436310520023738, 1509.902867357751347, 216.0097923534701749 ) ) ;
#45351=ORIENTED_EDGE ( 'NONE', *, *, #80382, .F. ) ;
#45353=CARTESIAN_POINT ( 'NONE',  ( -17.84636972919999920, 1416.824060884729988, 211.9816702729980022 ) ) ;
#45358=CARTESIAN_POINT ( 'NONE',  ( -23.55087667009999919, 1411.110693366829764, 210.4794020521279947 ) ) ;
#45360=CARTESIAN_POINT ( 'NONE',  ( 14.82290709384709970, 1409.430687709029826, 210.9403263768460022 ) ) ;
#45363=CARTESIAN_POINT ( 'NONE',  ( -17.29603831340000042, 1410.862735422030028, 192.2532255665980188 ) ) ;
#45367=CARTESIAN_POINT ( 'NONE',  ( -0.7910245917146945249, 1426.918876941764893, 137.0999999980979851 ) ) ;
#45370=CARTESIAN_POINT ( 'NONE',  ( -11.97935895653369975, 1415.724942525250071, 194.9476232739520185 ) ) ;
#45371=CARTESIAN_POINT ( 'NONE',  ( -11.88165080699999976, 1433.650567186270109, 150.7135751917980144 ) ) ;
#45372=CARTESIAN_POINT ( 'NONE',  ( 16.18176546483328337, 1469.066097393567134, 269.3698469196583005 ) ) ;
#45374=CARTESIAN_POINT ( 'NONE',  ( 2.228686234730000049, 1395.990887825629898, 219.9947577375980359 ) ) ;
#45378=CARTESIAN_POINT ( 'NONE',  ( -1.447759217700000045, 1462.381657091629904, 183.4226446242979875 ) ) ;
#45380=CARTESIAN_POINT ( 'NONE',  ( -20.84167267519909927, 1473.796631674460059, 208.8510855306950020 ) ) ;
#45381=ADVANCED_FACE ( 'NONE', ( #5830 ), #15184, .T. ) ;
#45383=CARTESIAN_POINT ( 'NONE',  ( -12.97884118909520090, 1435.865575512450050, 150.7205278897419873 ) ) ;
#45384=CARTESIAN_POINT ( 'NONE',  ( 1.546896711520000078, 1416.831925117829996, 190.2226034001980111 ) ) ;
#45386=CARTESIAN_POINT ( 'NONE',  ( 9277.788495748482092, 2833.746317950237426, 5939.014819510221969 ) ) ;
#45390=FACE_OUTER_BOUND ( 'NONE', #2247, .T. ) ;
#45391=CARTESIAN_POINT ( 'NONE',  ( -25.55495559180000242, 1449.803351303929958, 207.8073733729480068 ) ) ;
#45392=CARTESIAN_POINT ( 'NONE',  ( 1.448541675109999760, 1507.271700846029944, 181.1064074016979930 ) ) ;
#45393=CARTESIAN_POINT ( 'NONE',  ( -1.468632328674980059, 1507.614846039610256, 232.0487233915610261 ) ) ;
#45396=CARTESIAN_POINT ( 'NONE',  ( 1.007819525709999926E-09, 1413.088571902429976, 250.5651368501980585 ) ) ;
#45400=CARTESIAN_POINT ( 'NONE',  ( 31.79026207699999773, 1451.347618454329904, 136.0085524639980008 ) ) ;
#45401=ORIENTED_EDGE ( 'NONE', *, *, #20636, .T. ) ;
#45404=CARTESIAN_POINT ( 'NONE',  ( 5.915282300339999466, 1509.133079420229933, 238.3429575466979884 ) ) ;
#45408=CARTESIAN_POINT ( 'NONE',  ( -23.56625521110860078, 1410.013281350479929, 208.7413815090230003 ) ) ;
#45409=VERTEX_POINT ( 'NONE', #69064 ) ;
#45410=CARTESIAN_POINT ( 'NONE',  ( 0.3641805756409999817, 1424.317995881729985, 227.5054904077979927 ) ) ;
#45412=CARTESIAN_POINT ( 'NONE',  ( -0.3409206044646166944, 1415.414754857631124, 233.4258456977717913 ) ) ;
#45413=CARTESIAN_POINT ( 'NONE',  ( -1.697089624030000188, 1470.485572925830184, 235.4907127086979699 ) ) ;
#45416=ORIENTED_EDGE ( 'NONE', *, *, #32198, .F. ) ;
#45417=CARTESIAN_POINT ( 'NONE',  ( 11.73650491189999912, 1426.280347616930158, 144.1690576437979985 ) ) ;
#45423=ORIENTED_EDGE ( 'NONE', *, *, #59764, .F. ) ;
#45424=CARTESIAN_POINT ( 'NONE',  ( 11.85970193668129902, 1431.889404567069960, 149.9640874058029851 ) ) ;
#45425=CARTESIAN_POINT ( 'NONE',  ( 13.36058313908647044, 1444.493815334265719, 187.6475059284200029 ) ) ;
#45428=CARTESIAN_POINT ( 'NONE',  ( -13.35741048202589809, 1443.913060387329324, 164.9741927960640453 ) ) ;
#45429=CARTESIAN_POINT ( 'NONE',  ( 10.84641677149999950, 1508.005366378329882, 234.2312760136979648 ) ) ;
#45431=CARTESIAN_POINT ( 'NONE',  ( 22.74411444316890041, 1452.118818409569940, 139.2434547346800002 ) ) ;
#45432=CARTESIAN_POINT ( 'NONE',  ( 4.301461580539999829, 1407.800349814830042, 270.1336327149980434 ) ) ;
#45438=CARTESIAN_POINT ( 'NONE',  ( 0.03183378633081759140, 1410.137908188304209, 233.2064185424406730 ) ) ;
#45440=CARTESIAN_POINT ( 'NONE',  ( 14.57547838410000018, 1434.997135647729920, 195.8289395455979900 ) ) ;
#45445=ORIENTED_EDGE ( 'NONE', *, *, #107596, .F. ) ;
#45446=CARTESIAN_POINT ( 'NONE',  ( 25.52872274739999980, 1431.191366579289934, 248.0989693021979861 ) ) ;
#45448=CARTESIAN_POINT ( 'NONE',  ( 19.74164504280149757, 1455.376031929259852, 226.0788368184279875 ) ) ;
#45450=B_SPLINE_SURFACE_WITH_KNOTS ( 'NONE', 5, 5, ( 
 ( #12144, #98352, #45225, #12697, #29490, #72093, #46879, #105112, #53631, #79916, #87773, #106747 ),
 ( #28959, #21624, #63148, #27850, #47415, #36248, #46335, #80465, #97249, #55829, #20525, #62031 ),
 ( #70436, #3779, #19988, #21074, #28402, #64228, #96153, #45781, #3229, #11054, #19430, #79364 ),
 ( #89950, #88859, #37911, #97796, #106207, #81536, #63685, #55279, #54731, #36802, #72616, #70994 ),
 ( #37356, #4313, #71556, #62602, #105676, #89409, #38441, #30035, #31142, #65329, #82097, #91046 ),
 ( #73162, #98898, #5398, #23286, #109518, #66435, #13772, #99438, #39556, #90497, #22715, #49622 ),
 ( #4838, #57482, #107307, #91607, #64788, #14334, #14884, #74281, #31693, #38986, #47957, #32255 ),
 ( #48524, #23831, #107853, #82663, #49075, #83210, #74824, #24388, #22167, #6499, #5954, #56915 ),
 ( #40099, #40651, #56366, #7052, #108968, #32794, #73730, #108410, #100551, #65876, #30601, #58023 ),
 ( #66978, #99995, #58572, #92158, #15431, #92700, #83755, #41209, #75379, #101089, #15977, #50179 ),
 ( #76459, #7597, #78112, #26031, #35555, #110613, #60226, #69750, #93255, #60795, #77574, #9265 ),
 ( #51827, #8688, #25484, #9806, #43425, #1414, #882, #16519, #103291, #85965, #33338, #17622 ) ),
 .UNSPECIFIED., .F., .F., .F.,
 ( 6, 3, 3, 6 ),
 ( 6, 3, 3, 6 ),
 ( 9.583913663940000660, 9.799048146840000584, 10.22931711260000043, 10.62862691149999961 ),
 ( 0.000000000000000000, 0.5190412869870000279, 1.557123860959999995, 2.181622595539999931 ),
 .UNSPECIFIED. ) ;
#45455=ORIENTED_EDGE ( 'NONE', *, *, #82845, .T. ) ;
#45457=CARTESIAN_POINT ( 'NONE',  ( -24.28111689179999999, 1443.009146190699994, 211.5138934351579962 ) ) ;
#45462=CARTESIAN_POINT ( 'NONE',  ( 5.368952396500120017, 1422.346041120678137, 139.6186957304907423 ) ) ;
#45463=CARTESIAN_POINT ( 'NONE',  ( 30.68911337542330031, 1510.023616807530061, 207.3140646301669960 ) ) ;
#45466=CARTESIAN_POINT ( 'NONE',  ( -13.38643379071410067, 1424.212137269759978, 222.1368579475470142 ) ) ;
#45467=CARTESIAN_POINT ( 'NONE',  ( 14.08419818750000019, 1417.423210508630063, 228.3178852520979945 ) ) ;
#45469=CARTESIAN_POINT ( 'NONE',  ( -15.95951032299999817, 1459.271785846329976, 230.7209114582980192 ) ) ;
#45471=CARTESIAN_POINT ( 'NONE',  ( 45.67178907760000328, 1438.934187320510091, 266.1885947808980291 ) ) ;
#45472=CARTESIAN_POINT ( 'NONE',  ( -17.08792848909999762, 1409.509783999230194, 223.5124184947979984 ) ) ;
#45473=CARTESIAN_POINT ( 'NONE',  ( 21.52776548289999781, 1435.248012972100014, 141.8788503976979882 ) ) ;
#45474=CARTESIAN_POINT ( 'NONE',  ( 21.56160677299999762, 1488.583446177329961, 192.9734763627979817 ) ) ;
#45476=CARTESIAN_POINT ( 'NONE',  ( 22.33217208762076567, 1507.117986420830903, 213.2665276028900223 ) ) ;
#45480=CARTESIAN_POINT ( 'NONE',  ( -35.96078749620780002, 1435.914108659089834, 135.0260228449310205 ) ) ;
#45481=CARTESIAN_POINT ( 'NONE',  ( -8.177500540760000547, 1409.018193663230022, 197.5736553931980097 ) ) ;
#45483=CARTESIAN_POINT ( 'NONE',  ( -12.22014152740000092, 1442.565459838870083, 186.7736584056979723 ) ) ;
#45485=CARTESIAN_POINT ( 'NONE',  ( -27.83433503068760118, 1508.487004160019978, 210.5257724136350248 ) ) ;
#45486=CARTESIAN_POINT ( 'NONE',  ( -32.76525573750000575, 1435.801895108220151, 135.9795175970980097 ) ) ;
#45487=SPHERICAL_SURFACE ( 'NONE', #99727, 2.000000000000000000 ) ;
#45489=ADVANCED_FACE ( 'NONE', ( #28135 ), #52805, .F. ) ;
#45491=CARTESIAN_POINT ( 'NONE',  ( -5.462998291771629766, 1409.103832491430012, 223.0682412077159995 ) ) ;
#45492=CARTESIAN_POINT ( 'NONE',  ( 13.04908991639337223, 1414.913372219064513, 198.1359170763897453 ) ) ;
#45493=DIRECTION ( 'NONE',  ( -1.000000000000000000, 0.000000000000000000, 0.000000000000000000 ) ) ;
#45495=CARTESIAN_POINT ( 'NONE',  ( -31.69092635890000054, 1466.505745313929992, 267.1138753099980363 ) ) ;
#45498=CARTESIAN_POINT ( 'NONE',  ( 0.4850247063263399827, 1418.706296401290047, 184.7123392401769877 ) ) ;
#45499=CARTESIAN_POINT ( 'NONE',  ( -25.66084629220000224, 1508.559638941529784, 218.3457568381680005 ) ) ;
#45503=CARTESIAN_POINT ( 'NONE',  ( 15.87297696450000117, 1415.931391677429929, 217.5250545781579774 ) ) ;
#45504=CARTESIAN_POINT ( 'NONE',  ( 15.82374665889999932, 1506.811133753330068, 224.4050091913979941 ) ) ;
#45505=EDGE_CURVE ( 'NONE', #101515, #35341, #107613, .T. ) ;
#45512=CARTESIAN_POINT ( 'NONE',  ( -11.65314573679999910, 1415.128105759529944, 195.5562631955979782 ) ) ;
#45514=CARTESIAN_POINT ( 'NONE',  ( 23.34735829830000142, 1409.892898176630069, 210.3646172626779958 ) ) ;
#45517=CARTESIAN_POINT ( 'NONE',  ( -15.64558125519999798, 1421.345168983629947, 227.1284469843980105 ) ) ;
#45518=CARTESIAN_POINT ( 'NONE',  ( -11.76895986610000122, 1432.299385031119982, 150.8120305877979774 ) ) ;
#45520=CARTESIAN_POINT ( 'NONE',  ( 1.360111617359999858, 1413.043121558629991, 232.7545279162980023 ) ) ;
#45521=CARTESIAN_POINT ( 'NONE',  ( -1.905692013638440199E-05, 1510.912288461360276, 238.4016852072749941 ) ) ;
#45524=CARTESIAN_POINT ( 'NONE',  ( -23.01761228259999825, 1420.939394082029821, 211.7869335952879908 ) ) ;
#45528=CARTESIAN_POINT ( 'NONE',  ( -18.07065601792569609, 1485.598387672470153, 188.8799623616880012 ) ) ;
#45536=CARTESIAN_POINT ( 'NONE',  ( 28.15433651829999917, 1508.637654299029919, 210.1278126086380098 ) ) ;
#45539=CARTESIAN_POINT ( 'NONE',  ( 1.442946131862450132, 1414.913527292460003, 192.0294442267889963 ) ) ;
#45540=CARTESIAN_POINT ( 'NONE',  ( 2.409586283469999923, 1426.663880916129983, 144.1938086916980239 ) ) ;
#45541=CARTESIAN_POINT ( 'NONE',  ( 15.69039281178419998, 1410.711140847010029, 191.5212508507599978 ) ) ;
#45543=CARTESIAN_POINT ( 'NONE',  ( -25.01942180936440252, 1452.023553701150149, 135.7955166689109774 ) ) ;
#45545=CARTESIAN_POINT ( 'NONE',  ( 11.06788630610000013, 1410.673659464129969, 229.4061172066979850 ) ) ;
#45546=( LENGTH_UNIT ( ) NAMED_UNIT ( * ) SI_UNIT ( .MILLI., .METRE. ) );
#45548=CARTESIAN_POINT ( 'NONE',  ( 41.54171725203300269, 1442.308966536529852, 134.0999999980950008 ) ) ;
#45550=CARTESIAN_POINT ( 'NONE',  ( -0.5649602707880300168, 1422.725929253230106, 228.0279234539580102 ) ) ;
#45554=ORIENTED_EDGE ( 'NONE', *, *, #68587, .F. ) ;
#45558=CARTESIAN_POINT ( 'NONE',  ( -1.371657577609999734, 1464.950064278530135, 237.5599504942979934 ) ) ;
#45559=CARTESIAN_POINT ( 'NONE',  ( 24.13517773408675637, 1450.842116807829370, 139.9688489162871861 ) ) ;
#45564=CARTESIAN_POINT ( 'NONE',  ( 4.232600372065029148, 1446.314696765329927, 164.3435975946949839 ) ) ;
#45569=CARTESIAN_POINT ( 'NONE',  ( 28.76621075204660016, 1440.913060387330006, 249.4063077180399830 ) ) ;
#45570=CARTESIAN_POINT ( 'NONE',  ( -13.70772810569999933, 1507.648154634329785, 184.2587348614979987 ) ) ;
#45572=CARTESIAN_POINT ( 'NONE',  ( 25.40180382489500133, 1449.929728973520014, 137.7573714004559804 ) ) ;
#45573=CARTESIAN_POINT ( 'NONE',  ( -13.50742185299999853, 1409.384749952230095, 191.0679001674980100 ) ) ;
#45575=CARTESIAN_POINT ( 'NONE',  ( -24.49670940789999918, 1441.012068752339928, 210.9962413173979883 ) ) ;
#45579=CARTESIAN_POINT ( 'NONE',  ( 26.46631635538070171, 1441.292691108139934, 137.7246575186629798 ) ) ;
#45580=CARTESIAN_POINT ( 'NONE',  ( -0.5624690339869999889, 1416.828040475229955, 227.7677324846980014 ) ) ;
#45582=CARTESIAN_POINT ( 'NONE',  ( 7.830985173529999344, 1465.248213122329844, 233.1377974544980134 ) ) ;
#45584=B_SPLINE_SURFACE_WITH_KNOTS ( 'NONE', 5, 5, ( 
 ( #86470, #84262, #9765, #43930, #78074, #110022, #33298, #24881, #61318 ),
 ( #38272, #37188, #63525, #18700, #28785, #2508, #72456, #36632, #80294 ),
 ( #104939, #87026, #97096, #10315, #62985, #46165, #70272, #79202, #88151 ),
 ( #44489, #95436, #19815, #27680, #53453, #28229, #62415, #12531, #78634 ),
 ( #97641, #88701, #20361, #11439, #89236, #1950, #70829, #36087, #106047 ),
 ( #19246, #104382, #46710, #71383, #71935, #3060, #80839, #3610, #61864 ),
 ( #52896, #45613, #4146, #95982, #45059, #106586, #37733, #11982, #96541 ),
 ( #20909, #87598, #29324, #10887, #54021, #79754, #54568, #55114, #105494 ),
 ( #56600, #39993, #59021, #83104, #101529, #6397, #76359, #24281, #67430 ) ),
 .UNSPECIFIED., .F., .F., .F.,
 ( 6, 3, 6 ),
 ( 6, 3, 6 ),
 ( 24.26519376777359938, 81.54878211889999307, 143.5773940184259914 ),
 ( -1.648442643857350279E-05, 1.000000000000000000, 2.000000000000000000 ),
 .UNSPECIFIED. ) ;
#45588=CARTESIAN_POINT ( 'NONE',  ( 28.30491475510000043, 1508.660124198729818, 209.1118525407709967 ) ) ;
#45595=CARTESIAN_POINT ( 'NONE',  ( 12.07243613799999871, 1460.326362140629954, 225.7701189090979881 ) ) ;
#45598=B_SPLINE_CURVE_WITH_KNOTS ( 'NONE', 5,
 ( #7978, #102570, #42145, #91988, #32640, #59509, #7433, #66817, #76295, #32086, #67368, #93620, #110446, #83578, #100918 ),
 .UNSPECIFIED., .F., .F.,
 ( 6, 3, 3, 3, 6 ),
 ( 0.000000000000000000, 0.4627888344713468327, 0.6711646527968716525, 0.8795404711197383207, 1.000000000000000000 ),
 .UNSPECIFIED. ) ;
#45599=CARTESIAN_POINT ( 'NONE',  ( 2.423063561509999797, 1413.145749552529878, 231.8690496875979932 ) ) ;
#45600=CARTESIAN_POINT ( 'NONE',  ( -21.85910063620000088, 1453.198086485429940, 221.3407792903979896 ) ) ;
#45602=CARTESIAN_POINT ( 'NONE',  ( 11.30563928619999992, 1432.585747834659969, 151.5215852997980051 ) ) ;
#45603=CARTESIAN_POINT ( 'NONE',  ( 2.500000000000000000, 1419.383622618830032, 144.0642111274979982 ) ) ;
#45606=ORIENTED_EDGE ( 'NONE', *, *, #29464, .T. ) ;
#45608=CARTESIAN_POINT ( 'NONE',  ( 2.764799436670000166, 1406.050782495030035, 266.9581426506979938 ) ) ;
#45613=CARTESIAN_POINT ( 'NONE',  ( 43.15564358093790531, 1451.913820396499887, 269.9353367763740721 ) ) ;
#45615=CARTESIAN_POINT ( 'NONE',  ( 11.60004869885203682, 1425.703865685336950, 137.2034341738751948 ) ) ;
#45617=CARTESIAN_POINT ( 'NONE',  ( -42.70248986958939952, 1440.913060410629896, 262.8263052157859647 ) ) ;
#45618=CARTESIAN_POINT ( 'NONE',  ( -26.10199334550000216, 1450.812712592959997, 136.5826195815980100 ) ) ;
#45619=CARTESIAN_POINT ( 'NONE',  ( 2.480969307444100824, 1449.204756430078305, 154.5165407172336813 ) ) ;
#45622=CARTESIAN_POINT ( 'NONE',  ( 2.428387238925930003, 1449.547206817880124, 154.5200438689840325 ) ) ;
#45624=CARTESIAN_POINT ( 'NONE',  ( 17.61232072907009183, 1419.013269976926495, 192.1957838308312603 ) ) ;
#45625=VERTEX_POINT ( 'NONE', #35996 ) ;
#45626=CARTESIAN_POINT ( 'NONE',  ( -8.518323185650000795, 1421.108130360029918, 243.9198229428980085 ) ) ;
#45630=CARTESIAN_POINT ( 'NONE',  ( -0.3370799029359999310, 1475.560362204430021, 269.2946826080980145 ) ) ;
#45631=CARTESIAN_POINT ( 'NONE',  ( -4.276217621826190474, 1446.770458205470050, 157.0792581084560311 ) ) ;
#45632=CARTESIAN_POINT ( 'NONE',  ( -29.03008525319999933, 1509.878129414930072, 210.7880756198580059 ) ) ;
#45633=CARTESIAN_POINT ( 'NONE',  ( -2.581589687633328190, 1448.238659858906885, 183.7528642536733798 ) ) ;
#45635=ADVANCED_FACE ( 'NONE', ( #71847 ), #2531, .T. ) ;
#45636=CARTESIAN_POINT ( 'NONE',  ( -18.26532265589999682, 1415.628674266529742, 208.3526068587169959 ) ) ;
#45637=CARTESIAN_POINT ( 'NONE',  ( 11.86629848900230044, 1432.349867578880094, 149.9824231379060109 ) ) ;
#45638=CARTESIAN_POINT ( 'NONE',  ( 26.57100915839980004, 1436.736808227760093, 136.7943505115389939 ) ) ;
#45640=CARTESIAN_POINT ( 'NONE',  ( -3.600652903801630167, 1396.038797957620091, 219.5432229722080137 ) ) ;
#45641=CARTESIAN_POINT ( 'NONE',  ( -15.06279246729999954, 1422.388300733229926, 229.4662110884979995 ) ) ;
#45642=CARTESIAN_POINT ( 'NONE',  ( -15.91967948788279941, 1410.116195902319987, 226.5116202349179844 ) ) ;
#45643=CARTESIAN_POINT ( 'NONE',  ( 19.35767929529869491, 1455.763342789462740, 225.4551115454407295 ) ) ;
#45648=CARTESIAN_POINT ( 'NONE',  ( 11.17535018360000088, 1426.465084552229882, 103.4411484046980121 ) ) ;
#45650=DIRECTION ( 'NONE',  ( 0.03489949670250328678, 0.9993908270190956511, 0.000000000000000000 ) ) ;
#45651=B_SPLINE_CURVE_WITH_KNOTS ( 'NONE', 5,
 ( #24300, #15885, #101546, #94830, #19770, #18106 ),
 .UNSPECIFIED., .F., .F.,
 ( 6, 6 ),
 ( -1.452619041900000019, -2.358414258996077706E-06 ),
 .UNSPECIFIED. ) ;
#45656=CARTESIAN_POINT ( 'NONE',  ( 6.806851077879999323, 1507.558626602530012, 182.5007774465980219 ) ) ;
#45657=CARTESIAN_POINT ( 'NONE',  ( -0.2223009154971570256, 1416.826860677879949, 191.0546700833079967 ) ) ;
#45662=ORIENTED_EDGE ( 'NONE', *, *, #69339, .F. ) ;
#45663=VERTEX_POINT ( 'NONE', #56100 ) ;
#45664=FACE_OUTER_BOUND ( 'NONE', #81430, .T. ) ;
#45665=CARTESIAN_POINT ( 'NONE',  ( -0.3345883534476049581, 1474.778737585120098, 235.9370569828869861 ) ) ;
#45666=CARTESIAN_POINT ( 'NONE',  ( 10.22570915140000025, 1431.113060387329824, 225.5143498067979806 ) ) ;
#45669=CARTESIAN_POINT ( 'NONE',  ( -2.055127378149999906, 1486.233656124230038, 181.7623468732980143 ) ) ;
#45672=CARTESIAN_POINT ( 'NONE',  ( 13.15570206748037307, 1428.769203746674748, 222.7935865483545967 ) ) ;
#45673=CARTESIAN_POINT ( 'NONE',  ( -37.06048519556479448, 1450.125392790749856, 136.1884239245549963 ) ) ;
#45675=CARTESIAN_POINT ( 'NONE',  ( -2.500000000000000000, 1448.295519077039899, 164.4141711672770043 ) ) ;
#45676=CARTESIAN_POINT ( 'NONE',  ( 9.070382607970518762, 1396.229805130280056, 215.4513483083970016 ) ) ;
#45677=CARTESIAN_POINT ( 'NONE',  ( -39.88064382167599575, 1440.876666208930146, 136.8074513327459840 ) ) ;
#45678=CARTESIAN_POINT ( 'NONE',  ( -1.520289120366909996, 1406.276897935829993, 269.2942228619830303 ) ) ;
#45679=ORIENTED_EDGE ( 'NONE', *, *, #87713, .T. ) ;
#45681=CARTESIAN_POINT ( 'NONE',  ( 13.02183306049999878, 1441.592108930330141, 188.8634220520980023 ) ) ;
#45682=EDGE_LOOP ( 'NONE', ( #76489, #20105, #83806, #110567, #43666, #38064, #104363, #91079 ) ) ;
#45683=ORIENTED_EDGE ( 'NONE', *, *, #79276, .T. ) ;
#45688=ORIENTED_EDGE ( 'NONE', *, *, #64741, .F. ) ;
#45695=B_SPLINE_SURFACE_WITH_KNOTS ( 'NONE', 5, 3, ( 
 ( #62915, #53946, #11369, #45540 ),
 ( #79680, #88629, #37657, #97026 ),
 ( #11908, #46083, #29801, #63989 ),
 ( #89704, #12985, #80215, #55033 ),
 ( #71862, #105980, #89160, #57236 ),
 ( #84052, #99743, #15717, #40398 ) ),
 .UNSPECIFIED., .F., .F., .F.,
 ( 6, 6 ),
 ( 4, 4 ),
 ( 0.000000000000000000, 52.98902693510000006 ),
 ( 37.69911184309999896, 40.20365518519999881 ),
 .UNSPECIFIED. ) ;
#45696=CARTESIAN_POINT ( 'NONE',  ( -41.28233839276082762, 1435.098719027513653, 269.6338957342284175 ) ) ;
#45698=CARTESIAN_POINT ( 'NONE',  ( -6.498943257060000533, 1410.073555944530199, 231.2704400879979971 ) ) ;
#45702=DIRECTION ( 'NONE',  ( 0.000000000000000000, 0.000000000000000000, -1.000000000000000000 ) ) ;
#45704=CARTESIAN_POINT ( 'NONE',  ( 15.73091604048637926, 1506.446781332931778, 224.4927539354196711 ) ) ;
#45705=CARTESIAN_POINT ( 'NONE',  ( 39.33429647749250080, 1428.581013311290235, 269.8320583910219739 ) ) ;
#45708=CARTESIAN_POINT ( 'NONE',  ( 0.02009193267265866820, 1507.207280861917752, 237.3586468649436938 ) ) ;
#45711=CARTESIAN_POINT ( 'NONE',  ( 17.38482601099109814, 1410.884446382940041, 192.4603632472940262 ) ) ;
#45713=ORIENTED_EDGE ( 'NONE', *, *, #102904, .F. ) ;
#45715=CARTESIAN_POINT ( 'NONE',  ( -1.684665908019999936, 1420.451874816630152, 233.3235451955980011 ) ) ;
#45717=ORIENTED_EDGE ( 'NONE', *, *, #101584, .F. ) ;
#45720=CARTESIAN_POINT ( 'NONE',  ( 18.79378390429650025, 1478.713334920350007, 228.4735663057359716 ) ) ;
#45722=CARTESIAN_POINT ( 'NONE',  ( -24.23891439175908147, 1437.877539721478342, 210.9599772510106277 ) ) ;
#45723=CARTESIAN_POINT ( 'NONE',  ( 11.79002570591860000, 1447.121451514569799, 187.8029540059399949 ) ) ;
#45724=CARTESIAN_POINT ( 'NONE',  ( -0.09448057143150000170, 1408.916359721629988, 231.7835052710979937 ) ) ;
#45725=CARTESIAN_POINT ( 'NONE',  ( 0.02235964058503960017, 1420.444490115599820, 182.6732928536509917 ) ) ;
#45726=B_SPLINE_CURVE_WITH_KNOTS ( 'NONE', 5,
 ( #7128, #25003, #48598, #66515, #75458, #92229, #75983, #40177, #31769 ),
 .UNSPECIFIED., .F., .F.,
 ( 6, 3, 6 ),
 ( 0.000000000000000000, 0.5050532947756587454, 1.000000000000000000 ),
 .UNSPECIFIED. ) ;
#45728=CARTESIAN_POINT ( 'NONE',  ( 23.28627655106232197, 1507.873435797507682, 223.2320360419293479 ) ) ;
#45729=CARTESIAN_POINT ( 'NONE',  ( 19.48412260369999771, 1509.357564207130281, 187.7562371571980009 ) ) ;
#45731=ORIENTED_EDGE ( 'NONE', *, *, #6974, .F. ) ;
#45732=CARTESIAN_POINT ( 'NONE',  ( -12.92134813639500024, 1416.521607925280023, 196.5106865475920301 ) ) ;
#45733=CARTESIAN_POINT ( 'NONE',  ( -0.7461436398870000541, 1508.913060260629891, 180.6894241092979883 ) ) ;
#45734=ORIENTED_EDGE ( 'NONE', *, *, #10291, .F. ) ;
#45739=CARTESIAN_POINT ( 'NONE',  ( 15.82264516024399903, 1421.172194390546792, 227.5204971587648970 ) ) ;
#45740=CARTESIAN_POINT ( 'NONE',  ( 21.71798588809999941, 1410.865989080929921, 202.0964915433179954 ) ) ;
#45741=LINE ( 'NONE', #86059, #48568 ) ;
#45742=CARTESIAN_POINT ( 'NONE',  ( -18.86348425649999783, 1425.765603139730047, 225.9037505451979939 ) ) ;
#45743=CARTESIAN_POINT ( 'NONE',  ( -16.03439795359999920, 1435.876017354450141, 148.8030225068980030 ) ) ;
#45745=CARTESIAN_POINT ( 'NONE',  ( 16.20713703829999730, 1428.791430359930018, 190.9630754147979701 ) ) ;
#45746=B_SPLINE_CURVE_WITH_KNOTS ( 'NONE', 5,
 ( #101248, #85019, #60403, #68813, #51434, #43045, #102376, #85564, #32961, #92316, #7767, #15587, #102914, #8313, #67702 ),
 .UNSPECIFIED., .F., .F.,
 ( 6, 3, 3, 3, 6 ),
 ( 0.000000000000000000, 0.2965494146486967186, 0.6162090003293669849, 0.8933765034092037149, 1.000000000000000000 ),
 .UNSPECIFIED. ) ;
#45747=CARTESIAN_POINT ( 'NONE',  ( 0.5818187789159990908, 1408.933377948760153, 232.0310414966060080 ) ) ;
#45752=CARTESIAN_POINT ( 'NONE',  ( -10.78302954206379560, 1424.941192272636954, 142.1511525142338712 ) ) ;
#45753=CARTESIAN_POINT ( 'NONE',  ( -24.01458399190000392, 1437.348856588880153, 212.3223689552080202 ) ) ;
#45755=CARTESIAN_POINT ( 'NONE',  ( -18.52542037779999973, 1508.846193921429858, 229.9902974711980050 ) ) ;
#45757=CARTESIAN_POINT ( 'NONE',  ( 12.10369631294569004, 1435.500269353037993, 151.1372464589562412 ) ) ;
#45758=FACE_OUTER_BOUND ( 'NONE', #84597, .T. ) ;
#45763=ADVANCED_FACE ( 'NONE', ( #12971 ), #16097, .F. ) ;
#45764=AXIS2_PLACEMENT_3D ( 'NONE', #36139, #104436, #53507 ) ;
#45766=CARTESIAN_POINT ( 'NONE',  ( -15.58634593545749780, 1506.535970897286916, 224.7451074557852735 ) ) ;
#45771=CARTESIAN_POINT ( 'NONE',  ( 19.89197732033110100, 1508.728142334059839, 229.5184948967959997 ) ) ;
#45774=VERTEX_POINT ( 'NONE', #28424 ) ;
#45777=CARTESIAN_POINT ( 'NONE',  ( 13.10420440301432876, 1443.028011217175617, 169.4053780122457340 ) ) ;
#45778=CARTESIAN_POINT ( 'NONE',  ( 18.42977693619575064, 1413.445009768722457, 269.3801010515786629 ) ) ;
#45779=CARTESIAN_POINT ( 'NONE',  ( -41.56052291839999668, 1443.484420489879994, 261.5689799724980276 ) ) ;
#45781=CARTESIAN_POINT ( 'NONE',  ( -11.57384147910000038, 1433.753257872449922, 151.2114678470979925 ) ) ;
#45782=CARTESIAN_POINT ( 'NONE',  ( 28.77729888390000212, 1509.917985808229787, 206.0039979917680171 ) ) ;
#45783=CARTESIAN_POINT ( 'NONE',  ( 11.65156729925299928, 1426.753153792180001, 138.0613224902349714 ) ) ;
#45784=CARTESIAN_POINT ( 'NONE',  ( 6.512000794579999585, 1410.074001341329904, 186.9789373606980121 ) ) ;
#45789=CARTESIAN_POINT ( 'NONE',  ( -9.129512800839998832, 1452.594250776829995, 151.6824240526980248 ) ) ;
#45791=ORIENTED_EDGE ( 'NONE', *, *, #43929, .T. ) ;
#45794=VECTOR ( 'NONE', #34994, 1000.000000000000000 ) ;
#45796=CARTESIAN_POINT ( 'NONE',  ( -10.92641736379999884, 1472.943607924629760, 270.2707055147980100 ) ) ;
#45798=CARTESIAN_POINT ( 'NONE',  ( 9.470907091730000005, 1435.946707556030105, 153.1784963645979758 ) ) ;
#45801=CARTESIAN_POINT ( 'NONE',  ( -13.95241924839999825, 1421.181435538830101, 227.8193205229979981 ) ) ;
#45802=AXIS2_PLACEMENT_3D ( 'NONE', #75036, #8347, #25694 ) ;
#45805=CARTESIAN_POINT ( 'NONE',  ( -43.84971736824440569, 1430.786840038769924, 268.8176679617099580 ) ) ;
#45807=CARTESIAN_POINT ( 'NONE',  ( 25.70088977221606541, 1435.395012714986251, 135.4164360916261955 ) ) ;
#45808=ORIENTED_EDGE ( 'NONE', *, *, #98959, .F. ) ;
#45812=CARTESIAN_POINT ( 'NONE',  ( -15.47784148859999931, 1410.406428057529865, 191.0438890190980032 ) ) ;
#45814=VERTEX_POINT ( 'NONE', #80487 ) ;
#45820=ORIENTED_EDGE ( 'NONE', *, *, #102366, .T. ) ;
#45821=CARTESIAN_POINT ( 'NONE',  ( -18.49698681803500122, 1413.444200939100028, 269.3800619411300090 ) ) ;
#45823=CARTESIAN_POINT ( 'NONE',  ( 3.677837710089999800E-15, 1426.566393376330097, 144.1938086916980239 ) ) ;
#45827=ORIENTED_EDGE ( 'NONE', *, *, #73887, .T. ) ;
#45828=CARTESIAN_POINT ( 'NONE',  ( 44.73266700618014369, 1447.687831433334622, 269.0000809591583106 ) ) ;
#45831=CARTESIAN_POINT ( 'NONE',  ( -0.02513066005776489961, 1409.073703610690018, 185.8050026937470136 ) ) ;
#45832=CARTESIAN_POINT ( 'NONE',  ( -18.43873448085470201, 1415.658863689850023, 207.5693132298119679 ) ) ;
#45834=CARTESIAN_POINT ( 'NONE',  ( -13.90031192530000048, 1420.171540284829916, 222.0121128021980041 ) ) ;
#45835=CARTESIAN_POINT ( 'NONE',  ( 12.60360202350000058, 1416.535385209630022, 223.3155814965980142 ) ) ;
#45836=B_SPLINE_CURVE_WITH_KNOTS ( 'NONE', 5,
 ( #50956, #92939, #86196, #103545, #25166, #110293 ),
 .UNSPECIFIED., .F., .F.,
 ( 6, 6 ),
 ( -20.28790020619999979, -6.591324572240001345 ),
 .UNSPECIFIED. ) ;
#45837=CARTESIAN_POINT ( 'NONE',  ( 8.987603741960001003, 1445.737909925099984, 185.1272997528979829 ) ) ;
#45841=CARTESIAN_POINT ( 'NONE',  ( 1.493635725151659877, 1469.335982536970050, 182.7613696330639925 ) ) ;
#45842=ORIENTED_EDGE ( 'NONE', *, *, #92607, .T. ) ;
#45843=CARTESIAN_POINT ( 'NONE',  ( 3.238472285647973514, 1457.571195284309624, 228.6299524684958442 ) ) ;
#45844=CARTESIAN_POINT ( 'NONE',  ( 24.50642912900270076, 1451.900605154380173, 137.2752955659460099 ) ) ;
#45845=CARTESIAN_POINT ( 'NONE',  ( 16.18746221460043344, 1409.478339023977696, 224.9965714503316576 ) ) ;
#45848=CARTESIAN_POINT ( 'NONE',  ( 21.99779377019999771, 1409.845345889329792, 206.2854409714980193 ) ) ;
#45849=B_SPLINE_CURVE_WITH_KNOTS ( 'NONE', 3,
 ( #105397, #104290, #28690, #81273, #46060, #72360, #29777, #89683, #96445, #53925, #11345, #89139, #97004, #2963, #95888, #63425, #19148, #97543, #55012, #79108, #88060, #20267, #21351, #70729 ),
 .UNSPECIFIED., .F., .F.,
 ( 4, 2, 2, 2, 2, 2, 2, 2, 2, 2, 2, 4 ),
 ( -1.636478521365379857, -1.584985545560960052, -1.533441748506799929, -1.430342195185549947, -1.224163068651749953, -0.8182278975005480293, -0.4129906964137790570, -0.2064832563783289832, -0.1032404805529840708, -0.05160657342599406228, -0.02578454166961874350, 0.000000000000000000 ),
 .UNSPECIFIED. ) ;
#45851=CARTESIAN_POINT ( 'NONE',  ( 17.60614391659999711, 1410.891372730630110, 225.2143943941980240 ) ) ;
#45853=CARTESIAN_POINT ( 'NONE',  ( 0.8425900835067681172, 1451.065773967280165, 182.3319842116689813 ) ) ;
#45854=CARTESIAN_POINT ( 'NONE',  ( 2.500000000000000000, 1439.522697744529978, 164.2180412838509938 ) ) ;
#45856=CARTESIAN_POINT ( 'NONE',  ( 25.86984728598680050, 1447.207353507300013, 138.1976246213770310 ) ) ;
#45857=VERTEX_POINT ( 'NONE', #39006 ) ;
#45859=DIRECTION ( 'NONE',  ( -0.03489949676615768798, 0.9993908270168727626, 1.192931611642853769E-09 ) ) ;
#45860=CARTESIAN_POINT ( 'NONE',  ( -0.3785191915233269699, 1409.088790390760096, 232.4100744083189909 ) ) ;
#45863=CARTESIAN_POINT ( 'NONE',  ( -35.95901143404110201, 1450.034299295669825, 136.2432003471689939 ) ) ;
#45864=CARTESIAN_POINT ( 'NONE',  ( 0.04210049761976375482, 1506.527232284500997, 231.1830146150431062 ) ) ;
#45865=CARTESIAN_POINT ( 'NONE',  ( 1.509903313490000218E-14, 1461.407663418029870, 243.9198229339980060 ) ) ;
#45866=CARTESIAN_POINT ( 'NONE',  ( 29.93311702910001415, 1467.353193293025925, 266.6089909078979190 ) ) ;
#45867=CARTESIAN_POINT ( 'NONE',  ( 11.42063316640000004, 1433.075813662200062, 151.3550505031980151 ) ) ;
#45869=CARTESIAN_POINT ( 'NONE',  ( -17.57263815903020188, 1409.691670451539949, 195.6049335520870045 ) ) ;
#45870=CARTESIAN_POINT ( 'NONE',  ( -22.21499610869999941, 1508.010819105329801, 225.8229464100980124 ) ) ;
#45875=CARTESIAN_POINT ( 'NONE',  ( -19.19677231483893109, 1485.580715045685565, 189.7096105684387339 ) ) ;
#45877=CARTESIAN_POINT ( 'NONE',  ( 2.899728573290000444, 1474.727573286329971, 234.5030603628979975 ) ) ;
#45878=CARTESIAN_POINT ( 'NONE',  ( 24.38832783640000201, 1430.357083400130023, 211.7627176485680138 ) ) ;
#45880=CARTESIAN_POINT ( 'NONE',  ( -12.71706127659999908, 1509.357149952429836, 235.0231910820979806 ) ) ;
#45883=CARTESIAN_POINT ( 'NONE',  ( 10.90933839120000037, 1409.294022878630130, 220.2163247819979972 ) ) ;
#45885=DIRECTION ( 'NONE',  ( -0.8771707857591169999, 0.03063147879954419839, 0.4792005061738630056 ) ) ;
#45886=CARTESIAN_POINT ( 'NONE',  ( -10.73220944925208187, 1434.662271276825777, 151.9792366751727002 ) ) ;
#45888=CARTESIAN_POINT ( 'NONE',  ( -1.210172143909999942, 1452.161324106529946, 183.6548506043980069 ) ) ;
#45890=CARTESIAN_POINT ( 'NONE',  ( -3.018074008395929653, 1440.716223013230092, 157.2134785397810219 ) ) ;
#45895=ORIENTED_EDGE ( 'NONE', *, *, #101536, .T. ) ;
#45898=CARTESIAN_POINT ( 'NONE',  ( -2.975637186240103205, 1509.038728186502112, 238.5532284157007155 ) ) ;
#45899=CARTESIAN_POINT ( 'NONE',  ( 23.06762021731623591, 1409.889826804416771, 208.2909805245021175 ) ) ;
#45902=CARTESIAN_POINT ( 'NONE',  ( 14.65346504764830193, 1409.424770662520132, 206.2342854941859969 ) ) ;
#45903=CARTESIAN_POINT ( 'NONE',  ( 18.12392718799999969, 1425.124928798529936, 224.9480847838979969 ) ) ;
#45905=DIRECTION ( 'NONE',  ( -0.009162664301380763279, -0.1630249973094845817, -0.9865793915520144619 ) ) ;
#45906=CARTESIAN_POINT ( 'NONE',  ( -10.78871504700000017, 1416.913060387330006, 209.1218460627730167 ) ) ;
#45910=CARTESIAN_POINT ( 'NONE',  ( -11.61894909938840037, 1415.258594621340080, 195.3027647187179809 ) ) ;
#45912=CARTESIAN_POINT ( 'NONE',  ( 19.01867779685918336, 1468.113705757313028, 269.3842191184903072 ) ) ;
#45914=CARTESIAN_POINT ( 'NONE',  ( -28.13497786889999830, 1508.084884472430076, 209.9324264222260013 ) ) ;
#45915=CARTESIAN_POINT ( 'NONE',  ( 1.275935406860000176, 1416.411557770830086, 232.9857732278980222 ) ) ;
#45916=CARTESIAN_POINT ( 'NONE',  ( -1.440135191710000040, 1453.598500553229997, 183.7985014944979980 ) ) ;
#45918=CARTESIAN_POINT ( 'NONE',  ( 9.577041028380113730, 1507.356930867539177, 234.6859123068956876 ) ) ;
#45920=B_SPLINE_CURVE_WITH_KNOTS ( 'NONE', 3,
 ( #69434, #77809, #84543, #68883, #102984, #26283, #60472, #86200, #9491, #1119 ),
 .UNSPECIFIED., .F., .F.,
 ( 4, 2, 2, 2, 4 ),
 ( 0.000000000000000000, 0.2500000000000000000, 0.5000000000000000000, 0.7500000000000000000, 1.000000000000000000 ),
 .UNSPECIFIED. ) ;
#45922=DIRECTION ( 'NONE',  ( 0.000000000000000000, 0.000000000000000000, -1.000000000000000000 ) ) ;
#45926=CARTESIAN_POINT ( 'NONE',  ( 2.798741260039999901, 1509.010794585729855, 238.1786444273980123 ) ) ;
#45929=CARTESIAN_POINT ( 'NONE',  ( 28.68962088199999982, 1414.662824323530231, 264.4914085171980105 ) ) ;
#45930=CARTESIAN_POINT ( 'NONE',  ( -26.16501621719999804, 1469.244469854430008, 206.7451401483880034 ) ) ;
#45931=CARTESIAN_POINT ( 'NONE',  ( -3.544220692770000181, 1502.026769662330025, 181.1943011134980281 ) ) ;
#45932=CARTESIAN_POINT ( 'NONE',  ( -33.91369120210140409, 1435.681798817159915, 134.0999999980979851 ) ) ;
#45933=CARTESIAN_POINT ( 'NONE',  ( 1.625726771580663810, 1508.862184707432107, 180.0252976343047919 ) ) ;
#45934=CARTESIAN_POINT ( 'NONE',  ( -14.70061896160000003, 1417.388462482530031, 244.5173668987980307 ) ) ;
#45936=CARTESIAN_POINT ( 'NONE',  ( 1.363639811660000145, 1415.765555525229956, 232.8698637559979829 ) ) ;
#45937=CARTESIAN_POINT ( 'NONE',  ( -23.56625796634288861, 1410.013281407407703, 208.7413938499740027 ) ) ;
#45938=EDGE_LOOP ( 'NONE', ( #59200, #18074, #96046, #97514 ) ) ;
#45939=CARTESIAN_POINT ( 'NONE',  ( -0.01233358747499999943, 1396.097901035330096, 197.1956428485979700 ) ) ;
#45941=CARTESIAN_POINT ( 'NONE',  ( 11.79165948289999832, 1509.456730002229961, 236.8935920530979899 ) ) ;
#45943=ORIENTED_EDGE ( 'NONE', *, *, #49612, .T. ) ;
#45949=CARTESIAN_POINT ( 'NONE',  ( 0.1923534468539999931, 1452.340213589330006, 183.2784190956980126 ) ) ;
#45950=CARTESIAN_POINT ( 'NONE',  ( -2.509810337609999831, 1489.062117308030111, 236.1277042400979838 ) ) ;
#45955=EDGE_CURVE ( 'NONE', #93518, #69912, #38916, .T. ) ;
#45956=CARTESIAN_POINT ( 'NONE',  ( -13.15726444150010011, 1415.434635989089884, 221.3440418462499792 ) ) ;
#45960=VERTEX_POINT ( 'NONE', #54206 ) ;
#45961=CARTESIAN_POINT ( 'NONE',  ( 11.85443421315619972, 1431.523992928169946, 149.9226482103390197 ) ) ;
#45962=EDGE_CURVE ( 'NONE', #19757, #98647, #62025, .T. ) ;
#45964=ORIENTED_EDGE ( 'NONE', *, *, #103472, .T. ) ;
#45967=EDGE_CURVE ( 'NONE', #84504, #102807, #14904, .T. ) ;
#45974=CARTESIAN_POINT ( 'NONE',  ( 0.4896011454402059981, 1407.928426433459890, 270.2927087822229737 ) ) ;
#45982=CARTESIAN_POINT ( 'NONE',  ( 16.15031516230000008, 1471.311257370829935, 195.1295159150980112 ) ) ;
#45984=CARTESIAN_POINT ( 'NONE',  ( 17.90387844572719800, 1420.535267245019895, 225.0886834623109962 ) ) ;
#45986=VERTEX_POINT ( 'NONE', #18757 ) ;
#45987=CARTESIAN_POINT ( 'NONE',  ( 23.03655028440000052, 1423.631548418229841, 255.3819207742980097 ) ) ;
#45996=ORIENTED_EDGE ( 'NONE', *, *, #33188, .T. ) ;
#45998=CARTESIAN_POINT ( 'NONE',  ( -24.02756305619999821, 1444.331317782170117, 212.2090029378380223 ) ) ;
#45999=DIRECTION ( 'NONE',  ( 0.000000000000000000, 0.000000000000000000, -1.000000000000000000 ) ) ;
#46002=CARTESIAN_POINT ( 'NONE',  ( -12.01638188689999964, 1440.881463209799904, 187.8051711800980001 ) ) ;
#46004=CARTESIAN_POINT ( 'NONE',  ( 12.99126122772529968, 1509.366722754649800, 181.4462959118600054 ) ) ;
#46005=CARTESIAN_POINT ( 'NONE',  ( 2.922712066004659714, 1412.240002439039927, 231.7135113672919999 ) ) ;
#46008=CARTESIAN_POINT ( 'NONE',  ( 15.07806947409999943, 1412.745289768429984, 227.5463952181980005 ) ) ;
#46010=CARTESIAN_POINT ( 'NONE',  ( -16.13112951687100249, 1459.078801168009932, 230.3616389713189960 ) ) ;
#46012=CARTESIAN_POINT ( 'NONE',  ( 44.11426962409999675, 1429.859647049230034, 268.2740853901979676 ) ) ;
#46013=CARTESIAN_POINT ( 'NONE',  ( -18.82531593190000052, 1410.932625384329867, 223.3083523618979882 ) ) ;
#46015=CARTESIAN_POINT ( 'NONE',  ( 18.77495633519999885, 1435.298717977980004, 145.7151766910979802 ) ) ;
#46016=EDGE_CURVE ( 'NONE', #103324, #11383, #3118, .T. ) ;
#46017=CARTESIAN_POINT ( 'NONE',  ( 19.55758403639999798, 1488.589959684130008, 189.8994889324980022 ) ) ;
#46018=B_SPLINE_CURVE_WITH_KNOTS ( 'NONE', 3,
 ( #31814, #23406, #57044, #63788, #49190, #21730 ),
 .UNSPECIFIED., .F., .F.,
 ( 4, 2, 4 ),
 ( 1.000070671099200032E-06, 0.09529849184413820284, 0.1904887692805259936 ),
 .UNSPECIFIED. ) ;
#46019=CARTESIAN_POINT ( 'NONE',  ( 29.78200767887302547, 1510.000544160475329, 209.1355521330470140 ) ) ;
#46021=CARTESIAN_POINT ( 'NONE',  ( -15.90377527599999929, 1418.369030882129891, 226.9588463030979710 ) ) ;
#46024=CARTESIAN_POINT ( 'NONE',  ( -12.07987659813839976, 1408.300217416430087, 215.9313631298179814 ) ) ;
#46026=CARTESIAN_POINT ( 'NONE',  ( -16.37832153215809328, 1409.485005020973631, 193.4350318287646644 ) ) ;
#46028=CARTESIAN_POINT ( 'NONE',  ( 12.06142474169999979, 1433.903238137760127, 146.5968191413979866 ) ) ;
#46029=CARTESIAN_POINT ( 'NONE',  ( -30.78500370360000105, 1435.572563320330119, 135.1635738117979884 ) ) ;
#46031=ORIENTED_EDGE ( 'NONE', *, *, #29537, .F. ) ;
#46036=CARTESIAN_POINT ( 'NONE',  ( -17.11714618744633754, 1443.086052842848630, 162.7561046190426737 ) ) ;
#46038=CARTESIAN_POINT ( 'NONE',  ( -44.82664241559999851, 1451.165400018629953, 266.7159563179980069 ) ) ;
#46041=CARTESIAN_POINT ( 'NONE',  ( -24.90809350219999985, 1507.935970483929850, 220.3557327460979991 ) ) ;
#46045=CARTESIAN_POINT ( 'NONE',  ( 21.32980800760000051, 1509.431603210329968, 227.7697269125980029 ) ) ;
#46046=CARTESIAN_POINT ( 'NONE',  ( 15.05032900819999853, 1485.054733288129910, 223.8431641993980179 ) ) ;
#46048=CARTESIAN_POINT ( 'NONE',  ( 2.500000000000000000, 1419.524771318244348, 137.0999999980979851 ) ) ;
#46050=EDGE_LOOP ( 'NONE', ( #103566, #83937, #61525 ) ) ;
#46052=CARTESIAN_POINT ( 'NONE',  ( -8.888245507000000669E-15, 1414.050155615230096, 164.5351017311979831 ) ) ;
#46053=EDGE_CURVE ( 'NONE', #27764, #103213, #88327, .T. ) ;
#46055=CARTESIAN_POINT ( 'NONE',  ( -12.78667948450000047, 1416.822690122329959, 195.3262913363980147 ) ) ;
#46057=CARTESIAN_POINT ( 'NONE',  ( 23.47111472610000149, 1410.227925161630083, 211.2550682413580034 ) ) ;
#46060=CARTESIAN_POINT ( 'NONE',  ( -5.383045099570169967, 1431.499107093909970, 154.5620711115419965 ) ) ;
#46067=CIRCLE ( 'NONE', #103241, 26.99999999999999645 ) ;
#46068=CARTESIAN_POINT ( 'NONE',  ( -1.110282348042360034, 1420.248281415159909, 184.7133612920480061 ) ) ;
#46071=CARTESIAN_POINT ( 'NONE',  ( 13.38054884590909843, 1507.805480882780103, 233.0860310194200054 ) ) ;
#46072=CARTESIAN_POINT ( 'NONE',  ( -17.39085484616060029, 1485.731293066659873, 188.3208887600499963 ) ) ;
#46079=CARTESIAN_POINT ( 'NONE',  ( 29.14447581790000186, 1509.936536293530253, 213.8494348557679814 ) ) ;
#46080=ORIENTED_EDGE ( 'NONE', *, *, #74972, .T. ) ;
#46082=CARTESIAN_POINT ( 'NONE',  ( 1.383993012819999979, 1414.983771848829747, 191.7538275864980051 ) ) ;
#46083=CARTESIAN_POINT ( 'NONE',  ( 0.7772817352909999755, 1427.305457135430061, 123.0297916884979941 ) ) ;
#46084=CARTESIAN_POINT ( 'NONE',  ( 15.73440523137610292, 1409.488452722919874, 192.6548270638369900 ) ) ;
#46085=CARTESIAN_POINT ( 'NONE',  ( 11.97827956719999776, 1441.604408666619975, 150.7817505876979851 ) ) ;
#46087=CARTESIAN_POINT ( 'NONE',  ( -25.75378511762339784, 1451.133596423730069, 136.7593279701780205 ) ) ;
#46089=CARTESIAN_POINT ( 'NONE',  ( 13.87080890250000031, 1409.899448471030155, 227.8810934041980261 ) ) ;
#46091=( NAMED_UNIT ( * ) SI_UNIT ( $, .STERADIAN. ) SOLID_ANGLE_UNIT ( ) );
#46093=CARTESIAN_POINT ( 'NONE',  ( 40.98974505593590578, 1446.927689382389872, 134.0999999985409943 ) ) ;
#46105=CARTESIAN_POINT ( 'NONE',  ( 15.60193763504558007, 1451.131520225134182, 149.3236191048951582 ) ) ;
#46111=CARTESIAN_POINT ( 'NONE',  ( 4.226171528248299225, 1446.259724416819836, 166.0438435565190218 ) ) ;
#46113=CARTESIAN_POINT ( 'NONE',  ( -0.04583980512609999586, 1508.666040292029948, 238.1629808674979927 ) ) ;
#46114=ORIENTED_EDGE ( 'NONE', *, *, #85304, .T. ) ;
#46116=ORIENTED_EDGE ( 'NONE', *, *, #58207, .F. ) ;
#46117=CARTESIAN_POINT ( 'NONE',  ( 30.00383565071140168, 1440.913060387330006, 252.1044819011040090 ) ) ;
#46118=B_SPLINE_CURVE_WITH_KNOTS ( 'NONE', 5,
 ( #88377, #98964, #48030, #97860, #11667, #55897, #30104, #73796, #5467 ),
 .UNSPECIFIED., .F., .F.,
 ( 6, 3, 6 ),
 ( 0.000000000000000000, 0.5000000000000000000, 1.000000000000000000 ),
 .UNSPECIFIED. ) ;
#46123=CARTESIAN_POINT ( 'NONE',  ( -14.49476690930000089, 1409.419228801430108, 191.6021942292979929 ) ) ;
#46129=CARTESIAN_POINT ( 'NONE',  ( -11.87742750661531410, 1433.145441672523930, 147.6581217067710554 ) ) ;
#46130=CARTESIAN_POINT ( 'NONE',  ( -11.94102939159999899, 1433.615517387009959, 149.9804957299980117 ) ) ;
#46132=ADVANCED_FACE ( 'NONE', ( #56803 ), #93004, .T. ) ;
#46133=DIRECTION ( 'NONE',  ( 0.01398399556878729237, -0.01017778278299899530, 0.9998504191155564991 ) ) ;
#46135=VECTOR ( 'NONE', #24, 1000.000000000000000 ) ;
#46136=B_SPLINE_CURVE_WITH_KNOTS ( 'NONE', 5,
 ( #11236, #25791, #52135, #9553, #35315, #30948, #7401, #82465, #100358 ),
 .UNSPECIFIED., .F., .F.,
 ( 6, 3, 6 ),
 ( 0.000000000000000000, 0.5198849050576186404, 1.000000000000000000 ),
 .UNSPECIFIED. ) ;
#46138=EDGE_CURVE ( 'NONE', #71548, #46325, #35338, .T. ) ;
#46144=CARTESIAN_POINT ( 'NONE',  ( -19.92213876099999936, 1452.807100929029957, 208.8541967413179918 ) ) ;
#46149=CARTESIAN_POINT ( 'NONE',  ( 30.53571888369999954, 1442.873932100699903, 240.1260121790979838 ) ) ;
#46152=CARTESIAN_POINT ( 'NONE',  ( -0.2745515581962330032, 1507.636705584799984, 237.3923196597329763 ) ) ;
#46153=CARTESIAN_POINT ( 'NONE',  ( -21.94178583340000088, 1452.077510002930239, 222.2803297732980070 ) ) ;
#46154=CARTESIAN_POINT ( 'NONE',  ( -23.00040066099999692, 1457.437332268930049, 219.0071613830780279 ) ) ;
#46155=CARTESIAN_POINT ( 'NONE',  ( 5.360347202541429823, 1422.243392962449889, 144.1217039821420087 ) ) ;
#46156=CARTESIAN_POINT ( 'NONE',  ( 0.04749300429670000323, 1488.809466528630082, 187.8102763656980017 ) ) ;
#46160=CARTESIAN_POINT ( 'NONE',  ( 1.779019444429999819, 1405.741471815129898, 267.8527215162980042 ) ) ;
#46163=CIRCLE ( 'NONE', #83594, 4.941741911590025182 ) ;
#46164=AXIS2_PLACEMENT_3D ( 'NONE', #64811, #28982, #22190 ) ;
#46165=CARTESIAN_POINT ( 'NONE',  ( 12.89647794391319913, 1471.158836576110161, 270.0761327948309827 ) ) ;
#46166=CARTESIAN_POINT ( 'NONE',  ( -15.36549427709999982, 1420.352425059129928, 229.0210324418980008 ) ) ;
#46169=CARTESIAN_POINT ( 'NONE',  ( -44.56994949339100742, 1440.913060401099983, 264.9967186962099959 ) ) ;
#46170=CARTESIAN_POINT ( 'NONE',  ( 1.590343439599928743, 1450.573397075630282, 154.2772178510776655 ) ) ;
#46172=CARTESIAN_POINT ( 'NONE',  ( 0.5703798115540580360, 1450.893142285409795, 154.7888392056570126 ) ) ;
#46174=CARTESIAN_POINT ( 'NONE',  ( 19.30499357109350811, 1478.515812373770359, 190.2772978286499495 ) ) ;
#46175=ORIENTED_EDGE ( 'NONE', *, *, #40661, .F. ) ;
#46176=CARTESIAN_POINT ( 'NONE',  ( -13.21926163189999848, 1421.359897795430015, 248.0989693021979861 ) ) ;
#46178=CARTESIAN_POINT ( 'NONE',  ( -0.3342637058910000181, 1475.047619362329897, 269.6500372387980065 ) ) ;
#46179=CARTESIAN_POINT ( 'NONE',  ( -16.68599179859999992, 1461.161699058329987, 228.2799821568980008 ) ) ;
#46180=AXIS2_PLACEMENT_3D ( 'NONE', #10759, #62857, #26999 ) ;
#46181=CARTESIAN_POINT ( 'NONE',  ( -28.91076495679999780, 1509.890507479829921, 211.0912775665780146 ) ) ;
#46182=CARTESIAN_POINT ( 'NONE',  ( -3.650443696216681744, 1448.291914533057479, 184.9508012256059999 ) ) ;
#46184=CARTESIAN_POINT ( 'NONE',  ( -17.62728127150000290, 1415.048591094029916, 207.6446436201280221 ) ) ;
#46185=CARTESIAN_POINT ( 'NONE',  ( 11.87450673426269887, 1432.968194686480047, 149.9806125890570172 ) ) ;
#46186=CARTESIAN_POINT ( 'NONE',  ( 26.79956694294169850, 1435.440314151020175, 135.4706125346669978 ) ) ;
#46187=CARTESIAN_POINT ( 'NONE',  ( -9.209528894577250213, 1396.234664223010213, 215.2427597039980185 ) ) ;
#46188=CARTESIAN_POINT ( 'NONE',  ( -15.49830443269999947, 1421.268164864530036, 227.1260603972979766 ) ) ;
#46189=CARTESIAN_POINT ( 'NONE',  ( 19.54803553591734300, 1455.513809965727887, 225.8158593003944645 ) ) ;
#46190=ORIENTED_EDGE ( 'NONE', *, *, #65200, .T. ) ;
#46191=CARTESIAN_POINT ( 'NONE',  ( -21.92423686380000092, 1509.678671609130106, 190.3411753256980035 ) ) ;
#46192=CARTESIAN_POINT ( 'NONE',  ( 1.674597368589999968, 1409.138563866230015, 231.5566276255979687 ) ) ;
#46194=CARTESIAN_POINT ( 'NONE',  ( 11.56890495900000104, 1426.389997043230096, 132.2071877881980129 ) ) ;
#46196=CARTESIAN_POINT ( 'NONE',  ( 11.65615920360559343, 1428.981702016564896, 138.1374390033663815 ) ) ;
#46197=CARTESIAN_POINT ( 'NONE',  ( -11.23388613411650638, 1442.762691980111640, 151.7784653951601399 ) ) ;
#46202=CARTESIAN_POINT ( 'NONE',  ( 4.112297488690000336, 1508.008646858429984, 181.4894093006979858 ) ) ;
#46208=EDGE_LOOP ( 'NONE', ( #97596, #78436, #12172, #27423 ) ) ;
#46210=B_SPLINE_CURVE_WITH_KNOTS ( 'NONE', 3,
 ( #56983, #94850, #91114, #100606, #67040, #23889, #109578, #18126, #7656, #14939, #31206, #58082, #66501, #74885, #33393, #86446, #48584, #49134, #92215, #73786, #6562, #24441 ),
 .UNSPECIFIED., .F., .F.,
 ( 4, 3, 3, 3, 3, 3, 3, 4 ),
 ( -1.499425824813870101, -1.379341959591650069, -1.182344938071870022, -0.9769786663024579987, -0.7652101314604189408, -0.5410848898833939824, -0.3077391086603749049, -0.06613165699310008527 ),
 .UNSPECIFIED. ) ;
#46211=CARTESIAN_POINT ( 'NONE',  ( 1.428000371958690007, 1474.800808632939834, 235.3830380111929799 ) ) ;
#46212=CARTESIAN_POINT ( 'NONE',  ( 4.255689356150000435, 1519.913060387329779, 231.5674970370980077 ) ) ;
#46215=CARTESIAN_POINT ( 'NONE',  ( -1.356962606528219872, 1410.665719724639985, 185.5898146020100228 ) ) ;
#46216=EDGE_CURVE ( 'NONE', #45625, #22768, #35001, .T. ) ;
#46217=CARTESIAN_POINT ( 'NONE',  ( 2.342170655370000354, 1410.304730194330205, 185.5336642671979916 ) ) ;
#46219=CARTESIAN_POINT ( 'NONE',  ( -38.96469809825319430, 1449.667656893509957, 135.7280615607639902 ) ) ;
#46221=CARTESIAN_POINT ( 'NONE',  ( -2.500000000000000000, 1448.200164017079942, 169.1288108960040120 ) ) ;
#46222=CARTESIAN_POINT ( 'NONE',  ( 0.1681681984989999989, 1416.866694505930127, 168.0175527136979667 ) ) ;
#46224=CARTESIAN_POINT ( 'NONE',  ( -5.362054705371839702, 1406.004091175200074, 268.4716808012279898 ) ) ;
#46225=B_SPLINE_CURVE_WITH_KNOTS ( 'NONE', 5,
 ( #37743, #2517, #71391, #95990, #70283, #106592 ),
 .UNSPECIFIED., .F., .F.,
 ( 6, 6 ),
 ( 0.000000000000000000, 1.000000000000000000 ),
 .UNSPECIFIED. ) ;
#46226=CARTESIAN_POINT ( 'NONE',  ( 40.27001047769999786, 1443.957955290329892, 137.1320999901979860 ) ) ;
#46231=AXIS2_PLACEMENT_3D ( 'NONE', #50811, #24482, #51355 ) ;
#46235=VECTOR ( 'NONE', #88974, 1000.000000000000114 ) ;
#46241=CARTESIAN_POINT ( 'NONE',  ( 2.500000000000000000, 1448.386321835900162, 162.4776903873720073 ) ) ;
#46245=CARTESIAN_POINT ( 'NONE',  ( 2.824000625309999624, 1415.931784855930118, 226.7557855299979792 ) ) ;
#46248=ADVANCED_FACE ( 'NONE', ( #97030 ), #33551, .F. ) ;
#46249=CARTESIAN_POINT ( 'NONE',  ( 11.85372022028200512, 1433.007143091356966, 150.3176643612456473 ) ) ;
#46250=CARTESIAN_POINT ( 'NONE',  ( -11.43071925370000130, 1410.242129527830002, 228.7924613954980089 ) ) ;
#46254=CARTESIAN_POINT ( 'NONE',  ( 27.01382310970000233, 1451.969724731730139, 134.9184576876980088 ) ) ;
#46257=DIRECTION ( 'NONE',  ( 0.000000000000000000, 1.000000000000000000, 0.000000000000000000 ) ) ;
#46258=EDGE_CURVE ( 'NONE', #87081, #57154, #51087, .T. ) ;
#46260=CARTESIAN_POINT ( 'NONE',  ( 25.90444642119999941, 1413.781696259030014, 270.1671806362980419 ) ) ;
#46263=ADVANCED_FACE ( 'NONE', ( #65632 ), #58143, .T. ) ;
#46264=CARTESIAN_POINT ( 'NONE',  ( 23.37417682859999957, 1410.122926439930097, 208.1639534942089824 ) ) ;
#46265=CARTESIAN_POINT ( 'NONE',  ( 0.01819570974567621957, 1507.514099832349757, 237.4105189671679739 ) ) ;
#46267=CARTESIAN_POINT ( 'NONE',  ( -11.60004869885203682, 1422.222932908413441, 135.5999999980979851 ) ) ;
#46270=CARTESIAN_POINT ( 'NONE',  ( 4.183002505363929480, 1421.631134843499922, 184.7734457259539909 ) ) ;
#46274=EDGE_LOOP ( 'NONE', ( #72396, #63262, #95818, #80372, #106116 ) ) ;
#46278=CARTESIAN_POINT ( 'NONE',  ( 18.87980474539999776, 1507.654596655130035, 188.5454329983980131 ) ) ;
#46281=DIRECTION ( 'NONE',  ( 0.000000000000000000, -0.9990482215818579093, -0.04361938736533144123 ) ) ;
#46287=ORIENTED_EDGE ( 'NONE', *, *, #46749, .F. ) ;
#46289=ADVANCED_FACE ( 'NONE', ( #17937 ), #97289, .T. ) ;
#46290=CARTESIAN_POINT ( 'NONE',  ( -18.91040668671855585, 1416.839570625527813, 208.2955991069221113 ) ) ;
#46291=VERTEX_POINT ( 'NONE', #8861 ) ;
#46293=CARTESIAN_POINT ( 'NONE',  ( 10.81270716706183599, 1434.527702263565516, 151.9104491927415665 ) ) ;
#46294=EDGE_CURVE ( 'NONE', #98127, #44371, #45746, .T. ) ;
#46297=CARTESIAN_POINT ( 'NONE',  ( -27.36410773769939908, 1509.677412868400097, 201.1425198521210120 ) ) ;
#46298=CARTESIAN_POINT ( 'NONE',  ( -2.707337055090000000, 1447.195466704469936, 162.7581527779979922 ) ) ;
#46299=CARTESIAN_POINT ( 'NONE',  ( -17.84295937140000277, 1424.580744259330004, 226.8532515114980299 ) ) ;
#46300=CARTESIAN_POINT ( 'NONE',  ( -14.75639819380000084, 1435.138401597589791, 148.9684811175980030 ) ) ;
#46303=CARTESIAN_POINT ( 'NONE',  ( 0.7692391029780000222, 1415.628674266529742, 190.8565233057979924 ) ) ;
#46304=CARTESIAN_POINT ( 'NONE',  ( 29.25495648800000126, 1509.872423544630010, 209.6024569297780147 ) ) ;
#46305=CARTESIAN_POINT ( 'NONE',  ( 2.531940903048510086E-08, 1457.850589566970029, 229.0733431205499926 ) ) ;
#46306=ORIENTED_EDGE ( 'NONE', *, *, #15063, .F. ) ;
#46308=CARTESIAN_POINT ( 'NONE',  ( -45.63702719927069751, 1439.462929478074329, 268.9748534858272819 ) ) ;
#46309=CARTESIAN_POINT ( 'NONE',  ( -24.11734304670000029, 1437.967394118240009, 211.4545401520780104 ) ) ;
#46314=CARTESIAN_POINT ( 'NONE',  ( 18.04400385319999955, 1497.713060387329961, 221.4191216194980143 ) ) ;
#46315=CARTESIAN_POINT ( 'NONE',  ( 26.81574339440005872, 1435.910933784995905, 136.5210778358012078 ) ) ;
#46317=VECTOR ( 'NONE', #47551, 1000.000000000000114 ) ;
#46321=CIRCLE ( 'NONE', #73147, 2.000000000088558050 ) ;
#46324=CARTESIAN_POINT ( 'NONE',  ( 20.58555848629999829, 1507.839439013330093, 189.9311647047979932 ) ) ;
#46325=VERTEX_POINT ( 'NONE', #94522 ) ;
#46328=EDGE_LOOP ( 'NONE', ( #64837, #26181, #73882, #70595 ) ) ;
#46329=CARTESIAN_POINT ( 'NONE',  ( 23.55087631299999984, 1411.110694763729953, 207.7642880164279973 ) ) ;
#46331=CARTESIAN_POINT ( 'NONE',  ( 12.68818856000646811, 1442.806559773770005, 169.4610080275735697 ) ) ;
#46332=CARTESIAN_POINT ( 'NONE',  ( 38.46381803922925258, 1428.620948229150599, 269.5839343762438034 ) ) ;
#46333=CARTESIAN_POINT ( 'NONE',  ( -14.70061896320000017, 1464.437658295030133, 244.5173668927980088 ) ) ;
#46334=CARTESIAN_POINT ( 'NONE',  ( -19.92390948350000102, 1487.986067298129910, 190.3334121447979896 ) ) ;
#46335=CARTESIAN_POINT ( 'NONE',  ( -11.73555011919999913, 1433.698852586370094, 150.9369036644980042 ) ) ;
#46337=CARTESIAN_POINT ( 'NONE',  ( -19.35364397750000265, 1485.770172091730046, 189.8349640065979997 ) ) ;
#46340=CARTESIAN_POINT ( 'NONE',  ( 4.435478739589999719, 1421.723673722030071, 185.0752384912979949 ) ) ;
#46343=CARTESIAN_POINT ( 'NONE',  ( 13.15366522099999891, 1428.703228679929907, 223.0784815109979888 ) ) ;
#46345=CARTESIAN_POINT ( 'NONE',  ( 1.394896777640000085, 1465.720900818929977, 235.3343343731980042 ) ) ;
#46348=CARTESIAN_POINT ( 'NONE',  ( -11.86488112544160067, 1432.250788954399923, 149.9817061855939926 ) ) ;
#46350=CARTESIAN_POINT ( 'NONE',  ( -24.79114683279999909, 1465.946749696029883, 269.6862801822979918 ) ) ;
#46353=CARTESIAN_POINT ( 'NONE',  ( -22.53878221424140094, 1411.058442688259902, 212.0450776560099939 ) ) ;
#46354=CARTESIAN_POINT ( 'NONE',  ( 0.3486255395347149788, 1450.932214069980091, 181.6278462867639973 ) ) ;
#46355=CARTESIAN_POINT ( 'NONE',  ( -11.91935979259999989, 1420.493316629130049, 231.2800121289980098 ) ) ;
#46358=CARTESIAN_POINT ( 'NONE',  ( -44.20424317085289800, 1432.326735547540011, 269.0150688337790257 ) ) ;
#46359=ORIENTED_EDGE ( 'NONE', *, *, #86486, .F. ) ;
#46360=CARTESIAN_POINT ( 'NONE',  ( -3.540123473188209857, 1498.107930687619955, 181.3611756044990102 ) ) ;
#46361=EDGE_LOOP ( 'NONE', ( #87536, #54772, #51422, #11227 ) ) ;
#46362=ORIENTED_EDGE ( 'NONE', *, *, #11938, .T. ) ;
#46365=CARTESIAN_POINT ( 'NONE',  ( 12.90973010816660071, 1420.801971354559782, 222.8292615723929941 ) ) ;
#46366=CARTESIAN_POINT ( 'NONE',  ( -14.44835241010000004, 1410.403412957530008, 190.4623667091979939 ) ) ;
#46367=AXIS2_PLACEMENT_3D ( 'NONE', #30499, #64688, #21524 ) ;
#46369=B_SPLINE_SURFACE_WITH_KNOTS ( 'NONE', 5, 5, ( 
 ( #72057, #87167, #61440, #46843, #97764, #10455 ),
 ( #80428, #96114, #46300, #19952, #71517, #18835 ),
 ( #2085, #54695, #21036, #88821, #53031, #55239 ),
 ( #106173, #11567, #63113, #44629, #45743, #36765 ),
 ( #37321, #3742, #27815, #27258, #19388, #28362 ),
 ( #12107, #79327, #28922, #2638, #29453, #63649 ),
 ( #70958, #97213, #20485, #78770, #35653, #105073 ),
 ( #62561, #80972, #96680, #89372, #69843, #36214 ),
 ( #70399, #104517, #54145, #61996, #53591, #87737 ),
 ( #45186, #79880, #3194, #74248, #83179, #92125 ),
 ( #6469, #48492, #4802, #107824, #55797, #5923 ),
 ( #39523, #4276, #56329, #40619, #65292, #5363 ) ),
 .UNSPECIFIED., .F., .F., .F.,
 ( 6, 3, 3, 6 ),
 ( 6, 6 ),
 ( 17.17643422080000093, 21.54070554389999970, 30.24627863650000137, 40.14628357800000202 ),
 ( 0.000000000000000000, 1.622089487970000077 ),
 .UNSPECIFIED. ) ;
#46379=CARTESIAN_POINT ( 'NONE',  ( -27.08078463060560281, 1414.294447406490008, 269.9731611881400113 ) ) ;
#46380=CARTESIAN_POINT ( 'NONE',  ( 2.840828255611359765, 1417.479495435399940, 232.6340383620710099 ) ) ;
#46384=ORIENTED_EDGE ( 'NONE', *, *, #85910, .T. ) ;
#46385=CARTESIAN_POINT ( 'NONE',  ( 44.72498031872709134, 1447.716264930823172, 269.0002976672203090 ) ) ;
#46387=CARTESIAN_POINT ( 'NONE',  ( -13.58978489722930050, 1436.182389225290081, 150.4598382135330041 ) ) ;
#46388=CARTESIAN_POINT ( 'NONE',  ( -0.3901548594470000131, 1486.096337175529925, 181.7750788774980037 ) ) ;
#46390=CARTESIAN_POINT ( 'NONE',  ( -19.81028112772915861, 1506.776553272468618, 219.5992980689768217 ) ) ;
#46394=CARTESIAN_POINT ( 'NONE',  ( 5.317239278416240111, 1475.759745378969910, 269.0458115274469719 ) ) ;
#46395=CARTESIAN_POINT ( 'NONE',  ( 11.54717405569999933, 1415.048591087029763, 222.4184568667979818 ) ) ;
#46396=CARTESIAN_POINT ( 'NONE',  ( 3.880449101349999985, 1446.827807606209944, 183.7827426791980088 ) ) ;
#46400=CARTESIAN_POINT ( 'NONE',  ( -21.96271729628280411, 1452.898244988618899, 220.9930576170047232 ) ) ;
#46402=CARTESIAN_POINT ( 'NONE',  ( 12.43875923093532343, 1454.082076206495913, 225.3359954487575010 ) ) ;
#46406=CARTESIAN_POINT ( 'NONE',  ( 18.87295847649999914, 1409.572118621430036, 197.2370177091979997 ) ) ;
#46407=CARTESIAN_POINT ( 'NONE',  ( 20.87866911129999892, 1445.052233488290085, 177.0630364655980031 ) ) ;
#46408=CARTESIAN_POINT ( 'NONE',  ( -23.91862134480000179, 1435.332757494850057, 136.7253933288979795 ) ) ;
#46412=CARTESIAN_POINT ( 'NONE',  ( 2.500000000000000000, 1439.624612761979961, 169.0979957011440149 ) ) ;
#46418=CARTESIAN_POINT ( 'NONE',  ( -1273.316865285699805, 2833.596074015789782, 9977.675558182170789 ) ) ;
#46419=CARTESIAN_POINT ( 'NONE',  ( -37.35391162073399585, 1449.318672761829930, 136.3174603101959974 ) ) ;
#46420=ADVANCED_FACE ( 'NONE', ( #49790 ), #23992, .F. ) ;
#46421=CARTESIAN_POINT ( 'NONE',  ( 10.91790884276356266, 1424.877151459083962, 138.2600712752583547 ) ) ;
#46422=DIRECTION ( 'NONE',  ( -1.000000000000000000, -5.823966869780190178E-19, 4.137698748469999823E-18 ) ) ;
#46423=CARTESIAN_POINT ( 'NONE',  ( -2.500000000000000000, 1426.216228438830058, 155.9944625376979843 ) ) ;
#46424=CARTESIAN_POINT ( 'NONE',  ( 11.87499166480000135, 1433.007134997589901, 150.0931860300979963 ) ) ;
#46425=CARTESIAN_POINT ( 'NONE',  ( -44.92381709066269480, 1440.913053709800124, 269.6913904019010033 ) ) ;
#46431=CARTESIAN_POINT ( 'NONE',  ( 11.23388613411650105, 1443.913060387330006, 150.9272215568489912 ) ) ;
#46432=CARTESIAN_POINT ( 'NONE',  ( -2.695946298204319636, 1485.848501370371878, 182.4462471310350793 ) ) ;
#46434=CARTESIAN_POINT ( 'NONE',  ( 2.116402719909999952, 1507.098271169029886, 236.1684022847979918 ) ) ;
#46437=CARTESIAN_POINT ( 'NONE',  ( -10.18845689910000019, 1507.986917720829979, 234.4944681294980171 ) ) ;
#46439=CARTESIAN_POINT ( 'NONE',  ( 19.44117294853580091, 1456.941945407359981, 224.4539793896520052 ) ) ;
#46440=CARTESIAN_POINT ( 'NONE',  ( 2.499944775320749990, 1419.515170344529906, 137.7430823675560134 ) ) ;
#46442=CARTESIAN_POINT ( 'NONE',  ( 1.742626253590000118, 1466.605724893630168, 234.7106070462979801 ) ) ;
#46444=VERTEX_POINT ( 'NONE', #100712 ) ;
#46445=CARTESIAN_POINT ( 'NONE',  ( -1.141221057759999935, 1450.801352449960177, 182.0259209118979982 ) ) ;
#46449=CARTESIAN_POINT ( 'NONE',  ( 1.547463896846929865, 1414.913060387349788, 192.3096116128920130 ) ) ;
#46452=EDGE_LOOP ( 'NONE', ( #11245, #30734, #49723 ) ) ;
#46454=CARTESIAN_POINT ( 'NONE',  ( 12.81436426557939967, 1447.032452139500037, 186.0874941928050248 ) ) ;
#46455=CARTESIAN_POINT ( 'NONE',  ( 13.80546151116429954, 1434.979654507460054, 148.5370226032280243 ) ) ;
#46460=CARTESIAN_POINT ( 'NONE',  ( 10.25464339219990073, 1409.271160421150171, 220.0084936090869974 ) ) ;
#46461=CARTESIAN_POINT ( 'NONE',  ( -33.91369110979979951, 1435.681798629080049, 135.0664268289980043 ) ) ;
#46463=DIRECTION ( 'NONE',  ( -0.9861488070177710785, 0.1648740218884660325, -0.01808555566601800085 ) ) ;
#46465=CIRCLE ( 'NONE', #96488, 2.000000000000000000 ) ;
#46469=( BOUNDED_CURVE ( )  B_SPLINE_CURVE ( 3, ( #2398, #12407, #46591, #79641 ),
 .UNSPECIFIED., .F., .F. ) 
 B_SPLINE_CURVE_WITH_KNOTS ( ( 4, 4 ),
 ( 1.070796326794966058, 1.570796326794965614 ),
 .UNSPECIFIED. ) 
 CURVE ( )  GEOMETRIC_REPRESENTATION_ITEM ( )  RATIONAL_B_SPLINE_CURVE ( ( 1.000000000000000000, 0.9792749478070965630, 0.9792749478070965630, 1.000000000000000000 ) ) 
 REPRESENTATION_ITEM ( '' )  );
#46471=CARTESIAN_POINT ( 'NONE',  ( -11.74953517305270090, 1415.393085341020196, 195.1736183478689668 ) ) ;
#46473=CARTESIAN_POINT ( 'NONE',  ( 16.29513934676993969, 1469.031411797243663, 269.3703662538208050 ) ) ;
#46474=CARTESIAN_POINT ( 'NONE',  ( -20.22039848381579574, 1495.569241252630036, 190.7459851463269729 ) ) ;
#46475=CARTESIAN_POINT ( 'NONE',  ( 4.487326635059999624, 1396.069761286429866, 219.5977994197980081 ) ) ;
#46477=CARTESIAN_POINT ( 'NONE',  ( -12.53380499174499896, 1445.052233488290085, 169.4755105688890069 ) ) ;
#46479=CARTESIAN_POINT ( 'NONE',  ( -20.11865724026149849, 1457.295805411310084, 208.8536593322139936 ) ) ;
#46483=CARTESIAN_POINT ( 'NONE',  ( -13.76849749719999849, 1435.338886191890197, 149.7896896373979985 ) ) ;
#46486=DIRECTION ( 'NONE',  ( 0.000000000000000000, 0.000000000000000000, 1.000000000000000000 ) ) ;
#46488=CARTESIAN_POINT ( 'NONE',  ( 41.02301855367610273, 1444.170996474450021, 136.8522558531069819 ) ) ;
#46489=VERTEX_POINT ( 'NONE', #24547 ) ;
#46490=CARTESIAN_POINT ( 'NONE',  ( 20.03573725999999766, 1421.675448603130008, 240.3194873134980014 ) ) ;
#46491=CARTESIAN_POINT ( 'NONE',  ( -26.66951752270000142, 1488.685949851729902, 205.2938759693780071 ) ) ;
#46492=CARTESIAN_POINT ( 'NONE',  ( -0.5406448194880001390, 1507.263894173830067, 180.8238120802979836 ) ) ;
#46493=CARTESIAN_POINT ( 'NONE',  ( 3.390830802950000193E-14, 1412.903649629229903, 264.4545146410980010 ) ) ;
#46495=TOROIDAL_SURFACE ( 'NONE', #96600, 20.98341875039999849, 2.000000000000000000 ) ;
#46496=CARTESIAN_POINT ( 'NONE',  ( -32.03901054129999437, 1430.123112395929866, 250.0966427571979978 ) ) ;
#46497=CARTESIAN_POINT ( 'NONE',  ( 19.64611444698550002, 1509.628769227909970, 231.3538552484560000 ) ) ;
#46498=CARTESIAN_POINT ( 'NONE',  ( 0.9264612404903812548, 1415.565606034773054, 233.1932629902654810 ) ) ;
#46499=CARTESIAN_POINT ( 'NONE',  ( 1.674813627306420027, 1416.913057013589878, 192.1894777045280023 ) ) ;
#46501=CARTESIAN_POINT ( 'NONE',  ( -11.22085815268440001, 1416.913060341719984, 220.6193217018360144 ) ) ;
#46503=CARTESIAN_POINT ( 'NONE',  ( 11.68641999220000116, 1509.361170997829959, 236.6365785814979859 ) ) ;
#46504=VERTEX_POINT ( 'NONE', #59309 ) ;
#46506=CARTESIAN_POINT ( 'NONE',  ( 2.890489020090289962, 1507.108937781499890, 235.9439513786750240 ) ) ;
#46507=CARTESIAN_POINT ( 'NONE',  ( -24.07937766809569879, 1410.986708645050157, 208.6133125710570084 ) ) ;
#46509=CARTESIAN_POINT ( 'NONE',  ( 0.08494797014840001215, 1421.818460406029999, 227.4435403455979952 ) ) ;
#46511=CARTESIAN_POINT ( 'NONE',  ( -14.76404367679999829, 1479.765582119930059, 230.2923287122980014 ) ) ;
#46514=CARTESIAN_POINT ( 'NONE',  ( 11.73704819359999973, 1426.695975325029849, 144.1715469084980157 ) ) ;
#46515=CARTESIAN_POINT ( 'NONE',  ( -12.93742170084479959, 1415.431750870119913, 221.3405841367710138 ) ) ;
#46517=ORIENTED_EDGE ( 'NONE', *, *, #45206, .T. ) ;
#46519=ORIENTED_EDGE ( 'NONE', *, *, #10545, .F. ) ;
#46520=CARTESIAN_POINT ( 'NONE',  ( 11.86211521484639952, 1432.057615692780018, 149.9751993002209929 ) ) ;
#46524=ORIENTED_EDGE ( 'NONE', *, *, #43271, .T. ) ;
#46526=CARTESIAN_POINT ( 'NONE',  ( 3.045280019940000305, 1464.258769156330118, 233.3054829794980094 ) ) ;
#46529=CARTESIAN_POINT ( 'NONE',  ( 17.79764678428299973, 1452.291552866509846, 145.5855917355939937 ) ) ;
#46534=CARTESIAN_POINT ( 'NONE',  ( -11.87490713740000103, 1433.006767100669776, 150.3951466367980174 ) ) ;
#46535=CARTESIAN_POINT ( 'NONE',  ( 0.03661006106857637304, 1409.805696954575524, 233.1128360409267657 ) ) ;
#46539=CARTESIAN_POINT ( 'NONE',  ( -25.51896244293709870, 1509.784549317990013, 223.0112913589669859 ) ) ;
#46541=ORIENTED_EDGE ( 'NONE', *, *, #85145, .F. ) ;
#46542=CARTESIAN_POINT ( 'NONE',  ( 12.15345577959999979, 1413.272114225030009, 265.6112252686980355 ) ) ;
#46551=CARTESIAN_POINT ( 'NONE',  ( -2.878008746956259856, 1440.267634386450027, 157.3979731866919849 ) ) ;
#46556=CARTESIAN_POINT ( 'NONE',  ( 17.14290233499820104, 1509.642557952590096, 233.9671050410080113 ) ) ;
#46559=CARTESIAN_POINT ( 'NONE',  ( 16.60571044980000366, 1417.431011486929947, 226.8588397439980042 ) ) ;
#46565=CARTESIAN_POINT ( 'NONE',  ( 46.05259010380000007, 1440.913083222670139, 266.6770556958979910 ) ) ;
#46566=CARTESIAN_POINT ( 'NONE',  ( -17.35552329220000090, 1409.519128615229874, 223.9298083007980154 ) ) ;
#46567=CARTESIAN_POINT ( 'NONE',  ( 20.76392971010000110, 1435.368631235799967, 143.5555241923979963 ) ) ;
#46568=CARTESIAN_POINT ( 'NONE',  ( 21.62573963749999706, 1508.012258617029829, 191.4661207822979918 ) ) ;
#46569=CARTESIAN_POINT ( 'NONE',  ( -17.00059099016130304, 1410.433725695080057, 191.9734673053639824 ) ) ;
#46570=CARTESIAN_POINT ( 'NONE',  ( -3.721063415729999695E-09, 1475.837061091930082, 266.9611530633980010 ) ) ;
#46573=CARTESIAN_POINT ( 'NONE',  ( 0.2173304821316540125, 1453.251628194559999, 183.2425976906270080 ) ) ;
#46574=CARTESIAN_POINT ( 'NONE',  ( -12.83650301490549950, 1408.840943845570109, 203.6725700213090136 ) ) ;
#46575=CARTESIAN_POINT ( 'NONE',  ( -15.56083348049999948, 1415.425433635630043, 200.9032378748180179 ) ) ;
#46580=CARTESIAN_POINT ( 'NONE',  ( -37.28324836091690742, 1436.551445511060138, 134.0999999968369991 ) ) ;
#46584=CARTESIAN_POINT ( 'NONE',  ( -1.893628906283649993, 1408.979187365889857, 223.9928269826189933 ) ) ;
#46587=CARTESIAN_POINT ( 'NONE',  ( 15.16119009004890117, 1509.174112450859866, 232.9869830570750082 ) ) ;
#46588=CARTESIAN_POINT ( 'NONE',  ( -30.19712123989999952, 1467.538238601129933, 267.1520868254980314 ) ) ;
#46590=CARTESIAN_POINT ( 'NONE',  ( 18.90776566690000138, 1416.839648768830102, 210.0259813939200058 ) ) ;
#46591=CARTESIAN_POINT ( 'NONE',  ( 1.347412987175395260, 1395.960113085665625, 217.1218459616980283 ) ) ;
#46597=CARTESIAN_POINT ( 'NONE',  ( 17.60627569411529691, 1410.895669416499913, 224.1775087544040161 ) ) ;
#46598=CARTESIAN_POINT ( 'NONE',  ( 0.4877217612525719947, 1418.262951728039980, 184.7316173986440333 ) ) ;
#46599=ORIENTED_EDGE ( 'NONE', *, *, #68110, .F. ) ;
#46601=EDGE_CURVE ( 'NONE', #108746, #60035, #61826, .T. ) ;
#46604=EDGE_CURVE ( 'NONE', #36273, #59045, #85431, .T. ) ;
#46605=CARTESIAN_POINT ( 'NONE',  ( 23.97466837309999832, 1430.490890388329944, 207.3419347240379977 ) ) ;
#46606=CARTESIAN_POINT ( 'NONE',  ( -12.61566532500000015, 1416.819756528530206, 194.9201883977979719 ) ) ;
#46610=CARTESIAN_POINT ( 'NONE',  ( 23.85787685490000243, 1410.668016354230076, 210.4985967482580236 ) ) ;
#46611=B_SPLINE_SURFACE_WITH_KNOTS ( 'NONE', 5, 5, ( 
 ( #64887, #81101, #65991, #107957, #100113, #23396 ),
 ( #64330, #14984, #84948, #67089, #34561, #59238 ),
 ( #101191, #24489, #50287, #101748, #25036, #9366 ),
 ( #67636, #60331, #109621, #43530, #68201, #68744 ),
 ( #440, #58675, #50817, #986, #77673, #84416 ),
 ( #102847, #42976, #15531, #26140, #92810, #76562 ) ),
 .UNSPECIFIED., .F., .F., .F.,
 ( 6, 6 ),
 ( 6, 6 ),
 ( 0.8543875779139999960, 1.193533517340000127 ),
 ( 0.000000000000000000, 2.000000000000000000 ),
 .UNSPECIFIED. ) ;
#46612=CARTESIAN_POINT ( 'NONE',  ( 3.914929521479999952, 1435.141524774260006, 184.8876600372980192 ) ) ;
#46615=FACE_OUTER_BOUND ( 'NONE', #10053, .T. ) ;
#46618=CARTESIAN_POINT ( 'NONE',  ( -7.228663065755881689, 1512.913060387330006, 183.1074954935087646 ) ) ;
#46624=CARTESIAN_POINT ( 'NONE',  ( -17.48302101486839888, 1486.143752436420073, 188.0522656724239994 ) ) ;
#46627=VERTEX_POINT ( 'NONE', #75829 ) ;
#46628=ORIENTED_EDGE ( 'NONE', *, *, #15063, .T. ) ;
#46629=CARTESIAN_POINT ( 'NONE',  ( 28.75306184379999763, 1509.589359938030157, 209.8852704373689733 ) ) ;
#46633=CARTESIAN_POINT ( 'NONE',  ( 15.74014332448429876, 1412.735343691740127, 191.4587741565329964 ) ) ;
#46634=CARTESIAN_POINT ( 'NONE',  ( 1.279965696769999939, 1508.893017011729853, 179.9879573282979948 ) ) ;
#46635=CARTESIAN_POINT ( 'NONE',  ( 12.00000000000000000, 1443.913060387330006, 150.5878346084980137 ) ) ;
#46637=CARTESIAN_POINT ( 'NONE',  ( -24.35936372944500050, 1451.998951890219814, 137.0312813218010035 ) ) ;
#46638=CARTESIAN_POINT ( 'NONE',  ( 12.13968626136060891, 1436.959392319449307, 151.4453562942360350 ) ) ;
#46639=CARTESIAN_POINT ( 'NONE',  ( 13.94099194679999876, 1410.772699170629949, 228.0747510220979848 ) ) ;
#46641=SURFACE_STYLE_USAGE ( .BOTH. , #10819 ) ;
#46642=EDGE_CURVE ( 'NONE', #93372, #86029, #246, .T. ) ;
#46643=CARTESIAN_POINT ( 'NONE',  ( 41.56910739862709647, 1442.487573087749979, 134.0999999980959956 ) ) ;
#46644=CIRCLE ( 'NONE', #71926, 1.999236069818542960 ) ;
#46646=ORIENTED_EDGE ( 'NONE', *, *, #68566, .T. ) ;
#46647=CARTESIAN_POINT ( 'NONE',  ( 14.57896927624650019, 1436.094750401150122, 149.8401917988270213 ) ) ;
#46648=CARTESIAN_POINT ( 'NONE',  ( -17.19011713638783334, 1410.879030080967823, 226.0567197966691992 ) ) ;
#46649=VERTEX_POINT ( 'NONE', #102112 ) ;
#46651=EDGE_CURVE ( 'NONE', #97278, #46489, #1714, .T. ) ;
#46656=CARTESIAN_POINT ( 'NONE',  ( 6.009315719639841014, 1451.457099272296318, 153.4908535104837313 ) ) ;
#46658=CARTESIAN_POINT ( 'NONE',  ( -15.81087456010765102, 1450.970563601593767, 221.9774777022516332 ) ) ;
#46661=CARTESIAN_POINT ( 'NONE',  ( -1.320018102479999955, 1507.624001479029857, 232.0809353007979894 ) ) ;
#46662=CARTESIAN_POINT ( 'NONE',  ( 9.790177624210000928, 1414.971287085330005, 195.6150972186979971 ) ) ;
#46667=CARTESIAN_POINT ( 'NONE',  ( 27.31982573739979969, 1440.913060387330006, 245.8751062284599982 ) ) ;
#46668=CONICAL_SURFACE ( 'NONE', #78767, 1.000000000000009104, 0.7853981633970000820 ) ;
#46669=CARTESIAN_POINT ( 'NONE',  ( -17.21313104309999886, 1509.582386186229769, 184.6661624875980010 ) ) ;
#46671=CARTESIAN_POINT ( 'NONE',  ( -33.93390012576846715, 1451.576011116597783, 135.5842836269593192 ) ) ;
#46672=CARTESIAN_POINT ( 'NONE',  ( -15.66085203299999762, 1409.459949385129903, 192.2846886866980185 ) ) ;
#46674=CARTESIAN_POINT ( 'NONE',  ( -24.67090459839999994, 1441.025736683209971, 210.6889990472880072 ) ) ;
#46675=CARTESIAN_POINT ( 'NONE',  ( -0.4558760921085245887, 1414.913060387330006, 225.2405208435152701 ) ) ;
#46678=CARTESIAN_POINT ( 'NONE',  ( 1.770390159249999984, 1406.013915744430051, 266.9599398126979963 ) ) ;
#46681=CARTESIAN_POINT ( 'NONE',  ( 2.887394341690000310, 1464.524587323030119, 235.8761363967979889 ) ) ;
#46682=CARTESIAN_POINT ( 'NONE',  ( -11.60004869885203682, 1425.894669240205303, 137.5118602016662237 ) ) ;
#46686=CARTESIAN_POINT ( 'NONE',  ( -0.04370337965792400053, 1508.780601165080043, 179.8640435178710106 ) ) ;
#46687=CARTESIAN_POINT ( 'NONE',  ( 19.42500282749999840, 1440.913060387330006, 212.4633492400480179 ) ) ;
#46689=CARTESIAN_POINT ( 'NONE',  ( -19.82086717690000199, 1452.811554597929899, 208.9556627768919839 ) ) ;
#46690=CARTESIAN_POINT ( 'NONE',  ( -4.044582423638403590, 1419.921508911728779, 137.0999999980979851 ) ) ;
#46693=CARTESIAN_POINT ( 'NONE',  ( -1.159637561150000051, 1415.063410489829948, 226.6648382762980134 ) ) ;
#46694=CARTESIAN_POINT ( 'NONE',  ( 19.57999186420000015, 1459.737765858830016, 238.2202666691980255 ) ) ;
#46695=CARTESIAN_POINT ( 'NONE',  ( -11.86606752090000150, 1432.333718217379783, 149.9825819519979859 ) ) ;
#46699=EDGE_CURVE ( 'NONE', #38044, #9577, #4097, .T. ) ;
#46700=CARTESIAN_POINT ( 'NONE',  ( -19.92408690999999976, 1457.445828243930009, 225.3974416310980189 ) ) ;
#46704=ORIENTED_EDGE ( 'NONE', *, *, #16149, .T. ) ;
#46706=CARTESIAN_POINT ( 'NONE',  ( 0.8854628104720000392, 1405.995467260429905, 266.9608410729979937 ) ) ;
#46708=AXIS2_PLACEMENT_3D ( 'NONE', #100571, #31715, #109542 ) ;
#46710=CARTESIAN_POINT ( 'NONE',  ( 39.82896661013450057, 1456.864206082610053, 270.1537018815570264 ) ) ;
#46712=DIRECTION ( 'NONE',  ( 0.000000000000000000, 1.000000000000000000, 0.000000000000000000 ) ) ;
#46717=CARTESIAN_POINT ( 'NONE',  ( -1.557202951210026276, 1451.015816330957477, 183.5890866117867688 ) ) ;
#46718=CARTESIAN_POINT ( 'NONE',  ( 1.967245043674230365, 1450.337415823809806, 154.7913109945830286 ) ) ;
#46719=CARTESIAN_POINT ( 'NONE',  ( -14.40791762929059949, 1416.384967875099846, 221.3406101171449905 ) ) ;
#46722=CARTESIAN_POINT ( 'NONE',  ( -26.42714720800000094, 1437.883259617029807, 243.9198229606980135 ) ) ;
#46725=CARTESIAN_POINT ( 'NONE',  ( -0.3399431336819999649, 1476.108518450929978, 267.8539949209979909 ) ) ;
#46727=CARTESIAN_POINT ( 'NONE',  ( -18.34590456075780196, 1416.851343895820037, 208.8605686865189739 ) ) ;
#46728=CARTESIAN_POINT ( 'NONE',  ( -3.207697512962450315, 1448.279240478991369, 184.6677887077926528 ) ) ;
#46734=CARTESIAN_POINT ( 'NONE',  ( -11.07153876272299975, 1396.299687040369918, 208.9417196923349991 ) ) ;
#46735=EDGE_CURVE ( 'NONE', #22237, #96609, #72509, .T. ) ;
#46737=CARTESIAN_POINT ( 'NONE',  ( -15.82161016549999921, 1420.644138379529750, 227.0290855803980037 ) ) ;
#46738=B_SPLINE_CURVE_WITH_KNOTS ( 'NONE', 3,
 ( #30185, #64377, #110771, #93960 ),
 .UNSPECIFIED., .F., .F.,
 ( 4, 4 ),
 ( 0.000000000000000000, 1.000000000000000000 ),
 .UNSPECIFIED. ) ;
#46739=CARTESIAN_POINT ( 'NONE',  ( 19.26863053809116622, 1456.090792970590655, 225.0961701050973431 ) ) ;
#46740=VERTEX_POINT ( 'NONE', #48856 ) ;
#46742=CARTESIAN_POINT ( 'NONE',  ( 2.760778241670000188, 1409.009468887930097, 230.1977506513979961 ) ) ;
#46743=CARTESIAN_POINT ( 'NONE',  ( -17.41081140942853622, 1485.005952666161875, 188.5080410486085896 ) ) ;
#46745=CARTESIAN_POINT ( 'NONE',  ( 11.48672039610000084, 1426.428532722830141, 126.2854488628979936 ) ) ;
#46747=FACE_OUTER_BOUND ( 'NONE', #20835, .T. ) ;
#46748=CARTESIAN_POINT ( 'NONE',  ( -11.23388613411650105, 1443.913060387330006, 151.7784653951599978 ) ) ;
#46749=EDGE_CURVE ( 'NONE', #43965, #61502, #32433, .T. ) ;
#46753=CARTESIAN_POINT ( 'NONE',  ( 4.486266698770000616, 1509.079604303730093, 179.9451462963979793 ) ) ;
#46758=EDGE_CURVE ( 'NONE', #73741, #104178, #37798, .T. ) ;
#46761=ORIENTED_EDGE ( 'NONE', *, *, #70127, .F. ) ;
#46762=CARTESIAN_POINT ( 'NONE',  ( -5.639077333919999546, 1396.170382963030079, 198.9228296477979825 ) ) ;
#46763=CARTESIAN_POINT ( 'NONE',  ( 1.156245593104790137, 1474.789461591380132, 235.6542973942920014 ) ) ;
#46764=CARTESIAN_POINT ( 'NONE',  ( -4.440892098499999806E-15, 1519.913060387329779, 231.7062449670980300 ) ) ;
#46767=CARTESIAN_POINT ( 'NONE',  ( -1.361090702285459919, 1413.800366288759960, 185.4570810730789958 ) ) ;
#46768=CARTESIAN_POINT ( 'NONE',  ( 14.72486392259999910, 1429.763008465929943, 190.7271437690980065 ) ) ;
#46770=CARTESIAN_POINT ( 'NONE',  ( -36.84775941671910005, 1449.744939508739890, 136.2617221972240031 ) ) ;
#46771=CARTESIAN_POINT ( 'NONE',  ( 39.80563939443820232, 1439.297435335050068, 136.4608509805550227 ) ) ;
#46773=FACE_OUTER_BOUND ( 'NONE', #93818, .T. ) ;
#46774=CARTESIAN_POINT ( 'NONE',  ( 11.55327403699999955, 1430.567211606730098, 150.9659738814980017 ) ) ;
#46776=ORIENTED_EDGE ( 'NONE', *, *, #80306, .F. ) ;
#46777=CARTESIAN_POINT ( 'NONE',  ( -12.53380499169999851, 1442.773887286369927, 169.4755105685979970 ) ) ;
#46779=ORIENTED_EDGE ( 'NONE', *, *, #73249, .T. ) ;
#46782=CARTESIAN_POINT ( 'NONE',  ( -19.57912521677359763, 1488.016130565860067, 228.2702076737010088 ) ) ;
#46784=CARTESIAN_POINT ( 'NONE',  ( -17.36305420999961058, 1410.600123101027066, 225.7636173774992017 ) ) ;
#46790=CARTESIAN_POINT ( 'NONE',  ( -8.956458691531819838, 1509.358275544009985, 180.2336362669479968 ) ) ;
#46793=CARTESIAN_POINT ( 'NONE',  ( 18.88659680459999990, 1416.522662136229883, 210.6651046700080201 ) ) ;
#46796=CARTESIAN_POINT ( 'NONE',  ( -41.79940509948184513, 1437.492528948050449, 269.6436970879940418 ) ) ;
#46797=CARTESIAN_POINT ( 'NONE',  ( -2.573074615509999941, 1409.002914132830028, 231.1540680731980046 ) ) ;
#46798=DIRECTION ( 'NONE',  ( 0.4857255149070415778, -0.7475168846447919346, -0.4530885469080344619 ) ) ;
#46799=ORIENTED_EDGE ( 'NONE', *, *, #77567, .T. ) ;
#46801=CARTESIAN_POINT ( 'NONE',  ( 28.30919303740000004, 1508.136605797730226, 209.0041157894929995 ) ) ;
#46803=CARTESIAN_POINT ( 'NONE',  ( 15.66042904549793136, 1506.491018775014027, 224.6173112146069002 ) ) ;
#46805=CARTESIAN_POINT ( 'NONE',  ( 28.35905216135870077, 1416.639651061350150, 270.3509323902579808 ) ) ;
#46808=CARTESIAN_POINT ( 'NONE',  ( 22.68006499860000247, 1409.705091528429875, 208.7629400170540066 ) ) ;
#46809=CARTESIAN_POINT ( 'NONE',  ( 0.008918347722598321536, 1508.393983269119872, 237.8902324756037672 ) ) ;
#46813=CARTESIAN_POINT ( 'NONE',  ( 4.363122683464830232, 1421.971318488559973, 183.8271341761570170 ) ) ;
#46814=CARTESIAN_POINT ( 'NONE',  ( -0.4152942141409999843, 1420.456388890930157, 233.6206558093980163 ) ) ;
#46817=ORIENTED_EDGE ( 'NONE', *, *, #87858, .F. ) ;
#46821=CARTESIAN_POINT ( 'NONE',  ( -20.79161711910150245, 1507.840252237830100, 228.0156062829520067 ) ) ;
#46824=CARTESIAN_POINT ( 'NONE',  ( 0.5096330788092879871, 1452.969753185240052, 183.2932557940929996 ) ) ;
#46825=EDGE_CURVE ( 'NONE', #52145, #96903, #8461, .T. ) ;
#46828=CARTESIAN_POINT ( 'NONE',  ( 18.87155961639999902, 1509.015964899329902, 188.0102586092980061 ) ) ;
#46832=CARTESIAN_POINT ( 'NONE',  ( 28.77213281030099878, 1509.917805400869838, 206.8662417278609951 ) ) ;
#46833=EDGE_LOOP ( 'NONE', ( #67045, #93247, #17235, #93060, #48103 ) ) ;
#46835=CARTESIAN_POINT ( 'NONE',  ( 11.60004869884797429, 1426.654319849603780, 134.6710116165313877 ) ) ;
#46836=DIRECTION ( 'NONE',  ( -0.03084237732693835901, -0.9990097606182641865, -0.03206627434332531140 ) ) ;
#46839=CARTESIAN_POINT ( 'NONE',  ( -26.48205241774240193, 1508.638501742070048, 201.4894952595709867 ) ) ;
#46841=CARTESIAN_POINT ( 'NONE',  ( -4.239021722809999559, 1446.365493693999952, 162.7142554342980247 ) ) ;
#46842=CARTESIAN_POINT ( 'NONE',  ( -19.00435212720000422, 1425.942472208630079, 225.6636987373979935 ) ) ;
#46843=CARTESIAN_POINT ( 'NONE',  ( -14.43917572210000166, 1435.432076402839812, 149.5787593319979862 ) ) ;
#46845=CARTESIAN_POINT ( 'NONE',  ( 16.45201478129999728, 1509.487577403229807, 185.2161393109980168 ) ) ;
#46847=CARTESIAN_POINT ( 'NONE',  ( -18.16584306366592116, 1435.617507662623666, 214.1170364969505044 ) ) ;
#46850=CARTESIAN_POINT ( 'NONE',  ( -2.496058351850642065, 1410.375802693013156, 186.5499807929696772 ) ) ;
#46851=EDGE_CURVE ( 'NONE', #107006, #76166, #20327, .T. ) ;
#46856=CARTESIAN_POINT ( 'NONE',  ( -18.56679401179999900, 1509.561427120029975, 231.0972437537980113 ) ) ;
#46858=CARTESIAN_POINT ( 'NONE',  ( -13.24295770958712737, 1443.166206736402501, 186.8421231537473943 ) ) ;
#46859=CARTESIAN_POINT ( 'NONE',  ( -17.11711237129999930, 1414.913528139930122, 207.5661155201680117 ) ) ;
#46865=CARTESIAN_POINT ( 'NONE',  ( 20.15452338710000291, 1507.845775801930131, 189.3412755345979690 ) ) ;
#46871=ORIENTED_EDGE ( 'NONE', *, *, #52584, .F. ) ;
#46872=CARTESIAN_POINT ( 'NONE',  ( 25.69821269425319699, 1461.615829411680124, 207.7065348595210139 ) ) ;
#46873=CARTESIAN_POINT ( 'NONE',  ( 13.63495199149999948, 1509.148422029330050, 233.7524325507980052 ) ) ;
#46875=CARTESIAN_POINT ( 'NONE',  ( 27.62485365530106307, 1417.942135513340645, 269.4472113980168047 ) ) ;
#46876=CARTESIAN_POINT ( 'NONE',  ( -31.95512683489999617, 1440.913060389640123, 244.1805851169980031 ) ) ;
#46878=CARTESIAN_POINT ( 'NONE',  ( -19.88572119940000249, 1484.728770958729910, 191.0592868864980005 ) ) ;
#46879=CARTESIAN_POINT ( 'NONE',  ( -11.74481771089999960, 1433.726929579510170, 150.9290601731980246 ) ) ;
#46880=ADVANCED_FACE ( 'NONE', ( #41119 ), #78478, .F. ) ;
#46883=CARTESIAN_POINT ( 'NONE',  ( 11.61068082338428376, 1426.780165915954285, 135.1396153442166508 ) ) ;
#46887=CARTESIAN_POINT ( 'NONE',  ( -12.89608512423069975, 1434.724840024559853, 149.2206170422699927 ) ) ;
#46892=CARTESIAN_POINT ( 'NONE',  ( 1.181658762251719971E-08, 1409.019473503670042, 260.8196857114169802 ) ) ;
#46895=CARTESIAN_POINT ( 'NONE',  ( -11.86550914360719844, 1432.294685167699981, 149.9822461645989904 ) ) ;
#46897=CARTESIAN_POINT ( 'NONE',  ( -14.88997911370000082, 1470.145154249029702, 270.0818331703979425 ) ) ;
#46898=CARTESIAN_POINT ( 'NONE',  ( -23.78956544001448137, 1436.033567404351288, 211.5876866959136180 ) ) ;
#46900=CARTESIAN_POINT ( 'NONE',  ( -14.12009054920000040, 1452.401137584329945, 223.0071355110979994 ) ) ;
#46902=CARTESIAN_POINT ( 'NONE',  ( 0.2108446687585300017, 1451.971434986430040, 183.0264145658140080 ) ) ;
#46903=CARTESIAN_POINT ( 'NONE',  ( -13.34103997769999950, 1419.849113831329760, 228.0065750030979927 ) ) ;
#46905=DIRECTION ( 'NONE',  ( 0.9993902469228587160, -0.03489947646764298556, -0.001077449651559719661 ) ) ;
#46907=CARTESIAN_POINT ( 'NONE',  ( -45.49343607084999519, 1434.389643311759983, 267.6171445062669250 ) ) ;
#46908=ORIENTED_EDGE ( 'NONE', *, *, #63971, .F. ) ;
#46909=CARTESIAN_POINT ( 'NONE',  ( -3.549085716194020357, 1506.761702413250077, 180.9924597521999772 ) ) ;
#46914=CARTESIAN_POINT ( 'NONE',  ( 33.08096890875820151, 1445.052233488291222, 154.3416101011785031 ) ) ;
#46917=CARTESIAN_POINT ( 'NONE',  ( -17.06344815410000137, 1425.426455383629900, 191.2828403587980119 ) ) ;
#46919=CARTESIAN_POINT ( 'NONE',  ( -2.382487917691452406, 1449.571493106297112, 183.0105235244745074 ) ) ;
#46920=VERTEX_POINT ( 'NONE', #34924 ) ;
#46927=CARTESIAN_POINT ( 'NONE',  ( -8.364488026064709203, 1410.621949147049918, 269.8709166813640650 ) ) ;
#46928=CARTESIAN_POINT ( 'NONE',  ( -30.78500370360000105, 1435.572563320330119, 135.1635738117979884 ) ) ;
#46929=CARTESIAN_POINT ( 'NONE',  ( 0.01233320375960000014, 1396.097901045329991, 197.1956428527979881 ) ) ;
#46933=CARTESIAN_POINT ( 'NONE',  ( 42.49826213307465395, 1453.378461683928663, 269.0622770231100844 ) ) ;
#46935=CARTESIAN_POINT ( 'NONE',  ( -2.500000000000000000, 1419.383167280829866, 144.0983880305979881 ) ) ;
#46936=CARTESIAN_POINT ( 'NONE',  ( -0.03529809467915469984, 1410.073064431770035, 185.0480559684600053 ) ) ;
#46938=CARTESIAN_POINT ( 'NONE',  ( -18.57053249869930056, 1415.834070658489964, 207.5706722826859902 ) ) ;
#46940=FACE_OUTER_BOUND ( 'NONE', #92415, .T. ) ;
#46941=CARTESIAN_POINT ( 'NONE',  ( 12.44601730950000018, 1416.547221147930031, 223.4678929843980200 ) ) ;
#46944=ORIENTED_EDGE ( 'NONE', *, *, #15820, .F. ) ;
#46945=CARTESIAN_POINT ( 'NONE',  ( -42.60628463920510001, 1443.705283414160021, 135.0584851923260032 ) ) ;
#46947=ORIENTED_EDGE ( 'NONE', *, *, #26073, .T. ) ;
#46948=CARTESIAN_POINT ( 'NONE',  ( 5.997518064628799550, 1456.982253578982636, 228.0100344516387736 ) ) ;
#46949=CARTESIAN_POINT ( 'NONE',  ( 24.60314935906709621, 1451.898314952959936, 137.0370639567690034 ) ) ;
#46950=CARTESIAN_POINT ( 'NONE',  ( -4.130945703660738211, 1439.900949266221915, 185.4738977992453215 ) ) ;
#46952=CARTESIAN_POINT ( 'NONE',  ( 21.82631551119999713, 1410.169362862829985, 203.3225918027780210 ) ) ;
#46953=CARTESIAN_POINT ( 'NONE',  ( -2.500000000000000000, 1448.210448412289907, 170.5244215879980061 ) ) ;
#46954=CARTESIAN_POINT ( 'NONE',  ( 17.28479430970000053, 1410.440253690029976, 225.9720111249980050 ) ) ;
#46957=CARTESIAN_POINT ( 'NONE',  ( 21.42399653786173630, 1453.892630570952861, 221.3230395484720532 ) ) ;
#46962=CARTESIAN_POINT ( 'NONE',  ( -10.97762738589999998, 1473.214251705830065, 270.1116084939980055 ) ) ;
#46963=CARTESIAN_POINT ( 'NONE',  ( -2.500000000000000000, 1448.235640331100058, 183.7014620552980091 ) ) ;
#46964=CARTESIAN_POINT ( 'NONE',  ( 2.320368942857389871E-14, 1422.005500615010078, 112.3240825799360039 ) ) ;
#46965=CARTESIAN_POINT ( 'NONE',  ( -40.26206638547280647, 1444.220281762339937, 137.0954650734020106 ) ) ;
#46966=CARTESIAN_POINT ( 'NONE',  ( 11.60004869885212919, 1425.574822748529868, 138.2968742054259508 ) ) ;
#46968=CARTESIAN_POINT ( 'NONE',  ( -1.912619103278670130, 1484.245594002130019, 182.9331903370400028 ) ) ;
#46969=CARTESIAN_POINT ( 'NONE',  ( 11.13831797289999948, 1433.014992880049931, 151.6441518879979924 ) ) ;
#46970=CARTESIAN_POINT ( 'NONE',  ( -44.68916218182129541, 1444.637905724729990, 269.6957224876979922 ) ) ;
#46971=CARTESIAN_POINT ( 'NONE',  ( 27.93016292933110023, 1440.913060387420046, 230.8733152401279938 ) ) ;
#46972=CARTESIAN_POINT ( 'NONE',  ( -20.00075399880000049, 1508.017360025530024, 229.1239405492979984 ) ) ;
#46974=ORIENTED_EDGE ( 'NONE', *, *, #24147, .T. ) ;
#46975=CARTESIAN_POINT ( 'NONE',  ( 11.23388613411650638, 1445.063428794548372, 207.0699376370758955 ) ) ;
#46977=CARTESIAN_POINT ( 'NONE',  ( -0.8732732019916324973, 1409.114783162738604, 186.1304715542366353 ) ) ;
#46981=CARTESIAN_POINT ( 'NONE',  ( -16.27856158940000242, 1509.481520284230101, 232.7807208966979999 ) ) ;
#46984=CARTESIAN_POINT ( 'NONE',  ( 6.688848995729999913, 1408.965348139829985, 221.4809136123979840 ) ) ;
#46985=DIRECTION ( 'NONE',  ( -1.989694733329999956E-13, -6.948167114159990914E-15, 1.000000000000000000 ) ) ;
#46986=CARTESIAN_POINT ( 'NONE',  ( 2.872763937410000246, 1464.652692451630173, 236.7382212475980054 ) ) ;
#46989=CARTESIAN_POINT ( 'NONE',  ( -0.8784639586519999988, 1452.142747003829982, 183.3918967091979937 ) ) ;
#46993=CARTESIAN_POINT ( 'NONE',  ( -16.38929703815969674, 1414.913060387399810, 208.0943756141269887 ) ) ;
#46996=ORIENTED_EDGE ( 'NONE', *, *, #4863, .T. ) ;
#46998=LINE ( 'NONE', #106870, #46235 ) ;
#47001=CARTESIAN_POINT ( 'NONE',  ( -15.33708062616911327, 1509.448643044570190, 233.9107056133578340 ) ) ;
#47003=CARTESIAN_POINT ( 'NONE',  ( 11.05349294225439927, 1409.299056866449973, 199.0526579458750120 ) ) ;
#47004=CYLINDRICAL_SURFACE ( 'NONE', #77711, 0.5000000000000379696 ) ;
#47006=CARTESIAN_POINT ( 'NONE',  ( -18.67323663170000003, 1463.212872143629966, 190.4754105328979961 ) ) ;
#47008=CARTESIAN_POINT ( 'NONE',  ( -17.14944456869280032, 1460.835971333450061, 230.2708732161399894 ) ) ;
#47011=ORIENTED_EDGE ( 'NONE', *, *, #104411, .T. ) ;
#47013=CARTESIAN_POINT ( 'NONE',  ( -12.24150297201249948, 1416.512142030569976, 194.6918193283640051 ) ) ;
#47014=B_SPLINE_CURVE_WITH_KNOTS ( 'NONE', 5,
 ( #108135, #102888, #99722, #57219, #8285, #48813 ),
 .UNSPECIFIED., .F., .F.,
 ( 6, 6 ),
 ( 0.000000000000000000, 1.000000000000000000 ),
 .UNSPECIFIED. ) ;
#47015=CARTESIAN_POINT ( 'NONE',  ( -12.06918120999999999, 1434.098677319379931, 150.5974712778979949 ) ) ;
#47016=CARTESIAN_POINT ( 'NONE',  ( -7.982875717626110139E-10, 1468.280901364470083, 249.1209479164010077 ) ) ;
#47017=CARTESIAN_POINT ( 'NONE',  ( -20.55923624469150113, 1506.544472774470023, 190.4275880989339953 ) ) ;
#47018=FACE_OUTER_BOUND ( 'NONE', #88433, .T. ) ;
#47020=CARTESIAN_POINT ( 'NONE',  ( -19.27069311609591651, 1486.269147065019297, 189.5747608116244578 ) ) ;
#47023=B_SPLINE_CURVE_WITH_KNOTS ( 'NONE', 3,
 ( #110799, #35756, #43610, #25674, #93992, #43059, #60422, #59324, #94539, #18927, #110242, #42491, #34090, #52569, #51449, #86703, #102391, #25119, #93435, #52012, #9996, #86154, #16704, #85582, #44167, #50905, #520, #34645, #77760, #69384, #85036, #101826, #69940, #78304, #59866, #8877, #68829, #102930, #103494, #27346 ),
 .UNSPECIFIED., .F., .F.,
 ( 4, 3, 3, 3, 3, 3, 3, 3, 3, 3, 3, 3, 3, 4 ),
 ( -167.7881597174699948, -162.0210453901829908, -153.2885860985529973, -144.2037312555439996, -134.8360698329800016, -124.8049311414389990, -114.1011191363109987, -102.2819146078059873, -87.23193074669060820, -72.32291041643570395, -60.59518579591799892, -49.91975445303839365, -39.91025693460328228, -30.37891568121239061 ),
 .UNSPECIFIED. ) ;
#47026=CARTESIAN_POINT ( 'NONE',  ( 2.522951803030079727E-08, 1397.914279477030050, 222.1218461579910297 ) ) ;
#47027=CARTESIAN_POINT ( 'NONE',  ( -13.10408799755770026, 1435.790188770230088, 150.6193508587029726 ) ) ;
#47029=ADVANCED_FACE ( 'NONE', ( #38231 ), #70470, .F. ) ;
#47030=CARTESIAN_POINT ( 'NONE',  ( 0.9042083405910000815, 1416.833018152729892, 190.2143527203979829 ) ) ;
#47031=CARTESIAN_POINT ( 'NONE',  ( 20.13590845398709916, 1492.832540254449896, 227.2160562042610081 ) ) ;
#47032=DIRECTION ( 'NONE',  ( -0.8023110876747339137, -0.5969061220947440294, 0.000000000000000000 ) ) ;
#47034=CARTESIAN_POINT ( 'NONE',  ( 31.20802388339999922, 1430.369980854530013, 248.1710554639980160 ) ) ;
#47036=CARTESIAN_POINT ( 'NONE',  ( -10.36174392853389925, 1425.413733281229952, 93.54415789945380766 ) ) ;
#47037=CARTESIAN_POINT ( 'NONE',  ( 17.33645362950000290, 1414.996442546130083, 210.3925741896480304 ) ) ;
#47038=EDGE_CURVE ( 'NONE', #68340, #5427, #16339, .T. ) ;
#47039=CARTESIAN_POINT ( 'NONE',  ( -40.61001291052744477, 1425.241084799366718, 269.7704882069099313 ) ) ;
#47040=CARTESIAN_POINT ( 'NONE',  ( -24.78057548010000133, 1437.622990999089780, 216.3901361313880329 ) ) ;
#47041=CARTESIAN_POINT ( 'NONE',  ( 20.08696296560329841, 1509.650477513600208, 231.0046925456110216 ) ) ;
#47043=CARTESIAN_POINT ( 'NONE',  ( 27.03406173819999836, 1451.512718515130018, 136.1495732049980063 ) ) ;
#47044=ORIENTED_EDGE ( 'NONE', *, *, #99580, .F. ) ;
#47047=CARTESIAN_POINT ( 'NONE',  ( 8.835340541969999961, 1509.234990883429873, 237.6028457034980192 ) ) ;
#47050=CARTESIAN_POINT ( 'NONE',  ( -10.10004869884733125, 1422.222932908416851, 137.0999999980979851 ) ) ;
#47051=CARTESIAN_POINT ( 'NONE',  ( -24.06078745206859892, 1410.858125197970139, 208.6187097067000025 ) ) ;
#47055=CARTESIAN_POINT ( 'NONE',  ( -13.30975985100000081, 1479.764766878030059, 231.2919490532979978 ) ) ;
#47058=DIRECTION ( 'NONE',  ( -0.08338001035890203749, 1.207410962451694502E-12, -0.9965178241619914168 ) ) ;
#47060=CARTESIAN_POINT ( 'NONE',  ( 14.07846764309999976, 1463.781906650229985, 224.7807885173980367 ) ) ;
#47063=CARTESIAN_POINT ( 'NONE',  ( -4.500000000000000000, 1426.966631815929986, 170.4008037693979816 ) ) ;
#47064=CARTESIAN_POINT ( 'NONE',  ( 12.58023385476424494, 1442.780465393927670, 186.4880924237379247 ) ) ;
#47065=ORIENTED_EDGE ( 'NONE', *, *, #10083, .F. ) ;
#47066=ORIENTED_EDGE ( 'NONE', *, *, #49612, .F. ) ;
#47069=CARTESIAN_POINT ( 'NONE',  ( 12.76760079159999961, 1508.356069781229962, 233.5455612081979950 ) ) ;
#47071=CARTESIAN_POINT ( 'NONE',  ( 13.23745870105759970, 1452.450798143380098, 148.9949343981280094 ) ) ;
#47075=CARTESIAN_POINT ( 'NONE',  ( -11.58636794539999926, 1433.009610086610110, 151.1946776885979773 ) ) ;
#47076=CARTESIAN_POINT ( 'NONE',  ( 0.03406326677807396813, 1410.027273331433889, 233.1845275417764469 ) ) ;
#47077=CARTESIAN_POINT ( 'NONE',  ( -16.80801311784789931, 1415.384652614329980, 191.6111484580369790 ) ) ;
#47080=B_SPLINE_CURVE_WITH_KNOTS ( 'NONE', 5,
 ( #84916, #93869, #65955, #48597, #82731, #100080 ),
 .UNSPECIFIED., .F., .F.,
 ( 6, 6 ),
 ( -15.04427212800000113, -3.432284964179999065 ),
 .UNSPECIFIED. ) ;
#47084=CARTESIAN_POINT ( 'NONE',  ( 12.22219588455229911, 1415.434635989089884, 222.2791104031980183 ) ) ;
#47085=CYLINDRICAL_SURFACE ( 'NONE', #90962, 2.000000000000000000 ) ;
#47092=CARTESIAN_POINT ( 'NONE',  ( -2.596326248400549819, 1439.736080710940087, 157.6563194317720047 ) ) ;
#47096=CARTESIAN_POINT ( 'NONE',  ( 13.00574619272959964, 1416.230844595159851, 196.4148928853770144 ) ) ;
#47098=FACE_OUTER_BOUND ( 'NONE', #5185, .T. ) ;
#47099=CARTESIAN_POINT ( 'NONE',  ( 14.73464909550000002, 1422.105278128630061, 228.1938737527979697 ) ) ;
#47100=B_SPLINE_CURVE_WITH_KNOTS ( 'NONE', 5,
 ( #101161, #50784, #99510, #49148, #67602, #40727, #92777, #16052, #58098, #91678, #15500, #74900 ),
 .UNSPECIFIED., .F., .F.,
 ( 6, 3, 3, 6 ),
 ( 13.03551675900000006, 13.93909308159999938, 15.74624572679999979, 17.56231401080000154 ),
 .UNSPECIFIED. ) ;
#47103=CARTESIAN_POINT ( 'NONE',  ( 45.11781237659999277, 1434.982694580879979, 266.2041965131979850 ) ) ;
#47104=CARTESIAN_POINT ( 'NONE',  ( -17.46956007389999854, 1409.523110867929972, 223.7310521786980075 ) ) ;
#47105=CARTESIAN_POINT ( 'NONE',  ( 16.25264133110000131, 1436.302628333469784, 148.7774457700980122 ) ) ;
#47106=CARTESIAN_POINT ( 'NONE',  ( -0.9041356904339998835, 1416.839648772129976, 228.0296119443979990 ) ) ;
#47107=CARTESIAN_POINT ( 'NONE',  ( 29.53677856842397631, 1509.959383199721287, 207.3087542667464618 ) ) ;
#47108=CARTESIAN_POINT ( 'NONE',  ( -1.770636241409999867, 1475.812198116930176, 266.9599394754979471 ) ) ;
#47111=CARTESIAN_POINT ( 'NONE',  ( -40.33412369041069923, 1439.452808492470012, 136.1315416014939785 ) ) ;
#47113=CARTESIAN_POINT ( 'NONE',  ( -8.786848204050000888, 1409.039826487530036, 220.7305139779979868 ) ) ;
#47114=CARTESIAN_POINT ( 'NONE',  ( -15.87297696440000117, 1415.931391677429929, 200.7186373451680197 ) ) ;
#47117=CARTESIAN_POINT ( 'NONE',  ( 12.06124454959999959, 1433.903398563020119, 147.6243995897980028 ) ) ;
#47118=DIRECTION ( 'NONE',  ( 0.1402804634180439824, 0.9901118076173108795, -3.469446951951086598E-18 ) ) ;
#47119=CARTESIAN_POINT ( 'NONE',  ( 4.219438956540000341, 1441.595895961080259, 182.7715286933980110 ) ) ;
#47122=CARTESIAN_POINT ( 'NONE',  ( 26.96383586069999794, 1437.662818847919880, 136.8825122631980094 ) ) ;
#47125=CARTESIAN_POINT ( 'NONE',  ( -14.67313656458610005, 1477.920145184079956, 193.6164693688140233 ) ) ;
#47126=CARTESIAN_POINT ( 'NONE',  ( -45.85459127630000609, 1440.913039247130200, 268.7562765203980462 ) ) ;
#47130=B_SPLINE_SURFACE_WITH_KNOTS ( 'NONE', 3, 5, ( 
 ( #88890, #54217, #87808, #11633, #71023, #79395 ),
 ( #106242, #21107, #10527, #97828, #105710, #88342 ),
 ( #72654, #2159, #71589, #62633, #106781, #54760 ),
 ( #3818, #2709, #28992, #87238, #36276, #55308 ) ),
 .UNSPECIFIED., .F., .F., .F.,
 ( 4, 4 ),
 ( 6, 6 ),
 ( 0.000000000000000000, 0.07116409211490000442 ),
 ( 0.000000000000000000, 2.000000000000000000 ),
 .UNSPECIFIED. ) ;
#47133=CARTESIAN_POINT ( 'NONE',  ( -26.80425739744236679, 1436.404103241545272, 136.7059128651563924 ) ) ;
#47134=CARTESIAN_POINT ( 'NONE',  ( -27.79584127320000420, 1451.487053449729956, 136.1260449201980123 ) ) ;
#47136=ADVANCED_FACE ( 'NONE', ( #48868 ), #7176, .F. ) ;
#47138=ORIENTED_EDGE ( 'NONE', *, *, #102233, .T. ) ;
#47140=CARTESIAN_POINT ( 'NONE',  ( -24.00439558080000069, 1410.673376339430206, 208.3492520220979998 ) ) ;
#47142=CARTESIAN_POINT ( 'NONE',  ( -12.07588402680000073, 1415.579607678529783, 195.0757015091980122 ) ) ;
#47145=CARTESIAN_POINT ( 'NONE',  ( 22.76066440079999609, 1410.202971864430083, 213.5588159894880107 ) ) ;
#47148=CARTESIAN_POINT ( 'NONE',  ( -3.666694481987490040, 1509.114858341099989, 179.5219341129400163 ) ) ;
#47149=CARTESIAN_POINT ( 'NONE',  ( 19.75084982879439721, 1455.504334177440114, 226.5702129464319796 ) ) ;
#47151=CARTESIAN_POINT ( 'NONE',  ( 25.74606117743979894, 1449.914928376210128, 209.5154968510050253 ) ) ;
#47154=CARTESIAN_POINT ( 'NONE',  ( -0.6609304440939999248, 1417.306157093830052, 234.7827881003979940 ) ) ;
#47157=CARTESIAN_POINT ( 'NONE',  ( -11.30203360114940025, 1485.177505568769902, 185.2631062660830139 ) ) ;
#47160=CARTESIAN_POINT ( 'NONE',  ( 17.40764059099999628, 1414.996444526030018, 210.6782161193179945 ) ) ;
#47164=CARTESIAN_POINT ( 'NONE',  ( 29.25495334450000229, 1509.872415968330188, 209.6024640478379979 ) ) ;
#47165=ORIENTED_EDGE ( 'NONE', *, *, #64430, .F. ) ;
#47166=CARTESIAN_POINT ( 'NONE',  ( 6.811012380346902262, 1507.262579170454046, 182.5160571386342951 ) ) ;
#47168=CARTESIAN_POINT ( 'NONE',  ( 15.90371042334150253, 1418.365809420349933, 191.2849450763380048 ) ) ;
#47171=CARTESIAN_POINT ( 'NONE',  ( -24.63384085366289966, 1451.895538293800200, 136.9985731684789982 ) ) ;
#47173=CARTESIAN_POINT ( 'NONE',  ( 13.25587788500000030, 1409.542715034829826, 227.8021890157979783 ) ) ;
#47176=CARTESIAN_POINT ( 'NONE',  ( 41.65974987187789935, 1443.430997017130267, 134.0999999981650035 ) ) ;
#47177=CARTESIAN_POINT ( 'NONE',  ( -18.70459388414779767, 1509.566239243649989, 231.7064163625079800 ) ) ;
#47180=ORIENTED_EDGE ( 'NONE', *, *, #101841, .F. ) ;
#47188=B_SPLINE_CURVE_WITH_KNOTS ( 'NONE', 5,
 ( #16115, #467, #7733, #51395, #34591, #9394 ),
 .UNSPECIFIED., .F., .F.,
 ( 6, 6 ),
 ( -20.59614117366909980, -15.24393013793890006 ),
 .UNSPECIFIED. ) ;
#47190=CARTESIAN_POINT ( 'NONE',  ( -16.83328027291899076, 1449.459041290944015, 219.8226804865572603 ) ) ;
#47193=CARTESIAN_POINT ( 'NONE',  ( 28.27265630610000002, 1508.146186351229971, 209.2480474313609875 ) ) ;
#47194=CARTESIAN_POINT ( 'NONE',  ( 5.414687584439999313, 1414.913060387329779, 193.6792642988980049 ) ) ;
#47196=ORIENTED_EDGE ( 'NONE', *, *, #44079, .T. ) ;
#47198=ORIENTED_EDGE ( 'NONE', *, *, #90389, .T. ) ;
#47200=CARTESIAN_POINT ( 'NONE',  ( 19.06412006440000084, 1467.189854735629979, 227.5855243549980287 ) ) ;
#47202=CARTESIAN_POINT ( 'NONE',  ( -0.1489371451341119923, 1450.907859387619965, 181.8882210233129797 ) ) ;
#47207=AXIS2_PLACEMENT_3D ( 'NONE', #32304, #66487, #74330 ) ;
#47209=CARTESIAN_POINT ( 'NONE',  ( 41.16455037149999896, 1425.337515733230020, 266.3184770345980041 ) ) ;
#47212=CARTESIAN_POINT ( 'NONE',  ( 2.805385066259999949, 1465.548011742730296, 234.3643945938979982 ) ) ;
#47213=CARTESIAN_POINT ( 'NONE',  ( -11.60004869885203682, 1422.586144007987514, 135.6000000023773282 ) ) ;
#47216=CARTESIAN_POINT ( 'NONE',  ( -0.1497422254867110114, 1507.486086595969937, 180.8511887974889873 ) ) ;
#47219=EDGE_CURVE ( 'NONE', #33927, #82900, #64142, .T. ) ;
#47220=CARTESIAN_POINT ( 'NONE',  ( -19.67719249089999778, 1452.817890304729872, 209.2087704682629976 ) ) ;
#47224=CARTESIAN_POINT ( 'NONE',  ( -20.06869840700000296, 1507.849569109330105, 229.0200580499979992 ) ) ;
#47225=CARTESIAN_POINT ( 'NONE',  ( 1.343386335820000024E-08, 1460.517119006129860, 217.3476459701080046 ) ) ;
#47226=CARTESIAN_POINT ( 'NONE',  ( -11.29459831670000014, 1431.803823149859909, 151.5027742212979831 ) ) ;
#47229=CARTESIAN_POINT ( 'NONE',  ( 5.106122016996108570, 1414.913060387329779, 193.4216302945174562 ) ) ;
#47232=CARTESIAN_POINT ( 'NONE',  ( -18.65643340519999782, 1444.808185763539996, 226.4043360155980054 ) ) ;
#47233=CARTESIAN_POINT ( 'NONE',  ( 5.368321057878550739, 1426.798736626489926, 152.9345200458829765 ) ) ;
#47234=CARTESIAN_POINT ( 'NONE',  ( -0.2223819995240000069, 1416.825245919230156, 191.0547458884979903 ) ) ;
#47237=CARTESIAN_POINT ( 'NONE',  ( 0.5588755390740001161, 1405.778268568529938, 268.4836505046980051 ) ) ;
#47239=CARTESIAN_POINT ( 'NONE',  ( 24.17267386829139753, 1436.406449779874038, 213.4172145310692201 ) ) ;
#47240=CARTESIAN_POINT ( 'NONE',  ( -25.74086641750000126, 1452.014152722630115, 135.1060044590980169 ) ) ;
#47241=CARTESIAN_POINT ( 'NONE',  ( 11.60004869885203682, 1424.621838078508063, 136.2521644537905559 ) ) ;
#47242=CARTESIAN_POINT ( 'NONE',  ( 4.219439031349260461, 1446.230224802979819, 182.3842141579679890 ) ) ;
#47244=CARTESIAN_POINT ( 'NONE',  ( -2.500290412864679901, 1448.931711032029853, 154.7923269189249993 ) ) ;
#47246=CARTESIAN_POINT ( 'NONE',  ( -19.83769288353390436, 1485.661834359392060, 190.4830555484894887 ) ) ;
#47247=CARTESIAN_POINT ( 'NONE',  ( -13.49369408200810128, 1415.034069327400175, 220.4142464946930033 ) ) ;
#47250=CARTESIAN_POINT ( 'NONE',  ( -14.73695825179999908, 1419.186926028530252, 255.3819207742980097 ) ) ;
#47252=CARTESIAN_POINT ( 'NONE',  ( 11.02688339341326440, 1425.203200046631764, 139.1360293941474993 ) ) ;
#47253=CARTESIAN_POINT ( 'NONE',  ( 4.221259200859999616, 1441.605854689579928, 166.9080625328979863 ) ) ;
#47254=CARTESIAN_POINT ( 'NONE',  ( -0.5546426699349999989, 1475.558885421630066, 269.2946135826979912 ) ) ;
#47260=LINE ( 'NONE', #81383, #103936 ) ;
#47261=B_SPLINE_SURFACE_WITH_KNOTS ( 'NONE', 5, 3, ( 
 ( #49049, #83186, #51233, #6475 ),
 ( #40625, #74796, #32229, #66409 ),
 ( #23806, #79214, #34432, #43945 ),
 ( #87611, #306, #851, #52365 ),
 ( #19262, #1391, #68605, #53465 ),
 ( #34978, #60201, #78088, #85937 ) ),
 .UNSPECIFIED., .F., .F., .F.,
 ( 6, 6 ),
 ( 4, 4 ),
 ( 0.000000000000000000, 11.48858425020000062 ),
 ( 37.69911184309999896, 40.20365518519999881 ),
 .UNSPECIFIED. ) ;
#47265=CARTESIAN_POINT ( 'NONE',  ( -10.41617235030460087, 1396.276801140979842, 212.8667543991859930 ) ) ;
#47266=CARTESIAN_POINT ( 'NONE',  ( -14.46798390520000055, 1422.172973043230058, 228.7514975090980158 ) ) ;
#47267=CARTESIAN_POINT ( 'NONE',  ( 19.28094568327996683, 1456.010430125557605, 225.1773291266683827 ) ) ;
#47270=CARTESIAN_POINT ( 'NONE',  ( -13.86092847646930082, 1410.765486861110048, 227.1170286572800023 ) ) ;
#47273=CARTESIAN_POINT ( 'NONE',  ( 10.44233456949999983, 1425.120996158829939, 121.0077805707980048 ) ) ;
#47275=CARTESIAN_POINT ( 'NONE',  ( 11.71230443242549057, 1428.980197708463947, 142.1750151601943912 ) ) ;
#47279=CARTESIAN_POINT ( 'NONE',  ( -11.81707110430000007, 1430.266231075130008, 147.2485970657980090 ) ) ;
#47280=CARTESIAN_POINT ( 'NONE',  ( 7.193668918159999315, 1509.090620986230078, 181.2520380256979990 ) ) ;
#47281=CARTESIAN_POINT ( 'NONE',  ( -21.33070998724348755, 1509.431296620148714, 190.3921826398929795 ) ) ;
#47284=CARTESIAN_POINT ( 'NONE',  ( 16.06273934902591094, 1410.858425379293749, 191.5167191839988163 ) ) ;
#47287=CARTESIAN_POINT ( 'NONE',  ( -12.03082380390000061, 1397.656013067930189, 203.3051016873779986 ) ) ;
#47288=CARTESIAN_POINT ( 'NONE',  ( 2.918579238077160021, 1409.742862551950111, 231.4428086086070095 ) ) ;
#47290=CARTESIAN_POINT ( 'NONE',  ( -12.79393335520562225, 1444.983108077871066, 169.4500695159219106 ) ) ;
#47291=CARTESIAN_POINT ( 'NONE',  ( -23.61227025210000008, 1435.322036687620084, 137.2858276859979867 ) ) ;
#47297=CARTESIAN_POINT ( 'NONE',  ( -41.27932424117140187, 1445.656587030789979, 136.3077099605269780 ) ) ;
#47298=CARTESIAN_POINT ( 'NONE',  ( 10.17615046018800129, 1396.268419396740001, 204.7703056290459926 ) ) ;
#47299=FACE_OUTER_BOUND ( 'NONE', #57601, .T. ) ;
#47300=CARTESIAN_POINT ( 'NONE',  ( 11.65217179949999959, 1425.851026166929842, 145.3825519544979841 ) ) ;
#47301=CARTESIAN_POINT ( 'NONE',  ( 41.65883123370000618, 1443.939564121179956, 136.1335272508979983 ) ) ;
#47302=EDGE_LOOP ( 'NONE', ( #32160, #27178, #39754, #4721 ) ) ;
#47303=CARTESIAN_POINT ( 'NONE',  ( 4.091329073579999864, 1425.301743040829933, 185.3866542801980017 ) ) ;
#47304=CARTESIAN_POINT ( 'NONE',  ( 12.45988844690000086, 1442.668228039740143, 187.1806564808980227 ) ) ;
#47308=CARTESIAN_POINT ( 'NONE',  ( -17.46087120122630054, 1458.256338415900018, 228.1902854820540085 ) ) ;
#47309=CARTESIAN_POINT ( 'NONE',  ( -14.35945310470000180, 1461.065408120830170, 229.7470706200979862 ) ) ;
#47310=CARTESIAN_POINT ( 'NONE',  ( -17.03290348309940683, 1409.881251522323964, 225.5427118406987006 ) ) ;
#47311=CARTESIAN_POINT ( 'NONE',  ( 12.61812115829999925, 1416.825245919230156, 196.1892291636980019 ) ) ;
#47314=ORIENTED_EDGE ( 'NONE', *, *, #85613, .F. ) ;
#47316=CARTESIAN_POINT ( 'NONE',  ( 0.05162197306659999790, 1509.009019568429949, 179.2212271949979936 ) ) ;
#47321=CARTESIAN_POINT ( 'NONE',  ( -19.97699668690000152, 1508.102459366529956, 229.1407657077979820 ) ) ;
#47322=CARTESIAN_POINT ( 'NONE',  ( -21.90170135886932457, 1414.871184935607744, 269.4017551159469690 ) ) ;
#47323=CARTESIAN_POINT ( 'NONE',  ( -0.4274081085919999579, 1409.096031296729961, 232.6209005452979852 ) ) ;
#47324=DIRECTION ( 'NONE',  ( -1.000000000000000000, 0.000000000000000000, 0.000000000000000000 ) ) ;
#47326=CARTESIAN_POINT ( 'NONE',  ( 2.500000000000000000, 1424.377232884329942, 154.7346221771979913 ) ) ;
#47327=CARTESIAN_POINT ( 'NONE',  ( -31.04776337085569793, 1440.913060388089889, 241.5191150371310016 ) ) ;
#47330=CARTESIAN_POINT ( 'NONE',  ( -0.1879632238746349882, 1466.387553677260030, 235.6886251357990147 ) ) ;
#47331=CARTESIAN_POINT ( 'NONE',  ( 27.66281618764540084, 1417.733632362909930, 269.4444038297550037 ) ) ;
#47335=CARTESIAN_POINT ( 'NONE',  ( 23.08676684170000115, 1409.825010724229969, 208.4789857369090100 ) ) ;
#47336=CARTESIAN_POINT ( 'NONE',  ( 0.02089856015480650100, 1507.111761549349922, 237.3522809668369860 ) ) ;
#47339=ADVANCED_FACE ( 'NONE', ( #37550 ), #70636, .T. ) ;
#47341=EDGE_CURVE ( 'NONE', #90450, #61502, #6828, .T. ) ;
#47342=CARTESIAN_POINT ( 'NONE',  ( 4.401092417150000102, 1420.174153566729956, 185.7217845719979721 ) ) ;
#47344=EDGE_CURVE ( 'NONE', #78256, #100339, #105201, .T. ) ;
#47345=EDGE_LOOP ( 'NONE', ( #25121, #99579, #103285, #60785 ) ) ;
#47347=CARTESIAN_POINT ( 'NONE',  ( 18.90720652019999903, 1416.826388498430106, 210.0261622758970077 ) ) ;
#47349=CARTESIAN_POINT ( 'NONE',  ( 0.2257619562299999771, 1417.282465340730141, 234.8473851690980041 ) ) ;
#47350=EDGE_CURVE ( 'NONE', #27144, #10158, #3315, .T. ) ;
#47351=B_SPLINE_SURFACE_WITH_KNOTS ( 'NONE', 5, 5, ( 
 ( #26467, #67406, #17495, #92566, #58997, #101504 ),
 ( #85834, #66853, #43297, #34877, #60662, #18064 ),
 ( #100962, #44967, #29243, #52806, #11895, #71848 ),
 ( #28137, #63433, #95345, #43842, #103743, #95895 ),
 ( #70188, #18607, #53932, #46068, #97550, #77988 ),
 ( #104297, #52258, #71291, #79666, #2970, #37088 ) ),
 .UNSPECIFIED., .F., .F., .F.,
 ( 6, 6 ),
 ( 6, 6 ),
 ( 3.274326487366419958, 6.007249690403580367 ),
 ( -2.359960357783379966E-05, 2.000000000000000000 ),
 .UNSPECIFIED. ) ;
#47352=FACE_OUTER_BOUND ( 'NONE', #17164, .T. ) ;
#47353=LINE ( 'NONE', #96658, #16875 ) ;
#47358=CARTESIAN_POINT ( 'NONE',  ( 18.16418870590809931, 1416.835419214280137, 209.1673351295509917 ) ) ;
#47359=CARTESIAN_POINT ( 'NONE',  ( -25.59985477246175378, 1450.799230641226586, 137.0693086342491256 ) ) ;
#47363=DIRECTION ( 'NONE',  ( 0.3282391760791589785, -0.000000000000000000, 0.9445946449598763284 ) ) ;
#47366=AXIS2_PLACEMENT_3D ( 'NONE', #5984, #88473, #107885 ) ;
#47367=CARTESIAN_POINT ( 'NONE',  ( 20.63648295220000151, 1455.268815933329961, 222.7070109917980290 ) ) ;
#47372=CARTESIAN_POINT ( 'NONE',  ( -28.01951961465029939, 1509.887603853479959, 200.8921116242010214 ) ) ;
#47374=CARTESIAN_POINT ( 'NONE',  ( -19.28416521189999955, 1426.095206623730064, 225.9565170197979853 ) ) ;
#47375=CARTESIAN_POINT ( 'NONE',  ( -29.59241942509761003, 1466.933728989316251, 269.3641340189501534 ) ) ;
#47377=FACE_OUTER_BOUND ( 'NONE', #7043, .T. ) ;
#47379=CARTESIAN_POINT ( 'NONE',  ( 28.27265630610000002, 1508.146186351229971, 209.2480474313609875 ) ) ;
#47384=VERTEX_POINT ( 'NONE', #25131 ) ;
#47385=DIRECTION ( 'NONE',  ( -0.0001837273416260859385, 0.9990401814439695549, 0.04380276366468503074 ) ) ;
#47390=CARTESIAN_POINT ( 'NONE',  ( -13.22806383169999833, 1431.113060387329824, 222.3499097936980036 ) ) ;
#47393=CARTESIAN_POINT ( 'NONE',  ( -12.65578976995832861, 1442.797870648871594, 186.1192285427375737 ) ) ;
#47395=CARTESIAN_POINT ( 'NONE',  ( -16.81223226430000039, 1414.913060387329779, 207.5743821216680089 ) ) ;
#47396=DIRECTION ( 'NONE',  ( 1.000000000000000000, 0.000000000000000000, 0.000000000000000000 ) ) ;
#47397=ADVANCED_FACE ( 'NONE', ( #84503 ), #41413, .F. ) ;
#47398=CARTESIAN_POINT ( 'NONE',  ( -7.798516306275617538, 1417.059749218360821, 231.0301366618491272 ) ) ;
#47399=CARTESIAN_POINT ( 'NONE',  ( -5.623474965688048840E-07, 1451.660737107639989, 154.0815186765750013 ) ) ;
#47400=CARTESIAN_POINT ( 'NONE',  ( 18.59804234570002279, 1425.273062378426175, 226.9839929844980304 ) ) ;
#47408=CARTESIAN_POINT ( 'NONE',  ( 16.88248175295160181, 1414.913057834419988, 210.3124741370610025 ) ) ;
#47409=CARTESIAN_POINT ( 'NONE',  ( 13.94913730080000036, 1509.400263820630016, 234.9268341509979905 ) ) ;
#47411=CARTESIAN_POINT ( 'NONE',  ( 34.75159598319835652, 1423.783191157365536, 269.5281025998144742 ) ) ;
#47412=CARTESIAN_POINT ( 'NONE',  ( -21.00608537319999769, 1461.014378767029939, 244.4374624616980043 ) ) ;
#47414=CARTESIAN_POINT ( 'NONE',  ( -20.40938849349999984, 1503.704554046830026, 189.8792483973980154 ) ) ;
#47415=CARTESIAN_POINT ( 'NONE',  ( -11.89389463660000068, 1433.576802385009842, 150.4827622296980110 ) ) ;
#47417=CARTESIAN_POINT ( 'NONE',  ( 11.68805093410779961, 1426.728226893330202, 140.6662312984289827 ) ) ;
#47418=CARTESIAN_POINT ( 'NONE',  ( 27.51968813986070117, 1491.156149288490042, 209.4200479053579897 ) ) ;
#47419=CARTESIAN_POINT ( 'NONE',  ( -1.356522590142140050, 1410.335674017130032, 185.6037846924129724 ) ) ;
#47426=CARTESIAN_POINT ( 'NONE',  ( 5.857070821897849958E-09, 1409.867647545549971, 258.8986024302779470 ) ) ;
#47428=ORIENTED_EDGE ( 'NONE', *, *, #11795, .F. ) ;
#47431=CARTESIAN_POINT ( 'NONE',  ( -25.02521468490000345, 1466.386952600029872, 270.1035466365980255 ) ) ;
#47432=CARTESIAN_POINT ( 'NONE',  ( -1.547118986179999878, 1416.568813549730066, 228.0093688194979791 ) ) ;
#47433=DIRECTION ( 'NONE',  ( 0.000000000000000000, 0.000000000000000000, -1.000000000000000000 ) ) ;
#47434=CARTESIAN_POINT ( 'NONE',  ( 35.18816452081259882, 1451.157525408279980, 135.9224998729500271 ) ) ;
#47437=CARTESIAN_POINT ( 'NONE',  ( 21.92444878912329997, 1509.678679009930192, 227.6602567754504491 ) ) ;
#47440=CARTESIAN_POINT ( 'NONE',  ( -33.19754209624489505, 1417.174461616820054, 269.2945989659730230 ) ) ;
#47441=ORIENTED_EDGE ( 'NONE', *, *, #85145, .T. ) ;
#47446=EDGE_CURVE ( 'NONE', #90113, #7633, #7793, .T. ) ;
#47447=CARTESIAN_POINT ( 'NONE',  ( 17.22592475669603473, 1444.324653571829685, 162.9227486557985003 ) ) ;
#47450=CARTESIAN_POINT ( 'NONE',  ( -17.78468008800000177, 1440.443143732879889, 191.0126434879979911 ) ) ;
#47451=CARTESIAN_POINT ( 'NONE',  ( -18.63578313170000200, 1416.568813547830132, 208.5538819738139864 ) ) ;
#47453=CARTESIAN_POINT ( 'NONE',  ( -26.64894350899999864, 1436.272083837089895, 136.6568872077980075 ) ) ;
#47461=CARTESIAN_POINT ( 'NONE',  ( -44.43458752740489359, 1435.686101446479825, 270.0922352104699939 ) ) ;
#47462=CARTESIAN_POINT ( 'NONE',  ( 2.936137002789280359, 1417.857599898479975, 233.6311759696189938 ) ) ;
#47463=CARTESIAN_POINT ( 'NONE',  ( -2.349329596450000057, 1396.056272350230074, 197.6305884707980169 ) ) ;
#47466=EDGE_LOOP ( 'NONE', ( #97162, #99898, #28353, #67451 ) ) ;
#47467=ORIENTED_EDGE ( 'NONE', *, *, #55611, .F. ) ;
#47468=CARTESIAN_POINT ( 'NONE',  ( 44.72902951799282079, 1447.701297687701526, 269.0001835098157699 ) ) ;
#47471=CARTESIAN_POINT ( 'NONE',  ( -2.793439694759999981, 1486.025328433629966, 182.0741016712979956 ) ) ;
#47476=CARTESIAN_POINT ( 'NONE',  ( 11.68483146220000002, 1415.296882296330068, 223.0065844743980108 ) ) ;
#47480=ORIENTED_EDGE ( 'NONE', *, *, #40496, .T. ) ;
#47481=CARTESIAN_POINT ( 'NONE',  ( -33.91369111065759512, 1451.728768197430099, 135.0584859664319879 ) ) ;
#47483=ORIENTED_EDGE ( 'NONE', *, *, #63813, .T. ) ;
#47484=CARTESIAN_POINT ( 'NONE',  ( 5.136464557128770814, 1457.210140256051773, 228.2402603896014739 ) ) ;
#47485=ADVANCED_FACE ( 'NONE', ( #58763 ), #104406, .F. ) ;
#47486=CARTESIAN_POINT ( 'NONE',  ( -18.89924245745137554, 1416.831922880734282, 207.5749492336007904 ) ) ;
#47487=CARTESIAN_POINT ( 'NONE',  ( 13.50890991390000018, 1415.048591094029916, 197.7020156336979824 ) ) ;
#47489=CARTESIAN_POINT ( 'NONE',  ( 22.30118273070000257, 1410.611534642730248, 204.7343940648379714 ) ) ;
#47490=CARTESIAN_POINT ( 'NONE',  ( 16.84507916019999740, 1409.666197915029898, 225.6438639091979894 ) ) ;
#47493=CARTESIAN_POINT ( 'NONE',  ( 24.58641666395997305, 1443.335256792440759, 213.0934990515747529 ) ) ;
#47498=DIRECTION ( 'NONE',  ( 0.9999999993216598382, 3.683192149143328935E-05, 3.002444966984699305E-07 ) ) ;
#47502=AXIS2_PLACEMENT_3D ( 'NONE', #42865, #26594, #8684 ) ;
#47503=CARTESIAN_POINT ( 'NONE',  ( -37.74895065031819996, 1449.030701455520102, 136.3532337052970149 ) ) ;
#47505=DIRECTION ( 'NONE',  ( 1.000000000000000000, 0.000000000000000000, 0.000000000000000000 ) ) ;
#47506=CARTESIAN_POINT ( 'NONE',  ( 18.00600711065910531, 1424.203672432876601, 225.4083150014673436 ) ) ;
#47510=CARTESIAN_POINT ( 'NONE',  ( 29.68293233167989698, 1440.913060386479856, 237.3170996871120053 ) ) ;
#47514=VERTEX_POINT ( 'NONE', #4122 ) ;
#47517=CARTESIAN_POINT ( 'NONE',  ( -1.725662463192670248, 1484.236887848700007, 182.7463278875050037 ) ) ;
#47526=CARTESIAN_POINT ( 'NONE',  ( -14.73399051909999891, 1489.466620109829819, 192.5160264904980068 ) ) ;
#47528=CARTESIAN_POINT ( 'NONE',  ( 1.613885712409999895, 1466.648931211529771, 234.8412340160980136 ) ) ;
#47529=CARTESIAN_POINT ( 'NONE',  ( -41.66090858750000336, 1443.836096447190130, 135.6920785174980040 ) ) ;
#47531=CARTESIAN_POINT ( 'NONE',  ( -0.7408122144259999819, 1450.887191310580192, 181.3422759365979857 ) ) ;
#47534=CARTESIAN_POINT ( 'NONE',  ( -17.97699752310530030, 1415.938742849230039, 208.9722450247610084 ) ) ;
#47537=ORIENTED_EDGE ( 'NONE', *, *, #32258, .T. ) ;
#47541=CARTESIAN_POINT ( 'NONE',  ( 36.22314289287339761, 1437.522903125109906, 136.5404214408590065 ) ) ;
#47543=CARTESIAN_POINT ( 'NONE',  ( -11.60004869885203327, 1426.721831802138922, 134.4552142047555208 ) ) ;
#47547=CARTESIAN_POINT ( 'NONE',  ( 18.02089981653400130, 1424.325684919356036, 225.2034556834539956 ) ) ;
#47549=CARTESIAN_POINT ( 'NONE',  ( -19.91421809350000061, 1485.651811164430228, 190.8591891487979808 ) ) ;
#47550=CARTESIAN_POINT ( 'NONE',  ( 11.30129387169999866, 1432.307760315640053, 151.5220333367980174 ) ) ;
#47551=DIRECTION ( 'NONE',  ( -0.0006352486380477548626, 0.9989931984823255950, -0.04485739454338198706 ) ) ;
#47553=ORIENTED_EDGE ( 'NONE', *, *, #74117, .T. ) ;
#47556=CARTESIAN_POINT ( 'NONE',  ( -11.69984112520000075, 1435.115366081830189, 151.3290766764980049 ) ) ;
#47557=CARTESIAN_POINT ( 'NONE',  ( -4.253586639292240192E-10, 1469.109899135820115, 251.5649450797509701 ) ) ;
#47558=CARTESIAN_POINT ( 'NONE',  ( -20.50883971185030319, 1504.912087959059818, 190.4750152204429980 ) ) ;
#47561=CARTESIAN_POINT ( 'NONE',  ( -0.9030881519919999878, 1483.390131495029891, 182.0736268275980194 ) ) ;
#47566=CARTESIAN_POINT ( 'NONE',  ( -15.15764896601350031, 1414.025930248449868, 226.8247619795940011 ) ) ;
#47568=CARTESIAN_POINT ( 'NONE',  ( -14.03821757262499936, 1435.593435673239810, 149.8875993374950042 ) ) ;
#47570=CARTESIAN_POINT ( 'NONE',  ( 6.639707775743658225, 1425.354353559006995, 226.3614492073465954 ) ) ;
#47572=EDGE_LOOP ( 'NONE', ( #109287, #87019, #85028, #36189 ) ) ;
#47573=CARTESIAN_POINT ( 'NONE',  ( 10.53938673299999884, 1414.594228655729921, 248.5638781382980085 ) ) ;
#47574=CARTESIAN_POINT ( 'NONE',  ( -28.18850436489999822, 1508.134789598230100, 208.4601711067210204 ) ) ;
#47575=CARTESIAN_POINT ( 'NONE',  ( -2.540026744920000024, 1494.212893936630053, 181.3995399813979930 ) ) ;
#47577=CARTESIAN_POINT ( 'NONE',  ( -17.72824029589999739, 1410.893857127930232, 194.8229014749980195 ) ) ;
#47578=CARTESIAN_POINT ( 'NONE',  ( -6.865865202968861603, 1408.020609328411410, 270.1276013130552656 ) ) ;
#47579=CARTESIAN_POINT ( 'NONE',  ( -25.95018329139999835, 1431.999486641019985, 231.7147496198979866 ) ) ;
#47580=CARTESIAN_POINT ( 'NONE',  ( -29.24989835495881252, 1509.943647848841238, 204.9747545366232657 ) ) ;
#47581=CARTESIAN_POINT ( 'NONE',  ( -11.21839826972749954, 1452.521305287280029, 150.0610815246930088 ) ) ;
#47582=CARTESIAN_POINT ( 'NONE',  ( 27.85271936110000013, 1451.938833075630100, 135.3270518959979825 ) ) ;
#47583=EDGE_LOOP ( 'NONE', ( #77455, #30697, #10364, #65454 ) ) ;
#47584=CARTESIAN_POINT ( 'NONE',  ( -5.360341398479370412, 1422.242775764549833, 144.1555102201419913 ) ) ;
#47586=B_SPLINE_CURVE_WITH_KNOTS ( 'NONE', 5,
 ( #2229, #44211, #71090, #94583, #20090, #1663, #52613, #36345, #104654, #95155, #35242, #27951 ),
 .UNSPECIFIED., .F., .F.,
 ( 6, 3, 3, 6 ),
 ( 0.000000000000000000, 0.3723444189143530481, 0.7907814729714509605, 1.000000000000000000 ),
 .UNSPECIFIED. ) ;
#47588=ORIENTED_EDGE ( 'NONE', *, *, #28178, .F. ) ;
#47589=ORIENTED_EDGE ( 'NONE', *, *, #102366, .F. ) ;
#47591=CARTESIAN_POINT ( 'NONE',  ( -22.81607804052979915, 1409.709800168469883, 208.9487546288140152 ) ) ;
#47593=CARTESIAN_POINT ( 'NONE',  ( 0.0002122017571388959824, 1432.353341358199941, 123.3907408769529894 ) ) ;
#47595=CARTESIAN_POINT ( 'NONE',  ( -1.122745254329999831, 1479.775692482730165, 236.0081096927980013 ) ) ;
#47596=CARTESIAN_POINT ( 'NONE',  ( -2.109056957580000002, 1421.166295015029846, 183.8085771866980167 ) ) ;
#47597=CONICAL_SURFACE ( 'NONE', #1172, 18.60900368820000850, 0.6981317007980000211 ) ;
#47599=CARTESIAN_POINT ( 'NONE',  ( 46.15241727715709885, 1441.855333579869921, 268.2045457479380275 ) ) ;
#47606=CARTESIAN_POINT ( 'NONE',  ( 13.12808455398275953, 1443.048474982209200, 187.4204472368715244 ) ) ;
#47610=EDGE_CURVE ( 'NONE', #56666, #80182, #109769, .T. ) ;
#47612=CARTESIAN_POINT ( 'NONE',  ( 13.31241404839999909, 1509.377940129630133, 234.8971984757980067 ) ) ;
#47614=CARTESIAN_POINT ( 'NONE',  ( 23.84533589473599946, 1452.080362908450070, 136.9869410992479857 ) ) ;
#47618=CARTESIAN_POINT ( 'NONE',  ( -10.97428490540760038, 1432.631986041290247, 151.7699425487470251 ) ) ;
#47619=CARTESIAN_POINT ( 'NONE',  ( 0.03374749302241145110, 1409.321302690946368, 232.7832470492207051 ) ) ;
#47620=CARTESIAN_POINT ( 'NONE',  ( -16.78589851036889868, 1414.704930897790064, 191.6301813728830155 ) ) ;
#47623=CARTESIAN_POINT ( 'NONE',  ( -24.46809548295560077, 1509.129436896289917, 222.5284892987700118 ) ) ;
#47624=CARTESIAN_POINT ( 'NONE',  ( 4.866999017969999564, 1428.784516533529995, 149.2390836726979728 ) ) ;
#47626=CARTESIAN_POINT ( 'NONE',  ( 19.80583403109999807, 1436.359101875030092, 219.6133833564979909 ) ) ;
#47635=B_SPLINE_CURVE_WITH_KNOTS ( 'NONE', 3,
 ( #12910, #97481, #96943, #20749 ),
 .UNSPECIFIED., .F., .F.,
 ( 4, 4 ),
 ( -105.4335682549999973, -86.05908296062720808 ),
 .UNSPECIFIED. ) ;
#47636=CARTESIAN_POINT ( 'NONE',  ( 4.425709718559999041E-15, 1434.541746329560056, 150.4759714514979976 ) ) ;
#47643=CARTESIAN_POINT ( 'NONE',  ( 16.84769428410000103, 1419.772082749829906, 226.8208912202979946 ) ) ;
#47646=CARTESIAN_POINT ( 'NONE',  ( -19.26254113000000245, 1410.947276881129937, 222.4619606201979991 ) ) ;
#47647=ADVANCED_FACE ( 'NONE', ( #10861 ), #55635, .T. ) ;
#47648=CARTESIAN_POINT ( 'NONE',  ( -0.3327850108241715565, 1508.979300183436180, 238.8653632281604757 ) ) ;
#47649=CARTESIAN_POINT ( 'NONE',  ( -0.9049687798709999953, 1422.347128627729944, 228.2716864167980191 ) ) ;
#47652=DIRECTION ( 'NONE',  ( 0.000000000000000000, 1.000000000000000000, 0.000000000000000000 ) ) ;
#47655=CARTESIAN_POINT ( 'NONE',  ( -34.93120292363229851, 1435.717329652130047, 135.0377845007600115 ) ) ;
#47659=CARTESIAN_POINT ( 'NONE',  ( -6.290310848379998987, 1409.132722882430016, 222.9509587267980066 ) ) ;
#47663=CARTESIAN_POINT ( 'NONE',  ( 12.40413062160000024, 1434.420063654429896, 149.0257888567980160 ) ) ;
#47664=PLANE ( 'NONE',  #48325 ) ;
#47665=CARTESIAN_POINT ( 'NONE',  ( 10.69787753770000016, 1442.513770420949868, 185.9957791832980263 ) ) ;
#47669=CARTESIAN_POINT ( 'NONE',  ( -2.554115229335069959, 1409.002252056529869, 223.8943861301169989 ) ) ;
#47672=CARTESIAN_POINT ( 'NONE',  ( 13.96283759872080132, 1508.693956055879880, 233.0808216126870036 ) ) ;
#47673=CARTESIAN_POINT ( 'NONE',  ( 40.50375002456848250, 1425.156793582443925, 269.1155438645719187 ) ) ;
#47674=CARTESIAN_POINT ( 'NONE',  ( 20.56164794690000264, 1453.151875979930082, 210.4536761478879896 ) ) ;
#47680=CARTESIAN_POINT ( 'NONE',  ( -28.57599588808039925, 1509.162863321990017, 208.7718535704119915 ) ) ;
#47683=CARTESIAN_POINT ( 'NONE',  ( -16.37947571190000318, 1409.734195298129862, 225.9725054800979933 ) ) ;
#47684=CARTESIAN_POINT ( 'NONE',  ( 0.5111074947771929722, 1410.993655183119927, 185.0427835985659897 ) ) ;
#47686=CARTESIAN_POINT ( 'NONE',  ( -11.82020261140000095, 1508.077988756929926, 183.1980805049979892 ) ) ;
#47690=CARTESIAN_POINT ( 'NONE',  ( -11.36018332909999984, 1414.996444518330009, 195.9645814724980255 ) ) ;
#47691=CARTESIAN_POINT ( 'NONE',  ( 0.001377745780720000032, 1465.018687260529987, 237.3906760667979938 ) ) ;
#47692=CARTESIAN_POINT ( 'NONE',  ( 18.88261216240000095, 1409.572455740129953, 220.0130051960980211 ) ) ;
#47693=CARTESIAN_POINT ( 'NONE',  ( 0.5697990016583959205, 1450.893162567740092, 181.2939912002310052 ) ) ;
#47695=CARTESIAN_POINT ( 'NONE',  ( -18.11291060900000005, 1424.770096122030054, 227.5276574296979959 ) ) ;
#47698=CARTESIAN_POINT ( 'NONE',  ( 26.62565391809450333, 1469.324738006449934, 208.6920304769689949 ) ) ;
#47701=CARTESIAN_POINT ( 'NONE',  ( -0.9237819473580000107, 1416.172288158230231, 233.4037497922979867 ) ) ;
#47704=DIRECTION ( 'NONE',  ( -0.9272785430170710219, -0.03238144682225380100, -0.3729690946470439750 ) ) ;
#47706=CARTESIAN_POINT ( 'NONE',  ( -3.500000000000000000, 1424.163060387329779, 172.2701767054979882 ) ) ;
#47707=CARTESIAN_POINT ( 'NONE',  ( 14.00898853540000033, 1416.833018152729892, 196.3916011246980133 ) ) ;
#47711=CARTESIAN_POINT ( 'NONE',  ( 28.13477516149999857, 1508.112005763430034, 210.1092937961579992 ) ) ;
#47714=CARTESIAN_POINT ( 'NONE',  ( -17.76091714769999896, 1410.905089322729964, 194.9382696558980115 ) ) ;
#47715=CARTESIAN_POINT ( 'NONE',  ( -11.69554736699999786, 1426.722884897929816, 141.2004217243980122 ) ) ;
#47716=CARTESIAN_POINT ( 'NONE',  ( 15.69540887480520119, 1410.567746757359828, 191.5434892055160105 ) ) ;
#47718=CARTESIAN_POINT ( 'NONE',  ( -24.62049690961300286, 1452.037610211400079, 136.1636793085519912 ) ) ;
#47719=CARTESIAN_POINT ( 'NONE',  ( -11.63666214179999869, 1425.864857562230100, 144.1663263557980201 ) ) ;
#47720=CARTESIAN_POINT ( 'NONE',  ( 9.055707583609999389, 1409.396424226330055, 229.6055981440979963 ) ) ;
#47723=CARTESIAN_POINT ( 'NONE',  ( 41.61795676512019782, 1442.846609226920009, 134.0999999981039821 ) ) ;
#47724=CARTESIAN_POINT ( 'NONE',  ( -39.87872480270220166, 1441.370340969270046, 136.8657547114230226 ) ) ;
#47731=DIRECTION ( 'NONE',  ( 0.000000000000000000, 0.000000000000000000, -1.000000000000000000 ) ) ;
#47735=CARTESIAN_POINT ( 'NONE',  ( -40.26396455803409680, 1444.186530478750001, 137.1012301494149881 ) ) ;
#47738=CARTESIAN_POINT ( 'NONE',  ( -1.517666159849999863, 1497.689500997429832, 231.6008634864979854 ) ) ;
#47739=CARTESIAN_POINT ( 'NONE',  ( 11.22085809280000035, 1414.913060387329779, 197.6243702818979955 ) ) ;
#47741=VERTEX_POINT ( 'NONE', #27653 ) ;
#47745=CARTESIAN_POINT ( 'NONE',  ( 34.07917771385839956, 1440.913060387330006, 259.4382560880169422 ) ) ;
#47746=CARTESIAN_POINT ( 'NONE',  ( 18.15454648420000083, 1457.025425127630115, 227.8110394751979868 ) ) ;
#47748=CARTESIAN_POINT ( 'NONE',  ( -0.3067201157339999873, 1452.334527121330211, 183.2866423852979949 ) ) ;
#47749=CARTESIAN_POINT ( 'NONE',  ( -16.22975407500000244, 1409.646465899229952, 192.1195335419979813 ) ) ;
#47750=CARTESIAN_POINT ( 'NONE',  ( -22.98095477630000261, 1420.941325299229902, 212.0408358845679970 ) ) ;
#47752=CARTESIAN_POINT ( 'NONE',  ( 22.17089962140870085, 1410.141205781899998, 206.2581381202189732 ) ) ;
#47754=CARTESIAN_POINT ( 'NONE',  ( -2.858129514550000305, 1507.751283221830136, 180.8639750916980233 ) ) ;
#47757=CARTESIAN_POINT ( 'NONE',  ( 14.88687292590000055, 1460.215022219430011, 231.2459449793980184 ) ) ;
#47758=CARTESIAN_POINT ( 'NONE',  ( -23.32556912959070061, 1416.023918999339912, 210.9192148309080039 ) ) ;
#47762=CARTESIAN_POINT ( 'NONE',  ( -0.1434969078204259840, 1507.634396196580155, 180.8101134974600086 ) ) ;
#47766=CARTESIAN_POINT ( 'NONE',  ( 18.64460737039999927, 1509.564144423530252, 186.5337401517980140 ) ) ;
#47771=CARTESIAN_POINT ( 'NONE',  ( 4.500000000000000000, 1448.210448412289907, 170.6974824052979898 ) ) ;
#47772=CARTESIAN_POINT ( 'NONE',  ( 6.216948005759999719E-09, 1459.726867864730139, 213.1264974772779794 ) ) ;
#47774=CARTESIAN_POINT ( 'NONE',  ( -11.57120699989999757, 1431.932395937310048, 151.1858022038979925 ) ) ;
#47775=CARTESIAN_POINT ( 'NONE',  ( 19.19771385826059884, 1456.936707467760243, 224.8620913037029823 ) ) ;
#47777=CARTESIAN_POINT ( 'NONE',  ( 1.547463896846929865, 1414.913060387349788, 192.3096116128920130 ) ) ;
#47779=CARTESIAN_POINT ( 'NONE',  ( 12.70914363729999863, 1445.041869922740034, 186.8564040585980024 ) ) ;
#47780=CARTESIAN_POINT ( 'NONE',  ( -23.50891559320000113, 1470.079355157530017, 219.2631860520979785 ) ) ;
#47783=CARTESIAN_POINT ( 'NONE',  ( -0.08461443291850000159, 1416.823634022829992, 191.0185729562979873 ) ) ;
#47784=EDGE_LOOP ( 'NONE', ( #37925, #59686, #85798, #35595 ) ) ;
#47786=CARTESIAN_POINT ( 'NONE',  ( 7.084494119980000448, 1406.178315946529892, 268.4624913171979870 ) ) ;
#47788=DIRECTION ( 'NONE',  ( 0.9417419115949053898, 0.3363363969979660806, 0.000000000000000000 ) ) ;
#47789=CARTESIAN_POINT ( 'NONE',  ( 22.93959776030420272, 1432.116225619942270, 216.2250907020126363 ) ) ;
#47790=B_SPLINE_CURVE_WITH_KNOTS ( 'NONE', 3,
 ( #31578, #4725, #38869, #30478, #68521, #50601, #76911, #43854, #85280, #8030, #60678, #8579, #34343, #59012, #43311, #94236, #69079, #7485, #9148 ),
 .UNSPECIFIED., .F., .F.,
 ( 4, 2, 2, 2, 1, 1, 1, 2, 2, 2, 4 ),
 ( 0.000000000000000000, 0.2500000000006191159, 0.3750000000009287016, 0.4375000000010938472, 0.4687500000012264634, 0.4843750000013014589, 0.4921875000013305468, 0.4960937500014176993, 0.5000000000015047963, 0.7500000000007523981, 1.000000000000000000 ),
 .UNSPECIFIED. ) ;
#47792=FACE_OUTER_BOUND ( 'NONE', #61467, .T. ) ;
#47794=CARTESIAN_POINT ( 'NONE',  ( -2.323033500480000235, 1449.800808693189992, 155.6080925164979760 ) ) ;
#47795=CARTESIAN_POINT ( 'NONE',  ( -12.53380136120000010, 1445.052233027470038, 185.6742673453979933 ) ) ;
#47796=CARTESIAN_POINT ( 'NONE',  ( 2.500094834180730086, 1448.919094884260176, 155.0643240262459983 ) ) ;
#47799=CARTESIAN_POINT ( 'NONE',  ( 5.329070518200000398E-15, 1416.825952160429779, 255.3819207742980097 ) ) ;
#47801=LINE ( 'NONE', #23683, #41246 ) ;
#47802=CARTESIAN_POINT ( 'NONE',  ( 3.655447866509999866, 1441.516748634489886, 170.5484046385980150 ) ) ;
#47803=CARTESIAN_POINT ( 'NONE',  ( -3.386669734929999898, 1474.956089833430042, 269.6463548828979810 ) ) ;
#47805=CARTESIAN_POINT ( 'NONE',  ( -8.759952407214090186, 1423.587288072539877, 144.1551656127980152 ) ) ;
#47810=CARTESIAN_POINT ( 'NONE',  ( -17.40764085468179800, 1414.996442620800053, 207.5654756526599840 ) ) ;
#47812=DIRECTION ( 'NONE',  ( 0.000000000000000000, 0.000000000000000000, -1.000000000000000000 ) ) ;
#47814=CARTESIAN_POINT ( 'NONE',  ( -22.40412009319999953, 1411.055624679330094, 203.1355812455580008 ) ) ;
#47815=CARTESIAN_POINT ( 'NONE',  ( -15.49572516138399969, 1421.633966799186055, 227.2929845234520201 ) ) ;
#47816=CARTESIAN_POINT ( 'NONE',  ( -45.08261358189999868, 1435.036897264239997, 268.9899376266980653 ) ) ;
#47819=CARTESIAN_POINT ( 'NONE',  ( 13.40958089240390017, 1414.996442620800053, 197.9133050684260127 ) ) ;
#47823=CARTESIAN_POINT ( 'NONE',  ( -16.09630756760823189, 1409.475146607743454, 225.1332669131820410 ) ) ;
#47825=B_SPLINE_CURVE_WITH_KNOTS ( 'NONE', 3,
 ( #50113, #109461, #7540, #75854, #49013, #110004, #83149, #23224, #83691, #33281 ),
 .UNSPECIFIED., .F., .F.,
 ( 4, 2, 2, 2, 4 ),
 ( 0.000000000000000000, 0.2500000000000000000, 0.5000000000000000000, 0.7500000000000000000, 1.000000000000000000 ),
 .UNSPECIFIED. ) ;
#47837=CARTESIAN_POINT ( 'NONE',  ( -6.220302174429999553, 1397.477102020930033, 197.7753768578980100 ) ) ;
#47838=CARTESIAN_POINT ( 'NONE',  ( -19.36881300869999833, 1410.511871308530090, 222.2034276849980188 ) ) ;
#47839=CARTESIAN_POINT ( 'NONE',  ( -1.316362887759999989, 1415.041103189330215, 226.7113481479980237 ) ) ;
#47840=CARTESIAN_POINT ( 'NONE',  ( -13.35314812681837360, 1444.506189530448182, 169.3733437756958438 ) ) ;
#47841=CARTESIAN_POINT ( 'NONE',  ( -26.60753868740000172, 1509.169818042129918, 201.4350758664580212 ) ) ;
#47844=CARTESIAN_POINT ( 'NONE',  ( 17.77226856539999744, 1416.272325472730017, 225.3684990499980074 ) ) ;
#47847=CARTESIAN_POINT ( 'NONE',  ( -40.94281863450720493, 1445.635000978330027, 136.6596512823030025 ) ) ;
#47848=CARTESIAN_POINT ( 'NONE',  ( 8.618023458351569133, 1396.214008466279893, 202.1935922150420026 ) ) ;
#47849=CARTESIAN_POINT ( 'NONE',  ( 0.5679639878839999323, 1416.568813547830132, 190.4860628299979908 ) ) ;
#47850=CARTESIAN_POINT ( 'NONE',  ( 11.84752247700000005, 1430.969153207809995, 150.2425949294979830 ) ) ;
#47854=CARTESIAN_POINT ( 'NONE',  ( 2.373304165714522629, 1449.620559872589865, 182.2130135973664551 ) ) ;
#47855=ORIENTED_EDGE ( 'NONE', *, *, #96727, .F. ) ;
#47858=CARTESIAN_POINT ( 'NONE',  ( -14.60046712539999980, 1460.133194728129865, 230.9282956282980024 ) ) ;
#47860=CARTESIAN_POINT ( 'NONE',  ( -13.58416853039999950, 1434.822844256989811, 196.0567512594979860 ) ) ;
#47864=ORIENTED_EDGE ( 'NONE', *, *, #99437, .T. ) ;
#47865=DIRECTION ( 'NONE',  ( -0.9995238204287079098, -0.03085664264949923227, 3.329727431759169316E-08 ) ) ;
#47866=CARTESIAN_POINT ( 'NONE',  ( 0.05018163627710000435, 1508.979242228630028, 179.3226982217979923 ) ) ;
#47868=CARTESIAN_POINT ( 'NONE',  ( 5.335637657409999512, 1416.823418193129783, 226.4969446031979885 ) ) ;
#47870=ORIENTED_EDGE ( 'NONE', *, *, #70919, .T. ) ;
#47872=CARTESIAN_POINT ( 'NONE',  ( -20.49660237009999975, 1509.524916194930029, 230.0429231069980176 ) ) ;
#47873=CARTESIAN_POINT ( 'NONE',  ( -16.23190381645581937, 1412.775336537543126, 269.3700702654938937 ) ) ;
#47876=ORIENTED_EDGE ( 'NONE', *, *, #93250, .T. ) ;
#47877=CARTESIAN_POINT ( 'NONE',  ( 2.500000000000000000, 1428.988705744230174, 157.0781314899979861 ) ) ;
#47878=CARTESIAN_POINT ( 'NONE',  ( -28.50339170433599989, 1440.913060387269979, 233.1297467994120041 ) ) ;
#47882=CARTESIAN_POINT ( 'NONE',  ( 5.349258415000000433, 1408.472118978329945, 270.3881948815980536 ) ) ;
#47886=CARTESIAN_POINT ( 'NONE',  ( 22.98387363149999985, 1409.741890572629927, 208.9143205900259943 ) ) ;
#47892=CARTESIAN_POINT ( 'NONE',  ( 25.10807187043309341, 1509.789853576705582, 224.8278757916732218 ) ) ;
#47893=FACE_OUTER_BOUND ( 'NONE', #35784, .T. ) ;
#47899=CARTESIAN_POINT ( 'NONE',  ( 0.3041635068690000665, 1415.771586802929960, 233.4346734808979988 ) ) ;
#47900=( BOUNDED_CURVE ( )  B_SPLINE_CURVE ( 3, ( #100174, #23459, #56534, #13945 ),
 .UNSPECIFIED., .F., .T. ) 
 B_SPLINE_CURVE_WITH_KNOTS ( ( 4, 4 ),
 ( 5.864774099209800085, 6.175064727860119618 ),
 .UNSPECIFIED. ) 
 CURVE ( )  GEOMETRIC_REPRESENTATION_ITEM ( )  RATIONAL_B_SPLINE_CURVE ( ( 1.000000000000000000, 0.9919927244685476930, 0.9919927244685476930, 1.000000000000000000 ) ) 
 REPRESENTATION_ITEM ( '' )  );
#47901=CARTESIAN_POINT ( 'NONE',  ( -21.22285432549390194, 1509.591297325790038, 229.2096536192680105 ) ) ;
#47907=CARTESIAN_POINT ( 'NONE',  ( -22.51990865419010035, 1410.619212616680215, 212.0399858957769936 ) ) ;
#47909=AXIS2_PLACEMENT_3D ( 'NONE', #74269, #14322, #39544 ) ;
#47912=CARTESIAN_POINT ( 'NONE',  ( -19.00334344016446764, 1416.835288280170971, 207.9336683422605461 ) ) ;
#47913=VERTEX_POINT ( 'NONE', #41001 ) ;
#47914=CARTESIAN_POINT ( 'NONE',  ( 11.60004869884797252, 1426.686844628437029, 134.5519029425135216 ) ) ;
#47915=CARTESIAN_POINT ( 'NONE',  ( 24.42191297719999810, 1445.300895561380003, 213.9593811286180198 ) ) ;
#47916=CARTESIAN_POINT ( 'NONE',  ( 8.882670428210953872, 1437.098088324273021, 153.1961944285610855 ) ) ;
#47919=CARTESIAN_POINT ( 'NONE',  ( 16.31056445758360951, 1421.543483176982136, 227.2422000032759115 ) ) ;
#47920=CARTESIAN_POINT ( 'NONE',  ( -2.500000000200000017, 1447.619163115419724, 168.9991030154980081 ) ) ;
#47921=CARTESIAN_POINT ( 'NONE',  ( -19.81973760889999880, 1426.576893715330016, 222.8594164923980259 ) ) ;
#47922=CARTESIAN_POINT ( 'NONE',  ( -21.83293579365600934, 1470.997130817396737, 269.4963378681733843 ) ) ;
#47924=CARTESIAN_POINT ( 'NONE',  ( 18.13816720160000173, 1445.350867493739770, 191.0157095493979966 ) ) ;
#47926=CARTESIAN_POINT ( 'NONE',  ( -17.51694058469201920, 1434.100402768573076, 216.1837452212066637 ) ) ;
#47927=CARTESIAN_POINT ( 'NONE',  ( -38.85577259545065942, 1452.541743301062752, 269.5906804772505438 ) ) ;
#47928=ORIENTED_EDGE ( 'NONE', *, *, #38446, .F. ) ;
#47931=CARTESIAN_POINT ( 'NONE',  ( 11.48266949309999951, 1442.832333866149838, 147.8781297902980043 ) ) ;
#47935=CARTESIAN_POINT ( 'NONE',  ( -15.96958168569999970, 1519.913060387329779, 225.0914276473980067 ) ) ;
#47936=CARTESIAN_POINT ( 'NONE',  ( 1.465959060849369999, 1490.245831247160140, 181.8489739673789813 ) ) ;
#47937=CARTESIAN_POINT ( 'NONE',  ( -3.527569048119670203, 1486.518325592330029, 181.8541486797999767 ) ) ;
#47938=CARTESIAN_POINT ( 'NONE',  ( -13.32047630834354379, 1444.558074092078868, 186.7651240210572610 ) ) ;
#47945=CARTESIAN_POINT ( 'NONE',  ( 12.27023112330000032, 1416.839692136459917, 223.5796784318309847 ) ) ;
#47953=CARTESIAN_POINT ( 'NONE',  ( 38.89347719239705725, 1429.350770580238759, 269.5911400078334736 ) ) ;
#47954=CARTESIAN_POINT ( 'NONE',  ( -4.694071443940000421, 1465.143864313730091, 238.2947549836979988 ) ) ;
#47955=CARTESIAN_POINT ( 'NONE',  ( -20.19216181010000000, 1506.518050785829928, 189.2324904367980309 ) ) ;
#47956=VECTOR ( 'NONE', #37724, 999.9999999999998863 ) ;
#47957=CARTESIAN_POINT ( 'NONE',  ( -11.12720837410000030, 1433.553190407860029, 151.6643070703979959 ) ) ;
#47959=CARTESIAN_POINT ( 'NONE',  ( 11.72449310896590013, 1426.703930266699899, 143.2718442946500090 ) ) ;
#47960=DIRECTION ( 'NONE',  ( 0.000000000000000000, 0.000000000000000000, 1.000000000000000000 ) ) ;
#47963=DIRECTION ( 'NONE',  ( -0.9993908263153354898, 0.03489949404026521790, 3.990594469010557284E-05 ) ) ;
#47966=CARTESIAN_POINT ( 'NONE',  ( -22.52609270459879909, 1509.699688878229836, 190.3921826462719764 ) ) ;
#47967=CARTESIAN_POINT ( 'NONE',  ( -6.143218938422219407E-10, 1412.721203181489955, 251.5507141014840045 ) ) ;
#47969=VERTEX_POINT ( 'NONE', #90295 ) ;
#47972=EDGE_CURVE ( 'NONE', #33967, #104880, #60534, .T. ) ;
#47974=CARTESIAN_POINT ( 'NONE',  ( -13.45498908600000121, 1472.108093304129852, 270.3655312995979898 ) ) ;
#47975=CARTESIAN_POINT ( 'NONE',  ( 13.43167025587599817, 1509.382104656720003, 235.1752264429409820 ) ) ;
#47978=CARTESIAN_POINT ( 'NONE',  ( -13.83973980200000220, 1452.407470494729978, 223.0844041600979892 ) ) ;
#47979=CARTESIAN_POINT ( 'NONE',  ( 0.2157562901360330077, 1451.841949984589974, 182.9506228356109716 ) ) ;
#47980=EDGE_CURVE ( 'NONE', #68835, #92411, #48315, .T. ) ;
#47982=EDGE_CURVE ( 'NONE', #59669, #88136, #74079, .T. ) ;
#47983=CARTESIAN_POINT ( 'NONE',  ( 12.78776258895000062, 1416.851343899079893, 222.7045348340550106 ) ) ;
#47986=CARTESIAN_POINT ( 'NONE',  ( -41.79789112272889895, 1426.458875065289931, 266.3000610535190162 ) ) ;
#47990=ORIENTED_EDGE ( 'NONE', *, *, #41892, .T. ) ;
#47992=CARTESIAN_POINT ( 'NONE',  ( 4.817341278711412933, 1423.525569767164825, 184.0959883682457132 ) ) ;
#47996=CARTESIAN_POINT ( 'NONE',  ( -7.781677482780000155, 1455.443741433530249, 185.5405848752979807 ) ) ;
#47997=CARTESIAN_POINT ( 'NONE',  ( -15.76201573909119880, 1470.477545809950243, 228.9865716979510069 ) ) ;
#47998=ORIENTED_EDGE ( 'NONE', *, *, #66484, .F. ) ;
#47999=CARTESIAN_POINT ( 'NONE',  ( -26.64155692649999807, 1435.970859033209990, 136.4793274970979837 ) ) ;
#48003=CARTESIAN_POINT ( 'NONE',  ( -37.55262740391170695, 1450.862648352295537, 134.7342543275423452 ) ) ;
#48005=CARTESIAN_POINT ( 'NONE',  ( 1.092787220074867172, 1508.991959848587385, 238.7857758380762903 ) ) ;
#48006=CARTESIAN_POINT ( 'NONE',  ( -27.13870397648479837, 1417.586336025329956, 269.4419590831910227 ) ) ;
#48008=CARTESIAN_POINT ( 'NONE',  ( -3.817532458140000085, 1397.107874215530046, 196.7824443944979862 ) ) ;
#48010=ORIENTED_EDGE ( 'NONE', *, *, #90466, .F. ) ;
#48011=ORIENTED_EDGE ( 'NONE', *, *, #9035, .T. ) ;
#48012=CARTESIAN_POINT ( 'NONE',  ( 0.2313785129550000041, 1452.338695476229759, 183.2832210453979940 ) ) ;
#48013=EDGE_CURVE ( 'NONE', #61056, #37055, #13565, .T. ) ;
#48016=CARTESIAN_POINT ( 'NONE',  ( -13.29541393167429852, 1436.106548041590031, 150.6070985400420170 ) ) ;
#48017=CARTESIAN_POINT ( 'NONE',  ( -0.03628264342808269760, 1409.501674693219911, 185.3028950835800117 ) ) ;
#48021=CARTESIAN_POINT ( 'NONE',  ( -23.42324794740000016, 1435.764285783320247, 213.6171179551379851 ) ) ;
#48022=CARTESIAN_POINT ( 'NONE',  ( -13.89764403649999913, 1426.832043286230146, 222.2177421718979815 ) ) ;
#48023=CARTESIAN_POINT ( 'NONE',  ( 12.26815783919999880, 1415.553739807329976, 222.8908496634980168 ) ) ;
#48027=CARTESIAN_POINT ( 'NONE',  ( -40.71747596589660390, 1448.637563225599934, 134.7398509209010058 ) ) ;
#48028=CARTESIAN_POINT ( 'NONE',  ( -23.94385147653602885, 1445.794803258163483, 213.0147832418295764 ) ) ;
#48029=EDGE_LOOP ( 'NONE', ( #1442, #88354, #54381, #386, #32632, #70630 ) ) ;
#48030=CARTESIAN_POINT ( 'NONE',  ( 17.96021206209637811, 1457.749394617433381, 229.4559061195007530 ) ) ;
#48031=CARTESIAN_POINT ( 'NONE',  ( -28.59841874989484367, 1509.911739175358662, 211.5620547949469312 ) ) ;
#48032=CARTESIAN_POINT ( 'NONE',  ( 13.20846943169999932, 1414.988017870030035, 197.7899243759980266 ) ) ;
#48034=CARTESIAN_POINT ( 'NONE',  ( 19.90019938289999857, 1410.103226705929956, 197.6288084474979883 ) ) ;
#48037=CARTESIAN_POINT ( 'NONE',  ( -0.04210048962123905114, 1506.527232291142582, 187.0606773027650434 ) ) ;
#48038=CARTESIAN_POINT ( 'NONE',  ( 24.64629085034158607, 1442.486177488785188, 212.7671816332840251 ) ) ;
#48039=CARTESIAN_POINT ( 'NONE',  ( -4.500000000000000000, 1439.615672362369878, 183.5288080717980108 ) ) ;
#48040=AXIS2_PLACEMENT_3D ( 'NONE', #52276, #24810, #59014 ) ;
#48047=CARTESIAN_POINT ( 'NONE',  ( -18.06717587838990013, 1416.826860677879949, 209.3441468771879954 ) ) ;
#48048=AXIS2_PLACEMENT_3D ( 'NONE', #73811, #47498, #91688 ) ;
#48049=CARTESIAN_POINT ( 'NONE',  ( 1.514738106409309948, 1507.606285602550088, 186.2052147526660235 ) ) ;
#48050=CARTESIAN_POINT ( 'NONE',  ( 1.547463896846929865, 1414.913060387349788, 192.3096116128920130 ) ) ;
#48051=CARTESIAN_POINT ( 'NONE',  ( 11.41850631254851578, 1425.727621129565023, 138.9282626850327631 ) ) ;
#48052=DIRECTION ( 'NONE',  ( 4.137698748470009068E-18, 0.000000000000000000, 1.000000000000000000 ) ) ;
#48054=CARTESIAN_POINT ( 'NONE',  ( 17.95318235374812588, 1423.997979201475118, 225.6706602935287265 ) ) ;
#48057=CARTESIAN_POINT ( 'NONE',  ( 30.96029428649589832, 1440.913060384339815, 241.2683408943260019 ) ) ;
#48058=FACE_OUTER_BOUND ( 'NONE', #100170, .T. ) ;
#48059=FACE_OUTER_BOUND ( 'NONE', #27489, .T. ) ;
#48061=ORIENTED_EDGE ( 'NONE', *, *, #91505, .T. ) ;
#48062=CARTESIAN_POINT ( 'NONE',  ( 12.53380498098208840, 1442.773887284840384, 150.7612718761199062 ) ) ;
#48064=EDGE_CURVE ( 'NONE', #39470, #58564, #24283, .T. ) ;
#48072=CARTESIAN_POINT ( 'NONE',  ( -5.519906363166400709, 1440.499855196290127, 154.7645174855159951 ) ) ;
#48076=CARTESIAN_POINT ( 'NONE',  ( -12.73048902499999890, 1416.839648768630013, 195.1127163454979723 ) ) ;
#48077=CARTESIAN_POINT ( 'NONE',  ( 22.59589169820000265, 1507.700907224229923, 209.5602205471840023 ) ) ;
#48080=ORIENTED_EDGE ( 'NONE', *, *, #51552, .T. ) ;
#48081=CARTESIAN_POINT ( 'NONE',  ( -1.034612360689999955, 1450.827783963229876, 181.5425543420979864 ) ) ;
#48088=ORIENTED_EDGE ( 'NONE', *, *, #29505, .F. ) ;
#48090=CARTESIAN_POINT ( 'NONE',  ( 35.25381697133219205, 1437.199467842329796, 136.5363498936850135 ) ) ;
#48097=CARTESIAN_POINT ( 'NONE',  ( 18.02334845919999751, 1424.404998451829897, 224.9094352651979989 ) ) ;
#48099=CARTESIAN_POINT ( 'NONE',  ( -19.22223935719999943, 1463.238052774929884, 191.9037305475980304 ) ) ;
#48100=CARTESIAN_POINT ( 'NONE',  ( 11.86538723930000039, 1432.286167281789858, 149.9824190668979895 ) ) ;
#48102=CARTESIAN_POINT ( 'NONE',  ( -2.434305826324310029, 1449.542286390619893, 183.0300738527029978 ) ) ;
#48103=ORIENTED_EDGE ( 'NONE', *, *, #32405, .T. ) ;
#48104=ORIENTED_EDGE ( 'NONE', *, *, #82382, .T. ) ;
#48107=CARTESIAN_POINT ( 'NONE',  ( 19.03068750294750089, 1456.518195700050001, 227.4971866881460016 ) ) ;
#48110=AXIS2_PLACEMENT_3D ( 'NONE', #104697, #19013, #63285 ) ;
#48112=CARTESIAN_POINT ( 'NONE',  ( -20.24618143411970195, 1496.404372048379855, 190.7218018821779992 ) ) ;
#48113=CARTESIAN_POINT ( 'NONE',  ( 13.43167025587599817, 1509.382104656720003, 235.1752264429409820 ) ) ;
#48115=CARTESIAN_POINT ( 'NONE',  ( 0.1595984450810000177, 1486.508833535129952, 181.8147410097979844 ) ) ;
#48117=CARTESIAN_POINT ( 'NONE',  ( -45.88369462358249251, 1440.913065976889811, 266.4123280151379731 ) ) ;
#48118=CARTESIAN_POINT ( 'NONE',  ( 13.43419142301149982, 1508.291771318299880, 233.2426489798709781 ) ) ;
#48120=EDGE_CURVE ( 'NONE', #9928, #29539, #33149, .T. ) ;
#48123=CARTESIAN_POINT ( 'NONE',  ( 2.807051378689749743, 1408.949923395980022, 223.3166750014169963 ) ) ;
#48125=CARTESIAN_POINT ( 'NONE',  ( -13.44914210490000173, 1435.283433589039760, 149.9761265592980237 ) ) ;
#48130=VERTEX_POINT ( 'NONE', #94154 ) ;
#48132=CARTESIAN_POINT ( 'NONE',  ( -2.712032821819999946E-09, 1413.088571902330159, 250.5651368503980052 ) ) ;
#48133=CARTESIAN_POINT ( 'NONE',  ( -28.27621775920000147, 1508.136061367030152, 209.0190599981050070 ) ) ;
#48134=CARTESIAN_POINT ( 'NONE',  ( -3.494005144269999974, 1464.122160809730076, 182.8043410306979979 ) ) ;
#48136=CARTESIAN_POINT ( 'NONE',  ( -44.93136599389160324, 1440.913052653349951, 269.6838063022050278 ) ) ;
#48137=CARTESIAN_POINT ( 'NONE',  ( -26.57890459689999929, 1439.181835129569890, 225.2395996781980045 ) ) ;
#48139=CARTESIAN_POINT ( 'NONE',  ( -17.80061515946090012, 1452.291449208500126, 145.5827938162609883 ) ) ;
#48140=CARTESIAN_POINT ( 'NONE',  ( -18.89905520810000183, 1416.828042640230024, 207.5748962046480131 ) ) ;
#48142=CARTESIAN_POINT ( 'NONE',  ( -2.500000000000000000, 1419.382898234900267, 144.1038724149900077 ) ) ;
#48144=CARTESIAN_POINT ( 'NONE',  ( 14.73070258383249964, 1421.964157080649784, 230.3680856299650088 ) ) ;
#48150=CARTESIAN_POINT ( 'NONE',  ( -22.92652434121600180, 1409.723337951930034, 209.1949791247940027 ) ) ;
#48152=CARTESIAN_POINT ( 'NONE',  ( -0.04545031206760000164, 1419.318382049229967, 227.3945661680980095 ) ) ;
#48153=CIRCLE ( 'NONE', #110718, 2.000000000000000000 ) ;
#48156=B_SPLINE_CURVE_WITH_KNOTS ( 'NONE', 5,
 ( #71624, #72691, #63214, #88922, #48031, #73797 ),
 .UNSPECIFIED., .F., .F.,
 ( 6, 6 ),
 ( 0.000000000000000000, 1.000000000000000000 ),
 .UNSPECIFIED. ) ;
#48157=CARTESIAN_POINT ( 'NONE',  ( -21.44134523410942350, 1436.476996378036119, 143.7821035677283703 ) ) ;
#48159=EDGE_LOOP ( 'NONE', ( #19356, #75432, #23930, #90303 ) ) ;
#48160=CARTESIAN_POINT ( 'NONE',  ( 45.10266683548830002, 1448.532721670820138, 268.2401720598069801 ) ) ;
#48161=CARTESIAN_POINT ( 'NONE',  ( -12.40160425681999889, 1414.913057846380070, 220.2831263726729958 ) ) ;
#48162=CARTESIAN_POINT ( 'NONE',  ( 0.01913614526999999829, 1420.208243963930045, 183.8949348176980152 ) ) ;
#48166=CARTESIAN_POINT ( 'NONE',  ( 13.23381494117745127, 1443.155553023363836, 187.6033365495667624 ) ) ;
#48172=CARTESIAN_POINT ( 'NONE',  ( -1.247677516857949989E-10, 1452.913060387320002, 152.5211338456990120 ) ) ;
#48177=DIRECTION ( 'NONE',  ( 0.03489949670250328678, -0.9993908270190956511, 0.000000000000000000 ) ) ;
#48178=CARTESIAN_POINT ( 'NONE',  ( -13.19868063547539805, 1434.864246101540175, 149.0205925190539915 ) ) ;
#48179=DIRECTION ( 'NONE',  ( 1.056181180700544810E-06, 0.03085828021460187628, -0.9995237698729737552 ) ) ;
#48182=CARTESIAN_POINT ( 'NONE',  ( 4.838067302830000749, 1426.802081400929865, 145.9750725641980011 ) ) ;
#48183=ORIENTED_EDGE ( 'NONE', *, *, #32722, .T. ) ;
#48184=LINE ( 'NONE', #14553, #58051 ) ;
#48185=CIRCLE ( 'NONE', #91086, 1.000002391826645187 ) ;
#48188=B_SPLINE_SURFACE_WITH_KNOTS ( 'NONE', 5, 5, ( 
 ( #43523, #88823, #53033, #52481, #19390, #77666 ),
 ( #95018, #27817, #19954, #11569, #36768, #87739 ),
 ( #97215, #37323, #69285, #53593, #44631, #103390 ),
 ( #2087, #11017, #36216, #70401, #71519, #979 ),
 ( #104520, #45188, #105075, #54147, #88276, #45745 ),
 ( #18288, #86609, #9903, #78210, #22132, #13189 ),
 ( #3744, #47924, #98315, #40071, #64756, #13740 ),
 ( #22685, #73700, #48494, #12666, #82634, #56885 ),
 ( #80430, #21594, #72584, #91015, #5925, #4278 ),
 ( #99963, #107271, #31114, #65843, #37876, #74250 ),
 ( #64193, #65294, #5365, #30566, #90463, #98867 ),
 ( #108381, #82060, #39525, #107826, #81502, #99407 ) ),
 .UNSPECIFIED., .F., .F., .F.,
 ( 6, 3, 3, 6 ),
 ( 6, 6 ),
 ( 31.55396738929999856, 52.61810161070000191, 100.7782915239999966, 170.0026156580000247 ),
 ( 0.000000000000000000, 2.000000002120000175 ),
 .UNSPECIFIED. ) ;
#48194=CARTESIAN_POINT ( 'NONE',  ( -2.500000048262839947, 1439.241542145249923, 157.7315144758069891 ) ) ;
#48197=CARTESIAN_POINT ( 'NONE',  ( 11.54535135419999925, 1433.804361866699992, 151.2566013386979762 ) ) ;
#48198=CARTESIAN_POINT ( 'NONE',  ( 31.70762145559999468, 1463.873751786229832, 271.1218459616979999 ) ) ;
#48201=CARTESIAN_POINT ( 'NONE',  ( -41.66135440509999910, 1443.796918820770088, 135.6885369501979994 ) ) ;
#48203=CARTESIAN_POINT ( 'NONE',  ( 15.64949383239999925, 1417.427322289930089, 227.4411827007979809 ) ) ;
#48207=CARTESIAN_POINT ( 'NONE',  ( 17.74184486700000107, 1415.163755984130148, 210.1742778932080000 ) ) ;
#48210=CARTESIAN_POINT ( 'NONE',  ( -1.340879483539999750, 1420.508801203329995, 228.2428596365979843 ) ) ;
#48212=CARTESIAN_POINT ( 'NONE',  ( -16.63038760358159962, 1409.493779246939994, 193.2365068857160111 ) ) ;
#48216=CARTESIAN_POINT ( 'NONE',  ( -1.487490402750000218, 1415.934222462230082, 227.8159478362979939 ) ) ;
#48217=CARTESIAN_POINT ( 'NONE',  ( 0.2162845618075959764, 1453.832447077659936, 183.2176829081640221 ) ) ;
#48218=CARTESIAN_POINT ( 'NONE',  ( -13.47229708513430069, 1408.353351118039882, 210.5674428809980157 ) ) ;
#48219=CARTESIAN_POINT ( 'NONE',  ( -14.85820445100000065, 1414.971262582530017, 201.3187579297980108 ) ) ;
#48222=CARTESIAN_POINT ( 'NONE',  ( 12.40441713279999902, 1434.419921576160050, 147.2730273303979800 ) ) ;
#48223=CARTESIAN_POINT ( 'NONE',  ( -3483.362668188789939, 1009.280138338860070, 1152.220656836879698 ) ) ;
#48224=PLANE ( 'NONE',  #30034 ) ;
#48225=ORIENTED_EDGE ( 'NONE', *, *, #83167, .T. ) ;
#48230=CARTESIAN_POINT ( 'NONE',  ( -1.216112039750000040, 1452.488429528330016, 183.6485174699979837 ) ) ;
#48231=CARTESIAN_POINT ( 'NONE',  ( 13.63492191947259968, 1509.148412430130065, 233.7524217023999995 ) ) ;
#48232=CARTESIAN_POINT ( 'NONE',  ( 41.05947484210914666, 1425.981672987238881, 269.1009201124458627 ) ) ;
#48234=CARTESIAN_POINT ( 'NONE',  ( 20.17495589095351605, 1508.361608986149804, 189.3322755138515276 ) ) ;
#48235=CARTESIAN_POINT ( 'NONE',  ( 2.660639375519999739, 1425.975332079029840, 184.4015672484980257 ) ) ;
#48239=CARTESIAN_POINT ( 'NONE',  ( -27.28818755810000241, 1451.506600565129929, 136.1456173926979716 ) ) ;
#48240=CARTESIAN_POINT ( 'NONE',  ( -16.44809876050000241, 1409.864299044730160, 226.1127107795979896 ) ) ;
#48241=CARTESIAN_POINT ( 'NONE',  ( 0.4944968420529889386, 1416.123307786990154, 184.8232262612689851 ) ) ;
#48245=CARTESIAN_POINT ( 'NONE',  ( -19.21422196745478672, 1410.945657666566831, 222.5551157027674947 ) ) ;
#48247=CARTESIAN_POINT ( 'NONE',  ( -0.07319975326350189326, 1420.201854830530237, 183.6697168662389856 ) ) ;
#48248=CARTESIAN_POINT ( 'NONE',  ( 0.6994960599189999906, 1465.970851562730104, 235.7517331751979839 ) ) ;
#48250=EDGE_CURVE ( 'NONE', #98647, #25318, #38950, .T. ) ;
#48251=CARTESIAN_POINT ( 'NONE',  ( 22.01146773749999852, 1410.176833643329928, 215.5333753336580003 ) ) ;
#48252=CARTESIAN_POINT ( 'NONE',  ( -2.187094087082049665, 1417.224187196630055, 186.0756805202190094 ) ) ;
#48254=CARTESIAN_POINT ( 'NONE',  ( -16.69877117700000113, 1422.038596365629928, 226.9905822485980025 ) ) ;
#48256=CARTESIAN_POINT ( 'NONE',  ( 22.03054413761287833, 1506.491018781251569, 209.0051989547683320 ) ) ;
#48257=CARTESIAN_POINT ( 'NONE',  ( 26.29932063603849812, 1469.338010392229990, 207.9704851390930003 ) ) ;
#48260=CARTESIAN_POINT ( 'NONE',  ( -23.98763429770000144, 1430.797664492329886, 210.9021853213379813 ) ) ;
#48264=CARTESIAN_POINT ( 'NONE',  ( -17.73406580063780069, 1423.343214054229975, 226.1884525926029994 ) ) ;
#48267=CARTESIAN_POINT ( 'NONE',  ( -4.221578081139290006, 1441.603993731499941, 169.6114286483189915 ) ) ;
#48269=VERTEX_POINT ( 'NONE', #104224 ) ;
#48270=EDGE_CURVE ( 'NONE', #93372, #5163, #53677, .T. ) ;
#48276=CARTESIAN_POINT ( 'NONE',  ( 15.80576494213290317, 1409.464993575840026, 192.9618696935270066 ) ) ;
#48284=CARTESIAN_POINT ( 'NONE',  ( 36.33941889804810188, 1451.266910394200067, 134.0999999986779869 ) ) ;
#48285=DIRECTION ( 'NONE',  ( 0.03489949670246784291, -0.9993908270190968723, 0.000000000000000000 ) ) ;
#48288=CARTESIAN_POINT ( 'NONE',  ( -18.16246261389999717, 1458.250829203630019, 228.1248121254980106 ) ) ;
#48290=ORIENTED_EDGE ( 'NONE', *, *, #37186, .F. ) ;
#48294=CARTESIAN_POINT ( 'NONE',  ( -3.428224537170000197, 1485.815345808829989, 182.6034298983980193 ) ) ;
#48295=CARTESIAN_POINT ( 'NONE',  ( -2.500000000000000000, 1439.534676059920230, 164.5282244803989897 ) ) ;
#48296=ADVANCED_FACE ( 'NONE', ( #61698 ), #79589, .F. ) ;
#48301=CARTESIAN_POINT ( 'NONE',  ( 26.84000533130000221, 1441.581970243590149, 137.4710795520979900 ) ) ;
#48303=CARTESIAN_POINT ( 'NONE',  ( 1.241868258699999839, 1415.088275290029969, 191.2755884483979969 ) ) ;
#48309=CARTESIAN_POINT ( 'NONE',  ( 37.22778720889070314, 1440.913060387330006, 263.9590491429840426 ) ) ;
#48310=CARTESIAN_POINT ( 'NONE',  ( -0.0002512067421216920273, 1452.090905546908516, 153.9203152429142563 ) ) ;
#48312=CARTESIAN_POINT ( 'NONE',  ( 0.03339020944234569882, 1451.699590288030095, 183.0337632313120082 ) ) ;
#48315=B_SPLINE_CURVE_WITH_KNOTS ( 'NONE', 5,
 ( #13575, #109330, #23649, #38795, #14696, #22514, #100889, #24184, #74627, #92499, #72970, #48329 ),
 .UNSPECIFIED., .F., .F.,
 ( 6, 3, 3, 6 ),
 ( 0.000000000000000000, 0.2203430568107523080, 0.6610070094751656633, 1.000000000000000000 ),
 .UNSPECIFIED. ) ;
#48319=CARTESIAN_POINT ( 'NONE',  ( -3.549608490489999824, 1507.276797643229884, 180.9704965481979855 ) ) ;
#48322=CARTESIAN_POINT ( 'NONE',  ( 13.91727111200000166, 1462.334475154630127, 230.6050055265979779 ) ) ;
#48323=DIRECTION ( 'NONE',  ( 0.03489949670250328678, -0.9993908270190956511, 0.000000000000000000 ) ) ;
#48324=CARTESIAN_POINT ( 'NONE',  ( -0.5133638609672289688, 1410.311096993930050, 233.1717005261690190 ) ) ;
#48325=AXIS2_PLACEMENT_3D ( 'NONE', #12937, #47118, #39247 ) ;
#48328=ORIENTED_EDGE ( 'NONE', *, *, #44360, .T. ) ;
#48329=CARTESIAN_POINT ( 'NONE',  ( -22.57319772750419773, 1409.701314710050156, 209.4509374963450057 ) ) ;
#48330=CARTESIAN_POINT ( 'NONE',  ( -0.1280106238597930046, 1507.928448683369879, 180.6911020812059689 ) ) ;
#48336=DIRECTION ( 'NONE',  ( 0.000000000000000000, -1.000000000000000000, 0.000000000000000000 ) ) ;
#48337=AXIS2_PLACEMENT_3D ( 'NONE', #71449, #62488, #53517 ) ;
#48338=CARTESIAN_POINT ( 'NONE',  ( 11.62345946000000119, 1459.569834436530073, 221.5884500235979999 ) ) ;
#48339=CARTESIAN_POINT ( 'NONE',  ( -10.94036871930000032, 1430.241478036630042, 151.4665561441980230 ) ) ;
#48342=CARTESIAN_POINT ( 'NONE',  ( 3.181555627136920084, 1425.362660434019972, 153.9433711340520290 ) ) ;
#48344=CARTESIAN_POINT ( 'NONE',  ( 12.59782697949999886, 1446.921545761879770, 188.3055334180980083 ) ) ;
#48345=CARTESIAN_POINT ( 'NONE',  ( -19.18209465460000018, 1457.448691500030009, 226.5728852009980017 ) ) ;
#48348=ORIENTED_EDGE ( 'NONE', *, *, #17290, .F. ) ;
#48350=CARTESIAN_POINT ( 'NONE',  ( 3.713169866679999931, 1406.888986113030114, 269.6455940986979840 ) ) ;
#48351=CARTESIAN_POINT ( 'NONE',  ( 0.1681183307230000035, 1408.918931226930226, 186.0198301081979935 ) ) ;
#48352=CARTESIAN_POINT ( 'NONE',  ( 17.99612260190000157, 1410.880106602829983, 193.4662733174980076 ) ) ;
#48353=CARTESIAN_POINT ( 'NONE',  ( 22.64711134129722225, 1431.381828419114072, 216.8252444415483922 ) ) ;
#48355=CARTESIAN_POINT ( 'NONE',  ( 26.88907266892866943, 1508.006188459404939, 215.2210763183871052 ) ) ;
#48357=CARTESIAN_POINT ( 'NONE',  ( -1.967245096925249737, 1450.337415777349861, 154.7913169777050086 ) ) ;
#48358=FACE_OUTER_BOUND ( 'NONE', #47466, .T. ) ;
#48359=CARTESIAN_POINT ( 'NONE',  ( 1.181727162679999887, 1450.812795825049989, 155.6080914332980001 ) ) ;
#48360=CARTESIAN_POINT ( 'NONE',  ( -14.43876446305799988, 1416.576002138890090, 221.3723411449140031 ) ) ;
#48364=CARTESIAN_POINT ( 'NONE',  ( -19.62446893450000118, 1438.771933937510084, 214.3676144203579952 ) ) ;
#48365=CARTESIAN_POINT ( 'NONE',  ( -26.88341108264370050, 1508.006303180540044, 211.8628327196680061 ) ) ;
#48366=FACE_OUTER_BOUND ( 'NONE', #20551, .T. ) ;
#48367=CARTESIAN_POINT ( 'NONE',  ( -6.133610941629999758, 1475.021496988630133, 269.4856170435980403 ) ) ;
#48368=CARTESIAN_POINT ( 'NONE',  ( -4.237127966724729689, 1446.355013308460002, 163.3938685498860366 ) ) ;
#48370=CARTESIAN_POINT ( 'NONE',  ( -11.39147210054831305, 1486.510883767746691, 184.0968824713255856 ) ) ;
#48373=CIRCLE ( 'NONE', #68046, 1.999999999999990452 ) ;
#48375=B_SPLINE_CURVE_WITH_KNOTS ( 'NONE', 3,
 ( #41785, #33370, #67564, #24957, #25514, #59166, #77059, #26063, #60258, #29388, #61382 ),
 .UNSPECIFIED., .F., .F.,
 ( 4, 2, 1, 2, 2, 4 ),
 ( 0.000000000000000000, 0.2500000000007147616, 0.3750000000009557910, 0.4375000000011197709, 0.5000000000012837509, 1.000000000000000000 ),
 .UNSPECIFIED. ) ;
#48379=CARTESIAN_POINT ( 'NONE',  ( -18.87340472369999844, 1410.495304298229939, 196.4667987001980123 ) ) ;
#48380=CARTESIAN_POINT ( 'NONE',  ( -15.03298775838899992, 1422.459395939136130, 229.1221294577470076 ) ) ;
#48381=CARTESIAN_POINT ( 'NONE',  ( 11.14671379024469999, 1434.019377051509991, 151.6529839732360188 ) ) ;
#48382=EDGE_CURVE ( 'NONE', #66538, #11383, #8206, .T. ) ;
#48390=CARTESIAN_POINT ( 'NONE',  ( 11.89909614660000159, 1409.328585981029846, 191.4548601458980102 ) ) ;
#48395=CARTESIAN_POINT ( 'NONE',  ( -11.34254097917190585, 1398.249336051535238, 202.7613412656716037 ) ) ;
#48404=CARTESIAN_POINT ( 'NONE',  ( 0.001991325594910000121, 1395.912990848730033, 220.4358217525980024 ) ) ;
#48405=CARTESIAN_POINT ( 'NONE',  ( -18.77065511170000178, 1409.568546107730072, 220.1541561005979872 ) ) ;
#48407=CARTESIAN_POINT ( 'NONE',  ( -12.66067528227170946, 1445.026872531248500, 169.4635260004347970 ) ) ;
#48408=CARTESIAN_POINT ( 'NONE',  ( 21.81321449130158285, 1509.707650915029944, 229.2662883381179029 ) ) ;
#48415=EDGE_CURVE ( 'NONE', #28591, #81651, #32225, .T. ) ;
#48418=CARTESIAN_POINT ( 'NONE',  ( 9.437563379819911447, 1396.242627386850018, 203.3496504048309816 ) ) ;
#48419=CARTESIAN_POINT ( 'NONE',  ( 1.352297191989999980, 1415.128105759529944, 191.2895120243979932 ) ) ;
#48420=CARTESIAN_POINT ( 'NONE',  ( 11.25794562449999958, 1429.128833963630086, 150.7790970959979973 ) ) ;
#48422=ORIENTED_EDGE ( 'NONE', *, *, #37258, .T. ) ;
#48423=CARTESIAN_POINT ( 'NONE',  ( 13.56071599880170098, 1435.044469485500031, 149.3995586837050098 ) ) ;
#48429=CARTESIAN_POINT ( 'NONE',  ( -13.53625262109999916, 1461.948139420029975, 230.2268504220980105 ) ) ;
#48436=CARTESIAN_POINT ( 'NONE',  ( -11.77320467545210114, 1509.437369347079994, 181.3954167328170115 ) ) ;
#48446=CARTESIAN_POINT ( 'NONE',  ( -13.59758770590147492, 1411.972790166096502, 269.3580573342126172 ) ) ;
#48447=CARTESIAN_POINT ( 'NONE',  ( -0.8853909531090000673, 1410.323732749430064, 233.0849705860979952 ) ) ;
#48448=CARTESIAN_POINT ( 'NONE',  ( -11.89850863680000082, 1497.713060387329961, 190.2034600782980078 ) ) ;
#48449=VERTEX_POINT ( 'NONE', #39775 ) ;
#48451=CARTESIAN_POINT ( 'NONE',  ( -34.33105695552479375, 1440.913060389319980, 249.5635140075729907 ) ) ;
#48453=CARTESIAN_POINT ( 'NONE',  ( -0.2569123757260329821, 1466.030216462040016, 235.8399092281299829 ) ) ;
#48454=CARTESIAN_POINT ( 'NONE',  ( 5.151086705716080516, 1410.620189125909974, 269.3380098377049876 ) ) ;
#48457=CARTESIAN_POINT ( 'NONE',  ( 22.88862305450000179, 1409.720888560930007, 208.9462140200429872 ) ) ;
#48458=CARTESIAN_POINT ( 'NONE',  ( -20.28810075950000069, 1508.873707194230064, 188.9657859483980076 ) ) ;
#48464=CARTESIAN_POINT ( 'NONE',  ( -14.34315653738819485, 1486.055971446375679, 185.9291880012369234 ) ) ;
#48466=VERTEX_POINT ( 'NONE', #30254 ) ;
#48468=CARTESIAN_POINT ( 'NONE',  ( 18.96271102769999928, 1416.819759739330038, 210.2433116420780266 ) ) ;
#48471=CARTESIAN_POINT ( 'NONE',  ( -13.67687855990000045, 1421.535259874829990, 230.0823906799980136 ) ) ;
#48474=CARTESIAN_POINT ( 'NONE',  ( -11.87275636863970085, 1432.783179063080070, 147.6501916617970096 ) ) ;
#48477=CARTESIAN_POINT ( 'NONE',  ( -21.99779490583109975, 1409.845346897619947, 211.9582521639920003 ) ) ;
#48481=CARTESIAN_POINT ( 'NONE',  ( 27.96976558946629865, 1509.201555284690130, 207.5796322897400046 ) ) ;
#48482=ORIENTED_EDGE ( 'NONE', *, *, #63202, .T. ) ;
#48484=CARTESIAN_POINT ( 'NONE',  ( 22.12750824849999987, 1452.642887229430244, 220.0678107083980137 ) ) ;
#48488=CARTESIAN_POINT ( 'NONE',  ( 7.212015265482224713, 1416.834466888146380, 231.0122356860012474 ) ) ;
#48490=CARTESIAN_POINT ( 'NONE',  ( -4.220206612590000184, 1446.210882134589838, 168.9980572494979754 ) ) ;
#48491=CARTESIAN_POINT ( 'NONE',  ( -19.54046289729999941, 1426.642498283530131, 224.7160149891979870 ) ) ;
#48492=CARTESIAN_POINT ( 'NONE',  ( -23.41403251080000203, 1435.314950308189964, 138.7792008531980059 ) ) ;
#48494=CARTESIAN_POINT ( 'NONE',  ( 18.31256684599999929, 1461.935672362830019, 190.2221303580979850 ) ) ;
#48496=CARTESIAN_POINT ( 'NONE',  ( -16.13319535987753284, 1469.080883781242164, 269.3696318216189525 ) ) ;
#48497=ORIENTED_EDGE ( 'NONE', *, *, #18482, .T. ) ;
#48499=CARTESIAN_POINT ( 'NONE',  ( 14.30333092830361075, 1506.380977037114235, 192.4362132687745941 ) ) ;
#48502=CARTESIAN_POINT ( 'NONE',  ( -7.215398911020000305, 1408.913060387329779, 225.6058586963979735 ) ) ;
#48503=CARTESIAN_POINT ( 'NONE',  ( -0.2286327670369999732, 1416.983677237929896, 234.1874105466980041 ) ) ;
#48504=CARTESIAN_POINT ( 'NONE',  ( -13.07753579797488896, 1443.006526933015039, 186.6367630675282214 ) ) ;
#48505=DIRECTION ( 'NONE',  ( 0.9822959463215400477, 0.1391731009607420078, -0.1254014426122810055 ) ) ;
#48510=CARTESIAN_POINT ( 'NONE',  ( 25.06810116750000006, 1436.599588250250008, 137.8027482626980031 ) ) ;
#48512=CARTESIAN_POINT ( 'NONE',  ( -13.30361737529999999, 1409.377632944630022, 226.2974604263980041 ) ) ;
#48516=ORIENTED_EDGE ( 'NONE', *, *, #69339, .T. ) ;
#48518=CARTESIAN_POINT ( 'NONE',  ( 17.85664671351629806, 1415.933499560010205, 208.9473542036010087 ) ) ;
#48522=CARTESIAN_POINT ( 'NONE',  ( -24.09667683720000042, 1455.346816438730002, 238.1639138257980051 ) ) ;
#48523=CARTESIAN_POINT ( 'NONE',  ( -20.10488467649999933, 1503.697545318330185, 189.3141326410979843 ) ) ;
#48524=CARTESIAN_POINT ( 'NONE',  ( -11.88526705700000008, 1433.193525880590187, 149.9681886515980125 ) ) ;
#48526=CARTESIAN_POINT ( 'NONE',  ( -27.69925887780000195, 1441.434395789990049, 137.3015763680980115 ) ) ;
#48527=CARTESIAN_POINT ( 'NONE',  ( -11.58478124459999847, 1415.063410489729904, 195.8970895505979968 ) ) ;
#48529=CARTESIAN_POINT ( 'NONE',  ( 1.167020444750000108, 1450.781019595759972, 181.8366706930980001 ) ) ;
#48532=CARTESIAN_POINT ( 'NONE',  ( -10.09491806113956791, 1509.391460115556811, 237.3755645815038235 ) ) ;
#48533=CARTESIAN_POINT ( 'NONE',  ( 4.873133187124399707E-09, 1406.012954286680042, 266.9164466110329954 ) ) ;
#48536=EDGE_CURVE ( 'NONE', #91965, #109427, #41556, .T. ) ;
#48539=CARTESIAN_POINT ( 'NONE',  ( -4.814686654720000902, 1471.386640766029814, 269.6174199348980096 ) ) ;
#48541=CARTESIAN_POINT ( 'NONE',  ( 9.400735251840000473, 1432.346452651970139, 153.1462979580980175 ) ) ;
#48543=CARTESIAN_POINT ( 'NONE',  ( 35.68489934706420286, 1450.614492635629858, 136.1526271777700288 ) ) ;
#48544=CARTESIAN_POINT ( 'NONE',  ( 0.2255011766491570036, 1451.657143026270205, 182.8204767894659994 ) ) ;
#48545=CARTESIAN_POINT ( 'NONE',  ( 19.30812218469289121, 1456.473178130213682, 228.7018492185203797 ) ) ;
#48546=EDGE_CURVE ( 'NONE', #63032, #8806, #57015, .T. ) ;
#48550=CARTESIAN_POINT ( 'NONE',  ( -33.35109133253590130, 1416.979667404030124, 269.1074273680090414 ) ) ;
#48551=ORIENTED_EDGE ( 'NONE', *, *, #34273, .T. ) ;
#48552=CARTESIAN_POINT ( 'NONE',  ( -3.539264903962820341, 1497.294491324139926, 181.3958076714880008 ) ) ;
#48553=VERTEX_POINT ( 'NONE', #109195 ) ;
#48557=CARTESIAN_POINT ( 'NONE',  ( 4.436453144186142339, 1423.828612835836338, 183.6460411026642703 ) ) ;
#48558=CARTESIAN_POINT ( 'NONE',  ( 40.92391338726710615, 1444.178192375350136, 136.9148929651390176 ) ) ;
#48561=CARTESIAN_POINT ( 'NONE',  ( -16.89981363069999887, 1455.454529709330018, 189.6846976769979847 ) ) ;
#48562=CARTESIAN_POINT ( 'NONE',  ( -2.281512216559187234, 1449.806067081884976, 182.9567416777415190 ) ) ;
#48564=CARTESIAN_POINT ( 'NONE',  ( -26.49085951069999822, 1436.258304344430144, 136.6654738169979737 ) ) ;
#48568=VECTOR ( 'NONE', #27256, 1000.000000000000114 ) ;
#48570=CARTESIAN_POINT ( 'NONE',  ( 0.01096402816149999980, 1407.225809180230044, 196.1218459610979892 ) ) ;
#48571=DIRECTION ( 'NONE',  ( 0.7067700363771036720, 0.03085824620770448445, -0.7067700363771035610 ) ) ;
#48572=CARTESIAN_POINT ( 'NONE',  ( -6.240887331089999712, 1397.787773551729970, 197.7178372010980070 ) ) ;
#48576=CARTESIAN_POINT ( 'NONE',  ( 0.2959633938429999667, 1452.979674875830142, 183.2640183118980133 ) ) ;
#48577=CARTESIAN_POINT ( 'NONE',  ( 3.752275789878676271, 1425.500837115214381, 185.1933876786509074 ) ) ;
#48579=CARTESIAN_POINT ( 'NONE',  ( -14.55974755836840018, 1436.247439882689832, 149.8925174081419982 ) ) ;
#48580=CARTESIAN_POINT ( 'NONE',  ( -0.03728113298654189833, 1409.749267624750019, 185.1545790610279880 ) ) ;
#48584=CARTESIAN_POINT ( 'NONE',  ( -2.549249301710439841, 1484.259727321469882, 183.2432226763939980 ) ) ;
#48592=CARTESIAN_POINT ( 'NONE',  ( -23.99652642515154000, 1445.345535593930663, 212.5605566193962943 ) ) ;
#48593=ORIENTED_EDGE ( 'NONE', *, *, #46294, .F. ) ;
#48595=CARTESIAN_POINT ( 'NONE',  ( 12.84218287614169896, 1435.936370184710086, 150.8117598946369924 ) ) ;
#48596=CARTESIAN_POINT ( 'NONE',  ( 13.31050682230000071, 1414.983773854429955, 197.8499836438979855 ) ) ;
#48597=CARTESIAN_POINT ( 'NONE',  ( -2.197413362389999847, 1507.220826622230106, 180.8381795179979861 ) ) ;
#48598=CARTESIAN_POINT ( 'NONE',  ( 12.72284891840000043, 1416.311719779230089, 222.6852781584979653 ) ) ;
#48599=CARTESIAN_POINT ( 'NONE',  ( 17.00063747520000135, 1410.433676325329998, 226.2701375890979989 ) ) ;
#48602=CARTESIAN_POINT ( 'NONE',  ( 24.03875944314501112, 1447.055054376208773, 215.2337187572886705 ) ) ;
#48606=VERTEX_POINT ( 'NONE', #13437 ) ;
#48608=STYLED_ITEM ( 'NONE', ( #62922 ), #43980 ) ;
#48609=CARTESIAN_POINT ( 'NONE',  ( -34.89169900679999614, 1462.401046348830278, 269.8669090264980355 ) ) ;
#48610=CARTESIAN_POINT ( 'NONE',  ( 0.6438251882000000093, 1419.376757820729836, 184.7188999000980232 ) ) ;
#48612=ADVANCED_FACE ( 'NONE', ( #83416 ), #98563, .F. ) ;
#48615=CARTESIAN_POINT ( 'NONE',  ( 30.39553402230279744, 1509.974493418120119, 207.3314266928840084 ) ) ;
#48617=CARTESIAN_POINT ( 'NONE',  ( 2.488503644649960655, 1417.702710168876592, 233.7328821538343107 ) ) ;
#48618=CARTESIAN_POINT ( 'NONE',  ( -2.500000000000000000, 1419.383100980419840, 144.1003751433630100 ) ) ;
#48621=CARTESIAN_POINT ( 'NONE',  ( 8.742163716520650412E-12, 1408.913060387359792, 224.1216835645979870 ) ) ;
#48622=CARTESIAN_POINT ( 'NONE',  ( 29.80083709734149977, 1440.913060386300003, 237.7077141819719657 ) ) ;
#48626=CARTESIAN_POINT ( 'NONE',  ( 12.95579922760000002, 1419.891847053030006, 221.9576903087979929 ) ) ;
#48628=ORIENTED_EDGE ( 'NONE', *, *, #48536, .T. ) ;
#48630=CARTESIAN_POINT ( 'NONE',  ( -19.67913117755652053, 1485.239616831768444, 190.3362610098068615 ) ) ;
#48636=DIRECTION ( 'NONE',  ( 0.000000000000000000, 0.000000000000000000, 1.000000000000000000 ) ) ;
#48640=CARTESIAN_POINT ( 'NONE',  ( -15.30113400179999772, 1507.624001450029937, 191.9539244739980006 ) ) ;
#48641=EDGE_CURVE ( 'NONE', #110334, #7633, #69714, .T. ) ;
#48642=CYLINDRICAL_SURFACE ( 'NONE', #37519, 1.999999999999915179 ) ;
#48650=VERTEX_POINT ( 'NONE', #30810 ) ;
#48653=CARTESIAN_POINT ( 'NONE',  ( 0.8266031666246391740, 1416.818673872118779, 190.2123423678451957 ) ) ;
#48655=DIRECTION ( 'NONE',  ( 0.000000000000000000, 1.000000000000000000, 0.000000000000000000 ) ) ;
#48656=CARTESIAN_POINT ( 'NONE',  ( -0.5624690339869999889, 1416.828040475229955, 227.7677324846980014 ) ) ;
#48662=CARTESIAN_POINT ( 'NONE',  ( 18.80400137410000028, 1425.877418581729899, 225.3118762411980072 ) ) ;
#48665=CARTESIAN_POINT ( 'NONE',  ( 11.76924708519999996, 1432.318127532269955, 150.8119212265980025 ) ) ;
#48667=CARTESIAN_POINT ( 'NONE',  ( -22.52609268272879817, 1509.699688877640028, 190.9355248210520131 ) ) ;
#48668=VERTEX_POINT ( 'NONE', #75043 ) ;
#48669=CARTESIAN_POINT ( 'NONE',  ( 1.632486301776860348E-07, 1509.047264794319972, 239.1218459617020073 ) ) ;
#48670=CARTESIAN_POINT ( 'NONE',  ( -10.86013104807563145, 1428.709904399815287, 134.0999999980980419 ) ) ;
#48672=CARTESIAN_POINT ( 'NONE',  ( -12.40096745299999981, 1434.347023119479900, 149.5501479441980166 ) ) ;
#48674=CARTESIAN_POINT ( 'NONE',  ( -20.46943290138029781, 1503.635669217179839, 190.5120838222930217 ) ) ;
#48675=ADVANCED_FACE ( 'NONE', ( #64987 ), #47085, .F. ) ;
#48678=CARTESIAN_POINT ( 'NONE',  ( 17.40764059099999628, 1414.996444526030018, 210.6782161193179945 ) ) ;
#48681=CARTESIAN_POINT ( 'NONE',  ( -22.72361261936710264, 1432.255920656152057, 217.6431712202583526 ) ) ;
#48682=CARTESIAN_POINT ( 'NONE',  ( 14.06807837553630058, 1452.482298946410083, 222.8064072038120003 ) ) ;
#48684=FACE_OUTER_BOUND ( 'NONE', #49138, .T. ) ;
#48685=CARTESIAN_POINT ( 'NONE',  ( 13.40566205669149902, 1429.098591087019940, 222.0107402452829888 ) ) ;
#48689=CARTESIAN_POINT ( 'NONE',  ( 31.95512683039999757, 1440.913060396209858, 244.1805851198980122 ) ) ;
#48690=CARTESIAN_POINT ( 'NONE',  ( -28.34110756850000001, 1508.137170135529914, 209.4584315255609965 ) ) ;
#48691=CARTESIAN_POINT ( 'NONE',  ( 0.5190711711569999665, 1464.113131884229915, 182.7836423421979930 ) ) ;
#48692=CARTESIAN_POINT ( 'NONE',  ( -17.59077195540000105, 1410.452734757129747, 194.3251796273980005 ) ) ;
#48694=CARTESIAN_POINT ( 'NONE',  ( -20.53795889179999890, 1428.561159746129988, 220.8089596197980029 ) ) ;
#48696=CARTESIAN_POINT ( 'NONE',  ( -20.21385637174950034, 1452.207176968400063, 142.9987421525109994 ) ) ;
#48697=CARTESIAN_POINT ( 'NONE',  ( 21.25708630131437360, 1435.239819464457241, 139.1347687464948137 ) ) ;
#48698=EDGE_LOOP ( 'NONE', ( #70932, #50264, #32192, #90547, #8578, #1187, #35826, #12487, #67526, #15406, #81717, #80637, #16946, #78575 ) ) ;
#48701=CARTESIAN_POINT ( 'NONE',  ( 16.80536496183709971, 1423.594528387539867, 228.4229711109250047 ) ) ;
#48704=ORIENTED_EDGE ( 'NONE', *, *, #77360, .F. ) ;
#48706=CARTESIAN_POINT ( 'NONE',  ( -24.11864498019999914, 1411.115042655630077, 209.4126620446369884 ) ) ;
#48707=EDGE_CURVE ( 'NONE', #38935, #102287, #38754, .T. ) ;
#48708=CARTESIAN_POINT ( 'NONE',  ( -3.827327107099999903, 1424.046157849130168, 184.1455919444979656 ) ) ;
#48712=CARTESIAN_POINT ( 'NONE',  ( -7.586230254490000213, 1507.634635854029966, 235.4684484327979987 ) ) ;
#48713=CARTESIAN_POINT ( 'NONE',  ( -17.47806757639999731, 1410.883707539230045, 225.6330995444980090 ) ) ;
#48715=CARTESIAN_POINT ( 'NONE',  ( 41.96559968512650585, 1455.508381183140045, 266.8112211961390017 ) ) ;
#48720=DIRECTION ( 'NONE',  ( 0.3363363969981410517, -0.6659120918163093927, 0.6659120918162816372 ) ) ;
#48722=CARTESIAN_POINT ( 'NONE',  ( 13.03096333729283529, 1442.971155689919669, 187.2524364873846707 ) ) ;
#48724=ORIENTED_EDGE ( 'NONE', *, *, #505, .T. ) ;
#48725=CARTESIAN_POINT ( 'NONE',  ( 2.995039991590000117, 1448.960486182170143, 183.8207280578979805 ) ) ;
#48731=CARTESIAN_POINT ( 'NONE',  ( -4.161170142461470434, 1448.299083512420111, 185.1109003841999936 ) ) ;
#48733=DIRECTION ( 'NONE',  ( 0.000000000000000000, 0.000000000000000000, 1.000000000000000000 ) ) ;
#48734=CARTESIAN_POINT ( 'NONE',  ( -16.68466689124240077, 1411.595104653460112, 191.7171691803239924 ) ) ;
#48735=CARTESIAN_POINT ( 'NONE',  ( 16.27110347889999886, 1489.469559537029909, 194.1428897389979795 ) ) ;
#48737=CARTESIAN_POINT ( 'NONE',  ( -25.45358342560510323, 1509.770361827349916, 222.9816713348759833 ) ) ;
#48739=CARTESIAN_POINT ( 'NONE',  ( 11.76598840989999850, 1428.979790717830156, 145.3128034382980047 ) ) ;
#48741=CARTESIAN_POINT ( 'NONE',  ( 15.71554773450000297, 1429.441490238930101, 224.8635561783979711 ) ) ;
#48750=EDGE_CURVE ( 'NONE', #30887, #33927, #9474, .T. ) ;
#48753=CARTESIAN_POINT ( 'NONE',  ( -13.58256621920000029, 1416.843576365230092, 221.9093687442980070 ) ) ;
#48754=CARTESIAN_POINT ( 'NONE',  ( 11.34078683589999947, 1433.855572862709778, 151.4803113887979862 ) ) ;
#48755=CARTESIAN_POINT ( 'NONE',  ( 43.50000000000000000, 1440.913060387330006, 271.1218459616979999 ) ) ;
#48757=CARTESIAN_POINT ( 'NONE',  ( -11.60004869885203860, 1428.971947790929107, 136.1000015555673599 ) ) ;
#48759=CARTESIAN_POINT ( 'NONE',  ( -4.963802804109999300, 1497.713060387329961, 230.9126810519979927 ) ) ;
#48762=DIRECTION ( 'NONE',  ( 0.3390050494208932674, 0.7071067811868654296, 0.6205445805634662859 ) ) ;
#48763=CARTESIAN_POINT ( 'NONE',  ( -17.57236383969999949, 1410.451431512329918, 225.4462110255979894 ) ) ;
#48768=CARTESIAN_POINT ( 'NONE',  ( 6.866540673400110493E-07, 1408.860257358530134, 194.6498732444090081 ) ) ;
#48769=CARTESIAN_POINT ( 'NONE',  ( 11.17826893112730957, 1434.135999025848378, 151.6295705600838062 ) ) ;
#48771=CARTESIAN_POINT ( 'NONE',  ( -5.548131016090000145, 1414.913060387229962, 224.8407497847980210 ) ) ;
#48773=CARTESIAN_POINT ( 'NONE',  ( 0.2074342776960350077, 1458.792499532430156, 183.0048892579440007 ) ) ;
#48774=CARTESIAN_POINT ( 'NONE',  ( 23.55087631299999984, 1411.110694763729953, 207.7642880164279973 ) ) ;
#48775=ORIENTED_EDGE ( 'NONE', *, *, #13885, .F. ) ;
#48776=CARTESIAN_POINT ( 'NONE',  ( 1.530052826864370052, 1452.704406626560058, 183.4894965714629791 ) ) ;
#48778=CARTESIAN_POINT ( 'NONE',  ( 11.87922978499999971, 1433.311594856540069, 149.1894924501980313 ) ) ;
#48779=CARTESIAN_POINT ( 'NONE',  ( -40.85417709071609949, 1440.196123997409813, 134.0999999980799657 ) ) ;
#48783=ADVANCED_FACE ( 'NONE', ( #67746 ), #77248, .F. ) ;
#48788=EDGE_CURVE ( 'NONE', #98856, #69002, #20113, .T. ) ;
#48789=CARTESIAN_POINT ( 'NONE',  ( 18.22805055419890152, 1459.311389626190021, 227.8763770136359881 ) ) ;
#48791=CARTESIAN_POINT ( 'NONE',  ( 45.63713418245465903, 1439.235619164679065, 268.9747475081824746 ) ) ;
#48794=CARTESIAN_POINT ( 'NONE',  ( 2.985881150139999995, 1431.471105595659992, 184.5967258471980017 ) ) ;
#48799=CARTESIAN_POINT ( 'NONE',  ( -28.61821586814939877, 1509.224669311890011, 208.7631243191599992 ) ) ;
#48800=CARTESIAN_POINT ( 'NONE',  ( -15.94765147786550052, 1409.469968486390144, 225.3462237114930247 ) ) ;
#48801=CARTESIAN_POINT ( 'NONE',  ( 0.5031299281221360831, 1413.437613018619913, 184.9381903630110173 ) ) ;
#48802=ORIENTED_EDGE ( 'NONE', *, *, #91174, .T. ) ;
#48805=CARTESIAN_POINT ( 'NONE',  ( 21.04382134430000306, 1508.388118399029963, 226.0922268082980224 ) ) ;
#48807=CARTESIAN_POINT ( 'NONE',  ( -0.08869625257939200980, 1419.939914807589957, 184.0372427730129914 ) ) ;
#48808=CARTESIAN_POINT ( 'NONE',  ( 1.221557978829999946, 1466.110857312230110, 235.2972512431979908 ) ) ;
#48809=CARTESIAN_POINT ( 'NONE',  ( 18.44309112110000015, 1409.721912672129974, 221.4648865221980145 ) ) ;
#48811=CARTESIAN_POINT ( 'NONE',  ( -16.97269670290000221, 1423.671420843229953, 228.0577291709979875 ) ) ;
#48813=CARTESIAN_POINT ( 'NONE',  ( -2.500000000000000000, 1439.615672362210034, 183.5288080682979910 ) ) ;
#48817=CARTESIAN_POINT ( 'NONE',  ( -1.377961559329999863, 1416.217220538330139, 233.2979951139980130 ) ) ;
#48820=CARTESIAN_POINT ( 'NONE',  ( -17.69798016750000258, 1424.268916621029803, 226.8670750680979893 ) ) ;
#48823=CARTESIAN_POINT ( 'NONE',  ( -4.239667262353160382, 1441.443752683740058, 162.8307151194100015 ) ) ;
#48826=ORIENTED_EDGE ( 'NONE', *, *, #4504, .T. ) ;
#48827=ADVANCED_FACE ( 'NONE', ( #548 ), #92921, .F. ) ;
#48829=VERTEX_POINT ( 'NONE', #78339 ) ;
#48832=CARTESIAN_POINT ( 'NONE',  ( -11.64262758805663545, 1425.861298859939552, 144.5853139168677046 ) ) ;
#48833=CARTESIAN_POINT ( 'NONE',  ( 15.85187002026029823, 1410.856221003509972, 191.5210852716889747 ) ) ;
#48836=CARTESIAN_POINT ( 'NONE',  ( 36.40062700991159517, 1436.005110244360139, 135.0217463105349793 ) ) ;
#48840=CARTESIAN_POINT ( 'NONE',  ( 11.21601427816997720, 1464.187623198618212, 231.8855071244460646 ) ) ;
#48842=CARTESIAN_POINT ( 'NONE',  ( 39.34220581737610445, 1449.349331648660154, 134.0999999980729740 ) ) ;
#48843=CARTESIAN_POINT ( 'NONE',  ( -26.86204968941349946, 1508.007394745769943, 212.0120970035400205 ) ) ;
#48846=CARTESIAN_POINT ( 'NONE',  ( -18.59366615780000132, 1458.580092697230157, 227.5321056525980055 ) ) ;
#48849=CARTESIAN_POINT ( 'NONE',  ( 16.66094735743510213, 1410.867388111209948, 226.5061907891179942 ) ) ;
#48851=EDGE_CURVE ( 'NONE', #89451, #59085, #46321, .T. ) ;
#48852=CARTESIAN_POINT ( 'NONE',  ( 0.1797482706320000234, 1451.166081239530058, 182.5410796217979907 ) ) ;
#48853=CARTESIAN_POINT ( 'NONE',  ( -2.987575625429999882, 1484.703021631029969, 183.3076216214979866 ) ) ;
#48854=CARTESIAN_POINT ( 'NONE',  ( -2.500000000000000000, 1439.621629191349939, 170.0481657697840205 ) ) ;
#48856=CARTESIAN_POINT ( 'NONE',  ( -2.500000000000000000, 1448.210448412289907, 183.1418046154980175 ) ) ;
#48857=CARTESIAN_POINT ( 'NONE',  ( 33.91369104887559871, 1451.728768199629940, 135.6938360226120039 ) ) ;
#48859=CARTESIAN_POINT ( 'NONE',  ( 25.85996285490000091, 1436.538141094960110, 136.9113464714980068 ) ) ;
#48860=CARTESIAN_POINT ( 'NONE',  ( 5.548131867839999565, 1414.913060387229962, 193.4029425950980112 ) ) ;
#48866=CARTESIAN_POINT ( 'NONE',  ( 33.53994528179689638, 1440.913060387330006, 258.5778273533969696 ) ) ;
#48868=FACE_OUTER_BOUND ( 'NONE', #22233, .T. ) ;
#48869=EDGE_LOOP ( 'NONE', ( #61611, #110674, #100793, #79355, #83628 ) ) ;
#48870=CARTESIAN_POINT ( 'NONE',  ( -0.05401770104373219972, 1452.351257629399925, 183.2652781389920165 ) ) ;
#48874=CARTESIAN_POINT ( 'NONE',  ( -13.20685506100000062, 1422.970547187230068, 222.0985264004979740 ) ) ;
#48876=CARTESIAN_POINT ( 'NONE',  ( 13.07458372279550041, 1436.035484542389895, 150.7116094860570001 ) ) ;
#48877=CARTESIAN_POINT ( 'NONE',  ( -0.8107957177449999220, 1507.658530268329969, 180.8255026719979810 ) ) ;
#48878=CARTESIAN_POINT ( 'NONE',  ( -11.94171318070000076, 1433.614828344400166, 146.4341822532980188 ) ) ;
#48880=CARTESIAN_POINT ( 'NONE',  ( 15.43028253750000189, 1459.840836958929913, 230.9090760540979943 ) ) ;
#48881=CARTESIAN_POINT ( 'NONE',  ( -10.16646205815034953, 1422.467730556536253, 137.0999999980976725 ) ) ;
#48886=CARTESIAN_POINT ( 'NONE',  ( -0.05571092667383620300, 1508.705957002570130, 179.9923125561219877 ) ) ;
#48890=CARTESIAN_POINT ( 'NONE',  ( -11.60004869885203682, 1426.109592824957417, 139.1549331605903035 ) ) ;
#48892=VERTEX_POINT ( 'NONE', #45313 ) ;
#48895=EDGE_CURVE ( 'NONE', #103816, #33631, #67720, .T. ) ;
#48896=CARTESIAN_POINT ( 'NONE',  ( -11.86497210549999970, 1432.257141527180011, 149.9820204226980138 ) ) ;
#48897=CARTESIAN_POINT ( 'NONE',  ( 19.13240566025299927, 1456.933378143550044, 225.0294012906809940 ) ) ;
#48901=CARTESIAN_POINT ( 'NONE',  ( 12.13521690389999996, 1446.772554461140089, 188.0265662329979932 ) ) ;
#48903=CARTESIAN_POINT ( 'NONE',  ( -24.77779169540000126, 1482.720791717229986, 217.1592320706580210 ) ) ;
#48905=CARTESIAN_POINT ( 'NONE',  ( -2.446862982530000341, 1485.861691786529946, 182.3251207059980175 ) ) ;
#48908=CARTESIAN_POINT ( 'NONE',  ( 9.910131830190000102, 1406.621495965729991, 267.1956846989980363 ) ) ;
#48909=CARTESIAN_POINT ( 'NONE',  ( 0.3331931608689999713, 1408.924695757129939, 186.0526652876979767 ) ) ;
#48910=CARTESIAN_POINT ( 'NONE',  ( -7.105427357599999217E-15, 1410.913060387329779, 137.0999999980979851 ) ) ;
#48912=CARTESIAN_POINT ( 'NONE',  ( 23.63185289614832385, 1434.172427200277298, 214.7039615058700690 ) ) ;
#48914=CARTESIAN_POINT ( 'NONE',  ( 28.13477516149999857, 1508.112005763430034, 210.1092937961579992 ) ) ;
#48916=CARTESIAN_POINT ( 'NONE',  ( -2.434526125190220380, 1449.527760103650053, 155.0642341674960107 ) ) ;
#48918=CARTESIAN_POINT ( 'NONE',  ( -19.88572122277579979, 1484.728771715989751, 191.0592865161910083 ) ) ;
#48919=CARTESIAN_POINT ( 'NONE',  ( -14.09832007171429957, 1415.595619977640126, 221.0238313356500157 ) ) ;
#48920=DIRECTION ( 'NONE',  ( 1.962482049179999770E-13, -8.350987443300000121E-15, -1.000000000000000000 ) ) ;
#48921=CARTESIAN_POINT ( 'NONE',  ( -8.555769954617961304, 1409.211834457770010, 196.8452873928659983 ) ) ;
#48923=CARTESIAN_POINT ( 'NONE',  ( -26.91728171915830004, 1508.004642862799983, 211.7160872265129967 ) ) ;
#48924=CARTESIAN_POINT ( 'NONE',  ( 3.118963903650000091, 1441.197690497029953, 165.1033354352979927 ) ) ;
#48925=CARTESIAN_POINT ( 'NONE',  ( -3.441725452600000068, 1475.954703585829975, 268.4787010635980096 ) ) ;
#48926=CARTESIAN_POINT ( 'NONE',  ( -4.242885033098620085, 1446.408270998030048, 162.3196225285890080 ) ) ;
#48928=EDGE_CURVE ( 'NONE', #94174, #22669, #65973, .T. ) ;
#48929=CARTESIAN_POINT ( 'NONE',  ( -18.43055515643429842, 1486.478983240757998, 188.6801967137396616 ) ) ;
#48936=CARTESIAN_POINT ( 'NONE',  ( -18.88112913370000001, 1409.572403950229955, 198.2284472637979889 ) ) ;
#48937=CARTESIAN_POINT ( 'NONE',  ( -15.23233646464800195, 1422.123670831245818, 227.7537345013419952 ) ) ;
#48938=CARTESIAN_POINT ( 'NONE',  ( -9.999959670399999112, 1407.452792677830075, 269.6172309327980088 ) ) ;
#48939=ORIENTED_EDGE ( 'NONE', *, *, #22039, .F. ) ;
#48941=CARTESIAN_POINT ( 'NONE',  ( 28.25086641300000068, 1508.135711190629991, 209.3856964555159834 ) ) ;
#48943=CARTESIAN_POINT ( 'NONE',  ( 10.70806905399999920, 1424.991205926329940, 137.4294028545979813 ) ) ;
#48946=LINE ( 'NONE', #66307, #29415 ) ;
#48947=CARTESIAN_POINT ( 'NONE',  ( 39.20827873999350288, 1450.609082524699943, 136.0286972522910105 ) ) ;
#48951=CARTESIAN_POINT ( 'NONE',  ( -7.255983564230000127, 1427.866122641229822, 147.4806042202980052 ) ) ;
#48953=CARTESIAN_POINT ( 'NONE',  ( -20.61542114843588536, 1508.364347659817440, 190.3921826368226675 ) ) ;
#48955=CARTESIAN_POINT ( 'NONE',  ( 21.32616491865039876, 1509.431678241010104, 227.8426383757489759 ) ) ;
#48958=ORIENTED_EDGE ( 'NONE', *, *, #47350, .T. ) ;
#48959=CARTESIAN_POINT ( 'NONE',  ( 11.92728121149999865, 1433.973591798999905, 150.6941211948980026 ) ) ;
#48960=CARTESIAN_POINT ( 'NONE',  ( -10.69384198020000021, 1396.286497578129911, 212.3513119892680265 ) ) ;
#48961=CARTESIAN_POINT ( 'NONE',  ( -18.45264828540000224, 1409.557441064630211, 220.8691094444980081 ) ) ;
#48963=CARTESIAN_POINT ( 'NONE',  ( -12.85133220204726001, 1444.958534272496763, 169.4430044350944513 ) ) ;
#48964=CARTESIAN_POINT ( 'NONE',  ( 22.24050427028109311, 1509.699967146265180, 228.5561123524984168 ) ) ;
#48967=CARTESIAN_POINT ( 'NONE',  ( -13.70786035851040019, 1507.754328159320039, 184.2519299535370010 ) ) ;
#48968=CARTESIAN_POINT ( 'NONE',  ( 0.3355459311639999997, 1449.243710373649947, 183.3896813568979951 ) ) ;
#48969=CARTESIAN_POINT ( 'NONE',  ( -10.07457507059999813, 1416.825421875629900, 193.4554633978979723 ) ) ;
#48972=B_SPLINE_SURFACE_WITH_KNOTS ( 'NONE', 2, 5, ( 
 ( #22252, #90582, #73812, #4926, #39070, #73246 ),
 ( #13863, #107941, #106830, #99521, #71640, #22806 ),
 ( #64315, #46963, #106292, #55357, #89490, #12784 ) ),
 .UNSPECIFIED., .F., .F., .F.,
 ( 3, 3 ),
 ( 6, 6 ),
 ( 72.92379873290001058, 73.89199858150000466 ),
 ( 0.000000000000000000, 2.000000000000000000 ),
 .UNSPECIFIED. ) ;
#48973=CARTESIAN_POINT ( 'NONE',  ( 9.707456031250101702, 1396.252052236789723, 203.8125232392220028 ) ) ;
#48974=CARTESIAN_POINT ( 'NONE',  ( 1.159637561179999832, 1415.063410489729904, 191.5788536471979739 ) ) ;
#48975=CARTESIAN_POINT ( 'NONE',  ( 10.86749701439999960, 1425.819625802929977, 148.2249929719979775 ) ) ;
#48977=EDGE_LOOP ( 'NONE', ( #35164, #12442, #81181, #50526, #13264, #41821 ) ) ;
#48978=CARTESIAN_POINT ( 'NONE',  ( 13.08958089826340121, 1434.843138717199963, 149.4032511664449885 ) ) ;
#48979=ORIENTED_EDGE ( 'NONE', *, *, #108387, .F. ) ;
#48980=ORIENTED_EDGE ( 'NONE', *, *, #104250, .F. ) ;
#48981=CARTESIAN_POINT ( 'NONE',  ( -17.84980107695580287, 1458.247813499710219, 228.0953541232100008 ) ) ;
#48982=CARTESIAN_POINT ( 'NONE',  ( -8.298541131280000371, 1464.648652832329844, 233.2149708747980128 ) ) ;
#48986=ORIENTED_EDGE ( 'NONE', *, *, #65112, .F. ) ;
#48988=CARTESIAN_POINT ( 'NONE',  ( 2.500000000000000000, 1448.200164369519825, 169.1292575994999936 ) ) ;
#48994=CARTESIAN_POINT ( 'NONE',  ( -20.67559711379999854, 1509.531575931029920, 229.8721981546979976 ) ) ;
#48995=CARTESIAN_POINT ( 'NONE',  ( -18.44378729667023009, 1413.503667190741908, 269.3810517491084511 ) ) ;
#48998=CARTESIAN_POINT ( 'NONE',  ( 0.08022770239931510672, 1416.524489948229984, 227.2134237566240245 ) ) ;
#48999=VERTEX_POINT ( 'NONE', #107386 ) ;
#49001=CARTESIAN_POINT ( 'NONE',  ( -30.26655853036449884, 1440.913060387089899, 239.1917914571189954 ) ) ;
#49003=CARTESIAN_POINT ( 'NONE',  ( -0.06241017250561379376, 1466.769691485820204, 235.6256240966490054 ) ) ;
#49004=CARTESIAN_POINT ( 'NONE',  ( 7.240562320799770468, 1410.843301754160166, 269.3412962850030112 ) ) ;
#49006=CARTESIAN_POINT ( 'NONE',  ( 22.91622274789999736, 1409.721715511730054, 209.0611398913850110 ) ) ;
#49011=CARTESIAN_POINT ( 'NONE',  ( -2.506258803592136264, 1448.698841201256073, 154.6270693172046151 ) ) ;
#49012=CARTESIAN_POINT ( 'NONE',  ( 0.4863422716760000264, 1418.702333073229966, 184.7128037028979861 ) ) ;
#49013=CARTESIAN_POINT ( 'NONE',  ( 1.160687054150907116, 1409.478223960041987, 232.4137843514840824 ) ) ;
#49018=CARTESIAN_POINT ( 'NONE',  ( 37.00351967400000319, 1461.786612606330209, 266.5576464536979984 ) ) ;
#49021=CARTESIAN_POINT ( 'NONE',  ( -17.28556289930000034, 1479.740378035829963, 228.8535607617980361 ) ) ;
#49022=CARTESIAN_POINT ( 'NONE',  ( -5.423605666139999393, 1436.253592627979742, 154.6924226254979828 ) ) ;
#49025=AXIS2_PLACEMENT_3D ( 'NONE', #16595, #95549, #85470 ) ;
#49029=CARTESIAN_POINT ( 'NONE',  ( 10.56467116463950084, 1423.845360445598999, 137.4573436676088818 ) ) ;
#49035=EDGE_CURVE ( 'NONE', #98070, #92390, #58793, .T. ) ;
#49036=CARTESIAN_POINT ( 'NONE',  ( 23.35526608410000193, 1448.827836771670036, 218.6598503475479731 ) ) ;
#49040=CARTESIAN_POINT ( 'NONE',  ( 11.66756983127008063, 1418.593453235695961, 229.5266030089004516 ) ) ;
#49041=CARTESIAN_POINT ( 'NONE',  ( 38.47356468767819848, 1448.369015667859912, 136.4419166358019879 ) ) ;
#49042=CARTESIAN_POINT ( 'NONE',  ( -18.65431773610000121, 1425.340119975330026, 225.0950243718980062 ) ) ;
#49043=CARTESIAN_POINT ( 'NONE',  ( -30.50754839409947650, 1466.330398693723737, 269.3461395109432033 ) ) ;
#49045=CARTESIAN_POINT ( 'NONE',  ( -17.23770320690000091, 1413.292237373229909, 226.2052584196979979 ) ) ;
#49046=CARTESIAN_POINT ( 'NONE',  ( 0.0001165990426140000018, 1408.913064459030011, 231.7797585373979814 ) ) ;
#49047=CARTESIAN_POINT ( 'NONE',  ( -28.45928379452146473, 1463.335201769019932, 269.4551648148650429 ) ) ;
#49049=CARTESIAN_POINT ( 'NONE',  ( -4.304798037349998904E-15, 1432.353341358199941, 150.3995506339979897 ) ) ;
#49051=CARTESIAN_POINT ( 'NONE',  ( 8.861632801989001607, 1506.578946199044594, 188.8712608442579608 ) ) ;
#49054=CARTESIAN_POINT ( 'NONE',  ( -1.804213505890000180, 1410.351307731129964, 186.0507930254979954 ) ) ;
#49055=CARTESIAN_POINT ( 'NONE',  ( -13.51254418754115427, 1443.799311687372438, 187.1419075245657666 ) ) ;
#49061=CARTESIAN_POINT ( 'NONE',  ( 17.60594182058157386, 1424.146952378337346, 228.5308900134957071 ) ) ;
#49062=CARTESIAN_POINT ( 'NONE',  ( -12.61661106525792952, 1442.788675913401448, 169.4674439222872024 ) ) ;
#49063=EDGE_CURVE ( 'NONE', #105370, #32165, #17636, .T. ) ;
#49064=CARTESIAN_POINT ( 'NONE',  ( 18.28672154731980015, 1425.324301384940100, 225.4653420784370326 ) ) ;
#49065=ORIENTED_EDGE ( 'NONE', *, *, #72591, .T. ) ;
#49066=CARTESIAN_POINT ( 'NONE',  ( 0.4156091144216609856, 1414.971513442450032, 192.3333892557660079 ) ) ;
#49067=CARTESIAN_POINT ( 'NONE',  ( -0.9647690717699999308, 1408.946750865729882, 231.5874088180979982 ) ) ;
#49068=ORIENTED_EDGE ( 'NONE', *, *, #82333, .F. ) ;
#49069=ORIENTED_EDGE ( 'NONE', *, *, #30443, .T. ) ;
#49070=CARTESIAN_POINT ( 'NONE',  ( 17.65703761238349756, 1415.429375168339902, 209.4485410505009781 ) ) ;
#49071=CARTESIAN_POINT ( 'NONE',  ( 13.43167055049999981, 1509.382104692529992, 235.1752292677980165 ) ) ;
#49073=CARTESIAN_POINT ( 'NONE',  ( -25.74056229059999978, 1440.913060583030074, 220.8687942643980193 ) ) ;
#49074=CARTESIAN_POINT ( 'NONE',  ( -20.55886062980000162, 1506.532306263230112, 190.1125840497979880 ) ) ;
#49075=CARTESIAN_POINT ( 'NONE',  ( -11.82447129959999899, 1433.241336066939994, 150.5548711859979676 ) ) ;
#49076=CARTESIAN_POINT ( 'NONE',  ( -9.867588125367669605, 1445.429986924526702, 184.5009753814391615 ) ) ;
#49077=CARTESIAN_POINT ( 'NONE',  ( 27.88515232864000026, 1499.645912665409924, 209.4023683382970091 ) ) ;
#49078=CARTESIAN_POINT ( 'NONE',  ( -26.46046315050000075, 1441.626270684899964, 137.7338459625980249 ) ) ;
#49079=CARTESIAN_POINT ( 'NONE',  ( -24.24596083330000340, 1438.629152405760124, 212.1147215154179833 ) ) ;
#49081=CARTESIAN_POINT ( 'NONE',  ( 1.546925190270000083, 1450.646712626299859, 182.0032008381979836 ) ) ;
#49083=CARTESIAN_POINT ( 'NONE',  ( -28.15666966853906672, 1510.007892114357674, 198.7595920586345244 ) ) ;
#49085=EDGE_LOOP ( 'NONE', ( #94374, #91601, #61263, #19981, #52713 ) ) ;
#49089=CARTESIAN_POINT ( 'NONE',  ( -3.196891731540000059, 1474.092834640029878, 270.1354749226979379 ) ) ;
#49093=CARTESIAN_POINT ( 'NONE',  ( 37.13154625033060086, 1450.996886497350033, 135.1616079744260048 ) ) ;
#49094=DIRECTION ( 'NONE',  ( 0.000000000000000000, 1.000000000000000000, 0.000000000000000000 ) ) ;
#49099=CARTESIAN_POINT ( 'NONE',  ( -43.70846434600260011, 1429.985737363310136, 268.5715736658989954 ) ) ;
#49102=CIRCLE ( 'NONE', #61656, 2.000175714736120991 ) ;
#49103=ORIENTED_EDGE ( 'NONE', *, *, #52259, .T. ) ;
#49104=ORIENTED_EDGE ( 'NONE', *, *, #101584, .T. ) ;
#49106=CARTESIAN_POINT ( 'NONE',  ( 4.639095080327251708, 1423.703679602264856, 183.8752827255912052 ) ) ;
#49110=CARTESIAN_POINT ( 'NONE',  ( -13.58956681059999916, 1455.448334937230129, 187.8199450490979814 ) ) ;
#49112=CARTESIAN_POINT ( 'NONE',  ( -11.60004869885203682, 1428.983126981193436, 135.0999999980979851 ) ) ;
#49115=CARTESIAN_POINT ( 'NONE',  ( -26.79697582150000201, 1435.433282762789986, 135.3785755500979917 ) ) ;
#49117=B_SPLINE_SURFACE_WITH_KNOTS ( 'NONE', 5, 5, ( 
 ( #104832, #53916, #2954, #105389, #62884, #9650 ),
 ( #96996, #95329, #20259, #77971, #54459, #88596 ),
 ( #1278, #35418, #18590, #52785, #86922, #10213 ),
 ( #44390, #78533, #1844, #35979, #70170, #5116 ),
 ( #38171, #14616, #39272, #72889, #47686, #91331 ),
 ( #5685, #23003, #55548, #106481, #20806, #81814 ) ),
 .UNSPECIFIED., .F., .F., .F.,
 ( 6, 6 ),
 ( 6, 6 ),
 ( 11.44766861079999920, 30.74049611620000277 ),
 ( 0.000000000000000000, 2.000000000000000000 ),
 .UNSPECIFIED. ) ;
#49120=CARTESIAN_POINT ( 'NONE',  ( -34.80158685906719995, 1420.241074056469870, 270.2980797153470007 ) ) ;
#49122=CARTESIAN_POINT ( 'NONE',  ( -5.072028222450000179, 1397.441753602630115, 197.1461490164979864 ) ) ;
#49123=DIRECTION ( 'NONE',  ( 0.4794255386042028388, 0.000000000000000000, 0.8775825618903727587 ) ) ;
#49124=ORIENTED_EDGE ( 'NONE', *, *, #104866, .F. ) ;
#49126=CARTESIAN_POINT ( 'NONE',  ( -8.881784196999999612E-15, 1446.564900598709983, 126.8032249175980155 ) ) ;
#49130=CARTESIAN_POINT ( 'NONE',  ( -24.48327685399999609, 1441.929089702420015, 211.0380465236279690 ) ) ;
#49134=CARTESIAN_POINT ( 'NONE',  ( -2.616546427032389932, 1484.260686020460071, 183.2626519981290016 ) ) ;
#49136=FACE_OUTER_BOUND ( 'NONE', #92067, .T. ) ;
#49138=EDGE_LOOP ( 'NONE', ( #58012, #108607, #108170, #11109 ) ) ;
#49139=CARTESIAN_POINT ( 'NONE',  ( -38.81202644809479807, 1436.797832379780175, 134.4203394024459897 ) ) ;
#49140=CARTESIAN_POINT ( 'NONE',  ( -11.00427874533239958, 1425.778358600110096, 91.15460183957679874 ) ) ;
#49142=CARTESIAN_POINT ( 'NONE',  ( -20.86737114567692331, 1455.046213227785756, 223.5104812541308092 ) ) ;
#49145=CARTESIAN_POINT ( 'NONE',  ( -25.48530486458319899, 1509.803026911279630, 223.7268176318329722 ) ) ;
#49146=CARTESIAN_POINT ( 'NONE',  ( 14.15450645269999974, 1415.628674276829770, 197.1631309957980136 ) ) ;
#49147=CARTESIAN_POINT ( 'NONE',  ( -41.66135440509999910, 1443.796918820770088, 135.6885369501979994 ) ) ;
#49148=CARTESIAN_POINT ( 'NONE',  ( 26.54193529589999656, 1451.986209443830148, 134.9390663417979965 ) ) ;
#49151=CARTESIAN_POINT ( 'NONE',  ( 0.09512346046118322351, 1506.606278688875818, 186.9942562802339125 ) ) ;
#49152=CARTESIAN_POINT ( 'NONE',  ( 23.59327449265760990, 1448.793542086508069, 216.5857998349242450 ) ) ;
#49153=CARTESIAN_POINT ( 'NONE',  ( -11.91388749740000108, 1435.945967586000052, 151.0354243678980026 ) ) ;
#49154=CARTESIAN_POINT ( 'NONE',  ( 34.59585293901231751, 1451.704947487630079, 134.6974134653648605 ) ) ;
#49156=VERTEX_POINT ( 'NONE', #14965 ) ;
#49159=CARTESIAN_POINT ( 'NONE',  ( 0.4863418399100000178, 1418.702334915129995, 184.7127967600980014 ) ) ;
#49164=CARTESIAN_POINT ( 'NONE',  ( 11.60004869885203682, 1426.458005118043047, 139.1709647423215301 ) ) ;
#49169=CARTESIAN_POINT ( 'NONE',  ( -4.946301771011410109E-07, 1406.984793698239855, 222.1228995466940148 ) ) ;
#49170=CARTESIAN_POINT ( 'NONE',  ( 29.22677911810859896, 1440.913060387069891, 235.7684569196479742 ) ) ;
#49179=CARTESIAN_POINT ( 'NONE',  ( -13.27700466185214090, 1506.366982258753751, 226.6204409654947085 ) ) ;
#49184=CARTESIAN_POINT ( 'NONE',  ( 27.54247199862367523, 1509.986917861693200, 221.0135325175801029 ) ) ;
#49188=B_SPLINE_CURVE_WITH_KNOTS ( 'NONE', 5,
 ( #14338, #7057, #83214, #102208, #101093, #31698, #32260, #48527, #82667 ),
 .UNSPECIFIED., .F., .F.,
 ( 6, 3, 6 ),
 ( 0.000000000000000000, 0.5050532947641763748, 1.000000000000000000 ),
 .UNSPECIFIED. ) ;
#49189=FACE_OUTER_BOUND ( 'NONE', #14586, .T. ) ;
#49190=CARTESIAN_POINT ( 'NONE',  ( -11.89599453256210104, 1434.596263801839996, 147.6475367371979814 ) ) ;
#49197=CARTESIAN_POINT ( 'NONE',  ( -20.92480426329999688, 1409.643770653630099, 213.2359878676279834 ) ) ;
#49202=CARTESIAN_POINT ( 'NONE',  ( -11.57168670579999947, 1440.669964955550086, 147.8294280051980252 ) ) ;
#49208=CARTESIAN_POINT ( 'NONE',  ( 11.70547067012559950, 1409.321824430400056, 199.8234607599930257 ) ) ;
#49209=CARTESIAN_POINT ( 'NONE',  ( 0.3331978421699999804, 1408.924695912329980, 186.0526675979979814 ) ) ;
#49212=CARTESIAN_POINT ( 'NONE',  ( -3.126071747161609515, 1441.074179428409934, 162.1943810228259792 ) ) ;
#49213=B_SPLINE_CURVE_WITH_KNOTS ( 'NONE', 5,
 ( #91304, #55519, #89647, #71804, #90186, #12933, #81240, #22411, #14587 ),
 .UNSPECIFIED., .F., .F.,
 ( 6, 3, 6 ),
 ( 0.000000000000000000, 0.4424181324985710373, 1.000000000000000000 ),
 .UNSPECIFIED. ) ;
#49214=CARTESIAN_POINT ( 'NONE',  ( -2.499996273572980154, 1448.894362898710142, 183.1109776662320030 ) ) ;
#49215=ORIENTED_EDGE ( 'NONE', *, *, #85776, .T. ) ;
#49217=CARTESIAN_POINT ( 'NONE',  ( -2.439001525050000119, 1430.488531030629929, 150.2249694046979869 ) ) ;
#49218=CARTESIAN_POINT ( 'NONE',  ( 18.39664307513569952, 1458.152682626249771, 227.7204897826050001 ) ) ;
#49219=CARTESIAN_POINT ( 'NONE',  ( -13.01562633140000003, 1434.791942642399817, 149.6201245377980058 ) ) ;
#49224=AXIS2_PLACEMENT_3D ( 'NONE', #55031, #1877, #18620 ) ;
#49225=CARTESIAN_POINT ( 'NONE',  ( 0.1762042766570000030, 1476.674948662830047, 182.2372324101980041 ) ) ;
#49228=CARTESIAN_POINT ( 'NONE',  ( 13.80301174034419986, 1509.225260488219874, 234.1284213510270149 ) ) ;
#49231=B_SPLINE_CURVE_WITH_KNOTS ( 'NONE', 3,
 ( #108843, #14778, #83095, #56244, #31027, #83635, #5846, #65756, #75265, #48408, #99873, #100443, #23726, #15317, #41088, #109955, #48964, #6931, #40536, #74712, #39986, #66325 ),
 .UNSPECIFIED., .F., .F.,
 ( 4, 2, 2, 2, 2, 2, 2, 2, 2, 2, 4 ),
 ( 0.000000000000000000, 0.2500000000000318634, 0.3750000000000477951, 0.4375000000000460187, 0.5000000000000442979, 0.6250000000000214273, 0.6875000000000214273, 0.7500000000000214273, 0.8125000000000214273, 0.8750000000000213163, 1.000000000000000000 ),
 .UNSPECIFIED. ) ;
#49232=CARTESIAN_POINT ( 'NONE',  ( -3.827327205999999649, 1432.413060387330006, 146.1721969590979882 ) ) ;
#49233=CARTESIAN_POINT ( 'NONE',  ( -4.026786250540000722, 1421.741487512030062, 169.4417495807979890 ) ) ;
#49234=B_SPLINE_SURFACE_WITH_KNOTS ( 'NONE', 5, 5, ( 
 ( #28016, #62771, #96886, #104727, #62204, #63850 ),
 ( #44849, #72250, #29122, #106378, #29665, #3394 ),
 ( #10115, #53245, #105843, #86824, #19609, #52688 ),
 ( #37524, #97427, #53811, #87386, #70065, #11238 ),
 ( #28573, #105280, #20696, #45400, #79539, #54892 ),
 ( #44287, #104177, #27461, #61649, #95776, #19043 ),
 ( #10681, #38613, #82821, #73335, #64398, #55444 ),
 ( #40822, #21232, #100181, #91770, #14507, #89571 ),
 ( #90112, #22892, #22339, #5577, #39160, #4482 ),
 ( #72791, #47582, #57658, #30767, #99608, #82279 ),
 ( #81707, #57102, #39727, #73893, #97962, #21787 ),
 ( #12862, #108019, #30207, #47043, #31868, #81167 ) ),
 .UNSPECIFIED., .F., .F., .F.,
 ( 6, 3, 3, 6 ),
 ( 6, 6 ),
 ( 13.40444266900000159, 16.17473073229999869, 20.23252678009999883, 23.15004421629999953 ),
 ( 0.000000000000000000, 1.553560449149999911 ),
 .UNSPECIFIED. ) ;
#49238=CARTESIAN_POINT ( 'NONE',  ( 30.28727320009999957, 1436.978278694869914, 240.1330978273979895 ) ) ;
#49239=CARTESIAN_POINT ( 'NONE',  ( -0.4818462150879999628, 1464.109908317130021, 182.6611701878979943 ) ) ;
#49240=CARTESIAN_POINT ( 'NONE',  ( -16.69108649869999894, 1409.495925968330084, 194.8380977668979881 ) ) ;
#49242=B_SPLINE_CURVE_WITH_KNOTS ( 'NONE', 3,
 ( #40052, #65826, #108915, #30548 ),
 .UNSPECIFIED., .F., .F.,
 ( 4, 4 ),
 ( 0.000000000000000000, 1.000000000000000000 ),
 .UNSPECIFIED. ) ;
#49243=CARTESIAN_POINT ( 'NONE',  ( -25.50660914920000266, 1437.541738164299886, 220.8252629115979744 ) ) ;
#49245=CARTESIAN_POINT ( 'NONE',  ( -1.965429846505029943, 1452.844426064699974, 152.4682849505009870 ) ) ;
#49248=CARTESIAN_POINT ( 'NONE',  ( -2.500000000000000000, 1419.454841297830171, 146.2312480424980095 ) ) ;
#49249=CARTESIAN_POINT ( 'NONE',  ( 16.79131591733570161, 1422.584993768290133, 227.0552595885409914 ) ) ;
#49252=ORIENTED_EDGE ( 'NONE', *, *, #61018, .T. ) ;
#49254=B_SPLINE_CURVE_WITH_KNOTS ( 'NONE', 3,
 ( #64087, #81390, #5257, #97120, #13082, #39411, #97664, #56218, #12559, #56773, #89263, #46189, #90348, #4703, #22568, #65182, #105527, #45643, #80322, #38846, #106069, #38299, #90911, #47267, #37216, #31003, #98760, #46739, #29349 ),
 .UNSPECIFIED., .F., .F.,
 ( 4, 2, 2, 2, 2, 2, 2, 2, 2, 2, 2, 2, 2, 1, 4 ),
 ( 0.000000000000000000, 0.06995772642207957748, 0.1049365896331837661, 0.1224260212388009333, 0.1311707370415980956, 0.1399154528443952439, 0.2098731792674686514, 0.2448520424790045502, 0.2798309056905404768, 0.4197463585366428829, 0.4897040849595805656, 0.4984488007624685579, 0.5071935165653566058, 0.5246829481713172205, 0.5596618113830474917 ),
 .UNSPECIFIED. ) ;
#49256=CARTESIAN_POINT ( 'NONE',  ( -22.91314480545359800, 1409.722892369710053, 209.2608525687020062 ) ) ;
#49259=CARTESIAN_POINT ( 'NONE',  ( 5.442563054701103908, 1446.864248024533254, 154.6441915987726645 ) ) ;
#49260=CARTESIAN_POINT ( 'NONE',  ( -1.947314920589999998, 1498.352006593830083, 236.6548988695980142 ) ) ;
#49261=CARTESIAN_POINT ( 'NONE',  ( -20.07053839829999831, 1410.870413675929967, 220.7218785659979972 ) ) ;
#49262=CARTESIAN_POINT ( 'NONE',  ( 41.12904693102370146, 1456.837557776329959, 266.8381811544340394 ) ) ;
#49264=CARTESIAN_POINT ( 'NONE',  ( 0.02416417718109999807, 1419.738504350029871, 184.3877211754980010 ) ) ;
#49266=ORIENTED_EDGE ( 'NONE', *, *, #80850, .F. ) ;
#49271=CARTESIAN_POINT ( 'NONE',  ( 2.500000005880000042, 1448.917482167679964, 182.8661755616980145 ) ) ;
#49272=CARTESIAN_POINT ( 'NONE',  ( 27.01376952885669880, 1451.969717919180084, 134.9180436286740132 ) ) ;
#49279=CARTESIAN_POINT ( 'NONE',  ( 7.487843116287019818, 1409.174541630780141, 188.9631191401809929 ) ) ;
#49281=CARTESIAN_POINT ( 'NONE',  ( -18.48751025675699111, 1424.257012546406941, 225.0485682924247328 ) ) ;
#49284=CARTESIAN_POINT ( 'NONE',  ( 11.74015320060000001, 1428.979986575930070, 144.1938086916980239 ) ) ;
#49285=VERTEX_POINT ( 'NONE', #83290 ) ;
#49286=CARTESIAN_POINT ( 'NONE',  ( 20.74408967690000338, 1436.077466332870017, 224.8635562027979802 ) ) ;
#49287=CARTESIAN_POINT ( 'NONE',  ( 3.118629927103340194, 1507.020745903789930, 237.9289446147130036 ) ) ;
#49289=AXIS2_PLACEMENT_3D ( 'NONE', #28044, #19638, #9040 ) ;
#49294=CARTESIAN_POINT ( 'NONE',  ( -12.85916294179999930, 1469.933320803330162, 268.3665355202980436 ) ) ;
#49296=CARTESIAN_POINT ( 'NONE',  ( 11.36329992970000013, 1433.927233001689956, 151.4629445730980137 ) ) ;
#49298=CARTESIAN_POINT ( 'NONE',  ( 5.052203704720000133, 1465.000168608229842, 255.3819207742980097 ) ) ;
#49303=CARTESIAN_POINT ( 'NONE',  ( -14.77963593050276181, 1422.241748325693834, 229.4612819255225986 ) ) ;
#49304=CARTESIAN_POINT ( 'NONE',  ( -17.74110947659999837, 1486.349883151629911, 188.0997659469979908 ) ) ;
#49305=CARTESIAN_POINT ( 'NONE',  ( 9.939393902556568960, 1441.236512650339819, 153.4167242010410064 ) ) ;
#49306=CARTESIAN_POINT ( 'NONE',  ( -16.66219966870000135, 1409.494917224029905, 225.0851005536980267 ) ) ;
#49307=CARTESIAN_POINT ( 'NONE',  ( -1.546867746839999835, 1416.839692138929877, 228.0214409766979884 ) ) ;
#49309=CARTESIAN_POINT ( 'NONE',  ( -12.26979726809049964, 1416.828039266780024, 194.6643405733680083 ) ) ;
#49310=CARTESIAN_POINT ( 'NONE',  ( 12.78723769039999958, 1416.835809830829930, 222.7043020969979921 ) ) ;
#49313=CARTESIAN_POINT ( 'NONE',  ( 0.7910245917146940808, 1426.918876941764893, 134.0999999980980135 ) ) ;
#49314=CARTESIAN_POINT ( 'NONE',  ( 0.2052161641460210073, 1460.044096025570070, 182.9511842453609916 ) ) ;
#49316=ORIENTED_EDGE ( 'NONE', *, *, #74348, .T. ) ;
#49317=CARTESIAN_POINT ( 'NONE',  ( -27.68130203340000151, 1444.740067931809790, 168.8183730152979933 ) ) ;
#49319=CARTESIAN_POINT ( 'NONE',  ( 11.87573510900000073, 1433.006578257460205, 147.2728728793979940 ) ) ;
#49320=CARTESIAN_POINT ( 'NONE',  ( -41.63894744326280062, 1444.312235790899877, 134.0999999983169744 ) ) ;
#49329=CARTESIAN_POINT ( 'NONE',  ( 22.39898792957995965, 1411.068911948053938, 269.4880229147564705 ) ) ;
#49332=CARTESIAN_POINT ( 'NONE',  ( 2.663080543119999977, 1439.661674899039781, 183.7921143496980108 ) ) ;
#49336=CARTESIAN_POINT ( 'NONE',  ( -30.95328531120000193, 1451.376546782129935, 136.0329327139980080 ) ) ;
#49337=CARTESIAN_POINT ( 'NONE',  ( -16.32630028360690133, 1410.439485329699892, 226.5641403730199954 ) ) ;
#49342=AXIS2_PLACEMENT_3D ( 'NONE', #95485, #18752, #52949 ) ;
#49344=CARTESIAN_POINT ( 'NONE',  ( -21.19290736559898747, 1411.012288320353946, 217.7512743417428283 ) ) ;
#49346=CARTESIAN_POINT ( 'NONE',  ( -0.3495969842318680243, 1418.819586111129865, 184.6927620590689969 ) ) ;
#49347=CARTESIAN_POINT ( 'NONE',  ( 17.57263694539999932, 1409.691668943730065, 222.6387570695980003 ) ) ;
#49349=CARTESIAN_POINT ( 'NONE',  ( -16.92248609410000171, 1422.998996083129896, 227.1571761638979865 ) ) ;
#49355=CARTESIAN_POINT ( 'NONE',  ( -8.345708061868009509, 1484.725363963600103, 184.3707301608639852 ) ) ;
#49358=CARTESIAN_POINT ( 'NONE',  ( -4.245709548939140099, 1441.390156672689955, 161.8216553765309982 ) ) ;
#49360=ORIENTED_EDGE ( 'NONE', *, *, #88472, .F. ) ;
#49364=EDGE_CURVE ( 'NONE', #32914, #108746, #9412, .T. ) ;
#49366=CARTESIAN_POINT ( 'NONE',  ( -11.15476667854829884, 1425.160639125820126, 144.1599692811499835 ) ) ;
#49367=CARTESIAN_POINT ( 'NONE',  ( 16.17926374062649941, 1410.436583420409988, 191.6392560135060137 ) ) ;
#49368=EDGE_CURVE ( 'NONE', #99066, #52145, #69578, .T. ) ;
#49370=CARTESIAN_POINT ( 'NONE',  ( 40.28310057935370025, 1441.046327069720064, 136.8133136135640200 ) ) ;
#49371=EDGE_CURVE ( 'NONE', #10428, #65683, #13346, .T. ) ;
#49376=PRODUCT_CONTEXT ( 'NONE', #43481, 'mechanical' ) ;
#49378=CARTESIAN_POINT ( 'NONE',  ( 39.03583412974440137, 1449.647124672710106, 134.0999999981079895 ) ) ;
#49379=CYLINDRICAL_SURFACE ( 'NONE', #68607, 1.999999999999912514 ) ;
#49381=DIRECTION ( 'NONE',  ( 0.000000000000000000, 1.000000000000000000, 0.000000000000000000 ) ) ;
#49383=VERTEX_POINT ( 'NONE', #10444 ) ;
#49385=CARTESIAN_POINT ( 'NONE',  ( 11.60004869885203682, 1425.894332500278097, 137.5113157688821275 ) ) ;
#49386=CARTESIAN_POINT ( 'NONE',  ( -17.60627563539920004, 1410.895669414250051, 194.0661810348550205 ) ) ;
#49389=CARTESIAN_POINT ( 'NONE',  ( -2.500000000000309974, 1439.152017482790143, 158.1892368472379928 ) ) ;
#49392=CARTESIAN_POINT ( 'NONE',  ( 38.81202640299100182, 1450.612734557460044, 135.6938359136109966 ) ) ;
#49393=CARTESIAN_POINT ( 'NONE',  ( 2.591728129302680372, 1421.338677576370173, 183.3108762431510002 ) ) ;
#49394=CARTESIAN_POINT ( 'NONE',  ( 25.38578281050000029, 1437.608079703630210, 137.6409390164979811 ) ) ;
#49395=SHAPE_REPRESENTATION ( 'Grinder Body', ( #21632 ), #91264 ) ;
#49405=CARTESIAN_POINT ( 'NONE',  ( -0.0008045307254439123222, 1451.918653371962137, 154.0008071823928333 ) ) ;
#49406=ORIENTED_EDGE ( 'NONE', *, *, #78222, .F. ) ;
#49407=CARTESIAN_POINT ( 'NONE',  ( -13.61423569610000150, 1415.579607672129896, 221.4543120760979775 ) ) ;
#49408=FACE_OUTER_BOUND ( 'NONE', #69375, .T. ) ;
#49410=ADVANCED_FACE ( 'NONE', ( #70388 ), #96379, .F. ) ;
#49412=CARTESIAN_POINT ( 'NONE',  ( 21.41707235578040169, 1409.688061885250136, 206.3726929586279653 ) ) ;
#49414=CARTESIAN_POINT ( 'NONE',  ( 0.01756135629899999856, 1508.846989029630095, 179.8793381870979999 ) ) ;
#49418=CARTESIAN_POINT ( 'NONE',  ( 15.74698736379999708, 1461.435657786630145, 229.5665177702979918 ) ) ;
#49419=CARTESIAN_POINT ( 'NONE',  ( 28.84709936330000346, 1507.919204206129962, 206.0039977793879871 ) ) ;
#49421=FACE_OUTER_BOUND ( 'NONE', #109698, .T. ) ;
#49424=DIRECTION ( 'NONE',  ( 0.000000000000000000, -1.000000000000000000, 0.000000000000000000 ) ) ;
#49425=CARTESIAN_POINT ( 'NONE',  ( -29.75208676459999779, 1462.665512622030064, 268.3665355202980436 ) ) ;
#49430=CARTESIAN_POINT ( 'NONE',  ( 18.46438756899999944, 1509.557851009430124, 186.5303332271980139 ) ) ;
#49431=CARTESIAN_POINT ( 'NONE',  ( -11.60004869885203682, 1426.340588536289033, 138.4439388390336205 ) ) ;
#49436=CARTESIAN_POINT ( 'NONE',  ( -11.85381821950000081, 1431.481266617950041, 149.9176055244979864 ) ) ;
#49437=CARTESIAN_POINT ( 'NONE',  ( 19.03103510197079729, 1456.919749049050097, 225.5349545045000070 ) ) ;
#49439=CARTESIAN_POINT ( 'NONE',  ( 11.73563908010000034, 1425.610159190430068, 144.1657657165980027 ) ) ;
#49441=CARTESIAN_POINT ( 'NONE',  ( 12.70812379699999894, 1446.012777043369852, 188.2701611988979948 ) ) ;
#49442=CARTESIAN_POINT ( 'NONE',  ( -19.87113920289999669, 1482.731852092930012, 227.4655975904979925 ) ) ;
#49443=CARTESIAN_POINT ( 'NONE',  ( -5.360233013665446578, 1422.336972233150618, 139.1415641799490004 ) ) ;
#49447=CARTESIAN_POINT ( 'NONE',  ( 3.729773516839999914, 1406.618697554530172, 269.4937607996980091 ) ) ;
#49448=CARTESIAN_POINT ( 'NONE',  ( 0.1940371082550000070, 1409.861619517429972, 185.0322270696979956 ) ) ;
#49449=DIRECTION ( 'NONE',  ( -0.06949073829049068340, 0.8615482456355327834, -0.5028972635978229411 ) ) ;
#49450=ADVANCED_FACE ( 'NONE', ( #62547 ), #92792, .F. ) ;
#49452=CARTESIAN_POINT ( 'NONE',  ( 24.51739935401977633, 1438.724131266478480, 212.6264403365555893 ) ) ;
#49453=EDGE_CURVE ( 'NONE', #1304, #45857, #19939, .T. ) ;
#49458=CARTESIAN_POINT ( 'NONE',  ( -12.61676759610000076, 1445.618655625439942, 187.3523340095979961 ) ) ;
#49459=CARTESIAN_POINT ( 'NONE',  ( 0.8767898189759999461, 1450.882442212169963, 155.6080914335980196 ) ) ;
#49463=B_SPLINE_CURVE_WITH_KNOTS ( 'NONE', 3,
 ( #3406, #18503, #12321, #2315, #52699, #10128, #1756, #19054, #87398, #10692, #79014, #62216, #96343, #72804, #55456, #74466, #49259, #12875 ),
 .UNSPECIFIED., .F., .F.,
 ( 4, 2, 2, 2, 2, 1, 1, 2, 2, 4 ),
 ( 0.000000000000000000, 0.1250000000000460743, 0.1875000000000671407, 0.2500000000000882072, 0.3750000000001271760, 0.4375000000001487699, 0.4687500000001563749, 0.4843750000001555422, 0.5000000000001546541, 1.000000000000000000 ),
 .UNSPECIFIED. ) ;
#49467=CARTESIAN_POINT ( 'NONE',  ( -2.732294677939999694, 1474.989683629730052, 269.6477038462979863 ) ) ;
#49468=CARTESIAN_POINT ( 'NONE',  ( -4.222017444537139674, 1446.225621437700056, 168.0528712459710050 ) ) ;
#49470=CARTESIAN_POINT ( 'NONE',  ( -11.94336904982903746, 1486.509466811693073, 184.3567047474556944 ) ) ;
#49474=CARTESIAN_POINT ( 'NONE',  ( -24.72115217916500285, 1457.432886049350145, 211.5135014677179868 ) ) ;
#49476=CARTESIAN_POINT ( 'NONE',  ( -46.27885827404714547, 1440.913026088479455, 267.5894365880741361 ) ) ;
#49477=CARTESIAN_POINT ( 'NONE',  ( -0.2491233477655999673, 1395.921759966339778, 220.1232053259499821 ) ) ;
#49480=EDGE_CURVE ( 'NONE', #14771, #42031, #98303, .T. ) ;
#49482=ORIENTED_EDGE ( 'NONE', *, *, #109065, .F. ) ;
#49483=CARTESIAN_POINT ( 'NONE',  ( -7.608841146861992755, 1410.551743274452065, 230.8008565250618744 ) ) ;
#49484=B_SPLINE_CURVE_WITH_KNOTS ( 'NONE', 5,
 ( #31927, #65557, #24059, #100768, #72849, #40330 ),
 .UNSPECIFIED., .F., .F.,
 ( 6, 6 ),
 ( -2.000000000000000000, 0.000000000000000000 ),
 .UNSPECIFIED. ) ;
#49488=CARTESIAN_POINT ( 'NONE',  ( 11.43729884800000107, 1425.481263111430053, 144.1595926346979866 ) ) ;
#49495=SPHERICAL_SURFACE ( 'NONE', #89318, 2.000000000000000000 ) ;
#49496=CARTESIAN_POINT ( 'NONE',  ( -4.838067302830000749, 1426.802081400929865, 145.9750725641980011 ) ) ;
#49500=CARTESIAN_POINT ( 'NONE',  ( 20.12920962994530427, 1508.860404140810033, 229.2672809891759869 ) ) ;
#49501=VECTOR ( 'NONE', #18564, 1000.000000000000000 ) ;
#49503=ORIENTED_EDGE ( 'NONE', *, *, #48013, .T. ) ;
#49505=CARTESIAN_POINT ( 'NONE',  ( 11.45674231629960005, 1434.121012763210047, 151.3920262788900004 ) ) ;
#49506=CARTESIAN_POINT ( 'NONE',  ( -2.455548337050000196, 1396.059955855629823, 220.7626888616979954 ) ) ;
#49507=CARTESIAN_POINT ( 'NONE',  ( -19.20692459609999858, 1410.079524434029736, 222.1170233296979859 ) ) ;
#49509=CARTESIAN_POINT ( 'NONE',  ( -13.32429459549980066, 1444.551508282647774, 169.3762542488305201 ) ) ;
#49510=EDGE_CURVE ( 'NONE', #64407, #69273, #89619, .T. ) ;
#49511=CARTESIAN_POINT ( 'NONE',  ( -27.04494217939999956, 1509.634156510529920, 201.2636846103279709 ) ) ;
#49514=CARTESIAN_POINT ( 'NONE',  ( 17.91995256730000108, 1424.306612487629991, 226.0000067931979970 ) ) ;
#49515=CARTESIAN_POINT ( 'NONE',  ( 2.537021495169999863, 1468.705327849529795, 183.0181505298980085 ) ) ;
#49516=EDGE_CURVE ( 'NONE', #22747, #17568, #24525, .T. ) ;
#49518=FACE_OUTER_BOUND ( 'NONE', #75200, .T. ) ;
#49520=CARTESIAN_POINT ( 'NONE',  ( 10.27541959654410064, 1396.271885950119895, 205.0171044993250007 ) ) ;
#49521=CARTESIAN_POINT ( 'NONE',  ( 2.500000000000000000, 1419.524771318244348, 137.0999999980979851 ) ) ;
#49522=CARTESIAN_POINT ( 'NONE',  ( 11.76949914230000083, 1432.337435368489878, 150.8120642620980050 ) ) ;
#49524=VERTEX_POINT ( 'NONE', #73685 ) ;
#49525=CARTESIAN_POINT ( 'NONE',  ( 13.15339656435630111, 1434.869048593249772, 149.3633147529739915 ) ) ;
#49526=EDGE_LOOP ( 'NONE', ( #99757, #55049, #55450, #107755 ) ) ;
#49528=EDGE_CURVE ( 'NONE', #46291, #83462, #44132, .T. ) ;
#49529=CARTESIAN_POINT ( 'NONE',  ( -20.15504139832039954, 1507.862952778380077, 228.9029379167619993 ) ) ;
#49530=CARTESIAN_POINT ( 'NONE',  ( -4.974760226879999969, 1466.059548552929982, 234.4497863035979890 ) ) ;
#49537=CARTESIAN_POINT ( 'NONE',  ( 2.500000000000000000, 1448.224507101739846, 166.8031351735940007 ) ) ;
#49544=CARTESIAN_POINT ( 'NONE',  ( -35.43904686644575008, 1424.538195867626882, 269.5376332876632546 ) ) ;
#49545=CARTESIAN_POINT ( 'NONE',  ( -1.331498055899999811, 1408.959557324029902, 231.4960598541979948 ) ) ;
#49546=CARTESIAN_POINT ( 'NONE',  ( -0.08760820896872960339, 1414.971390223319986, 225.8230290847160120 ) ) ;
#49548=CARTESIAN_POINT ( 'NONE',  ( 22.94282329279999999, 1432.044723198870088, 216.2486866827079837 ) ) ;
#49551=CARTESIAN_POINT ( 'NONE',  ( -0.09294118512049590053, 1465.101552668469822, 237.0126441520749836 ) ) ;
#49552=CARTESIAN_POINT ( 'NONE',  ( 7.954910151169818811, 1410.785611874080132, 269.6217138226900261 ) ) ;
#49553=EDGE_CURVE ( 'NONE', #82793, #66538, #60197, .T. ) ;
#49555=CARTESIAN_POINT ( 'NONE',  ( 22.91422305780000102, 1409.721956062029903, 209.2901359145519962 ) ) ;
#49561=CARTESIAN_POINT ( 'NONE',  ( 0.1282414636960000076, 1420.458860909030136, 183.3323408609980163 ) ) ;
#49562=CARTESIAN_POINT ( 'NONE',  ( 4.331998614493840272, 1420.009893967346898, 137.0999999980978146 ) ) ;
#49571=CARTESIAN_POINT ( 'NONE',  ( -22.83376452409999757, 1450.736906982369874, 218.4795132163679909 ) ) ;
#49574=CYLINDRICAL_SURFACE ( 'NONE', #33618, 1.999999999999994449 ) ;
#49579=CARTESIAN_POINT ( 'NONE',  ( 11.94203325640082269, 1433.494999503054714, 149.8940326207935243 ) ) ;
#49580=CARTESIAN_POINT ( 'NONE',  ( -27.03405988100176671, 1451.512678451428883, 136.1495578053978477 ) ) ;
#49582=CARTESIAN_POINT ( 'NONE',  ( 20.99698467690000214, 1453.431242447430122, 222.6481362127979935 ) ) ;
#49586=CARTESIAN_POINT ( 'NONE',  ( 10.91475598504960409, 1418.233546538132714, 229.8208136691085031 ) ) ;
#49587=CARTESIAN_POINT ( 'NONE',  ( 28.37194653194559635, 1436.817231666380167, 136.7331909724399850 ) ) ;
#49588=CARTESIAN_POINT ( 'NONE',  ( -18.18137283760000145, 1507.546748828630143, 231.7129783355979669 ) ) ;
#49589=CARTESIAN_POINT ( 'NONE',  ( -20.85759521329999799, 1428.229804328530236, 220.8445560111979944 ) ) ;
#49590=CARTESIAN_POINT ( 'NONE',  ( -30.96124148313727886, 1466.023121715494426, 269.3370833597967362 ) ) ;
#49592=CARTESIAN_POINT ( 'NONE',  ( 15.36989447449999879, 1507.878420424329761, 186.8363077536980086 ) ) ;
#49594=CARTESIAN_POINT ( 'NONE',  ( -34.97375764654307062, 1457.803496076289548, 269.5311906646001034 ) ) ;
#49595=ORIENTED_EDGE ( 'NONE', *, *, #103402, .T. ) ;
#49597=CARTESIAN_POINT ( 'NONE',  ( 9.082050437914793051, 1506.560172253591418, 188.9861834009692529 ) ) ;
#49599=CARTESIAN_POINT ( 'NONE',  ( 22.86388141461030088, 1452.114636054890070, 134.1000000004160029 ) ) ;
#49600=CARTESIAN_POINT ( 'NONE',  ( -7.612906430609999830, 1431.113060387329824, 226.5499313142980213 ) ) ;
#49601=CARTESIAN_POINT ( 'NONE',  ( -15.50799805586373026, 1451.351354359962215, 222.5219775576906045 ) ) ;
#49603=CARTESIAN_POINT ( 'NONE',  ( -29.78122807940000172, 1510.000412734329757, 209.3782614727080045 ) ) ;
#49606=CARTESIAN_POINT ( 'NONE',  ( -2.133044466942135564, 1415.621662746755874, 232.9983725193774262 ) ) ;
#49607=CARTESIAN_POINT ( 'NONE',  ( -9.280787195236113618, 1451.345929965323649, 152.5707864879639715 ) ) ;
#49610=CARTESIAN_POINT ( 'NONE',  ( 18.52154166987810058, 1425.594020092049732, 225.5394061038540201 ) ) ;
#49612=EDGE_CURVE ( 'NONE', #104566, #99650, #100240, .T. ) ;
#49613=CARTESIAN_POINT ( 'NONE',  ( 1.027470347560650143, 1414.913060387399810, 192.7325489235379905 ) ) ;
#49614=CARTESIAN_POINT ( 'NONE',  ( 21.41430793513470121, 1509.039033305942212, 226.4051922569614419 ) ) ;
#49617=CARTESIAN_POINT ( 'NONE',  ( 17.84204394271100114, 1415.932840154009909, 208.7774965389979798 ) ) ;
#49622=CARTESIAN_POINT ( 'NONE',  ( -11.04995494539999967, 1433.656863779019886, 151.7239346888979981 ) ) ;
#49627=CARTESIAN_POINT ( 'NONE',  ( -24.36776551069999996, 1440.043862457850082, 211.3220141222980146 ) ) ;
#49631=CARTESIAN_POINT ( 'NONE',  ( -28.53389208509380026, 1510.020793257407377, 218.3937296574966638 ) ) ;
#49632=CARTESIAN_POINT ( 'NONE',  ( -2.164019640618629963E-09, 1415.934403820770058, 241.0787384265379956 ) ) ;
#49635=CARTESIAN_POINT ( 'NONE',  ( -11.83710954711010110, 1430.357175028169877, 149.6181111097540111 ) ) ;
#49637=CARTESIAN_POINT ( 'NONE',  ( -6.266569382469999283, 1471.715264099330170, 270.0731618598979935 ) ) ;
#49640=CARTESIAN_POINT ( 'NONE',  ( 38.48525439408140159, 1449.940833192290029, 135.6993408459150032 ) ) ;
#49641=CARTESIAN_POINT ( 'NONE',  ( 13.92102725570000032, 1408.913060387329779, 196.5791615931979948 ) ) ;
#49642=EDGE_CURVE ( 'NONE', #67100, #54363, #88159, .T. ) ;
#49645=CARTESIAN_POINT ( 'NONE',  ( -22.93995821741350127, 1507.616838180419791, 207.8436709359779968 ) ) ;
#49647=CARTESIAN_POINT ( 'NONE',  ( -33.55732945208360007, 1416.697737133469900, 266.7792439498080057 ) ) ;
#49650=CARTESIAN_POINT ( 'NONE',  ( -8.301987938657498844, 1512.913060387330006, 185.0111222839169898 ) ) ;
#49651=ORIENTED_EDGE ( 'NONE', *, *, #21399, .T. ) ;
#49660=CARTESIAN_POINT ( 'NONE',  ( -17.60065947509999873, 1485.486750496030027, 188.6130784315979838 ) ) ;
#49663=CARTESIAN_POINT ( 'NONE',  ( -17.05283090761910003, 1489.045462354059964, 229.1850863498580111 ) ) ;
#49665=CARTESIAN_POINT ( 'NONE',  ( -26.35085852639999970, 1436.712581025230065, 136.8307534946980013 ) ) ;
#49666=B_SPLINE_CURVE_WITH_KNOTS ( 'NONE', 3,
 ( #35394, #44364, #61729, #69025, #26428, #79624, #78510, #19118, #53321, #35956, #60623, #61189, #28094, #70142, #104256 ),
 .UNSPECIFIED., .F., .F.,
 ( 4, 2, 2, 1, 1, 1, 2, 2, 4 ),
 ( 0.000000000000000000, 0.2500000000001068035, 0.3750000000001622036, 0.4375000000001886824, 0.4687500000001994516, 0.4843750000002050582, 0.4921875000002064460, 0.5000000000002078338, 1.000000000000000000 ),
 .UNSPECIFIED. ) ;
#49670=CARTESIAN_POINT ( 'NONE',  ( -40.17393788466059590, 1425.544852429910179, 270.1489469183769643 ) ) ;
#49672=CARTESIAN_POINT ( 'NONE',  ( 15.49546526515152323, 1506.491018782020319, 193.4614169200511355 ) ) ;
#49676=CARTESIAN_POINT ( 'NONE',  ( 14.38344716668426138, 1473.391868309870915, 269.5847338116742549 ) ) ;
#49678=PLANE ( 'NONE',  #78913 ) ;
#49679=CARTESIAN_POINT ( 'NONE',  ( -24.45793889359999795, 1435.630516549809954, 137.6701772224979834 ) ) ;
#49680=CARTESIAN_POINT ( 'NONE',  ( -24.90839019419999900, 1441.482377299550080, 210.4444839806880054 ) ) ;
#49682=ADVANCED_FACE ( 'NONE', ( #47098 ), #53476, .T. ) ;
#49686=CARTESIAN_POINT ( 'NONE',  ( -13.31050689240000118, 1414.983771850430003, 220.3937082497979816 ) ) ;
#49688=EDGE_CURVE ( 'NONE', #29251, #56464, #49484, .T. ) ;
#49689=ORIENTED_EDGE ( 'NONE', *, *, #44527, .T. ) ;
#49690=CARTESIAN_POINT ( 'NONE',  ( -2.338016501012529780, 1451.953771032099894, 184.5921950015619757 ) ) ;
#49692=CARTESIAN_POINT ( 'NONE',  ( -19.87038186279464114, 1456.668401910016200, 225.4203470789150288 ) ) ;
#49693=EDGE_LOOP ( 'NONE', ( #48011, #52160, #62912, #17884, #53434, #94914, #42606, #30550, #100182, #109983 ) ) ;
#49695=CARTESIAN_POINT ( 'NONE',  ( -22.68369965143373435, 1509.726148796831694, 228.1704579189521098 ) ) ;
#49696=CARTESIAN_POINT ( 'NONE',  ( -4.079975117419219366, 1440.506274563688521, 185.2719822077098115 ) ) ;
#49701=CARTESIAN_POINT ( 'NONE',  ( 4.258542316545229411, 1441.260261168030183, 159.7577179058740171 ) ) ;
#49702=CIRCLE ( 'NONE', #97945, 3.058258088409981923 ) ;
#49704=CARTESIAN_POINT ( 'NONE',  ( -11.89522282729999958, 1434.541161981840105, 151.0452005854980086 ) ) ;
#49708=CARTESIAN_POINT ( 'NONE',  ( -17.42486771672220058, 1470.242291900930013, 228.5603268348579888 ) ) ;
#49709=CARTESIAN_POINT ( 'NONE',  ( 16.11683780530001897, 1409.475866348431737, 193.1327335431978725 ) ) ;
#49710=CARTESIAN_POINT ( 'NONE',  ( 2.261143588150000383, 1421.220611668830088, 183.2247237651980356 ) ) ;
#49712=CARTESIAN_POINT ( 'NONE',  ( -4.500000000000000000, 1432.413060387330006, 146.1721969590979882 ) ) ;
#49713=CARTESIAN_POINT ( 'NONE',  ( -1234.711986934499919, 50.13405481564039690, -9668.243368258868941 ) ) ;
#49715=CARTESIAN_POINT ( 'NONE',  ( 1.797565579689999860, 1415.903556134529936, 232.4419632246980143 ) ) ;
#49716=CARTESIAN_POINT ( 'NONE',  ( 18.73327636269999985, 1416.067629296030191, 210.6711993623479771 ) ) ;
#49719=CARTESIAN_POINT ( 'NONE',  ( 43.06295132563239747, 1440.913060355180050, 263.2597293094730162 ) ) ;
#49722=CARTESIAN_POINT ( 'NONE',  ( 13.21848706260000128, 1426.029874525029982, 222.0236330272979899 ) ) ;
#49723=ORIENTED_EDGE ( 'NONE', *, *, #104902, .F. ) ;
#49726=CARTESIAN_POINT ( 'NONE',  ( -19.87223104929999806, 1484.291808912129909, 191.2808552885979907 ) ) ;
#49727=CARTESIAN_POINT ( 'NONE',  ( -24.40934744099999776, 1441.356666734659939, 212.0571328766980059 ) ) ;
#49728=CARTESIAN_POINT ( 'NONE',  ( 12.89607781515299934, 1434.724834403989917, 149.2206011272099886 ) ) ;
#49731=CARTESIAN_POINT ( 'NONE',  ( -1.835536242490369840, 1450.383119622699951, 182.7750508701979868 ) ) ;
#49732=VECTOR ( 'NONE', #56753, 1000.000000000000000 ) ;
#49737=CARTESIAN_POINT ( 'NONE',  ( -13.34833196689999824, 1435.008643399920174, 194.9659071978979910 ) ) ;
#49739=( BOUNDED_CURVE ( )  B_SPLINE_CURVE ( 3, ( #104665, #62144, #96270, #19547 ),
 .UNSPECIFIED., .F., .T. ) 
 B_SPLINE_CURVE_WITH_KNOTS ( ( 4, 4 ),
 ( 2.061459541078140223, 2.471661985137465045 ),
 .UNSPECIFIED. ) 
 CURVE ( )  GEOMETRIC_REPRESENTATION_ITEM ( )  RATIONAL_B_SPLINE_CURVE ( ( 1.000000000000000000, 0.9860269160151746703, 0.9860269160151746703, 1.000000000000000000 ) ) 
 REPRESENTATION_ITEM ( '' )  );
#49746=ORIENTED_EDGE ( 'NONE', *, *, #64602, .F. ) ;
#49749=CARTESIAN_POINT ( 'NONE',  ( 35.84871811701600564, 1437.378613743899905, 136.5365654117910026 ) ) ;
#49757=AXIS2_PLACEMENT_3D ( 'NONE', #52761, #86897, #71240 ) ;
#49759=CARTESIAN_POINT ( 'NONE',  ( 18.28845126389499853, 1425.323877885890170, 225.4753632769809997 ) ) ;
#49760=DIRECTION ( 'NONE',  ( 0.6450708608689574852, -0.04363816677874634425, -0.7628756745748105361 ) ) ;
#49762=CARTESIAN_POINT ( 'NONE',  ( -2.500000000000000000, 1439.638128487539916, 168.7284197513979791 ) ) ;
#49765=CARTESIAN_POINT ( 'NONE',  ( -2.416798835000000256, 1426.601114010129777, 146.0361887655980127 ) ) ;
#49766=CARTESIAN_POINT ( 'NONE',  ( 19.14017132134949861, 1456.338359336380108, 227.2099314066680051 ) ) ;
#49767=CARTESIAN_POINT ( 'NONE',  ( 16.15368040339999922, 1468.829548787329941, 189.5967691369980059 ) ) ;
#49768=CARTESIAN_POINT ( 'NONE',  ( -9.751780903386149743E-09, 1474.814788804160116, 265.0004365400300230 ) ) ;
#49773=CARTESIAN_POINT ( 'NONE',  ( -0.5526888975579999919, 1482.197366675030025, 182.0017022400980125 ) ) ;
#49776=CARTESIAN_POINT ( 'NONE',  ( 13.74984697784300103, 1509.157712962339929, 234.0060514757300041 ) ) ;
#49783=CARTESIAN_POINT ( 'NONE',  ( -25.80443457887890091, 1452.006586394169972, 135.2613506968589832 ) ) ;
#49784=EDGE_LOOP ( 'NONE', ( #34453, #49316, #75559, #2705 ) ) ;
#49786=CARTESIAN_POINT ( 'NONE',  ( 19.57999166029999927, 1422.088355037530164, 238.2202656793979827 ) ) ;
#49788=CARTESIAN_POINT ( 'NONE',  ( -17.41346946009999996, 1410.020394389830017, 194.0661810129979870 ) ) ;
#49789=CARTESIAN_POINT ( 'NONE',  ( -1.880825668594659827, 1419.500193221429981, 185.7240730368970105 ) ) ;
#49790=FACE_OUTER_BOUND ( 'NONE', #87811, .T. ) ;
#49793=CARTESIAN_POINT ( 'NONE',  ( -3.970108626409070585, 1452.774421139130027, 152.2533984705749788 ) ) ;
#49794=CARTESIAN_POINT ( 'NONE',  ( -18.96271102769999928, 1416.819759739330038, 208.0003802813079972 ) ) ;
#49796=CARTESIAN_POINT ( 'NONE',  ( -2.500000000000000000, 1424.573971167730178, 154.8453096575980226 ) ) ;
#49799=CARTESIAN_POINT ( 'NONE',  ( -3.121529044914340467, 1448.960344233920068, 184.5768609971525791 ) ) ;
#49804=CARTESIAN_POINT ( 'NONE',  ( -23.63025210133929832, 1410.151946025710231, 209.7191186103189864 ) ) ;
#49805=FACE_OUTER_BOUND ( 'NONE', #23339, .T. ) ;
#49807=CARTESIAN_POINT ( 'NONE',  ( -45.54451795790711088, 1438.304327561658965, 266.1921463157105450 ) ) ;
#49810=CARTESIAN_POINT ( 'NONE',  ( -0.05455680805710000358, 1507.644790440630004, 237.3838523299980068 ) ) ;
#49812=ORIENTED_EDGE ( 'NONE', *, *, #22156, .T. ) ;
#49814=CARTESIAN_POINT ( 'NONE',  ( 45.70155086610489548, 1446.155617659590007, 268.2197227342359724 ) ) ;
#49820=CARTESIAN_POINT ( 'NONE',  ( -11.93818408299999945, 1433.480074519959999, 149.8972116839979947 ) ) ;
#49823=ORIENTED_EDGE ( 'NONE', *, *, #79881, .F. ) ;
#49825=CARTESIAN_POINT ( 'NONE',  ( 26.55535786486069938, 1451.985785255079918, 135.0211946108499887 ) ) ;
#49829=CARTESIAN_POINT ( 'NONE',  ( 21.97669732130000142, 1409.680503568630002, 212.0880462296879898 ) ) ;
#49831=CARTESIAN_POINT ( 'NONE',  ( 1.838013827845350168, 1408.977245244529968, 186.8835531457910122 ) ) ;
#49832=CARTESIAN_POINT ( 'NONE',  ( 2.163834958349999837, 1417.651400129230069, 234.2791204608979854 ) ) ;
#49837=CARTESIAN_POINT ( 'NONE',  ( 11.15268687969999917, 1425.700851675330114, 101.7515397216980091 ) ) ;
#49839=CARTESIAN_POINT ( 'NONE',  ( 12.84940689358530008, 1416.524489948229984, 221.8577937504570059 ) ) ;
#49846=CARTESIAN_POINT ( 'NONE',  ( -40.73184307449999864, 1445.563106277890029, 268.3665355202980436 ) ) ;
#49847=CARTESIAN_POINT ( 'NONE',  ( -21.93662986374314627, 1509.528752971103586, 191.4093251536967273 ) ) ;
#49848=CARTESIAN_POINT ( 'NONE',  ( 11.94328307949999868, 1433.499933921140155, 150.0080830760979893 ) ) ;
#49851=CARTESIAN_POINT ( 'NONE',  ( 0.7241444745577421127, 1467.041521348942524, 235.5044523316612697 ) ) ;
#49854=CARTESIAN_POINT ( 'NONE',  ( -15.71374344840000070, 1486.113479385830033, 186.6263592044980157 ) ) ;
#49856=CARTESIAN_POINT ( 'NONE',  ( -17.63293958180000232, 1409.693803940329872, 224.3174265464980124 ) ) ;
#49859=CARTESIAN_POINT ( 'NONE',  ( -16.19484051460299767, 1409.478596682770103, 193.4350318415109768 ) ) ;
#49863=CARTESIAN_POINT ( 'NONE',  ( 2.370970874524634286, 1427.002265528474027, 134.0999999980980135 ) ) ;
#49865=CARTESIAN_POINT ( 'NONE',  ( 0.1732173507811780033, 1478.442703680379964, 182.1612834630160194 ) ) ;
#49870=CARTESIAN_POINT ( 'NONE',  ( 12.06083241689999852, 1433.903765800100018, 149.9805303072979825 ) ) ;
#49871=CARTESIAN_POINT ( 'NONE',  ( -40.98974505614270214, 1446.927689381900109, 134.0999999985419890 ) ) ;
#49880=FACE_OUTER_BOUND ( 'NONE', #25258, .T. ) ;
#49884=B_SPLINE_SURFACE_WITH_KNOTS ( 'NONE', 5, 5, ( 
 ( #105284, #29126, #107473, #96335, #55448, #30771 ),
 ( #89575, #71730, #28576, #46503, #106383, #45941 ),
 ( #11243, #29669, #47047, #20161, #39164, #73339 ),
 ( #80079, #2846, #45404, #37528, #53815, #3398 ),
 ( #38618, #106922, #30211, #64402, #21791, #55993 ),
 ( #90116, #13399, #13955, #5581, #58195, #76095 ) ),
 .UNSPECIFIED., .F., .F., .F.,
 ( 6, 6 ),
 ( 6, 6 ),
 ( 0.000000000000000000, 21.60352440750000014 ),
 ( 0.000000000000000000, 0.4689189027120000408 ),
 .UNSPECIFIED. ) ;
#49889=CIRCLE ( 'NONE', #26683, 63.69383906210463664 ) ;
#49890=CARTESIAN_POINT ( 'NONE',  ( -29.82725556129999944, 1451.416006550429984, 136.0664794209980073 ) ) ;
#49891=CARTESIAN_POINT ( 'NONE',  ( 13.32090919908814719, 1443.086052842850677, 169.4274452085888072 ) ) ;
#49892=CARTESIAN_POINT ( 'NONE',  ( 5.508554876272072853, 1427.333971811663332, 134.0999999980980135 ) ) ;
#49898=CARTESIAN_POINT ( 'NONE',  ( -0.09506836101312440834, 1419.889005963919999, 184.0928500010010112 ) ) ;
#49900=CARTESIAN_POINT ( 'NONE',  ( -16.98323195629999915, 1422.783711030229824, 226.9778976059980096 ) ) ;
#49901=CARTESIAN_POINT ( 'NONE',  ( 33.91369114349999592, 1451.728768196330066, 134.7155302118979989 ) ) ;
#49904=CARTESIAN_POINT ( 'NONE',  ( 12.54268436849999979, 1408.913060387329779, 223.0428732173979824 ) ) ;
#49907=CIRCLE ( 'NONE', #14074, 1.999999999999911182 ) ;
#49908=CARTESIAN_POINT ( 'NONE',  ( 4.222550915190000254, 1446.229941110429991, 170.5491765577980061 ) ) ;
#49909=ORIENTED_EDGE ( 'NONE', *, *, #26542, .T. ) ;
#49910=CARTESIAN_POINT ( 'NONE',  ( 15.57748978360000081, 1507.212883781729943, 225.5460497861979832 ) ) ;
#49913=ORIENTED_EDGE ( 'NONE', *, *, #102212, .F. ) ;
#49915=VERTEX_POINT ( 'NONE', #41995 ) ;
#49918=CARTESIAN_POINT ( 'NONE',  ( -11.16129001045304037, 1425.156829533156497, 144.5843009260746044 ) ) ;
#49919=CARTESIAN_POINT ( 'NONE',  ( 16.42165607296470142, 1410.864361973030100, 191.6455063637129967 ) ) ;
#49921=CARTESIAN_POINT ( 'NONE',  ( 41.66477750127440061, 1443.168168707889890, 136.0651127029709926 ) ) ;
#49922=CARTESIAN_POINT ( 'NONE',  ( -45.67177476579999507, 1438.126719573170021, 266.1885948884980166 ) ) ;
#49923=CARTESIAN_POINT ( 'NONE',  ( -1.139345301468810190, 1509.018038237069959, 179.3524220471120145 ) ) ;
#49924=CARTESIAN_POINT ( 'NONE',  ( 11.50641715432830736, 1464.045072788057723, 231.7617761124168965 ) ) ;
#49926=CARTESIAN_POINT ( 'NONE',  ( -34.01975398719280008, 1437.014669684349883, 136.5579423247930038 ) ) ;
#49927=ORIENTED_EDGE ( 'NONE', *, *, #97413, .T. ) ;
#49933=CARTESIAN_POINT ( 'NONE',  ( 14.10951807380980050, 1475.045409909879936, 225.3878574613659964 ) ) ;
#49939=CARTESIAN_POINT ( 'NONE',  ( 40.71747595839759981, 1438.773003563400152, 135.3769917806320109 ) ) ;
#49942=CARTESIAN_POINT ( 'NONE',  ( 38.70145357755679782, 1443.913060387331370, 136.9791754767358611 ) ) ;
#49948=CARTESIAN_POINT ( 'NONE',  ( 11.77042837613340076, 1427.129776104949997, 146.4520242493910018 ) ) ;
#49949=CIRCLE ( 'NONE', #94602, 2.005929996893950573 ) ;
#49950=CARTESIAN_POINT ( 'NONE',  ( 20.01779028520000026, 1497.692402115730147, 228.4662795307979763 ) ) ;
#49952=CARTESIAN_POINT ( 'NONE',  ( -13.43950372030000118, 1415.041103191730144, 220.5860819401979995 ) ) ;
#49953=CARTESIAN_POINT ( 'NONE',  ( -11.81416737476160073, 1432.336398752800051, 150.4603277358870059 ) ) ;
#49956=CARTESIAN_POINT ( 'NONE',  ( 21.36074642202770235, 1409.675868270709998, 206.3811398801530004 ) ) ;
#49959=CARTESIAN_POINT ( 'NONE',  ( -8.704510423752683579, 1410.592478084298364, 187.9732723534475554 ) ) ;
#49961=CARTESIAN_POINT ( 'NONE',  ( -16.43752754770000024, 1507.637957936329940, 224.7124590378979860 ) ) ;
#49962=CARTESIAN_POINT ( 'NONE',  ( 15.10715599449999935, 1460.034514856529995, 231.8277951913980246 ) ) ;
#49967=CIRCLE ( 'NONE', #82155, 1.000002391210522257 ) ;
#49968=CARTESIAN_POINT ( 'NONE',  ( 18.04482939365169969, 1424.490669045140066, 224.3459621598859997 ) ) ;
#49969=VECTOR ( 'NONE', #58155, 1000.000000000000114 ) ;
#49973=CARTESIAN_POINT ( 'NONE',  ( -11.60004869885203682, 1425.972729341162221, 137.6380926570295173 ) ) ;
#49976=CARTESIAN_POINT ( 'NONE',  ( 0.7195380765500000164, 1435.002040243880174, 189.5252041397980065 ) ) ;
#49978=CARTESIAN_POINT ( 'NONE',  ( -11.67186513969999950, 1426.308431726130038, 146.8889338853980178 ) ) ;
#49981=CARTESIAN_POINT ( 'NONE',  ( 3.165116523870669774, 1422.680542800070043, 151.1404971254699774 ) ) ;
#49984=CARTESIAN_POINT ( 'NONE',  ( -23.52532681639999979, 1495.365128451330065, 222.1069804199980240 ) ) ;
#49986=CARTESIAN_POINT ( 'NONE',  ( -16.61688624562800243, 1459.964452065093838, 228.4923530358620098 ) ) ;
#49987=CIRCLE ( 'NONE', #26705, 2.009043929815852891 ) ;
#49988=EDGE_LOOP ( 'NONE', ( #47553, #56012, #30508, #27159 ) ) ;
#49990=CARTESIAN_POINT ( 'NONE',  ( 3.425626849559999965, 1406.160538305030059, 269.0410133635979832 ) ) ;
#49991=CARTESIAN_POINT ( 'NONE',  ( 0.2517737633129999986, 1408.921852534829895, 186.0321150700980013 ) ) ;
#49992=CARTESIAN_POINT ( 'NONE',  ( 24.61387732900000103, 1469.149509504730077, 202.9020163039279794 ) ) ;
#49994=CARTESIAN_POINT ( 'NONE',  ( 9.898869979169477418, 1506.751914348593118, 229.0672400497726073 ) ) ;
#49995=EDGE_CURVE ( 'NONE', #78944, #48269, #85338, .T. ) ;
#49997=CARTESIAN_POINT ( 'NONE',  ( -1.634203459049999863, 1450.563733768360180, 183.1247155458980274 ) ) ;
#50000=VECTOR ( 'NONE', #47960, 1000.000000000000000 ) ;
#50001=CARTESIAN_POINT ( 'NONE',  ( -13.55026637619999974, 1443.926177729530082, 187.1800506178979902 ) ) ;
#50002=EDGE_CURVE ( 'NONE', #83651, #88136, #80604, .T. ) ;
#50003=CARTESIAN_POINT ( 'NONE',  ( -20.64585313979999981, 1475.513060387329915, 209.1218459620799877 ) ) ;
#50006=CARTESIAN_POINT ( 'NONE',  ( 6.501109236959999649, 1407.992916451829842, 270.1283629016979830 ) ) ;
#50009=B_SPLINE_SURFACE_WITH_KNOTS ( 'NONE', 5, 5, ( 
 ( #4141, #48905, #108782, #107685, #98725, #89776 ),
 ( #89228, #39929, #56177, #55104, #12524, #14161 ),
 ( #72450, #106580, #29867, #30969, #91439, #64053 ),
 ( #4675, #74098, #23107, #90316, #98172, #38814 ),
 ( #31514, #65145, #13594, #30419, #99258, #22536 ),
 ( #65696, #57312, #83032, #14715, #75199, #24206 ) ),
 .UNSPECIFIED., .F., .F., .F.,
 ( 6, 6 ),
 ( 6, 6 ),
 ( 5.115886119869999860, 6.089794067229999719 ),
 ( 0.000000000000000000, 2.000000000000000000 ),
 .UNSPECIFIED. ) ;
#50012=CARTESIAN_POINT ( 'NONE',  ( -14.64892204319999891, 1474.348028616230067, 267.7626043892980192 ) ) ;
#50014=CARTESIAN_POINT ( 'NONE',  ( -22.37111836880000126, 1509.698977978930088, 189.8981514860979871 ) ) ;
#50015=CARTESIAN_POINT ( 'NONE',  ( -11.14879642162034834, 1486.511453154069613, 183.9882609373381683 ) ) ;
#50018=CARTESIAN_POINT ( 'NONE',  ( -9.470907091730000005, 1435.946707556030105, 153.1784963645979758 ) ) ;
#50019=B_SPLINE_SURFACE_WITH_KNOTS ( 'NONE', 5, 5, ( 
 ( #94166, #17436, #7962, #51634, #33161, #52744 ),
 ( #24737, #86878, #75737, #42129, #26412, #59494 ),
 ( #76279, #16883, #51088, #19100, #97488, #3453 ),
 ( #20756, #79059, #27525, #53873, #61710, #80690 ),
 ( #2907, #20216, #28075, #37581, #96392, #10172 ),
 ( #104789, #105903, #71219, #29723, #19668, #46002 ) ),
 .UNSPECIFIED., .F., .F., .F.,
 ( 6, 6 ),
 ( 6, 6 ),
 ( 6.633448128299999524, 17.60361827769999721 ),
 ( 0.000000000000000000, 2.000000000000000000 ),
 .UNSPECIFIED. ) ;
#50023=CARTESIAN_POINT ( 'NONE',  ( -17.22539857820000009, 1409.514584561230095, 195.8673760792980261 ) ) ;
#50030=CARTESIAN_POINT ( 'NONE',  ( 0.8197920095480000224, 1434.541746329560056, 150.4759714514979976 ) ) ;
#50039=AXIS2_PLACEMENT_3D ( 'NONE', #8730, #34499, #57660 ) ;
#50043=CARTESIAN_POINT ( 'NONE',  ( -0.01096399726330679961, 1407.225809184080163, 222.1218459612420020 ) ) ;
#50045=LINE ( 'NONE', #32676, #15996 ) ;
#50046=CARTESIAN_POINT ( 'NONE',  ( -13.01311093543085029, 1398.298642562823261, 209.5298158007715301 ) ) ;
#50051=CARTESIAN_POINT ( 'NONE',  ( 21.06226352934189805, 1509.331904505479997, 228.5875131670700000 ) ) ;
#50055=CARTESIAN_POINT ( 'NONE',  ( 12.00150264383820087, 1433.875911295109745, 150.4160741115419739 ) ) ;
#50056=CARTESIAN_POINT ( 'NONE',  ( -2.669690553840000202, 1397.993164424230145, 222.1390482242979942 ) ) ;
#50059=CARTESIAN_POINT ( 'NONE',  ( -26.26217022840000226, 1509.606683261929902, 199.1929658363279998 ) ) ;
#50060=CARTESIAN_POINT ( 'NONE',  ( 0.0002840614181677549835, 1443.913060387330006, 126.7977857662820043 ) ) ;
#50064=CARTESIAN_POINT ( 'NONE',  ( 17.76240486127710128, 1488.411413908479972, 229.6751878506049991 ) ) ;
#50065=CARTESIAN_POINT ( 'NONE',  ( 12.55860337799999904, 1449.228661195309996, 188.0919213263979941 ) ) ;
#50066=CARTESIAN_POINT ( 'NONE',  ( -9.626137457809999631, 1415.087974639930053, 194.4605678413980172 ) ) ;
#50069=CARTESIAN_POINT ( 'NONE',  ( 0.5697989934087799302, 1450.893162568020216, 155.6080914323170248 ) ) ;
#50070=CARTESIAN_POINT ( 'NONE',  ( 14.45556168306229949, 1416.765224586759814, 196.8540595995450246 ) ) ;
#50071=CARTESIAN_POINT ( 'NONE',  ( 11.30246509490000051, 1432.392618652180090, 151.5218479388979915 ) ) ;
#50072=CARTESIAN_POINT ( 'NONE',  ( 17.22592475670000312, 1443.913060387330006, 162.9227486557980171 ) ) ;
#50074=CARTESIAN_POINT ( 'NONE',  ( 13.11641504695559846, 1435.029372730620025, 149.9328725522570096 ) ) ;
#50075=VERTEX_POINT ( 'NONE', #2776 ) ;
#50076=ORIENTED_EDGE ( 'NONE', *, *, #107596, .T. ) ;
#50077=CARTESIAN_POINT ( 'NONE',  ( 13.16074665768760887, 1444.747289922009486, 169.3968467459069416 ) ) ;
#50078=CARTESIAN_POINT ( 'NONE',  ( -8.514170057680001236, 1463.332792388330063, 234.7542372413980161 ) ) ;
#50086=CARTESIAN_POINT ( 'NONE',  ( 2.500000000000000000, 1448.206111001999943, 170.1385578322760068 ) ) ;
#50091=CARTESIAN_POINT ( 'NONE',  ( 21.61868135606060193, 1440.913060387330006, 225.5306503608640014 ) ) ;
#50093=CARTESIAN_POINT ( 'NONE',  ( -18.84923767200000100, 1508.518338890729865, 229.8981134190979958 ) ) ;
#50094=CARTESIAN_POINT ( 'NONE',  ( -5.849946180559999931, 1410.053889712929958, 187.1442103566980109 ) ) ;
#50096=CARTESIAN_POINT ( 'NONE',  ( -0.6611933175131969875, 1415.434635989099888, 227.0678344611339980 ) ) ;
#50098=CARTESIAN_POINT ( 'NONE',  ( 18.32525213830000155, 1425.583872255029974, 224.3060837809979660 ) ) ;
#50099=CARTESIAN_POINT ( 'NONE',  ( 26.79413740735880367, 1436.761939593030093, 136.7822073642480234 ) ) ;
#50101=CARTESIAN_POINT ( 'NONE',  ( 6.012564370750140813E-06, 1465.118921926949952, 238.1343525961189869 ) ) ;
#50104=CARTESIAN_POINT ( 'NONE',  ( 13.58968549309999929, 1409.153350369530017, 270.0972160545979932 ) ) ;
#50106=CARTESIAN_POINT ( 'NONE',  ( 23.01274080199999972, 1409.742907276529877, 209.3054936816029965 ) ) ;
#50107=CARTESIAN_POINT ( 'NONE',  ( -20.80191066480000117, 1508.906210763929948, 189.9702950884980055 ) ) ;
#50111=DIRECTION ( 'NONE',  ( 1.000000000000000000, -3.330669073900915523E-12, -7.524258993698327080E-10 ) ) ;
#50113=CARTESIAN_POINT ( 'NONE',  ( 1.356522472024429993, 1410.335674015750101, 232.6399073486850000 ) ) ;
#50118=EDGE_CURVE ( 'NONE', #75143, #67449, #107374, .T. ) ;
#50119=B_SPLINE_SURFACE_WITH_KNOTS ( 'NONE', 5, 5, ( 
 ( #108117, #65035, #63952, #39265, #98067, #4575 ),
 ( #31968, #4039, #56080, #48239, #90206, #14610 ),
 ( #90769, #57203, #5111, #55543, #89667, #73440 ),
 ( #12953, #31411, #99152, #47134, #22431, #82380 ),
 ( #59403, #42032, #41486, #101908, #92971, #6758 ),
 ( #102466, #34174, #91874, #25200, #25756, #32530 ),
 ( #15147, #16244, #16787, #49890, #58287, #85119 ),
 ( #84573, #7865, #42580, #49336, #75647, #66701 ),
 ( #50990, #57753, #84022, #7323, #8407, #109246 ),
 ( #110331, #76731, #109786, #43, #68360, #76181 ),
 ( #67253, #59956, #94072, #93515, #15684, #33064 ),
 ( #33603, #67799, #83463, #40918, #101347, #75098 ) ),
 .UNSPECIFIED., .F., .F., .F.,
 ( 6, 3, 3, 6 ),
 ( 6, 6 ),
 ( 47.73522590250000519, 49.52849703180000063, 53.11503929029999682, 57.48082753679999968 ),
 ( 0.000000000000000000, 1.553560449149999911 ),
 .UNSPECIFIED. ) ;
#50120=CARTESIAN_POINT ( 'NONE',  ( 39.71670572960000101, 1443.385948747099974, 259.0959245980980086 ) ) ;
#50124=CARTESIAN_POINT ( 'NONE',  ( -23.94395295139999646, 1445.403820339119875, 213.0920108038580167 ) ) ;
#50125=LINE ( 'NONE', #84792, #84450 ) ;
#50129=CARTESIAN_POINT ( 'NONE',  ( 10.62911018238626681, 1424.057524227967860, 137.5666922152020106 ) ) ;
#50132=ADVANCED_FACE ( 'NONE', ( #12241 ), #19533, .F. ) ;
#50136=CARTESIAN_POINT ( 'NONE',  ( 12.73639929490000178, 1425.726110608229874, 223.7524270774979982 ) ) ;
#50140=CARTESIAN_POINT ( 'NONE',  ( -37.66849514949689848, 1445.052233488579986, 137.0436250779820000 ) ) ;
#50141=ADVANCED_FACE ( 'NONE', ( #105214 ), #63360, .F. ) ;
#50142=CARTESIAN_POINT ( 'NONE',  ( 27.59657415728649710, 1435.460754930439862, 135.6994131913330079 ) ) ;
#50143=CARTESIAN_POINT ( 'NONE',  ( -38.62863167585439328, 1444.143249040989986, 137.1666610592409938 ) ) ;
#50144=CARTESIAN_POINT ( 'NONE',  ( -23.74109072509999763, 1436.296643562969848, 212.5883282660480234 ) ) ;
#50145=CARTESIAN_POINT ( 'NONE',  ( -38.58901838188198496, 1459.202134673285173, 269.1648952399591508 ) ) ;
#50147=CARTESIAN_POINT ( 'NONE',  ( -17.07770202869999565, 1418.344327071730049, 226.6533663141979957 ) ) ;
#50149=CARTESIAN_POINT ( 'NONE',  ( -32.18870921241107652, 1460.503927282295081, 269.4955099690564566 ) ) ;
#50150=VERTEX_POINT ( 'NONE', #70349 ) ;
#50151=CARTESIAN_POINT ( 'NONE',  ( -26.68654750115280194, 1491.210633211110007, 210.8409592960780117 ) ) ;
#50152=CARTESIAN_POINT ( 'NONE',  ( -32.12964233707795358, 1416.641442875106577, 269.3130421961114394 ) ) ;
#50155=CARTESIAN_POINT ( 'NONE',  ( 14.15078481402130173, 1419.841391265170159, 190.8422908333620285 ) ) ;
#50157=CARTESIAN_POINT ( 'NONE',  ( -2.193083880730000129E-05, 1417.262443296330048, 235.9145984659979831 ) ) ;
#50158=CARTESIAN_POINT ( 'NONE',  ( -28.45309225929999641, 1509.159855972630112, 208.7911923258060085 ) ) ;
#50163=CARTESIAN_POINT ( 'NONE',  ( 44.93133457081440696, 1436.268913138369953, 269.6838197541450199 ) ) ;
#50164=CARTESIAN_POINT ( 'NONE',  ( -19.99928269779077894, 1450.982390009973869, 145.5778244573470488 ) ) ;
#50165=CARTESIAN_POINT ( 'NONE',  ( -16.96258009527109678, 1415.088012641449950, 209.3926123311109961 ) ) ;
#50166=CARTESIAN_POINT ( 'NONE',  ( 24.63108249569999941, 1435.637769007679935, 137.3321585077979989 ) ) ;
#50169=VECTOR ( 'NONE', #68171, 1000.000000000000114 ) ;
#50170=CARTESIAN_POINT ( 'NONE',  ( -0.1956065448698070253, 1414.913060387399810, 193.0575752666509857 ) ) ;
#50174=CARTESIAN_POINT ( 'NONE',  ( 17.97082642953529685, 1416.218047878440075, 208.7667215553299798 ) ) ;
#50176=CARTESIAN_POINT ( 'NONE',  ( -7.528156686780000051, 1459.758987806329969, 216.2975364203180106 ) ) ;
#50179=CARTESIAN_POINT ( 'NONE',  ( -10.98575270039999907, 1433.172656335930014, 151.7674558586979856 ) ) ;
#50181=CARTESIAN_POINT ( 'NONE',  ( -2.712300100236232581, 1420.170182972836528, 186.0200053761597587 ) ) ;
#50183=CARTESIAN_POINT ( 'NONE',  ( -24.29993749309999984, 1439.467978180069849, 211.6888154952279990 ) ) ;
#50186=CARTESIAN_POINT ( 'NONE',  ( 3.322969174999999886, 1451.336469026030045, 183.9873339521979858 ) ) ;
#50187=EDGE_CURVE ( 'NONE', #97278, #10122, #54648, .T. ) ;
#50189=CARTESIAN_POINT ( 'NONE',  ( -20.67345146974625081, 1509.752679656905684, 230.8614569593614760 ) ) ;
#50193=CARTESIAN_POINT ( 'NONE',  ( -11.76828283236710071, 1427.072440769260083, 146.3134061956550056 ) ) ;
#50195=CARTESIAN_POINT ( 'NONE',  ( -6.401487761410000310, 1472.929829178429827, 270.4245279986980108 ) ) ;
#50196=CARTESIAN_POINT ( 'NONE',  ( 11.99692654816771764, 1433.680601540482940, 147.5897107170167999 ) ) ;
#50199=CARTESIAN_POINT ( 'NONE',  ( 20.64585313979999981, 1475.513060387329915, 209.1218459613160121 ) ) ;
#50201=B_SPLINE_SURFACE_WITH_KNOTS ( 'NONE', 4, 5, ( 
 ( #36894, #88405, #31795, #101743, #7154, #16615 ),
 ( #15526, #6600, #50812, #109616, #49722, #58669 ),
 ( #92805, #100108, #101186, #5499, #16077, #39655 ),
 ( #24483, #65986, #91705, #48626, #57579, #108508 ),
 ( #33432, #67083, #83854, #50280, #40200, #65429 ) ),
 .UNSPECIFIED., .F., .F., .F.,
 ( 5, 5 ),
 ( 6, 6 ),
 ( 140.3375011859999972, 157.7108139780000045 ),
 ( -2.775557561569999727E-17, 1.000000000000000000 ),
 .UNSPECIFIED. ) ;
#50203=CARTESIAN_POINT ( 'NONE',  ( -15.53391875520000021, 1431.113060387329824, 198.5194791727979862 ) ) ;
#50206=CARTESIAN_POINT ( 'NONE',  ( -6.096347920628879535, 1406.294202297779975, 266.9462307650929915 ) ) ;
#50207=CARTESIAN_POINT ( 'NONE',  ( -13.24203370085249887, 1434.890687171669924, 149.2201380983239858 ) ) ;
#50209=DIRECTION ( 'NONE',  ( 0.000000000000000000, 1.000000000000000000, 0.000000000000000000 ) ) ;
#50211=ORIENTED_EDGE ( 'NONE', *, *, #14464, .T. ) ;
#50212=CARTESIAN_POINT ( 'NONE',  ( 4.969930027270518913, 1422.577112182319297, 184.4052530213058958 ) ) ;
#50217=CIRCLE ( 'NONE', #94876, 0.5869591139725545137 ) ;
#50218=CARTESIAN_POINT ( 'NONE',  ( -17.58460357419609821, 1489.029734904510178, 229.1403506008609838 ) ) ;
#50229=CARTESIAN_POINT ( 'NONE',  ( -26.62563451980019735, 1469.324738576180152, 209.5519976422650075 ) ) ;
#50230=CARTESIAN_POINT ( 'NONE',  ( 25.57394743849999941, 1488.682087793829851, 216.3815040199180260 ) ) ;
#50235=VECTOR ( 'NONE', #48762, 999.9999999999998863 ) ;
#50236=CARTESIAN_POINT ( 'NONE',  ( -24.35749803060000218, 1441.519803165160056, 211.7220366884380098 ) ) ;
#50240=CIRCLE ( 'NONE', #86081, 24.94174191160003318 ) ;
#50241=CARTESIAN_POINT ( 'NONE',  ( -14.37239935340000052, 1413.178551036030058, 226.9209306701980040 ) ) ;
#50242=DIRECTION ( 'NONE',  ( 0.000000000000000000, 1.000000000000000000, 0.000000000000000000 ) ) ;
#50244=VERTEX_POINT ( 'NONE', #78716 ) ;
#50245=CARTESIAN_POINT ( 'NONE',  ( -2.111185581749480011, 1451.947978409319830, 184.4701806085570013 ) ) ;
#50247=CARTESIAN_POINT ( 'NONE',  ( -19.12315338958239153, 1457.731911782933594, 226.6848971428718471 ) ) ;
#50251=EDGE_CURVE ( 'NONE', #10827, #74353, #39597, .T. ) ;
#50252=CARTESIAN_POINT ( 'NONE',  ( 12.78027909502899995, 1434.687120491519863, 149.6292676778430177 ) ) ;
#50253=CARTESIAN_POINT ( 'NONE',  ( 12.69480686662079805, 1459.299630678179938, 231.0330950081669812 ) ) ;
#50255=CARTESIAN_POINT ( 'NONE',  ( -3.171072485709999889, 1451.871858332230204, 182.7750508701979868 ) ) ;
#50261=CARTESIAN_POINT ( 'NONE',  ( -11.98890328080000067, 1442.756953654919926, 147.5994355510979688 ) ) ;
#50262=CARTESIAN_POINT ( 'NONE',  ( 20.50069307629999926, 1509.057110917230148, 189.1022581845979857 ) ) ;
#50264=ORIENTED_EDGE ( 'NONE', *, *, #77712, .T. ) ;
#50267=CARTESIAN_POINT ( 'NONE',  ( 0.4555793700929999801, 1420.350633689530014, 183.9786678279979810 ) ) ;
#50274=CARTESIAN_POINT ( 'NONE',  ( 18.24476709642540584, 1425.305388862659356, 224.8416608642366725 ) ) ;
#50276=CARTESIAN_POINT ( 'NONE',  ( -2.482344662330000062, 1440.444625599219989, 150.5580151863979950 ) ) ;
#50277=CARTESIAN_POINT ( 'NONE',  ( 27.74152896581870209, 1446.393007474679962, 137.1637341980689939 ) ) ;
#50279=CARTESIAN_POINT ( 'NONE',  ( -17.14943674877569890, 1460.897686246159992, 228.2718295297070199 ) ) ;
#50280=CARTESIAN_POINT ( 'NONE',  ( 12.86077854309999857, 1416.823634022829992, 221.8629616260980129 ) ) ;
#50283=ORIENTED_EDGE ( 'NONE', *, *, #72947, .F. ) ;
#50285=EDGE_CURVE ( 'NONE', #57273, #35617, #32866, .T. ) ;
#50287=CARTESIAN_POINT ( 'NONE',  ( -28.23788176520000093, 1509.669894704329863, 211.0744985972580139 ) ) ;
#50288=CARTESIAN_POINT ( 'NONE',  ( 2.410646146274223245, 1410.375392720130321, 185.5500677950892623 ) ) ;
#50289=CARTESIAN_POINT ( 'NONE',  ( 17.02668221408760019, 1422.112876149069962, 226.8213126862850118 ) ) ;
#50291=DIRECTION ( 'NONE',  ( -0.03489949670254138131, 0.9993908270190944299, 0.000000000000000000 ) ) ;
#50296=CARTESIAN_POINT ( 'NONE',  ( 3.636730251570000405, 1451.537370930130010, 154.1168901888979974 ) ) ;
#50302=DIRECTION ( 'NONE',  ( 0.9993902469235412811, 0.03489947644508400310, -0.001077449749359510062 ) ) ;
#50304=CARTESIAN_POINT ( 'NONE',  ( 19.78127211569570321, 1508.034666168520062, 229.2988164385099878 ) ) ;
#50308=CARTESIAN_POINT ( 'NONE',  ( 38.23937796074390860, 1438.847880936179990, 136.6258318260159967 ) ) ;
#50311=ADVANCED_FACE ( 'NONE', ( #25559 ), #42945, .T. ) ;
#50315=VECTOR ( 'NONE', #41999, 1000.000000000000000 ) ;
#50316=CARTESIAN_POINT ( 'NONE',  ( -12.84158769360459651, 1435.935367691730562, 150.8118236764398716 ) ) ;
#50317=CARTESIAN_POINT ( 'NONE',  ( -3.482404828285579956, 1485.996524617339901, 182.2044860649310181 ) ) ;
#50319=CARTESIAN_POINT ( 'NONE',  ( 3.015183704140000032, 1410.395849601029795, 185.7217229209980189 ) ) ;
#50321=ADVANCED_FACE ( 'NONE', ( #41830 ), #46668, .T. ) ;
#50323=CARTESIAN_POINT ( 'NONE',  ( 11.86593337849999941, 1432.333320123749900, 150.3971781299979966 ) ) ;
#50324=CARTESIAN_POINT ( 'NONE',  ( 11.74015299229400000, 1428.979986577520094, 144.1937996693850152 ) ) ;
#50325=ORIENTED_EDGE ( 'NONE', *, *, #11795, .T. ) ;
#50328=CARTESIAN_POINT ( 'NONE',  ( 4.304798037349998904E-15, 1432.353341358199941, 150.3995506339979897 ) ) ;
#50329=CARTESIAN_POINT ( 'NONE',  ( -2.370970874524634286, 1427.002265528474027, 134.0999999980980135 ) ) ;
#50330=CARTESIAN_POINT ( 'NONE',  ( 17.38693183890000071, 1507.629775627629897, 188.3940375129979827 ) ) ;
#50332=CARTESIAN_POINT ( 'NONE',  ( -9.458129699028839708E-09, 1472.949333146100116, 261.1319930289780018 ) ) ;
#50334=CARTESIAN_POINT ( 'NONE',  ( -0.5679639878839999323, 1416.568813547830132, 227.7576290933980090 ) ) ;
#50338=CARTESIAN_POINT ( 'NONE',  ( -0.2120479655457991053, 1485.995122961834340, 181.8315243526895983 ) ) ;
#50340=CARTESIAN_POINT ( 'NONE',  ( -45.65239911430659703, 1439.849390212310027, 266.1890414226530197 ) ) ;
#50341=CARTESIAN_POINT ( 'NONE',  ( -3.087788399999999989, 1439.686999668429962, 185.1123624746980170 ) ) ;
#50344=CARTESIAN_POINT ( 'NONE',  ( -2.478556036580000121, 1437.233840397999984, 157.6736397610980021 ) ) ;
#50345=CARTESIAN_POINT ( 'NONE',  ( 19.26968731915079047, 1456.385665059119447, 224.8316692866741562 ) ) ;
#50348=CARTESIAN_POINT ( 'NONE',  ( -26.66940587972800003, 1451.815323532959837, 135.6567935292860057 ) ) ;
#50350=CARTESIAN_POINT ( 'NONE',  ( 29.87497007670000215, 1438.990456222089961, 238.0574376903979896 ) ) ;
#50352=CARTESIAN_POINT ( 'NONE',  ( -17.06592007889999962, 1409.674274294630095, 194.3954626038980109 ) ) ;
#50353=CARTESIAN_POINT ( 'NONE',  ( -2.644608989403160137, 1419.519946857050172, 186.1458476411769993 ) ) ;
#50355=CARTESIAN_POINT ( 'NONE',  ( -10.37096375755954192, 1396.275222422115121, 217.1218459616979999 ) ) ;
#50359=CARTESIAN_POINT ( 'NONE',  ( -0.5945626521397818776, 1410.034456817089904, 269.8654418808179685 ) ) ;
#50360=CARTESIAN_POINT ( 'NONE',  ( 17.02686444325469850, 1422.113038003860083, 226.8212050067879773 ) ) ;
#50364=CARTESIAN_POINT ( 'NONE',  ( -23.33367609749780414, 1409.843005415879816, 208.9560767717839838 ) ) ;
#50366=CARTESIAN_POINT ( 'NONE',  ( 16.18975884877226790, 1409.478419224255049, 223.4272596155709039 ) ) ;
#50367=CARTESIAN_POINT ( 'NONE',  ( -41.79795361626952399, 1426.458837659412211, 266.3001450109010193 ) ) ;
#50368=CARTESIAN_POINT ( 'NONE',  ( -3.369548796489999720, 1498.349935238530179, 236.3379732119980190 ) ) ;
#50369=CARTESIAN_POINT ( 'NONE',  ( -22.03715318569999937, 1410.866002606429902, 214.8824533464280080 ) ) ;
#50370=CARTESIAN_POINT ( 'NONE',  ( 45.76102518337949476, 1443.713172479500145, 266.4159216563020323 ) ) ;
#50372=CARTESIAN_POINT ( 'NONE',  ( -16.44336187847212827, 1421.265292702081524, 226.9958026168290246 ) ) ;
#50374=EDGE_LOOP ( 'NONE', ( #106238, #5018, #109271, #45808 ) ) ;
#50375=CARTESIAN_POINT ( 'NONE',  ( 19.00753814766553518, 1457.296012680650620, 226.5174060896799233 ) ) ;
#50378=ORIENTED_EDGE ( 'NONE', *, *, #80868, .F. ) ;
#50379=FACE_OUTER_BOUND ( 'NONE', #59837, .T. ) ;
#50380=CARTESIAN_POINT ( 'NONE',  ( 26.87482465513500074, 1451.958209271989972, 135.1663978525000118 ) ) ;
#50382=CARTESIAN_POINT ( 'NONE',  ( 8.642986837300808745, 1452.611240636269940, 151.1117272551699955 ) ) ;
#50384=CARTESIAN_POINT ( 'NONE',  ( -4.134291178206661144, 1425.982862007858557, 186.1112856665070865 ) ) ;
#50386=CARTESIAN_POINT ( 'NONE',  ( 1.776918358778360130, 1408.975111743729940, 186.8671107929409914 ) ) ;
#50389=CARTESIAN_POINT ( 'NONE',  ( -4.026786250540000722, 1418.913060387330006, 172.2701767054979882 ) ) ;
#50394=CARTESIAN_POINT ( 'NONE',  ( 12.93261306534300026, 1416.826860677879949, 221.7400780573829877 ) ) ;
#50395=CARTESIAN_POINT ( 'NONE',  ( 11.24996440847739976, 1432.343753997600061, 151.5214208984010043 ) ) ;
#50404=CARTESIAN_POINT ( 'NONE',  ( -18.93537658710000215, 1468.059964608330120, 268.3665355204980187 ) ) ;
#50406=CARTESIAN_POINT ( 'NONE',  ( 11.68281581620000154, 1433.662110734889893, 151.0231821035980033 ) ) ;
#50407=EDGE_CURVE ( 'NONE', #94948, #38397, #66329, .T. ) ;
#50408=CARTESIAN_POINT ( 'NONE',  ( 11.47403709489999990, 1467.186912539730201, 262.6648722463980334 ) ) ;
#50409=CARTESIAN_POINT ( 'NONE',  ( 12.30902781860649853, 1415.426561690380140, 196.6799914669740019 ) ) ;
#50413=CARTESIAN_POINT ( 'NONE',  ( -15.76003452500000179, 1486.230153518429915, 186.5609880657980284 ) ) ;
#50414=CARTESIAN_POINT ( 'NONE',  ( 11.86363518809157647, 1398.264811432181887, 214.4375779453321513 ) ) ;
#50415=CARTESIAN_POINT ( 'NONE',  ( -17.85347883109999856, 1410.900113656230133, 225.0193030873980149 ) ) ;
#50416=AXIS2_PLACEMENT_3D ( 'NONE', #4148, #5797, #32085 ) ;
#50426=CARTESIAN_POINT ( 'NONE',  ( 0.1733418428536109834, 1478.369830831500167, 182.1644135495710088 ) ) ;
#50427=DIRECTION ( 'NONE',  ( 0.000000000000000000, 0.7071067811865475727, 0.7071067811865475727 ) ) ;
#50429=CARTESIAN_POINT ( 'NONE',  ( -20.77846844200000120, 1444.740067931809790, 176.2781434906979996 ) ) ;
#50432=CARTESIAN_POINT ( 'NONE',  ( -40.01221335562710379, 1438.828034966029918, 134.0999999981109738 ) ) ;
#50434=EDGE_LOOP ( 'NONE', ( #102637, #3330, #14895, #68124 ) ) ;
#50435=DIRECTION ( 'NONE',  ( 1.000000000000000000, 0.000000000000000000, 0.000000000000000000 ) ) ;
#50442=CARTESIAN_POINT ( 'NONE',  ( 7.369537115729440480, 1409.170410294239900, 222.1470682314269993 ) ) ;
#50449=CARTESIAN_POINT ( 'NONE',  ( -15.73561791997630088, 1409.462558364120014, 225.3904801341000166 ) ) ;
#50451=ORIENTED_EDGE ( 'NONE', *, *, #78695, .T. ) ;
#50457=CARTESIAN_POINT ( 'NONE',  ( 41.27403068698424704, 1446.758019147874620, 269.6337390305045005 ) ) ;
#50459=CARTESIAN_POINT ( 'NONE',  ( 18.39211149378427379, 1435.897264093365948, 214.5601621755202757 ) ) ;
#50460=CARTESIAN_POINT ( 'NONE',  ( 1.552710838619999922, 1417.100030409630108, 233.1250354766980024 ) ) ;
#50466=CARTESIAN_POINT ( 'NONE',  ( 2.500000000000000000, 1448.210448412299911, 170.5244215879980061 ) ) ;
#50467=ORIENTED_EDGE ( 'NONE', *, *, #33938, .F. ) ;
#50469=CARTESIAN_POINT ( 'NONE',  ( 32.44714059009999829, 1466.431271693930057, 269.3248281139979667 ) ) ;
#50475=CARTESIAN_POINT ( 'NONE',  ( -23.51192877400000114, 1410.913812961229951, 206.4143556372079615 ) ) ;
#50476=CARTESIAN_POINT ( 'NONE',  ( -11.16073650870000122, 1426.886991639529924, 102.3049941106980043 ) ) ;
#50477=CARTESIAN_POINT ( 'NONE',  ( 15.80609125907960255, 1409.490806506669969, 192.6604916703820152 ) ) ;
#50479=CARTESIAN_POINT ( 'NONE',  ( 36.86583086841639556, 1437.713619129489871, 136.5403217841159744 ) ) ;
#50482=CARTESIAN_POINT ( 'NONE',  ( -39.71667698230000099, 1438.440173584909871, 259.0958797427979903 ) ) ;
#50483=CARTESIAN_POINT ( 'NONE',  ( -0.1339064907639219981, 1508.974573961829947, 179.3682901727229932 ) ) ;
#50486=CARTESIAN_POINT ( 'NONE',  ( 38.54572101799519857, 1450.058425145439969, 134.0999999982749955 ) ) ;
#50487=CARTESIAN_POINT ( 'NONE',  ( -39.17232000345539689, 1439.963336824750058, 136.7246149087999925 ) ) ;
#50500=CARTESIAN_POINT ( 'NONE',  ( -15.10371725490000117, 1409.440493816029857, 225.2902966875980155 ) ) ;
#50509=CARTESIAN_POINT ( 'NONE',  ( 11.80796784730199889, 1428.630476879899788, 148.5709776132119657 ) ) ;
#50512=CARTESIAN_POINT ( 'NONE',  ( 14.59277107062129986, 1436.244837967300100, 149.8707660814949918 ) ) ;
#50513=CARTESIAN_POINT ( 'NONE',  ( -16.68498601116327151, 1442.773887286369018, 162.0933193695679222 ) ) ;
#50516=CARTESIAN_POINT ( 'NONE',  ( 21.24774881647060099, 1409.658413723660033, 206.3980491481210038 ) ) ;
#50519=CARTESIAN_POINT ( 'NONE',  ( -9.123972348892126050, 1410.606870705112215, 188.1126544915522913 ) ) ;
#50521=CARTESIAN_POINT ( 'NONE',  ( -15.43453510460000011, 1462.585142083830078, 223.2687737027980006 ) ) ;
#50525=CARTESIAN_POINT ( 'NONE',  ( -5.437469379731239449, 1506.424482793976722, 187.8301161205860410 ) ) ;
#50526=ORIENTED_EDGE ( 'NONE', *, *, #94458, .F. ) ;
#50530=CARTESIAN_POINT ( 'NONE',  ( -2.947166520632872988, 1485.291949360874924, 182.9808020193160587 ) ) ;
#50533=ORIENTED_EDGE ( 'NONE', *, *, #9714, .T. ) ;
#50534=CARTESIAN_POINT ( 'NONE',  ( 1.331830187880000071, 1453.151875979030137, 188.5601980120979988 ) ) ;
#50536=CARTESIAN_POINT ( 'NONE',  ( -10.91072510809999940, 1428.225676817730118, 150.5333655099979921 ) ) ;
#50538=CYLINDRICAL_SURFACE ( 'NONE', #88496, 26.99999999999999289 ) ;
#50542=CARTESIAN_POINT ( 'NONE',  ( -19.52587859339999810, 1470.090240710929947, 227.0208896569980084 ) ) ;
#50547=CARTESIAN_POINT ( 'NONE',  ( 26.68674721769999891, 1413.099522324730060, 269.4193621475980081 ) ) ;
#50548=CARTESIAN_POINT ( 'NONE',  ( 22.89198443360000113, 1435.442148801120084, 140.5684033940979987 ) ) ;
#50549=CARTESIAN_POINT ( 'NONE',  ( 19.05265570330000102, 1449.733526242509924, 192.0691012804980176 ) ) ;
#50550=ADVANCED_FACE ( 'NONE', ( #53011 ), #78749, .T. ) ;
#50551=CARTESIAN_POINT ( 'NONE',  ( 20.01203290568441773, 1426.583398916021451, 221.2898012671467143 ) ) ;
#50553=CARTESIAN_POINT ( 'NONE',  ( 11.87823649874709986, 1433.207008023099888, 147.6493504979379736 ) ) ;
#50554=CARTESIAN_POINT ( 'NONE',  ( 2.500000000000000000, 1439.615672362369878, 176.6480837420980095 ) ) ;
#50556=CARTESIAN_POINT ( 'NONE',  ( -13.30879681040000051, 1445.197123204520040, 187.8034403054980146 ) ) ;
#50558=CARTESIAN_POINT ( 'NONE',  ( -16.66821264700000071, 1497.713060387329961, 224.4060481835979886 ) ) ;
#50565=CARTESIAN_POINT ( 'NONE',  ( -12.63400943340000104, 1474.287538769530101, 269.2355652850980050 ) ) ;
#50570=CARTESIAN_POINT ( 'NONE',  ( 19.03110457515579768, 1457.047041246000163, 226.1578386336209974 ) ) ;
#50571=CARTESIAN_POINT ( 'NONE',  ( -5.773159728049999117E-15, 1442.756953654919926, 155.7628527808980152 ) ) ;
#50574=DIRECTION ( 'NONE',  ( -1.000000000000000000, -1.267952440776734034E-09, 6.874604651021009972E-10 ) ) ;
#50575=CARTESIAN_POINT ( 'NONE',  ( -22.94994330970000362, 1410.635878578629899, 204.6714796687680007 ) ) ;
#50583=CARTESIAN_POINT ( 'NONE',  ( 11.70423387253950054, 1426.717280763200051, 141.8225260926249973 ) ) ;
#50587=CARTESIAN_POINT ( 'NONE',  ( 11.60004869885203860, 1428.965959225140750, 137.0999999980979851 ) ) ;
#50590=CARTESIAN_POINT ( 'NONE',  ( -11.80537760282536119, 1398.263100982790093, 203.6771685272100001 ) ) ;
#50591=DIRECTION ( 'NONE',  ( 0.4794255386042036160, 0.000000000000000000, 0.8775825618903725367 ) ) ;
#50594=CARTESIAN_POINT ( 'NONE',  ( 22.38660642171149817, 1509.694817746930084, 228.2841629394400229 ) ) ;
#50596=EDGE_LOOP ( 'NONE', ( #7243, #46947, #11187, #43984, #107879 ) ) ;
#50598=CARTESIAN_POINT ( 'NONE',  ( 11.97738863534810072, 1433.633111691630120, 150.0666321391890392 ) ) ;
#50599=CARTESIAN_POINT ( 'NONE',  ( -2.393224162990000181, 1395.996633616729923, 220.4495428705980089 ) ) ;
#50601=CARTESIAN_POINT ( 'NONE',  ( -0.0002584699284550677598, 1396.263918536362098, 221.2551011699866024 ) ) ;
#50604=CARTESIAN_POINT ( 'NONE',  ( 2.370970874524634286, 1427.002265528474027, 134.0999999980979851 ) ) ;
#50605=CARTESIAN_POINT ( 'NONE',  ( 17.43533191579999908, 1424.302130621530068, 226.6671662756980083 ) ) ;
#50606=CARTESIAN_POINT ( 'NONE',  ( 17.77010835247230247, 1498.112583753600120, 230.1664113477359876 ) ) ;
#50607=CARTESIAN_POINT ( 'NONE',  ( 0.8908956287060000312, 1468.708728676529972, 182.6671616012979769 ) ) ;
#50611=CARTESIAN_POINT ( 'NONE',  ( 2.211127611826209982, 1395.990274664960225, 198.3288829735440117 ) ) ;
#50612=CARTESIAN_POINT ( 'NONE',  ( 1.316362887779999991, 1415.041103189330215, 191.5323437754979921 ) ) ;
#50613=CARTESIAN_POINT ( 'NONE',  ( 10.96882372829999852, 1432.300972684430008, 151.7702498152980297 ) ) ;
#50616=CARTESIAN_POINT ( 'NONE',  ( 13.39145132700120122, 1435.009615361580018, 149.5108276884409975 ) ) ;
#50619=CARTESIAN_POINT ( 'NONE',  ( 13.22577696261745039, 1444.679985164650816, 169.3877355158035698 ) ) ;
#50620=CARTESIAN_POINT ( 'NONE',  ( -4.909144810329999942, 1464.788387721129993, 235.1559025205980049 ) ) ;
#50628=B_SPLINE_CURVE_WITH_KNOTS ( 'NONE', 3,
 ( #30398, #80817, #72431, #100364, #21968, #56160, #106563, #89758, #64589, #90854, #47216, #6306, #82469, #74628, #47762, #5203, #64036, #57295, #98152, #14141, #21426, #107666, #81343, #48330, #4656, #30952, #91958, #65127, #99240, #40451, #22515, #5767, #74080, #108209, #23087, #91422, #14697, #48886, #108763, #46686, #32055, #23650, #68853, #94563, #66790, #52040, #43082, #18952, #15235 ),
 .UNSPECIFIED., .F., .F.,
 ( 4, 3, 3, 3, 3, 3, 3, 3, 3, 3, 3, 3, 3, 3, 3, 3, 4 ),
 ( 0.000000000000000000, 0.1298111464596899967, 0.2614081304872279965, 0.3961310922636709919, 0.5284374970052909681, 0.6643687372991460283, 0.7931396734179789743, 0.8002999775929999782, 1.059465424392620037, 1.309520818660049990, 1.559475944711749884, 1.808681423173479796, 2.056514135787280040, 2.301333315630279763, 2.543978965925790092, 2.783061379017449877, 2.873623551990000191 ),
 .UNSPECIFIED. ) ;
#50631=ORIENTED_EDGE ( 'NONE', *, *, #18286, .T. ) ;
#50634=ADVANCED_FACE ( 'NONE', ( #105616 ), #52547, .T. ) ;
#50635=CARTESIAN_POINT ( 'NONE',  ( -4.163739766079999960, 1409.058461383930080, 188.2538941213980195 ) ) ;
#50638=CARTESIAN_POINT ( 'NONE',  ( -0.2679975439270000370, 1416.543503932829935, 227.4610302084980162 ) ) ;
#50640=CARTESIAN_POINT ( 'NONE',  ( 24.57285633690000282, 1439.622216053659940, 213.1838506830980009 ) ) ;
#50648=CARTESIAN_POINT ( 'NONE',  ( -21.86920309050000100, 1509.656483798930140, 190.1619192503980003 ) ) ;
#50652=CARTESIAN_POINT ( 'NONE',  ( 14.30200421219999996, 1410.347835407430239, 191.4195238701979633 ) ) ;
#50653=CARTESIAN_POINT ( 'NONE',  ( -11.54861356885641044, 1486.021746504592329, 184.4896162731949687 ) ) ;
#50657=CARTESIAN_POINT ( 'NONE',  ( 33.93600685300000208, 1457.486634655030002, 259.3468319324980484 ) ) ;
#50660=CARTESIAN_POINT ( 'NONE',  ( -23.95803383590000379, 1445.274057039780018, 213.2142028417179915 ) ) ;
#50661=CARTESIAN_POINT ( 'NONE',  ( 0.6079674380864850125, 1452.959918024070021, 183.3081617366339913 ) ) ;
#50662=CARTESIAN_POINT ( 'NONE',  ( -2.500000000000000000, 1425.929641636930000, 178.2078840400980084 ) ) ;
#50668=CARTESIAN_POINT ( 'NONE',  ( -0.2726096272919999453, 1487.204355548130025, 230.5507616997979881 ) ) ;
#50669=CARTESIAN_POINT ( 'NONE',  ( 24.62744524829999904, 1442.406980887019927, 212.8172870668879852 ) ) ;
#50672=CARTESIAN_POINT ( 'NONE',  ( 26.02899615147670076, 1450.772943025348695, 136.7241299949539552 ) ) ;
#50673=CARTESIAN_POINT ( 'NONE',  ( 10.73431074182437328, 1418.150870888782492, 229.8889230194085656 ) ) ;
#50674=CARTESIAN_POINT ( 'NONE',  ( 32.03035082978020398, 1436.091942216389953, 136.3581855157840153 ) ) ;
#50675=CARTESIAN_POINT ( 'NONE',  ( 39.75685596340139938, 1446.397812216890088, 136.7371007338339837 ) ) ;
#50676=CARTESIAN_POINT ( 'NONE',  ( 8.410267065803780360E-17, 1471.436294031830130, 269.3346704751489824 ) ) ;
#50679=CARTESIAN_POINT ( 'NONE',  ( 8.482872683409999226, 1508.704761105730086, 182.5447718006980153 ) ) ;
#50684=CARTESIAN_POINT ( 'NONE',  ( 13.27700334932523951, 1506.366982238135279, 191.6232499193883427 ) ) ;
#50688=CARTESIAN_POINT ( 'NONE',  ( -0.4966801320660000352, 1415.438062173830076, 233.3911217857980205 ) ) ;
#50690=CARTESIAN_POINT ( 'NONE',  ( -29.27919551730000336, 1509.872435209829746, 208.8759114952370055 ) ) ;
#50693=CARTESIAN_POINT ( 'NONE',  ( -11.19695579387275863, 1418.593385094034375, 229.3149266084969895 ) ) ;
#50694=CARTESIAN_POINT ( 'NONE',  ( -7.821557675210984328, 1451.395427275060001, 152.9976685588227951 ) ) ;
#50696=CARTESIAN_POINT ( 'NONE',  ( 25.06611318670000088, 1436.294882506480008, 137.6250933127980147 ) ) ;
#50697=( BOUNDED_CURVE ( )  B_SPLINE_CURVE ( 3, ( #78101, #9791, #36112, #35543 ),
 .UNSPECIFIED., .F., .F. ) 
 B_SPLINE_CURVE_WITH_KNOTS ( ( 4, 4 ),
 ( 4.177675728947532363, 5.247004315084660142 ),
 .UNSPECIFIED. ) 
 CURVE ( )  GEOMETRIC_REPRESENTATION_ITEM ( )  RATIONAL_B_SPLINE_CURVE ( ( 1.000000000000000000, 0.9069598253110926489, 0.9069598253110926489, 1.000000000000000000 ) ) 
 REPRESENTATION_ITEM ( '' )  );
#50698=CARTESIAN_POINT ( 'NONE',  ( 35.07315792529999499, 1444.191445724089817, 137.2843330345980064 ) ) ;
#50700=CARTESIAN_POINT ( 'NONE',  ( 0.3266950887905089584, 1415.429375168339902, 191.4648083493140120 ) ) ;
#50702=ORIENTED_EDGE ( 'NONE', *, *, #9075, .F. ) ;
#50703=VERTEX_POINT ( 'NONE', #24338 ) ;
#50707=CARTESIAN_POINT ( 'NONE',  ( -19.87540907819999703, 1452.861698873429987, 216.4112603940479858 ) ) ;
#50709=CARTESIAN_POINT ( 'NONE',  ( 4.169165030684239603, 1424.160883088660057, 184.4444951202710001 ) ) ;
#50712=CARTESIAN_POINT ( 'NONE',  ( -2.498700678426172939, 1421.135883849067341, 185.0048294103856676 ) ) ;
#50714=CARTESIAN_POINT ( 'NONE',  ( -24.19213419669999610, 1438.598800249630131, 211.7608300950280125 ) ) ;
#50716=CARTESIAN_POINT ( 'NONE',  ( 1.528898867239999904, 1450.858514550550126, 182.5684021596979960 ) ) ;
#50718=CARTESIAN_POINT ( 'NONE',  ( -27.56847755513489062, 1509.987811263605408, 197.2905327719515185 ) ) ;
#50719=CARTESIAN_POINT ( 'NONE',  ( -2.804568549241229620E-09, 1414.830288601209986, 244.9882278679610010 ) ) ;
#50720=ORIENTED_EDGE ( 'NONE', *, *, #26674, .T. ) ;
#50723=CARTESIAN_POINT ( 'NONE',  ( -19.88052731184480137, 1484.560536701516867, 191.1415595291306602 ) ) ;
#50724=CARTESIAN_POINT ( 'NONE',  ( -3.472352184000000008, 1472.519747990830183, 270.3710077336979793 ) ) ;
#50729=CARTESIAN_POINT ( 'NONE',  ( -22.91663120903140083, 1507.606285602550088, 207.6071078552859888 ) ) ;
#50732=CARTESIAN_POINT ( 'NONE',  ( -23.80723810840019894, 1411.676400612559974, 269.4670551916460113 ) ) ;
#50733=CARTESIAN_POINT ( 'NONE',  ( -14.56157998151809885, 1435.986635814069814, 149.8060811127620013 ) ) ;
#50734=ORIENTED_EDGE ( 'NONE', *, *, #32346, .F. ) ;
#50736=CARTESIAN_POINT ( 'NONE',  ( 13.43628448359999972, 1443.378768469500073, 188.3384116640980039 ) ) ;
#50739=CARTESIAN_POINT ( 'NONE',  ( 5.026278901445378366, 1423.016945676001569, 184.4099619136632953 ) ) ;
#50742=CARTESIAN_POINT ( 'NONE',  ( -19.28103481819999843, 1485.491211888429916, 189.7669585599980167 ) ) ;
#50744=ORIENTED_EDGE ( 'NONE', *, *, #49995, .T. ) ;
#50746=ADVANCED_FACE ( 'NONE', ( #92648 ), #89256, .F. ) ;
#50750=CARTESIAN_POINT ( 'NONE',  ( -26.92695807870000380, 1508.008395488129963, 203.1594552079080245 ) ) ;
#50755=CARTESIAN_POINT ( 'NONE',  ( -6.688849051720000105, 1408.965348141229924, 196.7627783315979855 ) ) ;
#50759=CARTESIAN_POINT ( 'NONE',  ( -25.19786267552049708, 1449.936431062559905, 210.5275732939500131 ) ) ;
#50760=CARTESIAN_POINT ( 'NONE',  ( 26.66930585240000084, 1508.126733773130127, 215.8812207616579997 ) ) ;
#50761=AXIS2_PLACEMENT_3D ( 'NONE', #80632, #35881, #71726 ) ;
#50765=CARTESIAN_POINT ( 'NONE',  ( -24.69200176050000195, 1435.857451379459917, 137.7788013625980170 ) ) ;
#50772=VERTEX_POINT ( 'NONE', #80828 ) ;
#50773=CARTESIAN_POINT ( 'NONE',  ( -40.71747596959829707, 1448.637563236699862, 134.4203405313490123 ) ) ;
#50774=CARTESIAN_POINT ( 'NONE',  ( -1.912834366250000029, 1412.842211185330143, 232.9360292305979954 ) ) ;
#50775=EDGE_CURVE ( 'NONE', #79540, #33227, #26582, .T. ) ;
#50776=CARTESIAN_POINT ( 'NONE',  ( -19.68132502244943893, 1456.948574072194788, 225.7511772315920950 ) ) ;
#50777=ORIENTED_EDGE ( 'NONE', *, *, #95243, .F. ) ;
#50779=CARTESIAN_POINT ( 'NONE',  ( 12.94392783832900129, 1435.642753611090029, 150.6515099629039867 ) ) ;
#50781=CARTESIAN_POINT ( 'NONE',  ( 15.19613196592609938, 1459.303298073210044, 229.7660246535220097 ) ) ;
#50784=CARTESIAN_POINT ( 'NONE',  ( 26.85712173870000186, 1451.975206518229925, 134.9164576279979997 ) ) ;
#50787=CARTESIAN_POINT ( 'NONE',  ( 13.15726448907880020, 1416.913057013679918, 198.3331256186419864 ) ) ;
#50791=CARTESIAN_POINT ( 'NONE',  ( 20.81411617090000021, 1509.690291770430122, 187.8298652661979986 ) ) ;
#50792=CARTESIAN_POINT ( 'NONE',  ( 0.1595995995380000143, 1486.508831850330125, 181.8147405652979671 ) ) ;
#50793=EDGE_LOOP ( 'NONE', ( #91039, #47138, #89653, #66733 ) ) ;
#50795=B_SPLINE_SURFACE_WITH_KNOTS ( 'NONE', 5, 5, ( 
 ( #36014, #70206, #104312, #27603, #95911, #42753 ),
 ( #53378, #104864, #87524, #10814, #44983, #28152 ),
 ( #62342, #79681, #90247, #20288, #21373, #72384 ),
 ( #12450, #98101, #29257, #54494, #97567, #30346 ),
 ( #5150, #46634, #3533, #39305, #4076, #71863 ),
 ( #89161, #107062, #28711, #20839, #99190, #88082 ) ),
 .UNSPECIFIED., .F., .F., .F.,
 ( 6, 6 ),
 ( 6, 6 ),
 ( 15.04009677950000068, 20.59615426749999756 ),
 ( 0.000000000000000000, 2.000000000000000000 ),
 .UNSPECIFIED. ) ;
#50797=ORIENTED_EDGE ( 'NONE', *, *, #16575, .F. ) ;
#50799=CARTESIAN_POINT ( 'NONE',  ( 0.3035066335680000060, 1419.252317566729971, 184.6483442805979962 ) ) ;
#50802=CARTESIAN_POINT ( 'NONE',  ( 9829.078716723830439, 2833.596074015639715, -1083.720023828199828 ) ) ;
#50805=CARTESIAN_POINT ( 'NONE',  ( 18.94485037129999583, 1416.547221147930031, 210.4653698564179933 ) ) ;
#50806=CARTESIAN_POINT ( 'NONE',  ( 14.88455792500072228, 1507.555497567031580, 232.3243931051981406 ) ) ;
#50808=CARTESIAN_POINT ( 'NONE',  ( -12.00000000000000000, 1443.913060387330006, 147.5878346084980137 ) ) ;
#50809=CARTESIAN_POINT ( 'NONE',  ( 26.04901694399470102, 1446.564900598870054, 138.1454005870479875 ) ) ;
#50811=CARTESIAN_POINT ( 'NONE',  ( 26.19952982486130111, 1509.827968087110094, 209.0871425590960087 ) ) ;
#50812=CARTESIAN_POINT ( 'NONE',  ( 13.09590858069999975, 1426.025605857829987, 222.2823526253980049 ) ) ;
#50813=ORIENTED_EDGE ( 'NONE', *, *, #83912, .F. ) ;
#50816=CARTESIAN_POINT ( 'NONE',  ( -19.74447868890439040, 1485.088289844508154, 190.4769327812108202 ) ) ;
#50817=CARTESIAN_POINT ( 'NONE',  ( -28.29497435070000222, 1509.672356513830209, 211.0137316004380068 ) ) ;
#50818=CARTESIAN_POINT ( 'NONE',  ( 3.457627847960712320, 1410.410824016061724, 185.8561312258957514 ) ) ;
#50819=CARTESIAN_POINT ( 'NONE',  ( -3.421145496696929023, 1426.005600530342690, 185.8301723314418155 ) ) ;
#50831=ORIENTED_EDGE ( 'NONE', *, *, #103398, .T. ) ;
#50832=CARTESIAN_POINT ( 'NONE',  ( -0.5133638609672289688, 1410.311096993930050, 233.1717005261690190 ) ) ;
#50835=ORIENTED_EDGE ( 'NONE', *, *, #77392, .F. ) ;
#50836=VERTEX_POINT ( 'NONE', #101449 ) ;
#50837=CARTESIAN_POINT ( 'NONE',  ( 18.11450235977809697, 1507.710540422290023, 230.4427282681980103 ) ) ;
#50839=CARTESIAN_POINT ( 'NONE',  ( 38.12415249455629862, 1438.740481096789836, 136.6172136615510055 ) ) ;
#50840=CARTESIAN_POINT ( 'NONE',  ( -11.87227031139999944, 1435.412617320299887, 147.6610825172980128 ) ) ;
#50847=CARTESIAN_POINT ( 'NONE',  ( -0.4725090652239359867, 1450.961208915834504, 181.9239884145632118 ) ) ;
#50849=CARTESIAN_POINT ( 'NONE',  ( 4.486565162759999836, 1409.573462333729822, 186.4102199717980284 ) ) ;
#50850=CARTESIAN_POINT ( 'NONE',  ( 4.087244338739999705, 1424.194161142730081, 184.7150739516980025 ) ) ;
#50852=CARTESIAN_POINT ( 'NONE',  ( -2.500000000000000000, 1439.245488529090153, 159.3585436906180348 ) ) ;
#50854=CARTESIAN_POINT ( 'NONE',  ( -2.951770618412270064, 1451.103496634380008, 184.7382020502219859 ) ) ;
#50855=CARTESIAN_POINT ( 'NONE',  ( 0.4196953096899999625, 1466.017965088330129, 235.8216877134980223 ) ) ;
#50858=CARTESIAN_POINT ( 'NONE',  ( -2.424063131930000115, 1427.257651041929876, 147.9020499575979954 ) ) ;
#50859=CARTESIAN_POINT ( 'NONE',  ( 11.78238356083980065, 1440.882651838439870, 188.1224447589279976 ) ) ;
#50860=CARTESIAN_POINT ( 'NONE',  ( 22.28696231330000188, 1506.798305107829947, 209.3970118511340104 ) ) ;
#50863=CARTESIAN_POINT ( 'NONE',  ( -1.299075913466369845E-09, 1471.155365519019824, 256.9781891023540652 ) ) ;
#50866=CARTESIAN_POINT ( 'NONE',  ( -0.8945944849849999381, 1417.298095640030169, 235.8147265461980169 ) ) ;
#50869=CARTESIAN_POINT ( 'NONE',  ( -0.04668112204882676752, 1486.220989728969016, 181.8154795728657405 ) ) ;
#50871=CARTESIAN_POINT ( 'NONE',  ( -46.19910792603680250, 1438.826958754830002, 267.5922038166469292 ) ) ;
#50872=CARTESIAN_POINT ( 'NONE',  ( 13.94394020758319819, 1509.346948278499895, 234.4482500451630074 ) ) ;
#50880=CARTESIAN_POINT ( 'NONE',  ( -25.27414439665539803, 1452.025395757659908, 135.5207945563980161 ) ) ;
#50882=CARTESIAN_POINT ( 'NONE',  ( 21.83685800909999841, 1429.816530635930121, 221.4941967423980032 ) ) ;
#50887=CARTESIAN_POINT ( 'NONE',  ( -2.115949517696979587, 1419.508337143739709, 185.9017425962819914 ) ) ;
#50889=CARTESIAN_POINT ( 'NONE',  ( -24.40164416920000079, 1439.300524262840099, 211.9534758538480332 ) ) ;
#50891=ADVANCED_FACE ( 'NONE', ( #15780 ), #84665, .F. ) ;
#50892=CARTESIAN_POINT ( 'NONE',  ( -14.27715603315103543, 1416.818673810148084, 221.7183468844290530 ) ) ;
#50893=CARTESIAN_POINT ( 'NONE',  ( -18.79647803339999967, 1416.822694190429729, 208.4084638389329882 ) ) ;
#50895=CARTESIAN_POINT ( 'NONE',  ( -1.243032230405529903, 1408.244502896100130, 270.3924218761350176 ) ) ;
#50896=CARTESIAN_POINT ( 'NONE',  ( 12.34120302092700072, 1420.636070528880055, 230.5426365944759937 ) ) ;
#50898=EDGE_LOOP ( 'NONE', ( #53980, #45000, #15929, #90528 ) ) ;
#50900=CARTESIAN_POINT ( 'NONE',  ( -23.01060016338059810, 1409.833637653050118, 209.8936558164379846 ) ) ;
#50903=CARTESIAN_POINT ( 'NONE',  ( -2.329729395510000245, 1427.373795049630189, 123.0297916884979941 ) ) ;
#50905=CARTESIAN_POINT ( 'NONE',  ( -19.14510341657199888, 1447.481386810810136, 194.0904547693720019 ) ) ;
#50907=CARTESIAN_POINT ( 'NONE',  ( -18.60329415920000073, 1410.876893835729788, 223.7172180216979882 ) ) ;
#50908=CARTESIAN_POINT ( 'NONE',  ( 32.63392384532819790, 1464.921899099569828, 269.3041819200249734 ) ) ;
#50910=CARTESIAN_POINT ( 'NONE',  ( -16.47782421224261995, 1421.308645812501709, 226.9890287628209649 ) ) ;
#50913=CARTESIAN_POINT ( 'NONE',  ( -11.93562773578777048, 1433.536277773312577, 150.1881492786055219 ) ) ;
#50918=CARTESIAN_POINT ( 'NONE',  ( 27.02694966472599702, 1451.203421905880077, 136.2754127003069868 ) ) ;
#50924=B_SPLINE_SURFACE_WITH_KNOTS ( 'NONE', 5, 5, ( 
 ( #9884, #51333, #68715, #10999, #27793, #104500 ),
 ( #35634, #102820, #44611, #17142, #2068, #9341 ),
 ( #95547, #96095, #10439, #42948, #27243, #44052 ),
 ( #53015, #86043, #61980, #415, #1503, #70383 ),
 ( #59755, #43503, #2622, #17699, #19371, #95001 ),
 ( #69828, #18269, #53574, #36199, #18820, #26676 ) ),
 .UNSPECIFIED., .F., .F., .F.,
 ( 6, 6 ),
 ( 6, 6 ),
 ( 5.220737937810000062, 7.751661675270000273 ),
 ( 0.000000000000000000, 2.000000000000000000 ),
 .UNSPECIFIED. ) ;
#50926=AXIS2_PLACEMENT_3D ( 'NONE', #94985, #43490, #104485 ) ;
#50927=CARTESIAN_POINT ( 'NONE',  ( 5.734105306875630248, 1409.113299756970036, 188.1906873671159985 ) ) ;
#50928=FACE_OUTER_BOUND ( 'NONE', #78281, .T. ) ;
#50934=CARTESIAN_POINT ( 'NONE',  ( 16.90814665888983015, 1423.564526555951034, 229.0298210386986852 ) ) ;
#50935=ORIENTED_EDGE ( 'NONE', *, *, #46138, .T. ) ;
#50937=VECTOR ( 'NONE', #36224, 1000.000000000000227 ) ;
#50938=CARTESIAN_POINT ( 'NONE',  ( 11.35815110745130063, 1432.342270311610037, 151.4015260409140069 ) ) ;
#50939=B_SPLINE_CURVE_WITH_KNOTS ( 'NONE', 3,
 ( #92190, #48557, #81036, #82693, #65363, #108444, #66472, #38476, #57514, #49106, #83240, #40685, #74858, #30069, #64260, #81570, #47992, #100580, #30635, #23862, #64822, #13806, #82130, #94377, #16549, #17657, #7085, #35037, #50739, #84874, #93286, #101121, #67013, #50212, #41241, #75413, #101667, #32824, #24418, #9294, #75942, #103325, #110095, #34492, #8722, #68126, #51289, #85423, #8170, #42339, #368, #109552 ),
 .UNSPECIFIED., .F., .F.,
 ( 4, 2, 2, 1, 1, 1, 2, 2, 2, 2, 1, 2, 2, 2, 2, 2, 2, 2, 2, 2, 1, 2, 2, 2, 2, 1, 2, 2, 4 ),
 ( 0.000000000000000000, 0.06249999999999765465, 0.09375000000000460743, 0.1093750000000183881, 0.1171874999999746036, 0.1210937499998826355, 0.1230468749998226835, 0.1249999999997627453, 0.1874999999982030763, 0.2187499999974809872, 0.2343749999971287690, 0.2421874999970357045, 0.2499999999969426123, 0.3124999999965559216, 0.3437499999963705699, 0.3749999999961852182, 0.4999999999961076136, 0.5624999999960688113, 0.6249999999960300645, 0.6874999999959913177, 0.7187499999960752506, 0.7343749999961173280, 0.7499999999961594055, 0.8124999999965581976, 0.8437499999968343101, 0.8593749999969143571, 0.8671874999970149434, 0.8749999999971155296, 1.000000000000000000 ),
 .UNSPECIFIED. ) ;
#50948=CARTESIAN_POINT ( 'NONE',  ( 11.87901658470000044, 1433.117702068830113, 149.9761015577979890 ) ) ;
#50949=CARTESIAN_POINT ( 'NONE',  ( 3.330669073880000148E-16, 1453.913060387330006, 209.1218459616979999 ) ) ;
#50950=B_SPLINE_SURFACE_WITH_KNOTS ( 'NONE', 5, 5, ( 
 ( #110281, #77255, #94029, #24596, #34679, #68867, #76684, #15103, #23516 ),
 ( #67203, #67752, #49294, #50404, #49425, #57708, #6718, #49846, #40874 ),
 ( #59360, #101862, #25707, #101302, #17293, #58789, #7818, #41988, #75051 ),
 ( #25156, #92928, #93468, #100760, #51488, #76137, #24051, #58245, #68317 ),
 ( #92367, #83976, #85071, #102425, #7276, #85619, #41441, #75606, #109736 ),
 ( #88399, #2767, #27942, #2220, #105206, #35792, #28494, #69976, #87300 ),
 ( #45865, #52052, #36334, #9479, #86187, #18407, #45318, #96250, #17850 ),
 ( #79457, #96810, #3322, #43643, #19524, #36887, #79998, #62123, #26835 ),
 ( #18964, #61563, #37447, #53730, #26268, #1656, #95147, #102970, #69421 ),
 ( #104645, #60458, #10033, #11158, #103534, #44203, #10593, #53159, #104092 ),
 ( #87868, #70528, #27384, #35233, #71081, #61023, #95697, #94575, #62686 ),
 ( #86741, #77796, #52605, #1105, #44763, #78915, #78347, #20080, #54274 ) ),
 .UNSPECIFIED., .F., .F., .F.,
 ( 6, 3, 3, 6 ),
 ( 6, 3, 6 ),
 ( 0.000000000000000000, 17.84603210599999912, 40.51038747020000130, 67.03953034199999195 ),
 ( 84.36360870500000431, 126.5454130579999941, 168.7272174100000086 ),
 .UNSPECIFIED. ) ;
#50954=CARTESIAN_POINT ( 'NONE',  ( -15.06279948716559680, 1422.388304403035136, 229.4662111949969301 ) ) ;
#50956=CARTESIAN_POINT ( 'NONE',  ( -14.16989796120989986, 1420.440730658529901, 227.4201728071160176 ) ) ;
#50957=CARTESIAN_POINT ( 'NONE',  ( -29.87022976070419844, 1509.969119424489918, 208.7889112562570233 ) ) ;
#50958=CARTESIAN_POINT ( 'NONE',  ( 24.30946323610000093, 1430.356462477430114, 212.0522589108380203 ) ) ;
#50960=CARTESIAN_POINT ( 'NONE',  ( -8.991592997889998884, 1509.227053733729917, 237.0094774837980083 ) ) ;
#50966=CARTESIAN_POINT ( 'NONE',  ( 0.1784803411008450136, 1475.371066012589836, 182.2932093119499939 ) ) ;
#50967=CARTESIAN_POINT ( 'NONE',  ( -5.680073728562159197, 1408.055878260910049, 221.5454655010989882 ) ) ;
#50968=EDGE_LOOP ( 'NONE', ( #39569, #95234, #14660, #101662, #11399, #14999 ) ) ;
#50969=CARTESIAN_POINT ( 'NONE',  ( -20.82705473220000059, 1444.994950788469851, 176.6587301488980017 ) ) ;
#50970=CARTESIAN_POINT ( 'NONE',  ( -38.13546499650039578, 1444.994950788468714, 136.8609531837178963 ) ) ;
#50971=CARTESIAN_POINT ( 'NONE',  ( 11.87502393270000134, 1433.007271228389982, 149.9804723947979994 ) ) ;
#50972=CARTESIAN_POINT ( 'NONE',  ( -39.48448845344529445, 1449.205409213619987, 134.0999999980729740 ) ) ;
#50975=CARTESIAN_POINT ( 'NONE',  ( -13.15726448929999925, 1416.913060387330006, 219.9105610086979823 ) ) ;
#50978=CARTESIAN_POINT ( 'NONE',  ( -15.65413333740000112, 1416.520322351130062, 219.1909222911980066 ) ) ;
#50980=B_SPLINE_CURVE_WITH_KNOTS ( 'NONE', 3,
 ( #76787, #68966, #103641, #85176, #86284, #44302, #70623, #44866, #85726, #79017, #70079, #95241, #69521, #61665, #103068, #95789, #26369, #43741, #52151 ),
 .UNSPECIFIED., .F., .F.,
 ( 4, 2, 2, 2, 1, 1, 1, 2, 2, 2, 4 ),
 ( 0.000000000000000000, 0.2500000000076687545, 0.3750000000115031318, 0.4375000000133325018, 0.4687500000142481582, 0.4843750000146268553, 0.4921875000148150936, 0.4960937500148319690, 0.5000000000148488999, 0.7500000000074245055, 1.000000000000000000 ),
 .UNSPECIFIED. ) ;
#50984=LINE ( 'NONE', #103576, #16366 ) ;
#50990=CARTESIAN_POINT ( 'NONE',  ( -32.05911371000000543, 1451.793557196030179, 134.7701858639979946 ) ) ;
#50991=CARTESIAN_POINT ( 'NONE',  ( -15.70046566381129871, 1410.429479579480130, 226.6601106372359880 ) ) ;
#50993=ORIENTED_EDGE ( 'NONE', *, *, #17536, .F. ) ;
#50995=CARTESIAN_POINT ( 'NONE',  ( 27.04494143110000337, 1509.634156398229834, 216.9800077211579890 ) ) ;
#50998=CARTESIAN_POINT ( 'NONE',  ( -5.389719915088219793, 1440.971386074470047, 154.8246291213590098 ) ) ;
#51000=CARTESIAN_POINT ( 'NONE',  ( 14.92518454057932331, 1430.567503116120179, 220.1855779226771404 ) ) ;
#51007=CARTESIAN_POINT ( 'NONE',  ( 3.133278283570000156, 1446.922686756950043, 159.4826872549980123 ) ) ;
#51012=DIRECTION ( 'NONE',  ( 0.000000000000000000, 0.000000000000000000, 1.000000000000000000 ) ) ;
#51015=CARTESIAN_POINT ( 'NONE',  ( -19.39159332910000089, 1430.347784943829993, 195.6539361813979951 ) ) ;
#51016=CARTESIAN_POINT ( 'NONE',  ( -11.19642886898100009, 1425.622699824140227, 127.8389159192909972 ) ) ;
#51018=CARTESIAN_POINT ( 'NONE',  ( 16.57071976326540153, 1410.582081926380170, 191.7433702585070137 ) ) ;
#51020=CARTESIAN_POINT ( 'NONE',  ( 27.92935577517391721, 1510.000134406965572, 220.0760090323809379 ) ) ;
#51021=CARTESIAN_POINT ( 'NONE',  ( 2.030980132853136944, 1450.182268141366194, 181.9754583269210855 ) ) ;
#51022=CARTESIAN_POINT ( 'NONE',  ( 19.25251418436180018, 1509.610172285510089, 231.6560777679470107 ) ) ;
#51023=CARTESIAN_POINT ( 'NONE',  ( 8.013639455417655100, 1465.494642556247300, 233.0458548789991937 ) ) ;
#51026=CARTESIAN_POINT ( 'NONE',  ( -36.55889210262929367, 1437.673941850749770, 136.5464336263889891 ) ) ;
#51028=CARTESIAN_POINT ( 'NONE',  ( 6.881122077359999700, 1396.213462846930042, 198.7274638095979924 ) ) ;
#51031=CARTESIAN_POINT ( 'NONE',  ( -16.13006593319999737, 1459.079424064530031, 230.3616556409980092 ) ) ;
#51033=VERTEX_POINT ( 'NONE', #61713 ) ;
#51035=CARTESIAN_POINT ( 'NONE',  ( 14.79248454883459907, 1496.752653259379940, 226.0610261129200182 ) ) ;
#51038=B_SPLINE_CURVE_WITH_KNOTS ( 'NONE', 5,
 ( #89892, #96657, #79859, #97744, #89348, #71495, #11546, #46278, #28898 ),
 .UNSPECIFIED., .F., .F.,
 ( 6, 3, 6 ),
 ( 0.000000000000000000, 0.4258971877630836622, 1.000000000000000000 ),
 .UNSPECIFIED. ) ;
#51043=CARTESIAN_POINT ( 'NONE',  ( -15.88507158550000042, 1470.477701853530107, 228.8906323047980038 ) ) ;
#51049=( BOUNDED_CURVE ( )  B_SPLINE_CURVE ( 3, ( #20648, #70561, #104678, #54850 ),
 .UNSPECIFIED., .F., .T. ) 
 B_SPLINE_CURVE_WITH_KNOTS ( ( 4, 4 ),
 ( 6.150868878552831376, 6.164145497763507286 ),
 .UNSPECIFIED. ) 
 CURVE ( )  GEOMETRIC_REPRESENTATION_ITEM ( )  RATIONAL_B_SPLINE_CURVE ( ( 1.000000000000000000, 0.9999853110024699010, 0.9999853110024699010, 1.000000000000000000 ) ) 
 REPRESENTATION_ITEM ( '' )  );
#51052=VERTEX_POINT ( 'NONE', #51636 ) ;
#51053=CARTESIAN_POINT ( 'NONE',  ( 11.73709356406289928, 1426.695943121369965, 144.1748013758129900 ) ) ;
#51055=CARTESIAN_POINT ( 'NONE',  ( 19.13278187119999885, 1487.527101359029984, 228.6867874049980003 ) ) ;
#51057=CARTESIAN_POINT ( 'NONE',  ( -13.58235846979999906, 1416.828040475229955, 221.9087530951979659 ) ) ;
#51062=CARTESIAN_POINT ( 'NONE',  ( -4.747361959010000021, 1423.750432747230207, 185.1131762002980281 ) ) ;
#51063=CARTESIAN_POINT ( 'NONE',  ( -7.842556662604346585, 1446.693600393765337, 154.0804530413156215 ) ) ;
#51064=CARTESIAN_POINT ( 'NONE',  ( -0.1613635196969999963, 1507.107001830130002, 180.9028739243980226 ) ) ;
#51065=CARTESIAN_POINT ( 'NONE',  ( 6.291724964230139605, 1441.035272546479973, 154.5485623116409784 ) ) ;
#51070=CARTESIAN_POINT ( 'NONE',  ( -5.027042350745985821, 1422.871757580189978, 184.8364420396860339 ) ) ;
#51073=EDGE_CURVE ( 'NONE', #68277, #68290, #16225, .T. ) ;
#51075=ORIENTED_EDGE ( 'NONE', *, *, #83599, .T. ) ;
#51078=CARTESIAN_POINT ( 'NONE',  ( -2.899134383046004348, 1484.388260718141055, 183.3068692522237200 ) ) ;
#51082=ORIENTED_EDGE ( 'NONE', *, *, #28345, .F. ) ;
#51083=CARTESIAN_POINT ( 'NONE',  ( 1.546867496849999801, 1416.839692139930094, 190.2222514364979986 ) ) ;
#51085=CARTESIAN_POINT ( 'NONE',  ( -11.19300148449999988, 1425.653304015530011, 147.1770035940979824 ) ) ;
#51086=CARTESIAN_POINT ( 'NONE',  ( 4.026786250540000722, 1415.442497638829991, 163.1427597075980032 ) ) ;
#51087=B_SPLINE_CURVE_WITH_KNOTS ( 'NONE', 5,
 ( #91908, #90808, #98658, #82962, #15185, #24134 ),
 .UNSPECIFIED., .F., .F.,
 ( 6, 6 ),
 ( 0.000000000000000000, 1.000000000000000000 ),
 .UNSPECIFIED. ) ;
#51088=CARTESIAN_POINT ( 'NONE',  ( -7.352292206439999589, 1441.815725582649975, 185.3605977109980074 ) ) ;
#51091=FACE_OUTER_BOUND ( 'NONE', #29666, .T. ) ;
#51092=CARTESIAN_POINT ( 'NONE',  ( -21.82073367870000169, 1482.726029602730023, 224.2880922674980013 ) ) ;
#51097=CARTESIAN_POINT ( 'NONE',  ( 23.62346383279999884, 1410.898849078630064, 268.8227235180979733 ) ) ;
#51099=CARTESIAN_POINT ( 'NONE',  ( 20.08216459950000043, 1449.729590668439869, 193.7700040052980057 ) ) ;
#51100=CARTESIAN_POINT ( 'NONE',  ( 10.70848634212536865, 1506.855035729306792, 228.7236287190453936 ) ) ;
#51101=AXIS2_PLACEMENT_3D ( 'NONE', #5282, #58455, #100979 ) ;
#51103=CARTESIAN_POINT ( 'NONE',  ( -41.53485087296149914, 1442.119024217849983, 135.5124738229289960 ) ) ;
#51104=CARTESIAN_POINT ( 'NONE',  ( 12.63038619288439968, 1428.207532477410041, 223.9332333053530135 ) ) ;
#51106=CARTESIAN_POINT ( 'NONE',  ( -14.16826824910000049, 1443.187051346489852, 188.6845770635979704 ) ) ;
#51112=CARTESIAN_POINT ( 'NONE',  ( 1.451959685182149906, 1503.840107181440089, 181.2560994760340236 ) ) ;
#51113=CARTESIAN_POINT ( 'NONE',  ( -13.81911144855440021, 1409.395634392820057, 214.7971903334679951 ) ) ;
#51116=CARTESIAN_POINT ( 'NONE',  ( -12.73087921850000015, 1474.751530140129944, 268.4159631503979995 ) ) ;
#51121=CYLINDRICAL_SURFACE ( 'NONE', #69698, 1.999999999999913181 ) ;
#51122=CARTESIAN_POINT ( 'NONE',  ( 12.11709951209460101, 1416.029511585410091, 223.4307279390160090 ) ) ;
#51123=FACE_OUTER_BOUND ( 'NONE', #50898, .T. ) ;
#51126=CARTESIAN_POINT ( 'NONE',  ( -23.56691185029999858, 1411.096426580230172, 206.5756125875680027 ) ) ;
#51130=CARTESIAN_POINT ( 'NONE',  ( -4.367411321880000158E-15, 1433.447543843880112, 150.4377610267980003 ) ) ;
#51137=CARTESIAN_POINT ( 'NONE',  ( 11.73572286974009948, 1426.696804897310130, 144.0764963122049949 ) ) ;
#51141=CARTESIAN_POINT ( 'NONE',  ( 3.007752987394139908E-09, 1406.911841295280055, 222.1218459617980159 ) ) ;
#51143=CARTESIAN_POINT ( 'NONE',  ( -8.235420378752696280, 1398.157615904283375, 219.1813604885521727 ) ) ;
#51149=ORIENTED_EDGE ( 'NONE', *, *, #87176, .F. ) ;
#51150=CARTESIAN_POINT ( 'NONE',  ( 12.01841008247880005, 1433.726417607980011, 149.8316427203229750 ) ) ;
#51158=CARTESIAN_POINT ( 'NONE',  ( 17.62013664171889715, 1498.112312558009990, 230.2633706911829847 ) ) ;
#51159=CARTESIAN_POINT ( 'NONE',  ( 0.3783643747870000240, 1468.710133949630062, 182.5713305459979949 ) ) ;
#51161=CARTESIAN_POINT ( 'NONE',  ( 15.14118775829999919, 1409.441802315629957, 226.2727750917980245 ) ) ;
#51162=CARTESIAN_POINT ( 'NONE',  ( 0.1334653011508349918, 1395.917721098340053, 198.1212205003539850 ) ) ;
#51163=CARTESIAN_POINT ( 'NONE',  ( 14.06293010156799994, 1415.542389211330146, 197.2558749039930035 ) ) ;
#51164=CARTESIAN_POINT ( 'NONE',  ( 10.96395513279999889, 1431.947606384360142, 151.7599316184980296 ) ) ;
#51166=ORIENTED_EDGE ( 'NONE', *, *, #48707, .T. ) ;
#51167=CARTESIAN_POINT ( 'NONE',  ( 14.13823592991809974, 1436.109943510260109, 150.1180615443350064 ) ) ;
#51169=ORIENTED_EDGE ( 'NONE', *, *, #95112, .F. ) ;
#51170=CARTESIAN_POINT ( 'NONE',  ( 13.51610093808350221, 1443.927065517340907, 169.3501091255430424 ) ) ;
#51171=CARTESIAN_POINT ( 'NONE',  ( -12.81329301000000065, 1461.300013870830071, 232.2698450468980127 ) ) ;
#51175=CARTESIAN_POINT ( 'NONE',  ( -19.08186866826044437, 1442.067311600292442, 210.3913232654338969 ) ) ;
#51179=EDGE_CURVE ( 'NONE', #27764, #45161, #22589, .T. ) ;
#51183=CARTESIAN_POINT ( 'NONE',  ( -19.06709057720000189, 1507.978133441429918, 229.6728830551980138 ) ) ;
#51185=CARTESIAN_POINT ( 'NONE',  ( -7.275747108760000081, 1410.543472109730146, 187.4914510093980198 ) ) ;
#51187=CARTESIAN_POINT ( 'NONE',  ( -0.4068402809140000409, 1415.948532225030021, 227.3221874807980214 ) ) ;
#51188=VERTEX_POINT ( 'NONE', #17438 ) ;
#51189=CARTESIAN_POINT ( 'NONE',  ( 24.21908197320000156, 1436.980893512170269, 213.8801751562779998 ) ) ;
#51197=CARTESIAN_POINT ( 'NONE',  ( 22.99941590693347138, 1409.742488441884007, 209.3674371477623595 ) ) ;
#51206=CARTESIAN_POINT ( 'NONE',  ( -8.446261695729999662E-10, 1468.737548875729999, 250.5651368549980305 ) ) ;
#51209=CARTESIAN_POINT ( 'NONE',  ( -2.864170848000150205, 1509.034024718710043, 238.6060105441289920 ) ) ;
#51211=CARTESIAN_POINT ( 'NONE',  ( 1.174449684515169956, 1452.839884179820046, 183.4104027199379914 ) ) ;
#51212=DIRECTION ( 'NONE',  ( 0.04361938736533144123, 0.9990482215818579093, 0.000000000000000000 ) ) ;
#51214=FACE_OUTER_BOUND ( 'NONE', #104204, .T. ) ;
#51220=CARTESIAN_POINT ( 'NONE',  ( 24.58439919890000169, 1442.301074160069902, 213.1549993496080333 ) ) ;
#51221=DIRECTION ( 'NONE',  ( 0.000000000000000000, -1.000000000000000000, 0.000000000000000000 ) ) ;
#51224=CARTESIAN_POINT ( 'NONE',  ( 28.39358856799220021, 1435.964832128500120, 136.4714687674249944 ) ) ;
#51225=CARTESIAN_POINT ( 'NONE',  ( 40.21456421019439631, 1444.725599080220036, 137.0098365210060081 ) ) ;
#51226=CARTESIAN_POINT ( 'NONE',  ( -2.907264515414449857, 1451.960119877520128, 184.7556101994359778 ) ) ;
#51228=CARTESIAN_POINT ( 'NONE',  ( 13.73944485519999859, 1508.116386186929958, 185.6413942156979999 ) ) ;
#51231=CARTESIAN_POINT ( 'NONE',  ( -40.82827697499264730, 1448.469058903514906, 269.6248674872855418 ) ) ;
#51233=CARTESIAN_POINT ( 'NONE',  ( 1.633469776390000128, 1432.353341358199941, 150.3624711946980028 ) ) ;
#51234=CARTESIAN_POINT ( 'NONE',  ( 12.40452786870000068, 1434.419866698830219, 146.5969156002979901 ) ) ;
#51236=DIRECTION ( 'NONE',  ( 0.9956776678953921378, -0.09285416003634892890, 0.002021538606455937359 ) ) ;
#51237=CARTESIAN_POINT ( 'NONE',  ( 11.39112423001730789, 1425.664172111152993, 138.8630547727001670 ) ) ;
#51239=CARTESIAN_POINT ( 'NONE',  ( -17.11714618750000128, 1444.740067931809790, 162.7561046190980107 ) ) ;
#51240=CARTESIAN_POINT ( 'NONE',  ( 24.63043001767085727, 1451.910743108596080, 137.3284549923116629 ) ) ;
#51244=CARTESIAN_POINT ( 'NONE',  ( -12.30704544771305997, 1419.221384995674498, 228.6548432408881126 ) ) ;
#51245=CARTESIAN_POINT ( 'NONE',  ( -5.352781315208301471, 1451.479376706958192, 153.6005146435509516 ) ) ;
#51246=CARTESIAN_POINT ( 'NONE',  ( -17.50151672410429882, 1415.426561690370136, 209.2157686050819905 ) ) ;
#51247=CARTESIAN_POINT ( 'NONE',  ( 25.04098008639999762, 1435.655091878980102, 136.8337871717980079 ) ) ;
#51248=CARTESIAN_POINT ( 'NONE',  ( -10.07831585545570086, 1396.265002934200083, 204.5499906845170131 ) ) ;
#51249=EDGE_LOOP ( 'NONE', ( #75627, #85552, #89157, #87609 ) ) ;
#51250=CARTESIAN_POINT ( 'NONE',  ( 0.2241001114877609890, 1414.913060387399810, 193.0224632409980074 ) ) ;
#51251=CARTESIAN_POINT ( 'NONE',  ( -5.505226529499999799, 1409.105307133929955, 230.1454130303979753 ) ) ;
#51252=ORIENTED_EDGE ( 'NONE', *, *, #80295, .T. ) ;
#51256=CARTESIAN_POINT ( 'NONE',  ( 11.01695271670000054, 1426.937849641930143, 91.93091727569790805 ) ) ;
#51258=CARTESIAN_POINT ( 'NONE',  ( 24.06753648839999826, 1410.675710978030111, 209.6250578378659668 ) ) ;
#51259=CARTESIAN_POINT ( 'NONE',  ( -0.1652168328899510097, 1507.119555385590047, 237.3426446390569993 ) ) ;
#51261=CARTESIAN_POINT ( 'NONE',  ( -2.497969711800415382, 1421.148623978353953, 184.9753524319759492 ) ) ;
#51264=CARTESIAN_POINT ( 'NONE',  ( -24.08426305480000451, 1411.115211393229856, 208.6111285346999864 ) ) ;
#51267=CARTESIAN_POINT ( 'NONE',  ( -23.59273067950500291, 1509.852083508271107, 190.5178204038475656 ) ) ;
#51271=ORIENTED_EDGE ( 'NONE', *, *, #79881, .T. ) ;
#51272=CARTESIAN_POINT ( 'NONE',  ( -11.85531524228330014, 1431.584718363120146, 149.9327016396569832 ) ) ;
#51274=CARTESIAN_POINT ( 'NONE',  ( -2.339369569539999638, 1474.134115800729887, 270.1366117264980176 ) ) ;
#51275=CARTESIAN_POINT ( 'NONE',  ( 13.31848378016444734, 1434.903344954230306, 146.7688399487844606 ) ) ;
#51277=CARTESIAN_POINT ( 'NONE',  ( 19.76034656259999878, 1519.913060387329779, 196.6657374964980249 ) ) ;
#51279=CARTESIAN_POINT ( 'NONE',  ( 38.64678288495740333, 1443.959461509469975, 137.1848747843469880 ) ) ;
#51282=CARTESIAN_POINT ( 'NONE',  ( -15.53177320253059968, 1407.736001233250136, 267.4358752646630251 ) ) ;
#51283=CARTESIAN_POINT ( 'NONE',  ( -14.50855428415770021, 1436.251820910509878, 149.9260813992850103 ) ) ;
#51286=CARTESIAN_POINT ( 'NONE',  ( 13.64985700350000108, 1444.557014110619775, 188.8602261534980187 ) ) ;
#51289=CARTESIAN_POINT ( 'NONE',  ( 4.664360135691749676, 1422.142640414709604, 184.1192042709404291 ) ) ;
#51292=CARTESIAN_POINT ( 'NONE',  ( -18.13447789030000123, 1470.472875412729991, 189.7357867468980146 ) ) ;
#51293=DIRECTION ( 'NONE',  ( 0.3363363969979658030, 0.9417419115949056119, 0.000000000000000000 ) ) ;
#51294=ORIENTED_EDGE ( 'NONE', *, *, #27771, .F. ) ;
#51297=CARTESIAN_POINT ( 'NONE',  ( -28.19408351100000232, 1508.123162623830012, 208.4952225986349958 ) ) ;
#51298=CARTESIAN_POINT ( 'NONE',  ( 3.947090874974254149, 1427.113278099589934, 134.0999999980980704 ) ) ;
#51300=CARTESIAN_POINT ( 'NONE',  ( -1.284214933530000158, 1407.590765156830003, 196.0582559783980230 ) ) ;
#51301=CARTESIAN_POINT ( 'NONE',  ( -13.85929445400000048, 1410.325638502529955, 227.0940372023979990 ) ) ;
#51304=CARTESIAN_POINT ( 'NONE',  ( -26.50580188063009857, 1469.329502110289923, 209.9352390060020070 ) ) ;
#51305=CARTESIAN_POINT ( 'NONE',  ( 27.42581371220000008, 1488.692458006830066, 209.3595745165729909 ) ) ;
#51307=CARTESIAN_POINT ( 'NONE',  ( 19.07029180426959769, 1456.930551391809786, 225.1474799417119925 ) ) ;
#51308=CARTESIAN_POINT ( 'NONE',  ( -23.80235451360000098, 1435.328707481769925, 136.9030858810979794 ) ) ;
#51316=ORIENTED_EDGE ( 'NONE', *, *, #16619, .F. ) ;
#51317=CARTESIAN_POINT ( 'NONE',  ( -2.068751723726309777, 1451.946575739190166, 184.4429135660199961 ) ) ;
#51318=CARTESIAN_POINT ( 'NONE',  ( -0.5133635713019999436, 1410.311096974030079, 233.1717008067979862 ) ) ;
#51321=CARTESIAN_POINT ( 'NONE',  ( -13.02322703936409987, 1416.825784014559986, 196.6108461303639672 ) ) ;
#51323=CARTESIAN_POINT ( 'NONE',  ( 11.83454512112139945, 1434.825470695330068, 151.1770841828369782 ) ) ;
#51324=CARTESIAN_POINT ( 'NONE',  ( -4.138348461501534459, 1441.507286901806310, 184.0825983021243815 ) ) ;
#51325=B_SPLINE_CURVE_WITH_KNOTS ( 'NONE', 3,
 ( #65504, #22897, #57106, #15595, #49799, #1061, #25112, #17248, #51441, #94529 ),
 .UNSPECIFIED., .F., .F.,
 ( 4, 2, 2, 2, 4 ),
 ( 0.000000000000000000, 0.2500000000000000000, 0.5000000000000000000, 0.7500000000000000000, 1.000000000000000000 ),
 .UNSPECIFIED. ) ;
#51326=CARTESIAN_POINT ( 'NONE',  ( -22.04195665738010135, 1508.943562127990162, 226.5634866290460252 ) ) ;
#51328=DIRECTION ( 'NONE',  ( 1.006446316953035876E-09, 1.000000000000000000, -9.896731379374899561E-10 ) ) ;
#51330=DIRECTION ( 'NONE',  ( -0.000000000000000000, 1.000000000000000000, -0.000000000000000000 ) ) ;
#51331=EDGE_CURVE ( 'NONE', #10158, #25299, #105549, .T. ) ;
#51333=CARTESIAN_POINT ( 'NONE',  ( -2.466766482289999729, 1421.294048410029973, 184.8150638888980097 ) ) ;
#51334=CARTESIAN_POINT ( 'NONE',  ( 21.21436153039999795, 1509.702916644130028, 188.2361191047979787 ) ) ;
#51336=AXIS2_PLACEMENT_3D ( 'NONE', #109993, #42239, #110536 ) ;
#51337=ORIENTED_EDGE ( 'NONE', *, *, #61681, .T. ) ;
#51338=CARTESIAN_POINT ( 'NONE',  ( -12.58190538649999901, 1415.948532224930204, 195.9645815321979967 ) ) ;
#51349=CARTESIAN_POINT ( 'NONE',  ( 17.50215275067818865, 1422.936145674484123, 226.4538908241968045 ) ) ;
#51352=CARTESIAN_POINT ( 'NONE',  ( -11.91321771470000002, 1435.943783413959864, 147.6429393588979906 ) ) ;
#51353=CARTESIAN_POINT ( 'NONE',  ( 26.80104177516750141, 1446.506287311350206, 137.4021340779750062 ) ) ;
#51355=DIRECTION ( 'NONE',  ( 0.7059182309095664021, 0.02465121832729061380, -0.7078642304174497246 ) ) ;
#51356=CARTESIAN_POINT ( 'NONE',  ( 11.23256922559021653, 1433.984535818029144, 151.5862715624802490 ) ) ;
#51359=CARTESIAN_POINT ( 'NONE',  ( 18.82859584293606758, 1461.935129172100915, 190.8088398609367857 ) ) ;
#51364=CARTESIAN_POINT ( 'NONE',  ( 2.923521462801879967, 1410.394928839790055, 231.6309329194170061 ) ) ;
#51370=CARTESIAN_POINT ( 'NONE',  ( 22.73270563069999994, 1451.307588288230136, 142.3779184700979954 ) ) ;
#51371=B_SPLINE_CURVE_WITH_KNOTS ( 'NONE', 3,
 ( #72350, #81812, #23001, #46598, #72887, #108119, #31413, #57205, #48241, #82384, #80733, #99155, #107027, #64502, #38169, #48801, #56084, #82924, #106479, #6215, #90210, #98619, #47684, #5114, #39270 ),
 .UNSPECIFIED., .F., .F.,
 ( 4, 3, 3, 3, 3, 3, 3, 3, 4 ),
 ( -41.86545604797390041, -41.27964960583160092, -39.51168084002180336, -37.86278309458619873, -36.27358298899350331, -34.76523579414600107, -33.29895478326900360, -31.86861058327169971, -30.44048980260000548 ),
 .UNSPECIFIED. ) ;
#51372=PLANE ( 'NONE',  #53620 ) ;
#51373=CARTESIAN_POINT ( 'NONE',  ( 13.86092937120069912, 1410.765486813650114, 191.1266627561969926 ) ) ;
#51375=CARTESIAN_POINT ( 'NONE',  ( 23.57642905779999865, 1509.468438641930106, 193.4040834977980126 ) ) ;
#51376=ORIENTED_EDGE ( 'NONE', *, *, #24045, .F. ) ;
#51377=CARTESIAN_POINT ( 'NONE',  ( -18.15370184069965731, 1459.449025707702049, 227.9319138183309974 ) ) ;
#51379=EDGE_CURVE ( 'NONE', #55526, #34578, #31933, .T. ) ;
#51384=CARTESIAN_POINT ( 'NONE',  ( 19.85686604346530260, 1508.846387636299823, 229.4817185467019840 ) ) ;
#51386=CARTESIAN_POINT ( 'NONE',  ( 39.38156440427009386, 1440.303727024390128, 136.7574120630100083 ) ) ;
#51387=DIRECTION ( 'NONE',  ( -0.9965074780644831431, -0.004098122787124980695, 0.08340294689748870005 ) ) ;
#51392=CARTESIAN_POINT ( 'NONE',  ( -12.81719096786032352, 1435.925157283035560, 150.8223353154213839 ) ) ;
#51394=CARTESIAN_POINT ( 'NONE',  ( 3.277154590789999933, 1409.963920169630228, 185.8200990145979858 ) ) ;
#51395=CARTESIAN_POINT ( 'NONE',  ( 0.6879128371797639252, 1508.983932488360097, 179.4145436916340088 ) ) ;
#51396=CARTESIAN_POINT ( 'NONE',  ( 40.27278867766426629, 1443.694772336818687, 137.1246062732301141 ) ) ;
#51398=CARTESIAN_POINT ( 'NONE',  ( -4.284965797313190272, 1440.956314292269781, 155.9224932556410010 ) ) ;
#51400=CARTESIAN_POINT ( 'NONE',  ( -3.793561831505700255, 1450.899630787780097, 184.9307162316310098 ) ) ;
#51401=CARTESIAN_POINT ( 'NONE',  ( 1.119830458929999883, 1465.309628979130139, 236.0546564598980126 ) ) ;
#51404=CARTESIAN_POINT ( 'NONE',  ( -41.09355243439999583, 1449.585181137809968, 270.0512738362979803 ) ) ;
#51405=ADVANCED_FACE ( 'NONE', ( #26131 ), #977, .F. ) ;
#51408=CARTESIAN_POINT ( 'NONE',  ( 17.55838294249999976, 1488.199839363530145, 189.1289626450980279 ) ) ;
#51411=CARTESIAN_POINT ( 'NONE',  ( -1.547930050009999947, 1416.311719782429918, 227.9539241407980228 ) ) ;
#51412=CARTESIAN_POINT ( 'NONE',  ( -4.139355080849999702, 1416.968741244730154, 232.7076405003979858 ) ) ;
#51416=CARTESIAN_POINT ( 'NONE',  ( 0.08971693578977467387, 1486.409952364518176, 181.8122316423428799 ) ) ;
#51418=CARTESIAN_POINT ( 'NONE',  ( -46.14657524832199442, 1438.245561584440111, 267.5940402666269620 ) ) ;
#51419=CARTESIAN_POINT ( 'NONE',  ( 13.72406976976210125, 1509.120045271949948, 233.9463300173069911 ) ) ;
#51421=ADVANCED_FACE ( 'NONE', ( #1520 ), #93345, .F. ) ;
#51422=ORIENTED_EDGE ( 'NONE', *, *, #48851, .F. ) ;
#51424=CARTESIAN_POINT ( 'NONE',  ( -5.439681134809999818, 1437.306888242379955, 154.7134157797979981 ) ) ;
#51426=CARTESIAN_POINT ( 'NONE',  ( 19.26518044636202731, 1456.127854578388451, 225.0603431000050421 ) ) ;
#51428=CARTESIAN_POINT ( 'NONE',  ( -25.94056929255189914, 1451.122515486970087, 136.6312467053010096 ) ) ;
#51430=CARTESIAN_POINT ( 'NONE',  ( 4.385438019169999535, 1418.241830526729927, 231.9989422736980202 ) ) ;
#51433=CARTESIAN_POINT ( 'NONE',  ( 11.60004869885203682, 1423.633685391621384, 135.8154921816039007 ) ) ;
#51434=CARTESIAN_POINT ( 'NONE',  ( -23.51884061320912878, 1448.078341978384287, 217.4024159428893199 ) ) ;
#51437=CARTESIAN_POINT ( 'NONE',  ( -18.90690578109999720, 1416.819760216030090, 208.2173865545289857 ) ) ;
#51439=CARTESIAN_POINT ( 'NONE',  ( -8.718177347727909421, 1408.261084764490079, 270.1210383458869728 ) ) ;
#51440=CARTESIAN_POINT ( 'NONE',  ( 4.075906014412360001, 1417.644700588070236, 232.4454855814549887 ) ) ;
#51441=CARTESIAN_POINT ( 'NONE',  ( -2.500000810785663052, 1448.904868584106680, 183.3442529213150181 ) ) ;
#51442=CARTESIAN_POINT ( 'NONE',  ( -2.500000000000000000, 1439.615921247279857, 167.6891699144290158 ) ) ;
#51444=ORIENTED_EDGE ( 'NONE', *, *, #64539, .T. ) ;
#51445=CARTESIAN_POINT ( 'NONE',  ( -23.63499367410939911, 1410.853431111550208, 210.3632786977680098 ) ) ;
#51446=CARTESIAN_POINT ( 'NONE',  ( 0.03284348760489309849, 1410.296499662470069, 185.0199513014300123 ) ) ;
#51447=DIRECTION ( 'NONE',  ( -0.7628756745748126455, -0.04363816677874606670, -0.6450708608689551538 ) ) ;
#51448=CARTESIAN_POINT ( 'NONE',  ( -9.253402716490001012, 1428.330636036430178, 123.0297916884979941 ) ) ;
#51449=CARTESIAN_POINT ( 'NONE',  ( -20.15668535170019737, 1479.813499036020175, 193.0638610647490054 ) ) ;
#51450=CARTESIAN_POINT ( 'NONE',  ( -22.46702269440000421, 1420.825031629329715, 215.0041689658179962 ) ) ;
#51452=CARTESIAN_POINT ( 'NONE',  ( 28.47708477731459809, 1468.479349472730064, 266.9011526386389619 ) ) ;
#51453=CARTESIAN_POINT ( 'NONE',  ( -2.941982104803258835, 1466.821624837357149, 235.0423269388574852 ) ) ;
#51457=CARTESIAN_POINT ( 'NONE',  ( 18.92306020057025862, 1457.652989641058639, 226.8765308104140956 ) ) ;
#51459=CARTESIAN_POINT ( 'NONE',  ( 4.500000000000000000, 1448.210448412289907, 182.3842140122979743 ) ) ;
#51461=CARTESIAN_POINT ( 'NONE',  ( -3.304926829299330709E-16, 1420.443991414029824, 172.2701767054979882 ) ) ;
#51462=CARTESIAN_POINT ( 'NONE',  ( 26.72825992618109936, 1451.963087292549972, 135.1721373074829842 ) ) ;
#51466=CARTESIAN_POINT ( 'NONE',  ( 17.02706952559999820, 1409.507658761130187, 193.7554158992979865 ) ) ;
#51467=CARTESIAN_POINT ( 'NONE',  ( 13.35741048202589809, 1443.913060387329324, 164.9741927960640453 ) ) ;
#51468=CARTESIAN_POINT ( 'NONE',  ( 0.3812827203925389652, 1408.926375073290046, 186.5173452701070005 ) ) ;
#51469=CARTESIAN_POINT ( 'NONE',  ( 1.220192692170000148, 1416.035373678829956, 233.0189416646979907 ) ) ;
#51470=DIRECTION ( 'NONE',  ( 0.000000000000000000, -0.7071067811865474617, -0.7071067811865474617 ) ) ;
#51471=CIRCLE ( 'NONE', #13878, 26.99999999999999645 ) ;
#51472=CARTESIAN_POINT ( 'NONE',  ( 11.95779796459999922, 1409.330635893630188, 227.4564908493979942 ) ) ;
#51473=EDGE_CURVE ( 'NONE', #77609, #43125, #97388, .T. ) ;
#51477=CARTESIAN_POINT ( 'NONE',  ( 5.007662633622221193, 1418.086932660744651, 233.9718093764707305 ) ) ;
#51478=ORIENTED_EDGE ( 'NONE', *, *, #96141, .T. ) ;
#51479=CARTESIAN_POINT ( 'NONE',  ( 12.70695307632060000, 1416.230844595159851, 222.1275921544260257 ) ) ;
#51480=CARTESIAN_POINT ( 'NONE',  ( 11.86176262958469962, 1432.335962564359988, 150.1420606180239758 ) ) ;
#51481=VECTOR ( 'NONE', #85852, 1000.000000000000000 ) ;
#51488=CARTESIAN_POINT ( 'NONE',  ( -26.42894385079999964, 1460.505561531929970, 262.6648722463980334 ) ) ;
#51491=CARTESIAN_POINT ( 'NONE',  ( 11.18950481729999957, 1433.539833593499907, 151.6108599932980212 ) ) ;
#51492=CARTESIAN_POINT ( 'NONE',  ( 26.42714721250000309, 1443.942861156509935, 243.9198229606980135 ) ) ;
#51497=CARTESIAN_POINT ( 'NONE',  ( -13.63663271600000115, 1486.121807553629878, 185.3134443986979818 ) ) ;
#51498=CARTESIAN_POINT ( 'NONE',  ( 11.90436745871180690, 1398.266016359466903, 214.3454593262396202 ) ) ;
#51499=CARTESIAN_POINT ( 'NONE',  ( -25.72757591410449862, 1509.824537483000086, 193.1381027855750006 ) ) ;
#51500=AXIS2_PLACEMENT_3D ( 'NONE', #60480, #69441, #36909 ) ;
#51501=CARTESIAN_POINT ( 'NONE',  ( 22.35979953500000050, 1410.906900721630109, 215.2033244915180035 ) ) ;
#51503=CARTESIAN_POINT ( 'NONE',  ( 26.08009213506066715, 1436.684477317271103, 136.9230107608492233 ) ) ;
#51506=ADVANCED_FACE ( 'NONE', ( #11015 ), #46369, .F. ) ;
#51510=CARTESIAN_POINT ( 'NONE',  ( 0.1727113076434980132, 1478.739035586289901, 182.1485550913949965 ) ) ;
#51513=ORIENTED_EDGE ( 'NONE', *, *, #89125, .T. ) ;
#51514=CARTESIAN_POINT ( 'NONE',  ( -13.51610093809999924, 1443.913060387330006, 169.3501091259980171 ) ) ;
#51515=CARTESIAN_POINT ( 'NONE',  ( -38.71377205869448801, 1444.324653571827866, 136.9322096537518973 ) ) ;
#51522=CARTESIAN_POINT ( 'NONE',  ( -17.16585533279999964, 1415.931391677329884, 214.4037704070680093 ) ) ;
#51536=CARTESIAN_POINT ( 'NONE',  ( 17.22623662315568893, 1443.501467202830781, 162.9225832754749490 ) ) ;
#51544=CARTESIAN_POINT ( 'NONE',  ( 38.90834013964843052, 1452.449200603389727, 269.5913925115327743 ) ) ;
#51546=CARTESIAN_POINT ( 'NONE',  ( 16.18610113297054198, 1432.064054184273346, 218.4257206746670192 ) ) ;
#51547=CARTESIAN_POINT ( 'NONE',  ( 2.961376673209999755, 1417.751980673930120, 234.4067280231980135 ) ) ;
#51552=EDGE_CURVE ( 'NONE', #18384, #62647, #44, .T. ) ;
#51557=EDGE_CURVE ( 'NONE', #34085, #60010, #73408, .T. ) ;
#51563=B_SPLINE_CURVE_WITH_KNOTS ( 'NONE', 5,
 ( #72819, #21262, #20186, #3424, #54384, #63878, #30794, #3976, #4511, #63339, #73365, #106410 ),
 .UNSPECIFIED., .F., .F.,
 ( 6, 3, 3, 6 ),
 ( 39.80009975441029724, 56.26732510819999789, 56.97897492249999374, 58.84485018950000068 ),
 .UNSPECIFIED. ) ;
#51564=CARTESIAN_POINT ( 'NONE',  ( 15.68557540059999766, 1410.853897593529837, 191.5168599455980143 ) ) ;
#51565=ORIENTED_EDGE ( 'NONE', *, *, #90567, .F. ) ;
#51568=CARTESIAN_POINT ( 'NONE',  ( -24.57539793409999973, 1430.358747824730244, 207.2090478296979938 ) ) ;
#51569=CARTESIAN_POINT ( 'NONE',  ( -11.24026918932699992, 1425.602988694570058, 130.8057374633750101 ) ) ;
#51570=CARTESIAN_POINT ( 'NONE',  ( 16.57550902493450096, 1410.866907009090028, 191.7134341172800021 ) ) ;
#51572=CARTESIAN_POINT ( 'NONE',  ( 19.80907117253899585, 1509.722913433488202, 186.5213986624754909 ) ) ;
#51574=CARTESIAN_POINT ( 'NONE',  ( 1.630002283467431701, 1450.546079252429763, 181.7385653295009149 ) ) ;
#51575=CARTESIAN_POINT ( 'NONE',  ( -45.67177475829999622, 1440.913060392909983, 266.1885948849979968 ) ) ;
#51576=CARTESIAN_POINT ( 'NONE',  ( 17.88484985822620033, 1509.549773635790189, 232.6392117127710151 ) ) ;
#51577=CARTESIAN_POINT ( 'NONE',  ( 17.35588498053416018, 1460.101161736126869, 228.4988312450949195 ) ) ;
#51580=CARTESIAN_POINT ( 'NONE',  ( -37.50393792736510079, 1438.236878684590010, 136.5796126580320049 ) ) ;
#51582=CARTESIAN_POINT ( 'NONE',  ( 10.77364935086789899, 1398.232638417850012, 200.3335059216469745 ) ) ;
#51584=CARTESIAN_POINT ( 'NONE',  ( -17.27928175550000134, 1460.220522733030066, 228.2633105307979804 ) ) ;
#51585=EDGE_LOOP ( 'NONE', ( #28857, #92506, #11663, #82280 ) ) ;
#51586=ORIENTED_EDGE ( 'NONE', *, *, #78500, .F. ) ;
#51588=CARTESIAN_POINT ( 'NONE',  ( 1.143529715360000064E-14, 1421.542806690330053, 144.1893924737979944 ) ) ;
#51590=AXIS2_PLACEMENT_3D ( 'NONE', #61797, #27072, #61256 ) ;
#51596=CARTESIAN_POINT ( 'NONE',  ( 33.79495575609362845, 1443.086052842850904, 154.8158086860452158 ) ) ;
#51598=ORIENTED_EDGE ( 'NONE', *, *, #52715, .F. ) ;
#51601=ORIENTED_EDGE ( 'NONE', *, *, #95406, .F. ) ;
#51602=CARTESIAN_POINT ( 'NONE',  ( 11.74262852945270019, 1426.700939307690078, 144.5631990736900150 ) ) ;
#51605=ORIENTED_EDGE ( 'NONE', *, *, #68016, .T. ) ;
#51606=CARTESIAN_POINT ( 'NONE',  ( -13.57909981250000087, 1416.568813547830132, 221.8977233994979770 ) ) ;
#51607=CARTESIAN_POINT ( 'NONE',  ( -15.95383389570000077, 1506.798305147730161, 224.6865364803979901 ) ) ;
#51608=CARTESIAN_POINT ( 'NONE',  ( 7.009648883750000614, 1508.650232072529889, 235.9040373969980067 ) ) ;
#51610=CARTESIAN_POINT ( 'NONE',  ( -5.982287179200000082, 1424.434878864929942, 186.5640619623980001 ) ) ;
#51613=B_SPLINE_CURVE_WITH_KNOTS ( 'NONE', 5,
 ( #61895, #54052, #88178, #20391, #46191, #104415 ),
 .UNSPECIFIED., .F., .F.,
 ( 6, 6 ),
 ( -2.000000000000000000, 0.000000000000000000 ),
 .UNSPECIFIED. ) ;
#51616=CARTESIAN_POINT ( 'NONE',  ( 25.28594636015140296, 1472.590752081330038, 206.2214039951899736 ) ) ;
#51617=CARTESIAN_POINT ( 'NONE',  ( 17.53810613550000141, 1458.155921961129934, 230.1375793178980302 ) ) ;
#51619=CARTESIAN_POINT ( 'NONE',  ( 15.45814005882069786, 1507.562498016489826, 226.0579763435260077 ) ) ;
#51620=EDGE_CURVE ( 'NONE', #65987, #69312, #108263, .T. ) ;
#51621=CARTESIAN_POINT ( 'NONE',  ( -2.499955718113179959, 1419.779050710960064, 121.7745100861179992 ) ) ;
#51622=ORIENTED_EDGE ( 'NONE', *, *, #52796, .F. ) ;
#51623=CARTESIAN_POINT ( 'NONE',  ( 18.42577555256999844, 1424.509265906519886, 223.4215472205989954 ) ) ;
#51625=CARTESIAN_POINT ( 'NONE',  ( -2.938567406957015127, 1485.191830619298344, 183.0435406588377703 ) ) ;
#51626=CARTESIAN_POINT ( 'NONE',  ( -17.52110315343864855, 1410.887420241879909, 192.7668757445707115 ) ) ;
#51629=CARTESIAN_POINT ( 'NONE',  ( 1.532287138359999856, 1453.154034701829914, 188.6110597941980132 ) ) ;
#51632=CARTESIAN_POINT ( 'NONE',  ( -11.51579808750000034, 1427.983711584930006, 149.6431119016979778 ) ) ;
#51633=CARTESIAN_POINT ( 'NONE',  ( -10.87386229588725861, 1426.225512375807057, 148.5386954957300247 ) ) ;
#51634=CARTESIAN_POINT ( 'NONE',  ( -4.039629965989999683, 1440.883721145919935, 185.1940559541980065 ) ) ;
#51636=CARTESIAN_POINT ( 'NONE',  ( -10.85852385830536448, 1424.794007418652882, 138.1924915167475660 ) ) ;
#51638=CARTESIAN_POINT ( 'NONE',  ( -2.493947715939999643, 1442.756953654919926, 150.6345094620980092 ) ) ;
#51641=CARTESIAN_POINT ( 'NONE',  ( -17.15173707733800157, 1460.896355352879937, 228.2717902142180151 ) ) ;
#51644=VECTOR ( 'NONE', #99874, 1000.000000000000000 ) ;
#51645=CARTESIAN_POINT ( 'NONE',  ( 27.10793701029999880, 1412.310179361130167, 268.1710502007979926 ) ) ;
#51646=CARTESIAN_POINT ( 'NONE',  ( -4.363122647530000009, 1409.354802298930053, 121.6099336315979969 ) ) ;
#51647=CIRCLE ( 'NONE', #94538, 8.000000000000007105 ) ;
#51648=CARTESIAN_POINT ( 'NONE',  ( 19.16352043740000255, 1449.733021707809939, 192.2423658547980097 ) ) ;
#51649=CARTESIAN_POINT ( 'NONE',  ( -0.2658531787139999936, 1507.120040072329857, 237.3289624399980084 ) ) ;
#51650=CARTESIAN_POINT ( 'NONE',  ( 10.81507089421240053, 1424.921187596799882, 144.1620444706739761 ) ) ;
#51651=CARTESIAN_POINT ( 'NONE',  ( 21.32617020629999871, 1509.431680019330088, 227.8426433468980292 ) ) ;
#51654=CARTESIAN_POINT ( 'NONE',  ( -13.42598331690000002, 1444.386710359030076, 186.9377794141980189 ) ) ;
#51655=EDGE_CURVE ( 'NONE', #51991, #7508, #20048, .T. ) ;
#51658=CARTESIAN_POINT ( 'NONE',  ( -3.810473913917186373, 1457.645299305861499, 229.1842260504324997 ) ) ;
#51662=CARTESIAN_POINT ( 'NONE',  ( -14.75167259043490020, 1409.428200145470100, 206.7901764737640065 ) ) ;
#51663=CARTESIAN_POINT ( 'NONE',  ( 11.44928335637692918, 1425.357787524876585, 138.1871431916367499 ) ) ;
#51666=CARTESIAN_POINT ( 'NONE',  ( -23.62453004620000030, 1470.926794567029901, 268.8227032888980261 ) ) ;
#51670=CARTESIAN_POINT ( 'NONE',  ( -24.33268552243512062, 1444.628224150390679, 211.2399863042838888 ) ) ;
#51673=CARTESIAN_POINT ( 'NONE',  ( 18.09890889826640148, 1424.873618492820015, 225.7493724871799827 ) ) ;
#51674=CARTESIAN_POINT ( 'NONE',  ( 12.18885905831090177, 1416.259629946529913, 223.5006617761420102 ) ) ;
#51679=CARTESIAN_POINT ( 'NONE',  ( -23.66755926680000144, 1411.100008216330025, 206.9440434488080029 ) ) ;
#51680=CARTESIAN_POINT ( 'NONE',  ( 14.45747078059999957, 1416.828040557830036, 196.8519857451980215 ) ) ;
#51689=CARTESIAN_POINT ( 'NONE',  ( 11.72625744468970055, 1426.702793517190003, 143.3981854150229935 ) ) ;
#51693=CARTESIAN_POINT ( 'NONE',  ( -17.25022837948109711, 1507.614846716840020, 224.2951197320900008 ) ) ;
#51695=CARTESIAN_POINT ( 'NONE',  ( -10.57136850119649374, 1398.226370804211456, 216.7217188148681544 ) ) ;
#51696=CARTESIAN_POINT ( 'NONE',  ( -4.045957869977510057, 1440.951247040982707, 156.1595413419819920 ) ) ;
#51698=CARTESIAN_POINT ( 'NONE',  ( 1.430007510489999856, 1507.678536141130053, 236.8162301602979767 ) ) ;
#51699=ADVANCED_FACE ( 'NONE', ( #68055 ), #41722, .F. ) ;
#51701=CIRCLE ( 'NONE', #53475, 28.41070217520000440 ) ;
#51705=ORIENTED_EDGE ( 'NONE', *, *, #19215, .T. ) ;
#51706=CARTESIAN_POINT ( 'NONE',  ( 11.96561352722999949, 1433.598104579079973, 150.0754075377500101 ) ) ;
#51707=CARTESIAN_POINT ( 'NONE',  ( 27.04486969230000071, 1509.634167057629838, 216.9802351812680001 ) ) ;
#51708=ORIENTED_EDGE ( 'NONE', *, *, #38008, .F. ) ;
#51710=CARTESIAN_POINT ( 'NONE',  ( -23.82022599419999764, 1509.070378065730210, 195.5050499778980111 ) ) ;
#51713=CARTESIAN_POINT ( 'NONE',  ( 9.110233712619999480, 1428.462521060929930, 112.4493539157979995 ) ) ;
#51715=CARTESIAN_POINT ( 'NONE',  ( 19.64145264752830045, 1498.117040017750014, 228.8701979158510085 ) ) ;
#51717=CIRCLE ( 'NONE', #110676, 2.000000000000001776 ) ;
#51718=CARTESIAN_POINT ( 'NONE',  ( 4.365873002549999882, 1507.637804422629870, 181.7436736497979837 ) ) ;
#51721=CARTESIAN_POINT ( 'NONE',  ( 16.17522453369999980, 1409.477911658830180, 225.6432838665979830 ) ) ;
#51725=CARTESIAN_POINT ( 'NONE',  ( 13.46591420274270057, 1415.020374543940079, 197.8571796951229942 ) ) ;
#51726=CARTESIAN_POINT ( 'NONE',  ( 11.57593930269999838, 1432.295998248850083, 151.1968184610979620 ) ) ;
#51729=CARTESIAN_POINT ( 'NONE',  ( 13.76712058163199970, 1435.795625921070041, 150.2004772032130120 ) ) ;
#51732=CARTESIAN_POINT ( 'NONE',  ( 12.99399919968730011, 1444.879491996346360, 169.4223100370116981 ) ) ;
#51733=CARTESIAN_POINT ( 'NONE',  ( -1.085166694420000022, 1466.317866144730033, 235.5238959666980065 ) ) ;
#51737=B_SPLINE_SURFACE_WITH_KNOTS ( 'NONE', 5, 5, ( 
 ( #5882, #55758, #23213, #57951, #38908, #65797, #92084, #39482, #108886 ),
 ( #107784, #32730, #99361, #48453, #6432, #14816, #89876, #31069, #98274 ),
 ( #57413, #82018, #47330, #64710, #81459, #4764, #65250, #73090, #41127 ),
 ( #56842, #90974, #5323, #108336, #100482, #74206, #107230, #31619, #99918 ),
 ( #98828, #49003, #22088, #56285, #23764, #49551, #90415, #6973, #75307 ),
 ( #68563, #110539, #94278, #15901, #33272, #58498, #8617, #24854, #50101 ) ),
 .UNSPECIFIED., .F., .F., .F.,
 ( 6, 6 ),
 ( 6, 3, 6 ),
 ( 1.365479238354990077, 2.643755244583379849 ),
 ( 0.000000000000000000, 1.000000000000000000, 2.000011373467919906 ),
 .UNSPECIFIED. ) ;
#51738=VECTOR ( 'NONE', #67191, 1000.000000000000114 ) ;
#51746=CARTESIAN_POINT ( 'NONE',  ( 22.91311234439279687, 1440.913060387330006, 231.3965099084779808 ) ) ;
#51747=CARTESIAN_POINT ( 'NONE',  ( -19.01903537849999992, 1509.560719700929894, 231.2847914768979933 ) ) ;
#51749=CARTESIAN_POINT ( 'NONE',  ( -5.751971152109999430, 1409.281467972630026, 187.6758683908980174 ) ) ;
#51751=CARTESIAN_POINT ( 'NONE',  ( -11.36018337610000195, 1414.996442546130083, 195.9645814914979951 ) ) ;
#51753=CARTESIAN_POINT ( 'NONE',  ( 22.56647849180000165, 1431.126951193569994, 217.0164414152080212 ) ) ;
#51759=B_SPLINE_SURFACE_WITH_KNOTS ( 'NONE', 5, 5, ( 
 ( #38049, #28545, #45371, #78399, #96863, #72226 ),
 ( #104146, #19011, #53212, #87353, #10649, #44816 ),
 ( #78970, #2275, #62175, #96301, #19581, #79511 ),
 ( #71131, #22866, #39128, #107442, #56513, #12835 ),
 ( #30177, #40244, #47015, #55961, #13367, #108553 ),
 ( #74426, #23437, #66028, #109123, #4983, #73307 ),
 ( #82796, #81139, #57072, #100151, #89544, #47556 ),
 ( #48672, #106888, #4455, #83345, #57631, #38582 ),
 ( #81677, #72761, #91199, #31843, #64369, #31290 ),
 ( #82248, #91745, #99583, #30739, #22310, #90640 ),
 ( #98491, #99033, #15021, #21760, #40797, #6642 ),
 ( #32403, #49219, #13921, #100689, #23972, #74975 ) ),
 .UNSPECIFIED., .F., .F., .F.,
 ( 6, 3, 3, 6 ),
 ( 6, 6 ),
 ( 5.135474514900000287, 7.195071677909999686, 11.31426600390000026, 15.30658226960000157 ),
 ( 0.000000000000000000, 2.031188710939999975 ),
 .UNSPECIFIED. ) ;
#51762=CARTESIAN_POINT ( 'NONE',  ( -21.25831203310000106, 1509.376731495729928, 190.0552735725980256 ) ) ;
#51766=CARTESIAN_POINT ( 'NONE',  ( -15.48152669746104060, 1486.079334726010075, 186.6356546698670513 ) ) ;
#51768=EDGE_LOOP ( 'NONE', ( #52138, #57230, #22463, #62228 ) ) ;
#51770=CARTESIAN_POINT ( 'NONE',  ( 33.60183515439999979, 1440.913060383429865, 248.0844435622979915 ) ) ;
#51771=CARTESIAN_POINT ( 'NONE',  ( 2.851403222469678145, 1451.784497409910728, 183.8440006949768701 ) ) ;
#51773=CARTESIAN_POINT ( 'NONE',  ( -5.272191020579219511, 1507.500514379029937, 236.2607515669679970 ) ) ;
#51777=CARTESIAN_POINT ( 'NONE',  ( 19.74853702200000427, 1455.472137956930283, 226.4474092902979976 ) ) ;
#51783=CARTESIAN_POINT ( 'NONE',  ( 27.68253990799999897, 1507.989615297430191, 207.6661388674179989 ) ) ;
#51785=CARTESIAN_POINT ( 'NONE',  ( 24.57684147700000210, 1440.965848065480031, 212.8359072196480213 ) ) ;
#51789=CARTESIAN_POINT ( 'NONE',  ( 30.84776965385309921, 1436.903798512589901, 136.6563984318939902 ) ) ;
#51790=CARTESIAN_POINT ( 'NONE',  ( -26.03280816719999891, 1448.977735834329906, 137.1485333417979859 ) ) ;
#51791=CARTESIAN_POINT ( 'NONE',  ( -12.27023110815660090, 1416.839692126590080, 194.6640136892829958 ) ) ;
#51798=CARTESIAN_POINT ( 'NONE',  ( -39.47393889809999479, 1426.323565199129916, 271.1218459616979999 ) ) ;
#51802=CARTESIAN_POINT ( 'NONE',  ( 10.93642306640074224, 1424.903169850106678, 138.2808805187167707 ) ) ;
#51805=CARTESIAN_POINT ( 'NONE',  ( -12.93281143504288089, 1444.916649965908391, 186.1917424862305381 ) ) ;
#51808=TOROIDAL_SURFACE ( 'NONE', #103671, 7.016581249619999738, 2.000000000000000000 ) ;
#51809=CARTESIAN_POINT ( 'NONE',  ( -13.70524990486647887, 1420.114476090270955, 227.7448751836718372 ) ) ;
#51810=CARTESIAN_POINT ( 'NONE',  ( -7.686253120226395730, 1451.400019608767252, 153.0367187530530941 ) ) ;
#51812=CARTESIAN_POINT ( 'NONE',  ( -18.06717587838990013, 1416.826860677879949, 209.3441468771879954 ) ) ;
#51813=CARTESIAN_POINT ( 'NONE',  ( 25.09552600510000175, 1436.154465690999814, 137.4570931897980017 ) ) ;
#51814=CARTESIAN_POINT ( 'NONE',  ( -6.458058201505220808, 1396.138580749159928, 200.1630282699710222 ) ) ;
#51816=ORIENTED_EDGE ( 'NONE', *, *, #53466, .T. ) ;
#51817=CARTESIAN_POINT ( 'NONE',  ( -17.12363160903159809, 1410.143831958050214, 225.8068293093689931 ) ) ;
#51822=DIRECTION ( 'NONE',  ( -1.987380029059999976E-13, 6.832419524060000430E-15, 1.000000000000000000 ) ) ;
#51824=CARTESIAN_POINT ( 'NONE',  ( 10.70864553689999887, 1425.696178928829795, 94.99429751269789790 ) ) ;
#51827=CARTESIAN_POINT ( 'NONE',  ( -11.87502380990000006, 1433.007271236840097, 149.9804568709980117 ) ) ;
#51832=CARTESIAN_POINT ( 'NONE',  ( 7.865891863719999932, 1508.177616610530094, 182.6824962180979810 ) ) ;
#51833=CARTESIAN_POINT ( 'NONE',  ( 2.493346804579999798, 1449.100684543890111, 182.3308732938979801 ) ) ;
#51837=ORIENTED_EDGE ( 'NONE', *, *, #3615, .T. ) ;
#51838=DIRECTION ( 'NONE',  ( 1.000000000000000000, 0.000000000000000000, 0.000000000000000000 ) ) ;
#51840=CARTESIAN_POINT ( 'NONE',  ( -1.438086367899999773, 1472.604997560230004, 270.3713140929979772 ) ) ;
#51841=CARTESIAN_POINT ( 'NONE',  ( 12.60016312909735881, 1434.521797930790854, 147.2295963768206661 ) ) ;
#51842=CARTESIAN_POINT ( 'NONE',  ( -3.476453357950000100, 1485.977928129130078, 182.2504961336979932 ) ) ;
#51846=CARTESIAN_POINT ( 'NONE',  ( -35.15227308153860264, 1451.683551734719913, 135.1171324062460144 ) ) ;
#51848=CARTESIAN_POINT ( 'NONE',  ( -16.48401273470000206, 1408.913060387329779, 201.9064470506779685 ) ) ;
#51850=FACE_OUTER_BOUND ( 'NONE', #61167, .T. ) ;
#51851=CARTESIAN_POINT ( 'NONE',  ( -18.60991398711139766, 1409.400608050520077, 269.3767701890689636 ) ) ;
#51852=CARTESIAN_POINT ( 'NONE',  ( -14.07097133599449990, 1435.229630904430223, 149.3999849555079891 ) ) ;
#51854=CARTESIAN_POINT ( 'NONE',  ( -11.76883255979999987, 1432.286228545659924, 150.8119424982980092 ) ) ;
#51855=CARTESIAN_POINT ( 'NONE',  ( 13.12953739719999824, 1444.897984030819998, 187.7977427021979793 ) ) ;
#51856=B_SPLINE_SURFACE_WITH_KNOTS ( 'NONE', 5, 5, ( 
 ( #84994, #32940, #43573, #92852, #41911, #8289 ),
 ( #67129, #35158, #25081, #68792, #58717, #50334 ),
 ( #51411, #85542, #84460, #76065, #95074, #1035 ),
 ( #34606, #8839, #59284, #17772, #93402, #42451 ),
 ( #76611, #102892, #110763, #94500, #34053, #483 ),
 ( #102353, #25636, #77180, #26191, #60379, #55713 ),
 ( #36266, #1579, #27870, #56796, #70455, #5280 ),
 ( #98782, #89834, #38322, #47839, #64665, #38868 ),
 ( #65206, #81972, #39436, #4724, #13106, #87225 ) ),
 .UNSPECIFIED., .F., .F., .F.,
 ( 6, 3, 6 ),
 ( 6, 6 ),
 ( 0.7655572723410000169, 2.316155491850000026, 3.835724788409999864 ),
 ( 0.000000000000000000, 1.000000000000000000 ),
 .UNSPECIFIED. ) ;
#51862=CARTESIAN_POINT ( 'NONE',  ( -14.01202549919999996, 1470.465034534930055, 187.2960763698980031 ) ) ;
#51865=CARTESIAN_POINT ( 'NONE',  ( 9.382531478650001588, 1414.913060387329779, 223.2369444284979920 ) ) ;
#51868=CARTESIAN_POINT ( 'NONE',  ( -26.99539266469999887, 1509.166234529530129, 202.5158776357180272 ) ) ;
#51869=B_SPLINE_SURFACE_WITH_KNOTS ( 'NONE', 5, 5, ( 
 ( #24211, #88271, #32081, #45740, #109356, #30424, #99263, #57855, #3191, #5793, #15259, #90321, #32636, #73557, #81924, #107691, #30974, #99820, #56743, #14167, #48352, #82492, #74103, #39935, #31519, #7427, #68462 ),
 ( #69576, #60061, #18016, #159, #85224, #85785, #77941, #101463, #59504, #109893, #9622, #86336, #84128, #41593, #67913, #75748, #103122, #43791, #42140, #93077, #33172, #102566, #69017, #34282, #1248, #43250, #24749 ),
 ( #35388, #84674, #103694, #26423, #94178, #25859, #60617, #102020, #94738, #25304, #42691, #51099, #58398, #67362, #17449, #58947, #16352, #7973, #701, #51648, #50549, #76290, #34831, #52211, #92523, #110440, #9084 ),
 ( #15791, #33720, #49992, #93615, #16894, #8516, #77399, #76849, #2375, #36491, #95301, #35951, #44923, #71232, #27540, #97500, #29194, #20768, #54428, #61722, #61183, #70137, #78503, #88561, #18561, #104249, #95844 ),
 ( #19112, #70688, #38137, #80146, #1814, #96962, #86889, #37594, #3466, #104800, #45474, #105355, #71796, #53315, #54968, #52756, #28646, #87458, #11844, #62849, #89095, #2921, #10752, #79070, #46017, #28088, #62275 ),
 ( #105914, #19681, #96405, #10184, #20227, #44358, #63384, #53886, #88022, #11306, #79617, #37038, #12382, #46568, #80703, #4012, #72319, #26994, #73406, #57721, #55511, #5080, #108647, #107544, #91839, #89640, #39231 ) ),
 .UNSPECIFIED., .F., .F., .F.,
 ( 6, 6 ),
 ( 6, 3, 3, 3, 3, 3, 3, 3, 6 ),
 ( 2.177958220529999878, 99.41336299639999652 ),
 ( 27.66640414800000158, 34.17054740399999702, 36.60181165779999901, 37.81744378469999646, 38.42525984819999962, 39.03307591160000101, 39.44347959870000153, 39.85388328589999674, 40.67469066009999779 ),
 .UNSPECIFIED. ) ;
#51873=CARTESIAN_POINT ( 'NONE',  ( -5.805073486770000457, 1409.115778020430298, 195.2388944971980038 ) ) ;
#51875=AXIS2_PLACEMENT_3D ( 'NONE', #20143, #46486, #96314 ) ;
#51876=CARTESIAN_POINT ( 'NONE',  ( -9.042061235680000308, 1445.734082586790009, 185.2473999953979842 ) ) ;
#51879=CARTESIAN_POINT ( 'NONE',  ( 27.33420534990000306, 1488.691127165830039, 209.8949700443229744 ) ) ;
#51880=CARTESIAN_POINT ( 'NONE',  ( 20.10214423559910202, 1487.444758163989945, 225.8674582954020025 ) ) ;
#51881=CARTESIAN_POINT ( 'NONE',  ( -25.54454699020000064, 1436.325264848330107, 137.1090852991980285 ) ) ;
#51882=AXIS2_PLACEMENT_3D ( 'NONE', #94636, #93525, #604 ) ;
#51885=CARTESIAN_POINT ( 'NONE',  ( -13.93822302919999956, 1413.184296187929931, 227.1928256324979998 ) ) ;
#51888=VERTEX_POINT ( 'NONE', #103838 ) ;
#51889=CARTESIAN_POINT ( 'NONE',  ( -1.772459524117049989, 1451.934256328719812, 184.2034882996969998 ) ) ;
#51890=CARTESIAN_POINT ( 'NONE',  ( -4.148108818479999904, 1412.836893066629955, 232.2745409437980015 ) ) ;
#51892=ORIENTED_EDGE ( 'NONE', *, *, #84946, .T. ) ;
#51895=CARTESIAN_POINT ( 'NONE',  ( 12.67555790997639953, 1434.596121652720058, 149.5884656837649800 ) ) ;
#51896=CARTESIAN_POINT ( 'NONE',  ( 15.62608574728940170, 1459.304094441330108, 229.5211440070559945 ) ) ;
#51897=CARTESIAN_POINT ( 'NONE',  ( -21.67692661982870206, 1509.608767922699826, 228.6318993757969906 ) ) ;
#51898=CARTESIAN_POINT ( 'NONE',  ( -1.498828828049999951, 1408.965400643329986, 187.6521917822979901 ) ) ;
#51900=CARTESIAN_POINT ( 'NONE',  ( 4.229538064822990329, 1441.537955797840141, 165.0787593380850069 ) ) ;
#51903=CARTESIAN_POINT ( 'NONE',  ( 15.91624037646960055, 1491.015088416080062, 194.0444298851370206 ) ) ;
#51904=CARTESIAN_POINT ( 'NONE',  ( 20.20853917690000401, 1508.359852710729911, 189.3077113257979818 ) ) ;
#51907=CARTESIAN_POINT ( 'NONE',  ( -12.72965190870000107, 1416.819760216229952, 195.1130952921980111 ) ) ;
#51911=CARTESIAN_POINT ( 'NONE',  ( 1.533058233270000015, 1417.373139556630122, 235.5867829536979912 ) ) ;
#51912=CARTESIAN_POINT ( 'NONE',  ( 8.313287170068500487, 1507.316777277299934, 183.0869016502879845 ) ) ;
#51917=CARTESIAN_POINT ( 'NONE',  ( 13.36997651309999924, 1416.851343894929869, 196.3340833727979771 ) ) ;
#51921=CARTESIAN_POINT ( 'NONE',  ( 41.45644848187150444, 1440.913060354650042, 261.2593951003379971 ) ) ;
#51924=CARTESIAN_POINT ( 'NONE',  ( 11.14671379024469999, 1434.019377051509991, 151.6529839732360188 ) ) ;
#51927=CARTESIAN_POINT ( 'NONE',  ( 24.27272702730000020, 1449.843846490510032, 206.2143647668480071 ) ) ;
#51929=CARTESIAN_POINT ( 'NONE',  ( 4.286107831027711867, 1410.438896930658757, 186.1261285953802087 ) ) ;
#51934=CARTESIAN_POINT ( 'NONE',  ( 13.17906415938499975, 1414.913527275050001, 198.1030012665459878 ) ) ;
#51936=EDGE_CURVE ( 'NONE', #28587, #106610, #94589, .T. ) ;
#51940=ORIENTED_EDGE ( 'NONE', *, *, #2873, .T. ) ;
#51941=CARTESIAN_POINT ( 'NONE',  ( -17.64542808779836491, 1460.260031838558461, 228.1847870265016525 ) ) ;
#51945=EDGE_CURVE ( 'NONE', #80494, #87520, #69924, .T. ) ;
#51948=CARTESIAN_POINT ( 'NONE',  ( 3.118627138969999990, 1507.020746158230168, 237.9289388427980043 ) ) ;
#51950=CARTESIAN_POINT ( 'NONE',  ( 40.26153007682929541, 1443.187744381950097, 137.0666827882720042 ) ) ;
#51951=CARTESIAN_POINT ( 'NONE',  ( 22.09833645820000214, 1506.806593688229896, 209.1697492017360105 ) ) ;
#51952=CARTESIAN_POINT ( 'NONE',  ( -19.16279666149999983, 1470.534631754830116, 262.3396919526979900 ) ) ;
#51956=CARTESIAN_POINT ( 'NONE',  ( -12.82658623871375347, 1435.929109846025995, 150.8182851086763208 ) ) ;
#51957=CARTESIAN_POINT ( 'NONE',  ( -20.53890917329999866, 1486.102232517730044, 191.0326899443980153 ) ) ;
#51958=CARTESIAN_POINT ( 'NONE',  ( 3.773835479270000182, 1410.421536211630155, 185.9548053891980146 ) ) ;
#51960=CARTESIAN_POINT ( 'NONE',  ( -7.981991148520000579, 1441.362204533440035, 154.1152758918979941 ) ) ;
#51963=AXIS2_PLACEMENT_3D ( 'NONE', #74315, #107339, #31175 ) ;
#51964=CARTESIAN_POINT ( 'NONE',  ( -23.90685205709999650, 1451.267540530529914, 140.4958681723980192 ) ) ;
#51965=CARTESIAN_POINT ( 'NONE',  ( 1.420259601960000229, 1466.712985171129958, 235.0376566307980113 ) ) ;
#51969=CARTESIAN_POINT ( 'NONE',  ( -42.06231866970000510, 1440.913089571779892, 269.6487540859979504 ) ) ;
#51971=CARTESIAN_POINT ( 'NONE',  ( 17.60627587029999930, 1410.895669429430200, 224.1775087542980032 ) ) ;
#51974=CARTESIAN_POINT ( 'NONE',  ( 2.760778564396810353, 1409.009468899150079, 230.1977509304229841 ) ) ;
#51976=CARTESIAN_POINT ( 'NONE',  ( -10.37900483499999993, 1419.722126144429922, 232.2032976616980022 ) ) ;
#51979=LINE ( 'NONE', #35160, #16205 ) ;
#51981=CARTESIAN_POINT ( 'NONE',  ( -45.44490940612519125, 1437.744605196359998, 268.9801658155380437 ) ) ;
#51984=ORIENTED_EDGE ( 'NONE', *, *, #48641, .F. ) ;
#51986=AXIS2_PLACEMENT_3D ( 'NONE', #54808, #10590, #86738 ) ;
#51987=DIRECTION ( 'NONE',  ( -0.000000000000000000, 1.000000000000000000, 0.000000000000000000 ) ) ;
#51990=CARTESIAN_POINT ( 'NONE',  ( -25.23019512061160086, 1452.032085083439824, 135.4492350236539835 ) ) ;
#51991=VERTEX_POINT ( 'NONE', #29328 ) ;
#51992=CARTESIAN_POINT ( 'NONE',  ( -16.35911259859972233, 1409.492701125528583, 225.1152623397985337 ) ) ;
#51994=CARTESIAN_POINT ( 'NONE',  ( 14.13297884659999859, 1452.811554597230042, 195.2238856287980013 ) ) ;
#51995=CARTESIAN_POINT ( 'NONE',  ( 1.797565579689999860, 1415.903556134529936, 232.4419632246980143 ) ) ;
#51999=CARTESIAN_POINT ( 'NONE',  ( -18.64588645199999917, 1416.828044802730119, 208.5593772625580016 ) ) ;
#52000=ORIENTED_EDGE ( 'NONE', *, *, #56916, .F. ) ;
#52001=CARTESIAN_POINT ( 'NONE',  ( -3.129454527291580135, 1407.723237535949920, 270.1357211735799524 ) ) ;
#52003=CARTESIAN_POINT ( 'NONE',  ( 8.734601244239950546, 1418.821511342440090, 231.3068792023239837 ) ) ;
#52006=ORIENTED_EDGE ( 'NONE', *, *, #59298, .T. ) ;
#52007=VERTEX_POINT ( 'NONE', #37194 ) ;
#52008=CARTESIAN_POINT ( 'NONE',  ( -23.64670054153389955, 1410.982901525189845, 210.3775373128219996 ) ) ;
#52009=CARTESIAN_POINT ( 'NONE',  ( -4.086401651919999267, 1424.208576867429883, 185.4429785608980126 ) ) ;
#52011=CARTESIAN_POINT ( 'NONE',  ( -4.823778297959999684, 1426.859560269130043, 144.1938086916980239 ) ) ;
#52012=CARTESIAN_POINT ( 'NONE',  ( -19.76012964183019704, 1467.135250698569962, 193.4660110028719942 ) ) ;
#52013=CARTESIAN_POINT ( 'NONE',  ( -22.29148574759999946, 1425.804551132829829, 216.5767124936379844 ) ) ;
#52014=CARTESIAN_POINT ( 'NONE',  ( 28.58215788712900007, 1468.635916194609990, 268.1351379920200202 ) ) ;
#52016=CARTESIAN_POINT ( 'NONE',  ( -10.22810209145352900, 1464.519780891043638, 232.1939053660614718 ) ) ;
#52018=( BOUNDED_CURVE ( )  B_SPLINE_CURVE ( 3, ( #83475, #22446, #82395, #47693 ),
 .UNSPECIFIED., .F., .F. ) 
 B_SPLINE_CURVE_WITH_KNOTS ( ( 4, 4 ),
 ( 3.142823553869715347, 3.152136943596000052 ),
 .UNSPECIFIED. ) 
 CURVE ( )  GEOMETRIC_REPRESENTATION_ITEM ( )  RATIONAL_B_SPLINE_CURVE ( ( 1.000000000000000000, 0.9999927717440458830, 0.9999927717440458830, 1.000000000000000000 ) ) 
 REPRESENTATION_ITEM ( '' )  );
#52020=ORIENTED_EDGE ( 'NONE', *, *, #93906, .T. ) ;
#52022=CARTESIAN_POINT ( 'NONE',  ( 1.510002137662999955, 1461.120581648620146, 183.1207398647079856 ) ) ;
#52023=CARTESIAN_POINT ( 'NONE',  ( 22.91483027350000157, 1409.739594360729825, 208.7501026320239816 ) ) ;
#52027=ADVANCED_FACE ( 'NONE', ( #52359 ), #33100, .F. ) ;
#52028=CARTESIAN_POINT ( 'NONE',  ( 25.97075925569999910, 1451.764531650130039, 135.9704145892980023 ) ) ;
#52029=B_SPLINE_SURFACE_WITH_KNOTS ( 'NONE', 5, 5, ( 
 ( #71188, #77362, #35910, #26953, #25821, #19071, #104207, #79031, #1773 ),
 ( #43755, #2332, #60020, #62234, #94140, #53841, #87979, #52168, #1213 ),
 ( #77906, #17972, #61680, #11267, #51608, #60578, #10144, #27493, #43212 ),
 ( #663, #95803, #34794, #95258, #53275, #86299, #79573, #18519, #86851 ),
 ( #68981, #94698, #69535, #61144, #87414, #2875, #45429, #30237, #55472 ),
 ( #12891, #47612, #96919, #72278, #5044, #47069, #89599, #81193, #38100 ) ),
 .UNSPECIFIED., .F., .F., .F.,
 ( 6, 6 ),
 ( 6, 3, 6 ),
 ( 11.16857693960000120, 24.00668087930000283 ),
 ( 0.000000000000000000, 1.000000000000000000, 2.000000000000000000 ),
 .UNSPECIFIED. ) ;
#52034=CARTESIAN_POINT ( 'NONE',  ( 18.42637209560000144, 1409.556523480330043, 196.3080071043980013 ) ) ;
#52035=CARTESIAN_POINT ( 'NONE',  ( 27.48389906189999721, 1443.913060387330006, 168.8435737885979790 ) ) ;
#52036=CARTESIAN_POINT ( 'NONE',  ( 3.421791868836843165, 1439.691577471224718, 184.4543791659172314 ) ) ;
#52038=CARTESIAN_POINT ( 'NONE',  ( -23.47750638058768757, 1434.817782033998583, 212.9234740453307779 ) ) ;
#52039=CARTESIAN_POINT ( 'NONE',  ( 11.03217570710000039, 1409.298312452229993, 227.8647431501979952 ) ) ;
#52040=CARTESIAN_POINT ( 'NONE',  ( -0.007173723813013069966, 1508.946327270009988, 179.4591247994410139 ) ) ;
#52044=CARTESIAN_POINT ( 'NONE',  ( 11.01105141466669934, 1414.913060387399810, 221.0326450546259878 ) ) ;
#52046=CARTESIAN_POINT ( 'NONE',  ( 11.13648443495080009, 1432.345323076100158, 151.6342730693140197 ) ) ;
#52052=CARTESIAN_POINT ( 'NONE',  ( -4.290289618250000103, 1461.407663418029870, 243.9198229205979942 ) ) ;
#52054=CARTESIAN_POINT ( 'NONE',  ( 11.80976821910000041, 1433.247602250280124, 150.6126538827979857 ) ) ;
#52055=CARTESIAN_POINT ( 'NONE',  ( 9.562842983910000427, 1454.397736359230066, 219.6133833293980047 ) ) ;
#52056=CARTESIAN_POINT ( 'NONE',  ( 11.61527099316350231, 1414.971349104640012, 197.1579164385690035 ) ) ;
#52062=CARTESIAN_POINT ( 'NONE',  ( 1.448679645196929933, 1507.129709964000085, 181.1126013477120011 ) ) ;
#52064=CARTESIAN_POINT ( 'NONE',  ( 13.01603395294319476, 1398.298686285902704, 209.4299075615936374 ) ) ;
#52065=CARTESIAN_POINT ( 'NONE',  ( 0.04734028010245310697, 1508.924978232730155, 238.6962546503989984 ) ) ;
#52067=CARTESIAN_POINT ( 'NONE',  ( 12.78654151607593015, 1416.818673880716915, 223.0773805434268127 ) ) ;
#52068=CARTESIAN_POINT ( 'NONE',  ( 26.50108598912411750, 1436.729172686955735, 136.8088966875825179 ) ) ;
#52076=CARTESIAN_POINT ( 'NONE',  ( -0.7130142951239999416, 1416.844618638430120, 227.9191939111979934 ) ) ;
#52078=CARTESIAN_POINT ( 'NONE',  ( 2.500000000000000000, 1443.913060387330006, 150.6726614421979775 ) ) ;
#52079=CARTESIAN_POINT ( 'NONE',  ( 12.40402065109999974, 1434.420118205629933, 149.6993386520979925 ) ) ;
#52081=CARTESIAN_POINT ( 'NONE',  ( -37.66742087365959435, 1450.649596001770078, 134.0999999985879754 ) ) ;
#52085=AXIS2_PLACEMENT_3D ( 'NONE', #43109, #34692, #24609 ) ;
#52087=CARTESIAN_POINT ( 'NONE',  ( -14.44608864360000133, 1416.522662137629823, 221.3854392607979946 ) ) ;
#52088=CARTESIAN_POINT ( 'NONE',  ( -6.227663043015771116, 1509.133838473635024, 237.8782978115028470 ) ) ;
#52090=CARTESIAN_POINT ( 'NONE',  ( 45.63712937690380755, 1440.913060387330006, 268.9747523971630017 ) ) ;
#52095=CARTESIAN_POINT ( 'NONE',  ( -16.69507587579999708, 1411.915237329530100, 191.7082158511979912 ) ) ;
#52099=CARTESIAN_POINT ( 'NONE',  ( -15.77423603240969996, 1409.463753444150143, 225.3878024414169943 ) ) ;
#52100=CARTESIAN_POINT ( 'NONE',  ( -0.7910245917146945249, 1426.918876941764893, 134.0999999980979851 ) ) ;
#52101=ORIENTED_EDGE ( 'NONE', *, *, #45319, .F. ) ;
#52103=ORIENTED_EDGE ( 'NONE', *, *, #75552, .T. ) ;
#52104=CARTESIAN_POINT ( 'NONE',  ( 27.59578647829999909, 1509.876726487329734, 217.1913344172780000 ) ) ;
#52107=CARTESIAN_POINT ( 'NONE',  ( 39.37269659054818050, 1451.600413132400945, 269.5993111650432752 ) ) ;
#52109=CARTESIAN_POINT ( 'NONE',  ( 18.48763279861755748, 1436.139455391317370, 214.3615573111846118 ) ) ;
#52112=CARTESIAN_POINT ( 'NONE',  ( -16.68599179819999989, 1461.099982565929849, 230.2790296985980092 ) ) ;
#52124=DIRECTION ( 'NONE',  ( 0.4794255386041986200, 0.000000000000000000, 0.8775825618903752012 ) ) ;
#52125=ORIENTED_EDGE ( 'NONE', *, *, #105425, .T. ) ;
#52126=CARTESIAN_POINT ( 'NONE',  ( 3.021259845790000085E-08, 1408.296884782030020, 262.4989465150980550 ) ) ;
#52127=CARTESIAN_POINT ( 'NONE',  ( -24.49050335060000094, 1430.357935323129823, 206.8695671012879984 ) ) ;
#52128=CARTESIAN_POINT ( 'NONE',  ( -10.60244528208989934, 1425.057211382899823, 130.8090886194080156 ) ) ;
#52129=CARTESIAN_POINT ( 'NONE',  ( 16.55649716813289984, 1410.443606432929982, 191.7825502688590120 ) ) ;
#52131=TOROIDAL_SURFACE ( 'NONE', #62886, 2.030931026690000252, 0.5000000000000000000 ) ;
#52132=CARTESIAN_POINT ( 'NONE',  ( 26.18610560624165018, 1509.940572648346006, 194.3908627882991311 ) ) ;
#52133=CARTESIAN_POINT ( 'NONE',  ( -18.79734767819999774, 1416.844618642430078, 208.4088319194450207 ) ) ;
#52135=CARTESIAN_POINT ( 'NONE',  ( 43.37195119983255864, 1452.013340143054393, 269.7132330850898256 ) ) ;
#52137=CARTESIAN_POINT ( 'NONE',  ( -35.45835282683830769, 1437.253800090359846, 136.5355674391020102 ) ) ;
#52138=ORIENTED_EDGE ( 'NONE', *, *, #5288, .T. ) ;
#52139=CARTESIAN_POINT ( 'NONE',  ( 13.97474060794100126, 1398.020587696859820, 206.9428454895969764 ) ) ;
#52141=CARTESIAN_POINT ( 'NONE',  ( -16.71362360910000078, 1459.161552659730205, 228.9915664566980240 ) ) ;
#52145=VERTEX_POINT ( 'NONE', #53894 ) ;
#52149=ADVANCED_FACE ( 'NONE', ( #19119 ), #84058, .T. ) ;
#52150=CARTESIAN_POINT ( 'NONE',  ( -19.59053950279439960, 1486.265866315750145, 189.8955481462990065 ) ) ;
#52151=CARTESIAN_POINT ( 'NONE',  ( 28.77729953137099983, 1509.917985831029910, 206.0039978706130057 ) ) ;
#52157=EDGE_LOOP ( 'NONE', ( #6709, #85317, #69656, #63817 ) ) ;
#52160=ORIENTED_EDGE ( 'NONE', *, *, #16760, .T. ) ;
#52161=CARTESIAN_POINT ( 'NONE',  ( 11.81926599889289875, 1429.255342282230004, 149.0484304434379794 ) ) ;
#52162=EDGE_CURVE ( 'NONE', #29251, #50772, #49213, .T. ) ;
#52165=VERTEX_POINT ( 'NONE', #48776 ) ;
#52167=CARTESIAN_POINT ( 'NONE',  ( -13.51610093809999924, 1443.501467202829872, 169.3501091259980171 ) ) ;
#52168=CARTESIAN_POINT ( 'NONE',  ( 4.908323279449999355, 1507.487947428030111, 235.7295937283979868 ) ) ;
#52171=CARTESIAN_POINT ( 'NONE',  ( -5.099269457000000116, 1423.012593427629781, 185.1299087936980072 ) ) ;
#52172=CARTESIAN_POINT ( 'NONE',  ( 4.146667765623250013, 1409.925191843709854, 270.0721511231989780 ) ) ;
#52177=CARTESIAN_POINT ( 'NONE',  ( 0.02188712286643353447, 1410.253115378247912, 233.2197962875069379 ) ) ;
#52178=EDGE_CURVE ( 'NONE', #85990, #81697, #106703, .T. ) ;
#52180=CARTESIAN_POINT ( 'NONE',  ( 16.71340900559999909, 1489.468502498129965, 194.5581736820979870 ) ) ;
#52181=CARTESIAN_POINT ( 'NONE',  ( -4.400896008966714845, 1423.841311741514801, 184.2785382031196377 ) ) ;
#52182=CARTESIAN_POINT ( 'NONE',  ( 17.99786997119990062, 1423.579729440439905, 225.1773348763740046 ) ) ;
#52184=VERTEX_POINT ( 'NONE', #21860 ) ;
#52185=CIRCLE ( 'NONE', #77194, 29.84605316733869174 ) ;
#52187=CARTESIAN_POINT ( 'NONE',  ( 38.63621011600843502, 1450.019461304174456, 134.8312852903657415 ) ) ;
#52188=CARTESIAN_POINT ( 'NONE',  ( -2.971677051434508776, 1485.527647794828226, 182.7973173799614131 ) ) ;
#52193=CARTESIAN_POINT ( 'NONE',  ( 17.33645362950000290, 1414.996442546130083, 210.3925741896480304 ) ) ;
#52195=CARTESIAN_POINT ( 'NONE',  ( -11.26505527650000005, 1429.630426659629848, 150.9929481330979968 ) ) ;
#52196=CARTESIAN_POINT ( 'NONE',  ( 19.33960037451650038, 1456.940524333479971, 224.5990868967689948 ) ) ;
#52198=EDGE_CURVE ( 'NONE', #43546, #80530, #73198, .T. ) ;
#52205=CARTESIAN_POINT ( 'NONE',  ( -16.67053790319999962, 1460.330596138029932, 228.3373634785979789 ) ) ;
#52207=CARTESIAN_POINT ( 'NONE',  ( 30.12542694869999593, 1414.418184686029917, 268.6829023064980220 ) ) ;
#52209=CARTESIAN_POINT ( 'NONE',  ( 23.55466122310000188, 1435.319754623780000, 138.4646105849980131 ) ) ;
#52211=CARTESIAN_POINT ( 'NONE',  ( 18.66630351470000093, 1449.735460805310140, 191.4766007327979764 ) ) ;
#52212=CARTESIAN_POINT ( 'NONE',  ( -21.59755472069999982, 1429.927022223929953, 220.3212187975979930 ) ) ;
#52216=CARTESIAN_POINT ( 'NONE',  ( -13.85929445549190042, 1410.325638904459993, 227.0940372234059907 ) ) ;
#52217=CARTESIAN_POINT ( 'NONE',  ( -16.90152335259999816, 1414.971339025629959, 205.6657720955479931 ) ) ;
#52218=CARTESIAN_POINT ( 'NONE',  ( -12.23547426050000020, 1441.747762228240163, 187.6912675146980121 ) ) ;
#52220=CARTESIAN_POINT ( 'NONE',  ( -33.52368713759999963, 1436.996791544049984, 136.5733088107979825 ) ) ;
#52222=ORIENTED_EDGE ( 'NONE', *, *, #30892, .F. ) ;
#52224=CARTESIAN_POINT ( 'NONE',  ( -14.56057633080500047, 1409.421526917029951, 205.7954462250399956 ) ) ;
#52225=CARTESIAN_POINT ( 'NONE',  ( 11.26238334597741719, 1425.491802413522009, 138.6337954581835845 ) ) ;
#52226=CARTESIAN_POINT ( 'NONE',  ( -5.327792725146696995, 1422.321596787008048, 138.7601748833760666 ) ) ;
#52227=CARTESIAN_POINT ( 'NONE',  ( -21.97983258780000071, 1471.906657365530009, 268.2775703267980134 ) ) ;
#52231=CARTESIAN_POINT ( 'NONE',  ( -24.42065677639604004, 1444.677908474019205, 211.1079349083759098 ) ) ;
#52233=CARTESIAN_POINT ( 'NONE',  ( 19.02704169900689735, 1456.915441405320053, 225.6706379604710264 ) ) ;
#52235=CARTESIAN_POINT ( 'NONE',  ( 14.57172186319999874, 1416.216739748630062, 219.6692783647980036 ) ) ;
#52236=CARTESIAN_POINT ( 'NONE',  ( 11.70773956419579953, 1415.348334734299897, 223.0287674909799875 ) ) ;
#52237=ADVANCED_FACE ( 'NONE', ( #34155 ), #94858, .F. ) ;
#52240=DIRECTION ( 'NONE',  ( -0.9536973892116009655, 0.1200132912778490019, -0.2757863298418440356 ) ) ;
#52241=CARTESIAN_POINT ( 'NONE',  ( -23.69628899429999791, 1410.235927737129941, 207.8525723050880174 ) ) ;
#52247=B_SPLINE_CURVE_WITH_KNOTS ( 'NONE', 3,
 ( #40444, #72965, #81337, #108755, #81891, #32047, #66236, #100355, #21418, #107658, #23643, #57825, #72425, #91951, #29844, #13024, #60029, #51616, #41563, #84097, #672, #102537, #24177, #93047, #94706, #83541, #85197, #17982, #58365, #8484, #58916, #75718, #6834, #75173, #94147, #109864, #16320, #76812, #34251, #128 ),
 .UNSPECIFIED., .F., .F.,
 ( 4, 3, 3, 3, 3, 3, 3, 3, 3, 3, 3, 3, 3, 4 ),
 ( -168.1723202510000021, -162.2888149943200062, -153.5620393927819975, -144.4833429881919926, -135.1231727132679907, -125.1025808913170039, -114.4147035693629988, -102.6255519937520120, -87.74092214761390096, -72.67910686651640617, -60.92308613310270005, -50.23111378371720548, -40.21016113735100816, -30.67014438050000535 ),
 .UNSPECIFIED. ) ;
#52248=CARTESIAN_POINT ( 'NONE',  ( 0.8327748425420000711, 1442.756953654829886, 150.7628527808980152 ) ) ;
#52251=CARTESIAN_POINT ( 'NONE',  ( -37.65047686723229958, 1442.773887284729881, 137.1096749952629921 ) ) ;
#52252=CARTESIAN_POINT ( 'NONE',  ( -22.16158675810000034, 1409.686960050029938, 210.4767810254680001 ) ) ;
#52254=CARTESIAN_POINT ( 'NONE',  ( 1.075780832630000017, 1414.392608856630204, 233.0977785888980236 ) ) ;
#52258=CARTESIAN_POINT ( 'NONE',  ( -1.775961533719359942, 1421.047340809089974, 184.1901329777589922 ) ) ;
#52259=EDGE_CURVE ( 'NONE', #76760, #86613, #95507, .T. ) ;
#52261=CARTESIAN_POINT ( 'NONE',  ( -4.254615091958411810, 1398.039996049444881, 221.4059216359357265 ) ) ;
#52262=CARTESIAN_POINT ( 'NONE',  ( -3.119330264448041845, 1440.523299896550043, 157.1480219251303367 ) ) ;
#52264=CARTESIAN_POINT ( 'NONE',  ( 1.443907308950000079, 1507.678956818529741, 236.8026632909979980 ) ) ;
#52267=CARTESIAN_POINT ( 'NONE',  ( 40.21518593132410047, 1445.085294981540073, 136.9476663967080015 ) ) ;
#52270=ORIENTED_EDGE ( 'NONE', *, *, #11395, .T. ) ;
#52271=CARTESIAN_POINT ( 'NONE',  ( 11.15310914653060159, 1434.045385467309870, 151.6482511736529943 ) ) ;
#52272=CARTESIAN_POINT ( 'NONE',  ( 27.56163678460000099, 1509.624398677929776, 215.4636615634079817 ) ) ;
#52273=ORIENTED_EDGE ( 'NONE', *, *, #34350, .T. ) ;
#52276=CARTESIAN_POINT ( 'NONE',  ( -2.500000000000000000, 1432.413060387330006, 146.1721969590979882 ) ) ;
#52277=CARTESIAN_POINT ( 'NONE',  ( 3.827327205999999649, 1424.046157813729906, 177.8294128217980017 ) ) ;
#52278=CARTESIAN_POINT ( 'NONE',  ( 11.16223122930000144, 1428.970455832429934, 101.8807690336980016 ) ) ;
#52279=CARTESIAN_POINT ( 'NONE',  ( 18.08978621609999848, 1507.814340215129732, 230.4555789890980009 ) ) ;
#52280=ADVANCED_FACE ( 'NONE', ( #17879 ), #101946, .F. ) ;
#52282=CARTESIAN_POINT ( 'NONE',  ( -2.576993086239999897, 1414.913060387329779, 192.9504896103979945 ) ) ;
#52283=CARTESIAN_POINT ( 'NONE',  ( 15.88129808800000120, 1409.969386305029957, 226.7471413913980030 ) ) ;
#52285=CARTESIAN_POINT ( 'NONE',  ( 13.73229811442000248, 1415.184612914949867, 197.5903291147609764 ) ) ;
#52289=CARTESIAN_POINT ( 'NONE',  ( 13.90221499949599959, 1436.238194080860012, 150.2928919302390227 ) ) ;
#52290=EDGE_CURVE ( 'NONE', #44146, #104880, #102090, .T. ) ;
#52292=ORIENTED_EDGE ( 'NONE', *, *, #58614, .T. ) ;
#52294=CARTESIAN_POINT ( 'NONE',  ( 12.70061752951238887, 1445.015675426939197, 169.4597949495606883 ) ) ;
#52298=B_SPLINE_CURVE_WITH_KNOTS ( 'NONE', 5,
 ( #54161, #105653, #2653, #70972, #98880, #79895, #55257, #13204, #106726 ),
 .UNSPECIFIED., .F., .F.,
 ( 6, 3, 6 ),
 ( 21.34408555294309906, 21.90163172499999789, 30.14216317859590077 ),
 .UNSPECIFIED. ) ;
#52300=CARTESIAN_POINT ( 'NONE',  ( -19.07368456369233556, 1442.271103625454771, 210.5520796240281811 ) ) ;
#52302=CARTESIAN_POINT ( 'NONE',  ( 4.244840198528499364, 1446.426887755389998, 161.9784992303009972 ) ) ;
#52304=CARTESIAN_POINT ( 'NONE',  ( 0.4675733539479999812, 1508.925830125129778, 238.6310950794979817 ) ) ;
#52308=CARTESIAN_POINT ( 'NONE',  ( 21.38805416096829859, 1440.913060387330006, 224.3727411978530029 ) ) ;
#52309=CARTESIAN_POINT ( 'NONE',  ( -19.59880086690000311, 1507.802454088529885, 229.4381582326980151 ) ) ;
#52313=CARTESIAN_POINT ( 'NONE',  ( -14.70465958249999971, 1409.593213617929905, 191.2178800344979948 ) ) ;
#52314=CARTESIAN_POINT ( 'NONE',  ( -24.34654694089999794, 1442.312289605810065, 211.4248143116180358 ) ) ;
#52316=ORIENTED_EDGE ( 'NONE', *, *, #83741, .T. ) ;
#52323=DIRECTION ( 'NONE',  ( -1.000000000000000000, 0.000000000000000000, 0.000000000000000000 ) ) ;
#52325=ADVANCED_FACE ( 'NONE', ( #60482 ), #36465, .T. ) ;
#52327=CARTESIAN_POINT ( 'NONE',  ( -20.84948682980000001, 1508.934641637929872, 190.2319761415980111 ) ) ;
#52328=CARTESIAN_POINT ( 'NONE',  ( 28.66654218860000114, 1509.598009363130132, 207.9792368166280028 ) ) ;
#52330=CARTESIAN_POINT ( 'NONE',  ( 14.44229455070000157, 1409.585625628630169, 192.0310987722980087 ) ) ;
#52331=CARTESIAN_POINT ( 'NONE',  ( -17.60921851184225417, 1486.151197990332548, 188.1605117022275522 ) ) ;
#52333=VERTEX_POINT ( 'NONE', #41874 ) ;
#52334=CARTESIAN_POINT ( 'NONE',  ( 33.33289073369999755, 1445.199364519750134, 248.0947902374979890 ) ) ;
#52336=CARTESIAN_POINT ( 'NONE',  ( -28.50728667541919847, 1509.908556774140152, 216.1167956888880042 ) ) ;
#52338=CARTESIAN_POINT ( 'NONE',  ( -8.364995774877499457, 1509.202158754189895, 236.9158755863900012 ) ) ;
#52339=ADVANCED_FACE ( 'NONE', ( #7715 ), #25048, .F. ) ;
#52340=CARTESIAN_POINT ( 'NONE',  ( -21.73553347590000229, 1452.603807136129944, 221.7739260095980001 ) ) ;
#52341=CARTESIAN_POINT ( 'NONE',  ( -3995.587774573430124, 778.1435722443549139, 210.2209376587489942 ) ) ;
#52342=CARTESIAN_POINT ( 'NONE',  ( 19.01828621289999788, 1456.631844032529898, 226.0087226235980040 ) ) ;
#52343=CARTESIAN_POINT ( 'NONE',  ( -8.301987938657498844, 1519.913060387329779, 185.0111222839169898 ) ) ;
#52345=VERTEX_POINT ( 'NONE', #110179 ) ;
#52347=CARTESIAN_POINT ( 'NONE',  ( 0.3357109459749999525, 1406.507447809929999, 269.4986534845979236 ) ) ;
#52351=B_SPLINE_CURVE_WITH_KNOTS ( 'NONE', 5,
 ( #29400, #63603, #52981, #36167, #35601, #19898, #55195, #70351, #46249, #89321, #54100, #103912 ),
 .UNSPECIFIED., .F., .F.,
 ( 6, 3, 3, 6 ),
 ( 0.000000000000000000, 0.2428673809476307177, 0.7286021428483020479, 1.000000000000000000 ),
 .UNSPECIFIED. ) ;
#52352=CARTESIAN_POINT ( 'NONE',  ( 13.09755946009999938, 1428.691652272130113, 223.5005393930979949 ) ) ;
#52353=( BOUNDED_CURVE ( )  B_SPLINE_CURVE ( 3, ( #4793, #37864, #55790, #71509 ),
 .UNSPECIFIED., .F., .F. ) 
 B_SPLINE_CURVE_WITH_KNOTS ( ( 4, 4 ),
 ( 4.712388980384758952, 7.353981633974552068 ),
 .UNSPECIFIED. ) 
 CURVE ( )  GEOMETRIC_REPRESENTATION_ITEM ( )  RATIONAL_B_SPLINE_CURVE ( ( 1.000000000000000000, 0.4982693061696819581, 0.4982693061696819581, 1.000000000000000000 ) ) 
 REPRESENTATION_ITEM ( '' )  );
#52355=CARTESIAN_POINT ( 'NONE',  ( -40.11829264410000206, 1445.561899567880118, 136.8687421407979912 ) ) ;
#52357=CARTESIAN_POINT ( 'NONE',  ( -40.53150014929950373, 1440.913060405800024, 260.0257716865519910 ) ) ;
#52358=CARTESIAN_POINT ( 'NONE',  ( 37.23777575920910721, 1449.393681520200289, 136.3086112982300335 ) ) ;
#52359=FACE_OUTER_BOUND ( 'NONE', #79400, .T. ) ;
#52364=ORIENTED_EDGE ( 'NONE', *, *, #43925, .T. ) ;
#52365=CARTESIAN_POINT ( 'NONE',  ( 2.424063131930000115, 1427.257651041929876, 147.9020499575979954 ) ) ;
#52368=CARTESIAN_POINT ( 'NONE',  ( 16.26863210207389798, 1486.460469297460122, 188.7573094889239940 ) ) ;
#52369=CARTESIAN_POINT ( 'NONE',  ( 11.43347548804394620, 1425.764712714644475, 138.9807451318896483 ) ) ;
#52372=CARTESIAN_POINT ( 'NONE',  ( 19.77969251879999746, 1507.818093401829856, 229.2755605921979907 ) ) ;
#52375=CARTESIAN_POINT ( 'NONE',  ( -17.36801834869999794, 1414.983773852829927, 207.7378529790379957 ) ) ;
#52377=CARTESIAN_POINT ( 'NONE',  ( 25.03889118680000081, 1435.391010761600000, 136.0112995284980002 ) ) ;
#52378=B_SPLINE_CURVE_WITH_KNOTS ( 'NONE', 5,
 ( #88183, #55697, #46196, #79790, #47275, #13090 ),
 .UNSPECIFIED., .F., .F.,
 ( 6, 6 ),
 ( 16.38547747492637896, 26.49451346759999737 ),
 .UNSPECIFIED. ) ;
#52379=CARTESIAN_POINT ( 'NONE',  ( -6.241370329288110419, 1396.131013841920094, 200.0124121438620080 ) ) ;
#52385=VERTEX_POINT ( 'NONE', #50832 ) ;
#52388=CARTESIAN_POINT ( 'NONE',  ( 11.00536806779999921, 1426.523248317530033, 91.15359103569791444 ) ) ;
#52391=CARTESIAN_POINT ( 'NONE',  ( 4.148789385605260449, 1424.601256096389989, 184.9569090508520048 ) ) ;
#52392=CARTESIAN_POINT ( 'NONE',  ( -2.861850767359648273, 1419.693532390741893, 186.1800267117334897 ) ) ;
#52395=FACE_OUTER_BOUND ( 'NONE', #50793, .T. ) ;
#52403=CARTESIAN_POINT ( 'NONE',  ( -2.654130549429999957E-10, 1472.045055685429816, 270.0713874941980066 ) ) ;
#52404=CARTESIAN_POINT ( 'NONE',  ( 12.53132851702783945, 1434.462080285801449, 147.2718985355009238 ) ) ;
#52405=CARTESIAN_POINT ( 'NONE',  ( -2.052286426879999848, 1486.111609172430008, 181.8527502747979838 ) ) ;
#52408=CARTESIAN_POINT ( 'NONE',  ( -2.500000000000000000, 1448.532394040329791, 160.1065257882549986 ) ) ;
#52410=CARTESIAN_POINT ( 'NONE',  ( 13.45819569170899932, 1408.065586298919925, 204.5788124947870017 ) ) ;
#52411=CARTESIAN_POINT ( 'NONE',  ( -8.399633448627239929, 1406.327446574869782, 268.4546571330000120 ) ) ;
#52412=CARTESIAN_POINT ( 'NONE',  ( -13.94839511594039827, 1435.086904260040001, 149.1659738623210103 ) ) ;
#52415=CARTESIAN_POINT ( 'NONE',  ( 13.55140343089999888, 1443.942093640929897, 188.2793544314979783 ) ) ;
#52425=CARTESIAN_POINT ( 'NONE',  ( 12.16691165299999966, 1415.934222462230082, 223.3923867161979899 ) ) ;
#52428=CARTESIAN_POINT ( 'NONE',  ( -28.82219086300000299, 1509.870558443830078, 205.6292521904379953 ) ) ;
#52433=CARTESIAN_POINT ( 'NONE',  ( -10.73514660131351839, 1424.973046421745494, 139.1354236205272343 ) ) ;
#52434=CARTESIAN_POINT ( 'NONE',  ( -11.97780009940000134, 1446.811541358570139, 187.5041657661979855 ) ) ;
#52437=CARTESIAN_POINT ( 'NONE',  ( 28.07142279780000038, 1508.133443489229876, 210.4694181319080144 ) ) ;
#52439=CARTESIAN_POINT ( 'NONE',  ( -24.25923418980000079, 1435.344651399380155, 136.2870029874980276 ) ) ;
#52440=B_SPLINE_CURVE_WITH_KNOTS ( 'NONE', 3,
 ( #6483, #5938, #74807, #40635, #5383, #99421, #49606, #100535, #40084, #99977, #23270, #91592, #92142, #15415, #7035, #41193, #14867, #23815, #83738, #109503, #32779, #58556, #92684, #47398, #60780, #59660, #60212, #94330, #75896, #8125, #41737, #864, #34989, #50693, #8671, #94904, #51244, #17608, #18179, #7582, #102186, #9251, #51809, #42291, #85950 ),
 .UNSPECIFIED., .F., .F.,
 ( 4, 2, 2, 2, 2, 2, 2, 2, 2, 2, 1, 1, 1, 2, 2, 1, 1, 1, 1, 2, 2, 1, 1, 2, 2, 2, 4 ),
 ( 0.000000000000000000, 0.06249999999996011524, 0.09374999999994189370, 0.1093749999999354128, 0.1249999999999289457, 0.1874999999999078792, 0.2187499999999010236, 0.2343749999998975542, 0.2499999999998940847, 0.3749999999998194777, 0.4374999999997830624, 0.4687499999997576938, 0.4843749999997514211, 0.4921874999997538080, 0.4999999999997561950, 0.6249999999998158140, 0.6874999999998389066, 0.7187499999998422373, 0.7343749999998510081, 0.7421874999998467892, 0.7499999999998425704, 0.8124999999998735456, 0.8437499999998785416, 0.8593749999998905320, 0.8749999999999025224, 0.9374999999999512612, 1.000000000000000000 ),
 .UNSPECIFIED. ) ;
#52444=CARTESIAN_POINT ( 'NONE',  ( -14.37531793339999986, 1420.438789880430022, 227.2666485765979871 ) ) ;
#52449=CARTESIAN_POINT ( 'NONE',  ( -4.220676207128734703, 1446.230049502166139, 170.5366217123670083 ) ) ;
#52450=CARTESIAN_POINT ( 'NONE',  ( -0.8368026584929999512, 1412.845967393029923, 233.2028161353979954 ) ) ;
#52455=CARTESIAN_POINT ( 'NONE',  ( 12.63018941866619826, 1435.203127805050144, 150.6492594472580038 ) ) ;
#52456=CARTESIAN_POINT ( 'NONE',  ( 18.29787016638390185, 1469.011283450069868, 228.3214042137699948 ) ) ;
#52457=CARTESIAN_POINT ( 'NONE',  ( -23.29055829209999828, 1509.739042671430070, 227.3452689062980028 ) ) ;
#52458=CARTESIAN_POINT ( 'NONE',  ( 0.000000000000000000, 1405.413060387330006, 209.1218459616979999 ) ) ;
#52466=CARTESIAN_POINT ( 'NONE',  ( -12.77667375843740061, 1416.535698381769862, 196.1064608229909823 ) ) ;
#52467=EDGE_CURVE ( 'NONE', #8321, #3400, #2432, .T. ) ;
#52476=DIRECTION ( 'NONE',  ( -0.9999176245050241940, -0.003057966218349585878, 0.01246567474455440375 ) ) ;
#52477=LINE ( 'NONE', #51917, #102170 ) ;
#52478=CARTESIAN_POINT ( 'NONE',  ( -18.44401098650000037, 1424.710439251030039, 225.1596812334979916 ) ) ;
#52480=CARTESIAN_POINT ( 'NONE',  ( -9.821550493440000196, 1443.913060387330006, 148.8455630174979945 ) ) ;
#52481=CARTESIAN_POINT ( 'NONE',  ( 16.49692068119999888, 1410.833576258530002, 191.6204761995979879 ) ) ;
#52485=ORIENTED_EDGE ( 'NONE', *, *, #32935, .T. ) ;
#52486=CARTESIAN_POINT ( 'NONE',  ( 1.421471772691550006, 1507.619497824060090, 186.1880827579659865 ) ) ;
#52487=CARTESIAN_POINT ( 'NONE',  ( 23.63745125559999849, 1430.455784058630115, 206.9473789965179833 ) ) ;
#52488=CARTESIAN_POINT ( 'NONE',  ( -24.60733038660000105, 1437.330089494700132, 210.5677010675179872 ) ) ;
#52489=CARTESIAN_POINT ( 'NONE',  ( 6.366883779533799803, 1410.509502214471695, 186.8986137100159794 ) ) ;
#52494=CARTESIAN_POINT ( 'NONE',  ( 13.13054719219040045, 1414.913526854310021, 198.0719216339290085 ) ) ;
#52497=CARTESIAN_POINT ( 'NONE',  ( 6.232532001850000114, 1398.098440471829917, 220.5304192662980256 ) ) ;
#52498=CARTESIAN_POINT ( 'NONE',  ( -23.17538855434040101, 1409.994298099240268, 210.0642958403453235 ) ) ;
#52501=CARTESIAN_POINT ( 'NONE',  ( -18.04763499721657993, 1459.633086045522305, 228.0005121999546986 ) ) ;
#52503=CARTESIAN_POINT ( 'NONE',  ( 20.36394027541210150, 1509.531394767829852, 230.2454094804139970 ) ) ;
#52506=CARTESIAN_POINT ( 'NONE',  ( 14.26589412800000112, 1443.159997941379970, 189.6457918547979773 ) ) ;
#52508=CARTESIAN_POINT ( 'NONE',  ( 39.80925673091419981, 1441.186665741440038, 136.8465300712809949 ) ) ;
#52509=CARTESIAN_POINT ( 'NONE',  ( 15.61002862346814268, 1412.588789359010207, 269.3672926532146334 ) ) ;
#52510=CARTESIAN_POINT ( 'NONE',  ( -44.59183195640000008, 1449.238671483380131, 266.2372565378979630 ) ) ;
#52514=CARTESIAN_POINT ( 'NONE',  ( -20.04281941989999893, 1485.210412383429912, 191.3717997072980097 ) ) ;
#52515=CARTESIAN_POINT ( 'NONE',  ( 1.811394514909999920, 1409.481637553129985, 185.5992571243980080 ) ) ;
#52516=CARTESIAN_POINT ( 'NONE',  ( 5.031185190540000463, 1423.053909769329948, 184.8938659814980099 ) ) ;
#52517=CARTESIAN_POINT ( 'NONE',  ( -9.894253967190000054, 1435.855537208829901, 152.5794184983980131 ) ) ;
#52518=CARTESIAN_POINT ( 'NONE',  ( -2.500000000000000000, 1440.913060387330006, 137.0999999980979851 ) ) ;
#52520=CARTESIAN_POINT ( 'NONE',  ( -3.105266140399999930, 1452.658929098130102, 153.4127541622980004 ) ) ;
#52525=CARTESIAN_POINT ( 'NONE',  ( -41.37369176849999519, 1449.696618274529783, 270.1889136745979840 ) ) ;
#52527=FACE_OUTER_BOUND ( 'NONE', #31270, .T. ) ;
#52530=CARTESIAN_POINT ( 'NONE',  ( 2.882600136576499938, 1409.337436188870015, 231.1024624802110168 ) ) ;
#52532=CARTESIAN_POINT ( 'NONE',  ( -4.504634474840000458, 1417.895784275830010, 234.4460694219980041 ) ) ;
#52533=DIRECTION ( 'NONE',  ( -0.7074300732359156685, -0.02470400251506888953, -0.7063514732349346348 ) ) ;
#52535=CARTESIAN_POINT ( 'NONE',  ( -45.66135036215970189, 1437.717918248189790, 268.7621968117340430 ) ) ;
#52536=CARTESIAN_POINT ( 'NONE',  ( -2.500000000000000000, 1434.141256042250006, 183.7754221751980026 ) ) ;
#52540=ORIENTED_EDGE ( 'NONE', *, *, #16548, .T. ) ;
#52543=CARTESIAN_POINT ( 'NONE',  ( 19.29437764624872642, 1456.521983837815696, 224.7265922325017300 ) ) ;
#52547=B_SPLINE_SURFACE_WITH_KNOTS ( 'NONE', 5, 5, ( 
 ( #79308, #80408, #3721, #18266, #96659, #87717 ),
 ( #28900, #54677, #94998, #2619, #36745, #88255 ),
 ( #54128, #27789, #70938, #3171, #105054, #37853 ),
 ( #45724, #88803, #103942, #1500, #28343, #79861 ),
 ( #61421, #95544, #35631, #12086, #62539, #69824 ),
 ( #44608, #20466, #37303, #72038, #44049, #27240 ) ),
 .UNSPECIFIED., .F., .F., .F.,
 ( 6, 6 ),
 ( 6, 6 ),
 ( 4.505366048469999996, 5.371483694130000153 ),
 ( 0.000000000000000000, 1.435063413269999977 ),
 .UNSPECIFIED. ) ;
#52549=CARTESIAN_POINT ( 'NONE',  ( -15.64624339300000067, 1506.809279316930088, 193.6024923478979929 ) ) ;
#52552=CARTESIAN_POINT ( 'NONE',  ( 11.60004869885203682, 1422.222932908421853, 135.5999999980979851 ) ) ;
#52557=CARTESIAN_POINT ( 'NONE',  ( -0.5972104939277330660, 1409.781079465039966, 270.0713840979290126 ) ) ;
#52560=CARTESIAN_POINT ( 'NONE',  ( 7.944617962720000648, 1417.384938173330056, 230.8476712041980079 ) ) ;
#52561=CARTESIAN_POINT ( 'NONE',  ( -0.2669961437037675078, 1507.379266396976391, 237.3398728226291894 ) ) ;
#52564=ORIENTED_EDGE ( 'NONE', *, *, #29192, .T. ) ;
#52565=CARTESIAN_POINT ( 'NONE',  ( -23.44004119578789869, 1410.414350826220016, 210.3440813114680168 ) ) ;
#52566=CARTESIAN_POINT ( 'NONE',  ( -4.031755536680000418, 1424.742300799430041, 185.9020548737979937 ) ) ;
#52567=CARTESIAN_POINT ( 'NONE',  ( 3.648661080172654891, 1424.949000758327884, 184.9096943055786255 ) ) ;
#52569=CARTESIAN_POINT ( 'NONE',  ( -20.23041878443079966, 1482.171314072119912, 192.9891252425980213 ) ) ;
#52570=CARTESIAN_POINT ( 'NONE',  ( -20.07551605200000111, 1420.830474780429995, 221.7733367695979894 ) ) ;
#52571=ADVANCED_FACE ( 'NONE', ( #36791 ), #76031, .F. ) ;
#52572=CARTESIAN_POINT ( 'NONE',  ( 39.35319033365500019, 1459.582669346870034, 267.8286354669800176 ) ) ;
#52573=CARTESIAN_POINT ( 'NONE',  ( -8.779614049866278691, 1465.164895044473724, 232.9239790886660160 ) ) ;
#52574=CARTESIAN_POINT ( 'NONE',  ( -16.62457289494420110, 1421.497728909477473, 226.9554053466772814 ) ) ;
#52576=ORIENTED_EDGE ( 'NONE', *, *, #94421, .F. ) ;
#52578=CARTESIAN_POINT ( 'NONE',  ( 1.476609825382830143, 1480.675250368899924, 182.2662939368339892 ) ) ;
#52580=CARTESIAN_POINT ( 'NONE',  ( 23.86968260200000103, 1411.113062188429922, 208.1586362411949835 ) ) ;
#52583=CARTESIAN_POINT ( 'NONE',  ( 26.27737804779999919, 1451.834422488929931, 135.7154755371979888 ) ) ;
#52584=EDGE_CURVE ( 'NONE', #6013, #62471, #110666, .T. ) ;
#52588=CARTESIAN_POINT ( 'NONE',  ( 17.09517797430000030, 1409.510037156830094, 194.7435863138979926 ) ) ;
#52590=CARTESIAN_POINT ( 'NONE',  ( 18.64337105059429689, 1444.324653571830140, 162.1710875046050830 ) ) ;
#52591=CARTESIAN_POINT ( 'NONE',  ( 2.499999945294461678, 1439.622149924839277, 182.9152359685302827 ) ) ;
#52592=CARTESIAN_POINT ( 'NONE',  ( 0.3620268206439999914, 1416.991477563229864, 234.1672957265980131 ) ) ;
#52593=CARTESIAN_POINT ( 'NONE',  ( -19.70148083128903238, 1425.942341657287670, 223.0221936444421829 ) ) ;
#52594=CARTESIAN_POINT ( 'NONE',  ( 1.228127824989470041, 1450.757128850169920, 181.5372027678210145 ) ) ;
#52597=CARTESIAN_POINT ( 'NONE',  ( 3.043251597425320032, 1417.779699503100119, 234.3208248802520188 ) ) ;
#52598=ORIENTED_EDGE ( 'NONE', *, *, #77429, .T. ) ;
#52600=DIRECTION ( 'NONE',  ( 0.000000000000000000, 0.000000000000000000, 1.000000000000000000 ) ) ;
#52601=CARTESIAN_POINT ( 'NONE',  ( -0.5149987733311249816, 1410.090151802530045, 233.1456135000190102 ) ) ;
#52604=CARTESIAN_POINT ( 'NONE',  ( -0.09512347170599190493, 1506.606278694979437, 231.2494356483143747 ) ) ;
#52605=CARTESIAN_POINT ( 'NONE',  ( -5.969073325650000150, 1453.512197679029896, 209.1218459616979999 ) ) ;
#52607=CARTESIAN_POINT ( 'NONE',  ( 11.12882730979999835, 1433.637661252139878, 151.6637046936980084 ) ) ;
#52608=CARTESIAN_POINT ( 'NONE',  ( 24.08292308420000083, 1450.076351702270131, 243.9198229606980135 ) ) ;
#52609=CARTESIAN_POINT ( 'NONE',  ( 24.89297638757900089, 1440.913060396979972, 215.3507704242990144 ) ) ;
#52613=CARTESIAN_POINT ( 'NONE',  ( 24.32116265780000219, 1435.530952642309785, 137.6072328918980077 ) ) ;
#52614=CARTESIAN_POINT ( 'NONE',  ( 22.71503220009999779, 1409.706269051729805, 209.0936436305159987 ) ) ;
#52616=FACE_OUTER_BOUND ( 'NONE', #98286, .T. ) ;
#52617=CARTESIAN_POINT ( 'NONE',  ( 25.75587219230000002, 1449.806259868670168, 209.4579355261629985 ) ) ;
#52620=CARTESIAN_POINT ( 'NONE',  ( 26.63291560383849799, 1436.743680851771842, 136.7889385594793055 ) ) ;
#52625=CARTESIAN_POINT ( 'NONE',  ( 0.1595995995380000143, 1486.508831850330125, 181.8147405652979671 ) ) ;
#52631=CARTESIAN_POINT ( 'NONE',  ( -38.20286890324609885, 1450.309401038109854, 134.0999999984079807 ) ) ;
#52634=ORIENTED_EDGE ( 'NONE', *, *, #22156, .F. ) ;
#52638=CARTESIAN_POINT ( 'NONE',  ( -2.683679964788079353, 1509.031199887366938, 238.5977189156948555 ) ) ;
#52639=CARTESIAN_POINT ( 'NONE',  ( 22.83133757149967380, 1409.745586299351999, 208.5326685875802752 ) ) ;
#52642=CARTESIAN_POINT ( 'NONE',  ( 14.24559479254840078, 1409.410527519360130, 204.6418239650080011 ) ) ;
#52643=CARTESIAN_POINT ( 'NONE',  ( 8.970106519850705951, 1421.589190746440181, 137.0999999980978146 ) ) ;
#52645=CARTESIAN_POINT ( 'NONE',  ( -17.00560698389999814, 1410.862957975729842, 191.9516635397980053 ) ) ;
#52647=ORIENTED_EDGE ( 'NONE', *, *, #8986, .F. ) ;
#52653=CARTESIAN_POINT ( 'NONE',  ( 24.68678492890000342, 1508.521768884430230, 220.7077148987980024 ) ) ;
#52656=CARTESIAN_POINT ( 'NONE',  ( 32.06156897976659792, 1460.613316927345750, 269.4940338796959054 ) ) ;
#52658=CARTESIAN_POINT ( 'NONE',  ( 19.38237504630382091, 1439.882993612299288, 212.4558745127706914 ) ) ;
#52659=CARTESIAN_POINT ( 'NONE',  ( 18.64672481363430379, 1416.851343896850040, 209.6839434896919840 ) ) ;
#52661=CARTESIAN_POINT ( 'NONE',  ( -20.37004171859861401, 1507.842607393826938, 228.6074707356000602 ) ) ;
#52664=CARTESIAN_POINT ( 'NONE',  ( -16.06782005780000233, 1459.209651374430223, 230.7189234877979800 ) ) ;
#52668=B_SPLINE_SURFACE_WITH_KNOTS ( 'NONE', 5, 5, ( 
 ( #87809, #80501, #87239, #29529, #106243, #27323, #95635, #11094, #10528, #12177, #63719, #62064, #36277, #46366, #20558, #54761, #54218, #88891, #11634, #45812, #78851, #53665, #97829, #104588, #69917, #27883, #96191 ),
 ( #37947, #3262, #19465, #45261, #79396, #1591, #2710, #36834, #28993, #71024, #105145, #62634, #3819, #96753, #37388, #72128, #105711, #55309, #89443, #12735, #78279, #22754, #5436, #100584, #13810, #46917, #81574 ),
 ( #5987, #64263, #72655, #40690, #91642, #106782, #21658, #39020, #30073, #14367, #100034, #98387, #99474, #38478, #39593, #31729, #56958, #89987, #73197, #55866, #40135, #107342, #107888, #13260, #74319, #73765, #47450 ),
 ( #4877, #30638, #90534, #47996, #109007, #64824, #56402, #49110, #98932, #32292, #74863, #22206, #82133, #31179, #65368, #14918, #66476, #91085, #48561, #82697, #108449, #57518, #65916, #23866, #23325, #83244, #6538 ),
 ( #58060, #92194, #81038, #4349, #25517, #17661, #59170, #51862, #93289, #110646, #8173, #69219, #75418, #59711, #32827, #109556, #41788, #68671, #8726, #67018, #103329, #85998, #51292, #94380, #110098, #26636, #17099 ),
 ( #26066, #33932, #16552, #35041, #68129, #9297, #43460, #60261, #93824, #77608, #77062, #916, #60832, #85426, #15467, #42905, #49660, #83795, #33373, #371, #16015, #7089, #34496, #75946, #67567, #50742, #41245 ) ),
 .UNSPECIFIED., .F., .F., .F.,
 ( 6, 6 ),
 ( 6, 3, 3, 3, 3, 3, 3, 3, 6 ),
 ( 1.704359124380000035, 76.86370920020000597 ),
 ( 27.73790463739999979, 34.20638505209999636, 36.61973048189999957, 37.82640319669999940, 38.42973955419999754, 39.03307591160000101, 39.44352330040000254, 39.85397068919999697, 40.67486546690000182 ),
 .UNSPECIFIED. ) ;
#52670=CARTESIAN_POINT ( 'NONE',  ( 13.58245579929999991, 1416.835809767730098, 196.3346082735980076 ) ) ;
#52673=CARTESIAN_POINT ( 'NONE',  ( -33.91369265678890343, 1437.010538859309918, 136.5611844326260211 ) ) ;
#52676=CARTESIAN_POINT ( 'NONE',  ( -20.10054294789999929, 1449.792076513850134, 195.1552221568979917 ) ) ;
#52677=CARTESIAN_POINT ( 'NONE',  ( -11.55021905039999908, 1426.818422250529920, 130.8136715980980114 ) ) ;
#52678=CARTESIAN_POINT ( 'NONE',  ( 16.14453601094659874, 1409.476838033949889, 193.1642425871669957 ) ) ;
#52682=CARTESIAN_POINT ( 'NONE',  ( -19.70612301839999958, 1434.996842494430211, 207.5825951959979818 ) ) ;
#52683=CARTESIAN_POINT ( 'NONE',  ( -34.48978217860000228, 1440.913060385029894, 250.0021841876980488 ) ) ;
#52688=CARTESIAN_POINT ( 'NONE',  ( 33.12914038030000086, 1450.467761070830193, 136.2685675544979915 ) ) ;
#52690=CARTESIAN_POINT ( 'NONE',  ( 11.13883711037720126, 1398.243429064360271, 216.8406632416929938 ) ) ;
#52692=CARTESIAN_POINT ( 'NONE',  ( -17.07358046210000069, 1458.578126118629825, 230.5958457830979853 ) ) ;
#52693=VERTEX_POINT ( 'NONE', #6352 ) ;
#52697=VERTEX_POINT ( 'NONE', #39954 ) ;
#52698=CARTESIAN_POINT ( 'NONE',  ( -0.7127565730050000603, 1412.056601978030130, 185.0301737879979953 ) ) ;
#52699=CARTESIAN_POINT ( 'NONE',  ( 9.750569994704919807, 1446.597750952001888, 153.4809583364809384 ) ) ;
#52700=VECTOR ( 'NONE', #110158, 1000.000000000000227 ) ;
#52703=CARTESIAN_POINT ( 'NONE',  ( -0.3989523678029999743, 1461.200148461630079, 235.3477028770979871 ) ) ;
#52711=CARTESIAN_POINT ( 'NONE',  ( 11.84182917021260018, 1430.667802097110098, 149.7263372980079907 ) ) ;
#52712=CARTESIAN_POINT ( 'NONE',  ( 12.88207677529630502, 1444.943664110688587, 186.6979557653219501 ) ) ;
#52713=ORIENTED_EDGE ( 'NONE', *, *, #58849, .F. ) ;
#52715=EDGE_CURVE ( 'NONE', #38044, #100575, #74127, .T. ) ;
#52719=CARTESIAN_POINT ( 'NONE',  ( -5.969328413430000424, 1422.018310919130045, 186.6257062000979943 ) ) ;
#52720=CARTESIAN_POINT ( 'NONE',  ( 1.423691709839809860, 1409.795502070599923, 270.0714555743300025 ) ) ;
#52725=CARTESIAN_POINT ( 'NONE',  ( 0.02716074563118510421, 1410.223742506766712, 233.2171245275475542 ) ) ;
#52728=CARTESIAN_POINT ( 'NONE',  ( -4.586155245401363878, 1423.742087943514889, 184.4069333355399181 ) ) ;
#52729=CARTESIAN_POINT ( 'NONE',  ( 17.87507678963179814, 1419.602358105800022, 225.0615382930280077 ) ) ;
#52730=CARTESIAN_POINT ( 'NONE',  ( -5.412016405372058969, 1422.582238247259966, 129.2850280054269945 ) ) ;
#52732=CARTESIAN_POINT ( 'NONE',  ( 6.438546668639999915, 1410.951844103429949, 268.3665355202980436 ) ) ;
#52741=CARTESIAN_POINT ( 'NONE',  ( -15.57748978299999898, 1507.212883763329955, 192.6976421578980023 ) ) ;
#52742=CARTESIAN_POINT ( 'NONE',  ( -11.15490121449999883, 1425.160561550830153, 144.1688093937980000 ) ) ;
#52743=DIRECTION ( 'NONE',  ( 1.000000000000000000, 0.000000000000000000, 0.000000000000000000 ) ) ;
#52744=CARTESIAN_POINT ( 'NONE',  ( -4.155670335940000015, 1439.704322206689994, 185.4969475932980174 ) ) ;
#52748=CARTESIAN_POINT ( 'NONE',  ( 13.43806146769999899, 1412.741207332130216, 228.4219197481980075 ) ) ;
#52751=CARTESIAN_POINT ( 'NONE',  ( -16.32193376780000094, 1459.453084261929916, 228.9511341082980209 ) ) ;
#52753=CARTESIAN_POINT ( 'NONE',  ( 30.03438762969999942, 1414.561137273029999, 268.9518563996979879 ) ) ;
#52755=CARTESIAN_POINT ( 'NONE',  ( 1.430288155006089523, 1465.025930583076388, 237.8691320678095167 ) ) ;
#52756=CARTESIAN_POINT ( 'NONE',  ( 20.75570910649999590, 1488.585678912729918, 191.6580715406979891 ) ) ;
#52757=CARTESIAN_POINT ( 'NONE',  ( 19.47833342507072274, 1506.473666147355971, 219.3888140167584027 ) ) ;
#52761=CARTESIAN_POINT ( 'NONE',  ( -1.598721155459999993E-13, 1416.913060387330006, 198.3331309146979891 ) ) ;
#52763=CARTESIAN_POINT ( 'NONE',  ( -13.45510625179999842, 1442.037881746980020, 188.3676330511979984 ) ) ;
#52765=CARTESIAN_POINT ( 'NONE',  ( -29.18335203569999692, 1435.678379713110189, 136.0914706953979874 ) ) ;
#52769=CARTESIAN_POINT ( 'NONE',  ( -13.17055926657740095, 1409.372986451539873, 202.0656305217389956 ) ) ;
#52773=CARTESIAN_POINT ( 'NONE',  ( -42.46955762170000526, 1456.102617841730080, 267.1011643380979876 ) ) ;
#52775=CARTESIAN_POINT ( 'NONE',  ( 0.1712859756662860056, 1420.019041673809852, 183.9765777425620001 ) ) ;
#52777=CARTESIAN_POINT ( 'NONE',  ( 18.31963684070830212, 1421.106839041940020, 223.3124397329580120 ) ) ;
#52780=CARTESIAN_POINT ( 'NONE',  ( 16.76434746429979938, 1422.577036823120125, 227.0063948903039943 ) ) ;
#52781=CARTESIAN_POINT ( 'NONE',  ( 15.56083348049999948, 1415.425433635630043, 217.3404540485179837 ) ) ;
#52782=CARTESIAN_POINT ( 'NONE',  ( -28.26734827197039834, 1508.339354041070010, 208.8484260271879975 ) ) ;
#52783=DIRECTION ( 'NONE',  ( 0.000000000000000000, 1.000000000000000000, 0.000000000000000000 ) ) ;
#52785=CARTESIAN_POINT ( 'NONE',  ( -7.811850951430000300, 1508.423641399529970, 181.5011841995979864 ) ) ;
#52787=CARTESIAN_POINT ( 'NONE',  ( -23.47537152620000356, 1410.228075751530014, 207.0042901657579932 ) ) ;
#52790=CARTESIAN_POINT ( 'NONE',  ( 15.03806483009999972, 1414.913060387229962, 201.9300244649979845 ) ) ;
#52795=CARTESIAN_POINT ( 'NONE',  ( -12.68266539220000055, 1434.593723365520191, 149.3604887061979696 ) ) ;
#52796=EDGE_CURVE ( 'NONE', #59575, #94675, #101317, .T. ) ;
#52800=CARTESIAN_POINT ( 'NONE',  ( -22.65427071730000108, 1411.066072191229750, 211.5467506970180125 ) ) ;
#52802=CARTESIAN_POINT ( 'NONE',  ( 1.358317420979999968, 1411.681908635930085, 232.6968902729979902 ) ) ;
#52805=SPHERICAL_SURFACE ( 'NONE', #31811, 2.000000000000000000 ) ;
#52806=CARTESIAN_POINT ( 'NONE',  ( -0.6083677694837460459, 1420.015852375959867, 184.4634389772880070 ) ) ;
#52808=CARTESIAN_POINT ( 'NONE',  ( -3.761263762889859752, 1398.025418639840154, 221.5750308120653074 ) ) ;
#52810=CARTESIAN_POINT ( 'NONE',  ( -14.59402636152660016, 1485.278995523290178, 186.7907175241479933 ) ) ;
#52811=CARTESIAN_POINT ( 'NONE',  ( -18.20455311950000166, 1430.274367750729880, 193.6929569324979923 ) ) ;
#52813=CARTESIAN_POINT ( 'NONE',  ( 41.65411205771810188, 1444.066986349939953, 136.1144878563849829 ) ) ;
#52817=CARTESIAN_POINT ( 'NONE',  ( 11.35222491904410091, 1434.076906344789904, 151.4872001750849790 ) ) ;
#52824=CARTESIAN_POINT ( 'NONE',  ( 13.42479616400980014, 1453.338203267170002, 224.7140346886050111 ) ) ;
#52825=CARTESIAN_POINT ( 'NONE',  ( -0.3602478992429999916, 1417.265131029429995, 235.9082177996980079 ) ) ;
#52827=CARTESIAN_POINT ( 'NONE',  ( 0.3235747208499999972, 1507.644137708130074, 180.9006323824980029 ) ) ;
#52829=CARTESIAN_POINT ( 'NONE',  ( -24.05569699374110115, 1444.796293269080024, 211.9644565330009982 ) ) ;
#52831=EDGE_CURVE ( 'NONE', #14771, #8790, #47260, .T. ) ;
#52832=CARTESIAN_POINT ( 'NONE',  ( 36.31760351622449434, 1436.138747408989957, 134.0999999970809995 ) ) ;
#52837=VERTEX_POINT ( 'NONE', #38840 ) ;
#52838=CARTESIAN_POINT ( 'NONE',  ( 13.90627238822369804, 1435.005108322179922, 148.8090833361299872 ) ) ;
#52842=EDGE_CURVE ( 'NONE', #5765, #45814, #78556, .T. ) ;
#52846=CARTESIAN_POINT ( 'NONE',  ( 22.71382099334196525, 1450.890321816409596, 142.2309692183697223 ) ) ;
#52849=ADVANCED_FACE ( 'NONE', ( #101485 ), #67102, .T. ) ;
#52850=CARTESIAN_POINT ( 'NONE',  ( -19.08445480129999794, 1440.913060387330006, 209.8212738029720299 ) ) ;
#52852=CARTESIAN_POINT ( 'NONE',  ( 4.288402489466680123, 1446.931632216600065, 155.2279950395780190 ) ) ;
#52855=ORIENTED_EDGE ( 'NONE', *, *, #85022, .F. ) ;
#52856=CARTESIAN_POINT ( 'NONE',  ( 30.44909158939109872, 1440.913060387330006, 253.0088576829679994 ) ) ;
#52858=CARTESIAN_POINT ( 'NONE',  ( -18.25434091379999657, 1509.489596267130310, 186.0409464828979935 ) ) ;
#52860=CARTESIAN_POINT ( 'NONE',  ( 27.00209765840460108, 1448.139277255909747, 136.8875338484010058 ) ) ;
#52861=CARTESIAN_POINT ( 'NONE',  ( -14.20408294209999944, 1409.911027547829917, 190.5440136396979938 ) ) ;
#52862=CARTESIAN_POINT ( 'NONE',  ( -24.31663051820000021, 1442.649873241249907, 211.4598721613180032 ) ) ;
#52863=CARTESIAN_POINT ( 'NONE',  ( -10.79382126600000014, 1414.913060387329779, 196.1395803457980094 ) ) ;
#52864=CARTESIAN_POINT ( 'NONE',  ( 16.81223453394349932, 1414.913060391199906, 210.6693087035600058 ) ) ;
#52865=CARTESIAN_POINT ( 'NONE',  ( 26.87832337146859629, 1441.334257626130011, 137.4807418192719979 ) ) ;
#52866=CARTESIAN_POINT ( 'NONE',  ( -13.50070407659999994, 1434.968958018969943, 149.9809230438979739 ) ) ;
#52871=CARTESIAN_POINT ( 'NONE',  ( 23.69134289970000395, 1410.129789027929974, 209.5325461888999996 ) ) ;
#52873=CARTESIAN_POINT ( 'NONE',  ( 28.09993147489999998, 1509.169756330429891, 207.7492410536980003 ) ) ;
#52876=EDGE_CURVE ( 'NONE', #13362, #44739, #61749, .T. ) ;
#52880=ORIENTED_EDGE ( 'NONE', *, *, #82507, .F. ) ;
#52881=CARTESIAN_POINT ( 'NONE',  ( 13.69365045770000044, 1462.915760504130049, 238.2645948893979835 ) ) ;
#52884=CARTESIAN_POINT ( 'NONE',  ( -5.749669252027449495, 1509.117800599190105, 238.0245596231779928 ) ) ;
#52885=CARTESIAN_POINT ( 'NONE',  ( -19.16951723229999871, 1456.627470220629903, 228.8719212425980061 ) ) ;
#52886=ADVANCED_FACE ( 'NONE', ( #35976 ), #62440, .F. ) ;
#52887=CARTESIAN_POINT ( 'NONE',  ( 10.97596755329999851, 1432.730980201519969, 151.7698537367980123 ) ) ;
#52888=CARTESIAN_POINT ( 'NONE',  ( 17.91001729305950008, 1410.383396254900163, 222.9072237126829918 ) ) ;
#52889=CARTESIAN_POINT ( 'NONE',  ( 0.1679668313380000000, 1470.808655612629764, 188.5134246798980087 ) ) ;
#52891=EDGE_LOOP ( 'NONE', ( #6861, #8490, #40001, #79850, #49069 ) ) ;
#52893=CARTESIAN_POINT ( 'NONE',  ( 0.2153512683669999983, 1405.989301470729970, 266.9611412585979906 ) ) ;
#52894=CARTESIAN_POINT ( 'NONE',  ( 28.29497430790000223, 1509.672356515530055, 207.2299602969580121 ) ) ;
#52895=AXIS2_PLACEMENT_3D ( 'NONE', #41446, #75611, #109741 ) ;
#52896=CARTESIAN_POINT ( 'NONE',  ( 43.37196902965609979, 1452.013348346279827, 269.7132147777479645 ) ) ;
#52897=CARTESIAN_POINT ( 'NONE',  ( -24.04686560566315023, 1437.475348716183362, 212.2910028660378998 ) ) ;
#52898=CARTESIAN_POINT ( 'NONE',  ( -39.24082110814379831, 1450.608897959999922, 136.0275758983839864 ) ) ;
#52901=EDGE_CURVE ( 'NONE', #96609, #56358, #21197, .T. ) ;
#52902=CARTESIAN_POINT ( 'NONE',  ( 37.34923688015930310, 1449.321946719639982, 136.3170601122349979 ) ) ;
#52913=CARTESIAN_POINT ( 'NONE',  ( -0.3001262975330000193, 1417.357112613329946, 235.2038291758979938 ) ) ;
#52920=CARTESIAN_POINT ( 'NONE',  ( 26.26971730801799865, 1435.434881028299969, 135.5857965276559867 ) ) ;
#52924=CARTESIAN_POINT ( 'NONE',  ( -16.14700684228250083, 1409.476921796170018, 225.0741814793740332 ) ) ;
#52931=CARTESIAN_POINT ( 'NONE',  ( 10.36044274480000027, 1425.414401215230100, 93.45973651769790536 ) ) ;
#52939=CARTESIAN_POINT ( 'NONE',  ( 3.439533802020000142, 1449.329777843420061, 184.0645408312979896 ) ) ;
#52941=ADVANCED_FACE ( 'NONE', ( #21337 ), #50119, .T. ) ;
#52942=DIRECTION ( 'NONE',  ( -1.987342477590000096E-13, 6.939952856120000821E-15, 1.000000000000000000 ) ) ;
#52944=ORIENTED_EDGE ( 'NONE', *, *, #31563, .T. ) ;
#52946=CARTESIAN_POINT ( 'NONE',  ( -41.65407267460000185, 1444.067062105530113, 136.1145731928979785 ) ) ;
#52947=CIRCLE ( 'NONE', #4660, 1.999994602477440653 ) ;
#52949=DIRECTION ( 'NONE',  ( 0.000000000000000000, -1.000000000000000000, 0.000000000000000000 ) ) ;
#52951=CARTESIAN_POINT ( 'NONE',  ( -1.316513911440000184, 1486.231707541229980, 181.7543151367980272 ) ) ;
#52952=CARTESIAN_POINT ( 'NONE',  ( 20.58555848629999829, 1507.839439013330093, 189.9311647047979932 ) ) ;
#52954=CARTESIAN_POINT ( 'NONE',  ( 22.55885583319999910, 1410.621632374630053, 206.4601081238480162 ) ) ;
#52956=CARTESIAN_POINT ( 'NONE',  ( 33.91368255268339738, 1435.681798330320134, 135.0664145109430194 ) ) ;
#52957=CARTESIAN_POINT ( 'NONE',  ( 27.32008277287192755, 1435.451596658461540, 135.2710114260797809 ) ) ;
#52958=CARTESIAN_POINT ( 'NONE',  ( 15.07167880837459961, 1409.439375008719935, 204.0198465041329996 ) ) ;
#52959=CARTESIAN_POINT ( 'NONE',  ( 5.661443424597549908E-05, 1405.842742645599856, 267.2348689328309774 ) ) ;
#52960=B_SPLINE_CURVE_WITH_KNOTS ( 'NONE', 3,
 ( #88167, #28805, #21467, #63002, #97110, #45631, #11455, #20376, #54581, #88716, #11996, #80309, #3625, #89797, #78653, #22557, #5809, #48926, #24230, #65717, #30441, #83054, #6347, #48368, #39949, #32099, #73012, #100934, #15275, #74121, #58415, #99837, #13616, #41044, #108250, #57871, #49468, #83588, #23129, #32651, #73575, #109374, #23686 ),
 .UNSPECIFIED., .F., .F.,
 ( 4, 3, 3, 3, 3, 3, 3, 3, 3, 3, 3, 3, 3, 3, 4 ),
 ( 9.298193603555128917, 10.98315671184179898, 12.97260628368140090, 15.05249941581099904, 16.75275777422749712, 18.32915130324699859, 19.75511727758679825, 19.90554483226650007, 21.13603391183419689, 22.44647941495799870, 23.82709552150320320, 25.30707762746569500, 27.06563981043629497, 29.15018126801379594, 30.45919393759999849 ),
 .UNSPECIFIED. ) ;
#52961=CARTESIAN_POINT ( 'NONE',  ( -14.11277764225159892, 1435.081315985899892, 149.0355979864779954 ) ) ;
#52962=ORIENTED_EDGE ( 'NONE', *, *, #63596, .F. ) ;
#52964=CARTESIAN_POINT ( 'NONE',  ( 13.97694847940000074, 1444.778227271800006, 189.3186977499980230 ) ) ;
#52965=ORIENTED_EDGE ( 'NONE', *, *, #9653, .T. ) ;
#52966=EDGE_CURVE ( 'NONE', #81429, #82793, #30555, .T. ) ;
#52967=EDGE_LOOP ( 'NONE', ( #51816, #21636, #97472, #60833 ) ) ;
#52979=CARTESIAN_POINT ( 'NONE',  ( -29.12655649119999879, 1509.869978475729795, 207.5400152816580146 ) ) ;
#52980=CARTESIAN_POINT ( 'NONE',  ( -0.5955487639629999386, 1497.701650616130109, 231.3320226370980208 ) ) ;
#52981=CARTESIAN_POINT ( 'NONE',  ( 11.13831797290559500, 1433.014992880461932, 151.6441518879982766 ) ) ;
#52984=CARTESIAN_POINT ( 'NONE',  ( -2.815577456780000265, 1409.178966352830003, 232.0007561677979879 ) ) ;
#52985=CARTESIAN_POINT ( 'NONE',  ( -5.737215272600000304, 1447.742823947540046, 185.4050672243980102 ) ) ;
#52990=CARTESIAN_POINT ( 'NONE',  ( 15.64138586982451251, 1506.512156827755462, 224.6616658709005776 ) ) ;
#52991=CARTESIAN_POINT ( 'NONE',  ( -24.99760032100000018, 1435.446235554499935, 136.3617712744980111 ) ) ;
#52995=CARTESIAN_POINT ( 'NONE',  ( -7.824237587485725953, 1425.785369531576407, 225.8505889053163287 ) ) ;
#53001=CARTESIAN_POINT ( 'NONE',  ( 18.11157372306810132, 1509.545530478630099, 186.5307137986639816 ) ) ;
#53002=CARTESIAN_POINT ( 'NONE',  ( -8.348226541789999899, 1410.293767215830030, 230.4853368651980077 ) ) ;
#53007=CARTESIAN_POINT ( 'NONE',  ( 11.90929545309599824, 1435.055828996039963, 151.1761558931260083 ) ) ;
#53008=CARTESIAN_POINT ( 'NONE',  ( 17.12655147364909780, 1478.709137272870066, 229.5900271960919952 ) ) ;
#53009=CARTESIAN_POINT ( 'NONE',  ( -24.29054017925709630, 1443.115968449809316, 212.2937530787580727 ) ) ;
#53010=CARTESIAN_POINT ( 'NONE',  ( -2.370751091799999877, 1409.499373923630174, 186.6993300599980046 ) ) ;
#53011=FACE_OUTER_BOUND ( 'NONE', #53266, .T. ) ;
#53015=CARTESIAN_POINT ( 'NONE',  ( -3.633167781729999657, 1421.710620309329897, 184.3832545295979912 ) ) ;
#53019=CARTESIAN_POINT ( 'NONE',  ( -11.69495607182969898, 1415.089948427380023, 196.2579977906119950 ) ) ;
#53020=CARTESIAN_POINT ( 'NONE',  ( -9.849896899200842881, 1519.913060387329779, 185.5490084180013923 ) ) ;
#53027=CARTESIAN_POINT ( 'NONE',  ( -16.66164933671169024, 1410.683962559431848, 191.7467638837736388 ) ) ;
#53031=CARTESIAN_POINT ( 'NONE',  ( -15.55222769949999950, 1435.858529176660113, 149.1409779191980078 ) ) ;
#53033=CARTESIAN_POINT ( 'NONE',  ( 16.86766716609999861, 1410.829200371529851, 191.8268629579980029 ) ) ;
#53035=CARTESIAN_POINT ( 'NONE',  ( -19.04725897784324573, 1440.081394454191695, 209.8288540874746388 ) ) ;
#53036=CARTESIAN_POINT ( 'NONE',  ( 11.93532938889599393, 1433.537187971887988, 150.1924424211269695 ) ) ;
#53038=CARTESIAN_POINT ( 'NONE',  ( 13.32670741457809882, 1443.315591726400044, 195.2732919480440330 ) ) ;
#53040=CARTESIAN_POINT ( 'NONE',  ( -11.90006702174173903, 1434.919293211649119, 147.6452046027968663 ) ) ;
#53054=CARTESIAN_POINT ( 'NONE',  ( 17.22174733035570071, 1507.619498552399818, 193.9103528060259976 ) ) ;
#53056=EDGE_CURVE ( 'NONE', #81697, #49156, #34514, .T. ) ;
#53059=ORIENTED_EDGE ( 'NONE', *, *, #60673, .F. ) ;
#53060=CARTESIAN_POINT ( 'NONE',  ( 19.18344385319309708, 1507.776479758349979, 229.7058228477820023 ) ) ;
#53062=CARTESIAN_POINT ( 'NONE',  ( 12.95237937484257706, 1442.920817661757610, 169.4286732187400162 ) ) ;
#53063=CARTESIAN_POINT ( 'NONE',  ( 21.31156959599999823, 1488.809466529329939, 209.1693389662900131 ) ) ;
#53064=CARTESIAN_POINT ( 'NONE',  ( -43.50118976839999618, 1440.913060407679950, 263.8966299864979987 ) ) ;
#53068=CARTESIAN_POINT ( 'NONE',  ( 26.34629031029999879, 1509.610131964929906, 199.6751120872679905 ) ) ;
#53069=CARTESIAN_POINT ( 'NONE',  ( -20.30769014010000006, 1485.515971530630168, 191.7674218760979841 ) ) ;
#53070=CARTESIAN_POINT ( 'NONE',  ( 10.06884348340000201, 1409.765578029430117, 188.8671861836979815 ) ) ;
#53071=CARTESIAN_POINT ( 'NONE',  ( 4.691567311940000096, 1422.090921882629800, 184.7225213113979976 ) ) ;
#53073=CARTESIAN_POINT ( 'NONE',  ( 11.23219740039999870, 1436.456445610539959, 151.7916777051979977 ) ) ;
#53076=CARTESIAN_POINT ( 'NONE',  ( 0.5968024102800000286, 1507.130435900830207, 237.3073193260979963 ) ) ;
#53079=CARTESIAN_POINT ( 'NONE',  ( -2.387854443607448918, 1426.854124017601634, 138.5187392187245052 ) ) ;
#53081=CARTESIAN_POINT ( 'NONE',  ( -39.31037117919999702, 1453.720620610329888, 270.1733326691979755 ) ) ;
#53083=CARTESIAN_POINT ( 'NONE',  ( 9.704564366399999642, 1443.913060387330006, 153.0477571643979786 ) ) ;
#53084=CARTESIAN_POINT ( 'NONE',  ( -14.31351010490000064, 1463.285154408930111, 223.3691465441979744 ) ) ;
#53085=CARTESIAN_POINT ( 'NONE',  ( 0.9756374909739999879, 1431.113060387329824, 189.4389011961980032 ) ) ;
#53087=CARTESIAN_POINT ( 'NONE',  ( 1.519498794560000032, 1507.960421343230109, 236.9808823833980114 ) ) ;
#53088=CARTESIAN_POINT ( 'NONE',  ( -6.380370694819999855, 1418.306873334029888, 233.0248977636979930 ) ) ;
#53091=CARTESIAN_POINT ( 'NONE',  ( -45.19191529902279569, 1433.651650798640048, 267.0047257956459816 ) ) ;
#53092=CARTESIAN_POINT ( 'NONE',  ( -3.085511914419999613, 1431.475301411720011, 185.4796394390980083 ) ) ;
#53095=VERTEX_POINT ( 'NONE', #98971 ) ;
#53101=CIRCLE ( 'NONE', #42361, 1.000000000000000000 ) ;
#53104=CARTESIAN_POINT ( 'NONE',  ( -17.21804373259962162, 1410.146604591630194, 225.6635976644989228 ) ) ;
#53109=CARTESIAN_POINT ( 'NONE',  ( -10.78872034305570082, 1416.913057013679918, 195.9645814724030117 ) ) ;
#53112=VERTEX_POINT ( 'NONE', #39635 ) ;
#53113=CARTESIAN_POINT ( 'NONE',  ( -22.23813439964190053, 1414.926657347039963, 269.4023535884739999 ) ) ;
#53115=CARTESIAN_POINT ( 'NONE',  ( 8.157130779410179500, 1418.866591275500014, 233.1788703964780041 ) ) ;
#53120=CARTESIAN_POINT ( 'NONE',  ( -23.37718023422289804, 1410.146351715440005, 210.1164981839299912 ) ) ;
#53121=CARTESIAN_POINT ( 'NONE',  ( -0.8068904912131519280, 1409.444758023880013, 185.4044988326020302 ) ) ;
#53123=CARTESIAN_POINT ( 'NONE',  ( -0.01306565375790010031, 1408.945229229399956, 186.1619460894229974 ) ) ;
#53125=CARTESIAN_POINT ( 'NONE',  ( -18.82790724813750316, 1416.384967866799798, 207.5738806952579978 ) ) ;
#53126=CARTESIAN_POINT ( 'NONE',  ( -18.55240991700000208, 1425.816903541530110, 225.0696803572979832 ) ) ;
#53127=CARTESIAN_POINT ( 'NONE',  ( 22.55223415318489799, 1471.819675376130135, 267.0319875137560075 ) ) ;
#53128=CARTESIAN_POINT ( 'NONE',  ( -8.103600148213331522, 1465.442638966462937, 233.2443155374635069 ) ) ;
#53133=CARTESIAN_POINT ( 'NONE',  ( 1.473482235510590099, 1483.325061647019993, 182.1507347926400087 ) ) ;
#53134=CARTESIAN_POINT ( 'NONE',  ( 23.60963409220000031, 1410.976028183930111, 207.8292014694679892 ) ) ;
#53137=CARTESIAN_POINT ( 'NONE',  ( 26.08016064264459999, 1451.549772369049833, 136.2273410839000007 ) ) ;
#53138=CARTESIAN_POINT ( 'NONE',  ( 11.53086876047703058, 1425.452087397813557, 137.7849336002779523 ) ) ;
#53140=CARTESIAN_POINT ( 'NONE',  ( -18.63864992402650955, 1509.044553702126677, 230.2784244607928770 ) ) ;
#53141=CARTESIAN_POINT ( 'NONE',  ( 17.54187789610000081, 1410.889696661429980, 192.7129300596980102 ) ) ;
#53142=CARTESIAN_POINT ( 'NONE',  ( 20.22153155800000235, 1444.740067931809790, 161.9155394238979966 ) ) ;
#53143=CARTESIAN_POINT ( 'NONE',  ( 2.618800203428223394, 1439.646264171884695, 183.4501813373113066 ) ) ;
#53145=CARTESIAN_POINT ( 'NONE',  ( -19.57795677556049796, 1425.757239151944532, 223.2432467385563939 ) ) ;
#53146=CARTESIAN_POINT ( 'NONE',  ( 0.6122773730909090162, 1450.961374533219896, 181.9623258240119696 ) ) ;
#53153=CARTESIAN_POINT ( 'NONE',  ( -3.666694481987490040, 1509.114858341099989, 179.5219341129400163 ) ) ;
#53155=CARTESIAN_POINT ( 'NONE',  ( -0.4760850685511259783, 1409.509622399980117, 232.8916950008960214 ) ) ;
#53159=CARTESIAN_POINT ( 'NONE',  ( -20.41675336379999806, 1443.170379801809759, 219.6133833292979887 ) ) ;
#53160=CARTESIAN_POINT ( 'NONE',  ( 28.38725554550000041, 1468.332764320925207, 266.6435172761978833 ) ) ;
#53162=CARTESIAN_POINT ( 'NONE',  ( 3.330669073880000049E-15, 1462.614442895030152, 248.0989693021979861 ) ) ;
#53170=CARTESIAN_POINT ( 'NONE',  ( -29.42360915972939850, 1510.018182097579938, 200.5862550365469872 ) ) ;
#53171=CARTESIAN_POINT ( 'NONE',  ( 24.71942444319999765, 1469.238022045029993, 216.2125151713479738 ) ) ;
#53172=AXIS2_PLACEMENT_3D ( 'NONE', #26325, #60517, #77853 ) ;
#53177=CARTESIAN_POINT ( 'NONE',  ( 2.632631803615880450, 1417.642869435429930, 234.7516633181379859 ) ) ;
#53181=EDGE_LOOP ( 'NONE', ( #22263, #10521, #18545, #7118, #3127, #98174 ) ) ;
#53182=CARTESIAN_POINT ( 'NONE',  ( -28.08752589700002744, 1445.052233488288948, 160.7519773376980936 ) ) ;
#53184=EDGE_CURVE ( 'NONE', #37255, #109848, #45058, .T. ) ;
#53185=CARTESIAN_POINT ( 'NONE',  ( -20.34464802829999996, 1507.870840051529967, 189.3862473984979999 ) ) ;
#53192=CARTESIAN_POINT ( 'NONE',  ( 11.44665326297827335, 1425.798162341591706, 139.1345266541928538 ) ) ;
#53198=CARTESIAN_POINT ( 'NONE',  ( 14.34357294504789948, 1409.413948991840016, 204.9548362799079939 ) ) ;
#53201=CARTESIAN_POINT ( 'NONE',  ( -17.93337622780000373, 1421.490724472430202, 193.1272588093980289 ) ) ;
#53212=CARTESIAN_POINT ( 'NONE',  ( -11.90604050199999975, 1433.732568523099872, 150.6972470776979947 ) ) ;
#53215=CARTESIAN_POINT ( 'NONE',  ( 16.23342327852422429, 1469.050322811229080, 269.3700830507254409 ) ) ;
#53217=CARTESIAN_POINT ( 'NONE',  ( 2.290107552079999831, 1395.993032705530140, 220.3039202953980009 ) ) ;
#53218=CARTESIAN_POINT ( 'NONE',  ( 1.789086269730000067, 1417.552112839030087, 233.6888163188979775 ) ) ;
#53220=CARTESIAN_POINT ( 'NONE',  ( -19.59053950279439960, 1486.265866315750145, 189.8955481462990065 ) ) ;
#53222=CARTESIAN_POINT ( 'NONE',  ( -26.55481977066866861, 1436.735068348699770, 136.8009166751634211 ) ) ;
#53223=CARTESIAN_POINT ( 'NONE',  ( 20.61542114513792257, 1508.364347661922238, 227.6602567161955051 ) ) ;
#53226=CARTESIAN_POINT ( 'NONE',  ( -0.5656601614563600000, 1424.194575819369902, 228.0927458373740251 ) ) ;
#53228=CARTESIAN_POINT ( 'NONE',  ( -0.3690012737985599589, 1443.315611438030146, 189.9060334618889954 ) ) ;
#53232=ORIENTED_EDGE ( 'NONE', *, *, #70043, .T. ) ;
#53233=CARTESIAN_POINT ( 'NONE',  ( 42.47347430450000161, 1432.913525160240169, 263.9447136157980367 ) ) ;
#53234=CARTESIAN_POINT ( 'NONE',  ( -26.60955424449999995, 1469.249567707230199, 208.9444902198429759 ) ) ;
#53235=CARTESIAN_POINT ( 'NONE',  ( -11.00605453490000052, 1426.944684141429889, 91.15820994169789060 ) ) ;
#53236=CARTESIAN_POINT ( 'NONE',  ( 16.63867649748380018, 1409.594336716910220, 192.8496594819030179 ) ) ;
#53239=CARTESIAN_POINT ( 'NONE',  ( 3.321478032336870001, 1396.029048956019778, 198.6099121833759966 ) ) ;
#53241=CARTESIAN_POINT ( 'NONE',  ( -27.17992431780000118, 1424.801532950129968, 248.2870168944980094 ) ) ;
#53243=CARTESIAN_POINT ( 'NONE',  ( 28.27864386421530085, 1508.411229478540008, 209.3995008269750144 ) ) ;
#53245=CARTESIAN_POINT ( 'NONE',  ( 33.14188593189999921, 1451.755856666429963, 135.1722003460979806 ) ) ;
#53246=ORIENTED_EDGE ( 'NONE', *, *, #96434, .F. ) ;
#53247=CARTESIAN_POINT ( 'NONE',  ( 6.232524879136110307, 1398.098455824979965, 220.5304231573819891 ) ) ;
#53249=CARTESIAN_POINT ( 'NONE',  ( -16.16332356590000074, 1459.159536845130106, 229.6201735760980114 ) ) ;
#53256=CARTESIAN_POINT ( 'NONE',  ( -1.356502621700000022, 1410.320696896230174, 185.6044186391980020 ) ) ;
#53260=CARTESIAN_POINT ( 'NONE',  ( -6.614451065750000858, 1470.478371390330040, 234.0809738164980160 ) ) ;
#53261=CARTESIAN_POINT ( 'NONE',  ( 0.4486526232410890103, 1420.573293467059784, 182.8046371172480065 ) ) ;
#53265=CARTESIAN_POINT ( 'NONE',  ( 14.57526300359999993, 1474.749940818629966, 224.7313656968979956 ) ) ;
#53266=EDGE_LOOP ( 'NONE', ( #77636, #72222, #75992, #74034 ) ) ;
#53270=CARTESIAN_POINT ( 'NONE',  ( 11.85935220418699920, 1431.865067821940102, 149.9620054296389924 ) ) ;
#53271=CARTESIAN_POINT ( 'NONE',  ( 12.64036215934078022, 1445.032014182524335, 186.2682781246677166 ) ) ;
#53273=CARTESIAN_POINT ( 'NONE',  ( -15.62326149431152089, 1506.535970900717984, 193.5355000223906075 ) ) ;
#53274=CARTESIAN_POINT ( 'NONE',  ( -13.35741048202589809, 1443.501467202830099, 164.9741927960640453 ) ) ;
#53275=CARTESIAN_POINT ( 'NONE',  ( 9.021136374670000180, 1508.721785377329979, 235.3723347276979894 ) ) ;
#53277=CARTESIAN_POINT ( 'NONE',  ( -4.789983303610000576, 1423.864849667030057, 185.3823132089979993 ) ) ;
#53278=CARTESIAN_POINT ( 'NONE',  ( 3.565775598909999733, 1407.753784349630223, 270.1349117941979898 ) ) ;
#53287=AXIS2_PLACEMENT_3D ( 'NONE', #17738, #10482, #19416 ) ;
#53288=CARTESIAN_POINT ( 'NONE',  ( 17.91313270363389876, 1420.835020208859987, 225.0974074490680152 ) ) ;
#53291=CARTESIAN_POINT ( 'NONE',  ( 12.85916294189999931, 1411.892799971530167, 268.3665355204980187 ) ) ;
#53293=CARTESIAN_POINT ( 'NONE',  ( 40.96765513241462742, 1447.290458505206743, 135.1834236911112441 ) ) ;
#53295=FACE_OUTER_BOUND ( 'NONE', #32510, .T. ) ;
#53302=DIRECTION ( 'NONE',  ( 0.7054602837376293678, -3.121166767548191889E-15, -0.7087494536638624387 ) ) ;
#53303=CARTESIAN_POINT ( 'NONE',  ( 5.370527602886283169, 1422.356908813907012, 139.1416118586824666 ) ) ;
#53304=CARTESIAN_POINT ( 'NONE',  ( 30.54334960032450041, 1509.992611366529900, 207.3226989945189871 ) ) ;
#53305=CARTESIAN_POINT ( 'NONE',  ( 13.33986755048250039, 1429.041205739520137, 222.0838351576450123 ) ) ;
#53306=CARTESIAN_POINT ( 'NONE',  ( -4.360582346120001063, 1431.113060387329824, 227.9437648745980027 ) ) ;
#53307=CARTESIAN_POINT ( 'NONE',  ( 16.18846431829999943, 1410.409213254730048, 226.7751941885980216 ) ) ;
#53309=AXIS2_PLACEMENT_3D ( 'NONE', #28123, #103154, #94208 ) ;
#53310=CARTESIAN_POINT ( 'NONE',  ( -16.62342269400000205, 1460.779327316729905, 228.2681772136979816 ) ) ;
#53312=CARTESIAN_POINT ( 'NONE',  ( 39.02011237019999612, 1422.796720904130098, 269.1561393349979880 ) ) ;
#53314=CARTESIAN_POINT ( 'NONE',  ( 15.43924878589999850, 1436.272480559940050, 149.3456521445980059 ) ) ;
#53315=CARTESIAN_POINT ( 'NONE',  ( 21.03034198799999999, 1488.584892799430008, 192.0921482354980014 ) ) ;
#53316=CARTESIAN_POINT ( 'NONE',  ( -21.08953343030000127, 1428.992258108429951, 221.5629153413979964 ) ) ;
#53318=CARTESIAN_POINT ( 'NONE',  ( -7.055157488669999921, 1475.427864936029891, 266.9413125670979525 ) ) ;
#53320=CARTESIAN_POINT ( 'NONE',  ( -41.49265034658910167, 1443.149328808269956, 136.5063902170460040 ) ) ;
#53321=CARTESIAN_POINT ( 'NONE',  ( -20.13566255811392480, 1506.560172253814471, 200.0397955187486048 ) ) ;
#53323=CARTESIAN_POINT ( 'NONE',  ( -12.68686629940000010, 1442.617705476030096, 187.1386741737979946 ) ) ;
#53324=CARTESIAN_POINT ( 'NONE',  ( -33.14721542679999544, 1436.549951028310034, 136.5342324578980140 ) ) ;
#53328=CARTESIAN_POINT ( 'NONE',  ( -13.55472914751489988, 1409.386401959430032, 215.4052957893119924 ) ) ;
#53330=CARTESIAN_POINT ( 'NONE',  ( -2.478067412690000193, 1440.020830691129959, 157.7869724642980032 ) ) ;
#53331=CARTESIAN_POINT ( 'NONE',  ( -21.13431252044160047, 1409.651086843229905, 211.8287216663260040 ) ) ;
#53332=CARTESIAN_POINT ( 'NONE',  ( -45.85460265660000800, 1445.993250122450036, 268.7562748562979777 ) ) ;
#53335=CARTESIAN_POINT ( 'NONE',  ( 0.1715103366868419854, 1420.360261608449946, 183.3974109806000001 ) ) ;
#53336=CARTESIAN_POINT ( 'NONE',  ( -26.91031503490000176, 1509.852789295929824, 218.7452626102079876 ) ) ;
#53339=CARTESIAN_POINT ( 'NONE',  ( 17.33879185520300226, 1422.603306420210174, 226.6220729339370052 ) ) ;
#53340=CARTESIAN_POINT ( 'NONE',  ( 20.61548266710000021, 1508.365537841329797, 227.7135694462980098 ) ) ;
#53341=AXIS2_PLACEMENT_3D ( 'NONE', #67777, #92953, #8947 ) ;
#53342=CARTESIAN_POINT ( 'NONE',  ( 3.552713678799999608E-15, 1432.353292893639946, 155.3998094795979910 ) ) ;
#53346=VECTOR ( 'NONE', #34810, 1000.000000000000000 ) ;
#53348=( BOUNDED_SURFACE ( )  B_SPLINE_SURFACE ( 1, 2, ( 
 ( #17244, #1056, #66610 ),
 ( #32964, #33504, #67705 ) ),
 .UNSPECIFIED., .F., .F., .F. ) 
 B_SPLINE_SURFACE_WITH_KNOTS ( ( 2, 2 ),
 ( 3, 3 ),
 ( -10000.00000000000000, 10000.00000000000000 ),
 ( 5.300753508068379638, 6.148747966334259907 ),
 .UNSPECIFIED. ) 
 GEOMETRIC_REPRESENTATION_ITEM ( )  RATIONAL_B_SPLINE_SURFACE ( (
 ( 0.8627701935022110691, 0.8231028658330309389, 0.9541560038134260235),
 ( 0.8627701935022110691, 0.8231028658330309389, 0.9541560038134260235) ) ) 
 REPRESENTATION_ITEM ( '' )  SURFACE ( )  );
#53349=CARTESIAN_POINT ( 'NONE',  ( 16.63199911499999928, 1416.518938591829965, 201.3741761614680001 ) ) ;
#53352=CARTESIAN_POINT ( 'NONE',  ( 23.68159507920000095, 1410.235400666329951, 210.4508981972280139 ) ) ;
#53355=CARTESIAN_POINT ( 'NONE',  ( -15.56072141409999965, 1422.731526910729826, 229.1456929959980187 ) ) ;
#53356=CARTESIAN_POINT ( 'NONE',  ( -11.86937547910000035, 1432.581147039740017, 149.9818613170979802 ) ) ;
#53358=CARTESIAN_POINT ( 'NONE',  ( 0.7119424177869999593, 1411.661590166830138, 233.1969697336979834 ) ) ;
#53364=AXIS2_PLACEMENT_3D ( 'NONE', #82668, #14339, #57487 ) ;
#53365=CARTESIAN_POINT ( 'NONE',  ( -19.61843130789999989, 1426.543110900729744, 225.3457329349979830 ) ) ;
#53372=CARTESIAN_POINT ( 'NONE',  ( 11.81528372083669964, 1433.677274197049883, 150.7650281621870079 ) ) ;
#53374=ORIENTED_EDGE ( 'NONE', *, *, #54196, .F. ) ;
#53377=CARTESIAN_POINT ( 'NONE',  ( 17.63154828746949931, 1477.220527230660082, 189.4679263864980214 ) ) ;
#53378=CARTESIAN_POINT ( 'NONE',  ( 0.2916220566639999845, 1508.974498516630092, 179.3904948502979835 ) ) ;
#53380=CARTESIAN_POINT ( 'NONE',  ( 0.7726025625319999923, 1488.176002970830268, 181.8096760246980068 ) ) ;
#53382=CARTESIAN_POINT ( 'NONE',  ( -24.47690167607559886, 1444.776640416369901, 211.0359720841289857 ) ) ;
#53384=CARTESIAN_POINT ( 'NONE',  ( 35.72409870452920444, 1435.953719464650021, 134.0999999973689967 ) ) ;
#53388=CARTESIAN_POINT ( 'NONE',  ( 14.37148033386480073, 1435.528465542959793, 149.6149653547480227 ) ) ;
#53390=ORIENTED_EDGE ( 'NONE', *, *, #5680, .F. ) ;
#53393=CARTESIAN_POINT ( 'NONE',  ( 12.68761320032887774, 1445.019507500634973, 169.4610301561137646 ) ) ;
#53394=LINE ( 'NONE', #68542, #84905 ) ;
#53395=CARTESIAN_POINT ( 'NONE',  ( 7.061178118806066273, 1451.421219515312714, 153.2201617045464559 ) ) ;
#53400=CARTESIAN_POINT ( 'NONE',  ( 4.240698138573309350, 1446.387872175620032, 162.7199821555450114 ) ) ;
#53405=CARTESIAN_POINT ( 'NONE',  ( 30.22378019458900056, 1440.913060387330006, 252.5570269051040100 ) ) ;
#53406=CARTESIAN_POINT ( 'NONE',  ( -20.01701400349999815, 1508.375006160530120, 188.9474772183980065 ) ) ;
#53408=CARTESIAN_POINT ( 'NONE',  ( 25.71410359372319832, 1448.114898661300003, 138.0507843406130064 ) ) ;
#53409=CARTESIAN_POINT ( 'NONE',  ( -13.57875502439999948, 1410.319880166030089, 190.0093725944979894 ) ) ;
#53411=CARTESIAN_POINT ( 'NONE',  ( -24.36454078510000087, 1441.184224637150010, 211.6994343379179782 ) ) ;
#53413=CARTESIAN_POINT ( 'NONE',  ( -10.79382126600000014, 1414.913060387329779, 196.1395803457980094 ) ) ;
#53414=CARTESIAN_POINT ( 'NONE',  ( 3.512785867830420180E-12, 1395.913060387330006, 198.1220674046479928 ) ) ;
#53415=CARTESIAN_POINT ( 'NONE',  ( -13.57096693066059245, 1434.971412459564817, 146.5999775064138078 ) ) ;
#53416=CARTESIAN_POINT ( 'NONE',  ( -13.50087351860000062, 1434.968964114900245, 149.2725308732979954 ) ) ;
#53420=B_SPLINE_CURVE_WITH_KNOTS ( 'NONE', 3,
 ( #100655, #73836, #39668, #40214, #14990, #40765, #81646 ),
 .UNSPECIFIED., .F., .F.,
 ( 4, 3, 4 ),
 ( -157.3797848890000068, -135.2383462476790044, -79.35007823249820547 ),
 .UNSPECIFIED. ) ;
#53425=DIRECTION ( 'NONE',  ( 4.440892098500004934E-16, 1.000000000000000000, -1.817990202819999994E-15 ) ) ;
#53427=CARTESIAN_POINT ( 'NONE',  ( 29.74048404330000039, 1509.991911966430052, 208.2083000408450175 ) ) ;
#53431=CARTESIAN_POINT ( 'NONE',  ( -20.60842128280000196, 1470.808655613029941, 208.9538791287869799 ) ) ;
#53432=CARTESIAN_POINT ( 'NONE',  ( -15.48476762197763712, 1486.079411782601710, 186.6377642270500132 ) ) ;
#53434=ORIENTED_EDGE ( 'NONE', *, *, #59412, .T. ) ;
#53435=CARTESIAN_POINT ( 'NONE',  ( -1.052431931479999916, 1415.163755984229965, 226.8636908286979974 ) ) ;
#53437=CARTESIAN_POINT ( 'NONE',  ( 24.68961616380000024, 1449.416966549430072, 225.7902685641979872 ) ) ;
#53440=CARTESIAN_POINT ( 'NONE',  ( -27.36363609755069959, 1509.868619615939906, 219.7361812052210155 ) ) ;
#53441=EDGE_CURVE ( 'NONE', #79053, #73912, #63693, .T. ) ;
#53442=CARTESIAN_POINT ( 'NONE',  ( -8.259315774359869522, 1509.138868980799998, 236.6356052361459774 ) ) ;
#53443=CARTESIAN_POINT ( 'NONE',  ( -22.59132398960000288, 1450.596213101380044, 220.3211801345979950 ) ) ;
#53444=CARTESIAN_POINT ( 'NONE',  ( 4.219439073160000220, 1446.230224797059918, 176.4605749492980067 ) ) ;
#53445=CARTESIAN_POINT ( 'NONE',  ( 17.99788318405029841, 1410.854924907409895, 222.9846978063220320 ) ) ;
#53446=CARTESIAN_POINT ( 'NONE',  ( -0.3713800987810000342, 1452.819910075930011, 189.4897211325980209 ) ) ;
#53449=ORIENTED_EDGE ( 'NONE', *, *, #65942, .F. ) ;
#53451=CARTESIAN_POINT ( 'NONE',  ( 1.624206324989999992E-09, 1405.716796065430117, 267.8540375962979851 ) ) ;
#53452=CARTESIAN_POINT ( 'NONE',  ( 27.89933032689999948, 1509.196990926829812, 207.5041886574580019 ) ) ;
#53453=CARTESIAN_POINT ( 'NONE',  ( 19.23545976010510117, 1469.948318476340091, 270.3616590758479674 ) ) ;
#53454=CARTESIAN_POINT ( 'NONE',  ( 2.478942931479999778, 1432.372492341360157, 157.5167539238979941 ) ) ;
#53457=CARTESIAN_POINT ( 'NONE',  ( -41.70033323359630373, 1440.913060410520075, 261.5743097596159714 ) ) ;
#53458=CARTESIAN_POINT ( 'NONE',  ( 34.72830299008759880, 1450.359847782400038, 136.2305431565669949 ) ) ;
#53459=CARTESIAN_POINT ( 'NONE',  ( 1.081131680213342827, 1450.824894072367897, 154.2469214281843506 ) ) ;
#53461=CARTESIAN_POINT ( 'NONE',  ( 1.171201999982100173, 1450.815562198650014, 154.2439547458699849 ) ) ;
#53463=EDGE_CURVE ( 'NONE', #31461, #56666, #94279, .T. ) ;
#53465=CARTESIAN_POINT ( 'NONE',  ( 2.416798835000000256, 1426.601114010129777, 146.0361887655980127 ) ) ;
#53466=EDGE_CURVE ( 'NONE', #22743, #65683, #3609, .T. ) ;
#53467=CARTESIAN_POINT ( 'NONE',  ( -1.262039348750485956, 1450.743516540221663, 181.7894505913149601 ) ) ;
#53469=CARTESIAN_POINT ( 'NONE',  ( -1.333756890899999936, 1476.036794647129909, 268.4830614120980385 ) ) ;
#53471=CARTESIAN_POINT ( 'NONE',  ( -29.61947536759999977, 1509.969965958529883, 210.6832956776279673 ) ) ;
#53472=B_SPLINE_CURVE_WITH_KNOTS ( 'NONE', 3,
 ( #22969, #48769, #6186, #34695, #2651, #102987, #19965, #88836, #94045, #63127, #53606, #85638, #54710, #20500, #87750, #62576, #28376, #13, #45757, #97229, #37889, #72072, #28937 ),
 .UNSPECIFIED., .F., .F.,
 ( 4, 2, 1, 1, 2, 2, 2, 1, 2, 2, 2, 2, 4 ),
 ( 0.000000000000000000, 0.1249999999999765188, 0.1874999999999680533, 0.2187499999998618327, 0.2343749999999021894, 0.2499999999999425460, 0.3749999999996026512, 0.4374999999995266564, 0.4687499999994845790, 0.4999999999994425015, 0.6249999999996125322, 0.7499999999997823963, 1.000000000000000000 ),
 .UNSPECIFIED. ) ;
#53473=CARTESIAN_POINT ( 'NONE',  ( -3.832095730067969441, 1448.295222384574345, 185.0250836445331970 ) ) ;
#53475=AXIS2_PLACEMENT_3D ( 'NONE', #64134, #98255, #39460 ) ;
#53476=B_SPLINE_SURFACE_WITH_KNOTS ( 'NONE', 5, 4, ( 
 ( #104240, #81225, #3456, #4540, #96396 ),
 ( #70129, #27530, #19103, #53306, #97492 ),
 ( #62266, #44915, #37029, #70678, #104792 ),
 ( #37584, #88552, #11298, #12372, #105346 ),
 ( #71787, #20760, #89085, #48759, #57716 ),
 ( #82341, #39224, #66665, #91831, #58253 ) ),
 .UNSPECIFIED., .F., .F., .F.,
 ( 6, 6 ),
 ( 5, 5 ),
 ( 0.000000000000000000, 111.1101480259999903 ),
 ( 25.81581217359999769, 39.03307591160000101 ),
 .UNSPECIFIED. ) ;
#53477=CARTESIAN_POINT ( 'NONE',  ( -17.74184486700000107, 1415.163755984229965, 208.0694140301980326 ) ) ;
#53479=CARTESIAN_POINT ( 'NONE',  ( 26.25308187535300419, 1435.420717402130094, 135.4969117712219884 ) ) ;
#53480=CARTESIAN_POINT ( 'NONE',  ( -7.087593545181670507, 1396.160564607840115, 200.6470654363129995 ) ) ;
#53481=CARTESIAN_POINT ( 'NONE',  ( -17.33378134921720104, 1410.882908438999948, 225.8654669597239888 ) ) ;
#53482=CARTESIAN_POINT ( 'NONE',  ( 4.989973902650000070, 1442.756953654919926, 150.3769280849980134 ) ) ;
#53486=CARTESIAN_POINT ( 'NONE',  ( 0.3788332004054269508, 1408.926289534200123, 231.6114332047860103 ) ) ;
#53487=CARTESIAN_POINT ( 'NONE',  ( 10.87934504459999907, 1425.316387834530133, 126.2846869380979911 ) ) ;
#53492=( GEOMETRIC_REPRESENTATION_CONTEXT ( 3 ) GLOBAL_UNCERTAINTY_ASSIGNED_CONTEXT ( ( #19946 ) ) GLOBAL_UNIT_ASSIGNED_CONTEXT ( ( #22879, #81507, #55246 ) ) REPRESENTATION_CONTEXT ( 'NONE', 'WORKASPACE' ) );
#53494=CARTESIAN_POINT ( 'NONE',  ( -14.82503814461925273, 1430.093753747135452, 221.8913042101295048 ) ) ;
#53496=CARTESIAN_POINT ( 'NONE',  ( -0.3621993323151809774, 1416.825784014559986, 191.0664209890499876 ) ) ;
#53504=CARTESIAN_POINT ( 'NONE',  ( -12.94626818629999931, 1441.161188681390058, 188.2109162517980110 ) ) ;
#53506=CARTESIAN_POINT ( 'NONE',  ( 0.04366246281853980449, 1474.775529741679975, 236.0040081736329967 ) ) ;
#53507=DIRECTION ( 'NONE',  ( 0.1324471657667971036, -0.9756113948842708439, -0.1750432930800552289 ) ) ;
#53509=DIRECTION ( 'NONE',  ( 0.000000000000000000, -2.622151149039999577E-17, 1.000000000000000000 ) ) ;
#53510=CARTESIAN_POINT ( 'NONE',  ( 23.69809918860000053, 1507.890500233530020, 195.1972782134980093 ) ) ;
#53513=CARTESIAN_POINT ( 'NONE',  ( -2.500000000000039968, 1448.775613387130079, 156.9598478879729839 ) ) ;
#53514=CARTESIAN_POINT ( 'NONE',  ( 28.37196897381756244, 1435.488267112151334, 135.2384693731098082 ) ) ;
#53515=CARTESIAN_POINT ( 'NONE',  ( 6.707555271009190356, 1408.966021048169750, 196.0542721895619991 ) ) ;
#53516=CARTESIAN_POINT ( 'NONE',  ( -5.365730855182169634, 1405.947096103700005, 267.8417508978809565 ) ) ;
#53517=DIRECTION ( 'NONE',  ( 0.4794255386042036160, 0.000000000000000000, 0.8775825618903725367 ) ) ;
#53519=CARTESIAN_POINT ( 'NONE',  ( -11.57646188839999901, 1432.336252568690043, 151.1966908189980074 ) ) ;
#53520=CARTESIAN_POINT ( 'NONE',  ( 12.53380416529999941, 1442.773886989730045, 186.4115681209980266 ) ) ;
#53522=EDGE_LOOP ( 'NONE', ( #78198, #92335, #546, #18572, #47870, #82221, #99615, #80924, #40678 ) ) ;
#53523=EDGE_CURVE ( 'NONE', #16284, #65282, #72636, .T. ) ;
#53526=CIRCLE ( 'NONE', #28483, 477.3395627918638411 ) ;
#53527=ADVANCED_FACE ( 'NONE', ( #45030 ), #29343, .F. ) ;
#53530=B_SPLINE_CURVE_WITH_KNOTS ( 'NONE', 5,
 ( #77109, #86594, #9886, #2070, #44054, #70385 ),
 .UNSPECIFIED., .F., .F.,
 ( 6, 6 ),
 ( 0.000000000000000000, 1.000000000000000000 ),
 .UNSPECIFIED. ) ;
#53531=EDGE_LOOP ( 'NONE', ( #93441, #33246, #8300, #90000, #109044 ) ) ;
#53534=CARTESIAN_POINT ( 'NONE',  ( 10.03978052889999972, 1416.217772598529791, 224.7103670548980006 ) ) ;
#53538=CARTESIAN_POINT ( 'NONE',  ( -41.48541085310784382, 1435.896297111339663, 269.6377304084467141 ) ) ;
#53540=CARTESIAN_POINT ( 'NONE',  ( -6.493240042750000107, 1410.513797117929926, 231.2937525223979947 ) ) ;
#53541=CARTESIAN_POINT ( 'NONE',  ( -7.303238992729999879, 1446.886847238160044, 185.6134793553979989 ) ) ;
#53543=LINE ( 'NONE', #11525, #92241 ) ;
#53544=CARTESIAN_POINT ( 'NONE',  ( 11.26564539523899100, 1425.481176323582531, 139.1357185245598487 ) ) ;
#53547=CARTESIAN_POINT ( 'NONE',  ( -24.83630077529999980, 1435.383754686160046, 136.1505334551980013 ) ) ;
#53552=CARTESIAN_POINT ( 'NONE',  ( -8.515748345960094667, 1426.079849815119815, 225.4758549209027478 ) ) ;
#53554=CARTESIAN_POINT ( 'NONE',  ( 20.78146551274081943, 1410.998373634254449, 199.3095149131587505 ) ) ;
#53558=LINE ( 'NONE', #1486, #15085 ) ;
#53559=CARTESIAN_POINT ( 'NONE',  ( -14.09893512380000047, 1417.904223768229940, 227.3332539714980101 ) ) ;
#53562=ORIENTED_EDGE ( 'NONE', *, *, #71271, .F. ) ;
#53564=VECTOR ( 'NONE', #90070, 1000.000000000000114 ) ;
#53567=CARTESIAN_POINT ( 'NONE',  ( 17.85726237922320081, 1469.009919690150127, 228.6204578493800170 ) ) ;
#53568=CARTESIAN_POINT ( 'NONE',  ( -24.69948770750570333, 1509.552006277990131, 222.6391526336500135 ) ) ;
#53569=CARTESIAN_POINT ( 'NONE',  ( -2.935740854740000128, 1409.954265560430031, 186.6342706574980070 ) ) ;
#53571=CARTESIAN_POINT ( 'NONE',  ( 0.05285025628535950509, 1420.446797781519990, 182.6782354290490105 ) ) ;
#53572=EDGE_CURVE ( 'NONE', #8387, #99599, #37098, .T. ) ;
#53574=CARTESIAN_POINT ( 'NONE',  ( -4.250070903060000127, 1421.703404100430134, 185.6649461332980025 ) ) ;
#53577=ORIENTED_EDGE ( 'NONE', *, *, #9321, .T. ) ;
#53578=CARTESIAN_POINT ( 'NONE',  ( -12.25440271872340148, 1415.429375168349907, 196.4054266176139834 ) ) ;
#53581=VECTOR ( 'NONE', #55247, 1000.000000000000000 ) ;
#53582=CARTESIAN_POINT ( 'NONE',  ( 0.3313159878120000013, 1417.263519912130050, 235.9102102634980156 ) ) ;
#53583=EDGE_CURVE ( 'NONE', #55469, #22181, #84268, .T. ) ;
#53584=CARTESIAN_POINT ( 'NONE',  ( 9.934585978703848852, 1435.770999680745945, 152.5360695867651089 ) ) ;
#53589=CARTESIAN_POINT ( 'NONE',  ( 17.86855543449999928, 1415.163755998629995, 210.6784302842380043 ) ) ;
#53590=CARTESIAN_POINT ( 'NONE',  ( -2.446787376320000096, 1432.353341358199941, 150.2884730787980061 ) ) ;
#53591=CARTESIAN_POINT ( 'NONE',  ( -22.85501015979999906, 1436.107805423079981, 141.7713381877979941 ) ) ;
#53593=CARTESIAN_POINT ( 'NONE',  ( 16.64856530119999789, 1416.208557986029973, 191.4534465615980139 ) ) ;
#53594=CARTESIAN_POINT ( 'NONE',  ( 0.6414547015549999509, 1416.067629290630066, 190.6212042380979881 ) ) ;
#53595=CARTESIAN_POINT ( 'NONE',  ( -18.97549637783819421, 1439.232629296661344, 210.2045300455428389 ) ) ;
#53596=EDGE_CURVE ( 'NONE', #53095, #81952, #57149, .T. ) ;
#53599=CARTESIAN_POINT ( 'NONE',  ( 13.73472823738089943, 1456.560500377009930, 194.8610419970869998 ) ) ;
#53600=CARTESIAN_POINT ( 'NONE',  ( 26.56868433090000181, 1488.557140808829899, 207.4007234374079758 ) ) ;
#53602=CARTESIAN_POINT ( 'NONE',  ( -23.67281635530000017, 1436.130135845430004, 211.8387132574179930 ) ) ;
#53604=CARTESIAN_POINT ( 'NONE',  ( -18.51591345220000306, 1509.559650331729927, 231.0978208730980157 ) ) ;
#53605=CARTESIAN_POINT ( 'NONE',  ( 0.3788332004054269508, 1408.926289534200123, 231.6114332047860103 ) ) ;
#53606=CARTESIAN_POINT ( 'NONE',  ( 11.52616021266821278, 1434.866878790148348, 151.4211076298512637 ) ) ;
#53607=B_SPLINE_SURFACE_WITH_KNOTS ( 'NONE', 4, 5, ( 
 ( #85991, #35032, #17653, #70891, #61378, #19318 ),
 ( #44002, #28294, #95497, #53519, #69211, #78137 ),
 ( #43452, #9289, #45123, #79265, #2575, #78703 ),
 ( #26059, #1440, #36697, #88211, #62490, #35586 ),
 ( #94372, #69778, #51854, #96610, #19879, #94949 ) ),
 .UNSPECIFIED., .F., .F., .F.,
 ( 5, 5 ),
 ( 6, 6 ),
 ( 13.83774376510000081, 13.94215241960000107 ),
 ( 0.000000000000000000, 2.228199836199999950 ),
 .UNSPECIFIED. ) ;
#53609=CARTESIAN_POINT ( 'NONE',  ( -22.59870855689359814, 1509.715337612740086, 188.9651625613269914 ) ) ;
#53615=CARTESIAN_POINT ( 'NONE',  ( -15.45308515272032501, 1506.474306115792388, 224.8043937606940688 ) ) ;
#53619=CARTESIAN_POINT ( 'NONE',  ( -18.41191564635506950, 1458.954972189355885, 227.7144718060530977 ) ) ;
#53620=AXIS2_PLACEMENT_3D ( 'NONE', #26154, #7169, #85506 ) ;
#53623=ORIENTED_EDGE ( 'NONE', *, *, #59118, .F. ) ;
#53624=EDGE_LOOP ( 'NONE', ( #29368, #41111, #82652, #86969 ) ) ;
#53625=CARTESIAN_POINT ( 'NONE',  ( 23.89882922079599936, 1419.330057139640076, 207.7533880750820003 ) ) ;
#53626=CARTESIAN_POINT ( 'NONE',  ( 13.70391237549999985, 1509.385661485429864, 234.3784090209980207 ) ) ;
#53627=CARTESIAN_POINT ( 'NONE',  ( 13.14452880787822586, 1443.063641493199384, 169.3992238275367299 ) ) ;
#53629=CARTESIAN_POINT ( 'NONE',  ( -39.40331983270000649, 1445.870378090409758, 259.1105268160980586 ) ) ;
#53631=CARTESIAN_POINT ( 'NONE',  ( -11.39963766959999880, 1433.910854737510135, 151.4262557347980191 ) ) ;
#53632=CARTESIAN_POINT ( 'NONE',  ( 25.78155807829999802, 1509.813372234129929, 195.1138720307980066 ) ) ;
#53633=CARTESIAN_POINT ( 'NONE',  ( -20.68237067309999944, 1485.791741470130091, 191.8803888813980052 ) ) ;
#53634=CARTESIAN_POINT ( 'NONE',  ( 9.698169174809999404, 1409.251727919130190, 189.5635320467980307 ) ) ;
#53636=CARTESIAN_POINT ( 'NONE',  ( -10.92774616719999869, 1436.036447822629952, 151.9134056697980100 ) ) ;
#53637=CARTESIAN_POINT ( 'NONE',  ( 10.64187387509999994, 1435.613679513749958, 152.0651251919979927 ) ) ;
#53639=CARTESIAN_POINT ( 'NONE',  ( -14.51584819470000021, 1452.406155798529880, 148.7179611920979880 ) ) ;
#53640=CARTESIAN_POINT ( 'NONE',  ( 1.348363413820000245, 1466.040058158929924, 235.1849735751980006 ) ) ;
#53644=CARTESIAN_POINT ( 'NONE',  ( -38.65570300630000133, 1453.321626439029842, 269.5859728025980075 ) ) ;
#53645=DIRECTION ( 'NONE',  ( 0.1159387279768451934, 0.9932563673871469545, 0.000000000000000000 ) ) ;
#53646=CARTESIAN_POINT ( 'NONE',  ( 3.312638106410000116, 1440.449723275869928, 155.6633363266980155 ) ) ;
#53647=CARTESIAN_POINT ( 'NONE',  ( -16.68599179819999989, 1461.099982565929849, 230.2790296985980092 ) ) ;
#53650=CARTESIAN_POINT ( 'NONE',  ( 2.905858652024770006, 1409.547798013280044, 231.3102161809150061 ) ) ;
#53652=CARTESIAN_POINT ( 'NONE',  ( -9.848894837239999589, 1418.540965017630015, 230.1861045164980055 ) ) ;
#53655=CARTESIAN_POINT ( 'NONE',  ( -45.56365896290319739, 1436.758397562629852, 266.4221133662970260 ) ) ;
#53656=CARTESIAN_POINT ( 'NONE',  ( -4.152137804869999727, 1434.229915741350169, 185.7429424955980153 ) ) ;
#53658=ORIENTED_EDGE ( 'NONE', *, *, #15065, .F. ) ;
#53659=CARTESIAN_POINT ( 'NONE',  ( 26.79414481833639883, 1435.433178084320161, 135.2874577367330176 ) ) ;
#53662=ADVANCED_FACE ( 'NONE', ( #50928 ), #18540, .F. ) ;
#53665=CARTESIAN_POINT ( 'NONE',  ( -15.71820076539999889, 1410.407305047730006, 191.1858524523979952 ) ) ;
#53666=AXIS2_PLACEMENT_3D ( 'NONE', #62158, #96285, #19562 ) ;
#53668=ORIENTED_EDGE ( 'NONE', *, *, #29677, .F. ) ;
#53669=CARTESIAN_POINT ( 'NONE',  ( 24.55901760909999965, 1439.292416066280111, 213.0859795990780015 ) ) ;
#53677=B_SPLINE_CURVE_WITH_KNOTS ( 'NONE', 5,
 ( #70660, #72294, #71206, #87997, #20744, #3991 ),
 .UNSPECIFIED., .F., .F.,
 ( 6, 6 ),
 ( 0.000000000000000000, 1.000000000000000000 ),
 .UNSPECIFIED. ) ;
#53679=ORIENTED_EDGE ( 'NONE', *, *, #101553, .T. ) ;
#53680=CARTESIAN_POINT ( 'NONE',  ( -23.16921277159769943, 1412.901786882649958, 270.3115576615130067 ) ) ;
#53682=CARTESIAN_POINT ( 'NONE',  ( 2.920857164672000295, 1415.930116342160090, 231.8786464872950148 ) ) ;
#53688=CARTESIAN_POINT ( 'NONE',  ( 45.59681776243620277, 1442.353254080252782, 268.9758503888685368 ) ) ;
#53690=CARTESIAN_POINT ( 'NONE',  ( 3.668705825779739804, 1424.252539915140460, 184.0936608447964886 ) ) ;
#53692=CARTESIAN_POINT ( 'NONE',  ( -0.009463166745531850083, 1408.928470256950050, 186.2540302668519985 ) ) ;
#53694=CARTESIAN_POINT ( 'NONE',  ( -20.90608034417369510, 1506.501081265402263, 216.1110890664156727 ) ) ;
#53695=CARTESIAN_POINT ( 'NONE',  ( -17.62832093970000003, 1420.842712498729952, 226.1633071633980023 ) ) ;
#53696=CARTESIAN_POINT ( 'NONE',  ( -0.0001227683397465710060, 1475.836931224890122, 266.9609101321269691 ) ) ;
#53698=FACE_OUTER_BOUND ( 'NONE', #55044, .T. ) ;
#53702=CARTESIAN_POINT ( 'NONE',  ( 1.514633574868839760, 1459.047947303010005, 183.2114944213780063 ) ) ;
#53703=ORIENTED_EDGE ( 'NONE', *, *, #98518, .T. ) ;
#53707=CARTESIAN_POINT ( 'NONE',  ( 26.47436799094689874, 1450.913174653700025, 136.4782587642529847 ) ) ;
#53708=CARTESIAN_POINT ( 'NONE',  ( 14.35445997400000095, 1416.822690122629865, 196.6654169409980000 ) ) ;
#53712=CARTESIAN_POINT ( 'NONE',  ( 18.06824345470000281, 1410.907293943229888, 193.5833886661979761 ) ) ;
#53713=CARTESIAN_POINT ( 'NONE',  ( 22.16158255899999929, 1409.686959905830236, 207.7669082622679753 ) ) ;
#53714=CARTESIAN_POINT ( 'NONE',  ( 2.515271632033067029, 1439.627825555826803, 183.0399134896231601 ) ) ;
#53715=CARTESIAN_POINT ( 'NONE',  ( 0.3238590051470000009, 1415.419573753229997, 233.4172068791979768 ) ) ;
#53716=CARTESIAN_POINT ( 'NONE',  ( -19.37919121348099338, 1425.467690119061444, 223.5898347255973988 ) ) ;
#53717=CARTESIAN_POINT ( 'NONE',  ( 0.7878817032865200742, 1452.621947969149915, 183.3487653229790055 ) ) ;
#53721=CARTESIAN_POINT ( 'NONE',  ( 26.34505535303209811, 1447.162759454769912, 137.4478556263329949 ) ) ;
#53725=CARTESIAN_POINT ( 'NONE',  ( -0.3999176547066230492, 1409.147139264330008, 232.5106188436409980 ) ) ;
#53726=EDGE_CURVE ( 'NONE', #9730, #73741, #59074, .T. ) ;
#53728=CARTESIAN_POINT ( 'NONE',  ( -37.14121207673490233, 1449.456133586259966, 136.3012389827200082 ) ) ;
#53730=CARTESIAN_POINT ( 'NONE',  ( -10.05164998770000118, 1455.338937666430184, 224.8635561661979807 ) ) ;
#53731=CARTESIAN_POINT ( 'NONE',  ( -1.941439933476549973, 1451.940361028549887, 184.3724788387269768 ) ) ;
#53732=CARTESIAN_POINT ( 'NONE',  ( 11.21314269340000180, 1433.085161743930030, 151.5744673939979918 ) ) ;
#53733=CARTESIAN_POINT ( 'NONE',  ( 8.934239303591028146E-06, 1474.175163912050039, 270.1377477021339928 ) ) ;
#53734=B_SPLINE_SURFACE_WITH_KNOTS ( 'NONE', 5, 4, ( 
 ( #88286, #96128, #8938, #97777, #11580 ),
 ( #11030, #106187, #569, #59926, #71532 ),
 ( #17311, #42549, #63662, #25726, #45199 ),
 ( #12122, #43112, #36779, #21052, #29469 ),
 ( #55255, #46314, #80443, #34148, #3757 ),
 ( #96695, #77271, #89387, #26286, #60475 ) ),
 .UNSPECIFIED., .F., .F., .F.,
 ( 6, 6 ),
 ( 5, 5 ),
 ( 0.000000000000000000, 111.1101480259999903 ),
 ( 25.81581217359999769, 39.03307591160000101 ),
 .UNSPECIFIED. ) ;
#53735=CARTESIAN_POINT ( 'NONE',  ( 27.46979534332119854, 1440.913060388420035, 228.9356845949239982 ) ) ;
#53736=CARTESIAN_POINT ( 'NONE',  ( -21.33960867280000073, 1508.012995197530017, 227.2182461948980006 ) ) ;
#53738=ORIENTED_EDGE ( 'NONE', *, *, #91505, .F. ) ;
#53739=CIRCLE ( 'NONE', #19729, 2.000000000000068390 ) ;
#53742=CARTESIAN_POINT ( 'NONE',  ( 14.56320595439999899, 1474.359403032329965, 224.0680315863980070 ) ) ;
#53743=CARTESIAN_POINT ( 'NONE',  ( -6.972327688130000034, 1486.046393097330110, 182.7313348475980206 ) ) ;
#53744=CARTESIAN_POINT ( 'NONE',  ( -1.116585105924089969E-07, 1397.914279478820163, 196.1218459578329885 ) ) ;
#53745=CARTESIAN_POINT ( 'NONE',  ( 2.371440457460000317, 1490.912983831230122, 235.3311647238980129 ) ) ;
#53748=CARTESIAN_POINT ( 'NONE',  ( 25.29760786760000002, 1449.800867294439968, 211.5544486736880003 ) ) ;
#53754=CARTESIAN_POINT ( 'NONE',  ( 2.158908090871114016, 1417.717801426661936, 234.2951402407404373 ) ) ;
#53755=CARTESIAN_POINT ( 'NONE',  ( 0.1596481920543649791, 1486.478835695869975, 181.8160301856430010 ) ) ;
#53756=DIRECTION ( 'NONE',  ( 0.7835778714266642409, -0.02736314221910695482, 0.6206907264156240611 ) ) ;
#53758=CARTESIAN_POINT ( 'NONE',  ( -1.121218466020000193, 1416.837080248530128, 228.0853546194979913 ) ) ;
#53760=CARTESIAN_POINT ( 'NONE',  ( -20.55810159319999997, 1507.794327612029974, 189.9655093376980233 ) ) ;
#53762=ORIENTED_EDGE ( 'NONE', *, *, #74069, .T. ) ;
#53768=LINE ( 'NONE', #3356, #73301 ) ;
#53771=CARTESIAN_POINT ( 'NONE',  ( 13.01686471861349936, 1409.367619315190041, 216.4512120152259911 ) ) ;
#53772=CARTESIAN_POINT ( 'NONE',  ( 18.52319328460000136, 1425.707465110329849, 225.1076900885979910 ) ) ;
#53781=CARTESIAN_POINT ( 'NONE',  ( -11.29240054898340162, 1415.034069335250024, 195.6281518637269983 ) ) ;
#53785=CARTESIAN_POINT ( 'NONE',  ( 29.24997129405418761, 1509.943677684565046, 213.2686300063438125 ) ) ;
#53787=CARTESIAN_POINT ( 'NONE',  ( 2.403403406279999821, 1396.180594103330122, 220.9064825637979936 ) ) ;
#53788=CARTESIAN_POINT ( 'NONE',  ( 2.241849513110000025, 1417.743522105730108, 234.2089936445980243 ) ) ;
#53790=CARTESIAN_POINT ( 'NONE',  ( -19.23500960428314954, 1486.267560991677101, 189.5407332401421741 ) ) ;
#53795=CARTESIAN_POINT ( 'NONE',  ( 6.305024129259999555, 1422.156209412130011, 144.1468801376980196 ) ) ;
#53798=CARTESIAN_POINT ( 'NONE',  ( 41.64578063898380123, 1444.020661637949843, 135.8457820201300024 ) ) ;
#53800=CARTESIAN_POINT ( 'NONE',  ( 13.01666426059999893, 1409.302076636529819, 262.4458742036980539 ) ) ;
#53801=CARTESIAN_POINT ( 'NONE',  ( -21.04266092970000201, 1508.126368072830019, 192.1685821131979992 ) ) ;
#53802=CARTESIAN_POINT ( 'NONE',  ( -10.08898255699300073, 1425.184020547399996, 99.92021504015251310 ) ) ;
#53803=CARTESIAN_POINT ( 'NONE',  ( 3.062523615019999729E-14, 1419.211677883429957, 248.0989693021979861 ) ) ;
#53805=AXIS2_PLACEMENT_3D ( 'NONE', #49650, #50209, #8718 ) ;
#53806=LINE ( 'NONE', #61108, #19406 ) ;
#53807=CARTESIAN_POINT ( 'NONE',  ( -32.18001475150000346, 1422.275299834130237, 259.4130713564979942 ) ) ;
#53809=CARTESIAN_POINT ( 'NONE',  ( 29.09134681033120273, 1509.695701322400055, 209.5707846826050229 ) ) ;
#53811=CARTESIAN_POINT ( 'NONE',  ( 32.75710912790000151, 1451.616054398930146, 135.6209638249980003 ) ) ;
#53813=CARTESIAN_POINT ( 'NONE',  ( -2.500000000000000000, 1432.334889290770207, 157.4941654934979738 ) ) ;
#53815=CARTESIAN_POINT ( 'NONE',  ( 5.969656829619999883, 1509.201939557829974, 238.6262948603979908 ) ) ;
#53823=AXIS2_PLACEMENT_3D ( 'NONE', #49232, #57087, #66598 ) ;
#53825=CARTESIAN_POINT ( 'NONE',  ( -4.681481053319999752, 1470.480737942429869, 234.7256992237980171 ) ) ;
#53826=CARTESIAN_POINT ( 'NONE',  ( 1.760102192101790086, 1421.041668313049968, 183.1006875787430204 ) ) ;
#53829=CARTESIAN_POINT ( 'NONE',  ( 14.76019812800000075, 1485.703140196630102, 225.4605170203979867 ) ) ;
#53833=ORIENTED_EDGE ( 'NONE', *, *, #47341, .F. ) ;
#53834=CARTESIAN_POINT ( 'NONE',  ( 11.85939795343059977, 1431.868251362790033, 149.9622777773220150 ) ) ;
#53840=CARTESIAN_POINT ( 'NONE',  ( -17.22592482065197927, 1443.501467202829190, 162.9227486220069920 ) ) ;
#53841=CARTESIAN_POINT ( 'NONE',  ( 4.922541436569999540, 1508.072814005929786, 235.9300658385979830 ) ) ;
#53844=CARTESIAN_POINT ( 'NONE',  ( -5.307042958110000264, 1425.580209374029891, 186.3543675766980243 ) ) ;
#53845=CARTESIAN_POINT ( 'NONE',  ( 4.832498183603440189, 1410.233947744540046, 269.8672858344739893 ) ) ;
#53850=CARTESIAN_POINT ( 'NONE',  ( 0.02372484621392087142, 1410.241830673391405, 233.2188489835018004 ) ) ;
#53852=LINE ( 'NONE', #2342, #26082 ) ;
#53855=CARTESIAN_POINT ( 'NONE',  ( 18.01326382707690144, 1424.078348992020210, 225.1918633016099704 ) ) ;
#53858=CARTESIAN_POINT ( 'NONE',  ( 9.019386498959999443, 1419.938649402030023, 248.0989692945980210 ) ) ;
#53859=CARTESIAN_POINT ( 'NONE',  ( 19.74623141735625254, 1455.440022657526697, 226.3245780267467921 ) ) ;
#53869=CARTESIAN_POINT ( 'NONE',  ( -24.25306927760000164, 1442.945495109479907, 211.8921142785780205 ) ) ;
#53873=CARTESIAN_POINT ( 'NONE',  ( -8.888076702530000262, 1441.588620940000283, 186.2917108085980260 ) ) ;
#53874=CARTESIAN_POINT ( 'NONE',  ( -0.05095195904217150046, 1508.992415879220061, 179.2594346809810020 ) ) ;
#53875=CARTESIAN_POINT ( 'NONE',  ( 13.15671565689999944, 1428.802034784529951, 222.6511392629980151 ) ) ;
#53876=CARTESIAN_POINT ( 'NONE',  ( 12.10956687129965914, 1433.934677003899651, 149.7611593085945287 ) ) ;
#53877=CARTESIAN_POINT ( 'NONE',  ( 12.57627033670000039, 1417.420077678930056, 229.0684564266980203 ) ) ;
#53880=CARTESIAN_POINT ( 'NONE',  ( -16.10352984969999923, 1459.579123770429760, 228.9550806997980033 ) ) ;
#53882=CARTESIAN_POINT ( 'NONE',  ( 46.08680262619999723, 1436.858513228260108, 267.5959981427980097 ) ) ;
#53883=CARTESIAN_POINT ( 'NONE',  ( -17.17898592970000138, 1409.512963795129963, 223.3525532678980312 ) ) ;
#53884=EDGE_CURVE ( 'NONE', #48466, #94675, #18227, .T. ) ;
#53885=CARTESIAN_POINT ( 'NONE',  ( 17.95374924460000088, 1435.124687891739995, 145.3138471459980110 ) ) ;
#53886=CARTESIAN_POINT ( 'NONE',  ( 23.15253664929999999, 1508.008712515430034, 194.0884348405979836 ) ) ;
#53887=CARTESIAN_POINT ( 'NONE',  ( 29.52808524179070915, 1509.958252097621653, 207.2780779163062732 ) ) ;
#53888=CARTESIAN_POINT ( 'NONE',  ( 3.932775080253070321, 1448.980696629100066, 184.2693358254829832 ) ) ;
#53889=CARTESIAN_POINT ( 'NONE',  ( -45.67177343128329881, 1440.913044206929953, 266.1885934837860077 ) ) ;
#53890=CARTESIAN_POINT ( 'NONE',  ( 6.522563371079319161, 1422.592431503280068, 144.1528597180129907 ) ) ;
#53891=CARTESIAN_POINT ( 'NONE',  ( -41.16998753702269198, 1440.713062679589939, 135.8149046629820305 ) ) ;
#53893=CARTESIAN_POINT ( 'NONE',  ( -13.75903336753860096, 1409.893113308419970, 226.9379569541520141 ) ) ;
#53894=CARTESIAN_POINT ( 'NONE',  ( 13.90334061950979994, 1519.913060387329779, 234.5717402564966960 ) ) ;
#53895=CARTESIAN_POINT ( 'NONE',  ( -11.99325728100000177, 1441.735653989300090, 187.5768839477979668 ) ) ;
#53897=CARTESIAN_POINT ( 'NONE',  ( -33.93529465689999824, 1436.159566638689967, 136.2997917595980084 ) ) ;
#53898=CARTESIAN_POINT ( 'NONE',  ( -8.196734810833769203, 1456.222872452821093, 227.1897744870182123 ) ) ;
#53899=VERTEX_POINT ( 'NONE', #5899 ) ;
#53901=CARTESIAN_POINT ( 'NONE',  ( -11.73233732503739901, 1409.322762634679975, 218.3858963278959777 ) ) ;
#53905=CARTESIAN_POINT ( 'NONE',  ( -30.24616429450000155, 1467.598942926229938, 268.0936122245979618 ) ) ;
#53907=CARTESIAN_POINT ( 'NONE',  ( 0.1905848792942149983, 1419.866718629129991, 184.1430962726229836 ) ) ;
#53912=CARTESIAN_POINT ( 'NONE',  ( 11.96393163419999972, 1414.971352895729979, 220.7371289333979973 ) ) ;
#53913=CARTESIAN_POINT ( 'NONE',  ( -9.400735251840000473, 1432.346452651970139, 153.1462979580980175 ) ) ;
#53914=CARTESIAN_POINT ( 'NONE',  ( 0.7910245917146940808, 1426.918876941764893, 137.0999999980980135 ) ) ;
#53916=CARTESIAN_POINT ( 'NONE',  ( -3.611928636060000031, 1508.978187703030244, 180.0004874563979911 ) ) ;
#53917=CARTESIAN_POINT ( 'NONE',  ( -23.82773097239999771, 1410.240654944330117, 208.3948794269180098 ) ) ;
#53918=CLOSED_SHELL ( 'NONE', ( #82885, #92446, #95326, #40379, #11390, #54366, #13853, #82298, #11693, #13986, #14735, #82091, #79479, #64716, #76820, #44565, #50321, #31002, #84977, #5782, #14611, #91208, #63504, #10537, #9185, #102711, #48827, #24057, #81242, #1458, #47339, #1931, #107659, #59103, #85487, #27526, #99272, #89951, #99264, #77563, #108231, #48783, #22798, #82293, #3319, #57610, #14636, #61756, #18581, #71372, #61928, #61838, #51405, #72758, #38309, #59879, #95883, #96574, #106982, #30408, #106894, #18728, #7109, #85576, #93838, #102089, #100675, #14497, #49682, #84032, #50132, #67872, #80388, #40588, #70785, #101307, #73689, #62742, #85670, #88106, #42692, #28217, #65910, #24677, #60552, #35578, #38148, #21064, #66274, #57901, #24367, #12718, #75492, #71514, #3036, #43934, #53527, #25525, #21359, #13968, #23333, #5091, #10330, #50746, #47136, #72851, #35067, #31945, #17007, #106414, #53662, #98732, #10473, #81442, #65300, #17394, #66892, #55098, #71273, #75596, #45763, #70122, #63790, #27909, #103303, #52325, #28170, #41134, #82232, #74169, #103529, #60066, #102012, #6395, #65168, #74958, #57115, #104746, #71387, #41553, #56920, #96006, #90480, #10572, #36613, #30129, #15510, #36328, #105367, #91106, #90430, #82655, #38500, #50141, #109064, #2668, #7328, #70, #82499, #40436, #33763, #7025, #104712, #101564, #12852, #18184, #73513, #85955, #47485, #106430, #12367, #84852, #14768, #71996, #37785, #5935, #87299, #52339, #78612, #74, #36964, #30987, #70282, #98444, #69274, #101381, #12736, #81266, #11067, #50634, #51421, #4281, #89679, #23478, #42057, #81099, #97368, #80843, #108361, #37750, #97337, #43415, #1257, #46132, #52149, #42941, #7319, #13680, #8249, #15859, #104381, #72176, #81091, #29632, #41140, #45489, #57245, #89292, #61016, #28080, #89330, #59883, #110283, #22519, #18667, #87904, #100191, #102096, #48675, #63087, #47647, #50311, #56510, #45635, #93086, #76689, #36756, #108419, #79249, #71675, #94270, #45342, #13949, #74051, #74932, #84541, #58372, #15941, #52027, #59031, #59706, #103081, #52237, #107290, #2949, #29146, #22529, #45381, #89799, #98802, #42814, #20507, #23570, #108191, #84276, #15168, #33323, #12453, #81758, #12400, #68270, #58008, #12627, #98206, #84380, #96787, #67130, #95152, #105146, #61417, #94576, #74026, #75422, #34911, #69232, #65257, #89852, #25406, #31797, #2421, #6371, #49450, #35365, #65217, #1691, #108131, #84282, #5794, #93829, #59253, #13198, #35209, #100000, #60237, #61074, #3049, #58241, #38747, #46248, #22138, #89210, #108411, #1453, #35662, #73429, #101414, #46263, #102800, #74020, #102806, #101598, #20953, #87042, #42645, #78987, #64572, #54809, #38013, #20199, #109845, #26233, #75104, #70817, #105545, #2565, #74929, #98655, #45305, #85768, #853, #76125, #52849, #82633, #51506, #58499, #26153, #93959, #28858, #26750, #58842, #87854, #36355, #57240, #76571, #82648, #109541, #59307, #52941, #73577, #67302, #109701, #35820, #101081, #101678, #85621, #15818, #84242, #92758, #24036, #100656, #81870, #2393, #69322, #63198, #16491, #47397, #107615, #59123, #55591, #108942, #39025, #87063, #91863, #16141, #46880, #34704, #63473, #80001, #98291, #7149, #74201, #79741, #52280, #52571, #985, #66758, #66083, #1541, #1794, #108123, #103313, #32427, #15301, #84413, #94469, #41320, #59434, #7164, #75987, #62708, #38591, #82839, #9083, #33819, #64452, #76749, #87139, #109658, #35073, #58753, #100056, #12544, #50891, #29429, #105028, #68289, #80293, #56193, #91823, #3723, #22168, #77548, #75292, #71282, #22658, #6250, #79779, #22678, #79711, #107001, #30299, #352, #43800, #60648, #80529, #13056, #55218, #67190, #40930, #85275, #110083, #59141, #68608, #109341, #16099, #57606, #92629, #26032, #74308, #18776, #15696, #81595, #11488, #68590, #19437, #89448, #76927, #72075, #56216, #23617, #38663, #75528, #58306, #97281, #9582, #76161, #65326, #63061, #4942, #51699, #46420, #75548, #90584, #17170, #26188, #31635, #62499, #5491, #84861, #107179, #12491, #93616, #99712, #67616, #66411, #8428, #46289, #63805, #78911, #27491, #61308, #49410, #47029, #99274, #69378, #26854, #68870, #74210, #64464, #67522, #11729, #78779, #89979, #1641, #86261, #78059, #1104, #14588, #37522, #70150, #84397, #39846, #41155, #72441, #10447, #32943, #76753, #34308, #96698, #71545, #38139, #71557, #62453, #79104, #32915, #104965, #28275, #76341, #26259, #89672, #50550, #27531, #192, #4882, #100942, #13178, #4546, #98118, #86995, #52886, #59921, #76172, #6875, #48612, #4355, #89896, #7186, #89194, #98809, #88968, #61901, #56303, #22646, #99911, #76789, #24477, #12435, #3151, #99909, #39200, #107926, #19258, #35894, #101074, #7051, #23398, #61034, #2912, #30164, #39745, #30764, #41920, #48296, #74765 ) ) ;
#53919=CARTESIAN_POINT ( 'NONE',  ( 17.16585544539999830, 1415.931391677429929, 203.8399221076179799 ) ) ;
#53920=CARTESIAN_POINT ( 'NONE',  ( -11.83559671189999918, 1415.245980412430072, 195.4349966776979670 ) ) ;
#53922=CARTESIAN_POINT ( 'NONE',  ( 22.91612949529999810, 1409.877774706829769, 211.9495050228480011 ) ) ;
#53925=CARTESIAN_POINT ( 'NONE',  ( -5.369163863342579113, 1427.164133926789873, 153.2148359060929863 ) ) ;
#53928=FACE_OUTER_BOUND ( 'NONE', #23825, .T. ) ;
#53931=CARTESIAN_POINT ( 'NONE',  ( -22.87440001419999902, 1415.994159370630086, 211.5426778979280016 ) ) ;
#53932=CARTESIAN_POINT ( 'NONE',  ( -1.244790792857130013, 1420.670971867490152, 184.3462124761589962 ) ) ;
#53935=CARTESIAN_POINT ( 'NONE',  ( -23.60070218908893480, 1435.435984317846305, 213.5551715964222979 ) ) ;
#53936=CARTESIAN_POINT ( 'NONE',  ( -18.40312947852670078, 1485.456034533320008, 189.1500380655480171 ) ) ;
#53938=CARTESIAN_POINT ( 'NONE',  ( -4.274194808379749411, 1441.075114845419876, 157.3205200675280082 ) ) ;
#53941=EDGE_LOOP ( 'NONE', ( #68540, #62041, #75303 ) ) ;
#53943=ORIENTED_EDGE ( 'NONE', *, *, #21399, .F. ) ;
#53946=CARTESIAN_POINT ( 'NONE',  ( 0.8041763403130000043, 1426.566393376330097, 144.1938086916980239 ) ) ;
#53947=CARTESIAN_POINT ( 'NONE',  ( 4.665393456780000392, 1427.510941591930077, 123.0297916884979941 ) ) ;
#53948=CARTESIAN_POINT ( 'NONE',  ( 27.74152896581870209, 1446.393007474679962, 137.1637341980689939 ) ) ;
#53950=CARTESIAN_POINT ( 'NONE',  ( 1.765878059339999862, 1488.173956647230170, 181.9972861322979725 ) ) ;
#53952=CARTESIAN_POINT ( 'NONE',  ( 7.289026058960000221, 1410.103226084029757, 230.7281513803979749 ) ) ;
#53955=CARTESIAN_POINT ( 'NONE',  ( 41.56943536068610001, 1444.920853409699930, 134.0999999984259716 ) ) ;
#53958=CARTESIAN_POINT ( 'NONE',  ( -9817.198717879920878, 2837.742859910730203, 1424.354596106799818 ) ) ;
#53960=CARTESIAN_POINT ( 'NONE',  ( 13.85413686636590036, 1434.981310748690021, 148.6151550497299922 ) ) ;
#53962=ORIENTED_EDGE ( 'NONE', *, *, #85411, .T. ) ;
#53963=ORIENTED_EDGE ( 'NONE', *, *, #62089, .F. ) ;
#53966=CARTESIAN_POINT ( 'NONE',  ( -0.9163463255799999541, 1464.976965922729960, 237.2656658263979921 ) ) ;
#53967=CARTESIAN_POINT ( 'NONE',  ( 21.15490488532373448, 1450.943175079559978, 144.2761602908674945 ) ) ;
#53968=CARTESIAN_POINT ( 'NONE',  ( -2.924053139080000197, 1485.138221895729885, 183.1581825105979817 ) ) ;
#53973=CARTESIAN_POINT ( 'NONE',  ( 4.227393864177829919, 1446.270024740570079, 165.6814982219489991 ) ) ;
#53975=ORIENTED_EDGE ( 'NONE', *, *, #96912, .F. ) ;
#53977=ORIENTED_EDGE ( 'NONE', *, *, #80072, .F. ) ;
#53978=CARTESIAN_POINT ( 'NONE',  ( 26.67958435172820231, 1440.913060387330006, 244.1583708425140173 ) ) ;
#53980=ORIENTED_EDGE ( 'NONE', *, *, #53441, .F. ) ;
#53982=CARTESIAN_POINT ( 'NONE',  ( -14.27906159650000006, 1409.411696205929957, 191.9865084241980071 ) ) ;
#53984=CARTESIAN_POINT ( 'NONE',  ( -24.67145409169999581, 1441.066589285630016, 210.6900421876080145 ) ) ;
#53988=CARTESIAN_POINT ( 'NONE',  ( -12.84999653021897359, 1434.699229520601421, 147.0734321989873763 ) ) ;
#53991=CARTESIAN_POINT ( 'NONE',  ( 9.888958272120000004, 1463.772371499329893, 232.6549650238979723 ) ) ;
#54006=CARTESIAN_POINT ( 'NONE',  ( 8.718798080230000025, 1462.898524229230134, 232.0462147568979958 ) ) ;
#54010=CARTESIAN_POINT ( 'NONE',  ( 2.190948469950000366, 1413.140243969430003, 231.9855873312979782 ) ) ;
#54011=CARTESIAN_POINT ( 'NONE',  ( -22.42321380570000144, 1451.074909188629817, 219.8762963758979936 ) ) ;
#54012=CIRCLE ( 'NONE', #23504, 9.000000000000007105 ) ;
#54013=CARTESIAN_POINT ( 'NONE',  ( -23.59318075118283531, 1411.097233843727054, 206.6698092424495599 ) ) ;
#54014=CARTESIAN_POINT ( 'NONE',  ( 5.372020988824510290, 1428.211245194210051, 153.7601568675739827 ) ) ;
#54019=CARTESIAN_POINT ( 'NONE',  ( 1.327512982840000078, 1406.079504512129915, 269.0450431314979483 ) ) ;
#54021=CARTESIAN_POINT ( 'NONE',  ( 43.48865956637619945, 1446.139721542620009, 270.3367078615700052 ) ) ;
#54022=CARTESIAN_POINT ( 'NONE',  ( 2.478548031669999929, 1437.283191558279896, 157.6756789685979925 ) ) ;
#54024=CARTESIAN_POINT ( 'NONE',  ( 11.60004869886325451, 1423.252659004586349, 137.0072935635085116 ) ) ;
#54026=CARTESIAN_POINT ( 'NONE',  ( -43.52170781963269519, 1440.913060407769990, 263.8029430533659934 ) ) ;
#54027=CARTESIAN_POINT ( 'NONE',  ( 36.90203174740399561, 1449.595941984130150, 136.2855500997040110 ) ) ;
#54030=CARTESIAN_POINT ( 'NONE',  ( 1.453744393529480039, 1450.692426104239985, 154.2448216313819955 ) ) ;
#54032=CARTESIAN_POINT ( 'NONE',  ( 7.105427357599999217E-15, 1418.913060387330006, 172.2701767054979882 ) ) ;
#54034=CARTESIAN_POINT ( 'NONE',  ( -26.42894385079999964, 1421.320559242730042, 262.6648722463980334 ) ) ;
#54035=CARTESIAN_POINT ( 'NONE',  ( -1.441072598602595400, 1450.659596873665123, 182.0284431214944618 ) ) ;
#54036=CARTESIAN_POINT ( 'NONE',  ( -22.91663120903140083, 1507.606285602550088, 207.6071078552859888 ) ) ;
#54037=CARTESIAN_POINT ( 'NONE',  ( -1.318284353409999943, 1475.306440821630076, 269.4981144188980124 ) ) ;
#54038=CARTESIAN_POINT ( 'NONE',  ( -32.05911371000000543, 1451.793557196030179, 134.7701858639979946 ) ) ;
#54039=CARTESIAN_POINT ( 'NONE',  ( -28.77213280049999966, 1509.917805404830006, 211.3774502238480295 ) ) ;
#54040=CARTESIAN_POINT ( 'NONE',  ( -3.910181740847316956, 1448.296520225016820, 185.0509912937746719 ) ) ;
#54042=CIRCLE ( 'NONE', #36109, 12.50000000000001066 ) ;
#54043=CARTESIAN_POINT ( 'NONE',  ( -17.80652095830000192, 1415.128105756529976, 207.8722581125280158 ) ) ;
#54045=CARTESIAN_POINT ( 'NONE',  ( 26.00338574347900078, 1435.702077567190145, 136.3120532782230043 ) ) ;
#54046=CARTESIAN_POINT ( 'NONE',  ( -3.088399681877699532, 1396.020909680820068, 219.6995886521329737 ) ) ;
#54049=CARTESIAN_POINT ( 'NONE',  ( -16.42060166099630081, 1409.511629218500048, 225.2012082830180191 ) ) ;
#54052=CARTESIAN_POINT ( 'NONE',  ( -20.61546995289999984, 1508.365016819430139, 190.3615313974979983 ) ) ;
#54053=CARTESIAN_POINT ( 'NONE',  ( 2.325354419860000021, 1408.994263553030123, 230.2593898277980031 ) ) ;
#54054=CARTESIAN_POINT ( 'NONE',  ( 10.66436153279999921, 1425.356347891630094, 112.6539006775979885 ) ) ;
#54057=CARTESIAN_POINT ( 'NONE',  ( -11.23388613411650638, 1445.063428794548372, 205.3674499604519212 ) ) ;
#54068=CARTESIAN_POINT ( 'NONE',  ( -41.65882839649999880, 1443.939635522049912, 136.1335186928980079 ) ) ;
#54070=CARTESIAN_POINT ( 'NONE',  ( -13.35522314810000033, 1409.379435056429884, 191.4683303614979764 ) ) ;
#54074=CARTESIAN_POINT ( 'NONE',  ( 0.1596058210269999944, 1486.508833526429953, 181.8147405216979848 ) ) ;
#54075=CARTESIAN_POINT ( 'NONE',  ( 20.15452300067990166, 1507.845791525220193, 189.3412703910400126 ) ) ;
#54077=CARTESIAN_POINT ( 'NONE',  ( -40.10254738438180055, 1447.671539697419803, 136.3432379383139903 ) ) ;
#54080=CARTESIAN_POINT ( 'NONE',  ( -2.500000000000000000, 1448.349747921640073, 163.1876093918550055 ) ) ;
#54081=CARTESIAN_POINT ( 'NONE',  ( 9.366452427309480910, 1396.240144116259899, 215.0016878971990195 ) ) ;
#54082=CARTESIAN_POINT ( 'NONE',  ( 11.93818824289999903, 1433.480083226980014, 149.8972169559980046 ) ) ;
#54083=CARTESIAN_POINT ( 'NONE',  ( -1.525162025860949955, 1406.078293633129988, 269.0451533397849744 ) ) ;
#54084=CARTESIAN_POINT ( 'NONE',  ( 41.49211893279999686, 1443.779781417970071, 136.5764383342979897 ) ) ;
#54097=CARTESIAN_POINT ( 'NONE',  ( 11.99296739220000063, 1415.426952351230057, 223.0765513814980068 ) ) ;
#54099=CARTESIAN_POINT ( 'NONE',  ( -42.06231979437640689, 1440.913089571769888, 269.6487552725350270 ) ) ;
#54100=CARTESIAN_POINT ( 'NONE',  ( 11.87499106303466867, 1433.007134994034459, 150.0931956004157541 ) ) ;
#54101=PLANE ( 'NONE',  #31170 ) ;
#54102=CARTESIAN_POINT ( 'NONE',  ( -10.94435082380000068, 1409.295245542529983, 227.9482308656980081 ) ) ;
#54103=CARTESIAN_POINT ( 'NONE',  ( -7.631942175340000745, 1445.746736454730126, 183.8563304949979909 ) ) ;
#54104=VERTEX_POINT ( 'NONE', #35508 ) ;
#54106=CARTESIAN_POINT ( 'NONE',  ( 1.712115010999669895, 1498.987102177869929, 236.1549197538539886 ) ) ;
#54107=CARTESIAN_POINT ( 'NONE',  ( -2.446860826606596540, 1485.861696308259752, 182.3251189179504479 ) ) ;
#54108=CARTESIAN_POINT ( 'NONE',  ( 15.76866870594087544, 1506.436298846738964, 224.4414140739798995 ) ) ;
#54109=CARTESIAN_POINT ( 'NONE',  ( 40.36598731044649924, 1427.956512246619923, 270.3380825022459817 ) ) ;
#54111=AXIS2_PLACEMENT_3D ( 'NONE', #26820, #95133, #41973 ) ;
#54113=CARTESIAN_POINT ( 'NONE',  ( 0.01998521568534358459, 1507.240582288022779, 237.3618852806027917 ) ) ;
#54117=ORIENTED_EDGE ( 'NONE', *, *, #28893, .T. ) ;
#54118=CARTESIAN_POINT ( 'NONE',  ( 0.05765900138281670334, 1424.300292107330051, 227.5770399881510002 ) ) ;
#54119=CARTESIAN_POINT ( 'NONE',  ( -6.024103323599999449, 1420.442878368530046, 231.9530688324979906 ) ) ;
#54121=EDGE_LOOP ( 'NONE', ( #46646, #2179, #85471, #10619 ) ) ;
#54123=CARTESIAN_POINT ( 'NONE',  ( 18.95884658670000178, 1416.837177087930058, 210.4637960667579932 ) ) ;
#54125=CARTESIAN_POINT ( 'NONE',  ( 18.19935571605649827, 1478.711533688430109, 228.8851065908069984 ) ) ;
#54128=CARTESIAN_POINT ( 'NONE',  ( -0.1416905494029999935, 1408.918008330330167, 231.7806227986979764 ) ) ;
#54129=CARTESIAN_POINT ( 'NONE',  ( 0.1336799119265279778, 1420.462095040470103, 182.7174734993599827 ) ) ;
#54131=CARTESIAN_POINT ( 'NONE',  ( 18.63535449669999977, 1508.532394786529949, 188.3246405779979966 ) ) ;
#54136=ORIENTED_EDGE ( 'NONE', *, *, #110279, .F. ) ;
#54137=CARTESIAN_POINT ( 'NONE',  ( 11.60004869885205103, 1426.752151907737016, 134.4009923342575235 ) ) ;
#54138=FACE_OUTER_BOUND ( 'NONE', #93425, .T. ) ;
#54141=CARTESIAN_POINT ( 'NONE',  ( -27.61919202599030143, 1509.794165504519924, 201.0446006437040296 ) ) ;
#54143=CARTESIAN_POINT ( 'NONE',  ( 18.50064172359999759, 1416.067629290630066, 209.7633006632509876 ) ) ;
#54144=CARTESIAN_POINT ( 'NONE',  ( -18.29297708900000075, 1425.080551783529927, 226.8406087971980014 ) ) ;
#54145=CARTESIAN_POINT ( 'NONE',  ( -22.37002394150000129, 1435.422720654210025, 141.4343147051980054 ) ) ;
#54147=CARTESIAN_POINT ( 'NONE',  ( 17.00461789839999938, 1428.771240263530217, 191.0631962805980208 ) ) ;
#54148=CARTESIAN_POINT ( 'NONE',  ( 1.039061157835060145, 1409.452459111349981, 232.6817842876129987 ) ) ;
#54149=CARTESIAN_POINT ( 'NONE',  ( -4.518180742295140181E-06, 1509.047264790930058, 179.1218459713510072 ) ) ;
#54151=B_SPLINE_CURVE_WITH_KNOTS ( 'NONE', 3,
 ( #70146, #87471, #38149, #72329, #36502, #44932, #27003, #70698, #45485, #79627, #2931, #37047, #62861, #88571, #66140, #30841, #83444, #106459, #74527, #64483, #72867, #73419, #99686, #4558, #99135, #63931, #100263, #39807, #90750, #98598, #23542, #12935, #57183, #6194, #91307, #73967, #107555, #21862, #6739, #40897, #57734, #22978, #56061 ),
 .UNSPECIFIED., .F., .F.,
 ( 4, 3, 3, 3, 3, 3, 3, 3, 3, 3, 3, 3, 3, 3, 4 ),
 ( -1.999999998298850112, -1.913740754577760050, -1.770581378075359869, -1.625369123173900032, -1.478912460535070084, -1.330584048827429866, -1.181323947785520190, -1.031451248172440049, -0.8813277763345430671, -0.7315909901474011434, -0.5826190372449879806, -0.4347499881818699397, -0.2882457491577810060, -0.1432907418691580226, -3.793644199889811830E-06 ),
 .UNSPECIFIED. ) ;
#54153=CARTESIAN_POINT ( 'NONE',  ( 1.552003028135559903, 1415.724942522449965, 190.6284710308260060 ) ) ;
#54154=CARTESIAN_POINT ( 'NONE',  ( 26.60755023664092533, 1509.169828502769633, 216.8086214747193310 ) ) ;
#54156=CARTESIAN_POINT ( 'NONE',  ( -24.17602266159999758, 1436.642150718030052, 210.9689740457980065 ) ) ;
#54160=CARTESIAN_POINT ( 'NONE',  ( -10.98649148439782230, 1433.355625015306487, 151.7689635225571578 ) ) ;
#54161=CARTESIAN_POINT ( 'NONE',  ( -24.89939545272470056, 1440.978110083920001, 210.4300214511639808 ) ) ;
#54162=CARTESIAN_POINT ( 'NONE',  ( -22.70690864871570014, 1509.745348826289955, 188.8675591137879906 ) ) ;
#54163=B_SPLINE_CURVE_WITH_KNOTS ( 'NONE', 3,
 ( #57590, #73834, #99549, #67093, #90048, #48072 ),
 .UNSPECIFIED., .F., .F.,
 ( 4, 2, 4 ),
 ( -0.04927314538870530142, -0.02504330357724929984, 0.000000000000000000 ),
 .UNSPECIFIED. ) ;
#54168=CARTESIAN_POINT ( 'NONE',  ( 18.64672481363430379, 1416.851343896850040, 209.6839434896919840 ) ) ;
#54170=CARTESIAN_POINT ( 'NONE',  ( -13.02294863090000021, 1410.743074594430027, 220.9912686835980082 ) ) ;
#54174=ORIENTED_EDGE ( 'NONE', *, *, #90884, .F. ) ;
#54177=CARTESIAN_POINT ( 'NONE',  ( 13.20177346510000049, 1508.090222725930062, 233.1545818560979910 ) ) ;
#54178=CARTESIAN_POINT ( 'NONE',  ( 13.13028867889093831, 1443.050727194750380, 169.4013764991958624 ) ) ;
#54179=CARTESIAN_POINT ( 'NONE',  ( 39.93378919416216632, 1431.329204280520116, 269.6090686156236416 ) ) ;
#54180=CARTESIAN_POINT ( 'NONE',  ( -16.98088719460000107, 1467.669747903330062, 255.1565003930980140 ) ) ;
#54185=CARTESIAN_POINT ( 'NONE',  ( -19.12700648050000041, 1485.852572981329786, 189.6184868647980011 ) ) ;
#54186=CARTESIAN_POINT ( 'NONE',  ( 5.281843194899999538, 1410.032092550429979, 186.4939589901979957 ) ) ;
#54187=CARTESIAN_POINT ( 'NONE',  ( 5.210622763619999986, 1424.684339385929889, 185.7917198324980177 ) ) ;
#54191=CARTESIAN_POINT ( 'NONE',  ( 0.05914941296659999292, 1451.662743609429981, 154.0810085997979968 ) ) ;
#54194=ORIENTED_EDGE ( 'NONE', *, *, #83645, .F. ) ;
#54196=EDGE_CURVE ( 'NONE', #66425, #20723, #54368, .T. ) ;
#54199=CARTESIAN_POINT ( 'NONE',  ( -12.94491415900000142, 1469.989349686730066, 269.3560571862979600 ) ) ;
#54201=CARTESIAN_POINT ( 'NONE',  ( 9.325873406849999120E-15, 1443.913060387330006, 155.8032249175980155 ) ) ;
#54203=CARTESIAN_POINT ( 'NONE',  ( -14.26333328529999989, 1452.396687225829965, 223.0069981153980052 ) ) ;
#54204=CARTESIAN_POINT ( 'NONE',  ( 4.561655832029999580, 1453.313060387329870, 189.3102883226979998 ) ) ;
#54205=EDGE_CURVE ( 'NONE', #2071, #84627, #107889, .T. ) ;
#54206=CARTESIAN_POINT ( 'NONE',  ( -0.4967073565345429542, 1415.438070636819930, 233.3911243540180180 ) ) ;
#54210=CARTESIAN_POINT ( 'NONE',  ( -45.16361212240940404, 1433.663185462369711, 268.2380307924040039 ) ) ;
#54214=ORIENTED_EDGE ( 'NONE', *, *, #37390, .T. ) ;
#54217=CARTESIAN_POINT ( 'NONE',  ( -21.92444879440000349, 1509.678679009930192, 190.3921826488979718 ) ) ;
#54218=CARTESIAN_POINT ( 'NONE',  ( -15.02738316969999843, 1410.405006173230049, 190.7838349957980029 ) ) ;
#54227=ORIENTED_EDGE ( 'NONE', *, *, #49510, .F. ) ;
#54228=CARTESIAN_POINT ( 'NONE',  ( -17.14221562505780128, 1410.074669699509968, 270.0731992386910179 ) ) ;
#54230=CARTESIAN_POINT ( 'NONE',  ( -27.23873044170000313, 1435.448403991980058, 135.2737774014979948 ) ) ;
#54234=ORIENTED_EDGE ( 'NONE', *, *, #80484, .F. ) ;
#54236=CARTESIAN_POINT ( 'NONE',  ( 45.55971553987971845, 1442.925831206288649, 268.9768701855822428 ) ) ;
#54238=CARTESIAN_POINT ( 'NONE',  ( 3.626131424302643236, 1424.567267193513317, 184.5641229779018317 ) ) ;
#54239=CARTESIAN_POINT ( 'NONE',  ( -0.002896907270607540063, 1408.914043369009960, 186.4050159525630193 ) ) ;
#54241=CARTESIAN_POINT ( 'NONE',  ( -18.60802716234039877, 1415.890045856200004, 207.5710866051209962 ) ) ;
#54242=CARTESIAN_POINT ( 'NONE',  ( -17.99573535500000077, 1435.780247436960053, 226.7275259980980024 ) ) ;
#54243=CARTESIAN_POINT ( 'NONE',  ( 5.319351013645369441, 1475.836928872520048, 266.9609103791869984 ) ) ;
#54244=CARTESIAN_POINT ( 'NONE',  ( -1.110837182595547201, 1467.058882683617185, 235.4628246916891783 ) ) ;
#54245=CARTESIAN_POINT ( 'NONE',  ( 7.144588282590000006, 1446.888283566400105, 185.2265207297980112 ) ) ;
#54247=EDGE_LOOP ( 'NONE', ( #33648, #93711, #3446, #96273 ) ) ;
#54248=CARTESIAN_POINT ( 'NONE',  ( 21.75593670543157288, 1411.033169560906572, 216.6130940229133728 ) ) ;
#54249=CARTESIAN_POINT ( 'NONE',  ( 1.470204857257540132, 1486.276663417369946, 182.0220377839359855 ) ) ;
#54250=ORIENTED_EDGE ( 'NONE', *, *, #15906, .F. ) ;
#54252=CARTESIAN_POINT ( 'NONE',  ( 25.07944958343669839, 1451.314395594800089, 137.5314305375449919 ) ) ;
#54253=CARTESIAN_POINT ( 'NONE',  ( -22.12673812478050195, 1409.685743108969973, 209.8966867368829980 ) ) ;
#54256=CARTESIAN_POINT ( 'NONE',  ( 21.03603951619999890, 1411.006939957029999, 199.9012218170380208 ) ) ;
#54257=CARTESIAN_POINT ( 'NONE',  ( 28.38894342380001490, 1444.994950788470987, 176.3316754166978910 ) ) ;
#54258=CARTESIAN_POINT ( 'NONE',  ( 17.40898828889999805, 1410.017881507529864, 225.1690343474979841 ) ) ;
#54259=CARTESIAN_POINT ( 'NONE',  ( -21.53076271701005240, 1429.163937548285730, 219.2231547731813919 ) ) ;
#54260=CARTESIAN_POINT ( 'NONE',  ( 0.5791559346779789896, 1451.093235343550077, 182.2615577885279947 ) ) ;
#54268=CARTESIAN_POINT ( 'NONE',  ( -0.3894626618421410114, 1409.116368191170068, 232.4611552482589900 ) ) ;
#54271=EDGE_CURVE ( 'NONE', #80182, #43125, #22528, .T. ) ;
#54272=CARTESIAN_POINT ( 'NONE',  ( -39.57266623269340045, 1446.793018509809826, 136.6753323040810244 ) ) ;
#54274=CARTESIAN_POINT ( 'NONE',  ( -19.00000000000000000, 1440.913060387330006, 209.1218459616979999 ) ) ;
#54277=CARTESIAN_POINT ( 'NONE',  ( -35.31631333859999700, 1462.797633448130000, 269.2416639850980005 ) ) ;
#54281=ORIENTED_EDGE ( 'NONE', *, *, #71422, .F. ) ;
#54285=CARTESIAN_POINT ( 'NONE',  ( -19.14870982884896478, 1485.551433189229783, 189.6725793120419894 ) ) ;
#54289=CARTESIAN_POINT ( 'NONE',  ( 25.53333737239999834, 1449.803091282509968, 210.5361858600879827 ) ) ;
#54291=CARTESIAN_POINT ( 'NONE',  ( -14.69790105030000049, 1509.426322401930065, 234.2227378565979734 ) ) ;
#54293=CARTESIAN_POINT ( 'NONE',  ( 1.275935789888901439, 1416.411555056025691, 232.9857727263382117 ) ) ;
#54298=CARTESIAN_POINT ( 'NONE',  ( -0.9464041199730000020, 1451.043408575430021, 182.5116545072980045 ) ) ;
#54301=CARTESIAN_POINT ( 'NONE',  ( -3.013235680273810058, 1440.805531640480012, 157.2037855315670072 ) ) ;
#54302=CARTESIAN_POINT ( 'NONE',  ( -16.88248175295160181, 1414.913057834419988, 207.9312177863439786 ) ) ;
#54303=ORIENTED_EDGE ( 'NONE', *, *, #81452, .T. ) ;
#54305=ORIENTED_EDGE ( 'NONE', *, *, #9303, .F. ) ;
#54308=CARTESIAN_POINT ( 'NONE',  ( -1.808982817633178586, 1509.008938970973759, 238.7270464612732894 ) ) ;
#54309=EDGE_CURVE ( 'NONE', #94269, #38319, #90419, .T. ) ;
#54314=CARTESIAN_POINT ( 'NONE',  ( 10.01139723437129980, 1409.262666079100200, 220.2341507100319973 ) ) ;
#54317=CARTESIAN_POINT ( 'NONE',  ( -17.50241060500000145, 1410.867113670829895, 192.6239589323980113 ) ) ;
#54326=EDGE_CURVE ( 'NONE', #67527, #91965, #8912, .T. ) ;
#54327=CARTESIAN_POINT ( 'NONE',  ( 28.55528612434519076, 1509.910687724684976, 216.1464615550907808 ) ) ;
#54329=CARTESIAN_POINT ( 'NONE',  ( -28.24318413590000176, 1508.132100804830088, 209.6063173613950141 ) ) ;
#54333=CARTESIAN_POINT ( 'NONE',  ( -25.79637238690366630, 1436.656401712661818, 137.0607721643913521 ) ) ;
#54335=CARTESIAN_POINT ( 'NONE',  ( -13.07366137487360014, 1434.838828088369837, 149.4347582794279674 ) ) ;
#54337=CARTESIAN_POINT ( 'NONE',  ( 1.342110471609999856, 1416.822692809430009, 190.1636843969979793 ) ) ;
#54339=DIRECTION ( 'NONE',  ( -0.5969061220947670110, 0.8023110876747169273, 0.000000000000000000 ) ) ;
#54344=CARTESIAN_POINT ( 'NONE',  ( -3.400317100450000321E-09, 1409.477337460029958, 259.9484463448980023 ) ) ;
#54345=CARTESIAN_POINT ( 'NONE',  ( -23.50062168420000219, 1488.679648898629921, 197.2621013953979912 ) ) ;
#54346=CARTESIAN_POINT ( 'NONE',  ( -11.08399775210000016, 1426.906423284629909, 96.73292351169779124 ) ) ;
#54349=CARTESIAN_POINT ( 'NONE',  ( -29.43658766380000102, 1426.244274385030167, 250.1802633625980263 ) ) ;
#54350=CARTESIAN_POINT ( 'NONE',  ( 20.46980501909149908, 1509.670375995580116, 230.6918749470270029 ) ) ;
#54352=CARTESIAN_POINT ( 'NONE',  ( -24.08426305480000451, 1411.115211393229856, 208.6111285346999864 ) ) ;
#54354=CARTESIAN_POINT ( 'NONE',  ( -5.386547031804509444, 1432.371148517990150, 154.6078450733400018 ) ) ;
#54356=B_SPLINE_CURVE_WITH_KNOTS ( 'NONE', 5,
 ( #96259, #86750, #19534, #28503, #86194, #80008 ),
 .UNSPECIFIED., .F., .F.,
 ( 6, 6 ),
 ( -158.0163518690000046, -29.52656374809998852 ),
 .UNSPECIFIED. ) ;
#54358=CARTESIAN_POINT ( 'NONE',  ( 38.39760561534620109, 1443.174109818610077, 137.1306153789140012 ) ) ;
#54359=ORIENTED_EDGE ( 'NONE', *, *, #93859, .T. ) ;
#54360=VERTEX_POINT ( 'NONE', #16882 ) ;
#54363=VERTEX_POINT ( 'NONE', #9069 ) ;
#54364=CARTESIAN_POINT ( 'NONE',  ( -0.04561968975039999707, 1424.313206842929958, 227.6130361704979919 ) ) ;
#54366=ADVANCED_FACE ( 'NONE', ( #35374 ), #43238, .T. ) ;
#54367=CARTESIAN_POINT ( 'NONE',  ( 0.3651880982969999967, 1451.159209398729899, 182.5636267636980108 ) ) ;
#54368=B_SPLINE_CURVE_WITH_KNOTS ( 'NONE', 5,
 ( #94294, #104368, #45046, #9213, #17572, #10302 ),
 .UNSPECIFIED., .F., .F.,
 ( 6, 6 ),
 ( 0.000000000000000000, 11.48858425020000240 ),
 .UNSPECIFIED. ) ;
#54369=CARTESIAN_POINT ( 'NONE',  ( -11.79378255399999986, 1479.764572231929833, 232.1975610188979999 ) ) ;
#54372=CARTESIAN_POINT ( 'NONE',  ( 11.73709356449999852, 1426.695943566229971, 144.1748013792980032 ) ) ;
#54373=CARTESIAN_POINT ( 'NONE',  ( -11.91079909292840000, 1414.913060387399810, 220.1328973762649923 ) ) ;
#54374=CARTESIAN_POINT ( 'NONE',  ( 15.59061307620000036, 1507.637957935030045, 225.5593735085980143 ) ) ;
#54377=ORIENTED_EDGE ( 'NONE', *, *, #49642, .F. ) ;
#54378=CARTESIAN_POINT ( 'NONE',  ( 11.86457202409800082, 1432.229187294399935, 149.9813147920380061 ) ) ;
#54380=ORIENTED_EDGE ( 'NONE', *, *, #34757, .T. ) ;
#54381=ORIENTED_EDGE ( 'NONE', *, *, #28433, .T. ) ;
#54384=CARTESIAN_POINT ( 'NONE',  ( -21.62302451687340010, 1409.668153042179938, 204.8506916389789865 ) ) ;
#54386=CARTESIAN_POINT ( 'NONE',  ( -4.653266759930000163, 1425.827076154429960, 186.2156706901979817 ) ) ;
#54387=CARTESIAN_POINT ( 'NONE',  ( 0.9453222513162000684, 1410.394701501269992, 269.3347007296789570 ) ) ;
#54391=CARTESIAN_POINT ( 'NONE',  ( -20.61514741043744792, 1509.679810159945191, 230.5809340611079108 ) ) ;
#54393=LINE ( 'NONE', #69543, #8826 ) ;
#54395=CARTESIAN_POINT ( 'NONE',  ( 14.76593576959999865, 1434.994542537580173, 195.9393237157979968 ) ) ;
#54397=CARTESIAN_POINT ( 'NONE',  ( 17.70992611605910128, 1414.252993047500013, 224.9060675817109995 ) ) ;
#54399=VERTEX_POINT ( 'NONE', #69006 ) ;
#54400=CARTESIAN_POINT ( 'NONE',  ( 1.199040866600000048E-14, 1416.825952160429779, 255.3819207742980097 ) ) ;
#54401=CIRCLE ( 'NONE', #86494, 1.000000000000000000 ) ;
#54402=CARTESIAN_POINT ( 'NONE',  ( 18.63864990483601858, 1509.044553701713312, 187.9652674624242366 ) ) ;
#54404=B_SPLINE_SURFACE_WITH_KNOTS ( 'NONE', 5, 5, ( 
 ( #99330, #73059, #57383, #39450, #82563, #38878 ),
 ( #73623, #107753, #47300, #107201, #31036, #108304 ),
 ( #64678, #29932, #31589, #13661, #32148, #65219 ),
 ( #99884, #30489, #65766, #23182, #22057, #48975 ),
 ( #83107, #91509, #12596, #6401, #40547, #74721 ),
 ( #98795, #55174, #108854, #5855, #90945, #66336 ),
 ( #56254, #55726, #22604, #98244, #48420, #21514 ),
 ( #100452, #39996, #56807, #74175, #90382, #14231 ),
 ( #89845, #13117, #89300, #46774, #4201, #106641 ),
 ( #80905, #47850, #81984, #5292, #38333, #72513 ),
 ( #81424, #34359, #77474, #17523, #85292, #75276 ),
 ( #102098, #68535, #43326, #100990, #16420, #33244 ),
 ( #25934, #59026, #24821, #41659, #67987, #24286 ),
 ( #42763, #25379, #67434, #8591, #8043, #6942 ),
 ( #775, #9162, #57923, #76923, #34904, #92055 ),
 ( #69090, #59571, #75815, #60130, #42211, #51164 ),
 ( #93685, #76362, #110511, #15868, #109967, #33793 ),
 ( #109423, #101532, #32700, #232, #93151, #23735 ),
 ( #94249, #102633, #84200, #51726, #85861, #50613 ),
 ( #7497, #15327, #49522, #83647, #41097, #66880 ),
 ( #84745, #16965, #58467, #92594, #50071, #10822 ) ),
 .UNSPECIFIED., .F., .F., .F.,
 ( 6, 3, 3, 3, 3, 3, 6 ),
 ( 6, 6 ),
 ( 3.497608506310000198, 12.90721938930000157, 16.34806485209999849, 18.06848758349999784, 18.75464242129999803, 19.44079725900000000, 19.78891031479999896 ),
 ( 0.000000000000000000, 2.205736517120000073 ),
 .UNSPECIFIED. ) ;
#54409=ORIENTED_EDGE ( 'NONE', *, *, #106852, .F. ) ;
#54410=CARTESIAN_POINT ( 'NONE',  ( 17.38235994490000280, 1414.983771850430003, 210.5633853858680027 ) ) ;
#54411=CARTESIAN_POINT ( 'NONE',  ( -24.11773784480000060, 1444.076521055339981, 211.7353999850080015 ) ) ;
#54412=CARTESIAN_POINT ( 'NONE',  ( -0.7006591791222261945, 1450.888592821566363, 154.2444655603070203 ) ) ;
#54416=CARTESIAN_POINT ( 'NONE',  ( 19.12393420247930109, 1509.659725678649920, 184.6857789466980080 ) ) ;
#54419=CARTESIAN_POINT ( 'NONE',  ( -13.23366354170440040, 1419.304941490409874, 221.9853583435139797 ) ) ;
#54420=B_SPLINE_CURVE_WITH_KNOTS ( 'NONE', 3,
 ( #78417, #9542, #95763, #68938 ),
 .UNSPECIFIED., .F., .F.,
 ( 4, 4 ),
 ( 0.000000000000000000, 1.000000000000000000 ),
 .UNSPECIFIED. ) ;
#54421=CARTESIAN_POINT ( 'NONE',  ( 5.856052932189999893, 1412.733406791530115, 231.2218989843980239 ) ) ;
#54423=CARTESIAN_POINT ( 'NONE',  ( -16.50825790430000239, 1460.843606021430105, 228.2701616867980192 ) ) ;
#54425=CARTESIAN_POINT ( 'NONE',  ( 46.27886452250000104, 1438.889480702049923, 267.5894389992980109 ) ) ;
#54426=CARTESIAN_POINT ( 'NONE',  ( -19.08749734139999887, 1410.075444410930004, 222.3596486551979865 ) ) ;
#54427=CARTESIAN_POINT ( 'NONE',  ( 21.17685425119999820, 1435.236150072139935, 141.6298919720979939 ) ) ;
#54428=CARTESIAN_POINT ( 'NONE',  ( 19.82449983040000063, 1469.159611771130130, 191.7468874958980223 ) ) ;
#54429=CARTESIAN_POINT ( 'NONE',  ( 24.59498489902570029, 1440.913044926110160, 213.3385239659299941 ) ) ;
#54431=CARTESIAN_POINT ( 'NONE',  ( -3.758278191160000059, 1475.720032253530007, 266.9554522522980164 ) ) ;
#54434=FACE_OUTER_BOUND ( 'NONE', #106919, .T. ) ;
#54436=CARTESIAN_POINT ( 'NONE',  ( -17.31002161700749653, 1410.038357211269840, 193.4350317523646368 ) ) ;
#54439=CARTESIAN_POINT ( 'NONE',  ( 11.87984373510000147, 1433.310963811120018, 146.4341632258980042 ) ) ;
#54440=CARTESIAN_POINT ( 'NONE',  ( -30.79850881079999780, 1436.468376053830070, 136.6063225575979914 ) ) ;
#54443=CARTESIAN_POINT ( 'NONE',  ( -11.06770810696790086, 1409.299553270950128, 219.1756186191919937 ) ) ;
#54444=CARTESIAN_POINT ( 'NONE',  ( -16.68463225901000158, 1445.052233488270076, 162.0935120915889911 ) ) ;
#54446=CARTESIAN_POINT ( 'NONE',  ( -16.68463225827704122, 1442.773887286370382, 162.0935120918187806 ) ) ;
#54447=CARTESIAN_POINT ( 'NONE',  ( -42.38294288630000040, 1456.046607473030008, 266.8007141661980199 ) ) ;
#54449=CARTESIAN_POINT ( 'NONE',  ( 0.3751301725765759931, 1419.058492625649933, 184.6369606967579955 ) ) ;
#54453=CARTESIAN_POINT ( 'NONE',  ( 18.29126995980630355, 1425.098100345099965, 226.7651582995079877 ) ) ;
#54454=CARTESIAN_POINT ( 'NONE',  ( 11.49747567979999907, 1414.913060387329779, 220.3427040543980127 ) ) ;
#54455=CARTESIAN_POINT ( 'NONE',  ( 15.14740264819999993, 1485.055112692129796, 223.7344915146980213 ) ) ;
#54456=CARTESIAN_POINT ( 'NONE',  ( 2.663428195552854927, 1419.688227176016881, 137.0999999980978430 ) ) ;
#54458=ORIENTED_EDGE ( 'NONE', *, *, #1598, .T. ) ;
#54459=CARTESIAN_POINT ( 'NONE',  ( -5.669846970490000082, 1507.854450105929800, 181.2109580980980184 ) ) ;
#54460=CARTESIAN_POINT ( 'NONE',  ( 4.786039370545940308, 1421.795857048071412, 137.9175743968286270 ) ) ;
#54462=CARTESIAN_POINT ( 'NONE',  ( -11.46423597849999965, 1415.041103191630100, 195.6823422413980040 ) ) ;
#54464=EDGE_CURVE ( 'NONE', #44414, #71213, #22177, .T. ) ;
#54465=FACE_OUTER_BOUND ( 'NONE', #62942, .T. ) ;
#54468=CARTESIAN_POINT ( 'NONE',  ( -15.06280285359999915, 1422.388303686929930, 229.4662104616980116 ) ) ;
#54469=CARTESIAN_POINT ( 'NONE',  ( -11.87111153510000072, 1432.721389748929823, 150.3961583812979939 ) ) ;
#54471=DIRECTION ( 'NONE',  ( 0.3538510588705020554, 0.9352971592855031657, 0.002941422902738410894 ) ) ;
#54473=EDGE_CURVE ( 'NONE', #35126, #51888, #79026, .T. ) ;
#54480=CARTESIAN_POINT ( 'NONE',  ( 13.38442537232469931, 1507.877059872409745, 233.1002377268139867 ) ) ;
#54481=CARTESIAN_POINT ( 'NONE',  ( -16.28589060890169549, 1485.388328323199858, 187.7393477621970135 ) ) ;
#54486=ORIENTED_EDGE ( 'NONE', *, *, #8293, .F. ) ;
#54488=ORIENTED_EDGE ( 'NONE', *, *, #87635, .T. ) ;
#54489=CARTESIAN_POINT ( 'NONE',  ( 28.79939580839999991, 1509.589065600929871, 209.5214383132930038 ) ) ;
#54493=CARTESIAN_POINT ( 'NONE',  ( 15.75137492476309831, 1413.122398938390006, 191.4468246197170060 ) ) ;
#54494=CARTESIAN_POINT ( 'NONE',  ( 0.8261844755670000318, 1508.165896155429891, 180.7872846942979947 ) ) ;
#54496=CARTESIAN_POINT ( 'NONE',  ( -25.70055298538810007, 1451.293284185210041, 136.6856562540129971 ) ) ;
#54497=CARTESIAN_POINT ( 'NONE',  ( 11.42137624728064793, 1437.875189691955484, 152.0075177772093582 ) ) ;
#54498=CARTESIAN_POINT ( 'NONE',  ( 11.50002771670000001, 1409.817236179030033, 229.0027380318980192 ) ) ;
#54502=CARTESIAN_POINT ( 'NONE',  ( 41.28347186110210032, 1446.141341654809821, 134.0999999985599800 ) ) ;
#54512=CARTESIAN_POINT ( 'NONE',  ( 8.020248913699530746, 1451.388689963839852, 152.9391484428220735 ) ) ;
#54513=DIRECTION ( 'NONE',  ( 0.000000000000000000, 0.000000000000000000, -1.000000000000000000 ) ) ;
#54517=CARTESIAN_POINT ( 'NONE',  ( -16.87886782060054358, 1449.383582043091110, 219.7154039679069797 ) ) ;
#54519=CARTESIAN_POINT ( 'NONE',  ( 4.279348318663660500, 1446.810037118880018, 156.6083306040470120 ) ) ;
#54521=CARTESIAN_POINT ( 'NONE',  ( -0.05360592782209999685, 1508.805584758630175, 238.3850021203980134 ) ) ;
#54522=AXIS2_PLACEMENT_3D ( 'NONE', #64585, #48323, #107105 ) ;
#54523=ORIENTED_EDGE ( 'NONE', *, *, #14612, .T. ) ;
#54526=CARTESIAN_POINT ( 'NONE',  ( 25.52987090084080180, 1440.913060387330006, 240.7947691460219914 ) ) ;
#54527=CARTESIAN_POINT ( 'NONE',  ( -20.99310676700000400, 1509.712615454430079, 187.9175748575979981 ) ) ;
#54528=VERTEX_POINT ( 'NONE', #11830 ) ;
#54529=CARTESIAN_POINT ( 'NONE',  ( -33.92644764715539196, 1450.868595403629342, 136.1710051450618835 ) ) ;
#54530=CARTESIAN_POINT ( 'NONE',  ( -13.30454290660000005, 1409.377665263330073, 191.4591812459979963 ) ) ;
#54532=CARTESIAN_POINT ( 'NONE',  ( -24.34453575608964826, 1439.510801930967091, 212.0368851435746933 ) ) ;
#54537=CARTESIAN_POINT ( 'NONE',  ( -13.80504973719999917, 1434.979586003610166, 149.9810040114979870 ) ) ;
#54539=CARTESIAN_POINT ( 'NONE',  ( 4.458165412510000536, 1464.757726041729939, 234.6072865489980188 ) ) ;
#54541=B_SPLINE_SURFACE_WITH_KNOTS ( 'NONE', 5, 5, ( 
 ( #80193, #2415, #45517, #44960, #55558, #11888, #80745, #79659, #54468 ),
 ( #104841, #37080, #4054, #38180, #4590, #20814, #27577, #53355, #3511 ),
 ( #37635, #87500, #10790, #58300, #14624, #92422, #109258, #39838, #82397 ),
 ( #23013, #48254, #15697, #21897, #5694, #82934, #64514, #65608, #23573 ),
 ( #24108, #65053, #49900, #49349, #74557, #48811, #40933, #74001, #75111 ),
 ( #57217, #31426, #66715, #84035, #108133, #83476, #56095, #31982, #38723 ),
 ( #15158, #100292, #99720, #32542, #6769, #57766, #91885, #91343, #72898 ),
 ( #107038, #73457, #30325, #90222, #14065, #108690, #56648, #6225, #39282 ),
 ( #40380, #99166, #90782, #66172, #100821, #13507, #98629, #47695, #81823 ) ),
 .UNSPECIFIED., .F., .F., .F.,
 ( 6, 3, 6 ),
 ( 6, 3, 6 ),
 ( 14.04571185090000007, 21.32310247789999735, 23.98960798969999786 ),
 ( 0.000000000000000000, 1.000000000000000000, 2.000000000000000000 ),
 .UNSPECIFIED. ) ;
#54545=CARTESIAN_POINT ( 'NONE',  ( 27.79064039369999861, 1508.605033448830227, 207.7520403698979976 ) ) ;
#54547=DIRECTION ( 'NONE',  ( -0.08340294689716752641, -0.004098122787120126072, -0.9965074780645100105 ) ) ;
#54550=ORIENTED_EDGE ( 'NONE', *, *, #25614, .F. ) ;
#54551=CARTESIAN_POINT ( 'NONE',  ( -18.51267908742608626, 1508.236097877770362, 229.7333076609436944 ) ) ;
#54552=CARTESIAN_POINT ( 'NONE',  ( 28.33103133819999897, 1450.578314058649994, 240.1819618854979979 ) ) ;
#54553=CARTESIAN_POINT ( 'NONE',  ( -16.48650050839999892, 1458.966229476530089, 230.7111281069979896 ) ) ;
#54555=CARTESIAN_POINT ( 'NONE',  ( -0.4228048877666359950, 1508.822484023469769, 238.3615180857069902 ) ) ;
#54558=CARTESIAN_POINT ( 'NONE',  ( 11.87312836989999987, 1432.864053697380086, 149.9809862119980153 ) ) ;
#54559=CARTESIAN_POINT ( 'NONE',  ( 2.500000000000000000, 1419.446092955830181, 146.1320802672979937 ) ) ;
#54562=ORIENTED_EDGE ( 'NONE', *, *, #73976, .F. ) ;
#54564=CARTESIAN_POINT ( 'NONE',  ( 1.334517921909999849, 1405.730281140330135, 267.8533188392980264 ) ) ;
#54565=AXIS2_PLACEMENT_3D ( 'NONE', #79603, #105343, #44346 ) ;
#54568=CARTESIAN_POINT ( 'NONE',  ( 42.54900313428320402, 1445.932418601849804, 270.0692078791809649 ) ) ;
#54569=CARTESIAN_POINT ( 'NONE',  ( 5.510117011110000185, 1440.199971711759872, 154.7606381671979818 ) ) ;
#54570=CARTESIAN_POINT ( 'NONE',  ( 11.60004869885203682, 1422.222932908421399, 137.0999999980977293 ) ) ;
#54571=CARTESIAN_POINT ( 'NONE',  ( -45.67177343128329881, 1440.913044206929953, 266.1885934837860077 ) ) ;
#54578=CARTESIAN_POINT ( 'NONE',  ( -3.804422478559999821, 1422.873164475230169, 234.3916895697979612 ) ) ;
#54580=CARTESIAN_POINT ( 'NONE',  ( -0.2144367069559999783, 1475.560912059630027, 269.2947081849980009 ) ) ;
#54581=CARTESIAN_POINT ( 'NONE',  ( -4.265921920120119282, 1446.647485887290031, 158.6289097731119853 ) ) ;
#54583=CARTESIAN_POINT ( 'NONE',  ( -18.46438761643240056, 1509.557851011080174, 231.7133587057680018 ) ) ;
#54585=CARTESIAN_POINT ( 'NONE',  ( -18.71036172829999700, 1415.996778984329922, 208.1550592490559950 ) ) ;
#54587=CARTESIAN_POINT ( 'NONE',  ( 26.68598823788470042, 1436.588321450659805, 136.7639126871760027 ) ) ;
#54589=CARTESIAN_POINT ( 'NONE',  ( -4.597933714602949529, 1396.073623771769917, 219.1466160566309895 ) ) ;
#54591=CARTESIAN_POINT ( 'NONE',  ( 7.320561577120000329, 1432.353341358199941, 149.5448088695980005 ) ) ;
#54595=CARTESIAN_POINT ( 'NONE',  ( 2.431084916239999671, 1409.932888328230092, 231.7225720581979829 ) ) ;
#54597=CARTESIAN_POINT ( 'NONE',  ( -11.73563882241239931, 1425.610159415710086, 144.1657444112690030 ) ) ;
#54598=CARTESIAN_POINT ( 'NONE',  ( 11.09525485650000043, 1425.652349456129969, 121.0021085274979953 ) ) ;
#54602=B_SPLINE_CURVE_WITH_KNOTS ( 'NONE', 5,
 ( #22786, #56992, #13843, #4380, #21133, #29025 ),
 .UNSPECIFIED., .F., .F.,
 ( 6, 6 ),
 ( 0.000000000000000000, 1.000000000000000000 ),
 .UNSPECIFIED. ) ;
#54606=CARTESIAN_POINT ( 'NONE',  ( 1.669890710080000007, 1508.956865050929991, 179.7751757191980175 ) ) ;
#54607=DIRECTION ( 'NONE',  ( 0.000000000000000000, 0.000000000000000000, 1.000000000000000000 ) ) ;
#54611=ORIENTED_EDGE ( 'NONE', *, *, #47038, .F. ) ;
#54612=ORIENTED_EDGE ( 'NONE', *, *, #51552, .F. ) ;
#54613=EDGE_CURVE ( 'NONE', #65987, #48650, #84055, .T. ) ;
#54614=CARTESIAN_POINT ( 'NONE',  ( -8.589176046050001290, 1397.858446770630053, 199.0029481086979786 ) ) ;
#54615=CARTESIAN_POINT ( 'NONE',  ( 0.4520741306692179773, 1482.864041210959840, 236.3239132953789863 ) ) ;
#54616=CARTESIAN_POINT ( 'NONE',  ( 13.91344329460000040, 1453.313060387329870, 224.4164659125979995 ) ) ;
#54619=CARTESIAN_POINT ( 'NONE',  ( 11.22085813615770000, 1414.913060387329779, 197.6243702374680140 ) ) ;
#54620=CARTESIAN_POINT ( 'NONE',  ( 6.602193856980000497, 1410.296089514130017, 187.0051498391979976 ) ) ;
#54622=CARTESIAN_POINT ( 'NONE',  ( -39.76109132672340252, 1448.193450711350124, 136.2665313895609813 ) ) ;
#54626=CARTESIAN_POINT ( 'NONE',  ( -3.818053759430319882, 1406.099154933030150, 266.9556830280999975 ) ) ;
#54629=CARTESIAN_POINT ( 'NONE',  ( 4.363122458829999495, 1423.854802366329977, 183.5697733487979804 ) ) ;
#54632=B_SPLINE_CURVE_WITH_KNOTS ( 'NONE', 3,
 ( #71567, #48533, #73740, #38996, #55840, #98362, #90509, #5963, #89962, #97806, #73173, #29501, #106758, #65888, #82109, #91616, #21084, #13785, #81549, #14893, #107863, #22727, #5407, #13236, #31152, #46892, #80474, #56929, #3792, #14343, #65341, #30048, #47426, #81016, #55288, #89418, #72627, #64240, #37923, #4324, #64799, #38454, #21635, #91057, #22180, #98908, #4849, #107317, #72104, #63695, #30612, #56377, #23295, #31704, #47967, #99450, #57492, #106219, #39567, #40108, #74290, #108421, #100007, #84848, #77035, #74835, #75920, #34470, #50719, #16528, #8149, #7607, #76470, #59144, #41218, #83219, #66987, #15441, #33348, #7063, #49632, #23840, #32265, #93797, #101098, #109527, #24398, #68100, #75390, #102215, #67543, #343, #84316, #42316 ),
 .UNSPECIFIED., .F., .F.,
 ( 4, 3, 3, 3, 3, 3, 3, 3, 3, 3, 3, 3, 3, 3, 3, 3, 3, 3, 3, 3, 3, 3, 3, 3, 3, 3, 3, 3, 3, 3, 3, 4 ),
 ( -31.18846563725180232, -31.00774817696539998, -29.91343961047510192, -28.82901376052130260, -27.75228773005839855, -26.68937329812260018, -25.63621693740660135, -24.59289539267759750, -23.55938141437490074, -22.54133121024409903, -21.54281980820089970, -20.54474872284400178, -19.55609317380470102, -18.57652819858910220, -17.60572709955240001, -16.64336675927789955, -15.67369350074630141, -14.07561117147439944, -12.28927372929120310, -10.62231242529870201, -8.938518733482830214, -7.370289770217699044, -5.839433697936598833, -4.341848494604818143, -4.231108194414311185, -2.815296474105110747, -1.445085169337431807, -0.1034094330291317476, 1.196738312870451182, 2.472340971179193048, 3.725905068250661145, 4.959507408170033216 ),
 .UNSPECIFIED. ) ;
#54633=EDGE_LOOP ( 'NONE', ( #103797, #98620, #98927, #26225 ) ) ;
#54640=CARTESIAN_POINT ( 'NONE',  ( 2.500000000000000000, 1448.397602632589951, 162.2732098858260201 ) ) ;
#54646=CARTESIAN_POINT ( 'NONE',  ( -31.17186646729999921, 1440.913060387330006, 255.0393818639979884 ) ) ;
#54647=B_SPLINE_SURFACE_WITH_KNOTS ( 'NONE', 5, 5, ( 
 ( #5891, #5333, #40037, #107796, #78615, #8080 ),
 ( #76962, #110550, #78053, #43910, #271, #85899 ),
 ( #43366, #85330, #52330, #42250, #34398, #1930 ),
 ( #93188, #84783, #27112, #68572, #50652, #67470 ),
 ( #101575, #1359, #25415, #18679, #77514, #59609 ),
 ( #815, #102137, #24863, #102672, #94286, #76397 ) ),
 .UNSPECIFIED., .F., .F., .F.,
 ( 6, 6 ),
 ( 6, 6 ),
 ( 8.853503526680000846, 11.83085891290000013 ),
 ( 0.000000000000000000, 1.446538132919999997 ),
 .UNSPECIFIED. ) ;
#54648=B_SPLINE_CURVE_WITH_KNOTS ( 'NONE', 5,
 ( #19896, #106663, #62506, #70905, #2588, #27755, #61948, #54646, #105585, #89319, #71467, #54099 ),
 .UNSPECIFIED., .F., .F.,
 ( 6, 3, 3, 6 ),
 ( -32.81232995010000053, -6.990622299171700860, 15.67373306494047114, 31.61444093042090486 ),
 .UNSPECIFIED. ) ;
#54650=CARTESIAN_POINT ( 'NONE',  ( -9.910331035380000486, 1409.425488993030058, 229.0636521845979985 ) ) ;
#54651=FACE_OUTER_BOUND ( 'NONE', #53181, .T. ) ;
#54653=CARTESIAN_POINT ( 'NONE',  ( 27.84004021000000151, 1451.940495779430194, 134.8938502556979984 ) ) ;
#54654=CARTESIAN_POINT ( 'NONE',  ( 1.726858845393010045, 1482.796399496739923, 235.4332745739710049 ) ) ;
#54655=CARTESIAN_POINT ( 'NONE',  ( 20.59684376970620079, 1507.762609625729965, 227.3086063979779965 ) ) ;
#54658=CARTESIAN_POINT ( 'NONE',  ( 41.83993043035380310, 1432.387293077269760, 270.1928086331030272 ) ) ;
#54661=CARTESIAN_POINT ( 'NONE',  ( -25.91590772737680126, 1441.261220175949802, 138.4451201564890255 ) ) ;
#54664=CARTESIAN_POINT ( 'NONE',  ( 19.42032769166468853, 1410.952570011139869, 196.1050306194517816 ) ) ;
#54666=ORIENTED_EDGE ( 'NONE', *, *, #56421, .F. ) ;
#54667=CARTESIAN_POINT ( 'NONE',  ( 23.10442899973940101, 1411.095127650270115, 207.3185325528490068 ) ) ;
#54668=CARTESIAN_POINT ( 'NONE',  ( -33.91369120209999721, 1435.681798817170147, 134.0999999980979851 ) ) ;
#54670=FACE_OUTER_BOUND ( 'NONE', #59737, .T. ) ;
#54671=ORIENTED_EDGE ( 'NONE', *, *, #92439, .T. ) ;
#54675=DIRECTION ( 'NONE',  ( -0.6456624059243071256, -0.004098122786995253737, 0.7636119845613070778 ) ) ;
#54677=CARTESIAN_POINT ( 'NONE',  ( -0.2517843955729999750, 1408.921852844929845, 232.2115700972980221 ) ) ;
#54678=CARTESIAN_POINT ( 'NONE',  ( 2.632631803615880450, 1417.642869435429930, 234.7516633181379859 ) ) ;
#54688=CARTESIAN_POINT ( 'NONE',  ( 10.56668910718356535, 1434.889276759676477, 152.0929273929996839 ) ) ;
#54689=CARTESIAN_POINT ( 'NONE',  ( 38.61927353243170558, 1444.188088105049928, 137.1592452208769828 ) ) ;
#54693=CARTESIAN_POINT ( 'NONE',  ( 6.301535050710000085, 1423.297843521130062, 186.2731961210980103 ) ) ;
#54694=CARTESIAN_POINT ( 'NONE',  ( -17.84818147429999868, 1423.997650907529987, 226.0612537164979869 ) ) ;
#54695=CARTESIAN_POINT ( 'NONE',  ( -14.99308972890000113, 1435.024836507099963, 148.2840791620979815 ) ) ;
#54696=CARTESIAN_POINT ( 'NONE',  ( 33.91369266730000476, 1450.440660192670066, 136.2454535554979884 ) ) ;
#54697=CARTESIAN_POINT ( 'NONE',  ( -1.735723226805210073, 1473.469101322430106, 183.2265203639830133 ) ) ;
#54699=CARTESIAN_POINT ( 'NONE',  ( -17.60714162564125118, 1434.290496652245110, 215.9208836820417332 ) ) ;
#54703=LINE ( 'NONE', #97771, #53581 ) ;
#54705=VERTEX_POINT ( 'NONE', #13447 ) ;
#54709=CARTESIAN_POINT ( 'NONE',  ( -6.896890933126118993E-05, 1408.913065613199933, 231.7784170915439859 ) ) ;
#54710=CARTESIAN_POINT ( 'NONE',  ( 11.67163616197805887, 1435.064040831317016, 151.3452733738369318 ) ) ;
#54712=CARTESIAN_POINT ( 'NONE',  ( -6.844578743112079700, 1507.263722753517868, 235.7154808215367723 ) ) ;
#54716=CIRCLE ( 'NONE', #45764, 86.30410767968433561 ) ;
#54717=CYLINDRICAL_SURFACE ( 'NONE', #12502, 2.000000000000001776 ) ;
#54719=CARTESIAN_POINT ( 'NONE',  ( 22.43276589599999937, 1508.963982320630066, 192.2846129824980324 ) ) ;
#54723=ORIENTED_EDGE ( 'NONE', *, *, #17320, .T. ) ;
#54725=CARTESIAN_POINT ( 'NONE',  ( 24.24763046536200051, 1427.549423795960138, 207.7433240213180170 ) ) ;
#54726=CARTESIAN_POINT ( 'NONE',  ( 13.77725779630000069, 1509.394201300130135, 235.0109963963979851 ) ) ;
#54727=CARTESIAN_POINT ( 'NONE',  ( 13.14336223832311568, 1443.062568900890710, 169.3993974764935047 ) ) ;
#54728=CARTESIAN_POINT ( 'NONE',  ( 40.51831965869402552, 1432.752226466759566, 269.6196524019716776 ) ) ;
#54729=CARTESIAN_POINT ( 'NONE',  ( -30.53571888289999947, 1442.873932102629851, 240.1260121736980011 ) ) ;
#54731=CARTESIAN_POINT ( 'NONE',  ( -11.36702043620000069, 1433.804590679680132, 151.4517328811979837 ) ) ;
#54733=CARTESIAN_POINT ( 'NONE',  ( -19.45775078520000179, 1486.277066373030038, 189.7536442620979926 ) ) ;
#54734=CARTESIAN_POINT ( 'NONE',  ( 10.14578895520000046, 1410.638169269630225, 188.6745756209980129 ) ) ;
#54735=CARTESIAN_POINT ( 'NONE',  ( 4.581316872830000442, 1422.049244984730194, 184.0357665752979983 ) ) ;
#54737=CARTESIAN_POINT ( 'NONE',  ( 16.88182070999999951, 1417.652932793330137, 226.6960533187979934 ) ) ;
#54738=CARTESIAN_POINT ( 'NONE',  ( 12.75521900933300046, 1428.291927597070071, 223.8668883416810047 ) ) ;
#54739=CARTESIAN_POINT ( 'NONE',  ( -22.28769322179999790, 1450.904749962159940, 143.2988008388979893 ) ) ;
#54743=CARTESIAN_POINT ( 'NONE',  ( -11.86119678505159847, 1431.993545301180120, 149.9716976446269996 ) ) ;
#54745=CARTESIAN_POINT ( 'NONE',  ( -12.98194342669999912, 1470.141184529730026, 269.6330410522980401 ) ) ;
#54746=CARTESIAN_POINT ( 'NONE',  ( -24.20882859423510070, 1435.739118765830199, 210.8967395777180229 ) ) ;
#54749=CARTESIAN_POINT ( 'NONE',  ( 0.2075316472611209995, 1452.106270034880026, 183.0908634647769873 ) ) ;
#54750=CARTESIAN_POINT ( 'NONE',  ( -13.12562721870000182, 1421.054977677129955, 228.8117867079979817 ) ) ;
#54751=AXIS2_PLACEMENT_3D ( 'NONE', #66785, #15762, #102539 ) ;
#54754=CARTESIAN_POINT ( 'NONE',  ( -45.11518327334809442, 1435.673159459739963, 268.9894092425899998 ) ) ;
#54755=VERTEX_POINT ( 'NONE', #92369 ) ;
#54756=CARTESIAN_POINT ( 'NONE',  ( -3.545193281622200043, 1502.970594565849979, 181.1540523117359953 ) ) ;
#54757=ORIENTED_EDGE ( 'NONE', *, *, #9057, .T. ) ;
#54760=CARTESIAN_POINT ( 'NONE',  ( -20.59678674160000256, 1507.763197054029888, 190.3721467792980206 ) ) ;
#54761=CARTESIAN_POINT ( 'NONE',  ( -14.81926257019999937, 1410.404433816730034, 190.6668097203979926 ) ) ;
#54768=CARTESIAN_POINT ( 'NONE',  ( -25.68853613209369868, 1416.734612324150021, 269.4293337505479826 ) ) ;
#54769=CARTESIAN_POINT ( 'NONE',  ( 2.913665321129999787E-15, 1426.935925255829943, 133.6118001900980232 ) ) ;
#54770=CARTESIAN_POINT ( 'NONE',  ( 0.006135415692569999579, 1395.974572303430023, 197.4936679487979916 ) ) ;
#54772=ORIENTED_EDGE ( 'NONE', *, *, #6203, .T. ) ;
#54774=CARTESIAN_POINT ( 'NONE',  ( 45.62655422193257237, 1441.650256554816224, 268.9750399244037453 ) ) ;
#54775=EDGE_CURVE ( 'NONE', #18861, #95096, #10099, .T. ) ;
#54777=CARTESIAN_POINT ( 'NONE',  ( -14.25110351248640050, 1436.256065985239957, 150.0865086527120127 ) ) ;
#54779=CARTESIAN_POINT ( 'NONE',  ( -18.11230055478630163, 1415.348334732599824, 207.5667894811009830 ) ) ;
#54780=CARTESIAN_POINT ( 'NONE',  ( -23.11183678279999754, 1435.763572499130078, 215.1866059518479801 ) ) ;
#54781=CARTESIAN_POINT ( 'NONE',  ( 22.35545660506620180, 1471.322756690530014, 269.3294010533080609 ) ) ;
#54782=CARTESIAN_POINT ( 'NONE',  ( 11.70751967719999875, 1415.128105756529976, 222.5965497224979970 ) ) ;
#54783=CARTESIAN_POINT ( 'NONE',  ( -17.73406580063780069, 1423.343214054229975, 226.1884525926029994 ) ) ;
#54787=CARTESIAN_POINT ( 'NONE',  ( -22.48690821953700691, 1451.619460217190408, 219.5055000607859483 ) ) ;
#54789=CARTESIAN_POINT ( 'NONE',  ( 10.58313173430331489, 1455.148896507045947, 226.2839261739179051 ) ) ;
#54790=CARTESIAN_POINT ( 'NONE',  ( 25.21692146640110010, 1450.980894760169804, 137.5957989584090058 ) ) ;
#54793=CARTESIAN_POINT ( 'NONE',  ( 21.01921312860000057, 1410.567660014329931, 199.9123866135879837 ) ) ;
#54794=CARTESIAN_POINT ( 'NONE',  ( -2.964074117308931111, 1446.907475440849339, 170.5322007353207994 ) ) ;
#54795=CARTESIAN_POINT ( 'NONE',  ( 17.29614329919999705, 1410.879761755329810, 225.9915122344980034 ) ) ;
#54797=CARTESIAN_POINT ( 'NONE',  ( 0.5349531902123869642, 1451.469306295839942, 182.7928085713219843 ) ) ;
#54798=B_SPLINE_CURVE_WITH_KNOTS ( 'NONE', 3,
 ( #47819, #23703, #24250, #57887 ),
 .UNSPECIFIED., .F., .F.,
 ( 4, 4 ),
 ( 0.000000000000000000, 1.000000000000000000 ),
 .UNSPECIFIED. ) ;
#54799=CARTESIAN_POINT ( 'NONE',  ( 2.500000000000000000, 1439.402073890429847, 161.8071954337849832 ) ) ;
#54803=LINE ( 'NONE', #45311, #72368 ) ;
#54808=CARTESIAN_POINT ( 'NONE',  ( -11.60004869885203682, 0.000000000000000000, 137.0999999980979851 ) ) ;
#54809=ADVANCED_FACE ( 'NONE', ( #99662 ), #1593, .F. ) ;
#54810=CARTESIAN_POINT ( 'NONE',  ( -36.80391333867880377, 1449.651525888219794, 136.2794198540989896 ) ) ;
#54812=CARTESIAN_POINT ( 'NONE',  ( 11.60004869885203682, 1425.221648007341628, 138.0074162802604860 ) ) ;
#54813=CARTESIAN_POINT ( 'NONE',  ( 2.378525042339323825, 1417.651026746295884, 233.6043764637433355 ) ) ;
#54817=CARTESIAN_POINT ( 'NONE',  ( 11.80036447210000006, 1433.149496178429899, 150.6216816897980095 ) ) ;
#54818=CARTESIAN_POINT ( 'NONE',  ( -3.323641320539999722, 1474.972506225130019, 269.6411426393979696 ) ) ;
#54824=ORIENTED_EDGE ( 'NONE', *, *, #98190, .T. ) ;
#54826=B_SPLINE_CURVE_WITH_KNOTS ( 'NONE', 3,
 ( #15219, #75712, #7392, #109858, #30938, #31483 ),
 .UNSPECIFIED., .F., .F.,
 ( 4, 2, 4 ),
 ( 0.000000000000000000, 0.5000000000000000000, 1.000000000000000000 ),
 .UNSPECIFIED. ) ;
#54827=CARTESIAN_POINT ( 'NONE',  ( 12.37499353609999986, 1442.762691980110048, 206.9242620747189960 ) ) ;
#54828=CARTESIAN_POINT ( 'NONE',  ( -19.39682342001572835, 1485.601863261859762, 189.9014862107358113 ) ) ;
#54829=CARTESIAN_POINT ( 'NONE',  ( 8.039070834880659433, 1398.151819186490229, 198.9054696569589566 ) ) ;
#54832=CARTESIAN_POINT ( 'NONE',  ( -13.97249221049999868, 1508.900185047429886, 233.0230284711979891 ) ) ;
#54835=CARTESIAN_POINT ( 'NONE',  ( 6.825986730469999486, 1409.091027440530070, 221.7399762292980085 ) ) ;
#54838=CARTESIAN_POINT ( 'NONE',  ( 1.540611278380000115, 1465.978124834829941, 234.9895109092980192 ) ) ;
#54839=CARTESIAN_POINT ( 'NONE',  ( -9.838665332836511013, 1435.926116633432457, 152.6147087539863776 ) ) ;
#54840=EDGE_LOOP ( 'NONE', ( #83185, #100075, #41642, #24272 ) ) ;
#54841=CARTESIAN_POINT ( 'NONE',  ( -0.6637618131060000204, 1452.913539784329942, 183.3365650660979895 ) ) ;
#54844=CARTESIAN_POINT ( 'NONE',  ( -18.33918424680000214, 1416.543503932829935, 208.8538484177919656 ) ) ;
#54845=EDGE_LOOP ( 'NONE', ( #101822, #42837, #61427, #54377, #52647 ) ) ;
#54850=CARTESIAN_POINT ( 'NONE',  ( 12.26979804483799974, 1416.828039243390094, 223.5793509210460002 ) ) ;
#54851=CARTESIAN_POINT ( 'NONE',  ( 11.87563351815570023, 1433.006677199550040, 147.6591432317509884 ) ) ;
#54855=FACE_OUTER_BOUND ( 'NONE', #46833, .T. ) ;
#54856=CARTESIAN_POINT ( 'NONE',  ( 14.14831249788200118, 1409.407130346769918, 204.3310347178599784 ) ) ;
#54859=CARTESIAN_POINT ( 'NONE',  ( -17.99328812619999951, 1452.004064770530022, 190.5764782675980200 ) ) ;
#54860=CARTESIAN_POINT ( 'NONE',  ( 11.86607075090000052, 1432.333944803479881, 149.9824168323980018 ) ) ;
#54866=CARTESIAN_POINT ( 'NONE',  ( -12.03450403503200050, 1415.834070663139983, 194.8936510722510036 ) ) ;
#54868=CARTESIAN_POINT ( 'NONE',  ( 28.15443155984639745, 1509.896245780209938, 217.4026704617729990 ) ) ;
#54870=CARTESIAN_POINT ( 'NONE',  ( 10.79382269979189957, 1414.913060387349788, 222.1041130917409987 ) ) ;
#54872=CARTESIAN_POINT ( 'NONE',  ( -0.8893320598190000981, 1471.149508548330232, 182.5957142173980117 ) ) ;
#54875=CARTESIAN_POINT ( 'NONE',  ( 1.575457917789999884, 1508.276376928829905, 237.0209898277979903 ) ) ;
#54884=CARTESIAN_POINT ( 'NONE',  ( 5.805165734619999185, 1411.425360653129928, 255.2684105968979793 ) ) ;
#54885=CARTESIAN_POINT ( 'NONE',  ( -20.38375079739999762, 1488.682100829629917, 192.7189053174979847 ) ) ;
#54886=CARTESIAN_POINT ( 'NONE',  ( -10.94414388512420011, 1426.072984913399978, 95.13475895991039977 ) ) ;
#54887=CARTESIAN_POINT ( 'NONE',  ( -17.99954561119999852, 1410.904693908129957, 195.2564680766979848 ) ) ;
#54888=CARTESIAN_POINT ( 'NONE',  ( 20.66004299446625936, 1506.560172253944756, 201.3057618805298432 ) ) ;
#54889=CARTESIAN_POINT ( 'NONE',  ( -16.98088666479999986, 1414.156373614329823, 255.1564980982979876 ) ) ;
#54890=CARTESIAN_POINT ( 'NONE',  ( 20.21586999686489960, 1509.657102485760106, 230.8999660037090109 ) ) ;
#54892=CARTESIAN_POINT ( 'NONE',  ( 31.77002021779999552, 1450.515383802559882, 136.3085377226980199 ) ) ;
#54894=CARTESIAN_POINT ( 'NONE',  ( -1.510341393340000337E-11, 1395.913060387330006, 198.1220674062979867 ) ) ;
#54900=CARTESIAN_POINT ( 'NONE',  ( -22.92254907261380126, 1409.723441571369904, 208.9286969261789864 ) ) ;
#54903=CARTESIAN_POINT ( 'NONE',  ( 0.1075107530840000020, 1413.831150726530041, 184.8303454653980111 ) ) ;
#54904=CIRCLE ( 'NONE', #56737, 29.84605316675209608 ) ;
#54905=CARTESIAN_POINT ( 'NONE',  ( 13.86092937120069912, 1410.765486813650114, 191.1266627561969926 ) ) ;
#54907=CARTESIAN_POINT ( 'NONE',  ( 0.3093786527580000278, 1452.335660944029769, 183.2932519483980229 ) ) ;
#54908=CARTESIAN_POINT ( 'NONE',  ( -0.5380077850789999339, 1489.065930492329926, 236.5124582711980281 ) ) ;
#54911=CARTESIAN_POINT ( 'NONE',  ( -12.61115941400189833, 1416.521607925270018, 222.0431940980950003 ) ) ;
#54912=CARTESIAN_POINT ( 'NONE',  ( 13.58657643929999992, 1452.821170783829984, 224.5924275984980056 ) ) ;
#54915=EDGE_LOOP ( 'NONE', ( #83275, #31943, #100305, #46287 ) ) ;
#54916=CARTESIAN_POINT ( 'NONE',  ( 11.85313628462840008, 1431.434643513689934, 149.9078370975529708 ) ) ;
#54920=ORIENTED_EDGE ( 'NONE', *, *, #25479, .T. ) ;
#54926=CARTESIAN_POINT ( 'NONE',  ( -1.646540591608269732E-05, 1410.389848909979946, 269.3346290179499647 ) ) ;
#54928=CARTESIAN_POINT ( 'NONE',  ( 11.09516193571039011, 1433.859332616970960, 151.6914986173777038 ) ) ;
#54929=CARTESIAN_POINT ( 'NONE',  ( -11.31243770530000070, 1433.012837821759831, 151.5204583838979886 ) ) ;
#54930=CARTESIAN_POINT ( 'NONE',  ( 0.02437641270083376263, 1409.059024698960911, 232.4096207990013454 ) ) ;
#54935=CARTESIAN_POINT ( 'NONE',  ( -24.38326756241049864, 1509.011140872309852, 222.4884894987410178 ) ) ;
#54937=ORIENTED_EDGE ( 'NONE', *, *, #78331, .F. ) ;
#54938=CARTESIAN_POINT ( 'NONE',  ( 26.42714720800000094, 1440.913060387330006, 243.9198229517980110 ) ) ;
#54940=AXIS2_PLACEMENT_3D ( 'NONE', #83879, #7183, #51387 ) ;
#54945=CARTESIAN_POINT ( 'NONE',  ( 44.92382426869910006, 1440.913067149190056, 269.6913831903979712 ) ) ;
#54947=ORIENTED_EDGE ( 'NONE', *, *, #31676, .F. ) ;
#54948=B_SPLINE_CURVE_WITH_KNOTS ( 'NONE', 5,
 ( #65074, #38201, #38745, #73478, #11370, #88630, #105419, #63448, #106513, #63990, #2986, #13529 ),
 .UNSPECIFIED., .F., .F.,
 ( 6, 3, 3, 6 ),
 ( 0.000000000000000000, 0.2983296735331202876, 0.5998977736818913442, 1.000000000000000000 ),
 .UNSPECIFIED. ) ;
#54951=CARTESIAN_POINT ( 'NONE',  ( -2.500000000000000000, 1439.114301494319989, 157.7261950941980331 ) ) ;
#54954=CARTESIAN_POINT ( 'NONE',  ( 17.99954443082109989, 1410.904693892220166, 222.9872220945560173 ) ) ;
#54955=CARTESIAN_POINT ( 'NONE',  ( 5.360207926212690488, 1422.242713656610022, 144.1549664376839814 ) ) ;
#54956=CARTESIAN_POINT ( 'NONE',  ( 29.96266749478790103, 1509.959379792560185, 213.6203565918929996 ) ) ;
#54958=CARTESIAN_POINT ( 'NONE',  ( 12.89607781515299934, 1434.724834403989917, 149.2206011272099886 ) ) ;
#54960=EDGE_CURVE ( 'NONE', #28184, #91418, #106293, .T. ) ;
#54964=CARTESIAN_POINT ( 'NONE',  ( 45.86410423099999889, 1436.891480617990283, 266.6830272419979906 ) ) ;
#54965=CARTESIAN_POINT ( 'NONE',  ( -16.97531057559999823, 1409.505851295029970, 223.7086794493979767 ) ) ;
#54967=CARTESIAN_POINT ( 'NONE',  ( 23.38999613540000055, 1436.126019947570057, 140.8856778375979957 ) ) ;
#54968=CARTESIAN_POINT ( 'NONE',  ( 20.84753735790000206, 1488.585408351930027, 191.8019074006979849 ) ) ;
#54970=CARTESIAN_POINT ( 'NONE',  ( 5.361102066162420243, 1423.469345717320039, 149.3894558389860094 ) ) ;
#54971=CARTESIAN_POINT ( 'NONE',  ( -3.427369262309999609, 1475.739996263529974, 266.9564229772980752 ) ) ;
#54974=CARTESIAN_POINT ( 'NONE',  ( -33.92723761326109866, 1436.576419602210080, 136.5094945797809771 ) ) ;
#54975=CARTESIAN_POINT ( 'NONE',  ( 0.2171626012915229831, 1453.344709657829981, 183.2386049330829962 ) ) ;
#54976=CARTESIAN_POINT ( 'NONE',  ( -11.20005611260000045, 1409.304174965030143, 199.4475870259680050 ) ) ;
#54980=CARTESIAN_POINT ( 'NONE',  ( 11.87973522909999957, 1433.311075274859832, 146.9202984917980359 ) ) ;
#54981=CARTESIAN_POINT ( 'NONE',  ( -37.09403179692020558, 1436.457961865149855, 134.0999999968530005 ) ) ;
#54982=CARTESIAN_POINT ( 'NONE',  ( 3.920880449199999784, 1439.701871945560015, 184.6839062468980046 ) ) ;
#54985=CARTESIAN_POINT ( 'NONE',  ( -9.578270037681749116, 1409.247540947460038, 220.6126654330650183 ) ) ;
#54989=CARTESIAN_POINT ( 'NONE',  ( -12.78776258895079998, 1416.851343896850040, 195.5391574246120001 ) ) ;
#54991=CARTESIAN_POINT ( 'NONE',  ( -26.68774699959999808, 1468.726062758129956, 269.4193446826980107 ) ) ;
#54993=CARTESIAN_POINT ( 'NONE',  ( -19.71128566253871384, 1498.214606263945370, 189.2503765500455586 ) ) ;
#54995=CARTESIAN_POINT ( 'NONE',  ( -27.59998769030000076, 1509.654128774529909, 212.1034408311279833 ) ) ;
#55000=CARTESIAN_POINT ( 'NONE',  ( 14.63637096480000110, 1474.175152404529854, 223.6336467093979934 ) ) ;
#55001=CARTESIAN_POINT ( 'NONE',  ( 17.74609922954199703, 1415.424669706240138, 224.3250650115680003 ) ) ;
#55004=CARTESIAN_POINT ( 'NONE',  ( 20.15452300067990166, 1507.845791525220193, 189.3412703910400126 ) ) ;
#55005=CARTESIAN_POINT ( 'NONE',  ( 1.448755922665179829, 1499.001568892050045, 236.4189104725390109 ) ) ;
#55007=CARTESIAN_POINT ( 'NONE',  ( -12.72284891840000043, 1416.311719779230089, 195.5584137648980061 ) ) ;
#55008=DIRECTION ( 'NONE',  ( -0.1976597336227498836, -0.9325250109992564429, -0.3022047874621121566 ) ) ;
#55009=CARTESIAN_POINT ( 'NONE',  ( 22.57032379820000045, 1409.701233462030132, 209.8663284536589799 ) ) ;
#55010=CARTESIAN_POINT ( 'NONE',  ( -12.78614179230000047, 1434.663150159289899, 149.2928482040979929 ) ) ;
#55012=CARTESIAN_POINT ( 'NONE',  ( -5.360091096029239388, 1422.252256049249809, 144.8358257923730150 ) ) ;
#55013=CARTESIAN_POINT ( 'NONE',  ( -1.600048698852036821, 1401.254281879943164, 134.0999999980979851 ) ) ;
#55014=CARTESIAN_POINT ( 'NONE',  ( -11.60666322014453655, 1426.782727568212294, 134.8522042001498278 ) ) ;
#55015=CARTESIAN_POINT ( 'NONE',  ( 24.99661049207140096, 1430.498659694909747, 209.1806683305300112 ) ) ;
#55022=CARTESIAN_POINT ( 'NONE',  ( -23.42260982742433129, 1434.595599714059972, 214.6024343348293826 ) ) ;
#55023=CARTESIAN_POINT ( 'NONE',  ( -16.31598018130440053, 1485.656693110169954, 187.6240192544399861 ) ) ;
#55025=CARTESIAN_POINT ( 'NONE',  ( -4.263963421918809615, 1441.192140480630087, 158.8199918691270227 ) ) ;
#55028=ORIENTED_EDGE ( 'NONE', *, *, #38039, .F. ) ;
#55029=CARTESIAN_POINT ( 'NONE',  ( 29.63837385289999915, 1509.975889318429836, 210.7975540006979998 ) ) ;
#55031=CARTESIAN_POINT ( 'NONE',  ( 0.2129864158460960111, 1450.905623043510104, 126.7681030205719850 ) ) ;
#55032=CARTESIAN_POINT ( 'NONE',  ( 1.471222536514999790, 1414.913526854310021, 192.0236705776529789 ) ) ;
#55033=CARTESIAN_POINT ( 'NONE',  ( 2.286265947080000416, 1427.727383903629971, 112.4493539157979995 ) ) ;
#55037=CARTESIAN_POINT ( 'NONE',  ( -25.17722015988540107, 1451.311918859900061, 137.3180140832189693 ) ) ;
#55038=CARTESIAN_POINT ( 'NONE',  ( 10.52994085932536272, 1438.877686223792125, 152.6194632825565236 ) ) ;
#55039=CARTESIAN_POINT ( 'NONE',  ( 11.03217570710000039, 1409.298312452229993, 227.8647431501979952 ) ) ;
#55042=CARTESIAN_POINT ( 'NONE',  ( 41.37151551531449911, 1441.555306590669943, 134.0999999980749919 ) ) ;
#55044=EDGE_LOOP ( 'NONE', ( #11002, #44807, #26909, #108040, #108029 ) ) ;
#55048=ORIENTED_EDGE ( 'NONE', *, *, #21584, .T. ) ;
#55049=ORIENTED_EDGE ( 'NONE', *, *, #88350, .T. ) ;
#55052=EDGE_CURVE ( 'NONE', #35056, #58564, #67642, .T. ) ;
#55053=CARTESIAN_POINT ( 'NONE',  ( 15.12819912197481997, 1451.147586662198137, 149.6391027733497765 ) ) ;
#55054=AXIS2_PLACEMENT_3D ( 'NONE', #69279, #52476, #86604 ) ;
#55060=CARTESIAN_POINT ( 'NONE',  ( 8.469420064130000370, 1416.216252248729916, 193.1369149110980175 ) ) ;
#55065=CARTESIAN_POINT ( 'NONE',  ( 27.48763482353140120, 1440.913060387330006, 246.3050835912150092 ) ) ;
#55069=FACE_OUTER_BOUND ( 'NONE', #36849, .T. ) ;
#55071=CARTESIAN_POINT ( 'NONE',  ( -22.53878221424140094, 1411.058442688259902, 212.0450776560099939 ) ) ;
#55072=CARTESIAN_POINT ( 'NONE',  ( -24.90627924569999863, 1441.326908584029979, 210.4393126625480193 ) ) ;
#55073=DIRECTION ( 'NONE',  ( -0.7074300732343287157, -0.02470400251501369063, -0.7063514732365258064 ) ) ;
#55076=CARTESIAN_POINT ( 'NONE',  ( 13.19226977985399962, 1436.077122747240082, 150.6574760380860312 ) ) ;
#55077=CARTESIAN_POINT ( 'NONE',  ( -2.178197975999999869, 1509.061250285029928, 179.3703848074979987 ) ) ;
#55079=CARTESIAN_POINT ( 'NONE',  ( -13.99196149959999858, 1471.299568757930047, 192.9718935549979903 ) ) ;
#55080=CARTESIAN_POINT ( 'NONE',  ( 7.920313882610000356, 1463.549343347430067, 235.1949569295980211 ) ) ;
#55085=CARTESIAN_POINT ( 'NONE',  ( 0.1681681984989999989, 1405.973120458229914, 121.6099336315979969 ) ) ;
#55088=CARTESIAN_POINT ( 'NONE',  ( -22.18308977499999912, 1506.802866779929900, 208.9507517862349744 ) ) ;
#55092=CARTESIAN_POINT ( 'NONE',  ( -0.6414547015529999952, 1416.067629290630066, 227.6224876852980117 ) ) ;
#55093=CARTESIAN_POINT ( 'NONE',  ( 27.85865497370000199, 1444.561642193520129, 231.9580019065979855 ) ) ;
#55094=EDGE_CURVE ( 'NONE', #66425, #78889, #110551, .T. ) ;
#55097=CARTESIAN_POINT ( 'NONE',  ( -0.2658002863356170309, 1507.120020817209934, 237.3289691923420150 ) ) ;
#55098=ADVANCED_FACE ( 'NONE', ( #19386 ), #80314, .F. ) ;
#55101=EDGE_CURVE ( 'NONE', #46504, #78944, #100914, .T. ) ;
#55102=CARTESIAN_POINT ( 'NONE',  ( -22.49223445950000055, 1444.795317305830167, 218.7498400625879924 ) ) ;
#55104=CARTESIAN_POINT ( 'NONE',  ( -1.855538017380000015, 1485.200156903630159, 182.6439197069979912 ) ) ;
#55106=EDGE_LOOP ( 'NONE', ( #51892, #21241, #99739, #10238 ) ) ;
#55109=CARTESIAN_POINT ( 'NONE',  ( 1.318101111460000086, 1406.519676335630038, 269.4981145789980133 ) ) ;
#55112=EDGE_CURVE ( 'NONE', #23029, #1304, #21854, .T. ) ;
#55114=CARTESIAN_POINT ( 'NONE',  ( 42.28244518683229813, 1445.873630544700063, 269.8809842817969411 ) ) ;
#55116=CARTESIAN_POINT ( 'NONE',  ( 10.63894069730948466, 1424.089672982063576, 137.5854534913812586 ) ) ;
#55118=CARTESIAN_POINT ( 'NONE',  ( -2.318887826942909847, 1449.808491734400150, 155.3361412615429913 ) ) ;
#55119=CARTESIAN_POINT ( 'NONE',  ( -40.07811080949989702, 1443.844543801569898, 135.1422523984039969 ) ) ;
#55121=CARTESIAN_POINT ( 'NONE',  ( -13.86388155186750026, 1415.301705645010088, 220.7860354755530068 ) ) ;
#55122=CARTESIAN_POINT ( 'NONE',  ( 20.15452300067990166, 1507.845791525220193, 189.3412703910400126 ) ) ;
#55125=CARTESIAN_POINT ( 'NONE',  ( -4.540901344669999951, 1419.211677879630088, 248.0989693021979861 ) ) ;
#55126=EDGE_CURVE ( 'NONE', #19628, #35056, #78341, .T. ) ;
#55128=CARTESIAN_POINT ( 'NONE',  ( -0.3397000419900000345, 1476.049357295929894, 268.4837298515980137 ) ) ;
#55132=EDGE_CURVE ( 'NONE', #48130, #64548, #38270, .T. ) ;
#55133=DIRECTION ( 'NONE',  ( -0.8383970168982890492, -0.5450600352768950607, 0.000000000000000000 ) ) ;
#55135=B_SPLINE_CURVE_WITH_KNOTS ( 'NONE', 3,
 ( #11108, #57526, #72134, #89450, #91650, #48005, #21666, #5993, #98939, #31189, #64273, #5442, #22214 ),
 .UNSPECIFIED., .F., .F.,
 ( 4, 2, 2, 1, 2, 2, 4 ),
 ( 0.000000000000000000, 0.2500000000000208722, 0.3750000000000297540, 0.4375000000000330846, 0.4687500000000325850, 0.5000000000000320854, 1.000000000000000000 ),
 .UNSPECIFIED. ) ;
#55140=CARTESIAN_POINT ( 'NONE',  ( -4.104299670009800671, 1396.056385690520074, 219.3587915975870146 ) ) ;
#55141=EDGE_CURVE ( 'NONE', #54528, #83462, #75567, .T. ) ;
#55142=CARTESIAN_POINT ( 'NONE',  ( -15.36549427490000141, 1420.414141484729953, 227.0219848979980100 ) ) ;
#55145=CARTESIAN_POINT ( 'NONE',  ( 2.196223613969999988, 1409.923853850330033, 231.8398400339980014 ) ) ;
#55146=CARTESIAN_POINT ( 'NONE',  ( -10.31340658039999880, 1484.355420805929953, 185.0384118475980131 ) ) ;
#55147=CARTESIAN_POINT ( 'NONE',  ( 11.23345602649999897, 1426.040909930530006, 115.7213397327980005 ) ) ;
#55149=CARTESIAN_POINT ( 'NONE',  ( -0.2658540493943280514, 1507.120020986029886, 237.3289608297170048 ) ) ;
#55150=FACE_OUTER_BOUND ( 'NONE', #86577, .T. ) ;
#55155=CARTESIAN_POINT ( 'NONE',  ( 7.385876586370000219, 1509.171843810430119, 180.6941627112979916 ) ) ;
#55161=ORIENTED_EDGE ( 'NONE', *, *, #22928, .T. ) ;
#55162=CARTESIAN_POINT ( 'NONE',  ( -10.19366155880000058, 1396.792506850929840, 201.2442953279479809 ) ) ;
#55163=CARTESIAN_POINT ( 'NONE',  ( -15.12918126009999931, 1409.441383038730010, 192.4788841068979934 ) ) ;
#55164=CARTESIAN_POINT ( 'NONE',  ( -17.78508617079999610, 1435.118679338368793, 145.5186544196980094 ) ) ;
#55167=CARTESIAN_POINT ( 'NONE',  ( 17.60565453690000126, 1410.875554451929929, 225.2140679527979898 ) ) ;
#55168=CARTESIAN_POINT ( 'NONE',  ( 8.522139242040001506, 1410.293599720429938, 187.8412052867980151 ) ) ;
#55170=CARTESIAN_POINT ( 'NONE',  ( -40.20780054482000310, 1448.389597071610069, 135.4753047060349900 ) ) ;
#55171=CARTESIAN_POINT ( 'NONE',  ( 39.12852302555769768, 1437.672249968900132, 135.5512840573979929 ) ) ;
#55173=CARTESIAN_POINT ( 'NONE',  ( -26.96382314767709687, 1437.662753688059865, 136.8825050232889851 ) ) ;
#55174=CARTESIAN_POINT ( 'NONE',  ( 11.82297588149999967, 1429.270096893229947, 149.5722024081979953 ) ) ;
#55175=CARTESIAN_POINT ( 'NONE',  ( 41.15075515969999742, 1443.752813495769942, 136.9300362400979907 ) ) ;
#55176=ORIENTED_EDGE ( 'NONE', *, *, #52178, .F. ) ;
#55179=ORIENTED_EDGE ( 'NONE', *, *, #76917, .F. ) ;
#55183=CARTESIAN_POINT ( 'NONE',  ( -13.88147930949999953, 1460.663431784329987, 231.8849065275979910 ) ) ;
#55192=CARTESIAN_POINT ( 'NONE',  ( 17.17379625170000423, 1415.087974639930053, 212.6822280708980202 ) ) ;
#55195=CARTESIAN_POINT ( 'NONE',  ( 11.68203264560385790, 1433.008677914359623, 150.9219369944972868 ) ) ;
#55196=CARTESIAN_POINT ( 'NONE',  ( -3.200019046440000015, 1409.961299637529919, 232.4470946617979905 ) ) ;
#55197=CARTESIAN_POINT ( 'NONE',  ( -9.668109322589998555, 1408.913060387329779, 193.5713027961979833 ) ) ;
#55200=PLANE ( 'NONE',  #31751 ) ;
#55202=VECTOR ( 'NONE', #75137, 1000.000000000000114 ) ;
#55203=CARTESIAN_POINT ( 'NONE',  ( 20.15862645124139974, 1413.250162082850011, 270.0907330008120653 ) ) ;
#55206=CARTESIAN_POINT ( 'NONE',  ( 23.51556281730000109, 1410.708086401529954, 207.8137393032480134 ) ) ;
#55211=CARTESIAN_POINT ( 'NONE',  ( 4.325241530647730315, 1421.953609801759967, 183.9658289457019862 ) ) ;
#55212=CARTESIAN_POINT ( 'NONE',  ( -2.344105919239999558, 1417.913736160830013, 233.0442052094980170 ) ) ;
#55218=ADVANCED_FACE ( 'NONE', ( #29195 ), #95458, .T. ) ;
#55219=CARTESIAN_POINT ( 'NONE',  ( 10.98083629090000102, 1433.016921068679949, 151.7694307944979926 ) ) ;
#55225=CARTESIAN_POINT ( 'NONE',  ( 18.67054467720000233, 1509.506033878430117, 187.1506692567980110 ) ) ;
#55227=EDGE_LOOP ( 'NONE', ( #52485, #73900, #72259, #54612 ) ) ;
#55229=CARTESIAN_POINT ( 'NONE',  ( 27.78452742954910093, 1508.000976259739900, 207.7754991261529938 ) ) ;
#55233=CARTESIAN_POINT ( 'NONE',  ( -14.94707557629999961, 1464.258769156330118, 228.3755978434980136 ) ) ;
#55236=CARTESIAN_POINT ( 'NONE',  ( -26.76158160278550113, 1509.153336901769990, 201.3770876523819879 ) ) ;
#55238=CARTESIAN_POINT ( 'NONE',  ( -19.40520978109999817, 1426.254488764730240, 225.7391413128980275 ) ) ;
#55239=CARTESIAN_POINT ( 'NONE',  ( -15.59584108210000153, 1436.279046110379795, 149.2248470810979768 ) ) ;
#55240=CARTESIAN_POINT ( 'NONE',  ( -9.660544699540000835, 1432.353341358199941, 148.7316627034979888 ) ) ;
#55242=CARTESIAN_POINT ( 'NONE',  ( 0.9518847404210000196, 1415.296882282229944, 191.1939211731979924 ) ) ;
#55243=CARTESIAN_POINT ( 'NONE',  ( 28.26971844670000422, 1508.651302070430120, 209.4063442215349937 ) ) ;
#55246=( NAMED_UNIT ( * ) SI_UNIT ( $, .STERADIAN. ) SOLID_ANGLE_UNIT ( ) );
#55247=DIRECTION ( 'NONE',  ( -0.5412924984494058567, 0.1391731009594480151, 0.8292365640103740443 ) ) ;
#55248=CARTESIAN_POINT ( 'NONE',  ( 11.57168670579999947, 1440.669964955550086, 147.8294280051980252 ) ) ;
#55249=B_SPLINE_CURVE_WITH_KNOTS ( 'NONE', 3,
 ( #44301, #19055, #45412, #94123 ),
 .UNSPECIFIED., .F., .F.,
 ( 4, 4 ),
 ( 0.000000000000000000, 1.000000000000000000 ),
 .UNSPECIFIED. ) ;
#55253=CARTESIAN_POINT ( 'NONE',  ( -0.2626388801599250367, 1424.255108689230156, 227.7923674788299877 ) ) ;
#55255=CARTESIAN_POINT ( 'NONE',  ( 15.28420222229999936, 1497.713060387329961, 224.4060481836980046 ) ) ;
#55257=CARTESIAN_POINT ( 'NONE',  ( -24.80269070334470172, 1438.943490319260036, 210.4397421548250122 ) ) ;
#55266=CARTESIAN_POINT ( 'NONE',  ( 22.22649075570000221, 1507.849990204029837, 192.4185849886980009 ) ) ;
#55269=CARTESIAN_POINT ( 'NONE',  ( -0.4719925911955576980, 1416.019047136214112, 233.4884116122769910 ) ) ;
#55270=EDGE_LOOP ( 'NONE', ( #5259, #105571, #63721, #64640 ) ) ;
#55275=CARTESIAN_POINT ( 'NONE',  ( 12.74312375647451923, 1442.824085801858928, 169.4555944935701746 ) ) ;
#55276=CARTESIAN_POINT ( 'NONE',  ( 16.10313873473633706, 1412.736108363146059, 269.3694952781954726 ) ) ;
#55277=CARTESIAN_POINT ( 'NONE',  ( -31.69751081680000127, 1445.012237272740094, 244.1892870111979903 ) ) ;
#55279=CARTESIAN_POINT ( 'NONE',  ( -11.56494095969999947, 1433.721084582969979, 151.2190265359980117 ) ) ;
#55281=CARTESIAN_POINT ( 'NONE',  ( -19.19763038940000044, 1485.731754976029833, 189.6998267162979914 ) ) ;
#55283=CARTESIAN_POINT ( 'NONE',  ( -26.17054985310000248, 1441.643302933269752, 138.0857573384980128 ) ) ;
#55285=SPHERICAL_SURFACE ( 'NONE', #92654, 2.000000000000000000 ) ;
#55286=CARTESIAN_POINT ( 'NONE',  ( 13.02959953899969925, 1428.519719725350114, 223.5607415246620064 ) ) ;
#55287=CARTESIAN_POINT ( 'NONE',  ( -15.22421469840265473, 1509.566647593047492, 235.0174151826843172 ) ) ;
#55288=CARTESIAN_POINT ( 'NONE',  ( 4.323339341317169361E-09, 1410.103346783880170, 258.3459216912629586 ) ) ;
#55289=ORIENTED_EDGE ( 'NONE', *, *, #836, .F. ) ;
#55293=CARTESIAN_POINT ( 'NONE',  ( -26.02835829340000018, 1468.278484548229926, 269.9886483896979712 ) ) ;
#55294=CARTESIAN_POINT ( 'NONE',  ( -23.93171212618479515, 1435.912476962626442, 211.2679597967069753 ) ) ;
#55298=CARTESIAN_POINT ( 'NONE',  ( -13.67687855990000045, 1421.535259874829990, 230.0823906799980136 ) ) ;
#55301=CARTESIAN_POINT ( 'NONE',  ( -45.75303381261710456, 1435.540604548129977, 267.6079231741339868 ) ) ;
#55303=CARTESIAN_POINT ( 'NONE',  ( -3.538418511287639845, 1496.496384395020186, 181.4297818474599922 ) ) ;
#55305=EDGE_LOOP ( 'NONE', ( #25587, #60935, #83397 ) ) ;
#55308=CARTESIAN_POINT ( 'NONE',  ( -20.59664500250000074, 1507.763472350229904, 190.3621299374980254 ) ) ;
#55309=CARTESIAN_POINT ( 'NONE',  ( -15.76506831160000210, 1425.421718464029937, 190.4794369252980175 ) ) ;
#55310=TOROIDAL_SURFACE ( 'NONE', #46367, 4.000000000000000000, 1.000000000000000000 ) ;
#55311=CARTESIAN_POINT ( 'NONE',  ( -16.72257612350379929, 1470.459515107609832, 228.5670331555560040 ) ) ;
#55314=( BOUNDED_CURVE ( )  B_SPLINE_CURVE ( 3, ( #71370, #4137, #47229, #47777 ),
 .UNSPECIFIED., .F., .F. ) 
 B_SPLINE_CURVE_WITH_KNOTS ( ( 4, 4 ),
 ( 6.031750460840100025, 6.430154037858700100 ),
 .UNSPECIFIED. ) 
 CURVE ( )  GEOMETRIC_REPRESENTATION_ITEM ( )  RATIONAL_B_SPLINE_CURVE ( ( 1.000000000000000000, 0.9868165638310153476, 0.9868165638310153476, 1.000000000000000000 ) ) 
 REPRESENTATION_ITEM ( '' )  );
#55320=CARTESIAN_POINT ( 'NONE',  ( -8.333309592260910392, 1410.827525919379923, 269.6222470930029544 ) ) ;
#55321=CARTESIAN_POINT ( 'NONE',  ( -33.52368697869999892, 1435.668148531879979, 135.0787117157979935 ) ) ;
#55325=ORIENTED_EDGE ( 'NONE', *, *, #105782, .T. ) ;
#55326=CARTESIAN_POINT ( 'NONE',  ( 45.61858855260545909, 1441.895270504249311, 268.9752554369495670 ) ) ;
#55328=CARTESIAN_POINT ( 'NONE',  ( -13.72744925206639977, 1436.207725120319992, 150.3866072345499845 ) ) ;
#55329=CARTESIAN_POINT ( 'NONE',  ( -1.097975305679999902, 1484.781735349930159, 182.0978467051980090 ) ) ;
#55331=CARTESIAN_POINT ( 'NONE',  ( -18.05107215653380237, 1415.301705641620174, 207.5664288050670052 ) ) ;
#55332=CARTESIAN_POINT ( 'NONE',  ( -20.05750684869999745, 1435.770533046819992, 223.2611708394980212 ) ) ;
#55334=CARTESIAN_POINT ( 'NONE',  ( 10.62371075008579879, 1475.245696748350156, 266.9320703371920445 ) ) ;
#55335=CARTESIAN_POINT ( 'NONE',  ( -1.521307588799736710, 1467.014991327842608, 235.3760082200168995 ) ) ;
#55339=CARTESIAN_POINT ( 'NONE',  ( -40.71747595469150127, 1448.637563191999789, 135.6928038576120059 ) ) ;
#55343=CARTESIAN_POINT ( 'NONE',  ( 25.32437023980250146, 1451.152985641890155, 137.2266721702760037 ) ) ;
#55344=CARTESIAN_POINT ( 'NONE',  ( 14.34198504589999956, 1416.067629296030191, 196.9709775078979987 ) ) ;
#55345=CARTESIAN_POINT ( 'NONE',  ( 2.446787376320000096, 1432.353341358199941, 150.2884730787980061 ) ) ;
#55346=CARTESIAN_POINT ( 'NONE',  ( 20.84719162220000044, 1410.135659111530003, 199.9772158389280037 ) ) ;
#55347=CARTESIAN_POINT ( 'NONE',  ( 21.92806520379999924, 1409.678805295229949, 207.4538581684380176 ) ) ;
#55348=CARTESIAN_POINT ( 'NONE',  ( 16.47946573069999943, 1409.488537697930042, 225.3830611371980126 ) ) ;
#55351=AXIS2_PLACEMENT_3D ( 'NONE', #81464, #23768, #75312 ) ;
#55354=VERTEX_POINT ( 'NONE', #49309 ) ;
#55356=CARTESIAN_POINT ( 'NONE',  ( -43.33646147129999804, 1450.475004575490175, 269.7148345228980020 ) ) ;
#55357=CARTESIAN_POINT ( 'NONE',  ( -3.090150069089999896, 1448.281854555830023, 184.7281458456979806 ) ) ;
#55360=CARTESIAN_POINT ( 'NONE',  ( -40.24977539805779969, 1444.418635764679948, 137.0616282298240094 ) ) ;
#55361=CARTESIAN_POINT ( 'NONE',  ( 10.89360413264559924, 1424.843095330547385, 138.2325533482020887 ) ) ;
#55362=CARTESIAN_POINT ( 'NONE',  ( 1.871535769766313972, 1416.945233345094721, 232.8591253669631840 ) ) ;
#55363=AXIS2_PLACEMENT_3D ( 'NONE', #83619, #104154, #103601 ) ;
#55364=CARTESIAN_POINT ( 'NONE',  ( -1.736824869533450055, 1471.314969352929893, 183.3216726285400284 ) ) ;
#55365=CARTESIAN_POINT ( 'NONE',  ( 11.42843422490000016, 1433.204776730410003, 151.3497024267980180 ) ) ;
#55367=CARTESIAN_POINT ( 'NONE',  ( -0.2979719656898799918, 1474.175163955769904, 270.1377477033279888 ) ) ;
#55368=CARTESIAN_POINT ( 'NONE',  ( 33.36193798735060057, 1440.913060383689981, 247.4361487871759948 ) ) ;
#55370=DIRECTION ( 'NONE',  ( 0.000000000000000000, 0.000000000000000000, 1.000000000000000000 ) ) ;
#55376=CARTESIAN_POINT ( 'NONE',  ( 2.366960022969999855, 1499.008374605230074, 235.6905257228980020 ) ) ;
#55378=CARTESIAN_POINT ( 'NONE',  ( -10.16696763180000040, 1507.687626859330067, 234.4265286207979955 ) ) ;
#55381=CARTESIAN_POINT ( 'NONE',  ( 9.874625061749998878, 1408.732483999830038, 219.1535762145979902 ) ) ;
#55382=DIRECTION ( 'NONE',  ( 0.03489949670250328678, 0.9993908270190956511, 0.000000000000000000 ) ) ;
#55383=CARTESIAN_POINT ( 'NONE',  ( 1.668433438889999954, 1465.936335742929941, 234.8595247571979883 ) ) ;
#55386=CARTESIAN_POINT ( 'NONE',  ( -1.062268994950000156, 1452.003535646829960, 183.5021093084980066 ) ) ;
#55387=VECTOR ( 'NONE', #76015, 1000.000000000000000 ) ;
#55391=CARTESIAN_POINT ( 'NONE',  ( -17.78809123684730054, 1415.431750870129918, 208.6136599671049794 ) ) ;
#55397=SPHERICAL_SURFACE ( 'NONE', #97714, 2.000000000000000000 ) ;
#55401=CARTESIAN_POINT ( 'NONE',  ( 19.94580949735431119, 1509.638862839826970, 187.1591372636853237 ) ) ;
#55402=CARTESIAN_POINT ( 'NONE',  ( 3.284408969210909746, 1409.027754475830079, 194.4977616889150056 ) ) ;
#55405=CARTESIAN_POINT ( 'NONE',  ( -19.22188682119999825, 1463.226638649430242, 191.5163928844979750 ) ) ;
#55407=VECTOR ( 'NONE', #25302, 1000.000000000000000 ) ;
#55408=ORIENTED_EDGE ( 'NONE', *, *, #12469, .T. ) ;
#55411=CARTESIAN_POINT ( 'NONE',  ( -11.20854089327220038, 1414.996442620800053, 195.7122650692939771 ) ) ;
#55413=CARTESIAN_POINT ( 'NONE',  ( -5.978054922203370145E-10, 1467.128867830870149, 245.4363362049380157 ) ) ;
#55414=CARTESIAN_POINT ( 'NONE',  ( -20.08192399753360036, 1491.083939665490107, 190.8757460896890166 ) ) ;
#55415=CARTESIAN_POINT ( 'NONE',  ( -33.91376666158920017, 1435.681799711289841, 142.5056097235880088 ) ) ;
#55417=CARTESIAN_POINT ( 'NONE',  ( 0.2140911838630000230, 1455.057671371630022, 183.1651298794979823 ) ) ;
#55419=CARTESIAN_POINT ( 'NONE',  ( -26.53007446348713216, 1436.732360642813092, 136.8044313116533033 ) ) ;
#55420=CARTESIAN_POINT ( 'NONE',  ( -21.91582132105330061, 1491.015012752149914, 208.5287076380759856 ) ) ;
#55423=CARTESIAN_POINT ( 'NONE',  ( 11.31370220690210004, 1433.949489476620101, 151.5139277432949996 ) ) ;
#55424=CARTESIAN_POINT ( 'NONE',  ( -13.38570636064689801, 1434.932240567770123, 149.1199053445120057 ) ) ;
#55427=B_SPLINE_SURFACE_WITH_KNOTS ( 'NONE', 5, 5, ( 
 ( #91737, #49209, #107432, #83337, #109114, #66575 ),
 ( #100680, #99023, #23963, #7193, #92288, #30727 ),
 ( #75518, #67117, #24516, #58706, #64912, #18324 ),
 ( #17755, #92838, #26174, #34038, #95057, #16114 ),
 ( #9941, #68775, #1562, #52515, #93932, #25620 ),
 ( #33467, #44113, #102876, #103433, #34590, #35694 ),
 ( #35142, #69883, #43556, #77164, #78248, #7732 ),
 ( #466, #60361, #85527, #103999, #84446, #86645 ),
 ( #26739, #110194, #27296, #77706, #102335, #50319 ),
 ( #94483, #41893, #43006, #68229, #51394, #59812 ),
 ( #76050, #8821, #67668, #101774, #60927, #51958 ),
 ( #86100, #9393, #1016, #69325, #17198, #25065 ),
 ( #59268, #93385, #16652, #50849, #84978, #8272 ),
 ( #42437, #76596, #110747, #27853, #54186, #70997 ),
 ( #78812, #36806, #20528, #79367, #105679, #62034 ),
 ( #12147, #88313, #72097, #11606, #45784, #44671 ),
 ( #5829, #95604, #96157, #19434, #80468, #18872 ),
 ( #19993, #53634, #79919, #53070, #70439, #54734 ),
 ( #82533, #39968, #36251, #28407, #62605, #28963 ),
 ( #48390, #96720, #61477, #3232, #74144, #37360 ),
 ( #106212, #11058, #87777, #104558, #2681, #3784 ) ),
 .UNSPECIFIED., .F., .F., .F.,
 ( 6, 3, 3, 3, 3, 3, 6 ),
 ( 6, 6 ),
 ( 7.218912043000000445, 9.328012329869999064, 9.942138423719999452, 11.64113835680000086, 13.34013828990000050, 16.73813815620000156, 26.25736426930000178 ),
 ( 0.000000000000000000, 1.452619041900000019 ),
 .UNSPECIFIED. ) ;
#55428=CARTESIAN_POINT ( 'NONE',  ( 0.9043163146260000396, 1416.826388498530150, 190.2146394413979920 ) ) ;
#55430=CARTESIAN_POINT ( 'NONE',  ( -0.03226023477341029982, 1410.297896964309984, 185.0217421575940193 ) ) ;
#55432=CARTESIAN_POINT ( 'NONE',  ( 22.71362857069999919, 1419.354696852330108, 250.3594883046980044 ) ) ;
#55433=CARTESIAN_POINT ( 'NONE',  ( -25.79285008269999935, 1449.806912625419727, 208.9767609917279856 ) ) ;
#55434=CARTESIAN_POINT ( 'NONE',  ( -10.73442984997090122, 1425.687098426139983, 96.72829437425519927 ) ) ;
#55435=CARTESIAN_POINT ( 'NONE',  ( -17.37499910009999837, 1409.684548448330133, 195.3411345723980048 ) ) ;
#55439=CARTESIAN_POINT ( 'NONE',  ( -25.00557955649999897, 1440.913060507210048, 216.3898167415980254 ) ) ;
#55444=CARTESIAN_POINT ( 'NONE',  ( 30.22859042230000171, 1450.569347608749922, 136.3539440427979912 ) ) ;
#55448=CARTESIAN_POINT ( 'NONE',  ( 14.38071629740000112, 1509.494656480429967, 235.3234905946980007 ) ) ;
#55449=EDGE_LOOP ( 'NONE', ( #12863, #29938, #57128, #103918 ) ) ;
#55450=ORIENTED_EDGE ( 'NONE', *, *, #93946, .T. ) ;
#55451=CARTESIAN_POINT ( 'NONE',  ( -10.75295827156603679, 1424.459136614693080, 137.8404512415733905 ) ) ;
#55453=B_SPLINE_CURVE_WITH_KNOTS ( 'NONE', 5,
 ( #79458, #69978, #70529, #27943, #28495, #2222, #61564, #77797, #63237, #11692, #78916, #18965, #27385, #19525, #45866, #53160, #26838, #36335, #69422, #104093, #105766 ),
 .UNSPECIFIED., .F., .F.,
 ( 6, 3, 3, 3, 3, 3, 6 ),
 ( 0.000000000000000000, 0.08423072362349257047, 0.2167650270835284054, 0.3492993305435642126, 0.4887865076447485690, 0.6285375814380548265, 1.000000000000000000 ),
 .UNSPECIFIED. ) ;
#55456=CARTESIAN_POINT ( 'NONE',  ( 7.630940151131325067, 1446.706835311024179, 154.1372093844152857 ) ) ;
#55457=CARTESIAN_POINT ( 'NONE',  ( -0.1872094492630000107, 1489.066837873730037, 236.5711787574979894 ) ) ;
#55458=CARTESIAN_POINT ( 'NONE',  ( -1.499721489806784991, 1420.769012360254237, 184.5717010710991701 ) ) ;
#55460=CARTESIAN_POINT ( 'NONE',  ( 10.81512807170000023, 1424.921141247430114, 144.1662922863980043 ) ) ;
#55467=CARTESIAN_POINT ( 'NONE',  ( 12.93986011685568194, 1442.913450493105529, 187.0956378267197238 ) ) ;
#55469=VERTEX_POINT ( 'NONE', #31383 ) ;
#55472=CARTESIAN_POINT ( 'NONE',  ( 10.83634816680000057, 1507.403084768729968, 234.1451693812979897 ) ) ;
#55473=B_SPLINE_CURVE_WITH_KNOTS ( 'NONE', 3,
 ( #477, #26184, #77174, #59823, #110202, #87220, #10510, #93943, #34601, #97812, #2139, #97266, #96735, #46898, #29509, #37929, #37372, #70450, #11620, #106764, #55294, #21091, #44682, #20542, #36261, #54746 ),
 .UNSPECIFIED., .F., .F.,
 ( 4, 2, 2, 2, 1, 1, 2, 2, 2, 2, 1, 1, 2, 2, 4 ),
 ( 0.000000000000000000, 0.1250000000007177869, 0.2500000000014355739, 0.3750000000021533886, 0.4375000000025118796, 0.4687500000026916247, 0.4843750000027603475, 0.5000000000028289593, 0.6250000000029628522, 0.6875000000030297986, 0.7187500000030208058, 0.7343750000030150327, 0.7421875000029918290, 0.7500000000029686253, 1.000000000000000000 ),
 .UNSPECIFIED. ) ;
#55475=CARTESIAN_POINT ( 'NONE',  ( 14.11531660217920070, 1452.420142669970119, 148.4568864021009915 ) ) ;
#55476=CONICAL_SURFACE ( 'NONE', #98378, 1.000000000000009104, 0.7853981633970000820 ) ;
#55481=CARTESIAN_POINT ( 'NONE',  ( -2.500000000000000000, 1440.913060387330006, 209.1218459616979999 ) ) ;
#55482=CARTESIAN_POINT ( 'NONE',  ( -18.65765733967990059, 1472.695501767010001, 189.9835944018950329 ) ) ;
#55483=CARTESIAN_POINT ( 'NONE',  ( -3.509649680925187365, 1486.092192652074573, 181.9936301291397172 ) ) ;
#55485=CARTESIAN_POINT ( 'NONE',  ( -25.25982536658409927, 1509.711778463150040, 222.8936294031860257 ) ) ;
#55488=CARTESIAN_POINT ( 'NONE',  ( 5.995204332980000249E-15, 1425.981674191730008, 219.6133832206979832 ) ) ;
#55504=CARTESIAN_POINT ( 'NONE',  ( 11.87175427299999875, 1419.759279977630058, 229.4984939635980083 ) ) ;
#55508=CARTESIAN_POINT ( 'NONE',  ( 39.20291624600000091, 1422.646355417429959, 268.9552502776979281 ) ) ;
#55509=CARTESIAN_POINT ( 'NONE',  ( -18.69670922599999940, 1410.928318842029967, 223.5482325157979915 ) ) ;
#55510=CARTESIAN_POINT ( 'NONE',  ( 23.19273066879999945, 1435.733997910429935, 140.7572724421980013 ) ) ;
#55511=CARTESIAN_POINT ( 'NONE',  ( 20.66442127730000067, 1508.014906299830045, 190.0377508468980068 ) ) ;
#55512=CARTESIAN_POINT ( 'NONE',  ( 19.54819107935938760, 1426.815560993606596, 223.9911639112806654 ) ) ;
#55514=CARTESIAN_POINT ( 'NONE',  ( 12.45702690689999947, 1416.837177091229705, 223.4766769983980055 ) ) ;
#55516=CARTESIAN_POINT ( 'NONE',  ( -41.18636360906929639, 1440.753229491839875, 135.3771605954950132 ) ) ;
#55517=CARTESIAN_POINT ( 'NONE',  ( 0.2111961702294640197, 1456.676537660760005, 183.0956732919689784 ) ) ;
#55518=CARTESIAN_POINT ( 'NONE',  ( -13.12463360019999925, 1409.312163186730004, 216.5379860103879821 ) ) ;
#55519=CARTESIAN_POINT ( 'NONE',  ( 0.3823997583379999954, 1418.629108576230010, 184.6943103907979946 ) ) ;
#55523=CARTESIAN_POINT ( 'NONE',  ( 13.50135279390000065, 1434.968981356529866, 147.2733250035980177 ) ) ;
#55524=CARTESIAN_POINT ( 'NONE',  ( -38.86831401713799750, 1437.615293294849835, 134.0999999973729757 ) ) ;
#55525=CARTESIAN_POINT ( 'NONE',  ( 7.263998328199999577, 1441.808077109380065, 185.0069966186979968 ) ) ;
#55526=VERTEX_POINT ( 'NONE', #27396 ) ;
#55527=B_SPLINE_CURVE_WITH_KNOTS ( 'NONE', 3,
 ( #39245, #22412, #56615, #41469, #42558, #76710 ),
 .UNSPECIFIED., .F., .F.,
 ( 4, 2, 4 ),
 ( 1.348807851242469857E-06, 0.1489810127399329998, 0.2938202807443149878 ),
 .UNSPECIFIED. ) ;
#55529=CARTESIAN_POINT ( 'NONE',  ( -9.301708524574189951, 1409.237883206610150, 220.8339435818900256 ) ) ;
#55533=CARTESIAN_POINT ( 'NONE',  ( -15.07741626497340093, 1491.015094518580099, 193.2056053937430136 ) ) ;
#55534=CARTESIAN_POINT ( 'NONE',  ( 40.49911958459973960, 1425.150115471725485, 269.1156650676614390 ) ) ;
#55536=CARTESIAN_POINT ( 'NONE',  ( 18.96350828799999988, 1416.837080254230159, 210.2430641718779896 ) ) ;
#55537=EDGE_CURVE ( 'NONE', #36366, #77650, #104914, .T. ) ;
#55538=CARTESIAN_POINT ( 'NONE',  ( 10.73506988043325627, 1424.972993549859893, 139.1354236083641922 ) ) ;
#55542=CARTESIAN_POINT ( 'NONE',  ( -26.79978786656327827, 1435.433393365130087, 135.4693325801790422 ) ) ;
#55543=CARTESIAN_POINT ( 'NONE',  ( -27.54197030419999948, 1451.496360562029849, 136.1348864480979728 ) ) ;
#55547=EDGE_LOOP ( 'NONE', ( #49595, #89577, #61655, #40431, #77670, #107814 ) ) ;
#55548=CARTESIAN_POINT ( 'NONE',  ( -13.92523544520000023, 1509.057792580229943, 183.7758920630979844 ) ) ;
#55549=CARTESIAN_POINT ( 'NONE',  ( -22.70506393329999995, 1409.705938691230131, 208.9454431684370093 ) ) ;
#55551=CARTESIAN_POINT ( 'NONE',  ( -11.59504266670000128, 1415.140114704729967, 195.4687677443980078 ) ) ;
#55553=FACE_OUTER_BOUND ( 'NONE', #79822, .T. ) ;
#55555=B_SPLINE_SURFACE_WITH_KNOTS ( 'NONE', 5, 1, ( 
 ( #105496, #69147 ),
 ( #53454, #78635 ),
 ( #87599, #9228 ),
 ( #28786, #70830 ),
 ( #37190, #36088 ),
 ( #20362, #10888 ),
 ( #61865, #77534 ),
 ( #43931, #1951 ),
 ( #70273, #104383 ),
 ( #79203, #78075 ),
 ( #69713, #95983 ),
 ( #62986, #103833 ),
 ( #54022, #36634 ),
 ( #27681, #2509 ),
 ( #45060, #97097 ),
 ( #19248, #104940 ),
 ( #28230, #43386 ),
 ( #61319, #62417 ),
 ( #96542, #19817 ),
 ( #88152, #54569 ),
 ( #11440, #3061 ) ),
 .UNSPECIFIED., .F., .F., .F.,
 ( 6, 3, 3, 3, 3, 3, 6 ),
 ( 2, 2 ),
 ( 37.33063420879999939, 38.00991709350000036, 40.59642292560000243, 43.18292875779999918, 44.87875381330000124, 46.52360639289999966, 48.64583233200000478 ),
 ( -0.03002746163920000030, 4.116548514450000695 ),
 .UNSPECIFIED. ) ;
#55556=CARTESIAN_POINT ( 'NONE',  ( -2.921670480139039849, 1414.947723254120092, 186.4090400968400161 ) ) ;
#55558=CARTESIAN_POINT ( 'NONE',  ( -15.22948377059999814, 1422.122177990030195, 227.7536870161980005 ) ) ;
#55564=CARTESIAN_POINT ( 'NONE',  ( -1.801950444790000105, 1417.382180821630072, 235.5933117588980110 ) ) ;
#55568=CARTESIAN_POINT ( 'NONE',  ( -8.437274281626629957, 1485.523202050150076, 184.0031257927479942 ) ) ;
#55572=CARTESIAN_POINT ( 'NONE',  ( 17.64235773549999919, 1415.063410501330054, 210.6787325816779912 ) ) ;
#55574=EDGE_LOOP ( 'NONE', ( #96336, #6244, #98094, #40833 ) ) ;
#55575=ORIENTED_EDGE ( 'NONE', *, *, #31533, .T. ) ;
#55576=CARTESIAN_POINT ( 'NONE',  ( 28.83209696159999780, 1509.870577341629996, 212.5368620444479859 ) ) ;
#55578=CARTESIAN_POINT ( 'NONE',  ( 5.462208593446796989, 1507.217744690670997, 182.0617134843921292 ) ) ;
#55579=EDGE_CURVE ( 'NONE', #34578, #66863, #7532, .T. ) ;
#55580=DIRECTION ( 'NONE',  ( 0.6831251091958939758, -0.2299220283779639940, -0.6931637224008919684 ) ) ;
#55581=CARTESIAN_POINT ( 'NONE',  ( 15.78306734642190357, 1414.214202364269795, 191.4131174284399890 ) ) ;
#55584=EDGE_CURVE ( 'NONE', #60804, #5142, #38063, .T. ) ;
#55586=CARTESIAN_POINT ( 'NONE',  ( -25.29347491494340261, 1450.804999541210009, 137.5161610977569921 ) ) ;
#55587=CARTESIAN_POINT ( 'NONE',  ( 10.61724680206623717, 1438.780641373634808, 152.5602674268187400 ) ) ;
#55588=CARTESIAN_POINT ( 'NONE',  ( 12.45985175859999927, 1409.850499117530035, 228.5793928251979992 ) ) ;
#55591=ADVANCED_FACE ( 'NONE', ( #68331 ), #61509, .T. ) ;
#55592=CARTESIAN_POINT ( 'NONE',  ( 41.10614458601939702, 1440.770232258479837, 134.0999999980669770 ) ) ;
#55596=CARTESIAN_POINT ( 'NONE',  ( -16.73010185348729095, 1410.869507590151898, 226.4351792567899508 ) ) ;
#55602=CARTESIAN_POINT ( 'NONE',  ( -14.59279134157089963, 1436.244781760590058, 149.8708244536879874 ) ) ;
#55605=CARTESIAN_POINT ( 'NONE',  ( -2.959096334900000347, 1485.522887684729994, 182.9002838673980023 ) ) ;
#55606=CARTESIAN_POINT ( 'NONE',  ( -17.08557393600510821, 1449.031093638705670, 219.2146613812218447 ) ) ;
#55609=CARTESIAN_POINT ( 'NONE',  ( 28.25086641300000068, 1508.135711190629991, 209.3856964555159834 ) ) ;
#55610=CARTESIAN_POINT ( 'NONE',  ( 6.194272744020000054, 1415.931669658029932, 192.0649073719980038 ) ) ;
#55611=EDGE_CURVE ( 'NONE', #105306, #68439, #91553, .T. ) ;
#55615=ORIENTED_EDGE ( 'NONE', *, *, #27805, .T. ) ;
#55616=CARTESIAN_POINT ( 'NONE',  ( 11.30241272459999990, 1414.983771848930019, 222.3815203751980221 ) ) ;
#55618=CARTESIAN_POINT ( 'NONE',  ( -0.002288667334423727731, 1451.798321715683869, 154.0444463031279270 ) ) ;
#55621=CARTESIAN_POINT ( 'NONE',  ( -15.43255204080000098, 1409.451976979829851, 192.6616394286979812 ) ) ;
#55624=CARTESIAN_POINT ( 'NONE',  ( -24.15153490410000359, 1438.063247892820073, 212.1983423404379892 ) ) ;
#55627=CARTESIAN_POINT ( 'NONE',  ( 21.85509849029999785, 1410.191647020929850, 266.7712709411979972 ) ) ;
#55628=EDGE_CURVE ( 'NONE', #87844, #80209, #55849, .T. ) ;
#55631=CARTESIAN_POINT ( 'NONE',  ( 6.158422142889999229, 1465.359135116529842, 233.6544522023980051 ) ) ;
#55632=CARTESIAN_POINT ( 'NONE',  ( -23.10442739037580040, 1411.095127590459924, 210.9251608898400150 ) ) ;
#55635=PLANE ( 'NONE',  #28311 ) ;
#55637=CARTESIAN_POINT ( 'NONE',  ( 17.29245831912049525, 1448.484397839388748, 218.0081137152410520 ) ) ;
#55640=( BOUNDED_CURVE ( )  B_SPLINE_CURVE ( 3, ( #32930, #92840, #101220, #16116 ),
 .UNSPECIFIED., .F., .F. ) 
 B_SPLINE_CURVE_WITH_KNOTS ( ( 4, 4 ),
 ( 1.104799058897792063, 2.035744924573262615 ),
 .UNSPECIFIED. ) 
 CURVE ( )  GEOMETRIC_REPRESENTATION_ITEM ( )  RATIONAL_B_SPLINE_CURVE ( ( 1.000000000000000000, 0.9290729278587501749, 0.9290729278587501749, 1.000000000000000000 ) ) 
 REPRESENTATION_ITEM ( '' )  );
#55645=CARTESIAN_POINT ( 'NONE',  ( 4.127212203990000106, 1462.218800617230045, 225.7558667919979882 ) ) ;
#55646=CARTESIAN_POINT ( 'NONE',  ( -11.86315348299999961, 1432.130050080510046, 149.9794296056979874 ) ) ;
#55648=CARTESIAN_POINT ( 'NONE',  ( 1.978507516889999929, 1415.911868808130066, 232.2613842265979827 ) ) ;
#55651=CARTESIAN_POINT ( 'NONE',  ( -18.83990731639999794, 1444.807220488899929, 226.1209739433980133 ) ) ;
#55652=CARTESIAN_POINT ( 'NONE',  ( 2.500000000000000000, 1431.146244464689971, 157.4674042686979760 ) ) ;
#55656=CARTESIAN_POINT ( 'NONE',  ( 2.731915039460000028, 1406.836420814830035, 269.6477045013979819 ) ) ;
#55658=CARTESIAN_POINT ( 'NONE',  ( -22.62861454470000311, 1507.212883763329955, 208.5231287359179930 ) ) ;
#55659=EDGE_CURVE ( 'NONE', #7904, #98527, #109627, .T. ) ;
#55660=CARTESIAN_POINT ( 'NONE',  ( 24.16540420446059656, 1436.369459095317779, 213.4347722490431352 ) ) ;
#55665=CARTESIAN_POINT ( 'NONE',  ( -2.500592283260189674, 1448.944489445770159, 154.5202668489739892 ) ) ;
#55666=CARTESIAN_POINT ( 'NONE',  ( -1.574589970354772550, 1451.357591668891246, 183.8674059166829693 ) ) ;
#55667=CARTESIAN_POINT ( 'NONE',  ( 1.456572784391380049, 1450.690862361819882, 154.5176451698619928 ) ) ;
#55671=CARTESIAN_POINT ( 'NONE',  ( -21.37693747720000204, 1438.522492593769812, 224.8635562210979799 ) ) ;
#55672=EDGE_CURVE ( 'NONE', #18275, #107129, #54163, .T. ) ;
#55673=CARTESIAN_POINT ( 'NONE',  ( 10.85996935512256201, 1424.791572806463819, 138.1869648445997996 ) ) ;
#55674=CARTESIAN_POINT ( 'NONE',  ( 2.711756486579999681, 1440.323160983029993, 158.1834442036979738 ) ) ;
#55676=CARTESIAN_POINT ( 'NONE',  ( -0.7781449114299999748, 1476.045365520429868, 268.4835185334979997 ) ) ;
#55679=CARTESIAN_POINT ( 'NONE',  ( -2.971350363272212025, 1448.268441440509150, 184.4301633348362657 ) ) ;
#55685=CARTESIAN_POINT ( 'NONE',  ( -8.049959547940961357, 1396.194171169660194, 216.6974182996600007 ) ) ;
#55687=CARTESIAN_POINT ( 'NONE',  ( -15.51819189429999923, 1420.489765463529920, 227.0243196332980062 ) ) ;
#55689=CARTESIAN_POINT ( 'NONE',  ( -45.63712941939999723, 1440.717835916950207, 268.9747522934979997 ) ) ;
#55693=CARTESIAN_POINT ( 'NONE',  ( -11.78818130396880015, 1426.417830932260131, 148.5075460829759777 ) ) ;
#55694=AXIS2_PLACEMENT_3D ( 'NONE', #98456, #82766, #64889 ) ;
#55695=CARTESIAN_POINT ( 'NONE',  ( 11.34209814579999964, 1426.458889724530081, 115.7217992701980052 ) ) ;
#55697=CARTESIAN_POINT ( 'NONE',  ( 11.62807272172398498, 1428.982488964479899, 136.1186897298417477 ) ) ;
#55703=CARTESIAN_POINT ( 'NONE',  ( 5.462208597450000092, 1507.217744391630049, 182.0617134992979800 ) ) ;
#55709=ORIENTED_EDGE ( 'NONE', *, *, #78836, .F. ) ;
#55711=CARTESIAN_POINT ( 'NONE',  ( -10.86323185920000078, 1396.351599766229810, 203.8926020820279916 ) ) ;
#55712=DIRECTION ( 'NONE',  ( -0.8926073982886787439, -0.4508348173337058951, 0.000000000000000000 ) ) ;
#55713=CARTESIAN_POINT ( 'NONE',  ( -0.9518847404100000409, 1415.296882282229944, 227.0497707501980074 ) ) ;
#55714=CARTESIAN_POINT ( 'NONE',  ( -13.51610093808350754, 1443.925812197481491, 169.3501091255432982 ) ) ;
#55719=CARTESIAN_POINT ( 'NONE',  ( 17.29603771190000217, 1410.862603898330008, 225.9904529778980304 ) ) ;
#55720=FACE_OUTER_BOUND ( 'NONE', #84786, .T. ) ;
#55723=CARTESIAN_POINT ( 'NONE',  ( -40.62462454117719801, 1446.670089421630109, 136.4950496779409832 ) ) ;
#55724=CARTESIAN_POINT ( 'NONE',  ( 10.91486054658139970, 1396.294215716539838, 207.2818781998020086 ) ) ;
#55726=CARTESIAN_POINT ( 'NONE',  ( 11.82844634479999968, 1429.628886368029953, 149.7692666886979964 ) ) ;
#55730=EDGE_LOOP ( 'NONE', ( #19760, #100454, #37880 ) ) ;
#55733=CARTESIAN_POINT ( 'NONE',  ( -18.33192216791169926, 1488.027226577300098, 229.1094005703429843 ) ) ;
#55735=CARTESIAN_POINT ( 'NONE',  ( -13.34220071569999888, 1434.810047171210044, 195.4053903379979999 ) ) ;
#55743=CARTESIAN_POINT ( 'NONE',  ( 2.500000000000000000, 1448.668275834809947, 158.2599144857439910 ) ) ;
#55746=CARTESIAN_POINT ( 'NONE',  ( 17.56697300799999795, 1414.971439108430104, 210.2828043877179880 ) ) ;
#55750=CARTESIAN_POINT ( 'NONE',  ( -39.37261225819499799, 1430.225544555710712, 269.5993096230814672 ) ) ;
#55751=CARTESIAN_POINT ( 'NONE',  ( -1.541545454019999983, 1409.134736275329942, 232.3518812819980326 ) ) ;
#55752=CARTESIAN_POINT ( 'NONE',  ( -1.910176461450000064E-10, 1497.713060387329961, 187.5067198890980080 ) ) ;
#55756=CARTESIAN_POINT ( 'NONE',  ( -30.92058080866769743, 1440.913060387919813, 241.1530792290629961 ) ) ;
#55758=CARTESIAN_POINT ( 'NONE',  ( -0.3266760126305189860, 1466.747039041310018, 235.5969266249480256 ) ) ;
#55760=CARTESIAN_POINT ( 'NONE',  ( 19.91918620360440428, 1413.854353960929984, 269.3861823084499747 ) ) ;
#55761=EDGE_CURVE ( 'NONE', #7383, #62909, #76732, .T. ) ;
#55765=CARTESIAN_POINT ( 'NONE',  ( 23.71865610989999951, 1410.976819930530155, 207.9578859000980060 ) ) ;
#55768=CARTESIAN_POINT ( 'NONE',  ( -11.60004869885203505, 1425.328126621067440, 136.8077491627233542 ) ) ;
#55770=CARTESIAN_POINT ( 'NONE',  ( 4.173620666753329544, 1421.345241524500125, 185.1232336757030055 ) ) ;
#55771=CARTESIAN_POINT ( 'NONE',  ( -2.809255954350000195, 1417.912686254329856, 232.9149847042980070 ) ) ;
#55776=CARTESIAN_POINT ( 'NONE',  ( 42.46024960829999628, 1454.582938856229930, 266.3335672127980160 ) ) ;
#55783=CARTESIAN_POINT ( 'NONE',  ( 18.18137294690000161, 1507.546748832429785, 186.5307135875980009 ) ) ;
#55790=CARTESIAN_POINT ( 'NONE',  ( 12.93678125246493593, 1396.364822743412560, 211.1704015715083358 ) ) ;
#55791=CARTESIAN_POINT ( 'NONE',  ( 10.76227128012812173, 1434.602751777355252, 151.9483663934211108 ) ) ;
#55794=CARTESIAN_POINT ( 'NONE',  ( -26.60410256373840099, 1508.905103705679949, 201.4398633433799830 ) ) ;
#55795=CARTESIAN_POINT ( 'NONE',  ( 5.020440211750000437, 1420.408409142929941, 185.9185919516980334 ) ) ;
#55796=CARTESIAN_POINT ( 'NONE',  ( -18.69185054180000094, 1425.386843902630062, 225.0351303875980022 ) ) ;
#55797=CARTESIAN_POINT ( 'NONE',  ( -24.31326452180000075, 1436.157794028729995, 139.2594885554979953 ) ) ;
#55799=CARTESIAN_POINT ( 'NONE',  ( 17.74011895019999940, 1509.475909745830222, 187.0027172725980051 ) ) ;
#55801=CARTESIAN_POINT ( 'NONE',  ( 28.47876010940000313, 1509.161042319729859, 209.2859733393400177 ) ) ;
#55809=CARTESIAN_POINT ( 'NONE',  ( -18.54307511480000059, 1508.238692188029972, 229.7339851843979943 ) ) ;
#55811=CARTESIAN_POINT ( 'NONE',  ( -12.71757234210196863, 1442.815512338947428, 186.1937126296973588 ) ) ;
#55812=CARTESIAN_POINT ( 'NONE',  ( 6.251338861372889966, 1407.163727730510118, 197.0599927605450148 ) ) ;
#55820=CARTESIAN_POINT ( 'NONE',  ( -0.4967073565345429542, 1415.438070636819930, 233.3911243540180180 ) ) ;
#55821=VERTEX_POINT ( 'NONE', #7706 ) ;
#55823=CARTESIAN_POINT ( 'NONE',  ( 16.93235272047269646, 1414.913060387399810, 210.7966751255959821 ) ) ;
#55826=CARTESIAN_POINT ( 'NONE',  ( 38.34354232409781815, 1428.425844903683128, 269.5819412675198237 ) ) ;
#55827=CARTESIAN_POINT ( 'NONE',  ( -25.82475785010000280, 1456.303105448329916, 244.3435519225979817 ) ) ;
#55828=CARTESIAN_POINT ( 'NONE',  ( -19.96238765929999914, 1499.092665092829975, 189.4473116693979762 ) ) ;
#55829=CARTESIAN_POINT ( 'NONE',  ( -11.30827943520000112, 1433.910506711959897, 151.5171036033979988 ) ) ;
#55832=CARTESIAN_POINT ( 'NONE',  ( -19.49048793740000107, 1485.728846214529995, 189.9928713767980071 ) ) ;
#55833=CARTESIAN_POINT ( 'NONE',  ( 31.54050948178826985, 1436.927678415763012, 136.6348573598288567 ) ) ;
#55834=CARTESIAN_POINT ( 'NONE',  ( -26.06696396060000254, 1439.602491171669953, 137.5099056270979929 ) ) ;
#55836=CARTESIAN_POINT ( 'NONE',  ( 16.73334775859999723, 1413.089575119930259, 226.5682721348979953 ) ) ;
#55840=CARTESIAN_POINT ( 'NONE',  ( 6.466160837060870069E-09, 1406.204995675689815, 266.5559840362960244 ) ) ;
#55843=CARTESIAN_POINT ( 'NONE',  ( -11.86587318112040101, 1432.320133528169890, 149.9823971726779916 ) ) ;
#55845=CARTESIAN_POINT ( 'NONE',  ( -27.66276471549999982, 1464.092292077029924, 269.4444540537980401 ) ) ;
#55847=DIRECTION ( 'NONE',  ( 3.828588921590000582E-16, 0.000000000000000000, 1.000000000000000000 ) ) ;
#55848=CARTESIAN_POINT ( 'NONE',  ( 35.28259859119749819, 1451.607675694110185, 135.1248536069400075 ) ) ;
#55849=CIRCLE ( 'NONE', #79101, 3.058258088409981923 ) ;
#55851=CARTESIAN_POINT ( 'NONE',  ( 0.2056231781062039798, 1452.457109619009998, 183.2046317473360091 ) ) ;
#55854=CARTESIAN_POINT ( 'NONE',  ( 2.994691737410922094, 1448.276535295347912, 183.8510770426177885 ) ) ;
#55857=CARTESIAN_POINT ( 'NONE',  ( -37.43441710386299803, 1420.282330175009974, 266.6710652364679959 ) ) ;
#55859=CARTESIAN_POINT ( 'NONE',  ( -3.529581353950369760, 1488.333655974519843, 181.7769974444219940 ) ) ;
#55860=ORIENTED_EDGE ( 'NONE', *, *, #109927, .F. ) ;
#55863=CARTESIAN_POINT ( 'NONE',  ( 38.13540227561171747, 1444.994950788472124, 136.8611909968648490 ) ) ;
#55866=CARTESIAN_POINT ( 'NONE',  ( -16.55052382899999941, 1440.438682495240073, 190.2157002606980143 ) ) ;
#55868=CARTESIAN_POINT ( 'NONE',  ( -2.430884947309378319, 1449.420338891706024, 183.0400647790289383 ) ) ;
#55870=CARTESIAN_POINT ( 'NONE',  ( -26.32958567590000243, 1435.437712720879972, 135.5714638756980150 ) ) ;
#55874=CARTESIAN_POINT ( 'NONE',  ( -35.21702932733460045, 1419.789484414370236, 270.0611807039360315 ) ) ;
#55875=CARTESIAN_POINT ( 'NONE',  ( 4.320487685200830263, 1417.954612720860041, 234.1150779680949938 ) ) ;
#55876=LINE ( 'NONE', #66908, #26844 ) ;
#55878=ORIENTED_EDGE ( 'NONE', *, *, #18520, .F. ) ;
#55879=VERTEX_POINT ( 'NONE', #88422 ) ;
#55880=CARTESIAN_POINT ( 'NONE',  ( 42.12435291735053511, 1454.070699221729001, 269.0724519205328988 ) ) ;
#55882=CARTESIAN_POINT ( 'NONE',  ( -13.32470456501929768, 1436.115206346340074, 150.5929143813179962 ) ) ;
#55883=CARTESIAN_POINT ( 'NONE',  ( -1.590905593539999829, 1484.788648626130225, 182.5874796677979930 ) ) ;
#55886=CARTESIAN_POINT ( 'NONE',  ( -20.58544668775375186, 1506.578946204038630, 217.1750514325470647 ) ) ;
#55887=CARTESIAN_POINT ( 'NONE',  ( -18.83008980160000334, 1435.775426850719896, 225.4210710169979848 ) ) ;
#55888=CARTESIAN_POINT ( 'NONE',  ( 15.68102603203800172, 1473.621980054030018, 269.4240265004769981 ) ) ;
#55889=CARTESIAN_POINT ( 'NONE',  ( 12.71684466930000035, 1416.535385209229844, 223.1239581433979993 ) ) ;
#55894=CARTESIAN_POINT ( 'NONE',  ( -36.37832870507119765, 1451.642701156129988, 135.0584859581319961 ) ) ;
#55897=CARTESIAN_POINT ( 'NONE',  ( 17.87794079919627066, 1458.605263598233250, 228.2755591390006202 ) ) ;
#55898=CARTESIAN_POINT ( 'NONE',  ( 24.97086024365579959, 1451.596742172109998, 137.2431907379429958 ) ) ;
#55899=CARTESIAN_POINT ( 'NONE',  ( -4.096381100208427384, 1440.262533769546963, 185.3780353409536588 ) ) ;
#55900=CARTESIAN_POINT ( 'NONE',  ( -0.5717982397045180409, 1450.893092752919983, 154.2461502927169761 ) ) ;
#55901=CARTESIAN_POINT ( 'NONE',  ( 22.12147071639999751, 1410.179604348530120, 204.7719268904379817 ) ) ;
#55905=CARTESIAN_POINT ( 'NONE',  ( 24.40381529368770330, 1445.062036062823609, 213.9252878650337379 ) ) ;
#55906=CARTESIAN_POINT ( 'NONE',  ( 2.500000000000000000, 1439.384186984200142, 161.5055418213960081 ) ) ;
#55908=ORIENTED_EDGE ( 'NONE', *, *, #69548, .F. ) ;
#55910=CARTESIAN_POINT ( 'NONE',  ( -44.93135410500000404, 1442.582777215279975, 269.6838066175980089 ) ) ;
#55912=CARTESIAN_POINT ( 'NONE',  ( 1.887381601534039764E-14, 1421.846727242609859, 101.6566346230980002 ) ) ;
#55913=CARTESIAN_POINT ( 'NONE',  ( -39.12047235985080107, 1447.561823957390061, 136.5584948024710172 ) ) ;
#55914=CARTESIAN_POINT ( 'NONE',  ( 10.86957190218895697, 1424.809467336535363, 138.2051722130555333 ) ) ;
#55915=CARTESIAN_POINT ( 'NONE',  ( 2.501965634382995241, 1417.708848509867494, 233.7485306405076813 ) ) ;
#55916=CARTESIAN_POINT ( 'NONE',  ( -2.500000000000000000, 1419.365678373030050, 145.1702656710979795 ) ) ;
#55918=CARTESIAN_POINT ( 'NONE',  ( -0.8946033002169070381, 1474.169686496259828, 270.1375980655809599 ) ) ;
#55919=CARTESIAN_POINT ( 'NONE',  ( 30.68660490123130202, 1440.913060384770006, 240.4674097414240066 ) ) ;
#55921=CARTESIAN_POINT ( 'NONE',  ( -4.363122647530000009, 1422.407399603929889, 168.7758374889979791 ) ) ;
#55924=CARTESIAN_POINT ( 'NONE',  ( -3.054816033052110136, 1485.996906143959905, 182.1538611115439892 ) ) ;
#55925=CARTESIAN_POINT ( 'NONE',  ( -1.356522590142140050, 1410.335674017130032, 185.6037846924129724 ) ) ;
#55926=CARTESIAN_POINT ( 'NONE',  ( 2.121808125839999892, 1499.002874645929978, 235.8090782458980073 ) ) ;
#55932=CARTESIAN_POINT ( 'NONE',  ( 22.83806540279999808, 1452.115537569730122, 139.3226699072980068 ) ) ;
#55934=CARTESIAN_POINT ( 'NONE',  ( 1.678290706950000155, 1466.627378388229999, 234.7758880048979790 ) ) ;
#55937=CARTESIAN_POINT ( 'NONE',  ( -1.148217067119999824, 1451.929923922529952, 183.5619105232980246 ) ) ;
#55941=ORIENTED_EDGE ( 'NONE', *, *, #81590, .F. ) ;
#55945=CARTESIAN_POINT ( 'NONE',  ( 34.75665256036710105, 1437.096089887269954, 136.5416360476299928 ) ) ;
#55948=CARTESIAN_POINT ( 'NONE',  ( -2.321631234430000301, 1421.242214399630257, 184.0178362275980248 ) ) ;
#55950=CARTESIAN_POINT ( 'NONE',  ( 6.155896025694070239, 1409.128029013429796, 195.4707178546539978 ) ) ;
#55951=CARTESIAN_POINT ( 'NONE',  ( 18.80338089039999971, 1425.953332570529938, 225.0197130250980138 ) ) ;
#55953=CARTESIAN_POINT ( 'NONE',  ( -17.63150429730000113, 1440.791932874859867, 190.8949773138979822 ) ) ;
#55954=CARTESIAN_POINT ( 'NONE',  ( 11.86529747189999817, 1432.285508799240006, 150.3971901177980044 ) ) ;
#55956=EDGE_LOOP ( 'NONE', ( #46114, #16529, #101272, #70109 ) ) ;
#55957=ORIENTED_EDGE ( 'NONE', *, *, #48546, .T. ) ;
#55959=CARTESIAN_POINT ( 'NONE',  ( -12.26355851482949966, 1416.702560754919887, 194.6703901714200242 ) ) ;
#55960=( BOUNDED_CURVE ( )  B_SPLINE_CURVE ( 3, ( #81746, #30246, #55483, #89608 ),
 .UNSPECIFIED., .F., .T. ) 
 B_SPLINE_CURVE_WITH_KNOTS ( ( 4, 4 ),
 ( 0.9859787944923890102, 2.095227079056804609 ),
 .UNSPECIFIED. ) 
 CURVE ( )  GEOMETRIC_REPRESENTATION_ITEM ( )  RATIONAL_B_SPLINE_CURVE ( ( 1.000000000000000000, 0.9000656239593909369, 0.9000656239593909369, 1.000000000000000000 ) ) 
 REPRESENTATION_ITEM ( '' )  );
#55961=CARTESIAN_POINT ( 'NONE',  ( -11.92218722690000021, 1434.273876409569993, 150.9668191998980262 ) ) ;
#55963=CARTESIAN_POINT ( 'NONE',  ( 11.86610049460949945, 1432.336025080309810, 149.9824239092829998 ) ) ;
#55968=CARTESIAN_POINT ( 'NONE',  ( -46.16774349130800204, 1440.697242589380039, 266.9714508753160089 ) ) ;
#55969=CARTESIAN_POINT ( 'NONE',  ( -20.59710966430000312, 1507.771223779230013, 191.2037110683980075 ) ) ;
#55972=CARTESIAN_POINT ( 'NONE',  ( 5.135462867024300770, 1408.035052394380045, 221.3338201871839885 ) ) ;
#55973=CARTESIAN_POINT ( 'NONE',  ( -13.03770669738669952, 1434.798218780290199, 149.1309000377920029 ) ) ;
#55975=CARTESIAN_POINT ( 'NONE',  ( 9.236167301360001858, 1423.625854809029988, 144.1549878472980026 ) ) ;
#55977=CARTESIAN_POINT ( 'NONE',  ( 5426.659240076989590, 2833.746317950241519, 8449.939303198118068 ) ) ;
#55978=ORIENTED_EDGE ( 'NONE', *, *, #17846, .T. ) ;
#55980=CARTESIAN_POINT ( 'NONE',  ( 36.52133868079999957, 1436.268774900949893, 254.5789811318979616 ) ) ;
#55982=CARTESIAN_POINT ( 'NONE',  ( -3.480938413559999667, 1458.418752667929994, 183.0457556368980079 ) ) ;
#55983=CARTESIAN_POINT ( 'NONE',  ( -17.22039985489999836, 1409.679124340329963, 195.0448976402979895 ) ) ;
#55984=CARTESIAN_POINT ( 'NONE',  ( 21.97938480441199971, 1506.433683733499947, 208.7396655020440051 ) ) ;
#55985=CARTESIAN_POINT ( 'NONE',  ( -7.523989352620000126, 1422.078425209429952, 216.2367226431979930 ) ) ;
#55988=CARTESIAN_POINT ( 'NONE',  ( -4.468407265335279988, 1452.757020167219935, 152.1700944353500233 ) ) ;
#55989=CARTESIAN_POINT ( 'NONE',  ( -18.89924256150000303, 1416.831925117730179, 207.5749492501780082 ) ) ;
#55991=CARTESIAN_POINT ( 'NONE',  ( -0.02816757767735129925, 1396.454736580349845, 196.6640986795260062 ) ) ;
#55993=CARTESIAN_POINT ( 'NONE',  ( 2.970284549810000119, 1509.150405704829836, 239.1320982052979787 ) ) ;
#55994=EDGE_LOOP ( 'NONE', ( #29442, #78298 ) ) ;
#55996=CARTESIAN_POINT ( 'NONE',  ( -10.62939606198754738, 1424.058470519482398, 137.5671174789835618 ) ) ;
#56001=CARTESIAN_POINT ( 'NONE',  ( -16.14907631359999840, 1479.767009654729918, 229.2046367109979883 ) ) ;
#56004=CARTESIAN_POINT ( 'NONE',  ( 11.43737779389999965, 1425.481201409729920, 144.1652972826979635 ) ) ;
#56005=CARTESIAN_POINT ( 'NONE',  ( -13.00574619272840060, 1416.230844595159851, 221.8287990380179906 ) ) ;
#56008=ORIENTED_EDGE ( 'NONE', *, *, #36332, .T. ) ;
#56010=CARTESIAN_POINT ( 'NONE',  ( 13.31869894295501311, 1443.265307952794501, 187.7487017255434125 ) ) ;
#56012=ORIENTED_EDGE ( 'NONE', *, *, #26837, .T. ) ;
#56016=CARTESIAN_POINT ( 'NONE',  ( -4.653281936863520762, 1425.827070423550140, 186.2156739099499987 ) ) ;
#56017=CARTESIAN_POINT ( 'NONE',  ( 23.64676265546030010, 1452.087297239420195, 137.4473122821260063 ) ) ;
#56018=CARTESIAN_POINT ( 'NONE',  ( 0.4742219137227159931, 1409.781081933909945, 270.0713786262579674 ) ) ;
#56021=CARTESIAN_POINT ( 'NONE',  ( -19.50212806963730472, 1509.609157136526619, 231.3489388162998637 ) ) ;
#56022=CARTESIAN_POINT ( 'NONE',  ( 0.02070843297204195618, 1409.009641154224255, 232.2968665989713202 ) ) ;
#56023=CARTESIAN_POINT ( 'NONE',  ( -13.26406613303420023, 1434.886401268850022, 148.9734610765700040 ) ) ;
#56026=CARTESIAN_POINT ( 'NONE',  ( -24.89153249345189778, 1509.523145840989855, 222.7250669980219868 ) ) ;
#56029=CARTESIAN_POINT ( 'NONE',  ( 18.57221589319999921, 1434.150321779219894, 219.6133833291980011 ) ) ;
#56030=CARTESIAN_POINT ( 'NONE',  ( -10.81518761075750135, 1424.921099531289883, 144.1705495212430037 ) ) ;
#56037=CARTESIAN_POINT ( 'NONE',  ( 1.300519565079999921E-15, 1440.444625599219989, 150.6821045058979962 ) ) ;
#56044=CARTESIAN_POINT ( 'NONE',  ( 14.23529166910000043, 1422.104100209229955, 228.4651581752980007 ) ) ;
#56048=CARTESIAN_POINT ( 'NONE',  ( -17.84388054299999737, 1409.536182426630148, 223.0592386858980092 ) ) ;
#56049=CARTESIAN_POINT ( 'NONE',  ( 1.549965084495990020, 1416.007771869960152, 190.4473925629179973 ) ) ;
#56050=CARTESIAN_POINT ( 'NONE',  ( 4.468129420396740770, 1440.960114341679855, 155.7399635850599680 ) ) ;
#56051=CARTESIAN_POINT ( 'NONE',  ( 29.35128621234889934, 1441.653456125289949, 137.2693277896180177 ) ) ;
#56052=CARTESIAN_POINT ( 'NONE',  ( 5.376511155560629973, 1429.663370564680235, 154.2340444031499942 ) ) ;
#56053=CARTESIAN_POINT ( 'NONE',  ( 12.26979143420000007, 1416.828042686930075, 223.5793547218980279 ) ) ;
#56055=CARTESIAN_POINT ( 'NONE',  ( -41.01355532634549661, 1442.086579808119950, 136.7422881729029882 ) ) ;
#56056=CARTESIAN_POINT ( 'NONE',  ( -1.241866690459999978, 1415.088275290230058, 226.9681039297979908 ) ) ;
#56058=CARTESIAN_POINT ( 'NONE',  ( -8.168076443215248617, 1407.240959200780026, 219.8347814960359869 ) ) ;
#56061=CARTESIAN_POINT ( 'NONE',  ( -29.22959469711409852, 1509.933780326070064, 211.7723416727030212 ) ) ;
#56062=CARTESIAN_POINT ( 'NONE',  ( 13.80530362780000075, 1434.979595110789887, 149.0261668940979973 ) ) ;
#56063=CARTESIAN_POINT ( 'NONE',  ( -27.25232428270000185, 1436.344188865190063, 136.7193557181979884 ) ) ;
#56064=CARTESIAN_POINT ( 'NONE',  ( 7.185297835940000155, 1440.193071586459837, 185.7613749676980035 ) ) ;
#56068=CARTESIAN_POINT ( 'NONE',  ( -0.6034434167798160553, 1408.934133095820016, 224.1097741871060123 ) ) ;
#56071=CARTESIAN_POINT ( 'NONE',  ( -13.14670073217260082, 1428.477643202489844, 195.1720996079020267 ) ) ;
#56072=CARTESIAN_POINT ( 'NONE',  ( 31.99315161004722441, 1416.540825925197851, 269.3158597989070131 ) ) ;
#56080=CARTESIAN_POINT ( 'NONE',  ( -27.28811781800000347, 1451.810925661529836, 135.7818030516980059 ) ) ;
#56081=B_SPLINE_CURVE_WITH_KNOTS ( 'NONE', 3,
 ( #33762, #75248, #25352, #84170 ),
 .UNSPECIFIED., .F., .F.,
 ( 4, 4 ),
 ( 0.000000000000000000, 1.000000000000000000 ),
 .UNSPECIFIED. ) ;
#56083=CARTESIAN_POINT ( 'NONE',  ( -16.76087985708559813, 1410.448050361750120, 226.3463234497499741 ) ) ;
#56084=CARTESIAN_POINT ( 'NONE',  ( 0.5042866867199140568, 1413.080632846199933, 184.9534695539459790 ) ) ;
#56085=ORIENTED_EDGE ( 'NONE', *, *, #8408, .T. ) ;
#56088=CARTESIAN_POINT ( 'NONE',  ( 24.84138244430000242, 1449.855123928979992, 207.3631881002280295 ) ) ;
#56090=CARTESIAN_POINT ( 'NONE',  ( -0.3072900061734130106, 1418.957554290649796, 184.6599555451460049 ) ) ;
#56091=LINE ( 'NONE', #105954, #19291 ) ;
#56092=CARTESIAN_POINT ( 'NONE',  ( 22.43553758490000050, 1409.860968200830030, 213.4417271402680285 ) ) ;
#56095=CARTESIAN_POINT ( 'NONE',  ( -17.58819996659999774, 1424.269664099130068, 227.8357312002980279 ) ) ;
#56096=CARTESIAN_POINT ( 'NONE',  ( -11.30116487869999986, 1432.303974762190137, 151.5220930523979916 ) ) ;
#56097=CARTESIAN_POINT ( 'NONE',  ( 27.47789372709499744, 1488.737009538180018, 209.0498192191509759 ) ) ;
#56099=CARTESIAN_POINT ( 'NONE',  ( 25.48623307864125920, 1509.803059086864550, 194.5187256612674673 ) ) ;
#56100=CARTESIAN_POINT ( 'NONE',  ( 14.13195592840999915, 1452.421092199690065, 222.7290593210850034 ) ) ;
#56103=CARTESIAN_POINT ( 'NONE',  ( -17.97825106899999881, 1424.673537191730020, 227.3634650722979984 ) ) ;
#56105=CARTESIAN_POINT ( 'NONE',  ( -4.260246875749409412, 1441.234673244090118, 159.4002643389130185 ) ) ;
#56108=EDGE_LOOP ( 'NONE', ( #781, #54303, #33672, #24400 ) ) ;
#56113=CARTESIAN_POINT ( 'NONE',  ( -11.44042036928753170, 1425.479427483456220, 144.3717380689928689 ) ) ;
#56114=CARTESIAN_POINT ( 'NONE',  ( 15.70031134094579706, 1410.429114820810128, 191.5836651352509818 ) ) ;
#56116=CARTESIAN_POINT ( 'NONE',  ( -25.25892285357279832, 1450.980737957350129, 137.4961021865089776 ) ) ;
#56118=CARTESIAN_POINT ( 'NONE',  ( 11.20515980299999903, 1409.304353190929987, 228.2703101120980023 ) ) ;
#56120=CARTESIAN_POINT ( 'NONE',  ( 41.62352936865920583, 1444.515901152170045, 134.0999999983539794 ) ) ;
#56121=LINE ( 'NONE', #57249, #59726 ) ;
#56123=CARTESIAN_POINT ( 'NONE',  ( -8.301987938657498844, 1512.913060387330006, 186.6498241004079262 ) ) ;
#56125=ORIENTED_EDGE ( 'NONE', *, *, #20912, .F. ) ;
#56127=CARTESIAN_POINT ( 'NONE',  ( 13.23760251530267595, 1410.748325464791151, 228.4239685329596057 ) ) ;
#56128=CARTESIAN_POINT ( 'NONE',  ( 34.35673732775180156, 1445.503283704120122, 137.0830489816779902 ) ) ;
#56130=CARTESIAN_POINT ( 'NONE',  ( -3.066838699319999861, 1484.261994786129890, 183.3371859551980094 ) ) ;
#56132=CARTESIAN_POINT ( 'NONE',  ( -28.19408351100000232, 1508.123162623830012, 208.4952225986349958 ) ) ;
#56136=CARTESIAN_POINT ( 'NONE',  ( 3.949232805999999929, 1416.520322350429979, 190.9327904293980112 ) ) ;
#56142=CARTESIAN_POINT ( 'NONE',  ( 35.39978664942150033, 1440.913060387330006, 261.4306008630139786 ) ) ;
#56143=CARTESIAN_POINT ( 'NONE',  ( -0.0007575016918736815529, 1451.923243585050386, 153.9989249036371177 ) ) ;
#56144=EDGE_LOOP ( 'NONE', ( #58235, #72573, #73244, #40184 ) ) ;
#56145=CARTESIAN_POINT ( 'NONE',  ( -0.3637087824265209934, 1450.900359396770000, 181.9077912123260035 ) ) ;
#56146=CARTESIAN_POINT ( 'NONE',  ( -15.57473716419999832, 1409.623569226230074, 191.7218289598980050 ) ) ;
#56152=CARTESIAN_POINT ( 'NONE',  ( 6.178286635010000083, 1406.300107697530166, 266.9460459613980561 ) ) ;
#56153=CARTESIAN_POINT ( 'NONE',  ( -13.19913408319999881, 1434.900406177449895, 146.4345302607979988 ) ) ;
#56156=CARTESIAN_POINT ( 'NONE',  ( 17.04804198250000269, 1458.590950340129893, 229.8098020277979856 ) ) ;
#56157=CARTESIAN_POINT ( 'NONE',  ( -11.60004869885203682, 1422.941213647143968, 135.6422426697142782 ) ) ;
#56160=CARTESIAN_POINT ( 'NONE',  ( -0.1562604339309009993, 1507.298388591709909, 180.8861905666690006 ) ) ;
#56161=CARTESIAN_POINT ( 'NONE',  ( 16.95285180472732378, 1449.028869222066305, 218.6259880166646496 ) ) ;
#56163=CARTESIAN_POINT ( 'NONE',  ( 18.62830136119999835, 1508.852446408229753, 188.2546778553979721 ) ) ;
#56166=EDGE_LOOP ( 'NONE', ( #73916, #35845, #91528 ) ) ;
#56168=CARTESIAN_POINT ( 'NONE',  ( 16.14278285189999806, 1456.434606976529949, 217.4272506521679702 ) ) ;
#56169=CARTESIAN_POINT ( 'NONE',  ( -11.57591907649999996, 1432.294438222789950, 151.1967649998980221 ) ) ;
#56172=CARTESIAN_POINT ( 'NONE',  ( 2.425235212390000061, 1410.367075232029947, 231.7449734550979770 ) ) ;
#56174=CARTESIAN_POINT ( 'NONE',  ( 12.08639211120000034, 1446.204391809530080, 187.8374895246980145 ) ) ;
#56175=CARTESIAN_POINT ( 'NONE',  ( -20.58378676590000111, 1457.443618353330066, 224.2614987732980012 ) ) ;
#56176=CARTESIAN_POINT ( 'NONE',  ( 19.46473663940000165, 1455.600668601630105, 226.0207017425979927 ) ) ;
#56177=CARTESIAN_POINT ( 'NONE',  ( -2.153510090440000191, 1485.578724168830149, 182.5440842283980203 ) ) ;
#56181=CARTESIAN_POINT ( 'NONE',  ( 6.178286635010000083, 1406.300107697530166, 266.9460459613980561 ) ) ;
#56185=CARTESIAN_POINT ( 'NONE',  ( 23.66594833135497566, 1434.290763647069980, 214.6250708475496936 ) ) ;
#56189=EDGE_CURVE ( 'NONE', #96843, #35341, #49739, .T. ) ;
#56191=CARTESIAN_POINT ( 'NONE',  ( -0.8767898181709999905, 1450.882442212199976, 155.6080925170979867 ) ) ;
#56192=CARTESIAN_POINT ( 'NONE',  ( -1.673374938852186133, 1450.582197054855669, 183.1029605669776288 ) ) ;
#56193=ADVANCED_FACE ( 'NONE', ( #70547 ), #82770, .F. ) ;
#56194=CARTESIAN_POINT ( 'NONE',  ( 2.500000002650000219, 1449.201558846790022, 155.6080914321979947 ) ) ;
#56196=CARTESIAN_POINT ( 'NONE',  ( -13.46591419205600104, 1415.020374539180011, 220.3865122175670024 ) ) ;
#56197=CARTESIAN_POINT ( 'NONE',  ( 11.99447453070000158, 1410.787978747230227, 219.9627944869979785 ) ) ;
#56198=CARTESIAN_POINT ( 'NONE',  ( -23.03655027839999647, 1423.631548418229841, 255.3819207742980097 ) ) ;
#56199=B_SPLINE_CURVE_WITH_KNOTS ( 'NONE', 5,
 ( #41957, #92899, #15613, #85589, #76111, #528, #8885, #17265, #50913, #94001, #102938, #49820 ),
 .UNSPECIFIED., .F., .F.,
 ( 6, 3, 3, 6 ),
 ( 0.000000000000000000, 0.2862565181357951682, 0.7620907940255700064, 1.000000000000000000 ),
 .UNSPECIFIED. ) ;
#56200=B_SPLINE_CURVE_WITH_KNOTS ( 'NONE', 3,
 ( #70395, #104513, #11011, #94434, #12660, #29449, #72055, #64188, #56325, #63646, #71513, #46839, #3190, #80425, #39519, #55794, #65288, #105632, #98310, #55236, #99401, #38403, #80968, #89369, #72579, #29997, #4273, #79876, #38944, #3737, #46297, #37318, #106170, #21588, #54141, #106707, #13735, #28919, #89909, #13183, #47372, #81497, #4799 ),
 .UNSPECIFIED., .F., .F.,
 ( 4, 3, 3, 3, 3, 3, 3, 3, 3, 3, 3, 3, 3, 3, 4 ),
 ( -1.999999996503429855, -1.941402971639760056, -1.796657287308599971, -1.649920620429889961, -1.501917604718239874, -1.352028961624889947, -1.201168230678989923, -1.049651953167649809, -0.8978420048550590504, -0.7403908631910058880, -0.5896658738122080301, -0.4400322845055311127, -0.2917605857772640476, -0.1450427803553220318, 0.000000000000000000 ),
 .UNSPECIFIED. ) ;
#56201=CARTESIAN_POINT ( 'NONE',  ( -27.33473054107770039, 1507.985401980800134, 210.9306764114709836 ) ) ;
#56202=CARTESIAN_POINT ( 'NONE',  ( 2.500000000000000000, 1439.245504089100223, 159.3587695534980071 ) ) ;
#56203=CARTESIAN_POINT ( 'NONE',  ( -2.776816374990000114, 1476.015124969530007, 267.5339340712980061 ) ) ;
#56204=CARTESIAN_POINT ( 'NONE',  ( -11.44378745049835544, 1425.812029265508500, 138.6329405890633666 ) ) ;
#56211=B_SPLINE_SURFACE_WITH_KNOTS ( 'NONE', 4, 5, ( 
 ( #89404, #11597, #46873, #71550, #19983, #38435 ),
 ( #47409, #53626, #19424, #106742, #54177, #30029 ),
 ( #54726, #64223, #107302, #88305, #105671, #89944 ),
 ( #30595, #64783, #14880, #107849, #5394, #41748 ),
 ( #49071, #74818, #31138, #57478, #56361, #66974 ) ),
 .UNSPECIFIED., .F., .F., .F.,
 ( 5, 5 ),
 ( 6, 6 ),
 ( 0.000000000000000000, 1.224053340420000024 ),
 ( 0.000000000000000000, 2.000000000000000000 ),
 .UNSPECIFIED. ) ;
#56214=CARTESIAN_POINT ( 'NONE',  ( 0.2253789646234576893, 1420.493552874686429, 182.7575710290123823 ) ) ;
#56215=CARTESIAN_POINT ( 'NONE',  ( -1.793404623366990247, 1395.975687456799960, 219.9892326746640094 ) ) ;
#56216=ADVANCED_FACE ( 'NONE', ( #12805 ), #48642, .F. ) ;
#56218=CARTESIAN_POINT ( 'NONE',  ( 19.57339925981531792, 1455.491367452954591, 225.8543147067736641 ) ) ;
#56220=CARTESIAN_POINT ( 'NONE',  ( -5.074604691638342047, 1410.465630996212440, 231.8427962307575001 ) ) ;
#56224=CARTESIAN_POINT ( 'NONE',  ( 11.67304687340000058, 1426.321999969329909, 139.6389216567980043 ) ) ;
#56232=CARTESIAN_POINT ( 'NONE',  ( 6.820844401089999565, 1507.852259759629987, 182.4337134681979933 ) ) ;
#56235=EDGE_CURVE ( 'NONE', #76242, #94251, #46018, .T. ) ;
#56238=ORIENTED_EDGE ( 'NONE', *, *, #102675, .T. ) ;
#56240=CARTESIAN_POINT ( 'NONE',  ( -11.64940060459999849, 1396.319866421030156, 207.5851092805380063 ) ) ;
#56241=CARTESIAN_POINT ( 'NONE',  ( -20.51953016590000090, 1409.793898084230023, 218.1559997793979733 ) ) ;
#56243=CARTESIAN_POINT ( 'NONE',  ( -13.05984560479545209, 1444.833622568467035, 169.4122135708499286 ) ) ;
#56244=CARTESIAN_POINT ( 'NONE',  ( 21.29766439678459733, 1509.704854597507619, 229.9147211563969506 ) ) ;
#56247=CARTESIAN_POINT ( 'NONE',  ( 17.00560939319999676, 1410.862827255230059, 226.2920145422980340 ) ) ;
#56248=CARTESIAN_POINT ( 'NONE',  ( 8.785620242860000317, 1429.761447237529865, 187.0031388449980057 ) ) ;
#56249=CARTESIAN_POINT ( 'NONE',  ( -7.388976461649999550, 1415.087797054229895, 193.5183541347980167 ) ) ;
#56250=CARTESIAN_POINT ( 'NONE',  ( -41.63068410086079751, 1444.585398277480181, 136.0329946082410117 ) ) ;
#56252=CARTESIAN_POINT ( 'NONE',  ( 10.35233951385729867, 1396.274572049960170, 213.0386826886810070 ) ) ;
#56253=DIRECTION ( 'NONE',  ( 0.9995237709234254808, 0.03085824620771311644, 1.984178880230842443E-13 ) ) ;
#56254=CARTESIAN_POINT ( 'NONE',  ( 11.82873555240000130, 1429.816408930329999, 149.3973828046979975 ) ) ;
#56255=CARTESIAN_POINT ( 'NONE',  ( 8.991744574390811096, 1509.227061438039982, 181.2342617849590169 ) ) ;
#56257=CARTESIAN_POINT ( 'NONE',  ( 4.156129378920000228, 1425.920013205530040, 185.3798846555979765 ) ) ;
#56260=ORIENTED_EDGE ( 'NONE', *, *, #31669, .T. ) ;
#56266=CARTESIAN_POINT ( 'NONE',  ( -3.054816033052110136, 1485.996906143959905, 182.1538611115439892 ) ) ;
#56269=CARTESIAN_POINT ( 'NONE',  ( 2.500000000000000000, 1448.594374933610197, 159.2313818852420013 ) ) ;
#56271=( BOUNDED_CURVE ( )  B_SPLINE_CURVE ( 3, ( #13705, #47892, #12636, #4242 ),
 .UNSPECIFIED., .F., .F. ) 
 B_SPLINE_CURVE_WITH_KNOTS ( ( 4, 4 ),
 ( 5.474490172796000031, 5.884916938985190527 ),
 .UNSPECIFIED. ) 
 CURVE ( )  GEOMETRIC_REPRESENTATION_ITEM ( )  RATIONAL_B_SPLINE_CURVE ( ( 1.000000000000000000, 0.9860116829598833954, 0.9860116829598833954, 1.000000000000000000 ) ) 
 REPRESENTATION_ITEM ( '' )  );
#56272=CARTESIAN_POINT ( 'NONE',  ( 0.2707600216770000290, 1415.088016306429836, 226.0844321790980018 ) ) ;
#56276=CARTESIAN_POINT ( 'NONE',  ( -20.81411743600000008, 1509.690291818130163, 230.4138254417979681 ) ) ;
#56277=CARTESIAN_POINT ( 'NONE',  ( -38.90820051305949079, 1429.376674070663967, 269.5913902092726744 ) ) ;
#56279=CARTESIAN_POINT ( 'NONE',  ( -45.97229537702650504, 1578.884344667429787, 229.9350315244390117 ) ) ;
#56280=ORIENTED_EDGE ( 'NONE', *, *, #49510, .T. ) ;
#56281=CARTESIAN_POINT ( 'NONE',  ( 2.500000000000000000, 1432.232933817210096, 157.4922851969979831 ) ) ;
#56282=CARTESIAN_POINT ( 'NONE',  ( -30.14115132559009780, 1440.913060386970074, 238.7996103749989913 ) ) ;
#56285=CARTESIAN_POINT ( 'NONE',  ( -0.06137319429855010722, 1466.040928358300107, 235.8553063735670037 ) ) ;
#56287=CARTESIAN_POINT ( 'NONE',  ( 20.06106135328079887, 1413.496800473840267, 269.8982105628270460 ) ) ;
#56292=CARTESIAN_POINT ( 'NONE',  ( 22.92012589049999960, 1409.721659010730036, 209.2345283292779925 ) ) ;
#56293=CARTESIAN_POINT ( 'NONE',  ( -20.99310762600000047, 1509.712614273529880, 187.9175820947980071 ) ) ;
#56295=CARTESIAN_POINT ( 'NONE',  ( -11.60004869885203505, 1425.798876189259772, 137.3569514552391695 ) ) ;
#56297=CARTESIAN_POINT ( 'NONE',  ( 4.235082444282669556, 1421.836746427100024, 184.3796511902140196 ) ) ;
#56298=CARTESIAN_POINT ( 'NONE',  ( 0.4649457434059999783, 1418.687271102530076, 184.7086881091979933 ) ) ;
#56299=CARTESIAN_POINT ( 'NONE',  ( 6.736113117885867752, 1420.681901958687149, 137.0999999980981841 ) ) ;
#56303=ADVANCED_FACE ( 'NONE', ( #107965 ), #51372, .T. ) ;
#56305=CARTESIAN_POINT ( 'NONE',  ( 0.5533832822140000163, 1417.008313040729945, 234.1272609293980054 ) ) ;
#56307=CARTESIAN_POINT ( 'NONE',  ( -24.90665996499999935, 1442.497388197319879, 210.4939798944579934 ) ) ;
#56309=PLANE ( 'NONE',  #89802 ) ;
#56312=DIRECTION ( 'NONE',  ( -0.9993902469235412811, -0.03489947644508390595, 0.001077449749359510062 ) ) ;
#56314=ORIENTED_EDGE ( 'NONE', *, *, #51655, .T. ) ;
#56319=B_SPLINE_CURVE_WITH_KNOTS ( 'NONE', 3,
 ( #38054, #71137, #3373, #81145, #20137, #53790, #72231, #47020, #29641, #61621, #53220 ),
 .UNSPECIFIED., .F., .F.,
 ( 4, 2, 1, 2, 2, 4 ),
 ( 0.000000000000000000, 0.2500000000000126565, 0.3750000000000736078, 0.4375000000000877076, 0.5000000000001018075, 1.000000000000000000 ),
 .UNSPECIFIED. ) ;
#56320=EDGE_CURVE ( 'NONE', #79053, #28929, #25945, .T. ) ;
#56321=CARTESIAN_POINT ( 'NONE',  ( 23.85401727289999840, 1447.123143008870102, 216.1985342456480055 ) ) ;
#56322=CARTESIAN_POINT ( 'NONE',  ( 8.292451526740862278, 1437.777547255205945, 153.5278875412344632 ) ) ;
#56325=CARTESIAN_POINT ( 'NONE',  ( -26.41719155878330128, 1508.429547602710045, 201.5167586753940157 ) ) ;
#56326=CARTESIAN_POINT ( 'NONE',  ( -3.117854675340000270, 1446.609948778509988, 165.9235426434980241 ) ) ;
#56327=CARTESIAN_POINT ( 'NONE',  ( -19.80431309490000302, 1426.801393628430105, 224.9940485357979867 ) ) ;
#56329=CARTESIAN_POINT ( 'NONE',  ( -24.39385583620000020, 1435.492268184149907, 137.6392094220979914 ) ) ;
#56331=CARTESIAN_POINT ( 'NONE',  ( 17.25705130249999897, 1509.016679772330008, 187.6328010954979959 ) ) ;
#56332=CARTESIAN_POINT ( 'NONE',  ( 0.2723178306860529752, 1409.428891657669737, 233.0102446141029873 ) ) ;
#56333=CARTESIAN_POINT ( 'NONE',  ( -18.83575481127647677, 1438.179160179573500, 211.0549776618481701 ) ) ;
#56335=CARTESIAN_POINT ( 'NONE',  ( -30.25377815386013935, 1462.061561754708464, 269.4735075012114294 ) ) ;
#56339=CARTESIAN_POINT ( 'NONE',  ( -10.76706410755489429, 1424.951753425542847, 141.1458295590867067 ) ) ;
#56342=CARTESIAN_POINT ( 'NONE',  ( -8.407921469289998839, 1475.513060387329915, 228.4380765505979980 ) ) ;
#56343=CARTESIAN_POINT ( 'NONE',  ( 1.460159494251919821, 1495.777843760759879, 181.6077353377199870 ) ) ;
#56344=CARTESIAN_POINT ( 'NONE',  ( -0.1157304452309999981, 1415.757619356030091, 233.4560891803980098 ) ) ;
#56345=CARTESIAN_POINT ( 'NONE',  ( -13.47420130509332914, 1443.596551666932100, 187.1131726174379821 ) ) ;
#56347=CARTESIAN_POINT ( 'NONE',  ( -17.09817538394500147, 1414.913526854310021, 207.6506234252330216 ) ) ;
#56350=CARTESIAN_POINT ( 'NONE',  ( -13.86092847646930082, 1410.765486861110048, 227.1170286572800023 ) ) ;
#56352=CARTESIAN_POINT ( 'NONE',  ( 23.87593678670000230, 1435.337375081109940, 137.1350274835979803 ) ) ;
#56358=VERTEX_POINT ( 'NONE', #93912 ) ;
#56361=CARTESIAN_POINT ( 'NONE',  ( 12.70314174409999985, 1508.075973130829880, 233.3727141454980085 ) ) ;
#56362=CARTESIAN_POINT ( 'NONE',  ( 20.75139895264628009, 1414.320554380318072, 269.3935123240341341 ) ) ;
#56363=CARTESIAN_POINT ( 'NONE',  ( -30.28727319840000121, 1444.847842080029977, 240.1330978262979841 ) ) ;
#56364=CARTESIAN_POINT ( 'NONE',  ( -20.51588922700000239, 1505.140427506229798, 190.4683942995980033 ) ) ;
#56366=CARTESIAN_POINT ( 'NONE',  ( -11.87470928319999963, 1433.125601036669877, 150.1735720417980247 ) ) ;
#56368=CARTESIAN_POINT ( 'NONE',  ( 11.69192323821640045, 1426.725590720729997, 140.9428211002000069 ) ) ;
#56373=CARTESIAN_POINT ( 'NONE',  ( 5.630091722370000440, 1441.487383641189808, 154.7801822668979810 ) ) ;
#56376=CARTESIAN_POINT ( 'NONE',  ( -10.68607904894687444, 1509.411632735550029, 237.1549078682182312 ) ) ;
#56377=CARTESIAN_POINT ( 'NONE',  ( -1.599724557440349957E-10, 1412.168762487870026, 253.0958361106100369 ) ) ;
#56383=CARTESIAN_POINT ( 'NONE',  ( -28.35914775050000003, 1465.186344805629915, 270.3509322670980168 ) ) ;
#56386=CARTESIAN_POINT ( 'NONE',  ( 33.91363303768119408, 1450.440614253119975, 136.2454530761589808 ) ) ;
#56387=CARTESIAN_POINT ( 'NONE',  ( 0.2058156135791029961, 1452.245535141509890, 183.1437243635440097 ) ) ;
#56388=DIRECTION ( 'NONE',  ( -0.9417419115949053898, -0.3363363969979660806, 0.000000000000000000 ) ) ;
#56392=CARTESIAN_POINT ( 'NONE',  ( -42.13315488374279738, 1426.265673821560085, 268.3403209545570007 ) ) ;
#56394=CARTESIAN_POINT ( 'NONE',  ( -20.99310762600000047, 1509.712614273529880, 187.9175820947980071 ) ) ;
#56398=PLANE ( 'NONE',  #51963 ) ;
#56399=B_SPLINE_CURVE_WITH_KNOTS ( 'NONE', 3,
 ( #11314, #37046, #96971, #20235, #54436, #11853, #86345, #35396, #46026, #80154 ),
 .UNSPECIFIED., .F., .F.,
 ( 4, 2, 2, 2, 4 ),
 ( 0.000000000000000000, 0.2500000000000000000, 0.5000000000000000000, 0.7500000000000000000, 1.000000000000000000 ),
 .UNSPECIFIED. ) ;
#56402=CARTESIAN_POINT ( 'NONE',  ( -12.73123357059999883, 1455.447220867429905, 187.4137537217980025 ) ) ;
#56403=CARTESIAN_POINT ( 'NONE',  ( -2.399591520910798970, 1449.521109860346769, 183.0206712615461413 ) ) ;
#56404=VERTEX_POINT ( 'NONE', #43538 ) ;
#56405=CARTESIAN_POINT ( 'NONE',  ( -26.65016812680000058, 1436.423441677409983, 136.7215463643979945 ) ) ;
#56406=CIRCLE ( 'NONE', #108260, 12.50000000000001066 ) ;
#56407=B_SPLINE_CURVE_WITH_KNOTS ( 'NONE', 3,
 ( #84132, #8521, #66275, #57859, #94184, #41598, #42698 ),
 .UNSPECIFIED., .F., .F.,
 ( 4, 3, 4 ),
 ( -157.7301682620000065, -100.4765462162850014, -30.40177460649999830 ),
 .UNSPECIFIED. ) ;
#56409=CARTESIAN_POINT ( 'NONE',  ( 1.546943247107299912, 1416.828039266790029, 190.2227890105679933 ) ) ;
#56415=CARTESIAN_POINT ( 'NONE',  ( -1.248605592450000135, 1397.026870444829910, 196.3012639762980029 ) ) ;
#56417=EDGE_LOOP ( 'NONE', ( #48497, #34235, #18749, #40058 ) ) ;
#56419=CARTESIAN_POINT ( 'NONE',  ( 3.756948166784984444, 1425.519882450703790, 185.1998084200467360 ) ) ;
#56421=EDGE_CURVE ( 'NONE', #80510, #15749, #32904, .T. ) ;
#56422=CARTESIAN_POINT ( 'NONE',  ( -14.15891404902520101, 1436.253324085039822, 150.1419714444780027 ) ) ;
#56423=CARTESIAN_POINT ( 'NONE',  ( -0.03301841822632249623, 1409.280491802830056, 185.5015438497439959 ) ) ;
#56426=CARTESIAN_POINT ( 'NONE',  ( 2.877999451269170006, 1440.267615723689914, 157.3979800045339914 ) ) ;
#56428=CARTESIAN_POINT ( 'NONE',  ( -0.3530891408735000181, 1467.116854267079816, 235.6078141451939985 ) ) ;
#56432=CARTESIAN_POINT ( 'NONE',  ( -40.71747596219490362, 1448.637563214449983, 135.0584856682299915 ) ) ;
#56435=CARTESIAN_POINT ( 'NONE',  ( 6.284459336901857540, 1456.900407391064164, 227.9284455267091971 ) ) ;
#56437=CARTESIAN_POINT ( 'NONE',  ( 24.04111616115019956, 1452.073549554080046, 136.7274035651190047 ) ) ;
#56438=CARTESIAN_POINT ( 'NONE',  ( -4.120589916571496758, 1440.000613734177932, 185.4544762516224807 ) ) ;
#56439=CARTESIAN_POINT ( 'NONE',  ( 2.439001525050000119, 1430.488531030629929, 150.2249694046979869 ) ) ;
#56440=CARTESIAN_POINT ( 'NONE',  ( 22.00429000609999974, 1410.601272653630076, 203.2767770488879933 ) ) ;
#56441=CARTESIAN_POINT ( 'NONE',  ( -25.47400523009999773, 1435.387084339240118, 135.4904355849980107 ) ) ;
#56444=CARTESIAN_POINT ( 'NONE',  ( 4.264584969141440141, 1441.193324268380138, 158.8347230198679938 ) ) ;
#56454=CARTESIAN_POINT ( 'NONE',  ( 10.88555504727585799, 1424.831830838460974, 138.2234079619712190 ) ) ;
#56456=CARTESIAN_POINT ( 'NONE',  ( 17.86566981212778416, 1423.742594241267398, 225.9114519548369913 ) ) ;
#56461=CARTESIAN_POINT ( 'NONE',  ( 28.04879799853789990, 1440.913060387349788, 231.3508241056970292 ) ) ;
#56464=VERTEX_POINT ( 'NONE', #110726 ) ;
#56469=CARTESIAN_POINT ( 'NONE',  ( -19.06723915664710134, 1485.490521620860136, 189.6150037022410118 ) ) ;
#56471=DIRECTION ( 'NONE',  ( -0.03489949669041918917, 0.9993908270195176469, 2.562551298407829116E-09 ) ) ;
#56475=DIRECTION ( 'NONE',  ( -1.956929670128506950E-14, 1.000000000000000000, 0.000000000000000000 ) ) ;
#56479=CARTESIAN_POINT ( 'NONE',  ( 2.499945018050090173, 1419.382888684849831, 144.1035832394360057 ) ) ;
#56481=CARTESIAN_POINT ( 'NONE',  ( 1.522424741549999849, 1465.680318652129927, 235.2040100185980123 ) ) ;
#56482=CARTESIAN_POINT ( 'NONE',  ( -6.958472253045926870, 1439.213523565861578, 154.2072493331847056 ) ) ;
#56484=CARTESIAN_POINT ( 'NONE',  ( -0.5568085941520000137, 1452.298961472929932, 183.2685725910980068 ) ) ;
#56492=B_SPLINE_CURVE_WITH_KNOTS ( 'NONE', 3,
 ( #11411, #10281, #36596, #103803, #45579, #10855, #52865, #79721, #37151, #71347 ),
 .UNSPECIFIED., .F., .F.,
 ( 4, 2, 2, 2, 4 ),
 ( 4.187893579585400145E-10, 0.05103584884158749585, 0.1118202684977770006, 0.1535261566792579802, 0.2248365559521849910 ),
 .UNSPECIFIED. ) ;
#56495=CARTESIAN_POINT ( 'NONE',  ( -1.368191914778909890, 1419.344528075180278, 185.2221190139939893 ) ) ;
#56496=CARTESIAN_POINT ( 'NONE',  ( -11.60004869885204037, 1426.320647100494170, 137.6121510302394029 ) ) ;
#56500=CARTESIAN_POINT ( 'NONE',  ( 0.9835760575869921807, 1408.947407620089962, 194.1588551325519916 ) ) ;
#56501=CARTESIAN_POINT ( 'NONE',  ( 18.02091189525600257, 1424.326076159014065, 225.2020075002020008 ) ) ;
#56502=CARTESIAN_POINT ( 'NONE',  ( 0.4863421998530879642, 1418.702335047680208, 184.7127968358159933 ) ) ;
#56503=EDGE_CURVE ( 'NONE', #94490, #73277, #5314, .T. ) ;
#56504=CARTESIAN_POINT ( 'NONE',  ( -19.68379069659999914, 1478.188077225129973, 191.4618426609980020 ) ) ;
#56506=B_SPLINE_CURVE_WITH_KNOTS ( 'NONE', 3,
 ( #72233, #37502, #98499, #2283, #105259, #88997, #20674, #53222, #97942, #55419, #44826, #89553, #104703, #21210, #106357, #105826, #27998, #87929, #29643, #62183, #96870, #54333, #80054, #29104, #96309, #12842, #12285 ),
 .UNSPECIFIED., .F., .F.,
 ( 4, 2, 2, 1, 2, 2, 2, 2, 2, 2, 1, 1, 2, 2, 4 ),
 ( 0.000000000000000000, 0.06250000000007284451, 0.09375000000011163293, 0.1093750000001466327, 0.1171875000001659506, 0.1250000000001852685, 0.1875000000003016198, 0.2187500000003661516, 0.2500000000004307110, 0.3750000000006306067, 0.4375000000007188694, 0.4687500000007518430, 0.4843750000007574497, 0.5000000000007630563, 1.000000000000000000 ),
 .UNSPECIFIED. ) ;
#56507=CARTESIAN_POINT ( 'NONE',  ( -3.697944654365331818, 1424.333247977674091, 185.3305522059991972 ) ) ;
#56510=ADVANCED_FACE ( 'NONE', ( #2661 ), #69863, .F. ) ;
#56512=CARTESIAN_POINT ( 'NONE',  ( 18.18178698398020288, 1457.548798095479924, 228.6382434660380056 ) ) ;
#56513=CARTESIAN_POINT ( 'NONE',  ( -11.56247775979999837, 1434.196947835160017, 151.3456684532980034 ) ) ;
#56520=CARTESIAN_POINT ( 'NONE',  ( -45.66496797010459829, 1440.259989335280125, 266.1886939491620296 ) ) ;
#56525=CARTESIAN_POINT ( 'NONE',  ( -13.45595297782609912, 1435.788356003630042, 150.3939031303400213 ) ) ;
#56530=VERTEX_POINT ( 'NONE', #54168 ) ;
#56531=CARTESIAN_POINT ( 'NONE',  ( 9.545816653330000179, 1416.905270224830019, 240.4008508550979855 ) ) ;
#56532=CARTESIAN_POINT ( 'NONE',  ( -28.02912970359999889, 1508.133041382029887, 207.5417885384179897 ) ) ;
#56534=CARTESIAN_POINT ( 'NONE',  ( 26.80143075489152693, 1509.848986972751618, 220.9835789632684850 ) ) ;
#56535=CARTESIAN_POINT ( 'NONE',  ( -0.6192716172230079419, 1407.650954247345226, 270.1377424647723728 ) ) ;
#56536=CARTESIAN_POINT ( 'NONE',  ( -29.87496801699999693, 1440.913060384889832, 238.0574310451980296 ) ) ;
#56538=CARTESIAN_POINT ( 'NONE',  ( -13.00495165122699959, 1452.458917468459958, 149.1238935609289911 ) ) ;
#56539=CARTESIAN_POINT ( 'NONE',  ( -18.90720652019999903, 1416.826388498430106, 208.2175296474880213 ) ) ;
#56543=CARTESIAN_POINT ( 'NONE',  ( 14.39613795285440112, 1421.809772777419994, 229.5322598158189749 ) ) ;
#56545=ORIENTED_EDGE ( 'NONE', *, *, #20171, .F. ) ;
#56546=VERTEX_POINT ( 'NONE', #52497 ) ;
#56547=CARTESIAN_POINT ( 'NONE',  ( -10.43328091272586455, 1423.403754337453620, 137.2810607916168522 ) ) ;
#56548=CARTESIAN_POINT ( 'NONE',  ( -23.34267830565680057, 1409.843235500860146, 209.1109834998750046 ) ) ;
#56552=CARTESIAN_POINT ( 'NONE',  ( -21.65994954781430337, 1436.484406330281899, 143.5049664100171185 ) ) ;
#56553=CARTESIAN_POINT ( 'NONE',  ( 5.430576746648560160, 1440.816380464289978, 154.8042786433940137 ) ) ;
#56554=AXIS2_PLACEMENT_3D ( 'NONE', #89053, #21266, #105874 ) ;
#56555=ORIENTED_EDGE ( 'NONE', *, *, #51379, .T. ) ;
#56556=CARTESIAN_POINT ( 'NONE',  ( 45.02435768011299899, 1448.514094220139896, 266.7106273715389761 ) ) ;
#56558=CARTESIAN_POINT ( 'NONE',  ( -0.1387231356229999824, 1418.535612649829773, 184.6749245791980059 ) ) ;
#56560=VERTEX_POINT ( 'NONE', #35675 ) ;
#56562=CARTESIAN_POINT ( 'NONE',  ( 13.47253432440122367, 1443.597697226354512, 187.9990502360145683 ) ) ;
#56564=ORIENTED_EDGE ( 'NONE', *, *, #85787, .T. ) ;
#56566=PLANE ( 'NONE',  #59171 ) ;
#56567=CARTESIAN_POINT ( 'NONE',  ( -4.491579513878525276, 1425.338252514831993, 186.1547051059805540 ) ) ;
#56568=CARTESIAN_POINT ( 'NONE',  ( 6.210571358314980195, 1452.696182456529868, 151.8216972714639894 ) ) ;
#56569=CARTESIAN_POINT ( 'NONE',  ( 0.4691007450668729928, 1410.389848773719905, 269.3346290167360166 ) ) ;
#56574=CARTESIAN_POINT ( 'NONE',  ( -13.56684817831589918, 1434.956907115119748, 148.7388511781440172 ) ) ;
#56578=CARTESIAN_POINT ( 'NONE',  ( 7.320561577120000329, 1432.353341358199941, 149.5448088695980005 ) ) ;
#56580=CARTESIAN_POINT ( 'NONE',  ( 18.41412373400000035, 1436.828957585569924, 209.1218459616979999 ) ) ;
#56581=CARTESIAN_POINT ( 'NONE',  ( -11.73652925619994569, 1426.280330920429833, 144.1708004945943173 ) ) ;
#56588=CARTESIAN_POINT ( 'NONE',  ( 2.370970874524633398, 1427.002265528473799, 137.0999999980980135 ) ) ;
#56589=CARTESIAN_POINT ( 'NONE',  ( -2.953748537521290185, 1440.359176245339995, 157.3263145227589916 ) ) ;
#56590=CARTESIAN_POINT ( 'NONE',  ( -14.20165763179999807, 1416.819759806430056, 221.7375114452979972 ) ) ;
#56592=EDGE_CURVE ( 'NONE', #4376, #43234, #106087, .T. ) ;
#56600=CARTESIAN_POINT ( 'NONE',  ( 44.93138466476950299, 1440.913053015859987, 269.6837875441360097 ) ) ;
#56602=CARTESIAN_POINT ( 'NONE',  ( -1.546097701929999957, 1418.675484806429949, 228.1029857612980152 ) ) ;
#56607=CARTESIAN_POINT ( 'NONE',  ( 1.205374332583420191E-06, 1407.922920318890192, 195.8673945273630181 ) ) ;
#56609=CARTESIAN_POINT ( 'NONE',  ( -6.587888517611229844, 1432.346495048320094, 154.2385474615439875 ) ) ;
#56610=CARTESIAN_POINT ( 'NONE',  ( -1.543257077560000079, 1416.522662137829911, 228.0084432390979998 ) ) ;
#56611=CARTESIAN_POINT ( 'NONE',  ( 0.2117380174047990005, 1456.372610658380154, 183.1087122574759860 ) ) ;
#56612=CARTESIAN_POINT ( 'NONE',  ( -12.51283845067499989, 1408.316739414530048, 203.8172553575790005 ) ) ;
#56613=CARTESIAN_POINT ( 'NONE',  ( -16.04707966200000158, 1416.518532928429977, 200.6156669267779762 ) ) ;
#56615=CARTESIAN_POINT ( 'NONE',  ( -7.229059265610779939, 1441.096153944170055, 154.2643636803950073 ) ) ;
#56616=CARTESIAN_POINT ( 'NONE',  ( 11.87965657760000049, 1433.311156085379935, 147.2728768370980106 ) ) ;
#56617=CARTESIAN_POINT ( 'NONE',  ( -28.12790489320000020, 1436.808336956589756, 136.7412132036979813 ) ) ;
#56618=CARTESIAN_POINT ( 'NONE',  ( 10.30092211480000053, 1440.660729465949998, 187.2403783651980120 ) ) ;
#56625=CARTESIAN_POINT ( 'NONE',  ( 14.12036593068209989, 1509.406339180530040, 234.8413270297230042 ) ) ;
#56626=CARTESIAN_POINT ( 'NONE',  ( 2.852619981334113763, 1406.777728849647247, 269.6500679739756947 ) ) ;
#56629=CARTESIAN_POINT ( 'NONE',  ( 2.984390131719999673, 1428.733266614430022, 184.7181844846980141 ) ) ;
#56632=CARTESIAN_POINT ( 'NONE',  ( -26.81185573016960078, 1435.692944580150424, 136.1507310960283235 ) ) ;
#56633=CARTESIAN_POINT ( 'NONE',  ( -28.30911832768390113, 1508.554176145409883, 208.8345150349300070 ) ) ;
#56634=AXIS2_PLACEMENT_3D ( 'NONE', #69484, #77859, #18471 ) ;
#56635=CARTESIAN_POINT ( 'NONE',  ( -15.97071713983319974, 1409.722728690500162, 226.1176614794329964 ) ) ;
#56637=EDGE_LOOP ( 'NONE', ( #32016, #36421, #101958, #65221 ) ) ;
#56643=CARTESIAN_POINT ( 'NONE',  ( -0.1427736395143110182, 1420.459881824180002, 182.9082046469020213 ) ) ;
#56644=CARTESIAN_POINT ( 'NONE',  ( 1.121350373659999899, 1465.842768926529970, 235.5471876029980081 ) ) ;
#56645=CARTESIAN_POINT ( 'NONE',  ( 23.01825460670000112, 1410.638272742329946, 213.3724494741479987 ) ) ;
#56648=CARTESIAN_POINT ( 'NONE',  ( -17.85552477759999945, 1424.537816727530071, 227.5382918161980115 ) ) ;
#56658=CARTESIAN_POINT ( 'NONE',  ( -17.64330431710000013, 1423.732166419529904, 226.4225726569979997 ) ) ;
#56659=ORIENTED_EDGE ( 'NONE', *, *, #96826, .F. ) ;
#56661=CARTESIAN_POINT ( 'NONE',  ( -4.222911213134699970, 1441.593106041759938, 167.4128785044850076 ) ) ;
#56666=VERTEX_POINT ( 'NONE', #36786 ) ;
#56667=CARTESIAN_POINT ( 'NONE',  ( 8.313287170068500487, 1507.316777277299934, 183.0869016502879845 ) ) ;
#56669=FACE_OUTER_BOUND ( 'NONE', #67597, .T. ) ;
#56670=CARTESIAN_POINT ( 'NONE',  ( 15.82996380996429941, 1409.474171035389872, 192.7642349844859950 ) ) ;
#56672=CARTESIAN_POINT ( 'NONE',  ( -26.88456506701299986, 1450.694694235800171, 136.4506520073810236 ) ) ;
#56673=CARTESIAN_POINT ( 'NONE',  ( -11.43732278620000109, 1425.481241381329937, 144.1613654190979901 ) ) ;
#56677=CARTESIAN_POINT ( 'NONE',  ( 36.91977620337090116, 1451.033275236259897, 134.0999999987079718 ) ) ;
#56682=ORIENTED_EDGE ( 'NONE', *, *, #39094, .T. ) ;
#56685=CARTESIAN_POINT ( 'NONE',  ( 0.05562598889329999768, 1452.349460780129903, 183.2669973655980016 ) ) ;
#56686=CARTESIAN_POINT ( 'NONE',  ( -3.176595525550000243, 1485.137864157130025, 183.1894384333979815 ) ) ;
#56687=CARTESIAN_POINT ( 'NONE',  ( -2.500000000000000000, 1439.396215995059947, 161.7067243754309800 ) ) ;
#56693=CARTESIAN_POINT ( 'NONE',  ( 22.12673984907599944, 1409.685743169220132, 208.3470065775269973 ) ) ;
#56699=CARTESIAN_POINT ( 'NONE',  ( 36.38905843718290356, 1440.913060387330006, 262.8310855799430215 ) ) ;
#56700=CARTESIAN_POINT ( 'NONE',  ( -0.0002653596066196077410, 1452.517597898977101, 153.5752998968471275 ) ) ;
#56702=CARTESIAN_POINT ( 'NONE',  ( -0.1174241404373970038, 1452.347189664339794, 183.2668478624919999 ) ) ;
#56703=CARTESIAN_POINT ( 'NONE',  ( -16.57642552269999925, 1409.993768750830213, 191.9233248414979869 ) ) ;
#56704=CARTESIAN_POINT ( 'NONE',  ( 4.602958218326069779E-16, 1426.918876943007945, 134.0999999980979851 ) ) ;
#56707=CARTESIAN_POINT ( 'NONE',  ( -13.25186809610000083, 1419.889586077830018, 222.0034080458980270 ) ) ;
#56709=CARTESIAN_POINT ( 'NONE',  ( -1.436086187699999961, 1508.900106475729899, 179.8313947826979984 ) ) ;
#56710=CARTESIAN_POINT ( 'NONE',  ( -13.80580293259999891, 1434.979613021240084, 147.1507279520979807 ) ) ;
#56712=CARTESIAN_POINT ( 'NONE',  ( 13.80393196719999871, 1462.044328216929898, 230.7224726401980206 ) ) ;
#56713=CARTESIAN_POINT ( 'NONE',  ( -11.60004869885203682, 1424.622146315513419, 136.2523473544339083 ) ) ;
#56718=CARTESIAN_POINT ( 'NONE',  ( -0.3657342159832346895, 1486.413194173067495, 181.7790224318463856 ) ) ;
#56720=CARTESIAN_POINT ( 'NONE',  ( 4.311024656403059652, 1407.085546270103578, 221.5801435630039009 ) ) ;
#56722=FACE_OUTER_BOUND ( 'NONE', #78737, .T. ) ;
#56725=ORIENTED_EDGE ( 'NONE', *, *, #39266, .F. ) ;
#56726=DIRECTION ( 'NONE',  ( -0.1402804634180424004, -0.9901118076173111016, 0.000000000000000000 ) ) ;
#56728=CARTESIAN_POINT ( 'NONE',  ( -11.55098531880000046, 1430.396653715230059, 150.9171824720979771 ) ) ;
#56731=CARTESIAN_POINT ( 'NONE',  ( -3.774750576832590096E-15, 1432.353310171170051, 155.3998098058200128 ) ) ;
#56733=CARTESIAN_POINT ( 'NONE',  ( 12.54302623819999951, 1445.073512831690095, 186.6024346732980064 ) ) ;
#56735=CARTESIAN_POINT ( 'NONE',  ( -23.70830759550000266, 1457.436638280929856, 216.7744869258079916 ) ) ;
#56737=AXIS2_PLACEMENT_3D ( 'NONE', #70527, #79997, #43642 ) ;
#56741=CARTESIAN_POINT ( 'NONE',  ( 3.776163893200000121, 1405.832946398430067, 267.8478556236980239 ) ) ;
#56742=CARTESIAN_POINT ( 'NONE',  ( 0.1886752042949999819, 1409.088270638030053, 185.5766010327979814 ) ) ;
#56743=CARTESIAN_POINT ( 'NONE',  ( 18.18607966929999975, 1410.878986942329902, 193.7902918041979774 ) ) ;
#56745=CARTESIAN_POINT ( 'NONE',  ( 23.62496399655424284, 1434.148717771737438, 214.7198664209217611 ) ) ;
#56746=CARTESIAN_POINT ( 'NONE',  ( 8.991744574390811096, 1509.227061438039982, 181.2342617849590169 ) ) ;
#56747=CARTESIAN_POINT ( 'NONE',  ( 27.12603011487975380, 1508.017486813007508, 214.4686767731490988 ) ) ;
#56750=CARTESIAN_POINT ( 'NONE',  ( -2.310870060038839657, 1449.824111060830091, 154.7919463925260004 ) ) ;
#56751=CARTESIAN_POINT ( 'NONE',  ( -1.595915170252538928, 1451.462758934706926, 183.9376596482218815 ) ) ;
#56753=DIRECTION ( 'NONE',  ( 0.000000000000000000, 1.000000000000000000, 0.000000000000000000 ) ) ;
#56756=CARTESIAN_POINT ( 'NONE',  ( -7.417345643215089268, 1409.172079804809982, 196.1196827968989851 ) ) ;
#56757=CIRCLE ( 'NONE', #65712, 1.638701816490922836 ) ;
#56758=CARTESIAN_POINT ( 'NONE',  ( -27.19943328049049924, 1507.991540615329995, 211.1058746345759971 ) ) ;
#56759=CARTESIAN_POINT ( 'NONE',  ( 2.500000004939999965, 1439.742886558890177, 158.2293697702980069 ) ) ;
#56760=CARTESIAN_POINT ( 'NONE',  ( -3.426102627740000184, 1475.665556257130220, 269.0410120623980106 ) ) ;
#56766=VECTOR ( 'NONE', #99570, 1000.000000000000114 ) ;
#56771=CARTESIAN_POINT ( 'NONE',  ( -21.62801678940000016, 1409.668327376230081, 205.1400470743279811 ) ) ;
#56773=CARTESIAN_POINT ( 'NONE',  ( 19.56843215269274339, 1455.495710568705817, 225.8468362473698505 ) ) ;
#56774=ORIENTED_EDGE ( 'NONE', *, *, #62048, .T. ) ;
#56775=CARTESIAN_POINT ( 'NONE',  ( -3.500000000000000000, 1420.857604035629947, 170.3256330572980062 ) ) ;
#56778=CARTESIAN_POINT ( 'NONE',  ( 11.73643847070000135, 1426.280399246029901, 144.1643001595979854 ) ) ;
#56781=CARTESIAN_POINT ( 'NONE',  ( -3.827327205999999649, 1424.046157813729906, 172.2701767054979882 ) ) ;
#56786=CARTESIAN_POINT ( 'NONE',  ( -11.91590827042684886, 1398.266372442801185, 203.9246104138306350 ) ) ;
#56794=CARTESIAN_POINT ( 'NONE',  ( -12.78033923309999942, 1396.878026447830052, 207.4324367705480086 ) ) ;
#56795=CARTESIAN_POINT ( 'NONE',  ( -20.84521127210000202, 1410.135590990030096, 218.2730277501279943 ) ) ;
#56796=CARTESIAN_POINT ( 'NONE',  ( -1.249587849150000096, 1415.128105756529976, 226.9283669200980000 ) ) ;
#56797=CARTESIAN_POINT ( 'NONE',  ( -12.80792181777679239, 1444.977435535784252, 169.4484251894283489 ) ) ;
#56798=CARTESIAN_POINT ( 'NONE',  ( -24.66760647159999920, 1507.924356353729991, 197.5571972356979984 ) ) ;
#56802=CARTESIAN_POINT ( 'NONE',  ( 2.254275791129999984, 1429.771643255829986, 184.6574991238979919 ) ) ;
#56803=FACE_OUTER_BOUND ( 'NONE', #25203, .T. ) ;
#56805=CARTESIAN_POINT ( 'NONE',  ( 10.74800670940959968, 1396.288389052329876, 211.7634410043349931 ) ) ;
#56806=CARTESIAN_POINT ( 'NONE',  ( 14.44521984438589968, 1416.640375558050209, 196.8647061789440045 ) ) ;
#56807=CARTESIAN_POINT ( 'NONE',  ( 11.73918745480000148, 1430.041041296030016, 150.4070077459980155 ) ) ;
#56808=CARTESIAN_POINT ( 'NONE',  ( 8.778933807423072722, 1427.705008372408884, 144.1938086916980524 ) ) ;
#56809=ORIENTED_EDGE ( 'NONE', *, *, #19177, .F. ) ;
#56812=VERTEX_POINT ( 'NONE', #27835 ) ;
#56815=CARTESIAN_POINT ( 'NONE',  ( -14.41342808100000106, 1461.324647189130246, 229.5770031318979818 ) ) ;
#56818=B_SPLINE_CURVE_WITH_KNOTS ( 'NONE', 3,
 ( #58918, #83543, #24179, #17420 ),
 .UNSPECIFIED., .F., .F.,
 ( 4, 4 ),
 ( -0.5072555466292649751, -1.464889561797466655E-05 ),
 .UNSPECIFIED. ) ;
#56824=CARTESIAN_POINT ( 'NONE',  ( -5.967056112589649075, 1509.202713547270150, 179.6294632429990088 ) ) ;
#56827=EDGE_CURVE ( 'NONE', #18900, #32788, #79526, .T. ) ;
#56829=ORIENTED_EDGE ( 'NONE', *, *, #40810, .T. ) ;
#56831=CARTESIAN_POINT ( 'NONE',  ( -20.81915287150000182, 1509.403205472729951, 229.3701441624979793 ) ) ;
#56833=CARTESIAN_POINT ( 'NONE',  ( -37.04769550936495648, 1426.517324163738976, 269.5612620262075438 ) ) ;
#56835=CARTESIAN_POINT ( 'NONE',  ( -2.295852000570000495, 1409.930597616830028, 232.7102332357979719 ) ) ;
#56838=CARTESIAN_POINT ( 'NONE',  ( -0.01061436087871939909, 1451.719132097020065, 182.8647455669690203 ) ) ;
#56839=CARTESIAN_POINT ( 'NONE',  ( -33.56105288671160025, 1440.913060389879774, 247.8846291584730182 ) ) ;
#56842=CARTESIAN_POINT ( 'NONE',  ( -0.1401266656683599898, 1467.139399683509737, 235.6380456311810008 ) ) ;
#56843=CARTESIAN_POINT ( 'NONE',  ( 5.184301943030460436, 1410.264407675250141, 269.8675697800640023 ) ) ;
#56846=CARTESIAN_POINT ( 'NONE',  ( 24.11881256550000074, 1411.115306210429708, 209.4847445257949801 ) ) ;
#56847=CARTESIAN_POINT ( 'NONE',  ( -20.42683341999999769, 1508.879048844430145, 189.1348644687979856 ) ) ;
#56849=CARTESIAN_POINT ( 'NONE',  ( -11.60004869885203505, 1424.622146314968859, 136.2523473539528140 ) ) ;
#56851=CARTESIAN_POINT ( 'NONE',  ( 4.192373415348820131, 1421.117595978020063, 185.3194811860539915 ) ) ;
#56854=CARTESIAN_POINT ( 'NONE',  ( 3.187570095870436937, 1421.874552375644726, 137.0999999983294799 ) ) ;
#56856=ORIENTED_EDGE ( 'NONE', *, *, #9110, .T. ) ;
#56858=CARTESIAN_POINT ( 'NONE',  ( 16.66094735743510213, 1410.867388111209948, 226.5061907891179942 ) ) ;
#56860=EDGE_CURVE ( 'NONE', #93599, #57270, #106296, .T. ) ;
#56862=CARTESIAN_POINT ( 'NONE',  ( -5.387550183790000169, 1432.551483143010046, 154.6121797508980080 ) ) ;
#56867=CARTESIAN_POINT ( 'NONE',  ( -21.13431252044160047, 1409.651086843229905, 211.8287216663260040 ) ) ;
#56869=AXIS2_PLACEMENT_3D ( 'NONE', #103556, #53756, #68892 ) ;
#56874=CARTESIAN_POINT ( 'NONE',  ( -0.1685274451060000123, 1477.411888517829993, 230.0191311744979998 ) ) ;
#56875=CARTESIAN_POINT ( 'NONE',  ( 23.84753075949999968, 1447.297452739720029, 215.9843744054980164 ) ) ;
#56879=CARTESIAN_POINT ( 'NONE',  ( 10.69985963648862004, 1418.135228670047809, 229.9018306247701275 ) ) ;
#56881=CARTESIAN_POINT ( 'NONE',  ( -19.05061113289999852, 1426.018939432130082, 224.9263685105979960 ) ) ;
#56885=CARTESIAN_POINT ( 'NONE',  ( 17.18006689280000288, 1461.960330296729808, 189.9390536651980028 ) ) ;
#56887=CARTESIAN_POINT ( 'NONE',  ( -34.42417634216256772, 1458.387040857726333, 269.5237062428848844 ) ) ;
#56890=CARTESIAN_POINT ( 'NONE',  ( -14.11093413346683612, 1408.367734284578319, 269.5873373858704554 ) ) ;
#56891=VECTOR ( 'NONE', #20682, 1000.000000000000114 ) ;
#56894=CARTESIAN_POINT ( 'NONE',  ( -15.48407483730515644, 1451.379909330961709, 222.5591913156476949 ) ) ;
#56895=CARTESIAN_POINT ( 'NONE',  ( -13.15765241484907300, 1444.750370938229707, 186.5139969393457307 ) ) ;
#56897=CARTESIAN_POINT ( 'NONE',  ( -5.276062718737005497, 1507.211508871218712, 236.2464138374867844 ) ) ;
#56900=CARTESIAN_POINT ( 'NONE',  ( 24.92861831849999987, 1436.146573568669965, 137.7188798219979731 ) ) ;
#56902=CARTESIAN_POINT ( 'NONE',  ( -14.52033150799999994, 1409.926738554830081, 226.5601352792980094 ) ) ;
#56911=CARTESIAN_POINT ( 'NONE',  ( 3.176504636720000085E-09, 1468.737548874529921, 250.5651368536980215 ) ) ;
#56912=B_SPLINE_CURVE_WITH_KNOTS ( 'NONE', 3,
 ( #63532, #71940, #28795, #104392 ),
 .UNSPECIFIED., .F., .F.,
 ( 4, 4 ),
 ( 1.502771284927900908, 1.508489632590340079 ),
 .UNSPECIFIED. ) ;
#56913=CARTESIAN_POINT ( 'NONE',  ( -20.02495950560000182, 1491.257731268429779, 190.2391440648979994 ) ) ;
#56914=CIRCLE ( 'NONE', #46231, 4.004360693725719678 ) ;
#56915=CARTESIAN_POINT ( 'NONE',  ( -11.00793686009999917, 1433.412981438380029, 151.7533247267980130 ) ) ;
#56916=EDGE_CURVE ( 'NONE', #20305, #7608, #61216, .T. ) ;
#56920=ADVANCED_FACE ( 'NONE', ( #43818 ), #51121, .F. ) ;
#56921=CARTESIAN_POINT ( 'NONE',  ( -25.59514252499999998, 1439.610094980949953, 138.2637330278979846 ) ) ;
#56924=CARTESIAN_POINT ( 'NONE',  ( 3.102049425449999731, 1451.170629086630015, 183.9343634219979720 ) ) ;
#56927=CARTESIAN_POINT ( 'NONE',  ( -12.51566962417496143, 1509.474120198974106, 236.3954631667255626 ) ) ;
#56929=CARTESIAN_POINT ( 'NONE',  ( 1.013095580766330129E-08, 1409.267137198459977, 260.2682267152229656 ) ) ;
#56932=CARTESIAN_POINT ( 'NONE',  ( -11.85846968594809958, 1431.803688344790089, 149.9564276896689989 ) ) ;
#56935=CARTESIAN_POINT ( 'NONE',  ( -7.395436080089999642, 1472.163566644230059, 270.3697506832979798 ) ) ;
#56937=( BOUNDED_CURVE ( )  B_SPLINE_CURVE ( 3, ( #88953, #70540, #72724, #3882 ),
 .UNSPECIFIED., .F., .T. ) 
 B_SPLINE_CURVE_WITH_KNOTS ( ( 4, 4 ),
 ( 4.310049633749867937, 4.645868665744727011 ),
 .UNSPECIFIED. ) 
 CURVE ( )  GEOMETRIC_REPRESENTATION_ITEM ( )  RATIONAL_B_SPLINE_CURVE ( ( 1.000000000000000000, 0.9906241907223192200, 0.9906241907223192200, 1.000000000000000000 ) ) 
 REPRESENTATION_ITEM ( '' )  );
#56938=CARTESIAN_POINT ( 'NONE',  ( 1.600048698852036821, 1411.254281879943164, 137.0999999980979851 ) ) ;
#56939=CARTESIAN_POINT ( 'NONE',  ( 35.80456163590090313, 1451.000443318900125, 135.9277141877360293 ) ) ;
#56941=CARTESIAN_POINT ( 'NONE',  ( 0.2335509722129010257, 1451.541237093220161, 182.7232813895910226 ) ) ;
#56943=CARTESIAN_POINT ( 'NONE',  ( 12.27023112330000032, 1416.839692136459917, 223.5796784318309847 ) ) ;
#56946=CARTESIAN_POINT ( 'NONE',  ( -39.78160441305559658, 1422.810119569090148, 268.4168317394310179 ) ) ;
#56948=CARTESIAN_POINT ( 'NONE',  ( -3.534341588258910427, 1492.696478981339851, 181.5914780206049954 ) ) ;
#56953=CARTESIAN_POINT ( 'NONE',  ( -2.500000000000000000, 1425.929641636930000, 184.1455913746980002 ) ) ;
#56955=EDGE_CURVE ( 'NONE', #101745, #94269, #98437, .T. ) ;
#56957=CARTESIAN_POINT ( 'NONE',  ( -3.497130751176168673, 1441.358031377314319, 170.5351636631657755 ) ) ;
#56958=CARTESIAN_POINT ( 'NONE',  ( -16.07232597160000154, 1440.437412726279945, 189.9216664607980078 ) ) ;
#56959=CARTESIAN_POINT ( 'NONE',  ( -17.74184486700000107, 1415.163755984229965, 208.0694140301980326 ) ) ;
#56960=ORIENTED_EDGE ( 'NONE', *, *, #16997, .F. ) ;
#56961=CARTESIAN_POINT ( 'NONE',  ( -25.99289974769999745, 1436.215948439619979, 136.7796492369979831 ) ) ;
#56967=CARTESIAN_POINT ( 'NONE',  ( 0.06333900032629999344, 1408.725629451930217, 195.0481631164979888 ) ) ;
#56969=FACE_OUTER_BOUND ( 'NONE', #41485, .T. ) ;
#56971=ORIENTED_EDGE ( 'NONE', *, *, #57916, .F. ) ;
#56973=B_SPLINE_CURVE_WITH_KNOTS ( 'NONE', 3,
 ( #47270, #57886, #81953, #100419, #64641, #5260, #74138, #57349, #92021, #49483, #31554, #98762, #74687, #23702, #108820, #73590, #56220, #15291, #14197, #83606, #6904, #32665, #90351, #31005, #66843, #65185, #91474, #90913, #100953, #89813, #82526, #13084, #5823, #39962, #108268, #65732, #77977, #58429 ),
 .UNSPECIFIED., .F., .F.,
 ( 4, 2, 2, 1, 1, 1, 1, 2, 2, 2, 1, 1, 1, 1, 2, 2, 2, 2, 2, 2, 2, 2, 4 ),
 ( 0.000000000000000000, 0.2499999999999851230, 0.3749999999999770184, 0.4374999999999749090, 0.4687499999999736877, 0.4843749999999719669, 0.4921874999999717448, 0.4960937499999722444, 0.4999999999999726885, 0.6249999999999740208, 0.6874999999999745759, 0.7187499999999750200, 0.7343749999999742428, 0.7421874999999739098, 0.7460937499999727995, 0.7499999999999716893, 0.8124999999999706901, 0.8437499999999695799, 0.8593749999999681366, 0.8671874999999682476, 0.8710937499999690248, 0.8749999999999698019, 1.000000000000000000 ),
 .UNSPECIFIED. ) ;
#56975=CARTESIAN_POINT ( 'NONE',  ( 32.52417149305044575, 1464.889216426557823, 269.3047436042317599 ) ) ;
#56978=CARTESIAN_POINT ( 'NONE',  ( 2.500574528909250027, 1448.942056006560051, 154.5733147652059927 ) ) ;
#56979=CARTESIAN_POINT ( 'NONE',  ( -1.857324058419999924, 1485.892948864229993, 182.0392558147979969 ) ) ;
#56983=CARTESIAN_POINT ( 'NONE',  ( -1.725662463192670248, 1484.236887848700007, 182.7463278875050037 ) ) ;
#56985=CARTESIAN_POINT ( 'NONE',  ( 18.80431614589912925, 1425.839298383276855, 225.4579118312513799 ) ) ;
#56988=ORIENTED_EDGE ( 'NONE', *, *, #106963, .F. ) ;
#56989=CARTESIAN_POINT ( 'NONE',  ( -38.81202643688960308, 1436.797832322100021, 134.7398497853949948 ) ) ;
#56992=CARTESIAN_POINT ( 'NONE',  ( -12.78749341904959991, 1416.842625005220043, 196.1051283137009875 ) ) ;
#56993=EDGE_LOOP ( 'NONE', ( #35344, #46974, #400, #84474 ) ) ;
#56995=CARTESIAN_POINT ( 'NONE',  ( 12.52716981047909961, 1435.792588977599962, 150.9477529820620134 ) ) ;
#56996=CARTESIAN_POINT ( 'NONE',  ( 13.36846539799999967, 1415.041103189330215, 197.6149988125980030 ) ) ;
#57000=CARTESIAN_POINT ( 'NONE',  ( 17.13440814598840234, 1415.954755712160022, 210.5946189592040128 ) ) ;
#57001=CARTESIAN_POINT ( 'NONE',  ( -23.77630258579999634, 1416.435788914229988, 210.4864640035480079 ) ) ;
#57003=CARTESIAN_POINT ( 'NONE',  ( -0.02610323598444003190, 1506.535970902593817, 187.0533209056380315 ) ) ;
#57004=CARTESIAN_POINT ( 'NONE',  ( 4.273772382725350205, 1441.086506954710103, 157.4487869396440090 ) ) ;
#57005=CARTESIAN_POINT ( 'NONE',  ( 2.500000000000000000, 1439.396215927459934, 161.7067232356089903 ) ) ;
#57007=CARTESIAN_POINT ( 'NONE',  ( -16.68599179819999989, 1461.099982565929849, 230.2790296985980092 ) ) ;
#57011=CARTESIAN_POINT ( 'NONE',  ( -22.59589776172869691, 1507.700906949889941, 190.9355226902430047 ) ) ;
#57015=CIRCLE ( 'NONE', #31973, 2.000006057866878351 ) ;
#57018=CARTESIAN_POINT ( 'NONE',  ( 12.92703571545800045, 1509.364482422050060, 181.5834217730510147 ) ) ;
#57019=CARTESIAN_POINT ( 'NONE',  ( 11.11955572112504598, 1425.169096886590978, 138.4856970310274278 ) ) ;
#57020=CARTESIAN_POINT ( 'NONE',  ( 3.043251597425320032, 1417.779699503100119, 234.3208248802520188 ) ) ;
#57021=CARTESIAN_POINT ( 'NONE',  ( -2.500000000000000000, 1421.191390850129892, 151.1105839291980146 ) ) ;
#57024=CARTESIAN_POINT ( 'NONE',  ( 31.09959380193599898, 1440.913060384139953, 241.6673604977229957 ) ) ;
#57027=LINE ( 'NONE', #6049, #68968 ) ;
#57031=CARTESIAN_POINT ( 'NONE',  ( -11.66183466779353672, 1506.404057808254720, 227.7379997552472730 ) ) ;
#57035=CARTESIAN_POINT ( 'NONE',  ( 2.688586027246119947, 1509.006950727750109, 238.2845013960090057 ) ) ;
#57038=EDGE_CURVE ( 'NONE', #35225, #24399, #3185, .T. ) ;
#57042=CARTESIAN_POINT ( 'NONE',  ( -13.59753454029999808, 1453.151875978430098, 193.6408191069980091 ) ) ;
#57044=CARTESIAN_POINT ( 'NONE',  ( -11.88383462049809935, 1433.642778087510123, 147.6544717980860355 ) ) ;
#57045=CARTESIAN_POINT ( 'NONE',  ( -23.55087667009999919, 1411.110693366829764, 210.4794020521279947 ) ) ;
#57048=DIRECTION ( 'NONE',  ( -0.03489949670246857150, 0.9993908270190969834, 0.000000000000000000 ) ) ;
#57051=CARTESIAN_POINT ( 'NONE',  ( -17.55992563626299940, 1415.427621830080170, 208.9996007598010124 ) ) ;
#57052=ORIENTED_EDGE ( 'NONE', *, *, #51473, .F. ) ;
#57060=CARTESIAN_POINT ( 'NONE',  ( -8.991629940588330427, 1509.227055023859975, 237.0095830223739881 ) ) ;
#57062=CARTESIAN_POINT ( 'NONE',  ( -3.327638442502410143, 1485.035901024235045, 183.3370786331138902 ) ) ;
#57063=CARTESIAN_POINT ( 'NONE',  ( 4.898545953690760513, 1409.084121381390105, 194.9685614766650019 ) ) ;
#57064=CARTESIAN_POINT ( 'NONE',  ( 18.52260186970000433, 1425.593317732829973, 225.5454236923980034 ) ) ;
#57065=CARTESIAN_POINT ( 'NONE',  ( 3.741709429870000214, 1419.924742150030170, 185.5167356432980057 ) ) ;
#57066=CARTESIAN_POINT ( 'NONE',  ( -19.82310150189999831, 1485.643326822829977, 190.4781767699980151 ) ) ;
#57067=CARTESIAN_POINT ( 'NONE',  ( 11.57581721370000061, 1432.288378390559956, 151.1967356790979977 ) ) ;
#57069=ORIENTED_EDGE ( 'NONE', *, *, #48250, .T. ) ;
#57070=CARTESIAN_POINT ( 'NONE',  ( -2.189600725003922665, 1397.978978549970634, 196.1218685907498696 ) ) ;
#57071=CARTESIAN_POINT ( 'NONE',  ( 19.01768856890259940, 1456.707458847550015, 226.2400544105869926 ) ) ;
#57072=CARTESIAN_POINT ( 'NONE',  ( -12.28572370999999919, 1434.398876809329977, 150.4686729132979792 ) ) ;
#57073=AXIS2_PLACEMENT_3D ( 'NONE', #107036, #64512, #30323 ) ;
#57074=EDGE_CURVE ( 'NONE', #59250, #35478, #98265, .T. ) ;
#57076=CARTESIAN_POINT ( 'NONE',  ( -6.617837785385730167E-10, 1467.263505378270111, 245.8824296936540179 ) ) ;
#57077=CARTESIAN_POINT ( 'NONE',  ( -20.20716384489490025, 1495.140560500310130, 190.7583971611010156 ) ) ;
#57082=CARTESIAN_POINT ( 'NONE',  ( -45.85451249346039759, 1440.699916666199897, 268.7563676993480044 ) ) ;
#57083=CARTESIAN_POINT ( 'NONE',  ( -20.07368861760000200, 1427.190829891029807, 224.4645657875979907 ) ) ;
#57084=EDGE_CURVE ( 'NONE', #51188, #105370, #47188, .T. ) ;
#57085=CARTESIAN_POINT ( 'NONE',  ( -20.01067139950000140, 1507.877425041529932, 188.9709217985979706 ) ) ;
#57087=DIRECTION ( 'NONE',  ( -1.000000000000000000, 0.000000000000000000, 0.000000000000000000 ) ) ;
#57089=CARTESIAN_POINT ( 'NONE',  ( -2.320366121469999879E-14, 1422.005499580429841, 112.3240130698980010 ) ) ;
#57091=CIRCLE ( 'NONE', #62467, 2.000000000549930324 ) ;
#57093=CARTESIAN_POINT ( 'NONE',  ( 29.66529949999999971, 1430.834809503430051, 244.2516413529979786 ) ) ;
#57095=CARTESIAN_POINT ( 'NONE',  ( -2.509552835650000091, 1469.876049247530091, 182.4287443342980168 ) ) ;
#57098=CARTESIAN_POINT ( 'NONE',  ( -4.694071438699999987, 1416.682256490530108, 238.2947547715980079 ) ) ;
#57100=EDGE_CURVE ( 'NONE', #89175, #27764, #29912, .T. ) ;
#57101=CARTESIAN_POINT ( 'NONE',  ( -19.22419269387500051, 1452.241736785570083, 144.1488803750449961 ) ) ;
#57102=CARTESIAN_POINT ( 'NONE',  ( 27.43971470800000034, 1451.956092027530076, 135.3397597194980051 ) ) ;
#57104=CARTESIAN_POINT ( 'NONE',  ( -5.366169653819650165, 1425.895367196510051, 152.2258176257520290 ) ) ;
#57105=CARTESIAN_POINT ( 'NONE',  ( 16.10004403616710178, 1421.719552068429948, 227.3840503930599937 ) ) ;
#57106=CARTESIAN_POINT ( 'NONE',  ( -3.708479360574112871, 1448.977613576670137, 184.9605879005348470 ) ) ;
#57107=ORIENTED_EDGE ( 'NONE', *, *, #83741, .F. ) ;
#57110=CARTESIAN_POINT ( 'NONE',  ( -24.09440364030000126, 1410.858583525330005, 209.4069519282039948 ) ) ;
#57113=CARTESIAN_POINT ( 'NONE',  ( 0.2223819999059999941, 1416.825245919329973, 227.1889460349979970 ) ) ;
#57115=ADVANCED_FACE ( 'NONE', ( #25066 ), #10530, .F. ) ;
#57116=CARTESIAN_POINT ( 'NONE',  ( -4.763329158539999497, 1498.348145572129852, 235.9684822528980135 ) ) ;
#57118=CARTESIAN_POINT ( 'NONE',  ( 44.98134005857980355, 1448.496320712010174, 268.5302312373070208 ) ) ;
#57119=B_SPLINE_CURVE_WITH_KNOTS ( 'NONE', 3,
 ( #22581, #6918, #75252, #23712, #109942, #93128, #48395, #108830, #109401, #50590, #32127, #24262, #83082, #32677, #56786, #58442, #15841, #16395, #50046, #7473, #91484, #24795, #99861, #82538, #23158, #5834, #8019, #14763, #25354, #59547, #51695, #102608, #18067, #34332, #85836, #93660, #51143, #16941, #94223, #8567, #18609, #35436, #25908, #60106, #9674, #85269, #77990, #208, #94790, #68510, #42738, #9136, #52261, #27047, #110488, #86386, #76899, #52808, #102072, #69068, #17498, #43299 ),
 .UNSPECIFIED., .F., .F.,
 ( 4, 2, 2, 2, 1, 1, 1, 1, 2, 2, 2, 2, 2, 1, 1, 1, 2, 2, 2, 2, 2, 1, 1, 1, 1, 2, 2, 2, 2, 2, 1, 1, 1, 1, 1, 2, 2, 2, 4 ),
 ( 0.000000000000000000, 0.1249999999997849776, 0.1874999999996783406, 0.2187499999996239675, 0.2343749999995965727, 0.2421874999995830280, 0.2460937499995761168, 0.2480468749995727862, 0.2490234374995723421, 0.2499999999995718425, 0.3749999999996110334, 0.4374999999996306843, 0.4687499999996404543, 0.4843749999996453948, 0.4921874999996478373, 0.4960937499996490030, 0.4980468749996495581, 0.4999999999996500577, 0.6249999999997927214, 0.6874999999998652189, 0.7187499999999015232, 0.7343749999999198419, 0.7421874999999285016, 0.7460937499999318323, 0.7480468749999337197, 0.7490234374999340528, 0.7499999999999342748, 0.8124999999999202860, 0.8437499999999132916, 0.8593749999999095168, 0.8671874999999076294, 0.8710937499999068523, 0.8730468749999071854, 0.8740234374999071854, 0.8745117187499068523, 0.8747558593749064082, 0.8749999999999058531, 0.9374999999999529265, 1.000000000000000000 ),
 .UNSPECIFIED. ) ;
#57123=EDGE_LOOP ( 'NONE', ( #55176, #20589, #18616, #78136 ) ) ;
#57124=CYLINDRICAL_SURFACE ( 'NONE', #23956, 2.000000000000040856 ) ;
#57126=CARTESIAN_POINT ( 'NONE',  ( 13.49999674949678763, 1444.108888658031219, 187.9769059414830963 ) ) ;
#57128=ORIENTED_EDGE ( 'NONE', *, *, #44360, .F. ) ;
#57129=DIRECTION ( 'NONE',  ( 0.9993902469235412811, -0.03489947644508390595, -0.001077449749359510062 ) ) ;
#57138=CARTESIAN_POINT ( 'NONE',  ( 0.03595598587303577842, 1409.477698216540603, 232.9236783021701171 ) ) ;
#57140=CARTESIAN_POINT ( 'NONE',  ( -18.18137495006879689, 1507.546748573479817, 231.7129843945920129 ) ) ;
#57142=CARTESIAN_POINT ( 'NONE',  ( -25.65004514716680362, 1509.804860194309867, 223.0705507710869995 ) ) ;
#57144=CARTESIAN_POINT ( 'NONE',  ( 11.44291537990000052, 1428.994970000029980, 123.0297916884979941 ) ) ;
#57147=CARTESIAN_POINT ( 'NONE',  ( -0.1806136374258420219, 1424.270560426740076, 227.7175953970750015 ) ) ;
#57149=B_SPLINE_CURVE_WITH_KNOTS ( 'NONE', 3,
 ( #31906, #109186, #30245, #24032, #75035, #39767, #56574, #6151, #39197, #13991, #40859, #32471, #74490, #56023, #48178, #108617, #66645, #22934, #66094, #15087, #100221, #58230 ),
 .UNSPECIFIED., .F., .F.,
 ( 4, 3, 3, 3, 3, 3, 3, 4 ),
 ( -8.338844738667910761, -8.272689705420921413, -7.702803945130000329, -7.620147254847129403, -7.073208901094860224, -6.549836289219999941, -6.379554812754880011, -5.901451788533909948 ),
 .UNSPECIFIED. ) ;
#57154=VERTEX_POINT ( 'NONE', #5957 ) ;
#57156=CARTESIAN_POINT ( 'NONE',  ( -0.8307690413430001142, 1441.600846913440137, 150.7224806086979640 ) ) ;
#57159=CARTESIAN_POINT ( 'NONE',  ( 11.69137462480000167, 1433.691468119869796, 151.0156487431979997 ) ) ;
#57161=B_SPLINE_SURFACE_WITH_KNOTS ( 'NONE', 5, 5, ( 
 ( #62017, #102860, #35125, #69307, #44652, #87759 ),
 ( #60343, #104541, #17181, #26157, #76576, #34018 ),
 ( #103414, #27837, #94464, #42419, #26720, #18308 ),
 ( #96137, #110729, #51375, #35676, #69865, #103982 ),
 ( #95587, #78793, #81524, #54719, #21060, #55266 ),
 ( #62588, #63136, #30022, #3765, #88846, #36789 ),
 ( #70981, #12685, #79349, #12131, #37899, #19976 ),
 ( #28947, #22153, #11041, #88296, #3216, #46324 ),
 ( #45210, #89396, #97237, #11590, #64776, #46865 ) ),
 .UNSPECIFIED., .F., .F., .F.,
 ( 6, 3, 6 ),
 ( 6, 6 ),
 ( 52.44345828979999879, 59.24089506869999866, 65.18833056040000429 ),
 ( 0.000000000000000000, 2.000000000000000000 ),
 .UNSPECIFIED. ) ;
#57162=CARTESIAN_POINT ( 'NONE',  ( 0.6690161404288550440, 1450.887226503660031, 181.3223526815230002 ) ) ;
#57163=CARTESIAN_POINT ( 'NONE',  ( -16.19492410612830113, 1409.478599598990058, 194.0661808939520085 ) ) ;
#57167=CARTESIAN_POINT ( 'NONE',  ( 2.948872346249999943, 1422.097626302630033, 232.1500477468979966 ) ) ;
#57169=CARTESIAN_POINT ( 'NONE',  ( 8.178501070643639181, 1441.152429762079919, 153.9860758848200248 ) ) ;
#57170=CARTESIAN_POINT ( 'NONE',  ( -18.19301384260000276, 1410.911466596229957, 224.4445374971980129 ) ) ;
#57174=CARTESIAN_POINT ( 'NONE',  ( -17.29627815805059754, 1410.879850359289776, 192.2521459216479798 ) ) ;
#57178=CARTESIAN_POINT ( 'NONE',  ( -8.513184503609998899, 1416.823418193129783, 225.1807616044980023 ) ) ;
#57179=CARTESIAN_POINT ( 'NONE',  ( 0.2095880431046339976, 1457.579896474360112, 183.0569165344279838 ) ) ;
#57180=CARTESIAN_POINT ( 'NONE',  ( 17.99954443082109989, 1410.904693892220166, 222.9872220945560173 ) ) ;
#57182=CARTESIAN_POINT ( 'NONE',  ( -14.17095083369999919, 1415.425644477329797, 198.8594078928979911 ) ) ;
#57183=CARTESIAN_POINT ( 'NONE',  ( -28.69260574566120070, 1509.783796149900127, 211.3048446392940320 ) ) ;
#57184=CARTESIAN_POINT ( 'NONE',  ( 12.06097065039999983, 1433.903642588860066, 149.1895464303979963 ) ) ;
#57185=CARTESIAN_POINT ( 'NONE',  ( -36.90142499642229978, 1436.372079655220205, 134.0999999968939846 ) ) ;
#57186=CARTESIAN_POINT ( 'NONE',  ( 8.884500389519999430, 1442.039659523320097, 185.7099986671979934 ) ) ;
#57192=CARTESIAN_POINT ( 'NONE',  ( 19.79581223833070069, 1456.560079648279952, 208.7498543415190113 ) ) ;
#57194=CARTESIAN_POINT ( 'NONE',  ( 30.61211140304735423, 1415.566367963669336, 269.3440436895404559 ) ) ;
#57198=CARTESIAN_POINT ( 'NONE',  ( 2.662122199679999746, 1434.188649408250058, 184.0358250344979751 ) ) ;
#57202=ORIENTED_EDGE ( 'NONE', *, *, #5421, .F. ) ;
#57203=CARTESIAN_POINT ( 'NONE',  ( -27.53435635780000013, 1451.950595041229917, 135.3364336049980068 ) ) ;
#57204=CARTESIAN_POINT ( 'NONE',  ( -15.90322118183840061, 1409.851032194339950, 226.2872105686589919 ) ) ;
#57205=CARTESIAN_POINT ( 'NONE',  ( 0.4931964325117270675, 1416.531771736229985, 184.8057391746860105 ) ) ;
#57208=CARTESIAN_POINT ( 'NONE',  ( 40.26396420611710170, 1444.186530323160014, 137.1012295353969819 ) ) ;
#57209=CARTESIAN_POINT ( 'NONE',  ( 22.05719136570000316, 1509.683314482830156, 226.9345908605980071 ) ) ;
#57211=CARTESIAN_POINT ( 'NONE',  ( -11.27186231780000014, 1414.983773854429955, 195.8113391393980294 ) ) ;
#57212=CARTESIAN_POINT ( 'NONE',  ( 1.140627099109999820, 1464.949969008629978, 237.1896079457980022 ) ) ;
#57214=CARTESIAN_POINT ( 'NONE',  ( 22.19412108519999904, 1411.048331459529891, 215.6222843390580124 ) ) ;
#57217=CARTESIAN_POINT ( 'NONE',  ( -17.51054297519999992, 1422.888992222730167, 226.4554417862979960 ) ) ;
#57219=CARTESIAN_POINT ( 'NONE',  ( -2.695375846180000146, 1439.665988598389958, 184.6458907360980106 ) ) ;
#57220=CARTESIAN_POINT ( 'NONE',  ( 28.30907522670739951, 1508.149947046400030, 209.0156582300560331 ) ) ;
#57222=CARTESIAN_POINT ( 'NONE',  ( 22.66506344571072162, 1509.725666982945995, 190.0484376440009271 ) ) ;
#57223=CARTESIAN_POINT ( 'NONE',  ( -1.182106891199999898, 1417.417339269829881, 235.0246372144980000 ) ) ;
#57225=CARTESIAN_POINT ( 'NONE',  ( -12.72876562435690140, 1485.205841511860172, 185.8648739181089979 ) ) ;
#57226=ORIENTED_EDGE ( 'NONE', *, *, #3811, .T. ) ;
#57228=CARTESIAN_POINT ( 'NONE',  ( -4.223394594500030408, 1441.589115646509981, 167.1325015425969980 ) ) ;
#57230=ORIENTED_EDGE ( 'NONE', *, *, #68778, .T. ) ;
#57232=CARTESIAN_POINT ( 'NONE',  ( -18.00891391817198439, 1424.550919037707899, 228.0707037805817663 ) ) ;
#57236=CARTESIAN_POINT ( 'NONE',  ( 2.244413413239999766, 1428.081157166129969, 101.8807690336980016 ) ) ;
#57237=CARTESIAN_POINT ( 'NONE',  ( 15.78068549015720201, 1410.430256014650013, 191.5841938278840075 ) ) ;
#57239=CARTESIAN_POINT ( 'NONE',  ( 35.93245376812059533, 1437.277850137440055, 136.5217339136529802 ) ) ;
#57240=ADVANCED_FACE ( 'NONE', ( #39560 ), #32195, .F. ) ;
#57244=CARTESIAN_POINT ( 'NONE',  ( 17.10909533037560948, 1460.315389741178024, 228.6693725169167521 ) ) ;
#57245=ADVANCED_FACE ( 'NONE', ( #4317 ), #90501, .F. ) ;
#57248=CARTESIAN_POINT ( 'NONE',  ( 34.20278863698899841, 1451.714767517949895, 134.0999999981149813 ) ) ;
#57249=CARTESIAN_POINT ( 'NONE',  ( -9.849896899200842881, 1512.913060387330006, 185.5490084180013923 ) ) ;
#57252=AXIS2_PLACEMENT_3D ( 'NONE', #63180, #44702, #97286 ) ;
#57253=CARTESIAN_POINT ( 'NONE',  ( -18.58939038020000112, 1457.838465768930064, 227.5494389216979982 ) ) ;
#57257=CARTESIAN_POINT ( 'NONE',  ( -16.63505975150000182, 1409.493969474430060, 194.0661809352979787 ) ) ;
#57258=CARTESIAN_POINT ( 'NONE',  ( 0.07955197424319999933, 1452.993118421130021, 183.2407363517980343 ) ) ;
#57260=CARTESIAN_POINT ( 'NONE',  ( -2.500000000000000000, 1439.569237629489862, 165.5254341707220078 ) ) ;
#57264=CARTESIAN_POINT ( 'NONE',  ( 38.81202643689640297, 1450.612734567539974, 134.7402675994790116 ) ) ;
#57266=CARTESIAN_POINT ( 'NONE',  ( 26.25207344680000077, 1438.555629842469898, 137.1352270321980029 ) ) ;
#57267=( BOUNDED_CURVE ( )  B_SPLINE_CURVE ( 3, ( #94641, #84586, #103599, #17916 ),
 .UNSPECIFIED., .F., .F. ) 
 B_SPLINE_CURVE_WITH_KNOTS ( ( 4, 4 ),
 ( 2.055417531154359878, 2.292695976159725202 ),
 .UNSPECIFIED. ) 
 CURVE ( )  GEOMETRIC_REPRESENTATION_ITEM ( )  RATIONAL_B_SPLINE_CURVE ( ( 1.000000000000000000, 0.9953137455213650897, 0.9953137455213650897, 1.000000000000000000 ) ) 
 REPRESENTATION_ITEM ( '' )  );
#57268=CARTESIAN_POINT ( 'NONE',  ( 3.954004997530000232, 1416.825421875629900, 190.9202402641980143 ) ) ;
#57270=VERTEX_POINT ( 'NONE', #32259 ) ;
#57273=VERTEX_POINT ( 'NONE', #47419 ) ;
#57274=CARTESIAN_POINT ( 'NONE',  ( 39.56090833897850700, 1440.913060387330006, 266.8640727595400222 ) ) ;
#57275=CARTESIAN_POINT ( 'NONE',  ( -5.623474965688048840E-07, 1451.660737107639989, 154.0815186765750013 ) ) ;
#57276=VERTEX_POINT ( 'NONE', #97802 ) ;
#57281=CARTESIAN_POINT ( 'NONE',  ( -12.83610317870000017, 1419.900230477330069, 222.0779048188979914 ) ) ;
#57283=CARTESIAN_POINT ( 'NONE',  ( -0.7774504691479999785, 1508.162354399930109, 180.6410561175979979 ) ) ;
#57284=CARTESIAN_POINT ( 'NONE',  ( -13.50121300870000063, 1434.968976328030067, 147.8555663532980020 ) ) ;
#57285=CARTESIAN_POINT ( 'NONE',  ( 11.73700276280139931, 1426.696010850159837, 144.1682878426319974 ) ) ;
#57286=CARTESIAN_POINT ( 'NONE',  ( 11.98966118179999896, 1463.071801668629860, 231.6035992477980017 ) ) ;
#57287=FACE_OUTER_BOUND ( 'NONE', #1569, .T. ) ;
#57289=AXIS2_PLACEMENT_3D ( 'NONE', #48223, #5661, #5094 ) ;
#57291=EDGE_CURVE ( 'NONE', #2313, #75650, #64793, .T. ) ;
#57293=ORIENTED_EDGE ( 'NONE', *, *, #4212, .F. ) ;
#57295=CARTESIAN_POINT ( 'NONE',  ( -0.1382356955943349897, 1507.743408363169920, 180.7718112797529955 ) ) ;
#57296=CARTESIAN_POINT ( 'NONE',  ( 5.157704406284129827E-09, 1406.911841301380036, 222.1218459627310153 ) ) ;
#57302=VERTEX_POINT ( 'NONE', #85967 ) ;
#57303=CIRCLE ( 'NONE', #78690, 1.999999943602009500 ) ;
#57304=CARTESIAN_POINT ( 'NONE',  ( 23.90675415119999769, 1449.162507167900003, 221.6525748645979945 ) ) ;
#57305=CARTESIAN_POINT ( 'NONE',  ( -10.96880036559999816, 1432.299257934029811, 151.7701915755980053 ) ) ;
#57311=CARTESIAN_POINT ( 'NONE',  ( -21.63676776550000014, 1444.797379379979930, 220.8518329349979865 ) ) ;
#57312=CARTESIAN_POINT ( 'NONE',  ( -2.695946308289999926, 1485.848501370129952, 182.4462471358980054 ) ) ;
#57313=ORIENTED_EDGE ( 'NONE', *, *, #100040, .F. ) ;
#57315=CARTESIAN_POINT ( 'NONE',  ( 6.156919420700000423, 1406.564961868729824, 269.2805947264979523 ) ) ;
#57316=CARTESIAN_POINT ( 'NONE',  ( -21.39772323737049931, 1509.704958956720020, 229.7894127843639751 ) ) ;
#57318=CARTESIAN_POINT ( 'NONE',  ( 22.91784880816845771, 1432.059886029948530, 216.2703706859424813 ) ) ;
#57320=CARTESIAN_POINT ( 'NONE',  ( -15.73574044604409927, 1409.462552572229924, 225.2910003602459881 ) ) ;
#57324=CARTESIAN_POINT ( 'NONE',  ( -11.97778741359999977, 1446.811539678010149, 187.5041641196980038 ) ) ;
#57329=CARTESIAN_POINT ( 'NONE',  ( -9.623804485526918029, 1409.249131045419745, 197.6748203005379878 ) ) ;
#57332=CARTESIAN_POINT ( 'NONE',  ( 3.116195436109999939, 1441.243535601449821, 166.9150391423980011 ) ) ;
#57333=CARTESIAN_POINT ( 'NONE',  ( -2.764108551270000103, 1475.699858318429960, 269.0427152816980083 ) ) ;
#57334=CARTESIAN_POINT ( 'NONE',  ( 3.045280019940000305, 1464.258769156330118, 233.3054829794980094 ) ) ;
#57336=CARTESIAN_POINT ( 'NONE',  ( 17.72813534363540100, 1410.891380463280029, 223.4205987578280030 ) ) ;
#57344=CARTESIAN_POINT ( 'NONE',  ( -20.29148499160000085, 1410.117176396729974, 199.0828523262979957 ) ) ;
#57347=CARTESIAN_POINT ( 'NONE',  ( -6.597068289630000137, 1407.874253871329756, 270.1316426411979705 ) ) ;
#57349=CARTESIAN_POINT ( 'NONE',  ( -7.990695852699508883, 1410.564740250183377, 230.6243468353451078 ) ) ;
#57352=CARTESIAN_POINT ( 'NONE',  ( 11.60353182090000068, 1425.885547122130220, 141.8419080669979735 ) ) ;
#57356=CARTESIAN_POINT ( 'NONE',  ( 27.42679559861360161, 1448.207338318150050, 136.8613456938669799 ) ) ;
#57360=CARTESIAN_POINT ( 'NONE',  ( -13.57909981250000087, 1416.568813547830132, 221.8977233994979770 ) ) ;
#57364=CARTESIAN_POINT ( 'NONE',  ( 20.56174574396830224, 1508.351243507949903, 228.2043451791550126 ) ) ;
#57367=ORIENTED_EDGE ( 'NONE', *, *, #99676, .F. ) ;
#57368=CARTESIAN_POINT ( 'NONE',  ( -7.841281984380000125, 1397.234782632230008, 219.8176822113979938 ) ) ;
#57369=CARTESIAN_POINT ( 'NONE',  ( -18.97336374349999844, 1409.575624849130008, 219.6734443658980069 ) ) ;
#57371=CARTESIAN_POINT ( 'NONE',  ( -12.98571499817150610, 1444.884868618428754, 169.4235797359238518 ) ) ;
#57375=CARTESIAN_POINT ( 'NONE',  ( -14.25772450459819929, 1509.411936130120012, 183.1493227206160270 ) ) ;
#57377=CARTESIAN_POINT ( 'NONE',  ( 3.333430315160000212, 1468.704004404630041, 183.2171971980980061 ) ) ;
#57381=CARTESIAN_POINT ( 'NONE',  ( 5.535200594421139542, 1396.106353873259877, 199.5716390489739922 ) ) ;
#57382=CARTESIAN_POINT ( 'NONE',  ( 0.7692391029780000222, 1415.628674266529742, 190.8565233057979924 ) ) ;
#57383=CARTESIAN_POINT ( 'NONE',  ( 11.63669227459999966, 1425.864836378729933, 144.1684971660979784 ) ) ;
#57384=CARTESIAN_POINT ( 'NONE',  ( 6.466214386739325803, 1509.141720294096103, 180.4348274801477316 ) ) ;
#57386=CARTESIAN_POINT ( 'NONE',  ( 12.94454588817750107, 1434.758408665909883, 149.3917831800590079 ) ) ;
#57387=ORIENTED_EDGE ( 'NONE', *, *, #54464, .F. ) ;
#57390=CARTESIAN_POINT ( 'NONE',  ( -8.376976394739999776, 1464.979757639830041, 233.1143827394980121 ) ) ;
#57394=ORIENTED_EDGE ( 'NONE', *, *, #53523, .F. ) ;
#57399=ORIENTED_EDGE ( 'NONE', *, *, #31524, .F. ) ;
#57406=CARTESIAN_POINT ( 'NONE',  ( -30.02908938876808875, 1419.599146942571451, 269.4711195632991689 ) ) ;
#57408=CARTESIAN_POINT ( 'NONE',  ( -0.2112786387671690136, 1416.230844595159851, 227.3034699774860030 ) ) ;
#57411=CARTESIAN_POINT ( 'NONE',  ( -34.73433026547840541, 1440.913060388860004, 250.3950812228370353 ) ) ;
#57413=CARTESIAN_POINT ( 'NONE',  ( -0.2112467950247060022, 1467.134318679190073, 235.6312670970790180 ) ) ;
#57414=CARTESIAN_POINT ( 'NONE',  ( 7.260534597404889823, 1410.692748237529941, 269.6205518878410317 ) ) ;
#57416=CARTESIAN_POINT ( 'NONE',  ( 24.08125413579999829, 1410.714371472329958, 209.1807164637870073 ) ) ;
#57417=CARTESIAN_POINT ( 'NONE',  ( -21.07299109810000104, 1509.588070516929974, 188.6993481227979998 ) ) ;
#57422=CARTESIAN_POINT ( 'NONE',  ( 0.07980232208509999148, 1420.214783457930025, 183.9037909274979938 ) ) ;
#57424=CARTESIAN_POINT ( 'NONE',  ( -11.64460141611553290, 1486.022579393844580, 184.5329476470979841 ) ) ;
#57426=ORIENTED_EDGE ( 'NONE', *, *, #92734, .T. ) ;
#57428=CARTESIAN_POINT ( 'NONE',  ( 18.79678650740000023, 1416.830000968129980, 209.8350674583659838 ) ) ;
#57431=CARTESIAN_POINT ( 'NONE',  ( -12.81872062859999950, 1420.998869512129886, 230.6915806954980042 ) ) ;
#57432=CARTESIAN_POINT ( 'NONE',  ( -5.519906363166400709, 1440.499855196290127, 154.7645174855159951 ) ) ;
#57434=CARTESIAN_POINT ( 'NONE',  ( 0.3863944528677800139, 1452.976072371400051, 183.2761518715429929 ) ) ;
#57435=AXIS2_PLACEMENT_3D ( 'NONE', #50975, #85653, #43126 ) ;
#57438=FACE_OUTER_BOUND ( 'NONE', #59467, .T. ) ;
#57444=CARTESIAN_POINT ( 'NONE',  ( 20.46945555039999931, 1454.918353507129950, 222.9273423791979951 ) ) ;
#57445=CARTESIAN_POINT ( 'NONE',  ( 7.175204869421878406, 1438.963982221705010, 154.0862487876218836 ) ) ;
#57448=CARTESIAN_POINT ( 'NONE',  ( 13.48815433605667558, 1419.590937927324376, 228.7311886359687776 ) ) ;
#57451=CARTESIAN_POINT ( 'NONE',  ( -18.66067488629999715, 1424.984128575629938, 224.8203133075979849 ) ) ;
#57452=CARTESIAN_POINT ( 'NONE',  ( 1.704192342800000001E-13, 1475.048391919030109, 269.6500679772980220 ) ) ;
#57455=CARTESIAN_POINT ( 'NONE',  ( 0.003646682923689930148, 1409.082053264339947, 232.6631847236010060 ) ) ;
#57456=CARTESIAN_POINT ( 'NONE',  ( -28.87437517114842933, 1463.054888223776970, 269.4592160712932127 ) ) ;
#57459=CARTESIAN_POINT ( 'NONE',  ( 11.66183224573578592, 1506.404057882402867, 190.5056905578398982 ) ) ;
#57461=CARTESIAN_POINT ( 'NONE',  ( -0.9786431567949999133, 1497.713060387329961, 231.7156151907979904 ) ) ;
#57462=CARTESIAN_POINT ( 'NONE',  ( -0.2057087554429999909, 1415.760339075730144, 233.4522620454979744 ) ) ;
#57463=CARTESIAN_POINT ( 'NONE',  ( -13.13022493104261912, 1443.049912350888235, 186.7023179654335081 ) ) ;
#57466=AXIS2_PLACEMENT_3D ( 'NONE', #39054, #13295, #105748 ) ;
#57467=CARTESIAN_POINT ( 'NONE',  ( -15.05358279999999915, 1410.831827720429828, 226.7261506157979909 ) ) ;
#57469=CARTESIAN_POINT ( 'NONE',  ( 23.92297853920000250, 1435.332916329309910, 136.8723201152980096 ) ) ;
#57471=CARTESIAN_POINT ( 'NONE',  ( -14.54195348929999909, 1410.802016793630173, 226.7659970022979792 ) ) ;
#57473=CARTESIAN_POINT ( 'NONE',  ( 0.08631495460215440896, 1416.225364278609959, 191.0306605155550130 ) ) ;
#57474=CARTESIAN_POINT ( 'NONE',  ( -4.049849602479999255, 1409.054484251730173, 230.6815826274979884 ) ) ;
#57475=ORIENTED_EDGE ( 'NONE', *, *, #5143, .F. ) ;
#57478=CARTESIAN_POINT ( 'NONE',  ( 12.78641131260000030, 1508.670053872629978, 233.6149044717980132 ) ) ;
#57479=CARTESIAN_POINT ( 'NONE',  ( -11.60004869885203682, 1428.983126981193436, 134.0999999980979851 ) ) ;
#57480=CARTESIAN_POINT ( 'NONE',  ( -21.03384925780000003, 1451.606557712130098, 216.4230814408879837 ) ) ;
#57482=CARTESIAN_POINT ( 'NONE',  ( -11.89654451160000015, 1433.279017673690078, 150.0536589393980194 ) ) ;
#57485=CARTESIAN_POINT ( 'NONE',  ( -25.67332895650000069, 1437.578766584980031, 137.2860071276980136 ) ) ;
#57486=CARTESIAN_POINT ( 'NONE',  ( -14.76828617137338284, 1430.034860089873064, 221.9615281545119956 ) ) ;
#57487=DIRECTION ( 'NONE',  ( 1.000000000000000000, 0.000000000000000000, 0.000000000000000000 ) ) ;
#57488=CARTESIAN_POINT ( 'NONE',  ( -0.3530891408735000181, 1467.116854267079816, 235.6078141451939985 ) ) ;
#57492=CARTESIAN_POINT ( 'NONE',  ( -9.976795219788707390E-10, 1413.055502352579879, 250.5859860138529598 ) ) ;
#57495=CARTESIAN_POINT ( 'NONE',  ( -11.73709356416840066, 1426.695943276110029, 144.1748013770919954 ) ) ;
#57497=CARTESIAN_POINT ( 'NONE',  ( -3.437536580710000234, 1471.945857284229987, 270.0719186626980104 ) ) ;
#57507=CARTESIAN_POINT ( 'NONE',  ( -29.09911720097530008, 1413.508132907530126, 267.4910557585119477 ) ) ;
#57511=ORIENTED_EDGE ( 'NONE', *, *, #60329, .F. ) ;
#57513=AXIS2_PLACEMENT_3D ( 'NONE', #81958, #97127, #12566 ) ;
#57514=CARTESIAN_POINT ( 'NONE',  ( 4.636884161006338267, 1423.705390323189931, 183.8726706823395887 ) ) ;
#57515=CARTESIAN_POINT ( 'NONE',  ( 40.87172354942210006, 1444.180909089139959, 136.9416239419680039 ) ) ;
#57518=CARTESIAN_POINT ( 'NONE',  ( -17.33962123819999945, 1455.455747421229944, 189.9678388033980241 ) ) ;
#57519=CARTESIAN_POINT ( 'NONE',  ( -2.500000000000000000, 1448.894380913990062, 183.1110264324979937 ) ) ;
#57520=ORIENTED_EDGE ( 'NONE', *, *, #15359, .T. ) ;
#57521=CARTESIAN_POINT ( 'NONE',  ( -26.49667341909999863, 1436.410274429069887, 136.7318106552980055 ) ) ;
#57526=CARTESIAN_POINT ( 'NONE',  ( 0.2333221319680495176, 1508.978111603873231, 238.8758415329143645 ) ) ;
#57527=CARTESIAN_POINT ( 'NONE',  ( -42.28242670489790100, 1436.141010253410059, 269.8809773090360409 ) ) ;
#57528=PLANE ( 'NONE',  #41827 ) ;
#57529=CARTESIAN_POINT ( 'NONE',  ( -4.911963663459999907, 1396.617948295830047, 197.5941244856979893 ) ) ;
#57531=ORIENTED_EDGE ( 'NONE', *, *, #35735, .F. ) ;
#57533=CARTESIAN_POINT ( 'NONE',  ( 0.3241978586559999820, 1451.160671602629918, 182.5582981364979958 ) ) ;
#57534=CARTESIAN_POINT ( 'NONE',  ( 22.50300749498944342, 1470.712031562941547, 269.4864744541472987 ) ) ;
#57536=CARTESIAN_POINT ( 'NONE',  ( -24.93017278910000201, 1436.287966887830180, 137.8924530763979988 ) ) ;
#57537=CARTESIAN_POINT ( 'NONE',  ( -0.5825634934640000484, 1486.373388144130104, 181.7400882333980121 ) ) ;
#57541=CARTESIAN_POINT ( 'NONE',  ( 4.500000000000000000, 1411.429641636930000, 146.1721969590979882 ) ) ;
#57543=CARTESIAN_POINT ( 'NONE',  ( 11.36018332919999985, 1414.996444518330009, 222.2791104509979903 ) ) ;
#57547=PLANE ( 'NONE',  #84871 ) ;
#57549=CARTESIAN_POINT ( 'NONE',  ( -19.63352108752347291, 1457.018114316206947, 225.8333846437924421 ) ) ;
#57550=ORIENTED_EDGE ( 'NONE', *, *, #55672, .T. ) ;
#57552=CARTESIAN_POINT ( 'NONE',  ( -23.60843796118631488, 1509.747304671633628, 226.8699424759173269 ) ) ;
#57553=CARTESIAN_POINT ( 'NONE',  ( -4.115381908448215498, 1440.053995635950969, 185.4419112703371013 ) ) ;
#57556=CARTESIAN_POINT ( 'NONE',  ( 3.615556770349780180, 1450.594495358166796, 184.1047078091952471 ) ) ;
#57559=CARTESIAN_POINT ( 'NONE',  ( 23.25291252615955884, 1449.806690063141104, 217.4642867579325411 ) ) ;
#57560=EDGE_CURVE ( 'NONE', #50150, #9923, #75251, .T. ) ;
#57561=DIRECTION ( 'NONE',  ( 0.9993902469228813645, -0.03489947646212200605, -0.001077449809515390556 ) ) ;
#57564=ORIENTED_EDGE ( 'NONE', *, *, #51073, .T. ) ;
#57566=CARTESIAN_POINT ( 'NONE',  ( -13.58968549449999941, 1472.672770405929896, 270.0972160539979541 ) ) ;
#57567=CARTESIAN_POINT ( 'NONE',  ( 1.326685568770000101, 1419.628109660430027, 184.8664938030979954 ) ) ;
#57568=CARTESIAN_POINT ( 'NONE',  ( -8.320723051859999941, 1424.406562835429895, 91.09139192869778867 ) ) ;
#57573=CARTESIAN_POINT ( 'NONE',  ( 17.37532935126821698, 1422.700099411153360, 226.5752429006997204 ) ) ;
#57576=CARTESIAN_POINT ( 'NONE',  ( 35.42325710281800610, 1440.913060386559891, 251.7637193835429628 ) ) ;
#57579=CARTESIAN_POINT ( 'NONE',  ( 13.02791634859999803, 1419.893455390129930, 221.8345185033979874 ) ) ;
#57581=EDGE_LOOP ( 'NONE', ( #60860, #83869, #106809, #49124, #17962, #64936 ) ) ;
#57589=CARTESIAN_POINT ( 'NONE',  ( 21.51466898170138720, 1509.781121651418061, 230.0944450856692640 ) ) ;
#57590=CARTESIAN_POINT ( 'NONE',  ( -5.389719915088219793, 1440.971386074470047, 154.8246291213590098 ) ) ;
#57595=DIRECTION ( 'NONE',  ( 0.8529498740721102035, 0.5214612423255851059, 0.02355175306912486027 ) ) ;
#57601=EDGE_LOOP ( 'NONE', ( #53762, #100038, #34670, #64241, #60310, #51478 ) ) ;
#57603=AXIS2_PLACEMENT_3D ( 'NONE', #51086, #146, #52743 ) ;
#57606=ADVANCED_FACE ( 'NONE', ( #78407 ), #49495, .F. ) ;
#57610=ADVANCED_FACE ( 'NONE', ( #35858 ), #16394, .F. ) ;
#57613=DIRECTION ( 'NONE',  ( 0.5969061220947440294, -0.8023110876747339137, 0.000000000000000000 ) ) ;
#57615=EDGE_CURVE ( 'NONE', #61659, #64952, #18961, .T. ) ;
#57620=CARTESIAN_POINT ( 'NONE',  ( 7.365073210101819257, 1409.170254411169935, 196.0898092898519849 ) ) ;
#57621=CARTESIAN_POINT ( 'NONE',  ( 18.03147918629399982, 1424.668369977461907, 225.2961251598460137 ) ) ;
#57623=CARTESIAN_POINT ( 'NONE',  ( 11.86629849080000021, 1432.349867597399907, 149.9824147457980246 ) ) ;
#57624=AXIS2_PLACEMENT_3D ( 'NONE', #59911, #34682, #97345 ) ;
#57625=CARTESIAN_POINT ( 'NONE',  ( -3.768408416969716068, 1424.792709689574167, 185.8089501202686904 ) ) ;
#57627=CARTESIAN_POINT ( 'NONE',  ( -1.613214857710000061, 1426.534415841129885, 146.0564723340980038 ) ) ;
#57629=CARTESIAN_POINT ( 'NONE',  ( 18.94445953561779916, 1457.057774993960038, 226.8190492099999744 ) ) ;
#57631=CARTESIAN_POINT ( 'NONE',  ( -12.21221065219999957, 1435.118595363520171, 151.0037181377979891 ) ) ;
#57632=CARTESIAN_POINT ( 'NONE',  ( -8.040235583480250031E-10, 1467.681589800659822, 247.2443817431000070 ) ) ;
#57636=EDGE_CURVE ( 'NONE', #75664, #67655, #50045, .T. ) ;
#57644=CARTESIAN_POINT ( 'NONE',  ( 1.398757667669989990, 1408.961906081389998, 223.8083846529389973 ) ) ;
#57648=EDGE_CURVE ( 'NONE', #105791, #2110, #58953, .T. ) ;
#57649=ORIENTED_EDGE ( 'NONE', *, *, #72947, .T. ) ;
#57650=CARTESIAN_POINT ( 'NONE',  ( 25.15583052659999908, 1440.913060404589942, 217.2951523031179875 ) ) ;
#57651=CARTESIAN_POINT ( 'NONE',  ( -27.95183976699999917, 1508.132394783229984, 207.1324980664579982 ) ) ;
#57652=CARTESIAN_POINT ( 'NONE',  ( -3.536030895419999709, 1494.220633993530100, 181.5266943534980157 ) ) ;
#57654=CARTESIAN_POINT ( 'NONE',  ( -2.050401568548840370, 1419.506371351020107, 185.8591288081520077 ) ) ;
#57655=CARTESIAN_POINT ( 'NONE',  ( -22.53454638039999836, 1427.366758238030116, 231.7401250235980115 ) ) ;
#57656=CARTESIAN_POINT ( 'NONE',  ( -29.52155729519625638, 1509.963968224940345, 206.5808354184737254 ) ) ;
#57657=CARTESIAN_POINT ( 'NONE',  ( -16.66634793421699712, 1452.331058692820079, 146.5832199163500036 ) ) ;
#57658=CARTESIAN_POINT ( 'NONE',  ( 27.86016249569999914, 1451.782569911029896, 135.7658021331980081 ) ) ;
#57659=ORIENTED_EDGE ( 'NONE', *, *, #81221, .T. ) ;
#57660=DIRECTION ( 'NONE',  ( -1.000000000000000000, 0.000000000000000000, 0.000000000000000000 ) ) ;
#57661=CARTESIAN_POINT ( 'NONE',  ( 6.167425625146620593E-05, 1410.034441586050207, 269.8654409432670036 ) ) ;
#57662=CARTESIAN_POINT ( 'NONE',  ( 14.47776787345340033, 1421.911392191610048, 229.8149983301250074 ) ) ;
#57663=CARTESIAN_POINT ( 'NONE',  ( -17.73406580063780069, 1423.343214054229975, 226.1884525926029994 ) ) ;
#57664=ORIENTED_EDGE ( 'NONE', *, *, #35036, .F. ) ;
#57667=CARTESIAN_POINT ( 'NONE',  ( -23.03199747460190139, 1409.747173909519915, 209.2136270135010250 ) ) ;
#57668=CARTESIAN_POINT ( 'NONE',  ( -3.853475927979999938, 1424.036818987829975, 184.7819380313979991 ) ) ;
#57671=CARTESIAN_POINT ( 'NONE',  ( -22.69601814784311955, 1436.519530016244289, 142.0928716636521472 ) ) ;
#57674=CARTESIAN_POINT ( 'NONE',  ( 41.87330120854969806, 1455.441274400750217, 268.6302085777389834 ) ) ;
#57677=CARTESIAN_POINT ( 'NONE',  ( -0.01077498392880000058, 1420.442501270029879, 183.2891594270980136 ) ) ;
#57683=VERTEX_POINT ( 'NONE', #63290 ) ;
#57685=CARTESIAN_POINT ( 'NONE',  ( 26.81776656861889663, 1451.507007085510168, 136.0705416397969998 ) ) ;
#57689=CARTESIAN_POINT ( 'NONE',  ( 22.50003437009999629, 1409.698778901130254, 210.1517532643880202 ) ) ;
#57692=CARTESIAN_POINT ( 'NONE',  ( 2.084502382137720211, 1408.985852814510054, 186.9511601598070172 ) ) ;
#57693=CARTESIAN_POINT ( 'NONE',  ( -16.74159367139499821, 1413.343547140530063, 191.6682803937200106 ) ) ;
#57695=CARTESIAN_POINT ( 'NONE',  ( 2.499999999999999556, 1439.922972988470519, 170.5265280345823840 ) ) ;
#57698=FACE_OUTER_BOUND ( 'NONE', #47302, .T. ) ;
#57700=CARTESIAN_POINT ( 'NONE',  ( 9.145222436810001909, 1428.303966710129998, 214.3676144192479853 ) ) ;
#57703=CARTESIAN_POINT ( 'NONE',  ( 19.96892221239929910, 1487.423719650039857, 226.6548282969219770 ) ) ;
#57708=CARTESIAN_POINT ( 'NONE',  ( -36.99165393020000181, 1454.692295987030093, 268.3665355201979992 ) ) ;
#57710=CARTESIAN_POINT ( 'NONE',  ( -14.35456885730000032, 1416.827520116029973, 221.5785008559980156 ) ) ;
#57712=CARTESIAN_POINT ( 'NONE',  ( 2.220446049249999903E-15, 1468.063065667029832, 262.6648722463980334 ) ) ;
#57714=CARTESIAN_POINT ( 'NONE',  ( -11.60004869885203860, 1428.965959225140750, 137.0999999980979851 ) ) ;
#57716=CARTESIAN_POINT ( 'NONE',  ( -0.9786431567949999133, 1497.713060387329961, 231.7156151907979904 ) ) ;
#57720=CARTESIAN_POINT ( 'NONE',  ( -17.37381263529999842, 1410.444759175830086, 225.7669571254979815 ) ) ;
#57721=CARTESIAN_POINT ( 'NONE',  ( 20.79873180490000095, 1508.014473405230092, 190.2288953139980094 ) ) ;
#57723=CARTESIAN_POINT ( 'NONE',  ( -16.47946788473430146, 1409.488508717739933, 192.8607469751509882 ) ) ;
#57728=CARTESIAN_POINT ( 'NONE',  ( -0.9908514633770000302, 1414.913060387329779, 226.1016495930979886 ) ) ;
#57729=CARTESIAN_POINT ( 'NONE',  ( 0.2062144740239800211, 1459.480533006769974, 182.9753669427479963 ) ) ;
#57730=CARTESIAN_POINT ( 'NONE',  ( -3.043893720480000287, 1408.958240104829883, 223.4965448387980018 ) ) ;
#57732=CARTESIAN_POINT ( 'NONE',  ( -27.73716673060003757, 1444.324653571829003, 175.8274728504979976 ) ) ;
#57733=EDGE_CURVE ( 'NONE', #8806, #78872, #6873, .T. ) ;
#57734=CARTESIAN_POINT ( 'NONE',  ( -29.12047489647090259, 1509.926054659589909, 211.6780493401929846 ) ) ;
#57735=CARTESIAN_POINT ( 'NONE',  ( 13.50089340029999896, 1434.968964830010236, 149.1899395279980070 ) ) ;
#57736=CARTESIAN_POINT ( 'NONE',  ( -40.55649113755679736, 1439.640597909599819, 134.0999999981079895 ) ) ;
#57738=ORIENTED_EDGE ( 'NONE', *, *, #15109, .F. ) ;
#57744=EDGE_CURVE ( 'NONE', #3563, #66206, #56506, .T. ) ;
#57745=CARTESIAN_POINT ( 'NONE',  ( 39.76850916013371062, 1424.133492658783780, 269.1346536228787727 ) ) ;
#57748=CARTESIAN_POINT ( 'NONE',  ( 2.982880056399999980, 1425.995092949029868, 184.8396490932979930 ) ) ;
#57752=ORIENTED_EDGE ( 'NONE', *, *, #22062, .F. ) ;
#57753=CARTESIAN_POINT ( 'NONE',  ( -32.07183325839999810, 1451.793158448429949, 135.2032643032979990 ) ) ;
#57754=EDGE_CURVE ( 'NONE', #96120, #101013, #13833, .T. ) ;
#57756=CARTESIAN_POINT ( 'NONE',  ( -16.03272477472199853, 1410.858313914460041, 226.7018033498140142 ) ) ;
#57757=CARTESIAN_POINT ( 'NONE',  ( 4.026786250540000722, 1422.913060387330006, 172.2701767054979882 ) ) ;
#57764=CARTESIAN_POINT ( 'NONE',  ( 19.23182685600000141, 1409.584650579829940, 218.5516146816480045 ) ) ;
#57765=CARTESIAN_POINT ( 'NONE',  ( -2.184990249054419742, 1419.511891907180143, 185.9735355207210148 ) ) ;
#57766=CARTESIAN_POINT ( 'NONE',  ( -17.61956548329999706, 1424.285584503029895, 227.5004880819979860 ) ) ;
#57770=CARTESIAN_POINT ( 'NONE',  ( 25.17249022504864797, 1509.792581934430245, 193.9320483668153088 ) ) ;
#57771=CARTESIAN_POINT ( 'NONE',  ( -3.835404308833623155, 1396.046995657106436, 202.1011854665750036 ) ) ;
#57773=CARTESIAN_POINT ( 'NONE',  ( -10.31340658039999880, 1484.355420805929953, 185.0384118475980131 ) ) ;
#57774=ORIENTED_EDGE ( 'NONE', *, *, #99266, .F. ) ;
#57777=CARTESIAN_POINT ( 'NONE',  ( -4.238155808035029892, 1441.456966744900001, 163.0959397596959946 ) ) ;
#57782=CARTESIAN_POINT ( 'NONE',  ( 2.338461258401872023, 1507.140902121078398, 181.2734692029360986 ) ) ;
#57784=CARTESIAN_POINT ( 'NONE',  ( -10.82351740951083308, 1424.916036605491399, 144.6924919310794735 ) ) ;
#57785=CARTESIAN_POINT ( 'NONE',  ( 15.85937203857169742, 1410.570398459279886, 191.5484927328450055 ) ) ;
#57787=CARTESIAN_POINT ( 'NONE',  ( 36.33913412423270017, 1436.158733022410161, 135.8962114937069714 ) ) ;
#57792=DIRECTION ( 'NONE',  ( 0.000000000000000000, 1.000000000000000000, 0.000000000000000000 ) ) ;
#57795=CARTESIAN_POINT ( 'NONE',  ( -20.50000000000000000, 1442.773887286369927, 169.0968414572980123 ) ) ;
#57796=ORIENTED_EDGE ( 'NONE', *, *, #101731, .T. ) ;
#57798=FACE_OUTER_BOUND ( 'NONE', #33155, .T. ) ;
#57800=DIRECTION ( 'NONE',  ( 0.000000000000000000, -1.000000000000000000, 0.000000000000000000 ) ) ;
#57801=CARTESIAN_POINT ( 'NONE',  ( -3.344758901520000105, 1485.137791545830169, 183.2117113689980101 ) ) ;
#57804=CARTESIAN_POINT ( 'NONE',  ( 12.12358720160000125, 1442.555572165430021, 187.1519726473979972 ) ) ;
#57805=CARTESIAN_POINT ( 'NONE',  ( 38.81202641429280220, 1450.612734560829949, 135.3769929298369732 ) ) ;
#57807=CARTESIAN_POINT ( 'NONE',  ( 25.97440777459999950, 1440.634477712889975, 137.9745259500980126 ) ) ;
#57814=CARTESIAN_POINT ( 'NONE',  ( 37.43385382341080003, 1440.913060387330006, 264.2305522244909639 ) ) ;
#57815=CARTESIAN_POINT ( 'NONE',  ( -0.002187845253017860030, 1451.807059146780375, 154.0416503108188806 ) ) ;
#57816=VERTEX_POINT ( 'NONE', #23444 ) ;
#57817=CARTESIAN_POINT ( 'NONE',  ( -13.50890991390000018, 1415.048591094029916, 220.5416762897979766 ) ) ;
#57818=CARTESIAN_POINT ( 'NONE',  ( -10.96946876072200006, 1432.347663854339999, 151.7701362700559855 ) ) ;
#57821=CARTESIAN_POINT ( 'NONE',  ( 21.52851668485050141, 1409.719277583649955, 206.3559433526420150 ) ) ;
#57822=CARTESIAN_POINT ( 'NONE',  ( -10.80134480061119895, 1446.564900598669965, 153.0805715986579969 ) ) ;
#57823=CARTESIAN_POINT ( 'NONE',  ( -0.08880850522610000963, 1508.134875444430236, 180.6958675522979831 ) ) ;
#57824=CARTESIAN_POINT ( 'NONE',  ( -12.91333420139999966, 1434.774326854220135, 147.1504880069980175 ) ) ;
#57825=CARTESIAN_POINT ( 'NONE',  ( 25.92223975860549601, 1486.880094622480101, 206.2257269294839830 ) ) ;
#57826=CARTESIAN_POINT ( 'NONE',  ( 13.66288860260000071, 1461.271167413530065, 231.3349181382980078 ) ) ;
#57827=CARTESIAN_POINT ( 'NONE',  ( 0.000000000000000000, 1395.913060387330006, 215.6218459616979999 ) ) ;
#57831=CARTESIAN_POINT ( 'NONE',  ( -11.60004869885203682, -0.000000000000000000, 134.0999999980979851 ) ) ;
#57835=CARTESIAN_POINT ( 'NONE',  ( 18.47399033419999981, 1509.320896582529940, 187.7622940971980086 ) ) ;
#57838=ORIENTED_EDGE ( 'NONE', *, *, #108440, .F. ) ;
#57840=CARTESIAN_POINT ( 'NONE',  ( 7.330199424109999917, 1459.209061203830061, 213.1419610028279692 ) ) ;
#57842=CARTESIAN_POINT ( 'NONE',  ( -10.96944975070000083, 1432.346411317189904, 151.7703430070979778 ) ) ;
#57845=CARTESIAN_POINT ( 'NONE',  ( 27.02609455570868846, 1451.901622450774539, 135.4159887955381123 ) ) ;
#57847=CARTESIAN_POINT ( 'NONE',  ( 12.71634176899999957, 1445.234570782009996, 187.5504093200979980 ) ) ;
#57848=CARTESIAN_POINT ( 'NONE',  ( -20.08153501109999794, 1482.731068538430009, 227.1550935146979953 ) ) ;
#57850=DIRECTION ( 'NONE',  ( -0.7067625924915348357, 0.03085858548585030531, -0.7067774653711429433 ) ) ;
#57853=CARTESIAN_POINT ( 'NONE',  ( 6.971297644939999039, 1407.166808755230022, 269.6344828128980566 ) ) ;
#57854=CARTESIAN_POINT ( 'NONE',  ( 38.64592363763749461, 1443.862568456519739, 137.1880729169230051 ) ) ;
#57855=CARTESIAN_POINT ( 'NONE',  ( 19.76388419090000070, 1410.871606390429861, 196.8289662879980142 ) ) ;
#57856=CARTESIAN_POINT ( 'NONE',  ( 22.05653339442196881, 1430.082789188892320, 217.9551595525637993 ) ) ;
#57858=CARTESIAN_POINT ( 'NONE',  ( -5.992819232552545117, 1413.913060387330006, 198.1520639380683235 ) ) ;
#57859=CARTESIAN_POINT ( 'NONE',  ( 14.41568985214449938, 1457.296265504200164, 195.0854293786359790 ) ) ;
#57861=CARTESIAN_POINT ( 'NONE',  ( -1.554783491535979723, 1451.149365618095544, 183.7066068396813137 ) ) ;
#57863=CARTESIAN_POINT ( 'NONE',  ( 2.323033503200000460, 1449.800808688150028, 155.6080914323979982 ) ) ;
#57865=DIRECTION ( 'NONE',  ( -0.7074300732573280959, -0.02470400251971145017, 0.7063514732133270302 ) ) ;
#57867=CARTESIAN_POINT ( 'NONE',  ( -14.97660074589999901, 1430.165149044129976, 219.6133834379979817 ) ) ;
#57869=CARTESIAN_POINT ( 'NONE',  ( 3.691107917770000135, 1441.076188144620119, 158.1238300962979793 ) ) ;
#57870=CARTESIAN_POINT ( 'NONE',  ( -3.415211038299999835, 1475.467544519530065, 269.2902994287979936 ) ) ;
#57871=CARTESIAN_POINT ( 'NONE',  ( -4.222486080285369425, 1446.229412297520184, 167.6242796896230232 ) ) ;
#57875=CARTESIAN_POINT ( 'NONE',  ( 1.622533071855516207, 1508.277906825712080, 236.9750079835338852 ) ) ;
#57876=CARTESIAN_POINT ( 'NONE',  ( 16.71439081581360142, 1507.439214557219884, 193.5758153730089930 ) ) ;
#57878=CARTESIAN_POINT ( 'NONE',  ( -24.61074716929270068, 1457.438344121399950, 212.0276960468289928 ) ) ;
#57886=CARTESIAN_POINT ( 'NONE',  ( -12.90880567115966926, 1410.732768988275666, 227.8208098478615398 ) ) ;
#57887=CARTESIAN_POINT ( 'NONE',  ( 12.98226713004290112, 1414.913060387349788, 198.3280232619060257 ) ) ;
#57889=CARTESIAN_POINT ( 'NONE',  ( 10.79283000909999934, 1424.934955034829727, 142.7668711269979838 ) ) ;
#57894=CIRCLE ( 'NONE', #32841, 1.999994602259566712 ) ;
#57897=PLANE ( 'NONE',  #97640 ) ;
#57901=ADVANCED_FACE ( 'NONE', ( #91753 ), #88346, .T. ) ;
#57902=CARTESIAN_POINT ( 'NONE',  ( 20.25098345587720061, 1508.866247531380168, 229.1419343274569940 ) ) ;
#57906=CARTESIAN_POINT ( 'NONE',  ( 11.98438189353099936, 1433.653085447690046, 150.0614181868770061 ) ) ;
#57907=CARTESIAN_POINT ( 'NONE',  ( -10.55476389820000094, 1396.804446593130024, 216.5457841514580082 ) ) ;
#57908=CARTESIAN_POINT ( 'NONE',  ( -18.50902411670000447, 1409.559409753030195, 221.7674460617980117 ) ) ;
#57909=EDGE_LOOP ( 'NONE', ( #20322, #22199, #418, #83787, #63535, #24001 ) ) ;
#57910=CARTESIAN_POINT ( 'NONE',  ( -12.96794556044444846, 1444.895936098864695, 169.4262985252806004 ) ) ;
#57911=CARTESIAN_POINT ( 'NONE',  ( -28.15442719050000164, 1509.896234649429971, 200.8410286188979796 ) ) ;
#57912=CARTESIAN_POINT ( 'NONE',  ( 14.43289921540000087, 1509.539432541030010, 235.4218729623979982 ) ) ;
#57915=CARTESIAN_POINT ( 'NONE',  ( -13.96774116474500005, 1509.007359028199971, 183.7017197760899876 ) ) ;
#57916=EDGE_CURVE ( 'NONE', #85844, #94873, #94745, .T. ) ;
#57917=CARTESIAN_POINT ( 'NONE',  ( 16.38783789769999899, 1488.166949629130158, 188.7551421073980009 ) ) ;
#57918=CARTESIAN_POINT ( 'NONE',  ( -7.747669800249999739, 1416.518938591829965, 192.4898468467980024 ) ) ;
#57920=B_SPLINE_SURFACE_WITH_KNOTS ( 'NONE', 5, 1, ( 
 ( #97518, #19128 ),
 ( #53330, #11863 ),
 ( #89112, #87477 ),
 ( #35404, #10767 ),
 ( #27010, #18576 ),
 ( #60391, #94512 ),
 ( #110774, #25092 ),
 ( #50344, #51424 ),
 ( #67140, #76622 ),
 ( #77733, #77191 ),
 ( #17228, #17786 ),
 ( #42463, #34065 ),
 ( #102364, #85554 ),
 ( #494, #109675 ),
 ( #93963, #8851 ),
 ( #32951, #59840 ),
 ( #25649, #35169 ),
 ( #101238, #24538 ) ),
 .UNSPECIFIED., .F., .F., .F.,
 ( 6, 3, 3, 3, 3, 6 ),
 ( 2, 2 ),
 ( 14.02535798500000119, 16.90079360149999843, 18.14364336469999728, 21.12354018079999918, 24.53920724549999832, 25.26141522939999717 ),
 ( -0.02999077828059999729, 4.111335363550000288 ),
 .UNSPECIFIED. ) ;
#57921=CARTESIAN_POINT ( 'NONE',  ( 10.95578817948159944, 1396.295644941000091, 210.7241490613100154 ) ) ;
#57922=CARTESIAN_POINT ( 'NONE',  ( 1.383992982660000148, 1414.983773852829927, 191.7538276128979930 ) ) ;
#57923=CARTESIAN_POINT ( 'NONE',  ( 11.76383611999999879, 1431.900461285729989, 150.7976845351980160 ) ) ;
#57924=CARTESIAN_POINT ( 'NONE',  ( 41.15111437360000224, 1443.645439461449996, 136.9181462705980152 ) ) ;
#57926=CARTESIAN_POINT ( 'NONE',  ( 13.01599729242529868, 1434.868266845640164, 149.7301032413199948 ) ) ;
#57928=ORIENTED_EDGE ( 'NONE', *, *, #5896, .T. ) ;
#57929=CARTESIAN_POINT ( 'NONE',  ( -18.62426299532670271, 1497.950872138800150, 229.4157727875710009 ) ) ;
#57930=CARTESIAN_POINT ( 'NONE',  ( -8.257462432719998802, 1464.334752889730225, 233.3822669687979783 ) ) ;
#57937=CARTESIAN_POINT ( 'NONE',  ( 2.500000000000000000, 1448.261000471720081, 165.3796186243569935 ) ) ;
#57941=VERTEX_POINT ( 'NONE', #27737 ) ;
#57944=CARTESIAN_POINT ( 'NONE',  ( -16.66453347706279686, 1412.909409113607126, 269.3720812842371970 ) ) ;
#57945=CARTESIAN_POINT ( 'NONE',  ( -1.647892026280000088, 1409.908608567930060, 232.8799286543980145 ) ) ;
#57946=CARTESIAN_POINT ( 'NONE',  ( -0.1687944357496000136, 1416.535698381769862, 227.3595857086420153 ) ) ;
#57948=CARTESIAN_POINT ( 'NONE',  ( 2.500000000000000000, 1431.135902250849995, 157.4660731311979873 ) ) ;
#57949=CARTESIAN_POINT ( 'NONE',  ( -29.77671877493460073, 1440.913060386769985, 237.6287523421349874 ) ) ;
#57951=CARTESIAN_POINT ( 'NONE',  ( -0.3222280624858790410, 1466.023156909590170, 235.8295839634860158 ) ) ;
#57952=CARTESIAN_POINT ( 'NONE',  ( 5.377271148049999283, 1408.165475900730144, 270.2871877487980328 ) ) ;
#57954=CARTESIAN_POINT ( 'NONE',  ( 22.81920077950000092, 1409.709825997729922, 209.2267294936970075 ) ) ;
#57955=CARTESIAN_POINT ( 'NONE',  ( -21.47210458610000217, 1509.724521920430107, 188.4228462942980116 ) ) ;
#57961=CARTESIAN_POINT ( 'NONE',  ( -15.24860744008350544, 1486.073951134501840, 186.4853819756072255 ) ) ;
#57963=ORIENTED_EDGE ( 'NONE', *, *, #39113, .F. ) ;
#57966=CARTESIAN_POINT ( 'NONE',  ( 17.19449137966054053, 1410.877584405873222, 226.0689879175218948 ) ) ;
#57968=CARTESIAN_POINT ( 'NONE',  ( -1.801950444790000105, 1417.382180821630072, 235.5933117588980110 ) ) ;
#57975=CARTESIAN_POINT ( 'NONE',  ( -27.01380866140000236, 1450.681584507220123, 136.4483241423979791 ) ) ;
#57976=CARTESIAN_POINT ( 'NONE',  ( 10.23156695028191621, 1422.701445000401236, 137.1234503073714563 ) ) ;
#57977=ORIENTED_EDGE ( 'NONE', *, *, #61267, .T. ) ;
#57982=CARTESIAN_POINT ( 'NONE',  ( 19.18154864119999914, 1456.154625754229983, 224.9761355071979949 ) ) ;
#57983=CARTESIAN_POINT ( 'NONE',  ( 7.743430599797714642, 1438.376054508304833, 153.8132518338354657 ) ) ;
#57985=CARTESIAN_POINT ( 'NONE',  ( -16.06428792994629973, 1414.913060387329779, 209.3174441339999987 ) ) ;
#57986=CARTESIAN_POINT ( 'NONE',  ( 4.219439013950669448, 1441.595895969210005, 182.7715284958480026 ) ) ;
#57987=B_SPLINE_CURVE_WITH_KNOTS ( 'NONE', 5,
 ( #9891, #79319, #60882, #61988, #51911, #27250, #61431, #53582, #87729 ),
 .UNSPECIFIED., .F., .F.,
 ( 6, 3, 6 ),
 ( 0.000000000000000000, 0.4107976024515093694, 1.000000000000000000 ),
 .UNSPECIFIED. ) ;
#57988=CARTESIAN_POINT ( 'NONE',  ( 27.07880669207580127, 1435.598858538910008, 136.1558489245400096 ) ) ;
#57989=CARTESIAN_POINT ( 'NONE',  ( 39.23819738392720069, 1447.383198997459886, 136.5851928137900018 ) ) ;
#57990=CARTESIAN_POINT ( 'NONE',  ( -21.46437004979999941, 1429.716328564329842, 220.0955847048980161 ) ) ;
#57991=CARTESIAN_POINT ( 'NONE',  ( -10.80059289547383194, 1474.148535085230606, 269.6142578605208087 ) ) ;
#57994=CARTESIAN_POINT ( 'NONE',  ( -17.00646468379999732, 1415.800410784929909, 226.5733319496979732 ) ) ;
#57996=CARTESIAN_POINT ( 'NONE',  ( -13.57486036570845833, 1469.792362884156773, 269.3590160498212640 ) ) ;
#57997=ORIENTED_EDGE ( 'NONE', *, *, #76878, .F. ) ;
#57999=CARTESIAN_POINT ( 'NONE',  ( -32.46047264654747266, 1416.888327440118019, 269.3060940481729517 ) ) ;
#58001=CARTESIAN_POINT ( 'NONE',  ( -4.360582346120001063, 1431.113060387329824, 227.9437648745980027 ) ) ;
#58002=CARTESIAN_POINT ( 'NONE',  ( -15.31264328659269403, 1451.565714120024722, 222.7578395244654814 ) ) ;
#58003=CARTESIAN_POINT ( 'NONE',  ( -13.27459202670609173, 1444.621175491612121, 186.6925910478026367 ) ) ;
#58007=CARTESIAN_POINT ( 'NONE',  ( -7.863053483428857682, 1451.394019542978185, 152.9855632054714931 ) ) ;
#58008=ADVANCED_FACE ( 'NONE', ( #64123 ), #54404, .T. ) ;
#58011=CARTESIAN_POINT ( 'NONE',  ( -14.06591346399999942, 1410.775981576729919, 226.9656985104979867 ) ) ;
#58012=ORIENTED_EDGE ( 'NONE', *, *, #3790, .T. ) ;
#58013=CARTESIAN_POINT ( 'NONE',  ( 0.5081859945959991132, 1415.431750870129918, 191.3337547248510191 ) ) ;
#58014=CARTESIAN_POINT ( 'NONE',  ( 21.07223471314816265, 1508.254227089592632, 226.1111686167440951 ) ) ;
#58018=CARTESIAN_POINT ( 'NONE',  ( 16.38929703815969674, 1414.913060387399810, 210.1493163092779923 ) ) ;
#58021=CARTESIAN_POINT ( 'NONE',  ( -3.776117134630000205, 1460.308496303429820, 216.2848420587179987 ) ) ;
#58022=CARTESIAN_POINT ( 'NONE',  ( -20.49650080320000001, 1506.525074349130136, 189.7974850576979975 ) ) ;
#58023=CARTESIAN_POINT ( 'NONE',  ( -10.99125927559999916, 1433.250798529490112, 151.7641638922980007 ) ) ;
#58025=CARTESIAN_POINT ( 'NONE',  ( 16.19492434978379691, 1409.478599607480191, 224.1775087544979783 ) ) ;
#58027=CARTESIAN_POINT ( 'NONE',  ( -24.25757607999999976, 1438.852108944180145, 211.3728147305379821 ) ) ;
#58029=CARTESIAN_POINT ( 'NONE',  ( 2.480548060760000340, 1449.812485612440241, 182.9983066197980008 ) ) ;
#58031=CARTESIAN_POINT ( 'NONE',  ( -24.38581948224031137, 1509.879308922522114, 226.6760032255506871 ) ) ;
#58033=ORIENTED_EDGE ( 'NONE', *, *, #69999, .F. ) ;
#58034=EDGE_LOOP ( 'NONE', ( #141, #4908, #7387, #104600 ) ) ;
#58035=CARTESIAN_POINT ( 'NONE',  ( -11.81201955091739997, 1428.846405886920138, 148.7528568703669976 ) ) ;
#58037=CARTESIAN_POINT ( 'NONE',  ( -4.903602370519999809, 1472.418623804529943, 270.3706473056980144 ) ) ;
#58041=CARTESIAN_POINT ( 'NONE',  ( 41.19002696412830034, 1446.271008772989944, 136.2099985660260018 ) ) ;
#58042=CARTESIAN_POINT ( 'NONE',  ( 19.60393592299999810, 1475.513060387329915, 201.4085066119280043 ) ) ;
#58045=B_SPLINE_CURVE_WITH_KNOTS ( 'NONE', 5,
 ( #74297, #47432, #98914, #41225, #81555, #39573, #92176, #13242, #24404 ),
 .UNSPECIFIED., .F., .F.,
 ( 6, 3, 6 ),
 ( 0.7655572723410000169, 2.316155491850000026, 3.835724788409999420 ),
 .UNSPECIFIED. ) ;
#58048=CARTESIAN_POINT ( 'NONE',  ( -43.54088588253560488, 1430.059707464080248, 268.8270446202420203 ) ) ;
#58049=ORIENTED_EDGE ( 'NONE', *, *, #22971, .F. ) ;
#58051=VECTOR ( 'NONE', #73381, 1000.000000000000000 ) ;
#58059=CARTESIAN_POINT ( 'NONE',  ( -14.41619594183999986, 1509.538862653740125, 182.8126525573280219 ) ) ;
#58060=CARTESIAN_POINT ( 'NONE',  ( -2.840701075410000165, 1470.463058086329966, 183.9230798073980111 ) ) ;
#58061=CIRCLE ( 'NONE', #84801, 5.133097426430088817 ) ;
#58062=CARTESIAN_POINT ( 'NONE',  ( -17.28556280980830095, 1479.740375246909935, 228.8535606757079961 ) ) ;
#58063=B_SPLINE_SURFACE_WITH_KNOTS ( 'NONE', 2, 5, ( 
 ( #69858, #44088, #76569, #87185, #93908, #59243 ),
 ( #34012, #51934, #34566, #52494, #17733, #18301 ),
 ( #25041, #445, #86623, #78226, #85502, #103408 ) ),
 .UNSPECIFIED., .F., .F., .F.,
 ( 3, 3 ),
 ( 6, 6 ),
 ( 1.399803019419999961, 2.016961153140000018 ),
 ( 0.000000000000000000, 1.000000000000000000 ),
 .UNSPECIFIED. ) ;
#58067=B_SPLINE_SURFACE_WITH_KNOTS ( 'NONE', 5, 1, ( 
 ( #63581, #11501 ),
 ( #97151, #64677 ),
 ( #97698, #106640 ),
 ( #30488, #88758 ),
 ( #45677, #21513 ),
 ( #38877, #98243 ),
 ( #29931, #105564 ),
 ( #79815, #55173 ),
 ( #64122, #37249 ) ),
 .UNSPECIFIED., .F., .F., .F.,
 ( 6, 3, 6 ),
 ( 2, 2 ),
 ( 2.977480884639999825, 6.317148707589999468, 12.84608988247099859 ),
 ( -13.58503197309999955, -1.277641458209999969 ),
 .UNSPECIFIED. ) ;
#58070=CARTESIAN_POINT ( 'NONE',  ( -42.85029935319199978, 1436.020988110130020, 270.2009494392980287 ) ) ;
#58078=CARTESIAN_POINT ( 'NONE',  ( -12.84239665067440050, 1435.935719077439899, 150.8114796122480072 ) ) ;
#58079=CARTESIAN_POINT ( 'NONE',  ( -24.28687749879999913, 1442.594715683929962, 211.8376410442379836 ) ) ;
#58082=CARTESIAN_POINT ( 'NONE',  ( -2.234865362860189553, 1484.253666364170158, 183.1161028472960197 ) ) ;
#58088=CARTESIAN_POINT ( 'NONE',  ( -33.91369120209999721, 1451.728768194229815, 134.0999999980979851 ) ) ;
#58091=CARTESIAN_POINT ( 'NONE',  ( -18.92604478490211406, 1457.990945249578544, 226.9998699462371405 ) ) ;
#58094=CARTESIAN_POINT ( 'NONE',  ( 12.87368581495110043, 1434.742583859479964, 149.5707935314029839 ) ) ;
#58095=CARTESIAN_POINT ( 'NONE',  ( 4.454121045402620105, 1468.999327738519924, 234.0578715337849758 ) ) ;
#58098=CARTESIAN_POINT ( 'NONE',  ( 24.32432927030000158, 1452.063639817629792, 136.1371466596980042 ) ) ;
#58100=CARTESIAN_POINT ( 'NONE',  ( 2.404122373123565914, 1426.711430350427463, 142.7750368341233695 ) ) ;
#58101=CARTESIAN_POINT ( 'NONE',  ( 4.269138570313380399, 1441.141876082800081, 158.1427116847730190 ) ) ;
#58107=CARTESIAN_POINT ( 'NONE',  ( -17.97818486826909989, 1488.931524437730104, 229.1373185541280009 ) ) ;
#58109=CARTESIAN_POINT ( 'NONE',  ( 2.191804311359999868, 1420.975114716630060, 184.3756173852979714 ) ) ;
#58116=CARTESIAN_POINT ( 'NONE',  ( 17.67081254923106926, 1423.277421049964914, 226.2500432428864485 ) ) ;
#58119=CARTESIAN_POINT ( 'NONE',  ( 38.64164465084230216, 1440.913060378469936, 257.2879587844699927 ) ) ;
#58121=CARTESIAN_POINT ( 'NONE',  ( 14.31472612081786799, 1507.539056556547848, 186.0170524603447859 ) ) ;
#58126=CARTESIAN_POINT ( 'NONE',  ( -19.51279205535366046, 1485.520671005373060, 190.0467292662184491 ) ) ;
#58129=CARTESIAN_POINT ( 'NONE',  ( 1.400808530693328446, 1507.374882240569832, 236.8304372390393837 ) ) ;
#58131=DIRECTION ( 'NONE',  ( 0.06436433998262545975, 0.7055452152162795532, 0.7057359145062795935 ) ) ;
#58136=CARTESIAN_POINT ( 'NONE',  ( -13.18252224579999954, 1434.994542537020152, 194.3559101920980083 ) ) ;
#58137=B_SPLINE_CURVE_WITH_KNOTS ( 'NONE', 3,
 ( #101999, #17427, #84655, #43772, #9060, #1230, #25285, #51078, #68442, #94157, #84108, #93596, #110418, #7952, #34260, #60596, #76823, #75728, #8494, #33152, #95279, #16873, #16330, #94717, #17993, #85205, #102545, #25838, #41573, #85762, #103102, #34812, #42667, #138, #60039, #51625, #77923, #43231, #24729, #35367, #50530, #77379, #681, #52188, #42121, #69554, #68999, #76269, #26403, #86318, #33697, #109873, #9602, #103674 ),
 .UNSPECIFIED., .F., .F.,
 ( 4, 2, 2, 2, 2, 2, 1, 2, 2, 2, 2, 1, 2, 2, 2, 1, 1, 2, 2, 2, 1, 1, 2, 2, 2, 2, 1, 1, 2, 2, 4 ),
 ( 0.000000000000000000, 0.03125000000116372884, 0.04687500000159226105, 0.05468750000166328062, 0.06250000000173429326, 0.09375000000235139686, 0.1093750000026626479, 0.1171875000029593689, 0.1250000000032560898, 0.1875000000045450310, 0.2187500000051895155, 0.2343750000053846372, 0.2421875000053570204, 0.2500000000053294036, 0.3125000000048098747, 0.3437500000045571324, 0.3593750000044307336, 0.3671875000043675619, 0.3750000000043043347, 0.4375000000043617887, 0.4687500000045123350, 0.4843750000045782822, 0.4921875000046112558, 0.5000000000046441739, 0.6250000000040655257, 0.6875000000037638781, 0.7187500000035280667, 0.7343750000034996450, 0.7421875000034117154, 0.7500000000033237857, 1.000000000000000000 ),
 .UNSPECIFIED. ) ;
#58143=B_SPLINE_SURFACE_WITH_KNOTS ( 'NONE', 4, 5, ( 
 ( #99193, #107617, #4615, #64541, #13533, #65078 ),
 ( #72926, #107065, #47719, #31449, #83499, #32006 ),
 ( #81850, #6254, #5153, #22473, #6795, #66195 ),
 ( #109282, #39310, #32566, #56673, #89711, #12989 ),
 ( #85156, #58324, #33101, #85708, #7897, #33641 ) ),
 .UNSPECIFIED., .F., .F., .F.,
 ( 5, 5 ),
 ( 6, 6 ),
 ( 17.21936457409999832, 17.22979334940000129 ),
 ( 0.000000000000000000, 2.175007696500000254 ),
 .UNSPECIFIED. ) ;
#58145=CARTESIAN_POINT ( 'NONE',  ( 19.85783298583229950, 1508.594920224220004, 229.4585935219059820 ) ) ;
#58154=DIRECTION ( 'NONE',  ( 0.7071067811870476172, 0.000000000000000000, -0.7071067811860475283 ) ) ;
#58155=DIRECTION ( 'NONE',  ( -9.551066690030985733E-08, -1.946171181391529080E-07, 0.9999999999999764633 ) ) ;
#58158=CARTESIAN_POINT ( 'NONE',  ( 18.52279787119999810, 1425.631473512029970, 225.3995475816979877 ) ) ;
#58161=CARTESIAN_POINT ( 'NONE',  ( -4.220880940900710421, 1441.618787263769718, 168.7222756990960022 ) ) ;
#58162=CARTESIAN_POINT ( 'NONE',  ( 0.000000000000000000, 1412.913060387329779, 209.1218459616979999 ) ) ;
#58166=CARTESIAN_POINT ( 'NONE',  ( 19.27358882249560068, 1456.231984985270174, 227.7371637781419906 ) ) ;
#58168=CARTESIAN_POINT ( 'NONE',  ( -8.278637686411969791E-09, 1472.684511341680036, 260.5494539826829623 ) ) ;
#58169=CARTESIAN_POINT ( 'NONE',  ( 20.36084529355510142, 1436.440394646498589, 145.0484382341195726 ) ) ;
#58173=CARTESIAN_POINT ( 'NONE',  ( -1.215107678660000134, 1486.521536555729881, 182.1360231587979968 ) ) ;
#58180=B_SPLINE_SURFACE_WITH_KNOTS ( 'NONE', 5, 5, ( 
 ( #38091, #54912, #97449, #105300, #36984, #80094 ),
 ( #70629, #28034, #47060, #88506, #19060, #3414 ),
 ( #11789, #81184, #62791, #96906, #53265, #89038 ),
 ( #4500, #95793, #53829, #105862, #37543, #70083 ),
 ( #71745, #87404, #29685, #27480, #3964, #12326 ),
 ( #10698, #29141, #63329, #61670, #71178, #54374 ) ),
 .UNSPECIFIED., .F., .F., .F.,
 ( 6, 6 ),
 ( 6, 6 ),
 ( 16.36816738399999949, 93.94674272650000546 ),
 ( -2.775557561569999727E-17, 1.000000000000000000 ),
 .UNSPECIFIED. ) ;
#58181=CARTESIAN_POINT ( 'NONE',  ( -1.546867746862319981, 1416.839692133689823, 228.0214409764060122 ) ) ;
#58184=CARTESIAN_POINT ( 'NONE',  ( 11.18741891859999882, 1423.006079699629936, 217.1793481124879861 ) ) ;
#58185=CARTESIAN_POINT ( 'NONE',  ( -1.502588279119999815, 1469.871880491130014, 182.3802797567980178 ) ) ;
#58188=CARTESIAN_POINT ( 'NONE',  ( 3.156166260290000025, 1466.544008048530031, 236.1241471695980181 ) ) ;
#58189=CARTESIAN_POINT ( 'NONE',  ( -29.75012120250000081, 1509.993914124430148, 208.5595671623779879 ) ) ;
#58190=CARTESIAN_POINT ( 'NONE',  ( -13.86903295495070054, 1452.428743084420148, 148.6123537208110008 ) ) ;
#58191=CARTESIAN_POINT ( 'NONE',  ( 15.05358515032119904, 1410.831827804430077, 191.5175411757069810 ) ) ;
#58192=EDGE_LOOP ( 'NONE', ( #3277, #57963, #42779, #70608 ) ) ;
#58193=CARTESIAN_POINT ( 'NONE',  ( -2.500000000000000000, 1421.745358796729988, 151.9633565684980283 ) ) ;
#58194=CARTESIAN_POINT ( 'NONE',  ( -0.6164045617451590076, 1407.928388523590002, 270.2926945153609495 ) ) ;
#58195=CARTESIAN_POINT ( 'NONE',  ( -0.05082476190679999922, 1508.992422786230009, 238.9842641244979973 ) ) ;
#58196=CARTESIAN_POINT ( 'NONE',  ( 16.99532478070279851, 1414.913372219064513, 210.5807211179420619 ) ) ;
#58200=CARTESIAN_POINT ( 'NONE',  ( -23.96638063676619979, 1410.422153605740050, 209.1360332124949934 ) ) ;
#58202=CARTESIAN_POINT ( 'NONE',  ( 16.19492434978379691, 1409.478599607480191, 224.1775087544979783 ) ) ;
#58203=CARTESIAN_POINT ( 'NONE',  ( -45.67177343128329881, 1440.913044206929953, 266.1885934837860077 ) ) ;
#58204=CARTESIAN_POINT ( 'NONE',  ( -0.2366988889530000084, 1507.644349193429889, 237.3561800022980037 ) ) ;
#58207=EDGE_CURVE ( 'NONE', #110792, #101763, #99313, .T. ) ;
#58208=CARTESIAN_POINT ( 'NONE',  ( 41.99034683523260014, 1455.513645117400074, 268.3446858974320435 ) ) ;
#58212=CARTESIAN_POINT ( 'NONE',  ( 0.03978530575449999718, 1419.130000249829891, 184.6452573654979972 ) ) ;
#58214=EDGE_LOOP ( 'NONE', ( #34815, #46541, #28308, #88579, #18989, #45177 ) ) ;
#58219=ORIENTED_EDGE ( 'NONE', *, *, #6520, .F. ) ;
#58222=CARTESIAN_POINT ( 'NONE',  ( 27.02053382135309789, 1451.952557960830063, 135.1688879843840141 ) ) ;
#58229=CARTESIAN_POINT ( 'NONE',  ( 11.26174377530239923, 1409.306329145770178, 191.0634772139260065 ) ) ;
#58230=CARTESIAN_POINT ( 'NONE',  ( -12.89608512423069975, 1434.724840024559853, 149.2206170422699927 ) ) ;
#58231=CARTESIAN_POINT ( 'NONE',  ( -17.73406580063780069, 1423.343214054229975, 226.1884525926029994 ) ) ;
#58232=CARTESIAN_POINT ( 'NONE',  ( 2.571344636303355635, 1440.211256060247251, 170.5281974707060044 ) ) ;
#58234=CARTESIAN_POINT ( 'NONE',  ( 11.86716023049999968, 1432.353341358199941, 147.6509521729980179 ) ) ;
#58235=ORIENTED_EDGE ( 'NONE', *, *, #69304, .T. ) ;
#58236=CARTESIAN_POINT ( 'NONE',  ( 12.81185530964379815, 1416.835419214280137, 221.9980326694370092 ) ) ;
#58237=DIRECTION ( 'NONE',  ( 0.000000000000000000, 0.000000000000000000, -1.000000000000000000 ) ) ;
#58238=CARTESIAN_POINT ( 'NONE',  ( 17.01308443848121499, 1414.913060595379648, 210.6742099983445087 ) ) ;
#58241=ADVANCED_FACE ( 'NONE', ( #9138 ), #46495, .F. ) ;
#58245=CARTESIAN_POINT ( 'NONE',  ( -36.06124927020000115, 1445.049634742420039, 262.6648722463980334 ) ) ;
#58246=CARTESIAN_POINT ( 'NONE',  ( -21.94594868458499093, 1509.533995021516603, 191.4017675758697123 ) ) ;
#58248=CARTESIAN_POINT ( 'NONE',  ( 28.05448517229999794, 1461.575973716330054, 265.6112250856980381 ) ) ;
#58251=CIRCLE ( 'NONE', #24251, 1.500000000000001332 ) ;
#58252=CARTESIAN_POINT ( 'NONE',  ( -16.18976011259663750, 1409.478419268353264, 194.8164317614535150 ) ) ;
#58253=CARTESIAN_POINT ( 'NONE',  ( -0.9796450454589999968, 1519.913060387329779, 232.6858900125980085 ) ) ;
#58256=CARTESIAN_POINT ( 'NONE',  ( -18.23438631919999864, 1486.008731762530033, 188.8346238057980031 ) ) ;
#58259=CARTESIAN_POINT ( 'NONE',  ( 17.76091713730000166, 1410.905089306629861, 223.3054222800980142 ) ) ;
#58260=CARTESIAN_POINT ( 'NONE',  ( -25.58458546029999781, 1449.894445106999910, 137.3532228530980035 ) ) ;
#58261=CARTESIAN_POINT ( 'NONE',  ( -17.06940528265129942, 1409.674914835549998, 193.4350317209980119 ) ) ;
#58262=CARTESIAN_POINT ( 'NONE',  ( 8.106578671807320281E-07, 1407.561928582239943, 196.0178922782889686 ) ) ;
#58265=CARTESIAN_POINT ( 'NONE',  ( -3.747719220470000057, 1415.426091369430196, 226.7846717995979873 ) ) ;
#58266=CARTESIAN_POINT ( 'NONE',  ( 0.1694144171801959808, 1480.673780128910039, 182.0654477247749696 ) ) ;
#58267=CARTESIAN_POINT ( 'NONE',  ( -4.500000000000000000, 1423.874532569730036, 167.3087045231979744 ) ) ;
#58270=CARTESIAN_POINT ( 'NONE',  ( 11.94104774480000053, 1433.615498876629999, 149.8850687855980084 ) ) ;
#58271=CARTESIAN_POINT ( 'NONE',  ( -40.94560254916699193, 1440.384112706839915, 134.0999999980729740 ) ) ;
#58275=LINE ( 'NONE', #22984, #4580 ) ;
#58280=CARTESIAN_POINT ( 'NONE',  ( 22.15551762850000017, 1489.466917450329902, 210.2377471049379949 ) ) ;
#58287=CARTESIAN_POINT ( 'NONE',  ( -29.81974100089999880, 1451.010966676529733, 136.2919626754980129 ) ) ;
#58288=CARTESIAN_POINT ( 'NONE',  ( -17.02002156968800151, 1410.733189543489971, 226.2282921672789939 ) ) ;
#58289=AXIS2_PLACEMENT_3D ( 'NONE', #14439, #97898, #48636 ) ;
#58290=DIRECTION ( 'NONE',  ( 0.000000000000000000, -1.000000000000000000, 0.000000000000000000 ) ) ;
#58295=CARTESIAN_POINT ( 'NONE',  ( -17.56882915975198856, 1410.890595540249024, 225.4874358264362399 ) ) ;
#58297=CARTESIAN_POINT ( 'NONE',  ( -0.08394227893480489533, 1419.987834470179905, 183.9790430942110220 ) ) ;
#58298=CARTESIAN_POINT ( 'NONE',  ( 35.24315337100163248, 1457.507325202675929, 269.5348779185313219 ) ) ;
#58300=CARTESIAN_POINT ( 'NONE',  ( -16.14423341240000198, 1422.196820606129904, 227.3644137178979747 ) ) ;
#58304=CARTESIAN_POINT ( 'NONE',  ( 3.294994957250000134, 1408.913060387329779, 226.6118641217979928 ) ) ;
#58306=ADVANCED_FACE ( 'NONE', ( #104852 ), #90293, .T. ) ;
#58308=CARTESIAN_POINT ( 'NONE',  ( 2.500000000000000000, 1448.191388957269965, 168.9995349768979906 ) ) ;
#58311=CARTESIAN_POINT ( 'NONE',  ( -4.231842431855520559, 1441.513933367780055, 164.4206257021209865 ) ) ;
#58313=ORIENTED_EDGE ( 'NONE', *, *, #49553, .T. ) ;
#58319=CARTESIAN_POINT ( 'NONE',  ( -11.63658677818990128, 1425.864905157940257, 144.1610764294569833 ) ) ;
#58320=CARTESIAN_POINT ( 'NONE',  ( 16.36854146560279943, 1410.124658228839962, 191.8480414016150064 ) ) ;
#58322=CARTESIAN_POINT ( 'NONE',  ( 34.91588500242689719, 1437.049151938289924, 136.5304996461299822 ) ) ;
#58323=EDGE_CURVE ( 'NONE', #94600, #102101, #57303, .T. ) ;
#58324=CARTESIAN_POINT ( 'NONE',  ( -11.73643181629999965, 1426.280401702830204, 144.1638243106980042 ) ) ;
#58325=CARTESIAN_POINT ( 'NONE',  ( -0.0001187281342228439996, 1508.967929526819944, 179.3767679645770272 ) ) ;
#58326=CARTESIAN_POINT ( 'NONE',  ( 17.10224595388506330, 1460.321307548461164, 228.6740676894672788 ) ) ;
#58328=CARTESIAN_POINT ( 'NONE',  ( 38.20286890328719664, 1450.309401038089845, 134.0999999984079807 ) ) ;
#58329=CARTESIAN_POINT ( 'NONE',  ( -40.27308906366239682, 1443.612067134240078, 137.1163379626329970 ) ) ;
#58332=DIRECTION ( 'NONE',  ( -0.09872117914509953573, 0.9946471739456684835, 0.03051439250741381365 ) ) ;
#58334=ORIENTED_EDGE ( 'NONE', *, *, #78287, .T. ) ;
#58335=CARTESIAN_POINT ( 'NONE',  ( -29.47787601289847714, 1509.952111658624290, 211.1326834024595200 ) ) ;
#58336=CARTESIAN_POINT ( 'NONE',  ( -17.06941237829999736, 1409.674943312830010, 194.0661809782980072 ) ) ;
#58337=B_SPLINE_CURVE_WITH_KNOTS ( 'NONE', 5,
 ( #99153, #92835, #67114, #34036, #34588, #102333 ),
 .UNSPECIFIED., .F., .F.,
 ( 6, 6 ),
 ( 0.000000000000000000, 1.000000000000000000 ),
 .UNSPECIFIED. ) ;
#58341=CARTESIAN_POINT ( 'NONE',  ( -27.89972997509999786, 1508.077281474930032, 206.8466243103179920 ) ) ;
#58342=CARTESIAN_POINT ( 'NONE',  ( 42.60628463920169651, 1443.705283414120004, 135.0591082134169767 ) ) ;
#58344=EDGE_CURVE ( 'NONE', #45409, #77352, #20380, .T. ) ;
#58345=CARTESIAN_POINT ( 'NONE',  ( 26.06817282160000104, 1439.608707811800059, 137.5105934946979858 ) ) ;
#58352=CARTESIAN_POINT ( 'NONE',  ( 11.82617426117190007, 1429.667056798789872, 149.2970047124300095 ) ) ;
#58356=CARTESIAN_POINT ( 'NONE',  ( -14.34198504589999956, 1416.067629296030191, 221.2727144154980010 ) ) ;
#58357=CARTESIAN_POINT ( 'NONE',  ( -11.30564195107439929, 1432.342987153669810, 151.4629878985130063 ) ) ;
#58360=CARTESIAN_POINT ( 'NONE',  ( 21.99869784864110400, 1409.975627104619889, 206.2846292323520174 ) ) ;
#58365=CARTESIAN_POINT ( 'NONE',  ( 23.73948244347349856, 1437.917305470170049, 206.2095067639299941 ) ) ;
#58367=CARTESIAN_POINT ( 'NONE',  ( 13.85688183060000078, 1460.822580857430012, 232.2031414462979910 ) ) ;
#58372=ADVANCED_FACE ( 'NONE', ( #109806 ), #92138, .F. ) ;
#58374=CARTESIAN_POINT ( 'NONE',  ( -0.2726138066919999714, 1487.235664587629799, 230.5521328613980074 ) ) ;
#58378=CARTESIAN_POINT ( 'NONE',  ( -11.60004869885776024, 1425.683027346956351, 138.3963214575541940 ) ) ;
#58382=CARTESIAN_POINT ( 'NONE',  ( -15.54603058869099996, 1507.439214557209880, 192.4074551458910207 ) ) ;
#58383=CARTESIAN_POINT ( 'NONE',  ( -11.81867802130000022, 1429.211286938129888, 149.0416137968979911 ) ) ;
#58384=CARTESIAN_POINT ( 'NONE',  ( 19.02876048740180082, 1456.918022623920024, 225.5897448336330058 ) ) ;
#58386=DIRECTION ( 'NONE',  ( 0.5781790699150771706, 0.04201035868947775725, 0.8148276461159855710 ) ) ;
#58388=EDGE_CURVE ( 'NONE', #86873, #71251, #42051, .T. ) ;
#58389=CARTESIAN_POINT ( 'NONE',  ( -2.471608048749999842, 1438.194204504490017, 150.4833623973980252 ) ) ;
#58390=CARTESIAN_POINT ( 'NONE',  ( -21.04359474530000185, 1482.728143256829981, 225.6449476673980143 ) ) ;
#58395=CARTESIAN_POINT ( 'NONE',  ( 3.767309702620000422, 1405.959571974130085, 267.2290117651980381 ) ) ;
#58397=CARTESIAN_POINT ( 'NONE',  ( -0.001550886560859999954, 1408.913006230129895, 186.0211967747979998 ) ) ;
#58398=CARTESIAN_POINT ( 'NONE',  ( 20.00430653580000140, 1449.729862604200207, 193.6333489802979955 ) ) ;
#58400=CARTESIAN_POINT ( 'NONE',  ( 7.527653235111040786, 1506.538134868789029, 229.8708666564015175 ) ) ;
#58402=CARTESIAN_POINT ( 'NONE',  ( -0.5133638609672289688, 1410.311096993930050, 233.1717005261690190 ) ) ;
#58403=CARTESIAN_POINT ( 'NONE',  ( -18.51604897466450694, 1457.427690017132363, 227.8249311439416829 ) ) ;
#58405=CARTESIAN_POINT ( 'NONE',  ( -14.45727104390000051, 1444.967096565130078, 188.7843282767979929 ) ) ;
#58408=CARTESIAN_POINT ( 'NONE',  ( 0.4918993947909917619, 1407.650947846033205, 270.1377426664976156 ) ) ;
#58410=CARTESIAN_POINT ( 'NONE',  ( 1.463365724432849957, 1492.705009941090111, 181.7417394025019917 ) ) ;
#58414=CARTESIAN_POINT ( 'NONE',  ( -3.444139561100000080, 1476.012962394230044, 267.8489069608979776 ) ) ;
#58415=CARTESIAN_POINT ( 'NONE',  ( -4.227395202513110739, 1446.270036243080085, 165.6810918684970204 ) ) ;
#58417=CARTESIAN_POINT ( 'NONE',  ( -13.51891076255363089, 1486.505240369647936, 185.1172359407312342 ) ) ;
#58419=CARTESIAN_POINT ( 'NONE',  ( 2.798741256952680168, 1509.010794585639815, 238.1786444310339732 ) ) ;
#58420=CARTESIAN_POINT ( 'NONE',  ( -12.00000000000000000, 1443.913060387330006, 150.5878346084980137 ) ) ;
#58421=CARTESIAN_POINT ( 'NONE',  ( -25.73740863305900106, 1482.722876254420044, 212.0196469772590149 ) ) ;
#58424=CARTESIAN_POINT ( 'NONE',  ( -19.24979467460000038, 1409.749958184729849, 197.9967212150980060 ) ) ;
#58426=CARTESIAN_POINT ( 'NONE',  ( -0.4986843622567649348, 1508.982343520079894, 238.8510830230749775 ) ) ;
#58427=CARTESIAN_POINT ( 'NONE',  ( -9.858902522070000174, 1408.321029724029813, 270.1194230524980071 ) ) ;
#58429=CARTESIAN_POINT ( 'NONE',  ( -0.5133638609672289688, 1410.311096993930050, 233.1717005261690190 ) ) ;
#58433=FACE_OUTER_BOUND ( 'NONE', #50374, .T. ) ;
#58441=CARTESIAN_POINT ( 'NONE',  ( -0.1955981719786639705, 1416.913060341709979, 193.0575580088199956 ) ) ;
#58442=CARTESIAN_POINT ( 'NONE',  ( -12.49651378394149148, 1398.283529688983435, 205.2589461638358443 ) ) ;
#58446=CARTESIAN_POINT ( 'NONE',  ( 20.11526801819819710, 1508.362997783120136, 229.0140906582849993 ) ) ;
#58451=CARTESIAN_POINT ( 'NONE',  ( 11.78634442959999973, 1433.876985662710013, 150.9130302334980058 ) ) ;
#58452=CARTESIAN_POINT ( 'NONE',  ( -11.28524207019999892, 1396.366239101729889, 212.5318391717879933 ) ) ;
#58455=DIRECTION ( 'NONE',  ( 2.048418183714850102E-08, 0.03085826933284185197, -0.9995237702094840193 ) ) ;
#58459=CARTESIAN_POINT ( 'NONE',  ( 16.69463186169999958, 1507.812162581230041, 231.3306424561980066 ) ) ;
#58461=CARTESIAN_POINT ( 'NONE',  ( 5.538579248009999567, 1468.700840589029895, 183.8662599229979833 ) ) ;
#58462=CARTESIAN_POINT ( 'NONE',  ( -12.26359197939999923, 1416.522662136229883, 194.6757565915980024 ) ) ;
#58466=CARTESIAN_POINT ( 'NONE',  ( 2.500000000000000000, 1419.437602159330027, 141.5609288386980040 ) ) ;
#58467=CARTESIAN_POINT ( 'NONE',  ( 11.77006340779999860, 1432.381006235819996, 150.8117714391979973 ) ) ;
#58468=CARTESIAN_POINT ( 'NONE',  ( 40.27308735900000158, 1443.611949368910018, 137.1163358467979947 ) ) ;
#58469=VERTEX_POINT ( 'NONE', #53226 ) ;
#58470=CARTESIAN_POINT ( 'NONE',  ( 13.03861301673589956, 1434.799502881549870, 149.2342568181190074 ) ) ;
#58474=CARTESIAN_POINT ( 'NONE',  ( 13.50347664955267213, 1444.084118611255917, 169.3539558340694384 ) ) ;
#58475=CARTESIAN_POINT ( 'NONE',  ( -6.719960884899998987, 1465.583908313830079, 233.8333315335979989 ) ) ;
#58482=CARTESIAN_POINT ( 'NONE',  ( 2.500000000000000000, 1448.295510712299802, 164.4143809015409659 ) ) ;
#58488=CARTESIAN_POINT ( 'NONE',  ( -20.01040017649999925, 1508.355603652830041, 229.1813846036980067 ) ) ;
#58490=CARTESIAN_POINT ( 'NONE',  ( -11.19668478630000052, 1409.304057235629898, 189.9697753155979854 ) ) ;
#58493=CARTESIAN_POINT ( 'NONE',  ( -0.3166099825070000096, 1416.237488680629895, 227.4124177731980012 ) ) ;
#58494=ORIENTED_EDGE ( 'NONE', *, *, #94459, .F. ) ;
#58495=CARTESIAN_POINT ( 'NONE',  ( 22.48557446689999750, 1431.347824966569760, 217.2207584623980097 ) ) ;
#58498=CARTESIAN_POINT ( 'NONE',  ( 0.002041696164862339888, 1465.101599726780023, 237.0127939912499926 ) ) ;
#58499=ADVANCED_FACE ( 'NONE', ( #20141 ), #8122, .F. ) ;
#58500=CARTESIAN_POINT ( 'NONE',  ( 13.37958332529999872, 1410.033118652530220, 270.4094488018980087 ) ) ;
#58503=CARTESIAN_POINT ( 'NONE',  ( 24.13371414729999742, 1410.980460536530018, 209.3325957110889988 ) ) ;
#58504=CARTESIAN_POINT ( 'NONE',  ( 24.08426297012860218, 1411.115209414830133, 209.6325633951909708 ) ) ;
#58508=CARTESIAN_POINT ( 'NONE',  ( -2.936501545661585055, 1447.710472861017934, 154.8059207791675647 ) ) ;
#58512=EDGE_LOOP ( 'NONE', ( #54611, #34102, #102032, #76818 ) ) ;
#58514=CARTESIAN_POINT ( 'NONE',  ( 37.17593098820000108, 1458.776684284729981, 264.1765544691980381 ) ) ;
#58518=CARTESIAN_POINT ( 'NONE',  ( -5.388302382240000021, 1432.653872217849994, 154.6144426912980236 ) ) ;
#58519=CARTESIAN_POINT ( 'NONE',  ( -22.79362109059999852, 1450.012765720310199, 219.0613567770580232 ) ) ;
#58523=DIRECTION ( 'NONE',  ( -0.000000000000000000, -0.000000000000000000, 1.000000000000000000 ) ) ;
#58525=CARTESIAN_POINT ( 'NONE',  ( 11.87563351815570023, 1433.006677199550040, 147.6591432317509884 ) ) ;
#58527=ORIENTED_EDGE ( 'NONE', *, *, #17808, .F. ) ;
#58529=EDGE_CURVE ( 'NONE', #6757, #101455, #40420, .T. ) ;
#58530=CARTESIAN_POINT ( 'NONE',  ( -0.04744486741469999824, 1487.212584747929895, 230.3635807236979929 ) ) ;
#58531=CIRCLE ( 'NONE', #28143, 26.43993992909998525 ) ;
#58532=CARTESIAN_POINT ( 'NONE',  ( 20.89213389120000031, 1453.805113726430136, 224.2163675376980052 ) ) ;
#58537=CARTESIAN_POINT ( 'NONE',  ( 14.29986306199981705, 1420.106603705138014, 228.3309057200090706 ) ) ;
#58538=CARTESIAN_POINT ( 'NONE',  ( 26.81568938926840318, 1435.910991003079971, 136.5211442880660115 ) ) ;
#58540=CARTESIAN_POINT ( 'NONE',  ( -20.86012771369999896, 1428.511789623030154, 221.0723165858979939 ) ) ;
#58541=CARTESIAN_POINT ( 'NONE',  ( -45.28159994719300840, 1445.743959104784381, 268.9845966081527990 ) ) ;
#58543=CARTESIAN_POINT ( 'NONE',  ( 12.57505856210000061, 1509.295204559930198, 183.4866265921980073 ) ) ;
#58545=CARTESIAN_POINT ( 'NONE',  ( -29.35411896400288612, 1462.717522830221014, 269.4640705128969671 ) ) ;
#58548=CARTESIAN_POINT ( 'NONE',  ( -34.55887780631552886, 1418.580484962596984, 269.2604001755976242 ) ) ;
#58551=CARTESIAN_POINT ( 'NONE',  ( -0.004559919551130000963, 1417.346727339029940, 235.5710182631979706 ) ) ;
#58553=CARTESIAN_POINT ( 'NONE',  ( 24.95756540081792707, 1451.613964887439806, 137.4741668746740686 ) ) ;
#58556=CARTESIAN_POINT ( 'NONE',  ( -7.429475295173068261, 1416.924823922019868, 231.1912767165910907 ) ) ;
#58557=CARTESIAN_POINT ( 'NONE',  ( -15.08216819395825148, 1451.149145817307499, 149.6691153907744081 ) ) ;
#58558=CARTESIAN_POINT ( 'NONE',  ( 25.13854614859999970, 1436.603051257809966, 137.6783714398980010 ) ) ;
#58559=( BOUNDED_SURFACE ( )  B_SPLINE_SURFACE ( 1, 2, ( 
 ( #2033, #39331, #72407 ),
 ( #29826, #70350, #98124 ) ),
 .UNSPECIFIED., .F., .F., .F. ) 
 B_SPLINE_SURFACE_WITH_KNOTS ( ( 2, 2 ),
 ( 3, 3 ),
 ( -10000.00000000000000, 10000.00000000000000 ),
 ( 5.178100005973779396, 6.283185307179590673 ),
 .UNSPECIFIED. ) 
 GEOMETRIC_REPRESENTATION_ITEM ( )  RATIONAL_B_SPLINE_SURFACE ( (
 ( 0.8778166915500580370, 0.7939440108100890292, 1.000000000000000000),
 ( 0.8778166915500580370, 0.7939440108100890292, 1.000000000000000000) ) ) 
 REPRESENTATION_ITEM ( '' )  SURFACE ( )  );
#58562=CARTESIAN_POINT ( 'NONE',  ( -0.2223009154971570256, 1416.826860677879949, 191.0546700833079967 ) ) ;
#58564=VERTEX_POINT ( 'NONE', #94947 ) ;
#58566=CARTESIAN_POINT ( 'NONE',  ( 16.09938272070030152, 1414.913060387399810, 209.3459460732159982 ) ) ;
#58569=CARTESIAN_POINT ( 'NONE',  ( -23.75987188199999878, 1449.114753669629863, 220.8695786834980197 ) ) ;
#58571=B_SPLINE_CURVE_WITH_KNOTS ( 'NONE', 3,
 ( #105266, #38600, #4472, #37510, #105832, #97412, #72780 ),
 .UNSPECIFIED., .F., .F.,
 ( 4, 3, 4 ),
 ( -84.90067530945870544, -53.18660760086410022, -19.14976305580000826 ),
 .UNSPECIFIED. ) ;
#58572=CARTESIAN_POINT ( 'NONE',  ( -11.87231497000000147, 1433.085999529410174, 150.1763001176979913 ) ) ;
#58577=CARTESIAN_POINT ( 'NONE',  ( -24.15153490410000359, 1438.063247892820073, 212.1983423404379892 ) ) ;
#58579=CARTESIAN_POINT ( 'NONE',  ( 1.127298601310000148, 1450.859579147270097, 182.1360869505979849 ) ) ;
#58581=CARTESIAN_POINT ( 'NONE',  ( -28.69781424069330455, 1510.026368465050155, 200.3394183414388863 ) ) ;
#58583=VERTEX_POINT ( 'NONE', #86538 ) ;
#58585=CARTESIAN_POINT ( 'NONE',  ( -11.73951205012229870, 1426.693896884819878, 144.3445227941359974 ) ) ;
#58587=CARTESIAN_POINT ( 'NONE',  ( -7.954913669629999795, 1471.040533207630006, 269.6217432392980413 ) ) ;
#58593=CARTESIAN_POINT ( 'NONE',  ( 38.61927353243170558, 1444.188088105049928, 137.1592452208769828 ) ) ;
#58596=CARTESIAN_POINT ( 'NONE',  ( -24.00968221052989904, 1411.233756715259915, 269.0770596960790613 ) ) ;
#58597=CARTESIAN_POINT ( 'NONE',  ( -13.68160004434409949, 1436.078871575160065, 150.3811401317549894 ) ) ;
#58601=AXIS2_PLACEMENT_3D ( 'NONE', #29986, #22114, #15386 ) ;
#58602=EDGE_LOOP ( 'NONE', ( #80090, #46517, #34910, #88885 ) ) ;
#58609=CARTESIAN_POINT ( 'NONE',  ( 4.925527104771288300, 1409.085063583942656, 223.4852962484615375 ) ) ;
#58614=EDGE_CURVE ( 'NONE', #74953, #85887, #80481, .T. ) ;
#58620=ORIENTED_EDGE ( 'NONE', *, *, #18037, .F. ) ;
#58622=CARTESIAN_POINT ( 'NONE',  ( 26.91706399319999932, 1488.687396144229979, 211.9506526117480121 ) ) ;
#58625=CARTESIAN_POINT ( 'NONE',  ( -23.91862134480000179, 1435.332757494850057, 136.7253933288979795 ) ) ;
#58626=CARTESIAN_POINT ( 'NONE',  ( -24.90258955090000015, 1442.651874318690034, 210.5047954567180000 ) ) ;
#58631=DIRECTION ( 'NONE',  ( 0.000000000000000000, 1.000000000000000000, 0.000000000000000000 ) ) ;
#58635=CARTESIAN_POINT ( 'NONE',  ( -2.435720948416219667, 1451.955458385490147, 184.6330791665090203 ) ) ;
#58640=CARTESIAN_POINT ( 'NONE',  ( 12.68045462138680080, 1435.869917964839942, 150.8815144536550008 ) ) ;
#58641=CARTESIAN_POINT ( 'NONE',  ( -4.072368715194547129, 1441.029081303531029, 184.8776654416552674 ) ) ;
#58649=CARTESIAN_POINT ( 'NONE',  ( 40.62990393029997449, 1439.681967586943756, 135.2802163397979314 ) ) ;
#58652=ORIENTED_EDGE ( 'NONE', *, *, #70508, .F. ) ;
#58653=CARTESIAN_POINT ( 'NONE',  ( -17.70115280944790115, 1479.586903222029832, 228.8488225417430328 ) ) ;
#58656=CARTESIAN_POINT ( 'NONE',  ( 1.661580760779999943, 1421.006482085029802, 183.6687324547980040 ) ) ;
#58663=CARTESIAN_POINT ( 'NONE',  ( 17.22755355015131684, 1422.440680106109312, 226.6931585904254973 ) ) ;
#58664=CARTESIAN_POINT ( 'NONE',  ( 18.24797473426792394, 1425.311414221095447, 224.8433002223622168 ) ) ;
#58665=CARTESIAN_POINT ( 'NONE',  ( -2.488082932330000219, 1441.600846913620217, 150.5962877614979902 ) ) ;
#58666=CARTESIAN_POINT ( 'NONE',  ( 37.61101231473060125, 1440.913060385340032, 255.6516536714609629 ) ) ;
#58669=CARTESIAN_POINT ( 'NONE',  ( 13.31007525419999915, 1426.030389151729878, 221.9162573719980003 ) ) ;
#58670=ORIENTED_EDGE ( 'NONE', *, *, #85761, .T. ) ;
#58675=CARTESIAN_POINT ( 'NONE',  ( -28.73878198690000119, 1509.916640767629815, 211.4156715658480152 ) ) ;
#58678=CARTESIAN_POINT ( 'NONE',  ( 1.519498793946838067, 1507.960421343096868, 236.9808823838983187 ) ) ;
#58681=CARTESIAN_POINT ( 'NONE',  ( -1.517668881329999886, 1497.681034404829916, 231.6004894389980109 ) ) ;
#58685=CARTESIAN_POINT ( 'NONE',  ( 7.197032540600000416, 1452.516711882729851, 152.8386597052979994 ) ) ;
#58686=CARTESIAN_POINT ( 'NONE',  ( -27.56721773654333774, 1509.458873407235387, 212.0988943604728263 ) ) ;
#58689=EDGE_LOOP ( 'NONE', ( #40665, #82758, #26501, #25384 ) ) ;
#58692=CARTESIAN_POINT ( 'NONE',  ( 19.79142244099470105, 1508.177231791150007, 229.3266476993300103 ) ) ;
#58695=( BOUNDED_CURVE ( )  B_SPLINE_CURVE ( 3, ( #42403, #95570, #10460, #60896 ),
 .UNSPECIFIED., .F., .T. ) 
 B_SPLINE_CURVE_WITH_KNOTS ( ( 4, 4 ),
 ( 3.040788486948645009, 3.052744563067074868 ),
 .UNSPECIFIED. ) 
 CURVE ( )  GEOMETRIC_REPRESENTATION_ITEM ( )  RATIONAL_B_SPLINE_CURVE ( ( 1.000000000000000000, 0.9999880877224632814, 0.9999880877224632814, 1.000000000000000000 ) ) 
 REPRESENTATION_ITEM ( '' )  );
#58697=CARTESIAN_POINT ( 'NONE',  ( 40.05235817349409899, 1441.916377590050161, 136.9240625044390072 ) ) ;
#58702=CARTESIAN_POINT ( 'NONE',  ( -11.81894877114215348, 1435.231921587601164, 151.2719100762131177 ) ) ;
#58706=CARTESIAN_POINT ( 'NONE',  ( 1.103557112500000104, 1409.457326867330039, 185.4212059947979867 ) ) ;
#58707=CARTESIAN_POINT ( 'NONE',  ( 4.385995343010000269, 1424.610434865430079, 185.2880463713979964 ) ) ;
#58709=CARTESIAN_POINT ( 'NONE',  ( -4.270405931533109545, 1441.143229069919926, 158.1181609420549989 ) ) ;
#58710=CARTESIAN_POINT ( 'NONE',  ( 11.84030382862209940, 1430.235986815720025, 151.0624496527620124 ) ) ;
#58711=ORIENTED_EDGE ( 'NONE', *, *, #80949, .F. ) ;
#58712=CARTESIAN_POINT ( 'NONE',  ( -1.618115094650000030, 1427.197104430330000, 147.9439864917980287 ) ) ;
#58713=CARTESIAN_POINT ( 'NONE',  ( 18.47806089193409562, 1457.403878534810019, 229.7720814934239968 ) ) ;
#58714=CARTESIAN_POINT ( 'NONE',  ( 15.09717514449999953, 1449.518815468759840, 189.9127100080980028 ) ) ;
#58715=CARTESIAN_POINT ( 'NONE',  ( -1.118730856090010083E-08, 1473.460517805439849, 262.2339000674530212 ) ) ;
#58717=CARTESIAN_POINT ( 'NONE',  ( -0.7186627752419999515, 1416.547221146729953, 227.9060452208979939 ) ) ;
#58720=CARTESIAN_POINT ( 'NONE',  ( -0.02015038597255117483, 1486.257254326256998, 181.8141459044200872 ) ) ;
#58722=CARTESIAN_POINT ( 'NONE',  ( -45.72254065293900283, 1438.289221927810104, 268.7603399551510392 ) ) ;
#58727=CARTESIAN_POINT ( 'NONE',  ( 2.583688234164152497, 1424.460962572045901, 227.2704015761902667 ) ) ;
#58729=CARTESIAN_POINT ( 'NONE',  ( -26.29521927434609907, 1450.751943985090065, 136.5719960223099747 ) ) ;
#58731=CARTESIAN_POINT ( 'NONE',  ( 30.53571888249999944, 1440.913060393610067, 240.1260121784980015 ) ) ;
#58735=CARTESIAN_POINT ( 'NONE',  ( -24.40164415750000160, 1440.913060428330027, 211.9534758661580156 ) ) ;
#58739=VERTEX_POINT ( 'NONE', #105566 ) ;
#58740=DIRECTION ( 'NONE',  ( 0.000000000000000000, 0.000000000000000000, -1.000000000000000000 ) ) ;
#58744=ORIENTED_EDGE ( 'NONE', *, *, #30159, .F. ) ;
#58745=CARTESIAN_POINT ( 'NONE',  ( -23.95553366050739896, 1410.857329053969806, 209.8766206678370168 ) ) ;
#58746=CARTESIAN_POINT ( 'NONE',  ( -3.721277981550000113, 1424.084032539730060, 184.7565605802979860 ) ) ;
#58748=CARTESIAN_POINT ( 'NONE',  ( -45.41132133646503632, 1437.168779479949762, 266.1959130671517073 ) ) ;
#58751=CARTESIAN_POINT ( 'NONE',  ( -2.295501929209999847, 1507.640548290029983, 236.9905098398980101 ) ) ;
#58753=ADVANCED_FACE ( 'NONE', ( #71991 ), #4202, .F. ) ;
#58754=AXIS2_PLACEMENT_3D ( 'NONE', #80656, #29689, #85591 ) ;
#58755=CARTESIAN_POINT ( 'NONE',  ( 41.00042505258200265, 1456.753174803509864, 266.5635232765240517 ) ) ;
#58760=CARTESIAN_POINT ( 'NONE',  ( 18.51267396087533967, 1458.739381326464354, 227.6064210715596232 ) ) ;
#58761=B_SPLINE_CURVE_WITH_KNOTS ( 'NONE', 3,
 ( #87946, #81166, #89570, #4481 ),
 .UNSPECIFIED., .F., .F.,
 ( 4, 4 ),
 ( 0.000000000000000000, 1.000000000000000000 ),
 .UNSPECIFIED. ) ;
#58763=FACE_OUTER_BOUND ( 'NONE', #55106, .T. ) ;
#58766=B_SPLINE_CURVE_WITH_KNOTS ( 'NONE', 3,
 ( #35657, #10459, #88277, #103965, #27262, #53035, #87171, #44633, #70403, #104522, #53595, #105641, #63117, #98317, #37325, #4280, #3746, #97768, #56333, #89376, #63653, #28926, #97217, #90465, #38410, #98869, #5367, #13742, #82062, #71521, #38952, #46847, #80976, #20489, #54699, #47926, #107273, #73131, #21596, #106714, #88825, #3198, #106177, #37878, #79885, #30568 ),
 .UNSPECIFIED., .F., .F.,
 ( 4, 2, 2, 2, 2, 2, 1, 1, 2, 2, 2, 2, 2, 1, 1, 1, 2, 2, 2, 2, 1, 1, 1, 1, 1, 2, 2, 4 ),
 ( 0.000000000000000000, 0.06250000000046999904, 0.09375000000066381622, 0.1250000000008576473, 0.1875000000012422285, 0.2187500000014324097, 0.2343750000015297486, 0.2421875000015806800, 0.2460937500015798474, 0.2500000000015789592, 0.3750000000012674306, 0.4375000000011254886, 0.4687500000010677015, 0.4843750000010489387, 0.4921875000010395573, 0.4960937500010235146, 0.4980468750010155210, 0.5000000000010075274, 0.6250000000004316547, 0.6875000000001338929, 0.7187499999999865663, 0.7343749999999142908, 0.7421874999998850919, 0.7460937499998719913, 0.7480468749998668843, 0.7490234374998724354, 0.7499999999998779865, 1.000000000000000000 ),
 .UNSPECIFIED. ) ;
#58767=CARTESIAN_POINT ( 'NONE',  ( 27.03107214705890016, 1451.493449271870077, 136.0706941817539928 ) ) ;
#58768=EDGE_CURVE ( 'NONE', #36309, #65298, #87652, .T. ) ;
#58770=CARTESIAN_POINT ( 'NONE',  ( 4.226195811716859652, 1452.765478377580166, 152.2144321770960005 ) ) ;
#58774=CARTESIAN_POINT ( 'NONE',  ( 6.924940705133599828, 1409.154884645419997, 188.7083484210960194 ) ) ;
#58775=CARTESIAN_POINT ( 'NONE',  ( 1.837350884659999961, 1417.558700500429950, 234.5777813587980063 ) ) ;
#58781=ORIENTED_EDGE ( 'NONE', *, *, #33990, .F. ) ;
#58789=CARTESIAN_POINT ( 'NONE',  ( -34.84383440970000123, 1453.969943383929831, 265.6112250856980381 ) ) ;
#58790=CARTESIAN_POINT ( 'NONE',  ( -22.39540327093973104, 1509.695125100958421, 191.0396457048211403 ) ) ;
#58791=CARTESIAN_POINT ( 'NONE',  ( 11.08805915299999967, 1433.401164229489950, 151.6926779325980021 ) ) ;
#58792=CARTESIAN_POINT ( 'NONE',  ( 8.881784197000000993E-16, 1470.874276671130019, 268.3665355202980436 ) ) ;
#58793=B_SPLINE_CURVE_WITH_KNOTS ( 'NONE', 5,
 ( #13305, #72174, #29575, #65414, #99520, #90028, #107940, #30682, #23375, #65968, #63761, #5482, #64869, #46962, #57566, #31781, #22805, #91139, #22251, #48609, #98977, #39643, #55356, #39068, #3864, #55910, #74368 ),
 .UNSPECIFIED., .F., .F.,
 ( 6, 3, 3, 3, 3, 3, 3, 3, 6 ),
 ( 0.000000000000000000, 0.03529557405075641613, 0.06179070172895334556, 0.08828582939876877811, 0.1412760847467809111, 0.2826085572933068613, 0.5644389168522545575, 0.8435653545061785330, 1.000000000000000000 ),
 .UNSPECIFIED. ) ;
#58794=CARTESIAN_POINT ( 'NONE',  ( 11.41805403401209951, 1414.913057862230062, 197.3911482182210193 ) ) ;
#58798=CARTESIAN_POINT ( 'NONE',  ( -18.92783145980000370, 1486.091458575729803, 189.3401239504979969 ) ) ;
#58800=CARTESIAN_POINT ( 'NONE',  ( 17.33645362950000290, 1414.996442546130083, 210.3925741896480304 ) ) ;
#58801=B_SPLINE_CURVE_WITH_KNOTS ( 'NONE', 3,
 ( #10771, #45498, #78524, #44942, #88585, #27559, #61204, #11326, #54449, #71258, #26442, #94761, #70708, #86357, #36514, #105380, #28668, #103714, #19132, #69596, #1835, #53907, #104270, #79089, #52775, #86913, #11867, #61742, #44380, #62873, #9640, #77416, #95865, #53335, #18036, #87483, #95319, #62299, #2397, #96985, #96426, #104821, #20248 ),
 .UNSPECIFIED., .F., .F.,
 ( 4, 3, 3, 3, 3, 3, 3, 3, 3, 3, 3, 3, 3, 3, 4 ),
 ( -1.999999029881750046, -1.991354409435089901, -1.843127450874009865, -1.686255871866269906, -1.534783949317029883, -1.379712255795449982, -1.225304414952149923, -1.070191527292039924, -0.9147394646296638232, -0.7593381984712410659, -0.6048407093868408690, -0.4514088248038210516, -0.2993314472943329196, -0.1488170141350799724, -5.152078763615008938E-11 ),
 .UNSPECIFIED. ) ;
#58802=CARTESIAN_POINT ( 'NONE',  ( 19.39159332000000191, 1430.347784931329898, 222.5897557541980234 ) ) ;
#58803=CARTESIAN_POINT ( 'NONE',  ( -15.36549428884569934, 1420.414141511310163, 227.0219848988409979 ) ) ;
#58809=CARTESIAN_POINT ( 'NONE',  ( 0.1811898575556089852, 1473.797889089420096, 182.3607679443829852 ) ) ;
#58810=CARTESIAN_POINT ( 'NONE',  ( -5.816635555072360297, 1408.583828391070028, 221.8830431125730058 ) ) ;
#58811=ORIENTED_EDGE ( 'NONE', *, *, #105656, .F. ) ;
#58812=CARTESIAN_POINT ( 'NONE',  ( -17.22592482065197927, 1444.324653571828776, 162.9227486220069920 ) ) ;
#58816=CARTESIAN_POINT ( 'NONE',  ( -40.76227011288860069, 1440.007145189510084, 134.0999999980880091 ) ) ;
#58818=ORIENTED_EDGE ( 'NONE', *, *, #33520, .F. ) ;
#58819=B_SPLINE_SURFACE_WITH_KNOTS ( 'NONE', 5, 1, ( 
 ( #472, #24521 ),
 ( #34043, #58710 ),
 ( #92843, #68233 ),
 ( #25626, #93391 ),
 ( #16120, #93937 ),
 ( #50324, #16656 ) ),
 .UNSPECIFIED., .F., .F., .F.,
 ( 6, 6 ),
 ( 2, 2 ),
 ( 0.000000000000000000, 11.48860277639830052 ),
 ( -1.500000000000000000, 1.500000000000000000 ),
 .UNSPECIFIED. ) ;
#58825=CARTESIAN_POINT ( 'NONE',  ( 0.4863421998530879642, 1418.702335047680208, 184.7127968358159933 ) ) ;
#58827=CARTESIAN_POINT ( 'NONE',  ( 22.11623627239999834, 1489.468502498730004, 210.6419393784279919 ) ) ;
#58829=CARTESIAN_POINT ( 'NONE',  ( 3.917311521000000685, 1436.965663665770080, 184.8061579696979777 ) ) ;
#58830=B_SPLINE_SURFACE_WITH_KNOTS ( 'NONE', 5, 4, ( 
 ( #10511, #53083, #36262, #62619, #54201 ),
 ( #95069, #70451, #86659, #36819, #11072 ),
 ( #104571, #63166, #27866, #71009, #3247 ),
 ( #9954, #44126, #62046, #53646, #45242 ),
 ( #11621, #78261, #105130, #96736, #37373 ),
 ( #20007, #45798, #1574, #79931, #71574 ),
 ( #9406, #35707, #105695, #43568, #69897 ),
 ( #77718, #39003, #12162, #90517, #14350 ),
 ( #22187, #48541, #106765, #65349, #21642 ) ),
 .UNSPECIFIED., .F., .F., .F.,
 ( 6, 3, 6 ),
 ( 5, 5 ),
 ( 0.000000000000000000, 5.782490304330000441, 11.25975508159999983 ),
 ( 25.78146411700000229, 39.23969207129999859 ),
 .UNSPECIFIED. ) ;
#58834=ORIENTED_EDGE ( 'NONE', *, *, #76663, .T. ) ;
#58836=CARTESIAN_POINT ( 'NONE',  ( 11.93818824289999903, 1433.480083226980014, 149.8972169559980046 ) ) ;
#58837=CARTESIAN_POINT ( 'NONE',  ( 12.53517974735357576, 1442.773887286369700, 169.5044317858253464 ) ) ;
#58841=AXIS2_PLACEMENT_3D ( 'NONE', #96668, #43508, #77653 ) ;
#58842=ADVANCED_FACE ( 'NONE', ( #21515 ), #32236, .F. ) ;
#58843=CARTESIAN_POINT ( 'NONE',  ( -19.20111751579667114, 1410.945218301533487, 222.5811953199733466 ) ) ;
#58846=EDGE_CURVE ( 'NONE', #104880, #16730, #105888, .T. ) ;
#58847=CARTESIAN_POINT ( 'NONE',  ( 39.91348005095139939, 1450.504013711060225, 269.6087561242041488 ) ) ;
#58849=EDGE_CURVE ( 'NONE', #43125, #49156, #14723, .T. ) ;
#58850=CARTESIAN_POINT ( 'NONE',  ( 15.03154484612626263, 1430.682371875214812, 220.0467435185384204 ) ) ;
#58851=CARTESIAN_POINT ( 'NONE',  ( 2.572398481029999573, 1417.848201471729908, 233.8656960024980265 ) ) ;
#58853=CARTESIAN_POINT ( 'NONE',  ( 40.27308693906149273, 1443.611999474700042, 137.1163322506119755 ) ) ;
#58854=CARTESIAN_POINT ( 'NONE',  ( 1.910126501409999789E-10, 1431.113060387329824, 227.8291532366980050 ) ) ;
#58858=CARTESIAN_POINT ( 'NONE',  ( 2.704954423850000289, 1447.065239520190062, 170.5387359128979767 ) ) ;
#58859=ORIENTED_EDGE ( 'NONE', *, *, #33002, .F. ) ;
#58861=CARTESIAN_POINT ( 'NONE',  ( 14.35469249349999998, 1416.832348283729971, 196.6649917540980255 ) ) ;
#58864=CARTESIAN_POINT ( 'NONE',  ( -15.06280282045160135, 1422.388303761650150, 229.4662100962750060 ) ) ;
#58867=CARTESIAN_POINT ( 'NONE',  ( -20.29535751400000265, 1430.346966375530201, 196.9847315563980032 ) ) ;
#58868=CARTESIAN_POINT ( 'NONE',  ( -11.18248557239999919, 1426.884307463830055, 103.8973682686980169 ) ) ;
#58869=CARTESIAN_POINT ( 'NONE',  ( 15.87404176176099924, 1409.467377696719950, 192.9779251718159969 ) ) ;
#58871=CARTESIAN_POINT ( 'NONE',  ( 36.22678859348660296, 1436.464133680080067, 136.2561648524459770 ) ) ;
#58872=FACE_OUTER_BOUND ( 'NONE', #89901, .T. ) ;
#58873=CARTESIAN_POINT ( 'NONE',  ( -35.25148663959999595, 1420.828143575929971, 264.2529700431979904 ) ) ;
#58874=CARTESIAN_POINT ( 'NONE',  ( -0.7704842542331529209, 1509.002383188599879, 179.3520445167110040 ) ) ;
#58875=CARTESIAN_POINT ( 'NONE',  ( 17.06106173523173553, 1460.356808348517234, 228.7022572861417586 ) ) ;
#58881=CARTESIAN_POINT ( 'NONE',  ( -18.76125227649999871, 1457.009933317229979, 229.1040481900979842 ) ) ;
#58885=CARTESIAN_POINT ( 'NONE',  ( 13.76740486215110160, 1464.191801214029738, 225.0510466410910055 ) ) ;
#58891=CARTESIAN_POINT ( 'NONE',  ( 36.37832876739999932, 1451.642701153929920, 134.0999999898979809 ) ) ;
#58893=B_SPLINE_SURFACE_WITH_KNOTS ( 'NONE', 5, 5, ( 
 ( #82420, #90805, #6248, #66736, #14646, #57784 ),
 ( #31446, #67285, #48832, #65629, #49918, #99189 ),
 ( #82955, #83494, #14086, #23034, #23595, #74575 ),
 ( #33096, #15179, #39859, #56113, #40951, #100839 ),
 ( #91902, #107610, #66190, #7351, #108711, #74022 ),
 ( #90246, #41514, #58319, #6790, #49366, #75128 ),
 ( #75673, #109817, #108156, #109277, #92441, #13528 ),
 ( #47715, #81845, #5149, #39304, #30894, #43716 ),
 ( #67829, #35307, #1177, #68387, #43170, #8998 ),
 ( #26341, #77867, #18480, #69494, #86813, #35872 ),
 ( #52677, #623, #76213, #51569, #85702, #52128 ),
 ( #86256, #103043, #25784, #51016, #1733, #70056 ),
 ( #17930, #16816, #77324, #110358, #84600, #10105 ),
 ( #24669, #103616, #26914, #61102, #60537, #94659 ),
 ( #68942, #76763, #101940, #78422, #9546, #59982 ),
 ( #44278, #93543, #42062, #95219, #85151, #33635 ),
 ( #58868, #7891, #34203, #92998, #25228, #16274 ),
 ( #50476, #59431, #8437, #42610, #72, #34754 ),
 ( #102494, #94100, #17371, #36406, #97955, #53802 ),
 ( #20689, #95767, #71150, #97419, #79531, #37516 ),
 ( #54346, #89011, #44837, #55434, #21225, #19034 ),
 ( #62195, #10671, #54886, #96322, #78992, #104167 ),
 ( #87377, #2833, #71719, #2295, #47036, #89565 ),
 ( #12855, #19600, #81161, #3939, #3388, #105837 ),
 ( #80066, #11761, #70598, #4476, #87939, #11230 ),
 ( #53235, #105273, #12300, #36954, #29115, #28565 ) ),
 .UNSPECIFIED., .F., .F., .F.,
 ( 6, 5, 3, 3, 3, 3, 3, 6 ),
 ( 6, 6 ),
 ( 14.16850226231500010, 14.91778146530000093, 25.40568016630000159, 46.35833806440000160, 67.31099596259998918, 78.57834886320000578, 84.21202531349999276, 89.84570176380000817 ),
 ( 0.000000000000000000, 2.061429890987789726 ),
 .UNSPECIFIED. ) ;
#58894=CARTESIAN_POINT ( 'NONE',  ( 27.69925880659999962, 1441.434395406610065, 137.3015763229979882 ) ) ;
#58897=ORIENTED_EDGE ( 'NONE', *, *, #47446, .F. ) ;
#58898=( BOUNDED_CURVE ( )  B_SPLINE_CURVE ( 3, ( #23780, #22659, #33287, #83157 ),
 .UNSPECIFIED., .F., .T. ) 
 B_SPLINE_CURVE_WITH_KNOTS ( ( 4, 4 ),
 ( 2.890157840421000213, 3.288561460421139948 ),
 .UNSPECIFIED. ) 
 CURVE ( )  GEOMETRIC_REPRESENTATION_ITEM ( )  RATIONAL_B_SPLINE_CURVE ( ( 1.000000000000000000, 0.9868165609958530204, 0.9868165609958530204, 1.000000000000000000 ) ) 
 REPRESENTATION_ITEM ( '' )  );
#58901=ORIENTED_EDGE ( 'NONE', *, *, #2147, .F. ) ;
#58904=CARTESIAN_POINT ( 'NONE',  ( 20.28635835149999878, 1497.705735184930063, 227.7388624672979915 ) ) ;
#58906=CARTESIAN_POINT ( 'NONE',  ( -13.56558276610000036, 1415.128105759529944, 220.7749916984980132 ) ) ;
#58907=EDGE_CURVE ( 'NONE', #102101, #51188, #35062, .T. ) ;
#58908=CARTESIAN_POINT ( 'NONE',  ( -11.40717366248250109, 1432.341607270339864, 151.3374056301740040 ) ) ;
#58911=CARTESIAN_POINT ( 'NONE',  ( 21.63738260543960124, 1409.760734550770167, 206.3395242849809961 ) ) ;
#58913=CARTESIAN_POINT ( 'NONE',  ( -0.1318727118059999925, 1507.624523832230125, 180.8831098946980092 ) ) ;
#58916=CARTESIAN_POINT ( 'NONE',  ( 23.49278042014210044, 1432.394255265819993, 206.2073926321550061 ) ) ;
#58918=CARTESIAN_POINT ( 'NONE',  ( -10.70847609427080016, 1506.854789404229905, 189.5201119528840081 ) ) ;
#58923=CARTESIAN_POINT ( 'NONE',  ( -8.301987938657498844, 1512.913060387330006, 186.6498241004079262 ) ) ;
#58927=CARTESIAN_POINT ( 'NONE',  ( -11.41895509221428284, 1425.728710957366502, 138.9295753978231573 ) ) ;
#58929=ORIENTED_EDGE ( 'NONE', *, *, #89132, .F. ) ;
#58932=CARTESIAN_POINT ( 'NONE',  ( -10.87453050220000073, 1426.191206384630050, 148.6425034869979811 ) ) ;
#58933=CARTESIAN_POINT ( 'NONE',  ( 19.11490450420339826, 1456.932054066890032, 225.0864823901050045 ) ) ;
#58937=CARTESIAN_POINT ( 'NONE',  ( 11.10897332659999925, 1410.396565740230244, 229.3766474285979768 ) ) ;
#58939=CARTESIAN_POINT ( 'NONE',  ( -21.05893290610000079, 1495.370945771229799, 226.6524662259979834 ) ) ;
#58941=DIRECTION ( 'NONE',  ( 0.0009897943187279698019, -0.9990041106109668334, -0.04460725601959834169 ) ) ;
#58943=EDGE_LOOP ( 'NONE', ( #79389, #28368, #82848, #66064, #87474 ) ) ;
#58945=CARTESIAN_POINT ( 'NONE',  ( 27.10552972939999705, 1412.304471280730013, 267.5397075098980508 ) ) ;
#58946=CARTESIAN_POINT ( 'NONE',  ( -0.2565576784669999499, 1409.415731107930014, 185.2539421329980200 ) ) ;
#58947=CARTESIAN_POINT ( 'NONE',  ( 19.60616233339999681, 1449.731300271829923, 192.9561808612979803 ) ) ;
#58948=CARTESIAN_POINT ( 'NONE',  ( -0.04703443907195579976, 1508.971642086719839, 238.8756872305209811 ) ) ;
#58950=CARTESIAN_POINT ( 'NONE',  ( -1.524714358750000054, 1451.605638646529997, 183.9700909300979959 ) ) ;
#58953=CIRCLE ( 'NONE', #10676, 1.999999954377544853 ) ;
#58954=CARTESIAN_POINT ( 'NONE',  ( -13.41257183429999955, 1444.508158409760199, 187.3828037918979703 ) ) ;
#58955=CARTESIAN_POINT ( 'NONE',  ( -18.91838588339999916, 1497.713060387329961, 221.0203545984980167 ) ) ;
#58957=CARTESIAN_POINT ( 'NONE',  ( 36.48439548460181214, 1420.562375130034297, 269.8440692943977410 ) ) ;
#58958=CARTESIAN_POINT ( 'NONE',  ( 1.459360875619579945, 1496.550641856539869, 181.5740326910060105 ) ) ;
#58959=CARTESIAN_POINT ( 'NONE',  ( -19.02913997090000109, 1436.609546585079897, 214.3676144204279694 ) ) ;
#58962=CARTESIAN_POINT ( 'NONE',  ( -18.38476637639999822, 1473.248652006430120, 267.3950365521980075 ) ) ;
#58964=CARTESIAN_POINT ( 'NONE',  ( -21.24473942629999712, 1509.721192233729880, 188.1671532087979699 ) ) ;
#58965=CARTESIAN_POINT ( 'NONE',  ( -24.26250232874330237, 1444.584236750404443, 211.3627685846172710 ) ) ;
#58968=CARTESIAN_POINT ( 'NONE',  ( 12.17244369425279871, 1416.196255298699953, 223.4846811968139946 ) ) ;
#58974=CARTESIAN_POINT ( 'NONE',  ( -22.02805665500000032, 1409.682297076129998, 206.3742546035879855 ) ) ;
#58980=CARTESIAN_POINT ( 'NONE',  ( -16.59207410940000216, 1408.838686485329845, 269.5630249687979472 ) ) ;
#58982=B_SPLINE_SURFACE_WITH_KNOTS ( 'NONE', 5, 5, ( 
 ( #32903, #21729, #99000, #48076, #99552, #22837 ),
 ( #81647, #31261, #58136, #73271, #83865, #49737 ),
 ( #39095, #57042, #107411, #66553, #7168, #5513 ),
 ( #30707, #31813, #32372, #74396, #41326, #91168 ),
 ( #82209, #47526, #6062, #75496, #64893, #39669 ),
 ( #14446, #48640, #100120, #22277, #92269, #73837 ) ),
 .UNSPECIFIED., .F., .F., .F.,
 ( 6, 6 ),
 ( 6, 6 ),
 ( 29.50720980489999690, 158.0245753780000086 ),
 ( 0.000000000000000000, 1.000000000000000000 ),
 .UNSPECIFIED. ) ;
#58990=CARTESIAN_POINT ( 'NONE',  ( 11.73681854383099932, 1426.696124960400084, 144.1550751902559853 ) ) ;
#58993=LINE ( 'NONE', #93655, #11533 ) ;
#58997=CARTESIAN_POINT ( 'NONE',  ( -0.2148496144000409946, 1419.222389015129920, 184.6498064978729872 ) ) ;
#59000=CARTESIAN_POINT ( 'NONE',  ( -13.35004134540000109, 1415.296882282229944, 221.1257189973979962 ) ) ;
#59005=CARTESIAN_POINT ( 'NONE',  ( 21.17557709188830017, 1509.351061401330071, 228.3384711562210043 ) ) ;
#59007=ORIENTED_EDGE ( 'NONE', *, *, #26837, .F. ) ;
#59009=CARTESIAN_POINT ( 'NONE',  ( 11.53651591631439999, 1434.720663866509994, 151.3975021344279810 ) ) ;
#59010=CARTESIAN_POINT ( 'NONE',  ( -6.779985536469999907, 1396.149822699429933, 218.3141025366080044 ) ) ;
#59012=CARTESIAN_POINT ( 'NONE',  ( -0.0002532898294781912862, 1396.497903775337136, 221.5346559189089817 ) ) ;
#59014=DIRECTION ( 'NONE',  ( 0.000000000000000000, -1.000000000000000000, 0.000000000000000000 ) ) ;
#59016=CARTESIAN_POINT ( 'NONE',  ( -13.71800425710380011, 1507.970762863469872, 184.2200768164369720 ) ) ;
#59017=CARTESIAN_POINT ( 'NONE',  ( 19.29102239047420042, 1488.415415665300088, 228.6203174551539803 ) ) ;
#59018=EDGE_CURVE ( 'NONE', #76827, #17927, #18304, .T. ) ;
#59019=CARTESIAN_POINT ( 'NONE',  ( 1.309051754279999980, 1468.707717750329948, 182.7499832783979912 ) ) ;
#59021=CARTESIAN_POINT ( 'NONE',  ( 44.43457369424350389, 1440.913053162589904, 270.0922382296420210 ) ) ;
#59024=EDGE_CURVE ( 'NONE', #47969, #101819, #36452, .T. ) ;
#59025=CARTESIAN_POINT ( 'NONE',  ( 14.45145579027819949, 1416.702560754929891, 196.8582874468680188 ) ) ;
#59026=CARTESIAN_POINT ( 'NONE',  ( 11.85618979400000050, 1431.606717022440080, 150.3527028125979825 ) ) ;
#59029=CARTESIAN_POINT ( 'NONE',  ( 12.95217011737299906, 1434.756318633420051, 149.1861961083450012 ) ) ;
#59030=ORIENTED_EDGE ( 'NONE', *, *, #67325, .T. ) ;
#59031=ADVANCED_FACE ( 'NONE', ( #36565 ), #21888, .T. ) ;
#59032=ORIENTED_EDGE ( 'NONE', *, *, #12505, .T. ) ;
#59033=CARTESIAN_POINT ( 'NONE',  ( 13.44657628210572575, 1444.308568810446104, 169.3633758692288040 ) ) ;
#59034=CARTESIAN_POINT ( 'NONE',  ( -6.868311248510000411, 1463.903099144130010, 235.5040378045979992 ) ) ;
#59039=EDGE_CURVE ( 'NONE', #58469, #9890, #17584, .T. ) ;
#59041=CARTESIAN_POINT ( 'NONE',  ( 2.500000000000000000, 1448.349745776700047, 163.1876515373769791 ) ) ;
#59043=ORIENTED_EDGE ( 'NONE', *, *, #30159, .T. ) ;
#59045=VERTEX_POINT ( 'NONE', #28719 ) ;
#59046=CARTESIAN_POINT ( 'NONE',  ( 21.73410520339709961, 1440.913060387330006, 226.0964448684460137 ) ) ;
#59048=CARTESIAN_POINT ( 'NONE',  ( -19.34325532379999757, 1509.569025808630158, 231.1400346091979827 ) ) ;
#59049=CARTESIAN_POINT ( 'NONE',  ( -11.71720101390000046, 1409.322234063030010, 190.6809772676980117 ) ) ;
#59053=CARTESIAN_POINT ( 'NONE',  ( 20.62552256830000275, 1428.450544870129988, 221.6279733991980265 ) ) ;
#59061=CARTESIAN_POINT ( 'NONE',  ( 23.89892935376693828, 1410.398181730384294, 209.5833290241005500 ) ) ;
#59062=CARTESIAN_POINT ( 'NONE',  ( -11.20854089327220038, 1414.996442620800053, 195.7122650692939771 ) ) ;
#59064=CARTESIAN_POINT ( 'NONE',  ( 20.14739811709999984, 1412.328483943929996, 271.1218459616979999 ) ) ;
#59067=CARTESIAN_POINT ( 'NONE',  ( -10.59445717635187023, 1486.014368868439760, 184.0782091622903636 ) ) ;
#59073=CARTESIAN_POINT ( 'NONE',  ( 29.43658765730000226, 1455.581846386829966, 250.1802633525980184 ) ) ;
#59074=LINE ( 'NONE', #41148, #2058 ) ;
#59076=CARTESIAN_POINT ( 'NONE',  ( -0.8945946638535250406, 1417.298095655010002, 235.8147265033050246 ) ) ;
#59079=CARTESIAN_POINT ( 'NONE',  ( 0.9900606234040129072, 1452.889512402500031, 183.3744259742010172 ) ) ;
#59080=EDGE_CURVE ( 'NONE', #79053, #101350, #91247, .T. ) ;
#59082=DIRECTION ( 'NONE',  ( 0.000000000000000000, 0.000000000000000000, -1.000000000000000000 ) ) ;
#59085=VERTEX_POINT ( 'NONE', #65636 ) ;
#59087=CARTESIAN_POINT ( 'NONE',  ( -27.01382282590000017, 1451.969727051930022, 134.9184453750980026 ) ) ;
#59088=CARTESIAN_POINT ( 'NONE',  ( 12.97050746999999937, 1422.770599689629762, 223.1036895935980056 ) ) ;
#59090=CARTESIAN_POINT ( 'NONE',  ( -2.500000000000000000, 1423.874532570859856, 167.3087045243360080 ) ) ;
#59093=CARTESIAN_POINT ( 'NONE',  ( 29.70034918587519712, 1435.534590375950074, 135.6337138702669733 ) ) ;
#59095=CARTESIAN_POINT ( 'NONE',  ( 37.77054191136320327, 1449.013782357440050, 136.3553928163400144 ) ) ;
#59096=CARTESIAN_POINT ( 'NONE',  ( -3.793562082119010803, 1450.899618466582069, 184.9307169054388282 ) ) ;
#59098=CARTESIAN_POINT ( 'NONE',  ( 12.44163360890000014, 1509.176498968829947, 183.7399934378979935 ) ) ;
#59101=VERTEX_POINT ( 'NONE', #75138 ) ;
#59103=ADVANCED_FACE ( 'NONE', ( #107070 ), #91913, .T. ) ;
#59104=CARTESIAN_POINT ( 'NONE',  ( -42.89947813909407159, 1429.237451840416952, 269.0512739436722995 ) ) ;
#59106=CARTESIAN_POINT ( 'NONE',  ( 14.62884502624119953, 1434.834865051830093, 190.3726805430140132 ) ) ;
#59108=CARTESIAN_POINT ( 'NONE',  ( -0.3094189819459999824, 1415.413778627430020, 233.4271496902980232 ) ) ;
#59109=CARTESIAN_POINT ( 'NONE',  ( -11.43185072513739797, 1443.913060387330006, 147.9056598087979921 ) ) ;
#59110=CARTESIAN_POINT ( 'NONE',  ( -28.30491477860000060, 1508.660124211329958, 209.1318398264210145 ) ) ;
#59111=B_SPLINE_SURFACE_WITH_KNOTS ( 'NONE', 5, 4, ( 
 ( #101825, #52011, #33515, #32975, #84493 ),
 ( #43058, #17256, #16703, #77216, #86151 ),
 ( #50903, #9444, #92888, #51448, #43608 ),
 ( #93434, #94536, #24008, #16164, #85034 ),
 ( #59322, #66623, #67715, #24561, #41947 ),
 ( #34644, #85579, #8326, #92331, #68828 ) ),
 .UNSPECIFIED., .F., .F., .F.,
 ( 6, 6 ),
 ( 5, 5 ),
 ( 0.000000000000000000, 52.98902693510000006 ),
 ( 40.20365518519999881, 50.26548245740000453 ),
 .UNSPECIFIED. ) ;
#59114=CARTESIAN_POINT ( 'NONE',  ( 44.93136303398450337, 1440.913046276439900, 269.6838066906610152 ) ) ;
#59115=CARTESIAN_POINT ( 'NONE',  ( -17.35680393429759860, 1451.072033954267226, 148.0582205165680705 ) ) ;
#59116=CARTESIAN_POINT ( 'NONE',  ( -22.86388144358860330, 1435.295931049460023, 134.1000000049170069 ) ) ;
#59117=CARTESIAN_POINT ( 'NONE',  ( 25.71088399069999753, 1436.647695531819863, 137.0958841102980159 ) ) ;
#59118=EDGE_CURVE ( 'NONE', #84300, #45857, #56121, .T. ) ;
#59119=CARTESIAN_POINT ( 'NONE',  ( -13.02011975896744111, 1442.961602265839474, 169.4183208322911582 ) ) ;
#59120=ORIENTED_EDGE ( 'NONE', *, *, #83912, .T. ) ;
#59122=CARTESIAN_POINT ( 'NONE',  ( -0.3551244063711440080, 1416.218047878440075, 191.1510195321629908 ) ) ;
#59123=ADVANCED_FACE ( 'NONE', ( #74033 ), #49379, .F. ) ;
#59124=CARTESIAN_POINT ( 'NONE',  ( 21.38848997940215924, 1509.000357915978839, 226.3836373717206527 ) ) ;
#59125=VERTEX_POINT ( 'NONE', #83505 ) ;
#59130=CARTESIAN_POINT ( 'NONE',  ( -3.627898411379999910, 1459.479586690430096, 211.7966661443780083 ) ) ;
#59132=CARTESIAN_POINT ( 'NONE',  ( 4.243141308438709736, 1425.234291684319942, 185.3368633770080010 ) ) ;
#59133=EDGE_CURVE ( 'NONE', #106936, #50244, #41869, .T. ) ;
#59135=CARTESIAN_POINT ( 'NONE',  ( -2.586211294052060072, 1420.639117752620450, 185.6985776663195509 ) ) ;
#59137=CARTESIAN_POINT ( 'NONE',  ( -24.66478414839999900, 1440.651724578850235, 210.6803367953379791 ) ) ;
#59139=CARTESIAN_POINT ( 'NONE',  ( 2.054351737509999776, 1450.909068314819933, 183.2085949937979876 ) ) ;
#59141=ADVANCED_FACE ( 'NONE', ( #21928 ), #40409, .T. ) ;
#59142=CARTESIAN_POINT ( 'NONE',  ( -27.88347671565054497, 1509.998607907042697, 220.2191159836331735 ) ) ;
#59144=CARTESIAN_POINT ( 'NONE',  ( -2.787097905305880323E-09, 1415.115138440810142, 244.0122842078770020 ) ) ;
#59145=ORIENTED_EDGE ( 'NONE', *, *, #86680, .F. ) ;
#59148=CARTESIAN_POINT ( 'NONE',  ( -2.760778634279479782, 1409.009468901610035, 188.0459411385839985 ) ) ;
#59149=CARTESIAN_POINT ( 'NONE',  ( -6.198205771480000514, 1471.106402530630021, 269.3395160832980082 ) ) ;
#59153=CARTESIAN_POINT ( 'NONE',  ( -13.58268883541719951, 1416.851343898680170, 221.9096085506480165 ) ) ;
#59158=CARTESIAN_POINT ( 'NONE',  ( -18.82370638324319856, 1408.747051114209853, 268.3329375438490274 ) ) ;
#59159=CARTESIAN_POINT ( 'NONE',  ( -13.60407173860000007, 1435.200345218290067, 149.7125188640980014 ) ) ;
#59162=EDGE_CURVE ( 'NONE', #55526, #22209, #31102, .T. ) ;
#59163=CARTESIAN_POINT ( 'NONE',  ( 13.49221535360000068, 1444.360430239190009, 188.3140289464980128 ) ) ;
#59165=ORIENTED_EDGE ( 'NONE', *, *, #74475, .F. ) ;
#59166=CARTESIAN_POINT ( 'NONE',  ( -22.04844205606989149, 1506.512156832672417, 209.1936639346002949 ) ) ;
#59170=CARTESIAN_POINT ( 'NONE',  ( -13.12714717100000072, 1470.463974201930114, 186.8692217856980164 ) ) ;
#59171=AXIS2_PLACEMENT_3D ( 'NONE', #46526, #64428, #21261 ) ;
#59173=VERTEX_POINT ( 'NONE', #42620 ) ;
#59176=CARTESIAN_POINT ( 'NONE',  ( -27.42461697039999891, 1509.627276150529951, 202.3633461635780009 ) ) ;
#59177=CARTESIAN_POINT ( 'NONE',  ( 1.418617516391186495, 1507.072688282607032, 236.8007530455898006 ) ) ;
#59179=CARTESIAN_POINT ( 'NONE',  ( -2.658297512749999925, 1408.468078491630195, 195.7434692079979754 ) ) ;
#59180=AXIS2_PLACEMENT_3D ( 'NONE', #99546, #32896, #50291 ) ;
#59182=CARTESIAN_POINT ( 'NONE',  ( 15.56983241408575580, 1506.527232289068252, 193.4924744589925183 ) ) ;
#59184=CARTESIAN_POINT ( 'NONE',  ( -24.99664572855169808, 1430.498658011320231, 209.0631888998489956 ) ) ;
#59185=CARTESIAN_POINT ( 'NONE',  ( 26.66951752199999959, 1488.685949850129873, 212.9498159561979946 ) ) ;
#59193=DIRECTION ( 'NONE',  ( 1.000000000000000000, 0.000000000000000000, 0.000000000000000000 ) ) ;
#59196=EDGE_LOOP ( 'NONE', ( #95966, #48724, #77152, #19061, #47855 ) ) ;
#59200=ORIENTED_EDGE ( 'NONE', *, *, #31011, .T. ) ;
#59203=CARTESIAN_POINT ( 'NONE',  ( -23.97468780672586774, 1509.756983508501435, 226.3117272632610479 ) ) ;
#59204=CARTESIAN_POINT ( 'NONE',  ( -4.087001431972547394, 1440.394582734599453, 185.3240461973863660 ) ) ;
#59206=CARTESIAN_POINT ( 'NONE',  ( -11.41042431937685819, 1425.708686112080841, 138.9044708858078820 ) ) ;
#59211=LINE ( 'NONE', #14411, #94210 ) ;
#59212=CARTESIAN_POINT ( 'NONE',  ( 20.06869819519999965, 1507.849569125829930, 189.2236336047979819 ) ) ;
#59215=CARTESIAN_POINT ( 'NONE',  ( -12.45702696549999899, 1416.837177087930058, 194.7670149573980041 ) ) ;
#59218=CARTESIAN_POINT ( 'NONE',  ( 1.148639102450000005, 1420.599583713030142, 184.1279056854980070 ) ) ;
#59219=( BOUNDED_CURVE ( )  B_SPLINE_CURVE ( 3, ( #37218, #71961, #29351, #63551 ),
 .UNSPECIFIED., .F., .F. ) 
 B_SPLINE_CURVE_WITH_KNOTS ( ( 4, 4 ),
 ( 2.890157810870130017, 3.288561387820169823 ),
 .UNSPECIFIED. ) 
 CURVE ( )  GEOMETRIC_REPRESENTATION_ITEM ( )  RATIONAL_B_SPLINE_CURVE ( ( 1.000000000000000000, 0.9868165638355377300, 0.9868165638355377300, 1.000000000000000000 ) ) 
 REPRESENTATION_ITEM ( '' )  );
#59223=FACE_OUTER_BOUND ( 'NONE', #91076, .T. ) ;
#59226=CARTESIAN_POINT ( 'NONE',  ( 17.02668221408760019, 1422.112876149069962, 226.8213126862850118 ) ) ;
#59227=CARTESIAN_POINT ( 'NONE',  ( 18.02574679518840028, 1424.482682570480165, 224.6196048480980210 ) ) ;
#59229=CARTESIAN_POINT ( 'NONE',  ( -7.362632729190000447, 1435.943783413959864, 149.6281905168980302 ) ) ;
#59230=CARTESIAN_POINT ( 'NONE',  ( 40.29567722275079689, 1440.913060362669967, 259.7007748391999939 ) ) ;
#59236=CARTESIAN_POINT ( 'NONE',  ( 1.547965266439779830, 1416.384967866679972, 190.2939387135980098 ) ) ;
#59237=CARTESIAN_POINT ( 'NONE',  ( -8.899876699774402766, 1506.575639936663492, 229.3526251636746167 ) ) ;
#59238=CARTESIAN_POINT ( 'NONE',  ( -27.70374316190000030, 1507.991978473030031, 210.5564529905680047 ) ) ;
#59241=CARTESIAN_POINT ( 'NONE',  ( 27.55277507892554212, 1509.987269819408084, 220.9896407951380581 ) ) ;
#59243=CARTESIAN_POINT ( 'NONE',  ( 13.15726447020000123, 1414.996442546130083, 197.7616625855980033 ) ) ;
#59245=CARTESIAN_POINT ( 'NONE',  ( -0.04349597063549999476, 1452.084370640529869, 153.9873413333980068 ) ) ;
#59250=VERTEX_POINT ( 'NONE', #2842 ) ;
#59251=CARTESIAN_POINT ( 'NONE',  ( -1.228956895969999907, 1451.852644323129880, 183.6261370569979761 ) ) ;
#59253=ADVANCED_FACE ( 'NONE', ( #1743 ), #79001, .T. ) ;
#59255=VERTEX_POINT ( 'NONE', #78431 ) ;
#59257=CARTESIAN_POINT ( 'NONE',  ( 19.75505552754349736, 1509.267941800199878, 230.0092462747840045 ) ) ;
#59265=VECTOR ( 'NONE', #4695, 1000.000000000000000 ) ;
#59268=CARTESIAN_POINT ( 'NONE',  ( 4.099770245750000264, 1409.056227519030017, 187.5794659243979936 ) ) ;
#59271=CARTESIAN_POINT ( 'NONE',  ( -2.704712804207050070, 1440.782885268830114, 168.7248546753820051 ) ) ;
#59272=EDGE_CURVE ( 'NONE', #104782, #90951, #57894, .T. ) ;
#59273=CARTESIAN_POINT ( 'NONE',  ( -21.74667324010000158, 1452.010995276330050, 142.8652655935979965 ) ) ;
#59274=CARTESIAN_POINT ( 'NONE',  ( 0.3090117147110000295, 1467.131542599430077, 235.6271451561979973 ) ) ;
#59275=VERTEX_POINT ( 'NONE', #36415 ) ;
#59277=CARTESIAN_POINT ( 'NONE',  ( 2.632631803615880450, 1417.642869435429930, 234.7516633181379859 ) ) ;
#59280=CARTESIAN_POINT ( 'NONE',  ( 17.29256643469999943, 1488.208383692229972, 189.1286988683980042 ) ) ;
#59281=AXIS2_PLACEMENT_3D ( 'NONE', #90704, #100746, #22374 ) ;
#59282=CARTESIAN_POINT ( 'NONE',  ( -1.943334382303870373E-12, 1470.170431109869924, 254.4737176916079875 ) ) ;
#59284=CARTESIAN_POINT ( 'NONE',  ( -1.163296394699999903, 1415.996778985530000, 227.8825576561980313 ) ) ;
#59285=CARTESIAN_POINT ( 'NONE',  ( -23.67893809570000130, 1435.763822560270000, 211.7787295027080177 ) ) ;
#59289=CARTESIAN_POINT ( 'NONE',  ( -0.2553961933194452971, 1485.936309581204569, 181.8381039734772742 ) ) ;
#59291=CARTESIAN_POINT ( 'NONE',  ( -45.56241648270140132, 1438.493849736420088, 266.1915599396410244 ) ) ;
#59297=EDGE_CURVE ( 'NONE', #51052, #10764, #99016, .T. ) ;
#59298=EDGE_CURVE ( 'NONE', #110603, #68835, #8276, .T. ) ;
#59302=CARTESIAN_POINT ( 'NONE',  ( -26.60536840204009934, 1451.234345923490082, 136.3028184666089828 ) ) ;
#59304=CARTESIAN_POINT ( 'NONE',  ( 29.87497007650000214, 1440.913060390719920, 238.0574376938980095 ) ) ;
#59307=ADVANCED_FACE ( 'NONE', ( #38073 ), #49234, .T. ) ;
#59308=CARTESIAN_POINT ( 'NONE',  ( -2.309563177363039621, 1419.513509509170035, 186.0127616851229959 ) ) ;
#59309=CARTESIAN_POINT ( 'NONE',  ( 15.81201445386249915, 1506.433683730510211, 224.3933755863170063 ) ) ;
#59310=CARTESIAN_POINT ( 'NONE',  ( -4.438186827019999854E-16, 1395.913060387330006, 217.1218459616979999 ) ) ;
#59311=LINE ( 'NONE', #92876, #24855 ) ;
#59312=CARTESIAN_POINT ( 'NONE',  ( -18.95816156469999925, 1416.822692809329965, 207.7797354902180018 ) ) ;
#59314=CARTESIAN_POINT ( 'NONE',  ( -4.184099373191500604, 1410.387155536230011, 269.6167533213169349 ) ) ;
#59315=CARTESIAN_POINT ( 'NONE',  ( 12.29573117529999848, 1419.871834229630167, 229.5356804718979902 ) ) ;
#59319=CARTESIAN_POINT ( 'NONE',  ( -23.67543694167489932, 1410.417538101999980, 210.0557992214939986 ) ) ;
#59320=CARTESIAN_POINT ( 'NONE',  ( -0.9956478785452340663, 1409.114994574759976, 186.0079330497359820 ) ) ;
#59321=DIRECTION ( 'NONE',  ( -0.7071067811865475727, 0.000000000000000000, 0.7071067811865475727 ) ) ;
#59322=CARTESIAN_POINT ( 'NONE',  ( -2.244413413239999766, 1428.081157166129969, 101.8807690336980016 ) ) ;
#59324=CARTESIAN_POINT ( 'NONE',  ( -20.64441152918609745, 1495.412616601870241, 192.5697118770649752 ) ) ;
#59325=CARTESIAN_POINT ( 'NONE',  ( -22.54740219580000016, 1410.868171134329941, 211.9285665470380025 ) ) ;
#59326=CARTESIAN_POINT ( 'NONE',  ( 32.78481868098219820, 1465.118709357260059, 269.1179671746619988 ) ) ;
#59327=CARTESIAN_POINT ( 'NONE',  ( -1.378966749891139987, 1424.159261042490016, 228.3819189927079947 ) ) ;
#59328=B_SPLINE_CURVE_WITH_KNOTS ( 'NONE', 3,
 ( #9508, #93501, #61057, #77285, #16773, #17885 ),
 .UNSPECIFIED., .F., .F.,
 ( 4, 2, 4 ),
 ( 1.348463003743570024E-05, 0.01516384436121859941, 0.03032162875772679775 ),
 .UNSPECIFIED. ) ;
#59331=CARTESIAN_POINT ( 'NONE',  ( 18.69185951995306993, 1458.324745879651800, 227.3668699999246883 ) ) ;
#59333=B_SPLINE_CURVE_WITH_KNOTS ( 'NONE', 3,
 ( #62063, #97285, #11093, #20557, #80500, #37946, #72127, #29528, #12734, #45260 ),
 .UNSPECIFIED., .F., .F.,
 ( 4, 2, 2, 2, 4 ),
 ( 0.000000000000000000, 0.2500000000000000000, 0.5000000000000000000, 0.7500000000000000000, 1.000000000000000000 ),
 .UNSPECIFIED. ) ;
#59341=CARTESIAN_POINT ( 'NONE',  ( 22.40106396050000015, 1409.695322778229865, 210.5405262121579995 ) ) ;
#59344=CARTESIAN_POINT ( 'NONE',  ( 2.053713886625649909, 1408.984777656559800, 186.9425993992589952 ) ) ;
#59345=CARTESIAN_POINT ( 'NONE',  ( 1.461041045310000008, 1417.190561156129888, 233.6733459660979975 ) ) ;
#59350=CARTESIAN_POINT ( 'NONE',  ( 11.84704892624298012, 1420.366920634892949, 231.7806654029725735 ) ) ;
#59352=CARTESIAN_POINT ( 'NONE',  ( 13.01305160761890001, 1416.520646088589956, 221.6242373452080017 ) ) ;
#59353=CARTESIAN_POINT ( 'NONE',  ( 0.000000000000000000, 1405.413060387330006, 209.1218459616979999 ) ) ;
#59357=CARTESIAN_POINT ( 'NONE',  ( -35.61939005354069820, 1450.149788447230094, 136.2352736447359973 ) ) ;
#59358=CARTESIAN_POINT ( 'NONE',  ( 13.40566205669149902, 1429.098591087019940, 222.0107402452829888 ) ) ;
#59360=CARTESIAN_POINT ( 'NONE',  ( 1.021405182659999929E-14, 1469.463552837929910, 265.6112251771979800 ) ) ;
#59361=CARTESIAN_POINT ( 'NONE',  ( -21.03615331023111068, 1508.023275259974525, 192.1677045215957662 ) ) ;
#59362=CARTESIAN_POINT ( 'NONE',  ( 11.11327778789999954, 1433.557389433600065, 151.6749141554979872 ) ) ;
#59363=CARTESIAN_POINT ( 'NONE',  ( 2.886579864029999753E-15, 1458.952956299430070, 234.3916895801979763 ) ) ;
#59364=CARTESIAN_POINT ( 'NONE',  ( 11.87146819884729965, 1414.971390223329990, 197.3742744802259779 ) ) ;
#59368=CARTESIAN_POINT ( 'NONE',  ( -19.45240832520000041, 1485.997265531630092, 190.0281968953979970 ) ) ;
#59369=LINE ( 'NONE', #109748, #50315 ) ;
#59370=CARTESIAN_POINT ( 'NONE',  ( -7.546382087207799572, 1509.216843681829914, 238.8694033275340018 ) ) ;
#59372=CARTESIAN_POINT ( 'NONE',  ( 21.12097961079999919, 1430.346877874630081, 219.8772875276980017 ) ) ;
#59374=CARTESIAN_POINT ( 'NONE',  ( -3.469833849039999683E-16, 1426.566393376330097, 144.1938086916980239 ) ) ;
#59380=AXIS2_PLACEMENT_3D ( 'NONE', #80768, #29802, #80216 ) ;
#59381=CARTESIAN_POINT ( 'NONE',  ( 0.1698047298984949882, 1480.444372444690089, 182.0753023306870091 ) ) ;
#59382=CARTESIAN_POINT ( 'NONE',  ( -2.881142919476630038, 1408.476254411279797, 222.6699509515860029 ) ) ;
#59383=ORIENTED_EDGE ( 'NONE', *, *, #72276, .T. ) ;
#59386=CARTESIAN_POINT ( 'NONE',  ( 12.40400603319999817, 1434.420125459849942, 149.7889667278979857 ) ) ;
#59387=CARTESIAN_POINT ( 'NONE',  ( -41.53765979145569531, 1445.128430570340015, 134.0999999984609872 ) ) ;
#59392=CARTESIAN_POINT ( 'NONE',  ( -15.32781675520000064, 1414.971279908829956, 216.4146992301180035 ) ) ;
#59402=ORIENTED_EDGE ( 'NONE', *, *, #9707, .F. ) ;
#59403=CARTESIAN_POINT ( 'NONE',  ( -28.53738135360000072, 1451.916516915729972, 134.8736009463979997 ) ) ;
#59404=CARTESIAN_POINT ( 'NONE',  ( 13.51812398686129590, 1443.501467202829645, 169.4008117781763190 ) ) ;
#59412=EDGE_CURVE ( 'NONE', #101169, #575, #106942, .T. ) ;
#59415=CARTESIAN_POINT ( 'NONE',  ( 16.00594386000976499, 1431.827458374873913, 218.6954846823096830 ) ) ;
#59416=CARTESIAN_POINT ( 'NONE',  ( 1.467367638679999864, 1417.074472501330092, 233.2101326662979659 ) ) ;
#59418=CARTESIAN_POINT ( 'NONE',  ( -20.58241815119903961, 1507.840888067528340, 228.3121511827991696 ) ) ;
#59419=CARTESIAN_POINT ( 'NONE',  ( 4.255689356150000435, 1519.913060387329779, 231.5674970370980077 ) ) ;
#59422=CARTESIAN_POINT ( 'NONE',  ( 4.220206612560000181, 1446.210882134419990, 168.9980572354979813 ) ) ;
#59423=CARTESIAN_POINT ( 'NONE',  ( -2.500000000000000000, 1437.234369398040144, 157.6522023233980008 ) ) ;
#59427=CARTESIAN_POINT ( 'NONE',  ( -6.232532191338900240, 1398.098440470949981, 197.7132727547819968 ) ) ;
#59430=CARTESIAN_POINT ( 'NONE',  ( -24.85895335939999740, 1430.362482304829882, 208.4345430527690155 ) ) ;
#59431=CARTESIAN_POINT ( 'NONE',  ( -11.15980475191650001, 1426.466872868450082, 102.3027272071919924 ) ) ;
#59432=CARTESIAN_POINT ( 'NONE',  ( 16.84651400299079782, 1409.747734344990022, 192.6928343578630063 ) ) ;
#59434=ADVANCED_FACE ( 'NONE', ( #23464 ), #65306, .F. ) ;
#59435=CARTESIAN_POINT ( 'NONE',  ( 21.09276969954263947, 1509.766718187257993, 187.7199361994491937 ) ) ;
#59439=CARTESIAN_POINT ( 'NONE',  ( 15.16658111565280009, 1509.443839351920133, 234.3011174550109956 ) ) ;
#59442=CARTESIAN_POINT ( 'NONE',  ( -38.82359025196139868, 1439.487870305959859, 136.6807876477819832 ) ) ;
#59443=VERTEX_POINT ( 'NONE', #58191 ) ;
#59444=CARTESIAN_POINT ( 'NONE',  ( 9.441477048479999468, 1396.242764029729869, 201.4775236043080042 ) ) ;
#59446=CARTESIAN_POINT ( 'NONE',  ( -18.37698674530000176, 1457.555359684630048, 228.2935531249980272 ) ) ;
#59447=ORIENTED_EDGE ( 'NONE', *, *, #22789, .T. ) ;
#59449=CARTESIAN_POINT ( 'NONE',  ( -29.43467078477432253, 1509.947524417930026, 211.2629717639432840 ) ) ;
#59456=CARTESIAN_POINT ( 'NONE',  ( -14.28760104070000025, 1461.186940285030005, 229.6152737784979934 ) ) ;
#59457=CARTESIAN_POINT ( 'NONE',  ( 21.97938480441199971, 1506.433683733499947, 208.7396655020440051 ) ) ;
#59459=CARTESIAN_POINT ( 'NONE',  ( 17.22592475669953416, 1443.501467202839649, 162.9227486557969655 ) ) ;
#59465=CARTESIAN_POINT ( 'NONE',  ( 11.06583617892839833, 1414.913527292460003, 222.2283161299670269 ) ) ;
#59467=EDGE_LOOP ( 'NONE', ( #108311, #51598, #5438 ) ) ;
#59468=CARTESIAN_POINT ( 'NONE',  ( -14.15450645269999974, 1415.628674276829770, 221.0805609275980146 ) ) ;
#59469=CARTESIAN_POINT ( 'NONE',  ( -11.45640830748399885, 1432.340941395319987, 151.2730090707190129 ) ) ;
#59472=CARTESIAN_POINT ( 'NONE',  ( -4.533058655030000494, 1424.018048896529990, 185.2641154658980156 ) ) ;
#59473=CARTESIAN_POINT ( 'NONE',  ( 14.59277107062129986, 1436.244837967300100, 149.8707660814949918 ) ) ;
#59475=CARTESIAN_POINT ( 'NONE',  ( -2.923521517025829741, 1410.394928878200062, 186.6127595807840009 ) ) ;
#59477=CARTESIAN_POINT ( 'NONE',  ( -16.28504566760000216, 1496.371285614329963, 224.3646236400980172 ) ) ;
#59478=CARTESIAN_POINT ( 'NONE',  ( 17.33021867909999969, 1458.353808689130119, 229.6040141600979894 ) ) ;
#59480=CARTESIAN_POINT ( 'NONE',  ( -4.989978619240677205, 1423.182856176245650, 184.7654884127948094 ) ) ;
#59481=CARTESIAN_POINT ( 'NONE',  ( -2.499952938216249976, 1420.029941299070060, 100.9689851914940135 ) ) ;
#59482=EDGE_LOOP ( 'NONE', ( #61704, #24381, #3145, #27619 ) ) ;
#59490=CARTESIAN_POINT ( 'NONE',  ( 1.336626035159999892, 1434.994518313450044, 189.3609647309980062 ) ) ;
#59492=CARTESIAN_POINT ( 'NONE',  ( -11.50995325589999929, 1427.639127959429970, 149.3376616764980156 ) ) ;
#59493=CARTESIAN_POINT ( 'NONE',  ( -10.91327520126305117, 1428.362630744280750, 150.6705834258702907 ) ) ;
#59494=CARTESIAN_POINT ( 'NONE',  ( -5.772970091560000405, 1439.947079492359990, 185.7689619320979943 ) ) ;
#59495=FACE_OUTER_BOUND ( 'NONE', #78140, .T. ) ;
#59497=CARTESIAN_POINT ( 'NONE',  ( -24.52682765429999634, 1495.363418884229986, 219.7720737364980153 ) ) ;
#59499=CARTESIAN_POINT ( 'NONE',  ( -16.78746488157599970, 1460.262648982494056, 228.3352623233340069 ) ) ;
#59500=ORIENTED_EDGE ( 'NONE', *, *, #27571, .F. ) ;
#59502=CARTESIAN_POINT ( 'NONE',  ( 18.39953948240000159, 1408.534890842129926, 267.7101522853979532 ) ) ;
#59503=DIRECTION ( 'NONE',  ( -1.000000000000000000, 0.000000000000000000, 0.000000000000000000 ) ) ;
#59504=CARTESIAN_POINT ( 'NONE',  ( 20.03780167889999930, 1430.300308916730046, 195.4616010020980070 ) ) ;
#59506=CARTESIAN_POINT ( 'NONE',  ( 0.06174575640759859957, 1508.562174490289863, 237.9142381842480063 ) ) ;
#59509=CARTESIAN_POINT ( 'NONE',  ( 12.32422840039999912, 1461.784851115730135, 233.7517049971980043 ) ) ;
#59511=CARTESIAN_POINT ( 'NONE',  ( -13.45215185470000030, 1444.587159410089953, 187.5992218171979857 ) ) ;
#59512=CARTESIAN_POINT ( 'NONE',  ( -19.47227132649999959, 1453.313060387329870, 212.8011186786780229 ) ) ;
#59516=CARTESIAN_POINT ( 'NONE',  ( 1.454477355351579959, 1501.339712585870075, 181.3651619459799917 ) ) ;
#59517=CARTESIAN_POINT ( 'NONE',  ( -10.85260544259019966, 1409.292041720379984, 198.8351549789040007 ) ) ;
#59520=CARTESIAN_POINT ( 'NONE',  ( -18.35025482799999708, 1473.149480673029984, 267.0969222196980013 ) ) ;
#59522=CARTESIAN_POINT ( 'NONE',  ( -20.99310762600000047, 1509.712614273529880, 187.9175820947980071 ) ) ;
#59523=CARTESIAN_POINT ( 'NONE',  ( -24.08371411292216280, 1444.410970683369897, 211.9273017543515039 ) ) ;
#59526=CARTESIAN_POINT ( 'NONE',  ( -3.663735981259999979E-15, 1440.444625599219989, 155.6821044880979912 ) ) ;
#59530=CARTESIAN_POINT ( 'NONE',  ( -23.04389186530000089, 1409.882248337629790, 206.7352832536480207 ) ) ;
#59531=DIRECTION ( 'NONE',  ( 0.000000000000000000, 1.000000000000000000, 0.000000000000000000 ) ) ;
#59538=CARTESIAN_POINT ( 'NONE',  ( -21.20067971809999818, 1409.653404436829760, 211.3910486286680168 ) ) ;
#59540=CARTESIAN_POINT ( 'NONE',  ( 11.73426358108639889, 1426.697716059430149, 143.9718653054989943 ) ) ;
#59543=B_SPLINE_CURVE_WITH_KNOTS ( 'NONE', 5,
 ( #6180, #24606, #15116, #32497, #14017, #100773, #48207, #66670, #58800 ),
 .UNSPECIFIED., .F., .F.,
 ( 6, 3, 6 ),
 ( 0.000000000000000000, 0.5050532947624984947, 1.000000000000000000 ),
 .UNSPECIFIED. ) ;
#59545=CARTESIAN_POINT ( 'NONE',  ( -17.22174736099490033, 1507.619498584509984, 224.3333391233730083 ) ) ;
#59547=CARTESIAN_POINT ( 'NONE',  ( -11.72661338454730640, 1398.260517928511490, 214.9127125651629058 ) ) ;
#59550=CARTESIAN_POINT ( 'NONE',  ( 1.441485945039999939, 1507.073353643630071, 236.7786021845980144 ) ) ;
#59555=CARTESIAN_POINT ( 'NONE',  ( 11.55278678904199907, 1434.349239717640103, 151.3337279177310108 ) ) ;
#59556=CARTESIAN_POINT ( 'NONE',  ( -13.31309558959999961, 1398.000656151930116, 207.3565362264480143 ) ) ;
#59562=CARTESIAN_POINT ( 'NONE',  ( -13.89790203009249936, 1508.842249044219898, 183.8389499564130176 ) ) ;
#59563=CARTESIAN_POINT ( 'NONE',  ( 2.854897837073400169, 1498.106740913580097, 235.5480816206879808 ) ) ;
#59564=( BOUNDED_CURVE ( )  B_SPLINE_CURVE ( 3, ( #59923, #52067, #75618, #94042 ),
 .UNSPECIFIED., .F., .T. ) 
 B_SPLINE_CURVE_WITH_KNOTS ( ( 4, 4 ),
 ( 4.177898707858459737, 5.246900984146320113 ),
 .UNSPECIFIED. ) 
 CURVE ( )  GEOMETRIC_REPRESENTATION_ITEM ( )  RATIONAL_B_SPLINE_CURVE ( ( 1.000000000000000000, 0.9070152416445715904, 0.9070152416445715904, 1.000000000000000000 ) ) 
 REPRESENTATION_ITEM ( '' )  );
#59565=CARTESIAN_POINT ( 'NONE',  ( 1.520031180769999990, 1468.707239051229863, 182.7929238198979931 ) ) ;
#59567=CARTESIAN_POINT ( 'NONE',  ( 15.48869622149999969, 1409.453937571630149, 226.0647739019979952 ) ) ;
#59569=CARTESIAN_POINT ( 'NONE',  ( 2.753170620192659790, 1396.009203223909935, 198.4539142632749815 ) ) ;
#59570=CARTESIAN_POINT ( 'NONE',  ( 33.91369120210129751, 1435.681798817170147, 134.0999999980979851 ) ) ;
#59571=CARTESIAN_POINT ( 'NONE',  ( 11.86160965589999883, 1432.010073915890189, 150.3887981409980057 ) ) ;
#59573=ORIENTED_EDGE ( 'NONE', *, *, #22111, .F. ) ;
#59574=CARTESIAN_POINT ( 'NONE',  ( 13.68681530539999969, 1435.283985230760209, 149.7729792379979870 ) ) ;
#59575=VERTEX_POINT ( 'NONE', #16693 ) ;
#59578=CARTESIAN_POINT ( 'NONE',  ( 13.51596914371239500, 1443.950082444225018, 169.3503480695792121 ) ) ;
#59579=CARTESIAN_POINT ( 'NONE',  ( -4.248356950199999815, 1464.543264781329981, 236.4384044122979844 ) ) ;
#59580=CARTESIAN_POINT ( 'NONE',  ( -13.29011429918680065, 1407.447342471949923, 210.5442722391819927 ) ) ;
#59584=CARTESIAN_POINT ( 'NONE',  ( 2.500000000000000000, 1448.283969051469967, 164.7257521935120224 ) ) ;
#59589=CARTESIAN_POINT ( 'NONE',  ( 22.20198509923669761, 1440.913060387330006, 228.2955218435759832 ) ) ;
#59591=CARTESIAN_POINT ( 'NONE',  ( -19.27289889490000263, 1509.486203086629985, 230.8709054965979988 ) ) ;
#59592=CARTESIAN_POINT ( 'NONE',  ( -10.55778742260000058, 1409.281746448229796, 190.1804069070979892 ) ) ;
#59594=CARTESIAN_POINT ( 'NONE',  ( -1.457047359353270011, 1414.913057819779851, 226.2719804722950130 ) ) ;
#59596=CARTESIAN_POINT ( 'NONE',  ( 23.06896861730000126, 1432.937351989309946, 217.3496264744780149 ) ) ;
#59602=CARTESIAN_POINT ( 'NONE',  ( 22.99941532620000118, 1409.742488423629993, 209.3674398474389875 ) ) ;
#59603=CARTESIAN_POINT ( 'NONE',  ( -21.20923297919999584, 1509.358812534630033, 189.9045910904980019 ) ) ;
#59608=CARTESIAN_POINT ( 'NONE',  ( 43.50000000000000000, 1435.965051957929973, 271.1218459616979999 ) ) ;
#59609=CARTESIAN_POINT ( 'NONE',  ( 14.06591726819999977, 1410.775981654029920, 191.2779949321979984 ) ) ;
#59615=CARTESIAN_POINT ( 'NONE',  ( 32.79493994319999928, 1447.324624206830094, 248.1152222146980080 ) ) ;
#59616=EDGE_CURVE ( 'NONE', #59275, #43874, #75554, .T. ) ;
#59617=CARTESIAN_POINT ( 'NONE',  ( -29.16731927555590076, 1436.844791263991738, 136.7085273712292519 ) ) ;
#59619=EDGE_CURVE ( 'NONE', #66206, #84614, #29710, .T. ) ;
#59620=CARTESIAN_POINT ( 'NONE',  ( -8.313288157249999699, 1507.316777883029999, 235.1567909999980088 ) ) ;
#59621=CARTESIAN_POINT ( 'NONE',  ( -23.95707600360000100, 1445.781625871360120, 214.3999464195180167 ) ) ;
#59622=LINE ( 'NONE', #110014, #36179 ) ;
#59625=CARTESIAN_POINT ( 'NONE',  ( 17.57055179088690267, 1409.820984684919949, 222.6405620070939904 ) ) ;
#59628=ORIENTED_EDGE ( 'NONE', *, *, #35181, .T. ) ;
#59631=CARTESIAN_POINT ( 'NONE',  ( 27.87492299980000254, 1509.195406835429822, 207.4799702676380093 ) ) ;
#59632=CARTESIAN_POINT ( 'NONE',  ( 12.78776258910000152, 1416.851343903229917, 222.7045348341980002 ) ) ;
#59633=CARTESIAN_POINT ( 'NONE',  ( 38.41729418578510291, 1444.641748167779951, 137.0880170108979996 ) ) ;
#59638=CARTESIAN_POINT ( 'NONE',  ( 29.17442666288910047, 1435.515888873780113, 135.6503853385080163 ) ) ;
#59639=CARTESIAN_POINT ( 'NONE',  ( 40.06992063472939947, 1445.460187879419891, 136.8880302072950030 ) ) ;
#59640=CARTESIAN_POINT ( 'NONE',  ( -44.02689737971761730, 1450.201568725966808, 269.0198393128794692 ) ) ;
#59642=CARTESIAN_POINT ( 'NONE',  ( 14.53903903039999790, 1509.420774818030168, 184.2780880536979851 ) ) ;
#59647=EDGE_LOOP ( 'NONE', ( #77493, #73189, #97137, #57052, #27194 ) ) ;
#59653=CARTESIAN_POINT ( 'NONE',  ( 1.399926847669999974, 1507.072115598929940, 236.8180522793980174 ) ) ;
#59654=CARTESIAN_POINT ( 'NONE',  ( -0.4026299538800000022, 1417.288473575429862, 234.8326129995979841 ) ) ;
#59656=CARTESIAN_POINT ( 'NONE',  ( 13.15726447020000123, 1414.996442546130083, 197.7616625855980033 ) ) ;
#59657=CARTESIAN_POINT ( 'NONE',  ( -28.48686853690000120, 1509.161777456430173, 209.2972665594169825 ) ) ;
#59660=CARTESIAN_POINT ( 'NONE',  ( -7.910716753646842569, 1417.101719454672320, 230.9803857119551935 ) ) ;
#59662=CARTESIAN_POINT ( 'NONE',  ( -17.06443472855709942, 1415.088506334920112, 208.8111692386390246 ) ) ;
#59663=CARTESIAN_POINT ( 'NONE',  ( 25.76105412372420034, 1435.403606809190023, 135.5887298860220085 ) ) ;
#59664=CARTESIAN_POINT ( 'NONE',  ( -5.799069655498709785, 1396.115568362039767, 199.7279999695500123 ) ) ;
#59667=CARTESIAN_POINT ( 'NONE',  ( 21.30850089961481331, 1508.868632108111569, 226.3165434354574188 ) ) ;
#59669=VERTEX_POINT ( 'NONE', #41389 ) ;
#59672=CARTESIAN_POINT ( 'NONE',  ( 4.500000000000000000, 1423.874532569730036, 167.3087045231979744 ) ) ;
#59673=CARTESIAN_POINT ( 'NONE',  ( -23.79657349140000022, 1452.984769824329987, 231.7466849528980219 ) ) ;
#59675=CARTESIAN_POINT ( 'NONE',  ( -0.02433770998772320088, 1507.114569794609906, 237.3519378586950097 ) ) ;
#59677=CARTESIAN_POINT ( 'NONE',  ( -2.810123179937576765, 1419.851975481765294, 186.1424120031869052 ) ) ;
#59679=CARTESIAN_POINT ( 'NONE',  ( -24.71657962519999785, 1438.057265587329994, 210.4902010153179788 ) ) ;
#59681=CARTESIAN_POINT ( 'NONE',  ( 3.674243458920000371, 1449.362436213359842, 184.1757723556980011 ) ) ;
#59683=CARTESIAN_POINT ( 'NONE',  ( -29.78845675224144429, 1510.063610128411483, 205.2021543053915877 ) ) ;
#59686=ORIENTED_EDGE ( 'NONE', *, *, #95552, .T. ) ;
#59687=CARTESIAN_POINT ( 'NONE',  ( -11.77066367041570061, 1427.133876426280040, 146.4681802475080019 ) ) ;
#59690=CARTESIAN_POINT ( 'NONE',  ( -2.278119754840000066, 1472.579670685429846, 270.3712227850979843 ) ) ;
#59691=CARTESIAN_POINT ( 'NONE',  ( 12.55314581241474770, 1434.481572427596348, 147.2585247707476981 ) ) ;
#59694=CARTESIAN_POINT ( 'NONE',  ( 14.25730472222872258, 1435.139833118672186, 149.2707372188924921 ) ) ;
#59695=CARTESIAN_POINT ( 'NONE',  ( -14.69722372230000040, 1408.913060387329779, 199.0844487958979983 ) ) ;
#59698=CARTESIAN_POINT ( 'NONE',  ( -15.46198845756829954, 1407.981833872850075, 266.8669550737199643 ) ) ;
#59699=B_SPLINE_CURVE_WITH_KNOTS ( 'NONE', 3,
 ( #93069, #33164, #76282, #110430, #75740, #15781, #42132 ),
 .UNSPECIFIED., .F., .F.,
 ( 4, 3, 4 ),
 ( -157.7301682620000065, -100.4765180537589941, -30.40177460609999116 ),
 .UNSPECIFIED. ) ;
#59700=CARTESIAN_POINT ( 'NONE',  ( -13.80960823982659846, 1434.980805496569701, 148.6628371575099834 ) ) ;
#59703=CARTESIAN_POINT ( 'NONE',  ( 13.11558759679999930, 1445.024186261000068, 187.9997115717980023 ) ) ;
#59706=ADVANCED_FACE ( 'NONE', ( #77747 ), #53348, .F. ) ;
#59711=CARTESIAN_POINT ( 'NONE',  ( -16.44414657789999978, 1470.468951170730179, 188.6467452786979777 ) ) ;
#59712=CARTESIAN_POINT ( 'NONE',  ( -17.14890260233960362, 1507.633363089370050, 229.9813627781319951 ) ) ;
#59717=CARTESIAN_POINT ( 'NONE',  ( -28.34573470619999824, 1509.902915575630004, 201.4105953259380044 ) ) ;
#59718=CARTESIAN_POINT ( 'NONE',  ( -1.116639747240000036, 1477.815261412129985, 230.7657239923979944 ) ) ;
#59720=CARTESIAN_POINT ( 'NONE',  ( -5.082272206379999879, 1407.428259763930100, 197.0859678235980255 ) ) ;
#59722=CARTESIAN_POINT ( 'NONE',  ( -37.77042217320030204, 1442.790213540069999, 137.1073832721159818 ) ) ;
#59724=CARTESIAN_POINT ( 'NONE',  ( -24.98277631911100016, 1430.498769793900010, 209.4735117548389951 ) ) ;
#59725=CARTESIAN_POINT ( 'NONE',  ( 26.12765557829999707, 1469.244184476429837, 211.6578734458780104 ) ) ;
#59726=VECTOR ( 'NONE', #57792, 1000.000000000000000 ) ;
#59729=CARTESIAN_POINT ( 'NONE',  ( -23.61230847530000077, 1435.322064771759869, 137.2857865107980047 ) ) ;
#59733=CARTESIAN_POINT ( 'NONE',  ( -14.22059293429999904, 1415.601144549029868, 227.1159107520979887 ) ) ;
#59737=EDGE_LOOP ( 'NONE', ( #105577, #9363, #44538, #27599, #18641 ) ) ;
#59739=CARTESIAN_POINT ( 'NONE',  ( -1.034085896929999970, 1410.308950511429885, 233.0477810549980120 ) ) ;
#59740=CARTESIAN_POINT ( 'NONE',  ( -19.88336784562452664, 1456.648868693877375, 225.3973042494007757 ) ) ;
#59741=ORIENTED_EDGE ( 'NONE', *, *, #39759, .T. ) ;
#59744=CARTESIAN_POINT ( 'NONE',  ( 12.69471164485930004, 1434.997246021789806, 150.4091530359009994 ) ) ;
#59745=B_SPLINE_SURFACE_WITH_KNOTS ( 'NONE', 5, 5, ( 
 ( #38874, #97691, #89839, #73053, #55168, #54620, #98238, #82558, #106097, #65213, #14226, #13655, #30483, #89293, #64672, #97146, #46217, #4195, #38328, #105558, #80350, #98789, #22051, #5850, #20414, #106636, #12588 ),
 ( #46768, #73618, #13112, #28845, #56248, #29375, #71442, #22599, #29925, #80898, #81978, #63576, #5286, #3668, #107747, #99325, #56802, #88752, #37796, #72507, #76357, #75809, #109960, #74716, #67428, #6935, #84194 ),
 ( #41653, #24279, #50065, #25373, #39991, #100984, #101527, #32694, #110506, #8037, #31583, #65761, #85286, #41092, #33787, #14783, #93146, #84739, #109418, #108298, #99877, #91503, #83640, #75271, #74168, #48968, #33239 ),
 ( #66874, #40541, #67982, #108847, #93678, #66330, #42206, #58461, #23176, #92588, #32143, #57377, #102091, #15860, #49515, #24814, #100447, #7491, #83102, #59565, #59019, #16414, #50607, #16958, #51159, #6394, #23730 ),
 ( #57917, #92050, #15322, #86956, #8586, #10248, #103766, #18630, #104867, #42757, #69643, #70209, #1314, #44986, #87527, #226, #34352, #53950, #9694, #79134, #94242, #61792, #53380, #78008, #76918, #68527, #94810 ),
 ( #102626, #28156, #43862, #35454, #86406, #17517, #60125, #43321, #25927, #51718, #18086, #85855, #9156, #2442, #69085, #27068, #61252, #103186, #95367, #77467, #768, #10816, #34897, #52827, #95914, #26489, #44424 ) ),
 .UNSPECIFIED., .F., .F., .F.,
 ( 6, 6 ),
 ( 6, 3, 3, 3, 3, 3, 3, 3, 6 ),
 ( 1.603980125900000164, 99.04053975169999546 ),
 ( 27.66747965320000091, 34.17287967890000289, 36.60297779519999750, 37.81802685339999925, 38.42555138250000368, 39.03307591160000101, 39.44437685990000375, 39.85567780810000471, 40.67827970449999953 ),
 .UNSPECIFIED. ) ;
#59746=CARTESIAN_POINT ( 'NONE',  ( -4.085655924655085869, 1440.415659510594423, 185.3144063599575304 ) ) ;
#59748=CARTESIAN_POINT ( 'NONE',  ( -15.94347048536829803, 1409.469818645040050, 192.9752432267480060 ) ) ;
#59750=CARTESIAN_POINT ( 'NONE',  ( 28.15443155984639745, 1509.896245780209938, 217.4026704617729990 ) ) ;
#59751=DIRECTION ( 'NONE',  ( 0.000000000000000000, 0.000000000000000000, -1.000000000000000000 ) ) ;
#59752=CARTESIAN_POINT ( 'NONE',  ( 4.222470952326010440, 1441.596861596299959, 167.7009558891260212 ) ) ;
#59755=CARTESIAN_POINT ( 'NONE',  ( -3.998460401129999564, 1421.841081959129951, 184.4445580210980324 ) ) ;
#59756=CARTESIAN_POINT ( 'NONE',  ( 20.67635560069999912, 1509.397142797630067, 188.6960315703979916 ) ) ;
#59757=CARTESIAN_POINT ( 'NONE',  ( -4.406834599037237510, 1421.289441775209980, 144.1372251532988003 ) ) ;
#59763=CARTESIAN_POINT ( 'NONE',  ( 1.780863054839999959, 1419.796581447929839, 184.9705365426980279 ) ) ;
#59764=EDGE_CURVE ( 'NONE', #36772, #75744, #55135, .T. ) ;
#59770=FACE_OUTER_BOUND ( 'NONE', #56144, .T. ) ;
#59773=CARTESIAN_POINT ( 'NONE',  ( -9.690208402899999740, 1434.541746329560056, 148.7586030823979968 ) ) ;
#59774=CARTESIAN_POINT ( 'NONE',  ( 40.48639141129520169, 1440.913060360999907, 259.9639464203100374 ) ) ;
#59778=VERTEX_POINT ( 'NONE', #90541 ) ;
#59779=ORIENTED_EDGE ( 'NONE', *, *, #108896, .F. ) ;
#59782=CARTESIAN_POINT ( 'NONE',  ( -24.41216396249999931, 1440.964695643669984, 212.0310679874179982 ) ) ;
#59783=CARTESIAN_POINT ( 'NONE',  ( 6.688171886676422595, 1447.885435886052392, 185.1357882069593472 ) ) ;
#59784=CARTESIAN_POINT ( 'NONE',  ( -3.006969711954706526, 1425.989600909259252, 185.4751844751110923 ) ) ;
#59786=B_SPLINE_SURFACE_WITH_KNOTS ( 'NONE', 4, 5, ( 
 ( #48100, #55954, #98484, #57067, #13359, #31284 ),
 ( #5541, #39120, #39692, #21752, #47550, #63276 ),
 ( #14473, #30730, #48665, #97387, #64915, #20658 ),
 ( #54860, #50323, #66578, #23966, #83891, #40237 ),
 ( #57623, #67671, #74420, #83340, #40791, #25068 ) ),
 .UNSPECIFIED., .F., .F., .F.,
 ( 5, 5 ),
 ( 6, 6 ),
 ( 7.148411859579999472, 7.252819523530000367 ),
 ( 0.000000000000000000, 2.228199834939999846 ),
 .UNSPECIFIED. ) ;
#59787=CARTESIAN_POINT ( 'NONE',  ( 1.804213551060599885, 1410.351307734219972, 232.1928989352460064 ) ) ;
#59792=CARTESIAN_POINT ( 'NONE',  ( -28.17098632135910918, 1509.816547239969623, 212.1705146586627109 ) ) ;
#59793=CARTESIAN_POINT ( 'NONE',  ( -23.42685059075717646, 1410.407670574614940, 210.3305991070054972 ) ) ;
#59795=VERTEX_POINT ( 'NONE', #40145 ) ;
#59796=CARTESIAN_POINT ( 'NONE',  ( -1.270728227810000055, 1414.996442546230128, 226.4582995913979744 ) ) ;
#59798=CARTESIAN_POINT ( 'NONE',  ( 19.77866596905520069, 1507.914512822359939, 229.2835366231990122 ) ) ;
#59801=CARTESIAN_POINT ( 'NONE',  ( 17.32428483191130297, 1508.223220029260119, 230.9736489382000002 ) ) ;
#59802=DIRECTION ( 'NONE',  ( -0.4763271851929161138, 0.000000000000000000, 0.8792681119238848764 ) ) ;
#59803=CARTESIAN_POINT ( 'NONE',  ( 38.88009490570040327, 1439.559590605640096, 136.6872614661130001 ) ) ;
#59804=CARTESIAN_POINT ( 'NONE',  ( 21.49889961270000072, 1488.801231228130064, 209.3947183657330129 ) ) ;
#59805=SPHERICAL_SURFACE ( 'NONE', #44900, 2.000000000000000000 ) ;
#59812=CARTESIAN_POINT ( 'NONE',  ( 3.268551751039999953, 1410.404426152929773, 185.7978215306979735 ) ) ;
#59816=CARTESIAN_POINT ( 'NONE',  ( -4.263072128268690086, 1441.226134037160136, 159.2129237521010054 ) ) ;
#59818=CARTESIAN_POINT ( 'NONE',  ( -2.743100966568880139, 1450.921041808649989, 184.6046904293359887 ) ) ;
#59819=CARTESIAN_POINT ( 'NONE',  ( 0.6879682657500000298, 1464.995962445229907, 237.3245376353980021 ) ) ;
#59820=ORIENTED_EDGE ( 'NONE', *, *, #54775, .T. ) ;
#59822=CARTESIAN_POINT ( 'NONE',  ( -42.42054896300000166, 1443.932089742500011, 270.0676470778980161 ) ) ;
#59823=CARTESIAN_POINT ( 'NONE',  ( -23.69928159108154375, 1436.231577400298420, 212.2790965043357403 ) ) ;
#59825=CARTESIAN_POINT ( 'NONE',  ( 15.05055690159999848, 1410.738883364130061, 191.5204107739980088 ) ) ;
#59827=CARTESIAN_POINT ( 'NONE',  ( 22.41589833909626606, 1436.510086781942846, 142.7382537882818099 ) ) ;
#59829=CARTESIAN_POINT ( 'NONE',  ( -8.202992217649999418, 1418.657529326630083, 231.5784025581979790 ) ) ;
#59834=CARTESIAN_POINT ( 'NONE',  ( -45.54444238527090505, 1438.304335038940053, 266.1920658830019875 ) ) ;
#59835=CARTESIAN_POINT ( 'NONE',  ( 14.09058600726540078, 1509.404319979430056, 234.7755637671129989 ) ) ;
#59837=EDGE_LOOP ( 'NONE', ( #89171, #9703, #78560, #106384 ) ) ;
#59840=CARTESIAN_POINT ( 'NONE',  ( -5.387558624149999531, 1432.551536822860044, 154.6121729928979960 ) ) ;
#59841=CARTESIAN_POINT ( 'NONE',  ( 19.38028738881421731, 1456.807072245457448, 224.5317582173058213 ) ) ;
#59843=CARTESIAN_POINT ( 'NONE',  ( -26.75400904328050089, 1451.059527259639935, 136.3674970195820038 ) ) ;
#59844=ORIENTED_EDGE ( 'NONE', *, *, #82253, .T. ) ;
#59845=CARTESIAN_POINT ( 'NONE',  ( 24.48136660710000001, 1435.989032281489926, 217.2949255070680010 ) ) ;
#59847=CARTESIAN_POINT ( 'NONE',  ( 14.27633599229999994, 1452.807100928330101, 195.2240231267980164 ) ) ;
#59855=ORIENTED_EDGE ( 'NONE', *, *, #20564, .T. ) ;
#59856=CARTESIAN_POINT ( 'NONE',  ( -6.588284554585150055, 1410.390471986989951, 269.8687522186629622 ) ) ;
#59857=CARTESIAN_POINT ( 'NONE',  ( 4.143780836689379576, 1416.454745150250119, 231.7095439720729928 ) ) ;
#59859=CARTESIAN_POINT ( 'NONE',  ( 20.50000000000000000, 1445.052233488290085, 169.0968414572980123 ) ) ;
#59863=CARTESIAN_POINT ( 'NONE',  ( 0.004479545552087010364, 1409.421457559500141, 185.2262415390000001 ) ) ;
#59865=CARTESIAN_POINT ( 'NONE',  ( -45.65247486738287108, 1439.849382516791593, 266.1891217565876673 ) ) ;
#59866=CARTESIAN_POINT ( 'NONE',  ( -18.35772982613910287, 1422.336849757289883, 194.8914311005219986 ) ) ;
#59867=CARTESIAN_POINT ( 'NONE',  ( -18.17931802150000209, 1415.859000051729936, 224.8780086886979745 ) ) ;
#59868=CARTESIAN_POINT ( 'NONE',  ( 30.13944988253700075, 1467.656954244930148, 267.4649828126950410 ) ) ;
#59869=CARTESIAN_POINT ( 'NONE',  ( -11.09483971705885885, 1464.088240666073261, 231.7174097975078553 ) ) ;
#59870=CARTESIAN_POINT ( 'NONE',  ( -17.30312348755748530, 1422.521282115817712, 226.6250572771207317 ) ) ;
#59871=( BOUNDED_CURVE ( )  B_SPLINE_CURVE ( 3, ( #11622, #71575, #3248, #46353 ),
 .UNSPECIFIED., .F., .F. ) 
 B_SPLINE_CURVE_WITH_KNOTS ( ( 4, 4 ),
 ( 5.361618747459259815, 6.000063634424889436 ),
 .UNSPECIFIED. ) 
 CURVE ( )  GEOMETRIC_REPRESENTATION_ITEM ( )  RATIONAL_B_SPLINE_CURVE ( ( 1.000000000000000000, 0.9663198162573465311, 0.9663198162573465311, 1.000000000000000000 ) ) 
 REPRESENTATION_ITEM ( '' )  );
#59874=CARTESIAN_POINT ( 'NONE',  ( 18.50667789485245507, 1458.752429087900964, 227.6133156040012011 ) ) ;
#59877=ORIENTED_EDGE ( 'NONE', *, *, #45967, .F. ) ;
#59879=ADVANCED_FACE ( 'NONE', ( #44870 ), #58180, .T. ) ;
#59880=CARTESIAN_POINT ( 'NONE',  ( 26.92948524801489896, 1451.211802498159841, 136.2741858638970029 ) ) ;
#59883=ADVANCED_FACE ( 'NONE', ( #28590 ), #15229, .F. ) ;
#59885=CARTESIAN_POINT ( 'NONE',  ( -4.128104903896989697, 1425.965123590259509, 186.1105249954287331 ) ) ;
#59887=FACE_OUTER_BOUND ( 'NONE', #83124, .T. ) ;
#59889=CARTESIAN_POINT ( 'NONE',  ( 0.5844443723097010324, 1408.933469634509947, 186.5656055688390040 ) ) ;
#59896=CARTESIAN_POINT ( 'NONE',  ( 11.31580077666816742, 1420.115919293237539, 232.0087015463770115 ) ) ;
#59898=CARTESIAN_POINT ( 'NONE',  ( 11.46011354709300001, 1414.971717244350202, 221.6095414742599985 ) ) ;
#59900=DIRECTION ( 'NONE',  ( 0.4794255386042030054, 0.000000000000000000, 0.8775825618903727587 ) ) ;
#59903=B_SPLINE_SURFACE_WITH_KNOTS ( 'NONE', 5, 5, ( 
 ( #23006, #57209, #91333, #14618, #48805, #6220 ),
 ( #40372, #74551, #31976, #16791, #27429, #43146 ),
 ( #10647, #44814, #1707, #103021, #8974, #78968 ),
 ( #35285, #2273, #68365, #35847, #52653, #95195 ),
 ( #17345, #76738, #26317, #49, #19009, #103590 ),
 ( #36387, #52104, #50995, #9525, #70032, #43693 ) ),
 .UNSPECIFIED., .F., .F., .F.,
 ( 6, 6 ),
 ( 6, 6 ),
 ( 43.60693323619999973, 57.21764454529999711 ),
 ( 0.000000000000000000, 2.000000000000000000 ),
 .UNSPECIFIED. ) ;
#59909=CARTESIAN_POINT ( 'NONE',  ( -21.60872112289791147, 1509.279327801856198, 191.6769273891482612 ) ) ;
#59910=CARTESIAN_POINT ( 'NONE',  ( 11.83363686220000055, 1433.395016513080009, 150.5889480672979914 ) ) ;
#59911=CARTESIAN_POINT ( 'NONE',  ( -1.247529711191919932E-05, 1474.073207343779814, 267.9039250723909618 ) ) ;
#59912=B_SPLINE_SURFACE_WITH_KNOTS ( 'NONE', 5, 5, ( 
 ( #87781, #17758, #28410, #27299, #61480, #68779 ),
 ( #93935, #9396, #43559, #77709, #26742, #95608 ),
 ( #69328, #53637, #18875, #53073, #87211, #10502 ),
 ( #103436, #70442, #44674, #104562, #43009, #27856 ),
 ( #62037, #96160, #77167, #19438, #36809, #11061 ),
 ( #2685, #71000, #17201, #88866, #98904, #38991 ),
 ( #30043, #72100, #105683, #72622, #97255, #106216 ),
 ( #3235, #81544, #29498, #28966, #73169, #107313 ),
 ( #12703, #79922, #56373, #107859, #71563, #63156 ) ),
 .UNSPECIFIED., .F., .F., .F.,
 ( 6, 3, 6 ),
 ( 6, 6 ),
 ( 6.014757022580000445, 12.35992153179999953, 20.20875793540000132 ),
 ( -4.440892098509999801E-16, 10.00000000000000000 ),
 .UNSPECIFIED. ) ;
#59913=CARTESIAN_POINT ( 'NONE',  ( 12.50318290584439929, 1415.427621830080170, 196.7915438783630009 ) ) ;
#59918=CARTESIAN_POINT ( 'NONE',  ( -18.38973187710000090, 1486.345248910030023, 188.6648160310980131 ) ) ;
#59919=CARTESIAN_POINT ( 'NONE',  ( 11.72654505936638003, 1398.260515437505774, 203.3308392036481678 ) ) ;
#59921=ADVANCED_FACE ( 'NONE', ( #41407 ), #92895, .T. ) ;
#59923=CARTESIAN_POINT ( 'NONE',  ( 12.78690713350000152, 1416.828040475229955, 222.7042044314979989 ) ) ;
#59926=CARTESIAN_POINT ( 'NONE',  ( 18.82191891289999930, 1431.113060387329824, 213.4824283078179974 ) ) ;
#59932=CARTESIAN_POINT ( 'NONE',  ( 0.1890019494398779976, 1469.284980727640004, 182.5545442408230201 ) ) ;
#59934=ORIENTED_EDGE ( 'NONE', *, *, #70316, .T. ) ;
#59937=CARTESIAN_POINT ( 'NONE',  ( 13.19841768679999916, 1434.900414241469889, 149.7891824259980069 ) ) ;
#59938=CARTESIAN_POINT ( 'NONE',  ( -41.25063694456439833, 1441.159963068149864, 134.0999999980680002 ) ) ;
#59956=CARTESIAN_POINT ( 'NONE',  ( -33.30820988179999631, 1451.750048702429922, 135.1664504609980213 ) ) ;
#59957=CARTESIAN_POINT ( 'NONE',  ( -15.81585810399169922, 1410.113222428570225, 226.5225277695919885 ) ) ;
#59958=DIRECTION ( 'NONE',  ( -1.000000000000000000, 0.000000000000000000, 0.000000000000000000 ) ) ;
#59964=CARTESIAN_POINT ( 'NONE',  ( 36.70160066626374373, 1455.767766055568927, 269.5559760384784909 ) ) ;
#59965=CARTESIAN_POINT ( 'NONE',  ( -16.68463225901000158, 1442.773887286389936, 162.0935120915889911 ) ) ;
#59966=CARTESIAN_POINT ( 'NONE',  ( 19.41828847086908283, 1440.403404493772996, 212.4137351852459403 ) ) ;
#59969=CARTESIAN_POINT ( 'NONE',  ( 10.85845406881951192, 1424.793774302243946, 138.1921923613813590 ) ) ;
#59973=CARTESIAN_POINT ( 'NONE',  ( 2.713767649309999808, 1447.666028319260022, 156.1533243690980157 ) ) ;
#59975=CARTESIAN_POINT ( 'NONE',  ( 13.58256592070000046, 1416.843576337130116, 196.3343231799980231 ) ) ;
#59977=ORIENTED_EDGE ( 'NONE', *, *, #85252, .F. ) ;
#59979=ORIENTED_EDGE ( 'NONE', *, *, #64430, .T. ) ;
#59981=CARTESIAN_POINT ( 'NONE',  ( -23.92333147340000110, 1430.353917317029982, 204.8973678502680116 ) ) ;
#59982=CARTESIAN_POINT ( 'NONE',  ( -10.30849406833070070, 1425.144832954889807, 113.0135162854730027 ) ) ;
#59984=CARTESIAN_POINT ( 'NONE',  ( 16.96951548583769664, 1409.878878304549971, 192.5990281342199921 ) ) ;
#59988=CARTESIAN_POINT ( 'NONE',  ( -42.47346771400000875, 1432.913526188520109, 263.9447054790979905 ) ) ;
#59992=CARTESIAN_POINT ( 'NONE',  ( -36.20244804693129481, 1437.512936826869918, 136.5399734142819739 ) ) ;
#59993=ORIENTED_EDGE ( 'NONE', *, *, #47980, .T. ) ;
#59994=CARTESIAN_POINT ( 'NONE',  ( 11.89590846401610058, 1396.328474664730038, 207.2763644758680073 ) ) ;
#59996=CARTESIAN_POINT ( 'NONE',  ( -16.91389461470000199, 1458.999332487730271, 228.9792524216979928 ) ) ;
#59997=ORIENTED_EDGE ( 'NONE', *, *, #69995, .F. ) ;
#59998=ORIENTED_EDGE ( 'NONE', *, *, #89493, .T. ) ;
#60000=CARTESIAN_POINT ( 'NONE',  ( -11.78818154252719985, 1426.417843477500128, 148.5075632149639944 ) ) ;
#60002=DIRECTION ( 'NONE',  ( 0.000000000000000000, 0.000000000000000000, -1.000000000000000000 ) ) ;
#60004=CARTESIAN_POINT ( 'NONE',  ( 10.70848634212536865, 1506.855035729306792, 228.7236287190453936 ) ) ;
#60005=CARTESIAN_POINT ( 'NONE',  ( -0.8934505306369999733, 1461.198707732230105, 235.2527420635979638 ) ) ;
#60006=CARTESIAN_POINT ( 'NONE',  ( 2.322564298810700034, 1421.242547636910103, 183.2407391359299993 ) ) ;
#60010=VERTEX_POINT ( 'NONE', #524 ) ;
#60013=ORIENTED_EDGE ( 'NONE', *, *, #4980, .F. ) ;
#60014=CARTESIAN_POINT ( 'NONE',  ( 11.74616747385230120, 1426.722822852569834, 144.8102584898179828 ) ) ;
#60015=CARTESIAN_POINT ( 'NONE',  ( 19.45725490719999939, 1497.694397923730094, 228.9812751475980122 ) ) ;
#60018=EDGE_CURVE ( 'NONE', #59173, #77352, #104476, .T. ) ;
#60020=CARTESIAN_POINT ( 'NONE',  ( 5.089041851490000212, 1509.032960110130034, 237.0857944526979679 ) ) ;
#60024=CARTESIAN_POINT ( 'NONE',  ( -4.999592162339999923, 1422.499950720829929, 185.1272544950980148 ) ) ;
#60025=CARTESIAN_POINT ( 'NONE',  ( -4.291175242752039765, 1446.971469842819943, 154.7965863647420122 ) ) ;
#60027=CARTESIAN_POINT ( 'NONE',  ( -4.230274983775188069, 1410.439435280939961, 186.8053085259470549 ) ) ;
#60029=CARTESIAN_POINT ( 'NONE',  ( 25.39780210992439891, 1475.101801264620235, 206.2221860197550143 ) ) ;
#60030=CARTESIAN_POINT ( 'NONE',  ( 17.69068447980000158, 1457.992677922929943, 229.6631064895979932 ) ) ;
#60032=CARTESIAN_POINT ( 'NONE',  ( 15.28377178641770051, 1507.620489299410110, 226.2805935727439817 ) ) ;
#60033=B_SPLINE_SURFACE_WITH_KNOTS ( 'NONE', 5, 5, ( 
 ( #55823, #72087, #106201, #87767, #63679, #13218, #104548, #36796, #37350 ),
 ( #71549, #47408, #105670, #19423, #81530, #4832, #27844, #96145, #2671 ),
 ( #58018, #23826, #91602, #7045, #49070, #83205, #6494, #40646, #14329 ),
 ( #65869, #5393, #107301, #74817, #92696, #108963, #31687, #99989, #41204 ),
 ( #58566, #31137, #32250, #66430, #100546, #48518, #82092, #83750, #107848 ),
 ( #108405, #15425, #40094, #92153, #15972, #49617, #50174, #84301, #38979 ) ),
 .UNSPECIFIED., .F., .F., .F.,
 ( 6, 6 ),
 ( 6, 3, 6 ),
 ( 0.4666582264940000169, 2.797885342366120298 ),
 ( -1.082960611691029974E-05, 1.000000000000000000, 2.000000000000000000 ),
 .UNSPECIFIED. ) ;
#60034=CARTESIAN_POINT ( 'NONE',  ( -5.655232455200980723, 1423.184742756340029, 101.0239091077149993 ) ) ;
#60035=VERTEX_POINT ( 'NONE', #10001 ) ;
#60039=CARTESIAN_POINT ( 'NONE',  ( -2.933872690221072776, 1485.132197629912071, 183.0775065428524329 ) ) ;
#60040=DIRECTION ( 'NONE',  ( -1.065814103640150437E-14, 0.000000000000000000, 1.000000000000000000 ) ) ;
#60043=CARTESIAN_POINT ( 'NONE',  ( 0.7353240777269999251, 1489.474306033429912, 187.1311076040980197 ) ) ;
#60046=CARTESIAN_POINT ( 'NONE',  ( -11.82947776570000009, 1429.869038498530244, 149.4074658875980219 ) ) ;
#60047=CARTESIAN_POINT ( 'NONE',  ( -10.81518761075750135, 1424.921099531289883, 144.1705495212430037 ) ) ;
#60049=CARTESIAN_POINT ( 'NONE',  ( 16.82545552545150258, 1509.500615784180127, 233.4982582598109957 ) ) ;
#60053=CARTESIAN_POINT ( 'NONE',  ( -21.63817346260000107, 1508.012227572530037, 226.7581651977980073 ) ) ;
#60055=CARTESIAN_POINT ( 'NONE',  ( -16.16654775127000221, 1459.157660042964153, 229.6201166687930026 ) ) ;
#60058=CARTESIAN_POINT ( 'NONE',  ( 27.07453441790000070, 1412.356090134630222, 267.2274653296979636 ) ) ;
#60059=CARTESIAN_POINT ( 'NONE',  ( 24.54015759500000016, 1436.582034297039854, 138.9799141002980036 ) ) ;
#60061=CARTESIAN_POINT ( 'NONE',  ( 23.23294983419999937, 1430.294683446630188, 204.9340936284079930 ) ) ;
#60062=CARTESIAN_POINT ( 'NONE',  ( -0.1035247606053459890, 1508.569086740290004, 237.9121964778769893 ) ) ;
#60064=CARTESIAN_POINT ( 'NONE',  ( 9.814762245626701187, 1424.216260739349764, 144.1582897308169890 ) ) ;
#60065=CARTESIAN_POINT ( 'NONE',  ( -41.52520403286720807, 1442.071982413179967, 135.9507581816680215 ) ) ;
#60066=ADVANCED_FACE ( 'NONE', ( #53698 ), #39354, .F. ) ;
#60067=DIRECTION ( 'NONE',  ( 0.03489949670250328678, -0.9993908270190956511, 0.000000000000000000 ) ) ;
#60069=CARTESIAN_POINT ( 'NONE',  ( -13.68074494839999922, 1444.567011418389939, 188.0766381524979920 ) ) ;
#60073=CARTESIAN_POINT ( 'NONE',  ( 44.93136303390000563, 1440.913033067569813, 269.6838066906980202 ) ) ;
#60074=ORIENTED_EDGE ( 'NONE', *, *, #27629, .T. ) ;
#60075=CARTESIAN_POINT ( 'NONE',  ( 1.460943697043280087, 1495.022397442580086, 181.6406806417639928 ) ) ;
#60076=CARTESIAN_POINT ( 'NONE',  ( -12.13599495486779922, 1409.336858669690173, 200.3964593173120079 ) ) ;
#60079=CARTESIAN_POINT ( 'NONE',  ( -9.853196041699998631, 1474.808872623229945, 269.2594982597980220 ) ) ;
#60082=CARTESIAN_POINT ( 'NONE',  ( -24.14770755569024985, 1444.491430425563976, 211.6499922375425058 ) ) ;
#60084=CARTESIAN_POINT ( 'NONE',  ( 13.58235846979999906, 1416.828040475229955, 196.3349388281980055 ) ) ;
#60085=CARTESIAN_POINT ( 'NONE',  ( 11.78977346136659854, 1415.441076448360036, 223.1097579672979805 ) ) ;
#60088=CARTESIAN_POINT ( 'NONE',  ( -1.438891081339280120, 1452.191228260170192, 183.8587004481619829 ) ) ;
#60089=AXIS2_PLACEMENT_3D ( 'NONE', #95877, #19141, #104833 ) ;
#60090=CARTESIAN_POINT ( 'NONE',  ( -23.20723499460000028, 1410.644907069029841, 205.4415377791680157 ) ) ;
#60091=CARTESIAN_POINT ( 'NONE',  ( 13.49734317350000090, 1415.088275290029969, 197.3807697222979982 ) ) ;
#60097=CARTESIAN_POINT ( 'NONE',  ( -3.540693220810990471, 1508.270056219510025, 180.7688429917959922 ) ) ;
#60100=CARTESIAN_POINT ( 'NONE',  ( 11.73499481921169973, 1426.697258569849964, 144.0242909167239986 ) ) ;
#60101=CARTESIAN_POINT ( 'NONE',  ( 0.3722769099684289928, 1457.826255237599980, 228.9731060096619899 ) ) ;
#60104=CARTESIAN_POINT ( 'NONE',  ( -0.06979898363973670306, 1408.910622953150096, 223.8076866964610190 ) ) ;
#60106=CARTESIAN_POINT ( 'NONE',  ( -6.899998715920828474, 1398.118124432348850, 220.1627551181343563 ) ) ;
#60109=CARTESIAN_POINT ( 'NONE',  ( -19.05511642929999994, 1449.657101504390084, 193.8129821119980249 ) ) ;
#60111=CARTESIAN_POINT ( 'NONE',  ( 41.61763030636900140, 1445.085476029980100, 135.5083515819240176 ) ) ;
#60115=CARTESIAN_POINT ( 'NONE',  ( 11.94595818812160104, 1433.509642704729913, 149.8900677580190006 ) ) ;
#60117=VERTEX_POINT ( 'NONE', #98957 ) ;
#60121=CARTESIAN_POINT ( 'NONE',  ( 16.06157012919580040, 1423.788481394339897, 191.1175312021059938 ) ) ;
#60123=CARTESIAN_POINT ( 'NONE',  ( 8.271109682960839038, 1498.104299293129998, 234.5502916224329795 ) ) ;
#60125=CARTESIAN_POINT ( 'NONE',  ( 6.753106024830000109, 1507.635313380530079, 182.4733158664980124 ) ) ;
#60127=CARTESIAN_POINT ( 'NONE',  ( -24.56899124258660194, 1444.772254235220089, 210.9323875608310175 ) ) ;
#60129=CARTESIAN_POINT ( 'NONE',  ( 0.2669485111002459776, 1395.922382434750034, 198.1227973212599807 ) ) ;
#60130=CARTESIAN_POINT ( 'NONE',  ( 11.57170172580000056, 1431.970351487809921, 151.1874232329979861 ) ) ;
#60132=ORIENTED_EDGE ( 'NONE', *, *, #82845, .F. ) ;
#60133=CARTESIAN_POINT ( 'NONE',  ( 13.76019309406060032, 1436.072204996710070, 150.3335515433649903 ) ) ;
#60134=ORIENTED_EDGE ( 'NONE', *, *, #55101, .F. ) ;
#60136=CARTESIAN_POINT ( 'NONE',  ( 13.02399213288301105, 1444.859346537102965, 169.4177112119271271 ) ) ;
#60137=CARTESIAN_POINT ( 'NONE',  ( -1.466394352250000255, 1466.280833669130061, 235.4455910585979836 ) ) ;
#60141=CARTESIAN_POINT ( 'NONE',  ( -19.07569465070004711, 1442.225521153744921, 210.5149903700299205 ) ) ;
#60144=ORIENTED_EDGE ( 'NONE', *, *, #45240, .T. ) ;
#60147=CARTESIAN_POINT ( 'NONE',  ( 22.55659962669360041, 1440.913060387330006, 229.8770814074250097 ) ) ;
#60148=CARTESIAN_POINT ( 'NONE',  ( -18.87980335319999625, 1507.654596516530091, 229.6982590054979880 ) ) ;
#60150=CARTESIAN_POINT ( 'NONE',  ( -5.656834581150000041, 1409.110601402830071, 188.1059135931980109 ) ) ;
#60154=CARTESIAN_POINT ( 'NONE',  ( 23.72977224379999583, 1434.259526396529964, 214.5256004728379935 ) ) ;
#60164=AXIS2_PLACEMENT_3D ( 'NONE', #3355, #87902, #26872 ) ;
#60169=CARTESIAN_POINT ( 'NONE',  ( -17.45339170113992822, 1486.143972108528942, 188.0383730386266450 ) ) ;
#60170=B_SPLINE_CURVE_WITH_KNOTS ( 'NONE', 5,
 ( #2425, #105406, #63435, #44970, #11897, #82257, #108561, #82804, #11357, #6098, #108001, #5558, #53365, #39707, #19734, #57083, #28698, #80203, #88616, #74435, #70740, #28139, #48681, #31851, #55022, #53935, #37645 ),
 .UNSPECIFIED., .F., .F.,
 ( 6, 3, 3, 3, 3, 3, 3, 3, 6 ),
 ( 0.000000000000000000, 0.06058382609222391635, 0.1069330941294720783, 0.1211676521844478327, 0.1797127176077684407, 0.2382577830310894373, 0.3553479138777306812, 0.6482918569636776374, 1.000000000000000000 ),
 .UNSPECIFIED. ) ;
#60174=CARTESIAN_POINT ( 'NONE',  ( 16.98089203389999824, 1467.669754651430139, 255.1565212655980019 ) ) ;
#60176=CARTESIAN_POINT ( 'NONE',  ( 2.108362890389359645, 1452.419099747896553, 183.6319488572359262 ) ) ;
#60178=CARTESIAN_POINT ( 'NONE',  ( -7.828230685879998596, 1507.298741238030061, 235.3518363426980216 ) ) ;
#60179=CARTESIAN_POINT ( 'NONE',  ( -23.94933866970000125, 1445.534750183129972, 212.9709028766179983 ) ) ;
#60180=B_SPLINE_CURVE_WITH_KNOTS ( 'NONE', 3,
 ( #32772, #48499, #50684, #57459, #31668, #65849, #82639, #15408, #49597, #83730, #75889, #49051, #91586, #41182, #109495 ),
 .UNSPECIFIED., .F., .F.,
 ( 4, 2, 2, 1, 1, 1, 2, 2, 4 ),
 ( 0.000000000000000000, 0.2500000000000353051, 0.3750000000000530687, 0.4375000000000631162, 0.4687500000000695000, 0.4843750000000723865, 0.4921875000000711098, 0.5000000000000698330, 1.000000000000000000 ),
 .UNSPECIFIED. ) ;
#60181=PLANE ( 'NONE',  #1810 ) ;
#60182=CARTESIAN_POINT ( 'NONE',  ( 17.89017687474920137, 1410.330682765429856, 222.8911238419379970 ) ) ;
#60185=ORIENTED_EDGE ( 'NONE', *, *, #83387, .F. ) ;
#60187=CARTESIAN_POINT ( 'NONE',  ( 0.3396692986610000409, 1405.750286565129954, 267.5371225631980110 ) ) ;
#60188=CARTESIAN_POINT ( 'NONE',  ( 24.51495038730000076, 1443.562157032569758, 213.8565503907379934 ) ) ;
#60192=CARTESIAN_POINT ( 'NONE',  ( 27.60464170112659943, 1435.621481315979963, 136.1400934894720081 ) ) ;
#60194=CARTESIAN_POINT ( 'NONE',  ( 3.286444981498850021E-15, 1458.388061309670093, 231.5054671141039933 ) ) ;
#60197=B_SPLINE_CURVE_WITH_KNOTS ( 'NONE', 5,
 ( #7003, #49579, #108919, #102556, #72311, #79607, #61714, #87448, #38130, #28635, #53876, #19671, #71222, #29725, #105906, #2911, #63376, #54958 ),
 .UNSPECIFIED., .F., .F.,
 ( 6, 3, 3, 3, 3, 6 ),
 ( 0.000000000000000000, 0.04383986791751091211, 0.1036123950753678191, 0.2231574493812304161, 0.6694723481587087077, 1.000000000000000000 ),
 .UNSPECIFIED. ) ;
#60201=CARTESIAN_POINT ( 'NONE',  ( 0.8041763403130000043, 1426.566393376330097, 144.1938086916980239 ) ) ;
#60202=CARTESIAN_POINT ( 'NONE',  ( 12.91344045910000027, 1434.774313861569908, 146.5970547348979949 ) ) ;
#60204=CARTESIAN_POINT ( 'NONE',  ( 15.64943080881179682, 1466.933481671390155, 189.3680284421589874 ) ) ;
#60205=CARTESIAN_POINT ( 'NONE',  ( -0.2950133488750000255, 1415.766390753429960, 233.4435486769980059 ) ) ;
#60208=CARTESIAN_POINT ( 'NONE',  ( -28.78960605939999695, 1509.588732895030262, 209.8024020300809980 ) ) ;
#60212=CARTESIAN_POINT ( 'NONE',  ( -8.506922781476685458, 1417.327140144819396, 230.7140993806030735 ) ) ;
#60213=CARTESIAN_POINT ( 'NONE',  ( -15.06028995570763840, 1451.149887921017580, 149.6833329127408092 ) ) ;
#60215=CARTESIAN_POINT ( 'NONE',  ( 25.21992779760000047, 1436.607954016930080, 137.5621431200979998 ) ) ;
#60216=CARTESIAN_POINT ( 'NONE',  ( -9.843170653638850354, 1396.256791483090183, 204.0667884097820206 ) ) ;
#60218=FACE_OUTER_BOUND ( 'NONE', #22219, .T. ) ;
#60219=CARTESIAN_POINT ( 'NONE',  ( 4.915203104360000630, 1434.541746329560056, 150.1320020560979742 ) ) ;
#60224=CARTESIAN_POINT ( 'NONE',  ( 10.40857034289999916, 1425.394460820129780, 96.53362461269790629 ) ) ;
#60226=CARTESIAN_POINT ( 'NONE',  ( -11.62902870529999966, 1433.064885913230000, 151.0294648830980009 ) ) ;
#60227=CARTESIAN_POINT ( 'NONE',  ( -2.863573784786321408, 1419.688340288614654, 186.1810135818298875 ) ) ;
#60230=CARTESIAN_POINT ( 'NONE',  ( 8.149343875210002253, 1509.018734359930249, 181.8702896482980123 ) ) ;
#60231=CARTESIAN_POINT ( 'NONE',  ( 3.933035305499999801, 1449.187059537480081, 184.2601159103979853 ) ) ;
#60234=ORIENTED_EDGE ( 'NONE', *, *, #21920, .F. ) ;
#60235=EDGE_LOOP ( 'NONE', ( #4483, #29386, #49065, #46799 ) ) ;
#60236=CARTESIAN_POINT ( 'NONE',  ( -41.65674268029999894, 1443.992461967939789, 135.6790812281979868 ) ) ;
#60237=ADVANCED_FACE ( 'NONE', ( #19296 ), #63563, .T. ) ;
#60238=DIRECTION ( 'NONE',  ( 0.000000000000000000, 0.000000000000000000, 1.000000000000000000 ) ) ;
#60239=CARTESIAN_POINT ( 'NONE',  ( -2.002811041570000088E-09, 1473.589435999130046, 270.3925729408980487 ) ) ;
#60241=FACE_OUTER_BOUND ( 'NONE', #74571, .T. ) ;
#60245=CARTESIAN_POINT ( 'NONE',  ( -33.91368077465119768, 1451.728768558339880, 134.7155154936840233 ) ) ;
#60246=EDGE_CURVE ( 'NONE', #104782, #105791, #34856, .T. ) ;
#60248=CARTESIAN_POINT ( 'NONE',  ( -22.62861454470000311, 1507.212883763329955, 208.5231287359179930 ) ) ;
#60250=CARTESIAN_POINT ( 'NONE',  ( 9.688704068493601440, 1409.071838889859919, 198.0917906310850185 ) ) ;
#60251=CARTESIAN_POINT ( 'NONE',  ( -10.60628234125749891, 1406.913721737060087, 266.9166020718200230 ) ) ;
#60252=CARTESIAN_POINT ( 'NONE',  ( -13.71031927006879947, 1434.974885213249991, 148.6196309992409965 ) ) ;
#60255=CARTESIAN_POINT ( 'NONE',  ( 13.66368654969999952, 1443.423569391949968, 188.9472448265979949 ) ) ;
#60258=CARTESIAN_POINT ( 'NONE',  ( -22.12758967992428794, 1506.606278687006125, 209.0267225037276830 ) ) ;
#60261=CARTESIAN_POINT ( 'NONE',  ( -14.43173846279999850, 1485.481767227229966, 186.7711707502979834 ) ) ;
#60263=B_SPLINE_CURVE_WITH_KNOTS ( 'NONE', 3,
 ( #12316, #30774, #55451, #55996, #37531, #56547, #90675, #39167, #20164, #47050 ),
 .UNSPECIFIED., .F., .F.,
 ( 4, 2, 2, 2, 4 ),
 ( 0.000000000000000000, 0.0007438262484377516567, 0.001487652496875503313, 0.002231478745313254970, 0.002975304993751006627 ),
 .UNSPECIFIED. ) ;
#60265=CARTESIAN_POINT ( 'NONE',  ( -11.07527106836971775, 1414.913060387329779, 197.4018683738858044 ) ) ;
#60268=CARTESIAN_POINT ( 'NONE',  ( -28.99333967900000175, 1509.929026104229933, 203.7293937816380094 ) ) ;
#60271=EDGE_CURVE ( 'NONE', #45857, #29539, #20373, .T. ) ;
#60273=CARTESIAN_POINT ( 'NONE',  ( -6.972733185100000064, 1409.156553595530113, 196.2309095868979796 ) ) ;
#60275=CARTESIAN_POINT ( 'NONE',  ( -9.302446781629999606, 1445.510056962059934, 184.3653119834979748 ) ) ;
#60277=FACE_OUTER_BOUND ( 'NONE', #31822, .T. ) ;
#60278=CARTESIAN_POINT ( 'NONE',  ( 21.04266091710000097, 1508.126368074930269, 226.0751098261980019 ) ) ;
#60279=CARTESIAN_POINT ( 'NONE',  ( 20.39580838967040322, 1487.450036232110051, 225.4216937902110089 ) ) ;
#60280=CARTESIAN_POINT ( 'NONE',  ( -25.14723534630000046, 1435.562924969450251, 136.5603555134980240 ) ) ;
#60284=CARTESIAN_POINT ( 'NONE',  ( -14.85284859380000100, 1420.429529095230009, 227.0635863076980172 ) ) ;
#60285=CARTESIAN_POINT ( 'NONE',  ( 7.105427357599999217E-15, 1405.913060387330006, 146.1721969590979882 ) ) ;
#60289=CARTESIAN_POINT ( 'NONE',  ( -2.824333841560000113, 1412.839907593029920, 232.6864343732979989 ) ) ;
#60291=B_SPLINE_CURVE_WITH_KNOTS ( 'NONE', 3,
 ( #85538, #102349, #65610, #91345, #48256, #23015, #65055, #110203, #42447, #25632, #50860 ),
 .UNSPECIFIED., .F., .F.,
 ( 4, 2, 1, 2, 2, 4 ),
 ( 0.000000000000000000, 0.2500000000001129097, 0.3750000000001033618, 0.4375000000000550671, 0.5000000000000067724, 1.000000000000000000 ),
 .UNSPECIFIED. ) ;
#60292=EDGE_LOOP ( 'NONE', ( #7157, #72719, #88541, #67274 ) ) ;
#60295=CARTESIAN_POINT ( 'NONE',  ( 12.38050916831940107, 1435.706281718790024, 151.0122276686279861 ) ) ;
#60297=CARTESIAN_POINT ( 'NONE',  ( 16.47627392169409788, 1459.305803831369985, 229.0165498365500127 ) ) ;
#60298=CARTESIAN_POINT ( 'NONE',  ( -21.52252890938149932, 1508.917042082100124, 227.3600265264449831 ) ) ;
#60305=CARTESIAN_POINT ( 'NONE',  ( -3.453453303525895635, 1420.336231801281883, 144.1190299178094563 ) ) ;
#60307=ORIENTED_EDGE ( 'NONE', *, *, #11355, .F. ) ;
#60309=CARTESIAN_POINT ( 'NONE',  ( -11.60004869885203682, 1425.894669202444675, 137.5118601406020673 ) ) ;
#60310=ORIENTED_EDGE ( 'NONE', *, *, #26824, .T. ) ;
#60311=CARTESIAN_POINT ( 'NONE',  ( 3.126635617060000261, 1420.873695464229968, 185.0718492959979926 ) ) ;
#60318=CARTESIAN_POINT ( 'NONE',  ( 17.85311748929999709, 1415.140114704729967, 210.5770968554979845 ) ) ;
#60321=LINE ( 'NONE', #43522, #36039 ) ;
#60322=CARTESIAN_POINT ( 'NONE',  ( 45.19888506029440123, 1440.913060374670067, 265.6850257504329988 ) ) ;
#60324=CARTESIAN_POINT ( 'NONE',  ( -2.967510011182339813, 1486.005022665990055, 182.1268798534620146 ) ) ;
#60325=CARTESIAN_POINT ( 'NONE',  ( 10.85263098157019890, 1425.442989095870871, 147.0760006456408746 ) ) ;
#60326=ORIENTED_EDGE ( 'NONE', *, *, #53884, .F. ) ;
#60329=EDGE_CURVE ( 'NONE', #76242, #74855, #36130, .T. ) ;
#60331=CARTESIAN_POINT ( 'NONE',  ( -28.70471842169999732, 1509.915451241629853, 211.4532599174380039 ) ) ;
#60332=CARTESIAN_POINT ( 'NONE',  ( 5.503649956843871927, 1410.480191370396142, 186.5618691807696052 ) ) ;
#60340=CARTESIAN_POINT ( 'NONE',  ( 3.538898781339999911, 1452.789479317830001, 152.9844706352979813 ) ) ;
#60341=CARTESIAN_POINT ( 'NONE',  ( -27.23667361500285367, 1509.093168187175024, 212.0595736267784162 ) ) ;
#60343=CARTESIAN_POINT ( 'NONE',  ( 25.40371319049999954, 1509.800185459130034, 194.3524381038979811 ) ) ;
#60345=CARTESIAN_POINT ( 'NONE',  ( -18.64904950366887704, 1458.434616773794005, 227.4345046988593424 ) ) ;
#60347=CARTESIAN_POINT ( 'NONE',  ( 20.51884491728609916, 1509.640283927850078, 230.4689269196439909 ) ) ;
#60350=CARTESIAN_POINT ( 'NONE',  ( 16.84932903106719593, 1507.643820733580014, 231.2344440140070105 ) ) ;
#60352=CARTESIAN_POINT ( 'NONE',  ( 39.76846978917860298, 1441.086563173470040, 136.8361555895239974 ) ) ;
#60353=CARTESIAN_POINT ( 'NONE',  ( 2.752169640037664955, 1410.389826760280812, 269.3346704479379241 ) ) ;
#60358=CARTESIAN_POINT ( 'NONE',  ( -12.77945754873770312, 1435.908885557353415, 150.8386072880828408 ) ) ;
#60359=CARTESIAN_POINT ( 'NONE',  ( -20.21139152160000307, 1485.602675199130090, 191.2208696118980242 ) ) ;
#60361=CARTESIAN_POINT ( 'NONE',  ( 2.441025387419999859, 1408.998302871329997, 186.5920540833980112 ) ) ;
#60363=CARTESIAN_POINT ( 'NONE',  ( -8.510960889389998840, 1440.269029031439914, 153.6986479344980125 ) ) ;
#60367=CARTESIAN_POINT ( 'NONE',  ( -24.95756431429999722, 1451.613974120029980, 137.4741663018980091 ) ) ;
#60368=CARTESIAN_POINT ( 'NONE',  ( 2.463295240619999937, 1464.794365564629743, 237.1801197511979922 ) ) ;
#60369=ORIENTED_EDGE ( 'NONE', *, *, #102051, .T. ) ;
#60372=CARTESIAN_POINT ( 'NONE',  ( -44.01745644850000616, 1445.811985921539872, 270.0975557605979702 ) ) ;
#60373=CARTESIAN_POINT ( 'NONE',  ( 17.06941271609999689, 1409.674943327129995, 224.1775087769979962 ) ) ;
#60377=CARTESIAN_POINT ( 'NONE',  ( -1.120982774553380006E-08, 1474.398122755949998, 264.1710263624909771 ) ) ;
#60378=CARTESIAN_POINT ( 'NONE',  ( 2.920726586082400100, 1409.795150870450016, 231.4697806816330115 ) ) ;
#60379=CARTESIAN_POINT ( 'NONE',  ( -1.064544241000000113, 1415.263254644630024, 227.0974121259979768 ) ) ;
#60380=CARTESIAN_POINT ( 'NONE',  ( -3.454294121580000265, 1417.605600631229890, 235.1430308038980002 ) ) ;
#60383=CARTESIAN_POINT ( 'NONE',  ( -0.9697694473224367506, 1484.980380940773102, 182.0907361725558360 ) ) ;
#60385=CARTESIAN_POINT ( 'NONE',  ( -46.01202577552099626, 1439.422152723799854, 266.6782865154239630 ) ) ;
#60386=CARTESIAN_POINT ( 'NONE',  ( -3.599584570160000219, 1428.751101579730175, 185.8911643027980176 ) ) ;
#60391=CARTESIAN_POINT ( 'NONE',  ( -2.478438400780000439, 1438.044022645609857, 157.7045694735979851 ) ) ;
#60392=AXIS2_PLACEMENT_3D ( 'NONE', #108795, #60067, #23676 ) ;
#60393=CARTESIAN_POINT ( 'NONE',  ( 19.30109655617612674, 1456.551915534814498, 224.7044840561601120 ) ) ;
#60396=CARTESIAN_POINT ( 'NONE',  ( -26.87827581797160192, 1451.501870722200010, 136.0699096253820244 ) ) ;
#60398=CARTESIAN_POINT ( 'NONE',  ( -14.14461398200000097, 1452.819910075730149, 195.5024427521979931 ) ) ;
#60403=CARTESIAN_POINT ( 'NONE',  ( -23.95707600349131994, 1445.781625871585447, 214.3999464193026370 ) ) ;
#60407=ORIENTED_EDGE ( 'NONE', *, *, #104138, .F. ) ;
#60408=CARTESIAN_POINT ( 'NONE',  ( -1.255427878548490028, 1407.658860642259924, 270.1374946076119841 ) ) ;
#60410=CARTESIAN_POINT ( 'NONE',  ( 12.24805133206790053, 1420.337794571750010, 229.9787113497959865 ) ) ;
#60416=CARTESIAN_POINT ( 'NONE',  ( -23.55086081228390071, 1411.110693255149727, 210.4794179021569960 ) ) ;
#60417=CARTESIAN_POINT ( 'NONE',  ( -0.2257100754742899784, 1409.089074076840006, 185.5875059678090224 ) ) ;
#60420=CARTESIAN_POINT ( 'NONE',  ( -45.66504371789742578, 1440.259978084865224, 266.1887742723951646 ) ) ;
#60421=EDGE_CURVE ( 'NONE', #57270, #65905, #33355, .T. ) ;
#60422=CARTESIAN_POINT ( 'NONE',  ( -20.71123423377139972, 1497.550399210990008, 192.5020499071400195 ) ) ;
#60423=CARTESIAN_POINT ( 'NONE',  ( -19.19682044410000188, 1430.794004629730125, 224.3914492935979865 ) ) ;
#60424=CARTESIAN_POINT ( 'NONE',  ( 33.07189531519680514, 1465.514140148620072, 267.0777719542580257 ) ) ;
#60425=CARTESIAN_POINT ( 'NONE',  ( -9.277930374200103358, 1464.954721498918616, 232.6830885689707316 ) ) ;
#60426=CARTESIAN_POINT ( 'NONE',  ( -16.40477380347672209, 1421.217279018667796, 227.0028012172701040 ) ) ;
#60429=CARTESIAN_POINT ( 'NONE',  ( 18.84662620435946323, 1457.907283617477560, 227.0809673387096836 ) ) ;
#60434=CARTESIAN_POINT ( 'NONE',  ( 26.09509902904159873, 1452.001783465240123, 135.0935493681200228 ) ) ;
#60438=CARTESIAN_POINT ( 'NONE',  ( 16.49791572389999672, 1409.489180299430018, 193.7307885960979945 ) ) ;
#60439=CARTESIAN_POINT ( 'NONE',  ( 13.76936860679999874, 1444.324653571829003, 176.3340081878980641 ) ) ;
#60440=CARTESIAN_POINT ( 'NONE',  ( 3.492283213099107275, 1439.693639858082861, 184.4976232197295190 ) ) ;
#60447=CARTESIAN_POINT ( 'NONE',  ( 6.334329861979885123, 1418.381028394342138, 233.6652930423259704 ) ) ;
#60448=ORIENTED_EDGE ( 'NONE', *, *, #1613, .T. ) ;
#60449=CARTESIAN_POINT ( 'NONE',  ( 11.16128041097469925, 1414.913057846380070, 221.5234502185170129 ) ) ;
#60451=CARTESIAN_POINT ( 'NONE',  ( -0.4620612703160609791, 1409.418054490960003, 232.8178123332089910 ) ) ;
#60455=EDGE_CURVE ( 'NONE', #30887, #104987, #41885, .T. ) ;
#60458=CARTESIAN_POINT ( 'NONE',  ( -3.268607775400000026, 1455.844446697429930, 219.6133831120980062 ) ) ;
#60459=CARTESIAN_POINT ( 'NONE',  ( -21.87285697696509956, 1509.490620199582054, 191.4610675759308265 ) ) ;
#60460=CARTESIAN_POINT ( 'NONE',  ( 11.82457892589999915, 1433.344969013340005, 150.5980735906980215 ) ) ;
#60461=CARTESIAN_POINT ( 'NONE',  ( 18.57221607090000148, 1447.675799068749939, 219.6133835466979747 ) ) ;
#60467=CARTESIAN_POINT ( 'NONE',  ( -4.704661063000000532, 1486.518663884429998, 182.0064326752979866 ) ) ;
#60468=CARTESIAN_POINT ( 'NONE',  ( 12.66920257684705398, 1398.288630080463918, 206.2055005063946851 ) ) ;
#60469=CARTESIAN_POINT ( 'NONE',  ( -29.88894142145320032, 1509.995722311340160, 211.8654022664900083 ) ) ;
#60471=B_SPLINE_CURVE_WITH_KNOTS ( 'NONE', 5,
 ( #10529, #47451, #91644, #98389, #82135, #21659, #56959, #73767, #107344 ),
 .UNSPECIFIED., .F., .F.,
 ( 6, 3, 6 ),
 ( 0.000000000000000000, 0.5050532947554345897, 1.000000000000000000 ),
 .UNSPECIFIED. ) ;
#60472=CARTESIAN_POINT ( 'NONE',  ( 2.804856904796726003, 1447.114277549598228, 170.5309535257328548 ) ) ;
#60473=CARTESIAN_POINT ( 'NONE',  ( -33.91369110859999836, 1435.681798638700002, 135.0664268289980043 ) ) ;
#60475=CARTESIAN_POINT ( 'NONE',  ( 23.56404405089999798, 1519.913060387329779, 210.1014910071569943 ) ) ;
#60479=CARTESIAN_POINT ( 'NONE',  ( 0.1668001638216120019, 1482.213501802149949, 181.9993034263140146 ) ) ;
#60480=CARTESIAN_POINT ( 'NONE',  ( 28.84709935510000278, 1507.919204205830056, 206.0039977711180086 ) ) ;
#60481=ORIENTED_EDGE ( 'NONE', *, *, #56235, .F. ) ;
#60482=FACE_OUTER_BOUND ( 'NONE', #106775, .T. ) ;
#60484=CARTESIAN_POINT ( 'NONE',  ( 0.003568499702431209702, 1467.142144108200000, 235.6416276161930057 ) ) ;
#60485=CARTESIAN_POINT ( 'NONE',  ( 11.87504895220000023, 1433.007246834750049, 149.8850454502979801 ) ) ;
#60486=CARTESIAN_POINT ( 'NONE',  ( -34.20278863726849750, 1451.714767517939890, 134.0999999981159760 ) ) ;
#60488=VERTEX_POINT ( 'NONE', #39163 ) ;
#60489=DIRECTION ( 'NONE',  ( 0.000000000000000000, 1.000000000000000000, 0.000000000000000000 ) ) ;
#60501=CARTESIAN_POINT ( 'NONE',  ( 2.811694757223507146, 1464.674002724843604, 236.8041411256813547 ) ) ;
#60504=CARTESIAN_POINT ( 'NONE',  ( 16.68463233076019492, 1442.773887286370609, 162.0935120523188857 ) ) ;
#60507=CARTESIAN_POINT ( 'NONE',  ( 29.16732601703412442, 1436.844822267699328, 136.7085307917412820 ) ) ;
#60513=LINE ( 'NONE', #15694, #96565 ) ;
#60515=CARTESIAN_POINT ( 'NONE',  ( 6.016808910419999989, 1396.654460028929861, 220.0432386207980073 ) ) ;
#60517=DIRECTION ( 'NONE',  ( -0.000000000000000000, -0.000000000000000000, 1.000000000000000000 ) ) ;
#60520=B_SPLINE_CURVE_WITH_KNOTS ( 'NONE', 3,
 ( #92317, #23993, #23462, #66608, #31313, #31866, #101249, #13948, #47580, #30763, #65497, #15046, #73890, #82277, #91768, #57656, #83366, #99606, #99057, #58189 ),
 .UNSPECIFIED., .F., .F.,
 ( 4, 2, 1, 2, 2, 1, 1, 1, 1, 1, 2, 2, 4 ),
 ( 0.000000000000000000, 0.2499999999997811750, 0.3749999999996714295, 0.4374999999996159739, 0.4999999999995604627, 0.6249999999994507727, 0.6874999999993959277, 0.7187499999993685051, 0.7343749999993555155, 0.7421874999993490762, 0.7460937499993504085, 0.7499999999993517408, 1.000000000000000000 ),
 .UNSPECIFIED. ) ;
#60521=VECTOR ( 'NONE', #62565, 1000.000000000000000 ) ;
#60522=CARTESIAN_POINT ( 'NONE',  ( 2.664554167960305531, 1448.256636475937967, 183.4094032644174774 ) ) ;
#60526=CARTESIAN_POINT ( 'NONE',  ( 2.499999990390000093, 1447.656584284949986, 165.9523963823980068 ) ) ;
#60527=CARTESIAN_POINT ( 'NONE',  ( 16.68463225830000241, 1442.773887286369927, 162.0935120917980043 ) ) ;
#60528=CARTESIAN_POINT ( 'NONE',  ( 45.63713230949999655, 1446.564129982419900, 268.9747493906979798 ) ) ;
#60533=VERTEX_POINT ( 'NONE', #109690 ) ;
#60534=CIRCLE ( 'NONE', #101648, 7.975189853890007896 ) ;
#60536=CARTESIAN_POINT ( 'NONE',  ( -24.79630738070000007, 1449.797614630550015, 204.8702466810979956 ) ) ;
#60537=CARTESIAN_POINT ( 'NONE',  ( -10.71712433759610050, 1425.352709571739979, 115.9742016334039931 ) ) ;
#60538=CARTESIAN_POINT ( 'NONE',  ( 17.05828028330499890, 1410.454619143949913, 192.1468146258000047 ) ) ;
#60540=( BOUNDED_CURVE ( )  B_SPLINE_CURVE ( 3, ( #18387, #104067, #45845, #11669 ),
 .UNSPECIFIED., .F., .T. ) 
 B_SPLINE_CURVE_WITH_KNOTS ( ( 4, 4 ),
 ( 5.970709790778379933, 6.887917497424890456 ),
 .UNSPECIFIED. ) 
 CURVE ( )  GEOMETRIC_REPRESENTATION_ITEM ( )  RATIONAL_B_SPLINE_CURVE ( ( 1.000000000000000000, 0.9311142937961904842, 0.9311142937961904842, 1.000000000000000000 ) ) 
 REPRESENTATION_ITEM ( '' )  );
#60541=CARTESIAN_POINT ( 'NONE',  ( 18.39298867610254717, 1509.674607414416414, 185.4216858732138462 ) ) ;
#60543=CARTESIAN_POINT ( 'NONE',  ( -22.09712912739999879, 1489.469559537229998, 208.2081598746609927 ) ) ;
#60544=CARTESIAN_POINT ( 'NONE',  ( -38.63858781420000099, 1428.253854744629962, 261.7057204824979522 ) ) ;
#60546=CARTESIAN_POINT ( 'NONE',  ( 29.61157949199080264, 1509.955833108989964, 209.6611346260839923 ) ) ;
#60548=CARTESIAN_POINT ( 'NONE',  ( -39.39983805167630493, 1440.332349523559969, 136.7601460201240116 ) ) ;
#60550=CARTESIAN_POINT ( 'NONE',  ( 7.602373182780730154, 1397.519631357160051, 197.5586426691019994 ) ) ;
#60552=ADVANCED_FACE ( 'NONE', ( #32966 ), #76079, .F. ) ;
#60553=CARTESIAN_POINT ( 'NONE',  ( -18.16700093809999927, 1457.608413576630028, 229.6942240664980091 ) ) ;
#60556=CARTESIAN_POINT ( 'NONE',  ( -2.439001525050000119, 1430.488531030629929, 150.2249694046979869 ) ) ;
#60557=CARTESIAN_POINT ( 'NONE',  ( -6.413908422285220290, 1429.087440716829860, 154.6253968713650124 ) ) ;
#60563=CARTESIAN_POINT ( 'NONE',  ( -11.87326589167020074, 1432.874500706740037, 149.9809363116050065 ) ) ;
#60572=ORIENTED_EDGE ( 'NONE', *, *, #77509, .F. ) ;
#60573=CARTESIAN_POINT ( 'NONE',  ( 11.81466445377120067, 1428.992090789789927, 148.8655718450160066 ) ) ;
#60575=ORIENTED_EDGE ( 'NONE', *, *, #12720, .T. ) ;
#60576=CARTESIAN_POINT ( 'NONE',  ( -5.367396286529749538, 1487.256192968549840, 235.6479365767530112 ) ) ;
#60577=CARTESIAN_POINT ( 'NONE',  ( -1.549163664599672252, 1484.315319106566676, 182.5664047062095108 ) ) ;
#60578=CARTESIAN_POINT ( 'NONE',  ( 6.944731691349999458, 1508.146090184829973, 235.5513729331979960 ) ) ;
#60580=CARTESIAN_POINT ( 'NONE',  ( -4.938546209390000108, 1422.091193151429934, 185.5889896035980087 ) ) ;
#60581=CARTESIAN_POINT ( 'NONE',  ( 6.401487760110000202, 1408.896291596430046, 270.4245279989980304 ) ) ;
#60586=CARTESIAN_POINT ( 'NONE',  ( -16.92717818009999675, 1496.365422975929960, 223.9021671830980154 ) ) ;
#60588=CARTESIAN_POINT ( 'NONE',  ( 15.48102685469999962, 1453.151875979629949, 195.5243114212979947 ) ) ;
#60589=CARTESIAN_POINT ( 'NONE',  ( -4.734332965765398527, 1423.620278043627195, 184.5217912470845647 ) ) ;
#60590=B_SPLINE_CURVE_WITH_KNOTS ( 'NONE', 3,
 ( #81931, #4686, #106591, #14173, #38825, #89789, #83044, #56751, #90328, #22549, #55666, #23678, #73004, #57861, #21999, #13059, #23120, #40486, #46717, #107139, #91451, #90888, #21456, #5234, #4151, #14728, #30432, #38278, #74661, #108797, #65707, #56192, #64618, #32089 ),
 .UNSPECIFIED., .F., .F.,
 ( 4, 2, 2, 1, 2, 2, 2, 2, 1, 1, 2, 2, 2, 2, 1, 1, 1, 2, 2, 4 ),
 ( 0.03289823588023810252, 0.1537859563936441187, 0.2142298166503383006, 0.2444517467786946618, 0.2595627118428728286, 0.2746736769070509121, 0.3955613974205678396, 0.4560052576774560329, 0.4862271878060093200, 0.5013381528701812417, 0.5088936354023581021, 0.5164491179345348515, 0.6373368384519590979, 0.6977806987106713876, 0.7280026288399379375, 0.7431135939045582228, 0.7506690764368684210, 0.7544468177030233536, 0.7582245589691783971, 1.000000000000000000 ),
 .UNSPECIFIED. ) ;
#60591=CARTESIAN_POINT ( 'NONE',  ( 17.89459807364280053, 1420.234668421669994, 225.0799363196900060 ) ) ;
#60592=CARTESIAN_POINT ( 'NONE',  ( -0.3821804589910179906, 1506.433683733660018, 187.1424611576989889 ) ) ;
#60594=CARTESIAN_POINT ( 'NONE',  ( 18.10086162160209966, 1424.497286396790059, 224.0757393633220147 ) ) ;
#60596=CARTESIAN_POINT ( 'NONE',  ( -2.902930634495347384, 1484.532355139261654, 183.2864040210124301 ) ) ;
#60602=CARTESIAN_POINT ( 'NONE',  ( -11.78833996880000079, 1427.663080501330114, 147.5992344144979995 ) ) ;
#60603=CARTESIAN_POINT ( 'NONE',  ( -14.70619684508450042, 1424.824187292160104, 221.6451186432019824 ) ) ;
#60606=CARTESIAN_POINT ( 'NONE',  ( -1.600048698852036821, 1402.754281879943164, 135.5999999980979851 ) ) ;
#60609=B_SPLINE_CURVE_WITH_KNOTS ( 'NONE', 3,
 ( #73087, #31066, #65246, #31616, #39479, #98824, #4228, #92080, #83133, #5320, #22085, #90412, #56838, #6429, #13692, #64152, #73649, #98271, #107227, #32176 ),
 .UNSPECIFIED., .F., .F.,
 ( 4, 2, 2, 2, 2, 2, 2, 2, 2, 4 ),
 ( -0.3233081010012240353, -0.3219076690093550241, -0.3116608437711600454, -0.3014431805523019592, -0.2809394392387379868, -0.2394106768222920012, -0.1618956485691949998, -0.08327320055462403281, -0.04160395758957841084, 0.000000000000000000 ),
 .UNSPECIFIED. ) ;
#60611=CARTESIAN_POINT ( 'NONE',  ( -15.69727097450000031, 1459.325973232030037, 230.3695337202979658 ) ) ;
#60614=CARTESIAN_POINT ( 'NONE',  ( 26.93223535810000158, 1412.607180478629971, 266.6753325838979549 ) ) ;
#60617=CARTESIAN_POINT ( 'NONE',  ( 21.51393974440000179, 1449.725088386290281, 196.5704810921979799 ) ) ;
#60618=CARTESIAN_POINT ( 'NONE',  ( 18.61615544290965829, 1506.404057880957225, 220.7836781479866488 ) ) ;
#60620=CARTESIAN_POINT ( 'NONE',  ( -0.1860383248606379825, 1508.572757955850193, 237.9075060567579669 ) ) ;
#60622=CARTESIAN_POINT ( 'NONE',  ( -1.474488223160000056, 1450.666087581440024, 182.8694550166979980 ) ) ;
#60623=CARTESIAN_POINT ( 'NONE',  ( -20.23078143836107046, 1506.575640307561571, 200.2219735720721587 ) ) ;
#60625=CARTESIAN_POINT ( 'NONE',  ( -12.26000483520000017, 1442.221945175220071, 187.3548814074979987 ) ) ;
#60627=CARTESIAN_POINT ( 'NONE',  ( 1.476727066854436776, 1407.665894515924492, 270.1373298217981755 ) ) ;
#60629=B_SPLINE_CURVE_WITH_KNOTS ( 'NONE', 3,
 ( #110063, #84306, #51259, #35005, #42869, #59675, #43973 ),
 .UNSPECIFIED., .F., .F.,
 ( 4, 3, 4 ),
 ( 1.117154302310000125, 1.576268520389739969, 1.987970115610000033 ),
 .UNSPECIFIED. ) ;
#60631=CARTESIAN_POINT ( 'NONE',  ( -14.84172366651849906, 1409.431344798339978, 207.4607597228529983 ) ) ;
#60634=CARTESIAN_POINT ( 'NONE',  ( -21.96301590319999875, 1471.883841234629926, 267.3321493710980121 ) ) ;
#60637=DIRECTION ( 'NONE',  ( -0.1402804634174202869, 0.9901118076173992533, 0.000000000000000000 ) ) ;
#60638=CARTESIAN_POINT ( 'NONE',  ( -24.02854045990000031, 1507.902906315029895, 222.3115896357980148 ) ) ;
#60641=CARTESIAN_POINT ( 'NONE',  ( 18.59870848514470154, 1425.273973280189921, 226.9824610977420036 ) ) ;
#60642=CARTESIAN_POINT ( 'NONE',  ( -11.98951922200000020, 1442.759074889710064, 150.6922381223979812 ) ) ;
#60643=CARTESIAN_POINT ( 'NONE',  ( -27.43400997898509885, 1507.980975032430024, 210.8257058971020115 ) ) ;
#60646=CARTESIAN_POINT ( 'NONE',  ( -22.10231210369999744, 1409.684890133530189, 206.6229132878879966 ) ) ;
#60648=ADVANCED_FACE ( 'NONE', ( #32834 ), #40258, .F. ) ;
#60652=CARTESIAN_POINT ( 'NONE',  ( 1.665548205979999974, 1442.756953654919926, 150.7199974615980125 ) ) ;
#60656=CARTESIAN_POINT ( 'NONE',  ( -22.30625446560000213, 1409.857389892729771, 211.0156766885679929 ) ) ;
#60658=CARTESIAN_POINT ( 'NONE',  ( 11.72068376100859943, 1426.706399951889807, 142.9991350588749981 ) ) ;
#60662=CARTESIAN_POINT ( 'NONE',  ( -0.4432577660195479718, 1419.360889940619927, 184.6748336100029917 ) ) ;
#60667=CARTESIAN_POINT ( 'NONE',  ( -18.80219174870000032, 1449.632368031840087, 192.8071008208980004 ) ) ;
#60670=CARTESIAN_POINT ( 'NONE',  ( 41.65674512606190660, 1443.992382921810076, 135.6789720546150022 ) ) ;
#60673=EDGE_CURVE ( 'NONE', #19921, #107891, #34773, .T. ) ;
#60675=CARTESIAN_POINT ( 'NONE',  ( 11.18588343651039985, 1434.156361913030196, 151.6248574816150096 ) ) ;
#60676=CARTESIAN_POINT ( 'NONE',  ( 26.63180687360000221, 1507.995766902830155, 215.9642881313679936 ) ) ;
#60677=ORIENTED_EDGE ( 'NONE', *, *, #78500, .T. ) ;
#60678=CARTESIAN_POINT ( 'NONE',  ( -0.0002529191108078910699, 1396.476793851151797, 221.5132489248241541 ) ) ;
#60681=CARTESIAN_POINT ( 'NONE',  ( 16.08363593346519949, 1424.545651981700075, 191.0941551133240068 ) ) ;
#60682=CARTESIAN_POINT ( 'NONE',  ( 9.393138309199999370, 1428.175987565129844, 133.6118001900980232 ) ) ;
#60683=CARTESIAN_POINT ( 'NONE',  ( 17.62975177240000235, 1507.813572038729944, 230.7540342202979957 ) ) ;
#60687=CARTESIAN_POINT ( 'NONE',  ( -0.2210648318990000027, 1414.913060387329779, 192.7531927952979913 ) ) ;
#60688=CARTESIAN_POINT ( 'NONE',  ( 15.83431121279999942, 1409.466006706529924, 225.8541798896980026 ) ) ;
#60691=CARTESIAN_POINT ( 'NONE',  ( 13.77282262629899989, 1415.219159636060112, 197.5495014860289871 ) ) ;
#60695=CARTESIAN_POINT ( 'NONE',  ( 14.34562267347200049, 1435.962350135230054, 149.9318665393219874 ) ) ;
#60708=CARTESIAN_POINT ( 'NONE',  ( 4.285590139556119560, 1446.892837359970144, 155.6593302246760118 ) ) ;
#60709=CIRCLE ( 'NONE', #40758, 2.000000000550006263 ) ;
#60711=CARTESIAN_POINT ( 'NONE',  ( 0.02089333571419999674, 1507.111761158929994, 237.3522808961980104 ) ) ;
#60712=EDGE_LOOP ( 'NONE', ( #48704, #72263, #65342, #12904, #87555 ) ) ;
#60716=CARTESIAN_POINT ( 'NONE',  ( -18.97264762389999859, 1509.488247232329968, 230.9952461704979783 ) ) ;
#60719=CARTESIAN_POINT ( 'NONE',  ( -12.96785963179999968, 1409.365908024330110, 191.2854579259980312 ) ) ;
#60720=DIRECTION ( 'NONE',  ( -1.000000000000000000, 0.000000000000000000, -1.942890293094025713E-13 ) ) ;
#60723=CARTESIAN_POINT ( 'NONE',  ( 19.74776305319999636, 1427.029108294729895, 221.9964930508980103 ) ) ;
#60728=CARTESIAN_POINT ( 'NONE',  ( 5.440910205060000671, 1437.356219380560105, 154.7142170579979847 ) ) ;
#60730=B_SPLINE_SURFACE_WITH_KNOTS ( 'NONE', 5, 5, ( 
 ( #17519, #51721, #19176, #69645, #104316, #770 ),
 ( #2444, #60688, #94812, #61794, #95916, #102093 ),
 ( #18088, #59567, #103768, #52283, #27070, #61254 ),
 ( #95369, #51161, #18632, #85288, #98659, #71311 ),
 ( #89712, #12990, #107066, #106517, #29806, #70758 ),
 ( #11913, #37110, #105424, #46089, #90252, #46639 ),
 ( #88086, #4616, #47173, #28715, #11374, #21923 ),
 ( #81301, #12457, #13534, #55588, #62921, #38750 ),
 ( #55039, #56118, #96472, #54498, #5154, #72927 ),
 ( #80221, #62347, #30351, #97031, #64542, #45545 ),
 ( #89166, #72388, #47720, #81851, #80773, #19751 ),
 ( #104869, #20294, #28158, #88634, #53952, #63994 ),
 ( #79685, #2991, #4080, #3539, #38205, #37662 ),
 ( #98105, #71868, #105985, #97571, #29260, #63452 ),
 ( #20843, #21379, #101383, #84060, #82424, #73482 ) ),
 .UNSPECIFIED., .F., .F., .F.,
 ( 6, 3, 3, 3, 6 ),
 ( 6, 6 ),
 ( 21.66346097059999920, 24.40199430689999716, 27.78806269829999920, 31.17413108959999946, 40.68480120859999971 ),
 ( 0.000000000000000000, 1.455162240349999969 ),
 .UNSPECIFIED. ) ;
#60734=CARTESIAN_POINT ( 'NONE',  ( 27.92763725140000020, 1508.597377706630141, 207.9063415346780062 ) ) ;
#60741=CARTESIAN_POINT ( 'NONE',  ( 18.32013006829999924, 1469.450921912629838, 259.8063787264979965 ) ) ;
#60744=CARTESIAN_POINT ( 'NONE',  ( -8.365520703090000509, 1508.201466052729984, 235.3634618713980160 ) ) ;
#60745=CARTESIAN_POINT ( 'NONE',  ( -23.04921901699999864, 1449.613099141539806, 219.4632572156979791 ) ) ;
#60746=CARTESIAN_POINT ( 'NONE',  ( 11.31243771429999967, 1433.012838418620049, 151.5204583748979985 ) ) ;
#60747=CARTESIAN_POINT ( 'NONE',  ( 17.64171352730929954, 1409.900445066939938, 222.6954652476910042 ) ) ;
#60752=CARTESIAN_POINT ( 'NONE',  ( 0.2135597935630000055, 1406.506901924230078, 269.4986771210980123 ) ) ;
#60753=CARTESIAN_POINT ( 'NONE',  ( -16.68463225830000241, 1445.052233488290085, 162.0935120917980043 ) ) ;
#60757=CARTESIAN_POINT ( 'NONE',  ( -40.19808943040000315, 1445.100537817090071, 136.9456357583980264 ) ) ;
#60759=CARTESIAN_POINT ( 'NONE',  ( -41.30732298605509811, 1440.913060409350010, 261.0633855307339672 ) ) ;
#60761=CARTESIAN_POINT ( 'NONE',  ( -25.87097295179999890, 1447.207377453609979, 138.1950503254980163 ) ) ;
#60762=CARTESIAN_POINT ( 'NONE',  ( 3.996802888650000299E-15, 1462.614442895030152, 248.0989693021979861 ) ) ;
#60766=CARTESIAN_POINT ( 'NONE',  ( -41.84160635743404555, 1444.586462184261563, 269.6439780239310835 ) ) ;
#60769=CARTESIAN_POINT ( 'NONE',  ( -43.50000000000000000, 1440.913060387330006, 271.1218459616979999 ) ) ;
#60770=CARTESIAN_POINT ( 'NONE',  ( 12.06145328220000046, 1433.903212736219984, 146.4342173386980051 ) ) ;
#60772=CARTESIAN_POINT ( 'NONE',  ( 16.67515766384740061, 1499.299502726869832, 188.3559378578410133 ) ) ;
#60773=CARTESIAN_POINT ( 'NONE',  ( -0.4730976197839999453, 1415.788367959630023, 233.4112646266979993 ) ) ;
#60775=CARTESIAN_POINT ( 'NONE',  ( 12.98226713004290112, 1414.913060387349788, 198.3280232619060257 ) ) ;
#60776=CARTESIAN_POINT ( 'NONE',  ( -28.32265146449999804, 1509.673549455229931, 210.9825397907879960 ) ) ;
#60780=CARTESIAN_POINT ( 'NONE',  ( -7.872185816540564929, 1417.087241613852939, 230.9975226091719662 ) ) ;
#60781=CARTESIAN_POINT ( 'NONE',  ( -18.95816141779999953, 1416.822690122629865, 207.7797354037080027 ) ) ;
#60782=CARTESIAN_POINT ( 'NONE',  ( -16.09938272070019849, 1414.913060387399810, 208.8977458501949798 ) ) ;
#60783=CARTESIAN_POINT ( 'NONE',  ( 24.76897219210000145, 1435.437797603480021, 136.5355265435979959 ) ) ;
#60784=CARTESIAN_POINT ( 'NONE',  ( -8.919399434642100388, 1396.224532680279935, 202.5884989200089876 ) ) ;
#60785=ORIENTED_EDGE ( 'NONE', *, *, #66585, .F. ) ;
#60786=CARTESIAN_POINT ( 'NONE',  ( -17.25862514696109784, 1410.597661782969908, 225.9222092880160062 ) ) ;
#60787=CARTESIAN_POINT ( 'NONE',  ( 9.709302419510001059, 1435.943783413959864, 148.7752736812980174 ) ) ;
#60788=ORIENTED_EDGE ( 'NONE', *, *, #69222, .F. ) ;
#60789=ORIENTED_EDGE ( 'NONE', *, *, #102212, .T. ) ;
#60792=CARTESIAN_POINT ( 'NONE',  ( 11.08043720809999932, 1426.486562227929880, 96.53290481169779014 ) ) ;
#60795=CARTESIAN_POINT ( 'NONE',  ( -11.16671941230000087, 1433.086908617769950, 151.6208637079979837 ) ) ;
#60796=CARTESIAN_POINT ( 'NONE',  ( -2.505371996947532764, 1421.285840239624122, 184.5372720782322062 ) ) ;
#60798=B_SPLINE_CURVE_WITH_KNOTS ( 'NONE', 3,
 ( #88804, #37854, #27241, #19369, #54129, #106156, #61978, #11549, #27790, #29434, #72039, #2066, #53571, #3722, #88256, #36197, #63633, #45725, #70381, #95545, #18818, #87718, #78750, #79862, #21018, #37304, #3172, #12087, #10436, #105617, #9881, #104498, #28901, #63097, #45169, #80409, #86590, #44050, #78188, #4784 ),
 .UNSPECIFIED., .F., .F.,
 ( 4, 3, 3, 3, 3, 3, 3, 3, 3, 3, 3, 3, 3, 4 ),
 ( 0.8628048341553139489, 0.9513106579048509204, 1.049709543750630081, 1.141232170367520116, 1.227831679639869833, 1.304547853099820021, 1.314431188912210002, 1.386913577912220141, 1.463820618845149912, 1.546979327982200170, 1.643200469919150031, 1.736730672401769926, 1.817733512948600083, 1.883620747549999752 ),
 .UNSPECIFIED. ) ;
#60800=CARTESIAN_POINT ( 'NONE',  ( 7.823092546549999859, 1509.180139508929869, 181.1432147337980041 ) ) ;
#60801=CARTESIAN_POINT ( 'NONE',  ( 2.499404917449999708, 1449.013041636889966, 182.6008070574980025 ) ) ;
#60804=VERTEX_POINT ( 'NONE', #64566 ) ;
#60805=ORIENTED_EDGE ( 'NONE', *, *, #109539, .T. ) ;
#60807=CARTESIAN_POINT ( 'NONE',  ( -40.26396437200000378, 1444.186536724029793, 137.1012290770979973 ) ) ;
#60809=CARTESIAN_POINT ( 'NONE',  ( -2.328501808469999990, 1473.856926935030060, 270.2917565481980091 ) ) ;
#60811=CARTESIAN_POINT ( 'NONE',  ( -2.043810040229999903, 1485.976622560129954, 182.1080309692979995 ) ) ;
#60814=CARTESIAN_POINT ( 'NONE',  ( 14.03281819417741794, 1434.988470691964494, 148.9022204816306783 ) ) ;
#60816=CARTESIAN_POINT ( 'NONE',  ( 21.13431350049999935, 1409.651086877429861, 206.4149709229679956 ) ) ;
#60818=CARTESIAN_POINT ( 'NONE',  ( -2.500000000000000000, 1448.208035806080034, 170.3313966091649831 ) ) ;
#60820=CARTESIAN_POINT ( 'NONE',  ( 15.26728741790000043, 1409.446205812130074, 212.2704896688680094 ) ) ;
#60821=CARTESIAN_POINT ( 'NONE',  ( -24.18815601759459710, 1410.823802913859936, 267.6036696494369949 ) ) ;
#60824=FACE_OUTER_BOUND ( 'NONE', #1307, .T. ) ;
#60825=CARTESIAN_POINT ( 'NONE',  ( 13.46738723530000037, 1443.320881723499951, 188.5256231623980057 ) ) ;
#60827=ORIENTED_EDGE ( 'NONE', *, *, #84518, .F. ) ;
#60832=CARTESIAN_POINT ( 'NONE',  ( -16.64354896040000042, 1485.485022283829949, 188.0123015010980225 ) ) ;
#60833=ORIENTED_EDGE ( 'NONE', *, *, #96028, .F. ) ;
#60835=CARTESIAN_POINT ( 'NONE',  ( 10.06907646880000051, 1416.520322351229879, 224.7759792403979873 ) ) ;
#60838=CARTESIAN_POINT ( 'NONE',  ( -26.76880870690000336, 1508.588124793430097, 202.6010433452480015 ) ) ;
#60839=B_SPLINE_SURFACE_WITH_KNOTS ( 'NONE', 5, 5, ( 
 ( #87640, #110618, #17067, #85397, #34465, #68641, #77578, #18198, #103296 ),
 ( #102741, #1420, #26037, #60230, #17627, #51832, #103873, #85969, #35009 ),
 ( #69190, #60800, #35560, #27173, #69756, #61358, #38313, #3101, #13640 ),
 ( #55155, #12573, #47280, #2550, #88738, #71426, #56232, #45656, #36675 ),
 ( #22035, #97132, #98221, #79795, #20401, #70868, #105542, #4715, #55703 ),
 ( #46753, #12022, #11480, #89276, #37230, #46202, #90362, #19858, #21491 ),
 ( #28829, #89824, #13096, #80336, #97677, #80884, #81403, #63027, #73037 ),
 ( #4180, #88188, #64100, #72492, #107176, #104981, #96586, #38859, #3653 ),
 ( #37782, #54606, #106083, #71971, #30468, #29361, #63562, #28271, #106621 ) ),
 .UNSPECIFIED., .F., .F., .F.,
 ( 6, 3, 6 ),
 ( 6, 3, 6 ),
 ( 51.29209723529999820, 55.80647300139999345, 63.23243013249999933 ),
 ( 0.000000000000000000, 1.000000000000000000, 2.000000000000000000 ),
 .UNSPECIFIED. ) ;
#60840=CARTESIAN_POINT ( 'NONE',  ( -1.530913323750000110, 1457.944503865530123, 229.8438706612979843 ) ) ;
#60843=CARTESIAN_POINT ( 'NONE',  ( -5.096744314220000405, 1407.739527842629968, 197.0259025076979924 ) ) ;
#60844=CARTESIAN_POINT ( 'NONE',  ( -13.86092708470000012, 1410.765486845930127, 227.1170267252979897 ) ) ;
#60845=AXIS2_PLACEMENT_3D ( 'NONE', #35728, #79945, #21108 ) ;
#60846=CARTESIAN_POINT ( 'NONE',  ( -4.161170380569999772, 1448.299083496910043, 185.1109000857979936 ) ) ;
#60848=CARTESIAN_POINT ( 'NONE',  ( -25.80250405271350189, 1449.911705762070142, 209.5154266393010118 ) ) ;
#60849=CARTESIAN_POINT ( 'NONE',  ( 27.85639448530000095, 1508.131721228930019, 211.5797927016579933 ) ) ;
#60851=CARTESIAN_POINT ( 'NONE',  ( -25.11961111550000325, 1435.876096999659921, 137.1228181144979601 ) ) ;
#60855=CARTESIAN_POINT ( 'NONE',  ( -13.86092830220000138, 1410.765486874730186, 227.1170284388979894 ) ) ;
#60857=CARTESIAN_POINT ( 'NONE',  ( 17.74493927494756917, 1410.896455599894807, 193.0440146115597884 ) ) ;
#60860=ORIENTED_EDGE ( 'NONE', *, *, #110417, .F. ) ;
#60861=DIRECTION ( 'NONE',  ( 0.005791248591755682358, -0.9990828997313954130, -0.04242429615273902305 ) ) ;
#60862=CARTESIAN_POINT ( 'NONE',  ( -5.198406060209999957, 1412.834820857829982, 231.9113671903980105 ) ) ;
#60867=CARTESIAN_POINT ( 'NONE',  ( 12.71795666588089979, 1434.880588916799979, 150.2406740331289825 ) ) ;
#60868=CARTESIAN_POINT ( 'NONE',  ( 16.70365182916559732, 1488.409533293340019, 230.3427702791729814 ) ) ;
#60869=CARTESIAN_POINT ( 'NONE',  ( -22.16710374047699972, 1508.409791915999904, 225.9459590737800170 ) ) ;
#60870=CARTESIAN_POINT ( 'NONE',  ( -1.804213505890000180, 1410.351307731129964, 186.0507930254979954 ) ) ;
#60876=CARTESIAN_POINT ( 'NONE',  ( 19.59880151960000205, 1507.802454151830034, 188.8055342685979952 ) ) ;
#60882=CARTESIAN_POINT ( 'NONE',  ( 2.250613398900000117, 1417.526871923430008, 235.1186440458980087 ) ) ;
#60889=CARTESIAN_POINT ( 'NONE',  ( -2.500000000000000000, 1448.831161628929976, 156.2564907446979987 ) ) ;
#60892=LINE ( 'NONE', #68734, #70024 ) ;
#60896=CARTESIAN_POINT ( 'NONE',  ( 0.5624690339869999889, 1416.828040475229955, 190.4759594386979984 ) ) ;
#60897=EDGE_LOOP ( 'NONE', ( #25653, #97931, #70356, #66205 ) ) ;
#60898=CARTESIAN_POINT ( 'NONE',  ( 1.555728358237469910, 1415.258594621700013, 191.1344422060440138 ) ) ;
#60900=CARTESIAN_POINT ( 'NONE',  ( -24.35286325639999916, 1437.423069115099906, 210.8262286111179833 ) ) ;
#60901=CARTESIAN_POINT ( 'NONE',  ( 8.490083184937372351, 1410.581744779529799, 187.8574485642506318 ) ) ;
#60903=CARTESIAN_POINT ( 'NONE',  ( -5.682125987650000098, 1507.354943063129895, 181.2351845632980201 ) ) ;
#60908=CARTESIAN_POINT ( 'NONE',  ( 10.51221079110000112, 1452.545965898430040, 151.2436542503979808 ) ) ;
#60912=ORIENTED_EDGE ( 'NONE', *, *, #8257, .F. ) ;
#60913=CARTESIAN_POINT ( 'NONE',  ( -1.499137301450000237, 1414.988015881430101, 226.5174425183980134 ) ) ;
#60917=ORIENTED_EDGE ( 'NONE', *, *, #16880, .F. ) ;
#60918=CARTESIAN_POINT ( 'NONE',  ( 14.26923756360000084, 1444.927653052269989, 189.5513799252980220 ) ) ;
#60920=CARTESIAN_POINT ( 'NONE',  ( 39.05972573424099892, 1439.798937998340080, 136.7091803653709974 ) ) ;
#60922=CARTESIAN_POINT ( 'NONE',  ( -37.00345278059999998, 1461.786582490830142, 266.5575584642980402 ) ) ;
#60925=CARTESIAN_POINT ( 'NONE',  ( -0.3241128059390138150, 1452.022536283229101, 183.1062973748274203 ) ) ;
#60926=CARTESIAN_POINT ( 'NONE',  ( -19.96587381370000003, 1485.439095484030076, 190.8600527859979934 ) ) ;
#60927=CARTESIAN_POINT ( 'NONE',  ( 3.782002931730000128, 1409.981075011729899, 185.9772857123979861 ) ) ;
#60929=CARTESIAN_POINT ( 'NONE',  ( -10.64187455999999976, 1435.613678569329977, 152.0651246931979870 ) ) ;
#60931=CARTESIAN_POINT ( 'NONE',  ( -2.500000007081530029, 1439.558618342239924, 156.0464143015570073 ) ) ;
#60933=CARTESIAN_POINT ( 'NONE',  ( -15.34339624849999950, 1451.140281357629874, 150.0590434767980241 ) ) ;
#60934=DIRECTION ( 'NONE',  ( -1.000000000000000000, 0.000000000000000000, 0.000000000000000000 ) ) ;
#60935=ORIENTED_EDGE ( 'NONE', *, *, #11965, .F. ) ;
#60938=CARTESIAN_POINT ( 'NONE',  ( -42.85030839420000603, 1440.913081031859974, 270.2009482344979574 ) ) ;
#60940=CARTESIAN_POINT ( 'NONE',  ( 16.99430370389999823, 1409.506514545230175, 222.6853181780980151 ) ) ;
#60941=CARTESIAN_POINT ( 'NONE',  ( -14.93990653130000013, 1474.157326975930118, 223.6788132323979994 ) ) ;
#60943=CARTESIAN_POINT ( 'NONE',  ( 12.54268436849999979, 1408.913060387329779, 196.5791615931979948 ) ) ;
#60944=CARTESIAN_POINT ( 'NONE',  ( 2.808747117329370102, 1409.051439747440099, 230.5333268725640039 ) ) ;
#60947=CARTESIAN_POINT ( 'NONE',  ( -6.600008894830000195, 1418.414698087630086, 233.6632623300980072 ) ) ;
#60949=CARTESIAN_POINT ( 'NONE',  ( -0.03561849193722856077, 1486.236081325239866, 181.8148870998357438 ) ) ;
#60951=CARTESIAN_POINT ( 'NONE',  ( -45.59604923203520599, 1439.446907945650082, 268.9759714630910139 ) ) ;
#60955=ORIENTED_EDGE ( 'NONE', *, *, #88228, .F. ) ;
#60959=DIRECTION ( 'NONE',  ( -0.1580583862851100141, 0.05644942065497404043, -0.9858148961304372682 ) ) ;
#60961=CARTESIAN_POINT ( 'NONE',  ( -27.01407896124499786, 1450.680786773039927, 136.4484523802679803 ) ) ;
#60968=CARTESIAN_POINT ( 'NONE',  ( -11.60004869885204215, 1426.273944179774844, 138.2686100621498326 ) ) ;
#60972=CARTESIAN_POINT ( 'NONE',  ( -1.196949206029229940, 1410.397523253659983, 269.3347634687119694 ) ) ;
#60974=CARTESIAN_POINT ( 'NONE',  ( 13.24771706019070017, 1421.178600750019996, 230.4496027819150186 ) ) ;
#60975=CARTESIAN_POINT ( 'NONE',  ( -19.39905127559999798, 1468.965135066929861, 192.1826618881979982 ) ) ;
#60977=ORIENTED_EDGE ( 'NONE', *, *, #88350, .F. ) ;
#60979=CARTESIAN_POINT ( 'NONE',  ( -23.38128641711469768, 1410.008593999159984, 209.8535812185940017 ) ) ;
#60981=CARTESIAN_POINT ( 'NONE',  ( -0.3106955533052500051, 1408.923910294080088, 186.0628693114450130 ) ) ;
#60982=CARTESIAN_POINT ( 'NONE',  ( 3.746090737668994031, 1425.475261178803976, 185.1844613459034576 ) ) ;
#60983=CARTESIAN_POINT ( 'NONE',  ( 2.149988386126029882E-09, 1405.989059316979819, 266.9611530767110139 ) ) ;
#60984=CARTESIAN_POINT ( 'NONE',  ( -18.88141956535340071, 1416.640375553479998, 207.5746397123190263 ) ) ;
#60985=CARTESIAN_POINT ( 'NONE',  ( -18.27573668750000380, 1415.858434028029933, 224.7156095421980240 ) ) ;
#60986=CARTESIAN_POINT ( 'NONE',  ( 28.38717579456189810, 1468.332634182270112, 266.6432885125559551 ) ) ;
#60988=CARTESIAN_POINT ( 'NONE',  ( -16.74235579373888783, 1421.658761381258273, 226.9177557065965232 ) ) ;
#60991=CARTESIAN_POINT ( 'NONE',  ( -13.71357727154099848, 1452.801776351230046, 223.1831243803320035 ) ) ;
#60992=CARTESIAN_POINT ( 'NONE',  ( 1.500031508154069826, 1465.928657607109926, 182.9103486047420120 ) ) ;
#60993=CARTESIAN_POINT ( 'NONE',  ( 23.25743447129999808, 1409.985665278929901, 208.2666287018330138 ) ) ;
#60996=B_SPLINE_CURVE_WITH_KNOTS ( 'NONE', 3,
 ( #14694, #6839, #42662, #9055 ),
 .UNSPECIFIED., .F., .F.,
 ( 4, 4 ),
 ( 0.000000000000000000, 1.000000000000000000 ),
 .UNSPECIFIED. ) ;
#60997=CARTESIAN_POINT ( 'NONE',  ( 26.06503905432269974, 1450.770786748769979, 136.6891037940139881 ) ) ;
#60998=B_SPLINE_SURFACE_WITH_KNOTS ( 'NONE', 5, 5, ( 
 ( #29370, #105552, #63035, #29920, #79251, #44541 ),
 ( #96033, #97140, #19866, #63570, #20409, #3662 ),
 ( #10367, #96595, #97686, #89286, #104988, #36683 ),
 ( #104435, #12581, #87648, #54615, #10935, #19304 ),
 ( #46211, #46763, #18751, #28280, #53506, #45665 ),
 ( #88746, #78686, #80893, #27728, #70322, #2002 ) ),
 .UNSPECIFIED., .F., .F., .F.,
 ( 6, 6 ),
 ( 6, 6 ),
 ( 17.66400699469150126, 74.90934630149999407 ),
 ( -1.063042706849999883E-07, 2.000000253050000065 ),
 .UNSPECIFIED. ) ;
#61001=CARTESIAN_POINT ( 'NONE',  ( -18.67054469633437819, 1509.506033879027882, 231.0930226666867782 ) ) ;
#61002=CARTESIAN_POINT ( 'NONE',  ( 17.27342326200000144, 1409.516261619430225, 195.0577033843979962 ) ) ;
#61003=CARTESIAN_POINT ( 'NONE',  ( 13.59716640859999970, 1444.740067931808653, 176.5566119326980754 ) ) ;
#61005=CARTESIAN_POINT ( 'NONE',  ( 0.2586465989230000151, 1417.355845570129759, 235.2053782485980093 ) ) ;
#61006=CARTESIAN_POINT ( 'NONE',  ( -22.79821983952800935, 1432.341711721006504, 215.5993225015029395 ) ) ;
#61007=DIRECTION ( 'NONE',  ( -1.000000000000000000, -8.659264000688481006E-15, 8.115801398047521537E-15 ) ) ;
#61015=CARTESIAN_POINT ( 'NONE',  ( -0.5079764917598921237, 1409.869867835000150, 233.0824847780489790 ) ) ;
#61016=ADVANCED_FACE ( 'NONE', ( #19900 ), #54101, .F. ) ;
#61018=EDGE_CURVE ( 'NONE', #7065, #16730, #4342, .T. ) ;
#61022=CARTESIAN_POINT ( 'NONE',  ( 0.07181797918499399636, 1506.512156827046965, 231.1702880130284825 ) ) ;
#61023=CARTESIAN_POINT ( 'NONE',  ( -17.83186622679999900, 1447.284048007129968, 214.3676144197979738 ) ) ;
#61026=CARTESIAN_POINT ( 'NONE',  ( 11.33026613920000081, 1433.819327792829881, 151.4886452754979871 ) ) ;
#61027=CARTESIAN_POINT ( 'NONE',  ( 10.05164999379999990, 1455.338937666430184, 224.8635561966979708 ) ) ;
#61028=CARTESIAN_POINT ( 'NONE',  ( 25.87170757128150100, 1440.913060398189828, 221.1805615932169928 ) ) ;
#61029=EDGE_CURVE ( 'NONE', #5297, #69813, #105686, .T. ) ;
#61032=CARTESIAN_POINT ( 'NONE',  ( 22.93995821741230046, 1507.616838180419791, 210.4000209873630070 ) ) ;
#61034=ADVANCED_FACE ( 'NONE', ( #26678 ), #81200, .T. ) ;
#61035=CARTESIAN_POINT ( 'NONE',  ( -9.702419644859999082, 1486.515158439930019, 183.3000319968979852 ) ) ;
#61036=CARTESIAN_POINT ( 'NONE',  ( 11.68470739478344633, 1398.259505493948609, 214.8239554649159118 ) ) ;
#61037=CARTESIAN_POINT ( 'NONE',  ( -7.474145394509370099, 1509.174061155270010, 238.5777524316769984 ) ) ;
#61038=CARTESIAN_POINT ( 'NONE',  ( 24.49050335010000268, 1430.357935310629955, 211.3741248221880085 ) ) ;
#61040=CARTESIAN_POINT ( 'NONE',  ( 25.37586499933865980, 1436.619698531014137, 137.3878537005881526 ) ) ;
#61044=EDGE_CURVE ( 'NONE', #35056, #39470, #53530, .T. ) ;
#61046=CARTESIAN_POINT ( 'NONE',  ( 0.1599398962665600221, 1486.303002522280167, 181.8235866827639882 ) ) ;
#61049=CARTESIAN_POINT ( 'NONE',  ( -20.87866911129999892, 1445.052233488290085, 177.0630364655980031 ) ) ;
#61053=CARTESIAN_POINT ( 'NONE',  ( -34.54825073237489619, 1451.683981886159927, 134.0999999981819713 ) ) ;
#61056=VERTEX_POINT ( 'NONE', #50792 ) ;
#61057=CARTESIAN_POINT ( 'NONE',  ( -38.62985698160660775, 1443.711942231680041, 137.1840658718770101 ) ) ;
#61063=EDGE_CURVE ( 'NONE', #60035, #10764, #96345, .T. ) ;
#61070=CARTESIAN_POINT ( 'NONE',  ( -16.88443202019999845, 1417.732921807629964, 191.5454170170979751 ) ) ;
#61074=ADVANCED_FACE ( 'NONE', ( #105622 ), #104471, .T. ) ;
#61080=CARTESIAN_POINT ( 'NONE',  ( 10.80134480061119895, 1441.261220175989820, 153.0805715986579969 ) ) ;
#61083=CARTESIAN_POINT ( 'NONE',  ( 29.11541691865991055, 1509.936068994953985, 213.9146698034000167 ) ) ;
#61085=CARTESIAN_POINT ( 'NONE',  ( 18.99409280968322378, 1437.722685762978472, 213.2647665747184931 ) ) ;
#61086=CARTESIAN_POINT ( 'NONE',  ( 1.621061852049999974, 1416.517833579129956, 232.6452868846980095 ) ) ;
#61088=CARTESIAN_POINT ( 'NONE',  ( -23.54196934549975495, 1507.885283471533057, 223.3642576937991748 ) ) ;
#61090=CARTESIAN_POINT ( 'NONE',  ( 11.86629848900230044, 1432.349867578880094, 149.9824231379060109 ) ) ;
#61093=CARTESIAN_POINT ( 'NONE',  ( -12.95480792804799997, 1435.606741788159979, 150.6280057355330086 ) ) ;
#61095=DIRECTION ( 'NONE',  ( 0.000000000000000000, 0.000000000000000000, -1.000000000000000000 ) ) ;
#61101=CARTESIAN_POINT ( 'NONE',  ( -24.03538182599999828, 1410.920334414829995, 208.4371777575090050 ) ) ;
#61102=CARTESIAN_POINT ( 'NONE',  ( -11.02063524594970012, 1425.659888206090045, 115.9715217809829966 ) ) ;
#61103=CARTESIAN_POINT ( 'NONE',  ( 16.32935405069350310, 1409.491649162750036, 193.0798514163919890 ) ) ;
#61107=CARTESIAN_POINT ( 'NONE',  ( 29.78388735113269803, 1510.063495189237528, 213.0748577344430430 ) ) ;
#61108=CARTESIAN_POINT ( 'NONE',  ( 3.609688916579999299E-14, 1407.650947606430009, 270.1377425326979846 ) ) ;
#61109=CARTESIAN_POINT ( 'NONE',  ( -36.92073679659999641, 1428.724884009829793, 259.2254597838979748 ) ) ;
#61111=CARTESIAN_POINT ( 'NONE',  ( 17.15305875377343980, 1460.277650823117938, 228.6392876217846890 ) ) ;
#61113=CARTESIAN_POINT ( 'NONE',  ( -37.10899643540120252, 1437.976758828390075, 136.5628136915640027 ) ) ;
#61115=CARTESIAN_POINT ( 'NONE',  ( 9.494968296011210285, 1396.244631986520062, 215.6531529143859984 ) ) ;
#61117=CARTESIAN_POINT ( 'NONE',  ( -17.86382746079999606, 1458.127315681930213, 228.6833203829979766 ) ) ;
#61119=ORIENTED_EDGE ( 'NONE', *, *, #32476, .F. ) ;
#61120=CARTESIAN_POINT ( 'NONE',  ( -29.29953909818101110, 1509.936973869758503, 211.6148270279188353 ) ) ;
#61122=EDGE_CURVE ( 'NONE', #14800, #93336, #6893, .T. ) ;
#61123=ORIENTED_EDGE ( 'NONE', *, *, #91157, .T. ) ;
#61125=CARTESIAN_POINT ( 'NONE',  ( -0.1623179403020000022, 1419.314774686130022, 227.4763468986980115 ) ) ;
#61126=DIRECTION ( 'NONE',  ( 0.5161917810414575758, -0.8564730265368828421, 0.000000000000000000 ) ) ;
#61127=CARTESIAN_POINT ( 'NONE',  ( -11.95688248459999947, 1441.464442770860160, 187.7513092272979804 ) ) ;
#61128=CARTESIAN_POINT ( 'NONE',  ( -5.607190395569999986, 1461.190304871029866, 234.0072117241979868 ) ) ;
#61130=CARTESIAN_POINT ( 'NONE',  ( 16.06428795287859757, 1416.913060341709979, 208.9262477897280235 ) ) ;
#61137=CARTESIAN_POINT ( 'NONE',  ( 11.85286409514619876, 1431.415910222289767, 149.9047070638239916 ) ) ;
#61139=EDGE_CURVE ( 'NONE', #68458, #101156, #61571, .T. ) ;
#61144=CARTESIAN_POINT ( 'NONE',  ( 11.15178539160000071, 1509.130341218730109, 235.1839298150979971 ) ) ;
#61146=CARTESIAN_POINT ( 'NONE',  ( -6.086798803919999834, 1421.074767261429997, 186.7378509026979998 ) ) ;
#61147=CARTESIAN_POINT ( 'NONE',  ( 4.801570118712710666, 1410.589679230010006, 269.3375611599190051 ) ) ;
#61152=CARTESIAN_POINT ( 'NONE',  ( 0.02427673352570664661, 1410.268364199324424, 233.2207279706304917 ) ) ;
#61153=CARTESIAN_POINT ( 'NONE',  ( 17.52163758029999840, 1458.428370499130097, 228.8923014477979905 ) ) ;
#61156=CARTESIAN_POINT ( 'NONE',  ( 17.62513008079359977, 1411.506380282780128, 224.8263663906670047 ) ) ;
#61159=AXIS2_PLACEMENT_3D ( 'NONE', #69565, #148, #68451 ) ;
#61160=CARTESIAN_POINT ( 'NONE',  ( 18.36028095489519885, 1424.508247878629845, 223.5128313417529853 ) ) ;
#61167=EDGE_LOOP ( 'NONE', ( #4760, #344, #102748, #21100 ) ) ;
#61172=CARTESIAN_POINT ( 'NONE',  ( -10.88738708772158503, 1426.874992181416246, 149.3593185091482098 ) ) ;
#61176=CARTESIAN_POINT ( 'NONE',  ( 15.48246398699999915, 1412.746519260829928, 227.3113515368980018 ) ) ;
#61179=CARTESIAN_POINT ( 'NONE',  ( -16.32302350474599706, 1459.452451149466015, 228.9511142845270228 ) ) ;
#61181=CARTESIAN_POINT ( 'NONE',  ( 35.95138954689999622, 1418.606347009430010, 266.9995350096980360 ) ) ;
#61182=CARTESIAN_POINT ( 'NONE',  ( 23.74295614150000233, 1435.754861767519969, 139.8124097129980044 ) ) ;
#61183=CARTESIAN_POINT ( 'NONE',  ( 19.58675617150000292, 1469.160532835930098, 191.3852724613979888 ) ) ;
#61185=CARTESIAN_POINT ( 'NONE',  ( -23.47462919730000408, 1434.801338017199896, 212.9388864702380033 ) ) ;
#61188=CARTESIAN_POINT ( 'NONE',  ( -1.514898281969999871, 1450.642619721169922, 182.9341259013979766 ) ) ;
#61189=CARTESIAN_POINT ( 'NONE',  ( -20.25058511782390269, 1506.578946199203983, 200.2602131604447209 ) ) ;
#61191=CARTESIAN_POINT ( 'NONE',  ( -12.53141519090000067, 1442.576458613880050, 187.0189377207979931 ) ) ;
#61193=CARTESIAN_POINT ( 'NONE',  ( -33.52368697869999892, 1435.668148531879979, 135.0787117157979935 ) ) ;
#61194=CARTESIAN_POINT ( 'NONE',  ( -11.98993776207835360, 1454.255640063151986, 224.7705267360378798 ) ) ;
#61195=VERTEX_POINT ( 'NONE', #8095 ) ;
#61197=CARTESIAN_POINT ( 'NONE',  ( -13.86277928319429975, 1409.397159307180118, 203.5545281553519885 ) ) ;
#61201=CIRCLE ( 'NONE', #104076, 38.73358384181149461 ) ;
#61202=CARTESIAN_POINT ( 'NONE',  ( -23.35296189450000170, 1470.315870435830220, 269.4730450806980002 ) ) ;
#61204=CARTESIAN_POINT ( 'NONE',  ( 0.4176721281191659862, 1418.917014445500172, 184.6748447018700006 ) ) ;
#61206=CARTESIAN_POINT ( 'NONE',  ( 18.06747689609889918, 1424.498894469510105, 224.1058871671330053 ) ) ;
#61209=CARTESIAN_POINT ( 'NONE',  ( 17.71170296313739811, 1423.327007561619894, 226.2336102880809960 ) ) ;
#61210=CARTESIAN_POINT ( 'NONE',  ( 20.86076292830000156, 1508.959448910729861, 227.6903812582980038 ) ) ;
#61211=CARTESIAN_POINT ( 'NONE',  ( 14.03776961820000047, 1452.420640915330068, 222.8370746057979943 ) ) ;
#61214=CARTESIAN_POINT ( 'NONE',  ( 3483.362703962769956, 1009.280093926950144, 1152.220420213539910 ) ) ;
#61215=CARTESIAN_POINT ( 'NONE',  ( -23.88946018079999689, 1411.108009500230082, 207.7971124514679957 ) ) ;
#61216=( BOUNDED_CURVE ( )  B_SPLINE_CURVE ( 3, ( #103717, #102586, #9106, #42717 ),
 .UNSPECIFIED., .F., .T. ) 
 B_SPLINE_CURVE_WITH_KNOTS ( ( 4, 4 ),
 ( 3.232438304859030165, 3.299804565595920280 ),
 .UNSPECIFIED. ) 
 CURVE ( )  GEOMETRIC_REPRESENTATION_ITEM ( )  RATIONAL_B_SPLINE_CURVE ( ( 1.000000000000000000, 0.9996218513307064679, 0.9996218513307064679, 1.000000000000000000 ) ) 
 REPRESENTATION_ITEM ( '' )  );
#61217=CARTESIAN_POINT ( 'NONE',  ( 16.67302254290000008, 1414.971352895729979, 208.8753141282829802 ) ) ;
#61224=CARTESIAN_POINT ( 'NONE',  ( -31.03138008755339783, 1441.878430314559864, 137.2367898525090197 ) ) ;
#61228=DIRECTION ( 'NONE',  ( 0.000000000000000000, 1.000000000000000000, 0.000000000000000000 ) ) ;
#61230=CARTESIAN_POINT ( 'NONE',  ( -23.21169520710000000, 1420.930134560530178, 211.3054972004780154 ) ) ;
#61235=CARTESIAN_POINT ( 'NONE',  ( -15.43521629878640056, 1485.016445856970222, 187.3278621968299831 ) ) ;
#61237=AXIS2_PLACEMENT_3D ( 'NONE', #79985, #11143, #44751 ) ;
#61239=CARTESIAN_POINT ( 'NONE',  ( 37.36839315630000158, 1449.335722529840041, 136.3140007074979962 ) ) ;
#61243=CARTESIAN_POINT ( 'NONE',  ( 11.24610669039820010, 1434.034494598100082, 151.5766399473429829 ) ) ;
#61249=CARTESIAN_POINT ( 'NONE',  ( 16.02111279596229920, 1422.399697759369701, 191.1604070481699864 ) ) ;
#61250=CARTESIAN_POINT ( 'NONE',  ( 1.546867617820790075, 1416.839692126689897, 190.2222510973109877 ) ) ;
#61252=CARTESIAN_POINT ( 'NONE',  ( 1.990304530710000241, 1507.640980020629740, 181.1916917869979784 ) ) ;
#61253=CARTESIAN_POINT ( 'NONE',  ( -0.2465318334200000405, 1414.971352895729979, 192.4488234187979856 ) ) ;
#61254=CARTESIAN_POINT ( 'NONE',  ( 15.96357422200000009, 1410.842840262029995, 226.9345609355980002 ) ) ;
#61256=DIRECTION ( 'NONE',  ( 7.205227288424627209E-20, 0.9876883405951701889, 0.1564344650400262826 ) ) ;
#61259=ORIENTED_EDGE ( 'NONE', *, *, #36617, .T. ) ;
#61260=CARTESIAN_POINT ( 'NONE',  ( 13.68291348452850009, 1434.996735757539909, 148.9906729220649879 ) ) ;
#61262=ORIENTED_EDGE ( 'NONE', *, *, #32722, .F. ) ;
#61263=ORIENTED_EDGE ( 'NONE', *, *, #39933, .F. ) ;
#61264=ORIENTED_EDGE ( 'NONE', *, *, #32258, .F. ) ;
#61266=CARTESIAN_POINT ( 'NONE',  ( -3.068665118410000225, 1464.761382153330032, 237.1705660322979838 ) ) ;
#61267=EDGE_CURVE ( 'NONE', #48668, #89451, #25519, .T. ) ;
#61268=CARTESIAN_POINT ( 'NONE',  ( 29.22958591724099975, 1509.933780020319773, 206.4713313096740137 ) ) ;
#61271=CARTESIAN_POINT ( 'NONE',  ( -19.09275713913258699, 1441.344922765982346, 209.9503379368030380 ) ) ;
#61273=CARTESIAN_POINT ( 'NONE',  ( 4.221729048143290086, 1446.223289964359992, 169.8973273558370067 ) ) ;
#61275=EDGE_LOOP ( 'NONE', ( #20002, #68539, #12601, #1408 ) ) ;
#61277=ORIENTED_EDGE ( 'NONE', *, *, #29028, .F. ) ;
#61278=CARTESIAN_POINT ( 'NONE',  ( 19.62250382303630047, 1440.913060387330006, 213.8950623188489999 ) ) ;
#61280=CARTESIAN_POINT ( 'NONE',  ( -17.69093279879999869, 1507.793158530429764, 186.8252671473979944 ) ) ;
#61282=CARTESIAN_POINT ( 'NONE',  ( -33.93390015750107835, 1451.270656932794054, 135.9469490811935657 ) ) ;
#61283=CARTESIAN_POINT ( 'NONE',  ( -15.18915102340000089, 1410.375618971030008, 190.8776686048979911 ) ) ;
#61284=CARTESIAN_POINT ( 'NONE',  ( -24.35834046960000165, 1442.143026477599960, 211.4091606738980147 ) ) ;
#61286=CARTESIAN_POINT ( 'NONE',  ( 11.49747572422220188, 1414.913060387329779, 220.3427040978150160 ) ) ;
#61287=CARTESIAN_POINT ( 'NONE',  ( -13.06845456229791047, 1434.810982766093957, 146.9332176485133630 ) ) ;
#61289=CARTESIAN_POINT ( 'NONE',  ( -12.84579503169999803, 1434.992946303999815, 194.0992193082979895 ) ) ;
#61295=CARTESIAN_POINT ( 'NONE',  ( 28.45104061960000053, 1509.631525885230076, 207.4803073972880156 ) ) ;
#61298=CARTESIAN_POINT ( 'NONE',  ( -17.22789533397991235, 1486.134374014700143, 187.8660400835535711 ) ) ;
#61300=ORIENTED_EDGE ( 'NONE', *, *, #68243, .T. ) ;
#61301=CARTESIAN_POINT ( 'NONE',  ( 28.09269446560000105, 1442.732147117420254, 231.9538848060979888 ) ) ;
#61303=CARTESIAN_POINT ( 'NONE',  ( 3.838688366592032608, 1449.941958011591623, 184.1981631407757618 ) ) ;
#61304=CARTESIAN_POINT ( 'NONE',  ( -27.73912773776899954, 1509.881732072950172, 218.7146610652550009 ) ) ;
#61305=CARTESIAN_POINT ( 'NONE',  ( -8.472821806374909670, 1509.208940765679927, 237.1966872052409769 ) ) ;
#61307=CARTESIAN_POINT ( 'NONE',  ( -20.54907931089999806, 1454.472754293929938, 224.8058317932980117 ) ) ;
#61308=ADVANCED_FACE ( 'NONE', ( #81880 ), #4469, .F. ) ;
#61309=DIRECTION ( 'NONE',  ( 0.9861488065241343914, 0.1648740305507690185, -0.01808550361393360464 ) ) ;
#61310=CARTESIAN_POINT ( 'NONE',  ( 17.99628978319960027, 1410.830115193840129, 222.9828712447109922 ) ) ;
#61311=DIRECTION ( 'NONE',  ( 0.000000000000000000, 1.000000000000000000, 0.000000000000000000 ) ) ;
#61315=CARTESIAN_POINT ( 'NONE',  ( 0.1075625203479999986, 1405.989059426929998, 266.9611530679979978 ) ) ;
#61316=CARTESIAN_POINT ( 'NONE',  ( 27.79064032830000031, 1508.605033450530073, 207.7520403031080036 ) ) ;
#61318=CARTESIAN_POINT ( 'NONE',  ( -4.041028775053940565E-06, 1471.436293264230017, 269.3346704911970164 ) ) ;
#61319=CARTESIAN_POINT ( 'NONE',  ( 2.478173748110000130, 1439.527585047869934, 157.7653643411979658 ) ) ;
#61321=CARTESIAN_POINT ( 'NONE',  ( -20.01701399148389982, 1508.375005217440048, 188.9474772628149992 ) ) ;
#61322=CARTESIAN_POINT ( 'NONE',  ( -44.35579534389660239, 1440.913060402619976, 264.7564585019449623 ) ) ;
#61323=CARTESIAN_POINT ( 'NONE',  ( 34.03745954885479819, 1450.435860261120069, 136.2418865863519954 ) ) ;
#61324=CARTESIAN_POINT ( 'NONE',  ( -1.958645825849109734, 1450.346086741789804, 154.2463840937579960 ) ) ;
#61330=CARTESIAN_POINT ( 'NONE',  ( -31.70762145559999468, 1417.952368988429953, 271.1218459616979999 ) ) ;
#61333=CARTESIAN_POINT ( 'NONE',  ( -0.5895635512679999746, 1417.370800527230131, 235.1640457548979839 ) ) ;
#61339=CARTESIAN_POINT ( 'NONE',  ( -18.34708879960000161, 1415.579607672129896, 208.2154979986029844 ) ) ;
#61341=CARTESIAN_POINT ( 'NONE',  ( 26.52894651520460201, 1435.730259070040120, 136.2304755143660202 ) ) ;
#61342=CARTESIAN_POINT ( 'NONE',  ( -13.33659772418124767, 1443.292211361891077, 169.3747828019180872 ) ) ;
#61343=EDGE_CURVE ( 'NONE', #80182, #69002, #89584, .T. ) ;
#61345=CARTESIAN_POINT ( 'NONE',  ( -16.22271312188570036, 1409.479543335319931, 225.1382318463119816 ) ) ;
#61350=CARTESIAN_POINT ( 'NONE',  ( 11.09105272649999918, 1426.482985488930126, 97.30048952069790857 ) ) ;
#61351=CARTESIAN_POINT ( 'NONE',  ( -16.68597733941929917, 1461.099535985040120, 230.2790158113629957 ) ) ;
#61353=CARTESIAN_POINT ( 'NONE',  ( 4.408870434958439333, 1425.824683284920184, 185.4670092970000042 ) ) ;
#61358=CARTESIAN_POINT ( 'NONE',  ( 7.361717033309999714, 1508.153716861730118, 182.4941886473980048 ) ) ;
#61361=CARTESIAN_POINT ( 'NONE',  ( -5.374569360760125036, 1464.404629561533966, 236.8301563712954874 ) ) ;
#61365=CARTESIAN_POINT ( 'NONE',  ( 4.359368621329999693E-15, 1471.436294014630221, 269.3346704429980036 ) ) ;
#61367=CARTESIAN_POINT ( 'NONE',  ( -2.794587184679999670, 1486.518066062529897, 181.7593184408980278 ) ) ;
#61368=B_SPLINE_CURVE_WITH_KNOTS ( 'NONE', 5,
 ( #49521, #83106, #6941, #109422, #101531, #58466, #92593, #6400, #24820 ),
 .UNSPECIFIED., .F., .F.,
 ( 6, 3, 6 ),
 ( 127.6642502654205487, 131.5832540680000022, 137.5414126590000023 ),
 .UNSPECIFIED. ) ;
#61371=CARTESIAN_POINT ( 'NONE',  ( 21.62710397070000212, 1409.668295492329889, 206.7322786019380203 ) ) ;
#61372=FACE_OUTER_BOUND ( 'NONE', #93033, .T. ) ;
#61374=CARTESIAN_POINT ( 'NONE',  ( 6.993398322862810268, 1409.157275238040029, 195.4924656238740113 ) ) ;
#61375=CARTESIAN_POINT ( 'NONE',  ( 5.576759338873839723E-05, 1405.989119098810079, 266.9610487349989967 ) ) ;
#61376=CARTESIAN_POINT ( 'NONE',  ( -13.91110666395790041, 1435.008848373910041, 148.8314041724960077 ) ) ;
#61377=ORIENTED_EDGE ( 'NONE', *, *, #50407, .T. ) ;
#61378=CARTESIAN_POINT ( 'NONE',  ( -11.30198679499999947, 1432.355652606760032, 151.5220046058980188 ) ) ;
#61379=CARTESIAN_POINT ( 'NONE',  ( 13.50628347229999981, 1442.279780698270088, 189.1190317712979834 ) ) ;
#61380=VERTEX_POINT ( 'NONE', #13977 ) ;
#61381=VERTEX_POINT ( 'NONE', #91250 ) ;
#61382=CARTESIAN_POINT ( 'NONE',  ( -22.28696231330000188, 1506.798305107829947, 208.8466800722590051 ) ) ;
#61386=B_SPLINE_SURFACE_WITH_KNOTS ( 'NONE', 5, 5, ( 
 ( #87852, #62108, #19509, #62673, #11140, #79440 ),
 ( #2752, #36872, #96794, #54258, #88384, #45851 ),
 ( #79983, #3302, #89482, #105751, #91129, #39633 ),
 ( #12777, #55348, #47490, #73802, #46954, #54795 ),
 ( #64305, #97327, #88927, #30674, #48599, #12213 ),
 ( #38517, #82733, #64861, #81613, #90572, #39057 ) ),
 .UNSPECIFIED., .F., .F., .F.,
 ( 6, 6 ),
 ( 6, 6 ),
 ( 6.281102661440000290, 8.354490254749999067 ),
 ( 0.000000000000000000, 1.450255543799999991 ),
 .UNSPECIFIED. ) ;
#61387=ORIENTED_EDGE ( 'NONE', *, *, #32902, .F. ) ;
#61391=CARTESIAN_POINT ( 'NONE',  ( -26.57809186909999966, 1508.585461716229929, 202.0629932667179958 ) ) ;
#61399=CARTESIAN_POINT ( 'NONE',  ( 27.42695472179999783, 1451.955572177629847, 134.9063961680979844 ) ) ;
#61401=CARTESIAN_POINT ( 'NONE',  ( 19.28184285025260181, 1456.939734798050267, 224.6612775436279890 ) ) ;
#61402=CARTESIAN_POINT ( 'NONE',  ( -24.39026675770000097, 1435.355298166539797, 136.4119318075979947 ) ) ;
#61405=CARTESIAN_POINT ( 'NONE',  ( 0.01871782600107488662, 1507.454862520212146, 237.3968338320200075 ) ) ;
#61406=DIRECTION ( 'NONE',  ( -0.3363363969979660806, 0.9417419115949053898, 0.000000000000000000 ) ) ;
#61407=CARTESIAN_POINT ( 'NONE',  ( 19.18147675296038557, 1410.944559830756589, 195.6234844512586335 ) ) ;
#61409=ORIENTED_EDGE ( 'NONE', *, *, #68491, .T. ) ;
#61410=CARTESIAN_POINT ( 'NONE',  ( 2.500000000000000000, 1437.283720389809787, 157.6542335194979785 ) ) ;
#61411=CARTESIAN_POINT ( 'NONE',  ( -1.368591974409999912, 1412.843971119630169, 233.0744961443979832 ) ) ;
#61416=CARTESIAN_POINT ( 'NONE',  ( 11.84288159193510026, 1435.129470572849868, 151.2381383328829827 ) ) ;
#61417=ADVANCED_FACE ( 'NONE', ( #81187 ), #57124, .F. ) ;
#61418=CARTESIAN_POINT ( 'NONE',  ( 15.05624239712749990, 1469.004309107100198, 230.3228700955960164 ) ) ;
#61419=CARTESIAN_POINT ( 'NONE',  ( -22.10329645359099970, 1509.714832913870168, 228.9299748702250099 ) ) ;
#61420=FACE_OUTER_BOUND ( 'NONE', #104048, .T. ) ;
#61421=CARTESIAN_POINT ( 'NONE',  ( -0.04703688478509999993, 1408.914702951529762, 231.7816009520980174 ) ) ;
#61422=CARTESIAN_POINT ( 'NONE',  ( -14.45783243223209880, 1416.839692136300073, 221.3920770721769884 ) ) ;
#61427=ORIENTED_EDGE ( 'NONE', *, *, #31211, .T. ) ;
#61429=CARTESIAN_POINT ( 'NONE',  ( -6.195568093309999469, 1495.113783496430187, 181.4148133623980073 ) ) ;
#61430=ORIENTED_EDGE ( 'NONE', *, *, #16752, .T. ) ;
#61431=CARTESIAN_POINT ( 'NONE',  ( 0.6621667027629999369, 1417.277712856329799, 235.8679543975979982 ) ) ;
#61432=EDGE_CURVE ( 'NONE', #33631, #100091, #99082, .T. ) ;
#61437=CARTESIAN_POINT ( 'NONE',  ( 2.566893074593609807E-08, 1406.911841303630126, 196.1218459607310081 ) ) ;
#61438=CARTESIAN_POINT ( 'NONE',  ( -2.712106650090000404, 1447.524051941180005, 157.8378498936980066 ) ) ;
#61439=CARTESIAN_POINT ( 'NONE',  ( -11.86716023049999968, 1432.353341358199941, 147.6509521729980179 ) ) ;
#61440=CARTESIAN_POINT ( 'NONE',  ( -14.25739833390000122, 1435.140225252410119, 149.2707004493980207 ) ) ;
#61442=CARTESIAN_POINT ( 'NONE',  ( -11.86716023049999968, 1432.353341358199941, 147.6509521729980179 ) ) ;
#61443=CARTESIAN_POINT ( 'NONE',  ( -1.746314907631250080, 1462.701329518090006, 183.7072431146600024 ) ) ;
#61444=CARTESIAN_POINT ( 'NONE',  ( 1.234665194121939980, 1409.459554382089891, 232.4871809079789955 ) ) ;
#61445=CARTESIAN_POINT ( 'NONE',  ( 0.5950580025862760580, 1496.414336839329962, 186.9683653809459827 ) ) ;
#61448=CARTESIAN_POINT ( 'NONE',  ( 1.552532731868270011, 1415.658863691610122, 190.6831114793849906 ) ) ;
#61449=FACE_OUTER_BOUND ( 'NONE', #39032, .T. ) ;
#61450=CARTESIAN_POINT ( 'NONE',  ( -11.87502386937130083, 1433.007271227619867, 149.9804723889419904 ) ) ;
#61451=CARTESIAN_POINT ( 'NONE',  ( 2.866730800962757897, 1410.390819565074935, 185.6792981423243418 ) ) ;
#61452=CARTESIAN_POINT ( 'NONE',  ( -16.68463225901000158, 1445.052233488270076, 162.0935120915889911 ) ) ;
#61454=CARTESIAN_POINT ( 'NONE',  ( -14.38070771612859922, 1509.494654091789926, 182.9202028628729977 ) ) ;
#61459=DIRECTION ( 'NONE',  ( 0.6456859402676993209, 6.919574257186762174E-11, -0.7636030818040332457 ) ) ;
#61462=ORIENTED_EDGE ( 'NONE', *, *, #65928, .T. ) ;
#61463=CARTESIAN_POINT ( 'NONE',  ( -1.547463840030000037, 1414.913060387329779, 225.9340782259980074 ) ) ;
#61465=CARTESIAN_POINT ( 'NONE',  ( 20.00533500179399837, 1509.034491922330062, 229.7041300313120189 ) ) ;
#61467=EDGE_LOOP ( 'NONE', ( #103175, #74037, #92459, #82305 ) ) ;
#61468=CARTESIAN_POINT ( 'NONE',  ( 17.61796568584639999, 1509.217857668270199, 231.5269859153089840 ) ) ;
#61469=LINE ( 'NONE', #95595, #88597 ) ;
#61470=CARTESIAN_POINT ( 'NONE',  ( 12.77009498041144653, 1442.833833548704433, 169.4527319213308942 ) ) ;
#61472=CARTESIAN_POINT ( 'NONE',  ( -13.60516178560000000, 1473.691177536529949, 264.8398105707980221 ) ) ;
#61476=CARTESIAN_POINT ( 'NONE',  ( -19.69052972445629734, 1491.856921643429814, 228.3926998087940206 ) ) ;
#61477=CARTESIAN_POINT ( 'NONE',  ( 12.38635162149999935, 1409.511637224330116, 190.7239812732980226 ) ) ;
#61478=CARTESIAN_POINT ( 'NONE',  ( 5.210919876389999317, 1421.200875282130028, 185.9499441207979942 ) ) ;
#61479=CARTESIAN_POINT ( 'NONE',  ( -5.268693358010000161, 1440.707873534420060, 154.8524945673979971 ) ) ;
#61480=CARTESIAN_POINT ( 'NONE',  ( 12.48849012109999990, 1435.526020131319910, 150.8975386375979895 ) ) ;
#61483=CARTESIAN_POINT ( 'NONE',  ( 2.194849219480000002, 1464.708290797229893, 236.4512993078980116 ) ) ;
#61485=CARTESIAN_POINT ( 'NONE',  ( -18.64588652299999794, 1416.828040475229955, 208.5593769277110141 ) ) ;
#61487=CARTESIAN_POINT ( 'NONE',  ( -38.62502730119999939, 1456.952829106630134, 270.2651245533980386 ) ) ;
#61489=CARTESIAN_POINT ( 'NONE',  ( 17.45344422499999837, 1410.019001477129905, 223.6090892349980095 ) ) ;
#61490=CARTESIAN_POINT ( 'NONE',  ( -14.79501691930000007, 1474.161825565029858, 223.6789521170979924 ) ) ;
#61491=CARTESIAN_POINT ( 'NONE',  ( 0.9746356023110001043, 1408.913060387329779, 190.4091760167980283 ) ) ;
#61492=CARTESIAN_POINT ( 'NONE',  ( 2.769033333149520271, 1409.009757263489973, 230.2538554199990131 ) ) ;
#61493=CARTESIAN_POINT ( 'NONE',  ( 2.483039260530000014, 1508.999772102629777, 238.0619777341980239 ) ) ;
#61494=CARTESIAN_POINT ( 'NONE',  ( -4.174809892219999874, 1417.498982180929943, 233.1641891595979814 ) ) ;
#61497=CARTESIAN_POINT ( 'NONE',  ( -44.83505966559869904, 1432.107508427250195, 267.6405665847250361 ) ) ;
#61498=CARTESIAN_POINT ( 'NONE',  ( -3.598240451819999741, 1426.013882560829870, 186.0138310293980055 ) ) ;
#61499=VERTEX_POINT ( 'NONE', #14531 ) ;
#61502=VERTEX_POINT ( 'NONE', #40292 ) ;
#61507=CIRCLE ( 'NONE', #22121, 2.000000000000000000 ) ;
#61509=B_SPLINE_SURFACE_WITH_KNOTS ( 'NONE', 5, 5, ( 
 ( #50960, #42547, #43110, #94591, #17870, #44780, #89510, #104660, #97899 ),
 ( #88956, #96266, #20098, #12248, #72726, #29067, #46437, #55378, #80569 ),
 ( #105222, #45880, #79474, #21171, #72195, #38015, #105784, #27957, #30142 ),
 ( #54291, #3884, #80017, #2783, #54832, #3338, #81105, #70543, #20628 ),
 ( #12801, #46981, #106315, #87316, #62140, #36351, #78930, #37462, #63782 ),
 ( #11175, #4422, #19543, #63250, #97359, #38547, #106850, #29597, #36903 ) ),
 .UNSPECIFIED., .F., .F., .F.,
 ( 6, 6 ),
 ( 6, 3, 6 ),
 ( 18.71477090770000018, 31.31580451349999805 ),
 ( 0.000000000000000000, 1.000000000000000000, 2.000000000000000000 ),
 .UNSPECIFIED. ) ;
#61510=ORIENTED_EDGE ( 'NONE', *, *, #3542, .F. ) ;
#61513=CARTESIAN_POINT ( 'NONE',  ( 13.43268769770000048, 1434.818091166330078, 195.7542001346979816 ) ) ;
#61514=( BOUNDED_CURVE ( )  B_SPLINE_CURVE ( 3, ( #36227, #62008, #78223, #443 ),
 .UNSPECIFIED., .F., .F. ) 
 B_SPLINE_CURVE_WITH_KNOTS ( ( 4, 4 ),
 ( 3.450515127324310427, 4.712388980386121418 ),
 .UNSPECIFIED. ) 
 CURVE ( )  GEOMETRIC_REPRESENTATION_ITEM ( )  RATIONAL_B_SPLINE_CURVE ( ( 1.000000000000000000, 0.8716501122551647551, 0.8716501122551647551, 1.000000000000000000 ) ) 
 REPRESENTATION_ITEM ( '' )  );
#61520=CARTESIAN_POINT ( 'NONE',  ( -2.984254467278609990, 1410.459656091350098, 269.3356736250599965 ) ) ;
#61522=CARTESIAN_POINT ( 'NONE',  ( 12.44762265580000005, 1419.324415493729930, 229.2325656297979890 ) ) ;
#61525=ORIENTED_EDGE ( 'NONE', *, *, #12302, .F. ) ;
#61527=CARTESIAN_POINT ( 'NONE',  ( -15.56469051740000076, 1506.798305107229908, 193.1680121121979994 ) ) ;
#61528=CARTESIAN_POINT ( 'NONE',  ( -0.1587077902524139938, 1408.918602603690033, 186.0281839096400063 ) ) ;
#61529=CARTESIAN_POINT ( 'NONE',  ( -11.01799577076803338, 1438.323741232346265, 152.2811882100368450 ) ) ;
#61530=CARTESIAN_POINT ( 'NONE',  ( -0.02092469023549359958, 1409.011326956849871, 185.9381130483309903 ) ) ;
#61531=CARTESIAN_POINT ( 'NONE',  ( -18.89626061867770090, 1416.765224585220039, 207.5748551965540116 ) ) ;
#61532=CARTESIAN_POINT ( 'NONE',  ( -21.64080353419999980, 1425.805544261529803, 218.6154348525679723 ) ) ;
#61533=CARTESIAN_POINT ( 'NONE',  ( 33.01176666536340321, 1465.417536072469829, 268.6111601533029898 ) ) ;
#61534=CARTESIAN_POINT ( 'NONE',  ( -2.762021882724490229, 1466.850348183065080, 235.0881963227743654 ) ) ;
#61535=CARTESIAN_POINT ( 'NONE',  ( 10.97111050090000184, 1445.273638288909979, 185.1428967657980138 ) ) ;
#61539=CARTESIAN_POINT ( 'NONE',  ( 1.519281268484470093, 1457.051486531649971, 183.2989482105110142 ) ) ;
#61540=CARTESIAN_POINT ( 'NONE',  ( 23.23064387430000011, 1409.829316784929915, 208.7297343454509928 ) ) ;
#61542=LINE ( 'NONE', #10567, #7033 ) ;
#61543=CARTESIAN_POINT ( 'NONE',  ( 25.74098603697060028, 1450.968017009530058, 136.8501568074100021 ) ) ;
#61544=CARTESIAN_POINT ( 'NONE',  ( 14.45750869480000134, 1416.828040475729949, 196.8520545944980142 ) ) ;
#61547=CARTESIAN_POINT ( 'NONE',  ( 18.64060035870000220, 1410.060184558130004, 195.0159613159980267 ) ) ;
#61548=CARTESIAN_POINT ( 'NONE',  ( 17.11714625305219073, 1444.740067931810245, 162.7561045841208909 ) ) ;
#61549=CARTESIAN_POINT ( 'NONE',  ( 2.910924238241502149, 1439.670359696568312, 183.9847715977047073 ) ) ;
#61551=CARTESIAN_POINT ( 'NONE',  ( -18.59676279164743562, 1424.397502145024191, 224.8776118054202868 ) ) ;
#61552=CARTESIAN_POINT ( 'NONE',  ( 0.7034066635819330449, 1450.888494735919949, 181.3301578859269796 ) ) ;
#61560=CARTESIAN_POINT ( 'NONE',  ( 1234.711986934300057, 50.13405481578730161, -9668.243368257830298 ) ) ;
#61562=CARTESIAN_POINT ( 'NONE',  ( -0.2751659207381170202, 1506.798305148240161, 231.4088083080649767 ) ) ;
#61563=CARTESIAN_POINT ( 'NONE',  ( -3.444929438629999563, 1456.909266842430043, 224.8635561661979807 ) ) ;
#61564=CARTESIAN_POINT ( 'NONE',  ( 44.21391152859995088, 1449.831963904944814, 266.2303393994977796 ) ) ;
#61565=CARTESIAN_POINT ( 'NONE',  ( 11.68203264559999965, 1433.008677914059945, 150.9219369944979974 ) ) ;
#61566=CARTESIAN_POINT ( 'NONE',  ( 17.24149055319999846, 1446.934121893590145, 209.1218459616979999 ) ) ;
#61567=CARTESIAN_POINT ( 'NONE',  ( 27.13067724103490264, 1440.913060389899783, 227.4319135845050255 ) ) ;
#61570=B_SPLINE_CURVE_WITH_KNOTS ( 'NONE', 5,
 ( #78738, #2053, #36186, #18253, #86578, #27778, #9326, #35618, #94407, #70369, #11539, #19357, #61410, #18806, #62526, #17683, #79851, #69814, #10984, #103931, #10424 ),
 .UNSPECIFIED., .F., .F.,
 ( 6, 3, 3, 3, 3, 3, 6 ),
 ( 37.36625346989999485, 38.00991709350000036, 40.59642292560000243, 43.18292875779999918, 44.87875381330000124, 46.52360639289999966, 46.78685122110000094 ),
 .UNSPECIFIED. ) ;
#61571=CIRCLE ( 'NONE', #15005, 23.99999935407219454 ) ;
#61575=CARTESIAN_POINT ( 'NONE',  ( -7.580762144500440058, 1509.258003769659808, 239.0111317755749951 ) ) ;
#61576=CARTESIAN_POINT ( 'NONE',  ( 24.69009492180000009, 1430.360063174630113, 210.5561083012179893 ) ) ;
#61579=CARTESIAN_POINT ( 'NONE',  ( 25.91181804669769662, 1436.667520981494818, 136.9959711219258054 ) ) ;
#61584=CARTESIAN_POINT ( 'NONE',  ( 0.1663705600157490139, 1482.467207184779909, 181.9884040192069961 ) ) ;
#61586=ORIENTED_EDGE ( 'NONE', *, *, #74078, .F. ) ;
#61587=CARTESIAN_POINT ( 'NONE',  ( -0.9041356905230000240, 1416.839648764230105, 228.0296119439979918 ) ) ;
#61589=CARTESIAN_POINT ( 'NONE',  ( -20.47737311789999737, 1507.835268392529997, 189.6592733436979756 ) ) ;
#61590=CARTESIAN_POINT ( 'NONE',  ( -34.94829774809100087, 1451.625365366279766, 134.0999999983029909 ) ) ;
#61593=ORIENTED_EDGE ( 'NONE', *, *, #91091, .F. ) ;
#61596=CARTESIAN_POINT ( 'NONE',  ( -15.42960834800000036, 1414.913060387329779, 213.9579542055979857 ) ) ;
#61598=CARTESIAN_POINT ( 'NONE',  ( 23.42684948969804992, 1410.407670420856903, 207.9130917326585859 ) ) ;
#61601=CARTESIAN_POINT ( 'NONE',  ( 13.18296707766739928, 1409.373419738079974, 216.1545172977099867 ) ) ;
#61604=CARTESIAN_POINT ( 'NONE',  ( -17.62970124079999934, 1421.466017064829884, 191.9566022962980014 ) ) ;
#61606=EDGE_LOOP ( 'NONE', ( #18331, #29630, #79356, #27743 ) ) ;
#61611=ORIENTED_EDGE ( 'NONE', *, *, #63890, .T. ) ;
#61616=CARTESIAN_POINT ( 'NONE',  ( 29.83089294303868400, 1462.373024423122388, 269.4690121057988677 ) ) ;
#61618=CARTESIAN_POINT ( 'NONE',  ( -0.02816727408130000054, 1396.454734798629943, 221.5795905815979836 ) ) ;
#61621=CARTESIAN_POINT ( 'NONE',  ( -19.49005507420071481, 1486.272062043716232, 189.7901318363738596 ) ) ;
#61627=B_SPLINE_SURFACE_WITH_KNOTS ( 'NONE', 3, 5, ( 
 ( #84045, #5140, #41507, #109809, #67276, #101370 ),
 ( #24660, #58861, #13519, #47707, #25777, #59975 ),
 ( #42054, #102487, #95212, #33626, #43708, #52670 ),
 ( #103035, #86805, #17922, #10096, #70049, #64 ) ),
 .UNSPECIFIED., .F., .F., .F.,
 ( 4, 4 ),
 ( 6, 6 ),
 ( 5.479561955569999476, 5.505632801470000004 ),
 ( 0.000000000000000000, 1.000000000000000000 ),
 .UNSPECIFIED. ) ;
#61628=CARTESIAN_POINT ( 'NONE',  ( -15.85691707105240233, 1416.756521790129909, 226.9090633924639917 ) ) ;
#61629=DIRECTION ( 'NONE',  ( 3.828588921590000582E-16, 0.000000000000000000, 1.000000000000000000 ) ) ;
#61631=VERTEX_POINT ( 'NONE', #66078 ) ;
#61634=CARTESIAN_POINT ( 'NONE',  ( 20.04380005080000160, 1410.189663056929930, 264.7217086931980248 ) ) ;
#61635=EDGE_CURVE ( 'NONE', #84894, #109869, #56199, .T. ) ;
#61636=CARTESIAN_POINT ( 'NONE',  ( -26.53588231930000063, 1469.248395155229900, 208.5390332338009785 ) ) ;
#61637=CARTESIAN_POINT ( 'NONE',  ( -0.5349228561300000129, 1502.013778628930140, 181.0478107783980022 ) ) ;
#61638=CARTESIAN_POINT ( 'NONE',  ( 16.27481265766170182, 1409.481380943289878, 193.1811559459430043 ) ) ;
#61641=CARTESIAN_POINT ( 'NONE',  ( 8.991744574390811096, 1509.227061438039982, 181.2342617849590169 ) ) ;
#61642=CARTESIAN_POINT ( 'NONE',  ( -21.00608537249999941, 1420.811742010229864, 244.4374624675979817 ) ) ;
#61644=EDGE_CURVE ( 'NONE', #105869, #101745, #21335, .T. ) ;
#61645=CARTESIAN_POINT ( 'NONE',  ( 17.46643367109724210, 1460.003880594037355, 228.4215481240995302 ) ) ;
#61648=B_SPLINE_CURVE_WITH_KNOTS ( 'NONE', 3,
 ( #57020, #97882, #91145, #5489, #30688, #81629, #73817, #4405, #22813, #106834, #55915, #64319, #48617, #54813, #64875, #88940, #72180, #21157, #39648, #98982, #29582, #6041, #71645, #63767, #30127, #21711, #105765, #55362, #89495, #90034, #110703, #14971, #6593, #102292, #41846, #33994, #15518, #49715 ),
 .UNSPECIFIED., .F., .F.,
 ( 4, 2, 2, 2, 1, 1, 2, 2, 2, 2, 2, 1, 1, 2, 2, 2, 2, 1, 1, 2, 2, 4 ),
 ( 0.000000000000000000, 0.1250000000000867639, 0.1875000000001262046, 0.2187500000001459111, 0.2343750000001556810, 0.2421875000001605105, 0.2460937500001808276, 0.2500000000002011724, 0.3750000000002833844, 0.4375000000003333445, 0.4687500000002819966, 0.4843750000001906808, 0.4921875000001450506, 0.4960937500001328382, 0.5000000000001205702, 0.6249999999981388221, 0.6874999999972273290, 0.7187499999967783548, 0.7343749999965537567, 0.7421874999965470954, 0.7499999999965404340, 1.000000000000000000 ),
 .UNSPECIFIED. ) ;
#61649=CARTESIAN_POINT ( 'NONE',  ( 30.82338449939999947, 1451.380982548830161, 136.0366644220979992 ) ) ;
#61651=CARTESIAN_POINT ( 'NONE',  ( 12.55301046429960010, 1396.410217408039898, 207.1735117289620121 ) ) ;
#61653=CARTESIAN_POINT ( 'NONE',  ( -17.73420755029999896, 1458.087872027529784, 230.3493948207980395 ) ) ;
#61654=ORIENTED_EDGE ( 'NONE', *, *, #41943, .F. ) ;
#61655=ORIENTED_EDGE ( 'NONE', *, *, #25479, .F. ) ;
#61656=AXIS2_PLACEMENT_3D ( 'NONE', #103358, #60861, #26660 ) ;
#61657=CARTESIAN_POINT ( 'NONE',  ( -29.25822673101280103, 1509.934902468239898, 211.7095298021968688 ) ) ;
#61659=VERTEX_POINT ( 'NONE', #35204 ) ;
#61660=DIRECTION ( 'NONE',  ( -0.8771707016849432659, 0.03063147587993800616, 0.4792006602572261298 ) ) ;
#61663=CARTESIAN_POINT ( 'NONE',  ( 3.068292148159999111E-16, 1443.913060387330006, 150.8032249175980155 ) ) ;
#61665=CARTESIAN_POINT ( 'NONE',  ( 27.44625298708299965, 1509.338202929293629, 206.1591719864515539 ) ) ;
#61668=CARTESIAN_POINT ( 'NONE',  ( -7.105427357599999217E-15, 1405.913060387330006, 146.1721969590979882 ) ) ;
#61669=EDGE_CURVE ( 'NONE', #101516, #57941, #76230, .T. ) ;
#61670=CARTESIAN_POINT ( 'NONE',  ( 15.54069288670000049, 1507.627023022229878, 225.9574102441980017 ) ) ;
#61671=ORIENTED_EDGE ( 'NONE', *, *, #30125, .T. ) ;
#61675=CARTESIAN_POINT ( 'NONE',  ( 11.86432389000050058, 1432.211847865620030, 149.9809511090870160 ) ) ;
#61676=CARTESIAN_POINT ( 'NONE',  ( 12.90042423989156539, 1444.934230273330741, 186.7320187782142966 ) ) ;
#61678=CARTESIAN_POINT ( 'NONE',  ( -15.66042904120755530, 1506.491018782441415, 193.6263806956001758 ) ) ;
#61679=CARTESIAN_POINT ( 'NONE',  ( -13.32090919908733184, 1443.086052842848630, 169.4274452085711573 ) ) ;
#61680=CARTESIAN_POINT ( 'NONE',  ( 7.178613415919999241, 1509.106095133629879, 236.6937018893979996 ) ) ;
#61681=EDGE_CURVE ( 'NONE', #80762, #87917, #108233, .T. ) ;
#61683=CARTESIAN_POINT ( 'NONE',  ( -5.249809024070000163, 1423.060572135929988, 185.6431024777980099 ) ) ;
#61684=CARTESIAN_POINT ( 'NONE',  ( 1.476720148826540013, 1407.665894306529935, 270.1373298275569823 ) ) ;
#61690=CARTESIAN_POINT ( 'NONE',  ( 0.03018028484158630925, 1410.288634417731828, 233.2216252247569059 ) ) ;
#61692=CARTESIAN_POINT ( 'NONE',  ( 13.79590907669999922, 1416.844618642430078, 196.3342910144979783 ) ) ;
#61695=CARTESIAN_POINT ( 'NONE',  ( -3.910936927762319382, 1506.384142095322204, 187.5277711242953558 ) ) ;
#61696=EDGE_LOOP ( 'NONE', ( #32012, #95216, #110554, #93205 ) ) ;
#61697=CARTESIAN_POINT ( 'NONE',  ( 36.06124926539999365, 1440.913060387330006, 262.6648722463980334 ) ) ;
#61698=FACE_OUTER_BOUND ( 'NONE', #44771, .T. ) ;
#61704=ORIENTED_EDGE ( 'NONE', *, *, #86265, .T. ) ;
#61707=CARTESIAN_POINT ( 'NONE',  ( -1.538335019100957712, 1450.609501681909705, 154.2722877154876926 ) ) ;
#61710=CARTESIAN_POINT ( 'NONE',  ( -8.887191752339999695, 1441.011119473389954, 186.5506309111979704 ) ) ;
#61712=CARTESIAN_POINT ( 'NONE',  ( 14.31460734255390044, 1509.452787273769900, 235.1998026213640003 ) ) ;
#61713=CARTESIAN_POINT ( 'NONE',  ( 5.992819232552546005, 1414.913060387329779, 220.0916279853276762 ) ) ;
#61714=CARTESIAN_POINT ( 'NONE',  ( 11.97711953749976566, 1433.612589388432525, 149.8655202104944237 ) ) ;
#61715=CARTESIAN_POINT ( 'NONE',  ( 11.74455360470000187, 1415.078310370329973, 229.3304074566979978 ) ) ;
#61717=CARTESIAN_POINT ( 'NONE',  ( -16.16331440049999912, 1459.159538815530141, 229.6201761408979962 ) ) ;
#61719=CARTESIAN_POINT ( 'NONE',  ( 45.63714522919999439, 1438.938960590560100, 268.9747551788980218 ) ) ;
#61721=CARTESIAN_POINT ( 'NONE',  ( 22.15911651489999912, 1435.271885453649929, 140.1193622846980134 ) ) ;
#61722=CARTESIAN_POINT ( 'NONE',  ( 19.70550280570000012, 1469.160055952030007, 191.5645849787979955 ) ) ;
#61724=CARTESIAN_POINT ( 'NONE',  ( 20.13566257103952850, 1506.560172254411782, 218.2038963799658120 ) ) ;
#61726=CARTESIAN_POINT ( 'NONE',  ( -17.44898219039999887, 1420.862956884029927, 226.4473557759979769 ) ) ;
#61728=CARTESIAN_POINT ( 'NONE',  ( -41.49258008709740153, 1443.691026079749918, 136.5669671037899775 ) ) ;
#61729=CARTESIAN_POINT ( 'NONE',  ( -17.49859601832923417, 1506.366982239744175, 195.8448425805984527 ) ) ;
#61730=CARTESIAN_POINT ( 'NONE',  ( -18.00081235489999898, 1415.932617989529945, 205.2446752400179832 ) ) ;
#61731=CARTESIAN_POINT ( 'NONE',  ( -12.45220969719999893, 1442.685518086189859, 186.6444734887980132 ) ) ;
#61733=CARTESIAN_POINT ( 'NONE',  ( -28.12789902060000102, 1435.479491205339855, 135.2461919473980174 ) ) ;
#61736=CARTESIAN_POINT ( 'NONE',  ( -14.16617799454949989, 1409.407754223660049, 213.8599483261789942 ) ) ;
#61738=FACE_OUTER_BOUND ( 'NONE', #54845, .T. ) ;
#61739=CARTESIAN_POINT ( 'NONE',  ( -38.12305826662554864, 1442.831169986191071, 136.9078781414296486 ) ) ;
#61740=CARTESIAN_POINT ( 'NONE',  ( -44.90007994049999951, 1451.198737828930007, 268.2456369373979896 ) ) ;
#61741=CARTESIAN_POINT ( 'NONE',  ( -17.07205270619999737, 1501.040019927530011, 224.0489642073979724 ) ) ;
#61742=CARTESIAN_POINT ( 'NONE',  ( 0.1616573738338789867, 1420.153416094779914, 183.7945939761100078 ) ) ;
#61744=CARTESIAN_POINT ( 'NONE',  ( -26.64291118699999927, 1508.595174534829994, 214.1515268407479766 ) ) ;
#61747=CARTESIAN_POINT ( 'NONE',  ( 17.12821735161499959, 1423.039456014099869, 226.8410098145990048 ) ) ;
#61748=CARTESIAN_POINT ( 'NONE',  ( 20.85997183230000118, 1508.960091291929984, 227.7506528288980121 ) ) ;
#61749=LINE ( 'NONE', #62880, #295 ) ;
#61753=CARTESIAN_POINT ( 'NONE',  ( 1.420259601960000229, 1466.712985171129958, 235.0376566307980113 ) ) ;
#61756=ADVANCED_FACE ( 'NONE', ( #1627 ), #63210, .T. ) ;
#61758=CARTESIAN_POINT ( 'NONE',  ( 22.27261620720000224, 1409.690837284130112, 212.5637969276579895 ) ) ;
#61762=CARTESIAN_POINT ( 'NONE',  ( -14.45783243223209880, 1416.839692136300073, 221.3920770721769884 ) ) ;
#61763=CARTESIAN_POINT ( 'NONE',  ( -11.87502393780000176, 1433.007271555939951, 149.9804723930980117 ) ) ;
#61768=CARTESIAN_POINT ( 'NONE',  ( -24.91018336865660743, 1509.782943158774287, 193.9316171199673420 ) ) ;
#61771=B_SPLINE_CURVE_WITH_KNOTS ( 'NONE', 3,
 ( #63217, #82171, #5471, #20593 ),
 .UNSPECIFIED., .F., .F.,
 ( 4, 4 ),
 ( -36.72426899450000093, -23.80234877754210032 ),
 .UNSPECIFIED. ) ;
#61772=CARTESIAN_POINT ( 'NONE',  ( 1.058603163941309822, 1414.913060387330006, 192.7445404878875763 ) ) ;
#61774=CARTESIAN_POINT ( 'NONE',  ( -14.18548177819419998, 1485.573726300379803, 186.3991088774869809 ) ) ;
#61775=CARTESIAN_POINT ( 'NONE',  ( 1.932231105370000090, 1508.750808003230077, 237.3393916369980161 ) ) ;
#61777=CARTESIAN_POINT ( 'NONE',  ( 41.14071512850430423, 1444.183191039890062, 136.8991235379290003 ) ) ;
#61781=CARTESIAN_POINT ( 'NONE',  ( 11.16774673678820129, 1434.096752951460076, 151.6376635257900034 ) ) ;
#61783=ORIENTED_EDGE ( 'NONE', *, *, #83682, .F. ) ;
#61787=CARTESIAN_POINT ( 'NONE',  ( 1.547463840030000037, 1414.913060387329779, 192.3096136973980208 ) ) ;
#61788=CARTESIAN_POINT ( 'NONE',  ( 18.53418652026280000, 1507.620785850910124, 188.5293807599879869 ) ) ;
#61789=FACE_OUTER_BOUND ( 'NONE', #46328, .T. ) ;
#61790=FACE_OUTER_BOUND ( 'NONE', #93246, .T. ) ;
#61792=CARTESIAN_POINT ( 'NONE',  ( 1.100342456369999944, 1488.175276620729846, 181.8693589272980091 ) ) ;
#61794=CARTESIAN_POINT ( 'NONE',  ( 16.23184890680000336, 1409.981663893229779, 226.5335387243980279 ) ) ;
#61795=SURFACE_STYLE_FILL_AREA ( #28159 ) ;
#61797=CARTESIAN_POINT ( 'NONE',  ( -3.887243918150000104E-16, 1418.913060387330006, 172.2701767054979882 ) ) ;
#61801=ORIENTED_EDGE ( 'NONE', *, *, #53726, .T. ) ;
#61802=CARTESIAN_POINT ( 'NONE',  ( 13.65820430843470135, 1435.058683561780072, 149.3325756827849773 ) ) ;
#61804=ORIENTED_EDGE ( 'NONE', *, *, #14581, .F. ) ;
#61805=ORIENTED_EDGE ( 'NONE', *, *, #28761, .F. ) ;
#61807=CARTESIAN_POINT ( 'NONE',  ( 12.73783686771306378, 1445.004038133846052, 169.4561619195475544 ) ) ;
#61808=CARTESIAN_POINT ( 'NONE',  ( -1.063679678840000031, 1465.068952327929992, 237.9910134151979832 ) ) ;
#61809=CARTESIAN_POINT ( 'NONE',  ( 17.85438889637121918, 1451.055155745748152, 147.6149896967176289 ) ) ;
#61820=CARTESIAN_POINT ( 'NONE',  ( 26.83521609794189899, 1440.913060387330006, 244.5852667276629973 ) ) ;
#61821=CARTESIAN_POINT ( 'NONE',  ( -17.79309622859999962, 1508.782084903129999, 186.6536652249980079 ) ) ;
#61822=ORIENTED_EDGE ( 'NONE', *, *, #95986, .T. ) ;
#61823=CARTESIAN_POINT ( 'NONE',  ( 25.42631525001290171, 1450.800432264039955, 137.2067223160219953 ) ) ;
#61824=CARTESIAN_POINT ( 'NONE',  ( -14.94386443490000005, 1409.601552534729990, 191.3531982347979863 ) ) ;
#61826=B_SPLINE_CURVE_WITH_KNOTS ( 'NONE', 3,
 ( #60968, #64139, #95093, #18359, #44151, #98259, #78286, #1600, #35737, #104038 ),
 .UNSPECIFIED., .F., .F.,
 ( 4, 2, 2, 2, 4 ),
 ( 1.051150819890804081E-15, 0.0002615007907132596392, 0.0005230015814254681443, 0.0007845023721376766495, 0.001046003162849885263 ),
 .UNSPECIFIED. ) ;
#61827=CARTESIAN_POINT ( 'NONE',  ( -24.38909170209999999, 1441.406328540210097, 211.3558879569780231 ) ) ;
#61828=CARTESIAN_POINT ( 'NONE',  ( -10.79382126600000014, 1414.913060387329779, 196.1395803457980094 ) ) ;
#61830=CARTESIAN_POINT ( 'NONE',  ( -13.01246536547306398, 1434.785318802752727, 146.9694555298348462 ) ) ;
#61833=CARTESIAN_POINT ( 'NONE',  ( 22.68396052030000121, 1435.289475021379985, 139.2169948456979967 ) ) ;
#61834=CARTESIAN_POINT ( 'NONE',  ( 15.73551128017709466, 1409.462558017715537, 192.7683535211936317 ) ) ;
#61836=B_SPLINE_CURVE_WITH_KNOTS ( 'NONE', 5,
 ( #60101, #96449, #98633, #11892, #3515, #79112 ),
 .UNSPECIFIED., .F., .F.,
 ( 6, 6 ),
 ( -88.89713672530000110, -20.08879725519999226 ),
 .UNSPECIFIED. ) ;
#61838=ADVANCED_FACE ( 'NONE', ( #80531 ), #23267, .T. ) ;
#61839=DIRECTION ( 'NONE',  ( 0.000000000000000000, 0.000000000000000000, -1.000000000000000000 ) ) ;
#61848=DIRECTION ( 'NONE',  ( 0.03489949670250328678, -0.9993908270190956511, 0.000000000000000000 ) ) ;
#61849=CARTESIAN_POINT ( 'NONE',  ( 25.82475784490000237, 1456.303105448229871, 244.3435519335980075 ) ) ;
#61850=CARTESIAN_POINT ( 'NONE',  ( -18.63536074199999959, 1457.257477148429871, 229.6471845788980204 ) ) ;
#61852=CARTESIAN_POINT ( 'NONE',  ( -7.949591086192760336, 1509.190922234509799, 237.3729886602710053 ) ) ;
#61853=CARTESIAN_POINT ( 'NONE',  ( -21.13871847430000273, 1453.538022492230084, 224.2160773190980194 ) ) ;
#61855=CARTESIAN_POINT ( 'NONE',  ( 17.49213541791160154, 1409.748594249720099, 222.5804550065900287 ) ) ;
#61856=CARTESIAN_POINT ( 'NONE',  ( -0.08972462337150000078, 1506.809279316830043, 187.0844409784980371 ) ) ;
#61860=FACE_OUTER_BOUND ( 'NONE', #9929, .T. ) ;
#61863=CIRCLE ( 'NONE', #60089, 29.84605316702132072 ) ;
#61864=CARTESIAN_POINT ( 'NONE',  ( 37.91363576014470027, 1455.431640273400035, 269.5661993588879568 ) ) ;
#61865=CARTESIAN_POINT ( 'NONE',  ( 2.478856071480000089, 1433.873643567909994, 157.5618534805980175 ) ) ;
#61866=( BOUNDED_CURVE ( )  B_SPLINE_CURVE ( 3, ( #57467, #31127, #22149, #56350 ),
 .UNSPECIFIED., .F., .T. ) 
 B_SPLINE_CURVE_WITH_KNOTS ( ( 4, 4 ),
 ( 4.993841937945130205, 5.632217541602730471 ),
 .UNSPECIFIED. ) 
 CURVE ( )  GEOMETRIC_REPRESENTATION_ITEM ( )  RATIONAL_B_SPLINE_CURVE ( ( 1.000000000000000000, 0.9663270635670118125, 0.9663270635670118125, 1.000000000000000000 ) ) 
 REPRESENTATION_ITEM ( '' )  );
#61867=FACE_OUTER_BOUND ( 'NONE', #37942, .T. ) ;
#61868=CARTESIAN_POINT ( 'NONE',  ( -45.00576737213309997, 1440.913060397780100, 265.4746514701479896 ) ) ;
#61869=CARTESIAN_POINT ( 'NONE',  ( -26.72647157590000333, 1447.183840207770118, 137.1854294550980171 ) ) ;
#61870=CARTESIAN_POINT ( 'NONE',  ( 1.842704255619313169, 1450.383521515580469, 154.3038121965128653 ) ) ;
#61874=CARTESIAN_POINT ( 'NONE',  ( 17.53454537772509880, 1416.240002716455592, 192.2859374383096167 ) ) ;
#61875=CIRCLE ( 'NONE', #42176, 2.000006063936102141 ) ;
#61876=ORIENTED_EDGE ( 'NONE', *, *, #109015, .F. ) ;
#61877=CARTESIAN_POINT ( 'NONE',  ( 3.686666017499999892, 1448.977420087960127, 184.1966211689980071 ) ) ;
#61881=CARTESIAN_POINT ( 'NONE',  ( -0.3391533370919999624, 1475.982599279930128, 267.2349199512980249 ) ) ;
#61887=CARTESIAN_POINT ( 'NONE',  ( -18.89315557560000158, 1416.535385209229844, 208.2130245880870234 ) ) ;
#61888=CARTESIAN_POINT ( 'NONE',  ( -4.500000000000000000, 1439.615672362369878, 183.5288080717980108 ) ) ;
#61890=CARTESIAN_POINT ( 'NONE',  ( -10.55660206177969940, 1396.281705055399925, 205.8010626438610018 ) ) ;
#61892=CARTESIAN_POINT ( 'NONE',  ( -16.09626466356160179, 1409.475145151020115, 225.1332147237440040 ) ) ;
#61893=CARTESIAN_POINT ( 'NONE',  ( 11.97724519069999971, 1441.600846913620217, 147.6096801420980000 ) ) ;
#61895=CARTESIAN_POINT ( 'NONE',  ( -20.59664500270120158, 1507.763472350329948, 190.3621299389660066 ) ) ;
#61898=CARTESIAN_POINT ( 'NONE',  ( 9.958422982289999226, 1425.240937812430047, 91.92796437169779722 ) ) ;
#61900=CARTESIAN_POINT ( 'NONE',  ( 0.4156708952280039338, 1507.115992466239732, 180.9569215093680157 ) ) ;
#61901=ADVANCED_FACE ( 'NONE', ( #32854 ), #34519, .F. ) ;
#61902=CARTESIAN_POINT ( 'NONE',  ( -13.51610093808349333, 1442.913060377700731, 151.4871142704430440 ) ) ;
#61908=CARTESIAN_POINT ( 'NONE',  ( 3.895672787440000118, 1449.598608009080181, 184.2305619520979860 ) ) ;
#61910=CARTESIAN_POINT ( 'NONE',  ( -7.139643295716398441, 1463.933016821221599, 236.1633024888363934 ) ) ;
#61912=ORIENTED_EDGE ( 'NONE', *, *, #83503, .T. ) ;
#61914=CARTESIAN_POINT ( 'NONE',  ( -41.49212309149999811, 1443.779876761469950, 136.5764441233980051 ) ) ;
#61916=CARTESIAN_POINT ( 'NONE',  ( -14.82206140629999958, 1409.430658177129999, 192.2978730262979923 ) ) ;
#61917=CARTESIAN_POINT ( 'NONE',  ( -3.081957766449999969, 1471.965628206130077, 270.0718125651980017 ) ) ;
#61919=CARTESIAN_POINT ( 'NONE',  ( 0.1523726883269999888, 1486.225463480429880, 181.8688073209980018 ) ) ;
#61923=CARTESIAN_POINT ( 'NONE',  ( -35.92258139975950115, 1450.175254039669881, 136.2201275893520176 ) ) ;
#61924=CARTESIAN_POINT ( 'NONE',  ( -2.500000000000059952, 1448.813856349769821, 156.5098158667020130 ) ) ;
#61925=CARTESIAN_POINT ( 'NONE',  ( 5.795460316590049565, 1396.115442321129876, 218.5178396626099868 ) ) ;
#61926=CARTESIAN_POINT ( 'NONE',  ( 3.536371054309000339, 1409.036553185790126, 194.1218458967759943 ) ) ;
#61927=CARTESIAN_POINT ( 'NONE',  ( -1.507529438030280167, 1406.789552898120064, 269.6496621541520540 ) ) ;
#61928=ADVANCED_FACE ( 'NONE', ( #17127 ), #57547, .F. ) ;
#61929=CARTESIAN_POINT ( 'NONE',  ( -14.45919768630980151, 1435.871793938970086, 149.8088992138540050 ) ) ;
#61930=ORIENTED_EDGE ( 'NONE', *, *, #19397, .F. ) ;
#61932=CARTESIAN_POINT ( 'NONE',  ( 12.51650399660000090, 1442.246764597770152, 188.0677751049979918 ) ) ;
#61934=ORIENTED_EDGE ( 'NONE', *, *, #1613, .F. ) ;
#61935=EDGE_CURVE ( 'NONE', #11723, #35481, #36619, .T. ) ;
#61940=EDGE_CURVE ( 'NONE', #60010, #23487, #22723, .T. ) ;
#61942=ORIENTED_EDGE ( 'NONE', *, *, #86062, .F. ) ;
#61947=B_SPLINE_CURVE_WITH_KNOTS ( 'NONE', 4,
 ( #101698, #24989, #65392, #56985, #99497, #7658, #40163, #7116, #22779 ),
 .UNSPECIFIED., .F., .F.,
 ( 5, 4, 5 ),
 ( 0.000000000000000000, 0.9999685429682046989, 1.000000000000000000 ),
 .UNSPECIFIED. ) ;
#61948=CARTESIAN_POINT ( 'NONE',  ( -28.02005516190000023, 1440.913060387330006, 248.0989693021979861 ) ) ;
#61951=CARTESIAN_POINT ( 'NONE',  ( -5.824582710369999639, 1409.283474491729976, 230.9652227488979861 ) ) ;
#61952=CARTESIAN_POINT ( 'NONE',  ( -1.655764672069989230, 1452.024870244869135, 184.0828371579059137 ) ) ;
#61956=CARTESIAN_POINT ( 'NONE',  ( -25.37446848917170072, 1440.913060497199922, 218.3462857971420021 ) ) ;
#61959=CARTESIAN_POINT ( 'NONE',  ( -25.17810084989999808, 1436.605446963749955, 137.6240872485979878 ) ) ;
#61963=CARTESIAN_POINT ( 'NONE',  ( 0.01162473798205385794, 1508.119767624307997, 237.6719974036047347 ) ) ;
#61967=ORIENTED_EDGE ( 'NONE', *, *, #64427, .T. ) ;
#61969=CARTESIAN_POINT ( 'NONE',  ( -13.88578263259999979, 1410.294695765230017, 227.0726749396980040 ) ) ;
#61972=DIRECTION ( 'NONE',  ( 0.7382608262429739554, 0.6622882068469760908, -0.1278486742459950254 ) ) ;
#61974=CARTESIAN_POINT ( 'NONE',  ( 16.80235653624059822, 1469.007454033449903, 229.3029007443279852 ) ) ;
#61975=CARTESIAN_POINT ( 'NONE',  ( -24.02854486914899823, 1507.902871221900114, 222.3115732752750091 ) ) ;
#61978=CARTESIAN_POINT ( 'NONE',  ( 0.1132867808292180034, 1420.456998724389905, 182.7041194852360206 ) ) ;
#61980=CARTESIAN_POINT ( 'NONE',  ( -3.540703860449999851, 1421.447957905329986, 185.5466525330979835 ) ) ;
#61984=CARTESIAN_POINT ( 'NONE',  ( -11.16128041099520019, 1414.913057846380070, 196.7202417048659981 ) ) ;
#61988=CARTESIAN_POINT ( 'NONE',  ( 2.046266125239999845, 1417.477797419130184, 235.2693601201980016 ) ) ;
#61989=CARTESIAN_POINT ( 'NONE',  ( 9.152846453431976670, 1436.773426841208902, 153.0359782892105329 ) ) ;
#61993=CARTESIAN_POINT ( 'NONE',  ( -3.171072485709999889, 1451.871858332230204, 182.7750508701979868 ) ) ;
#61994=CARTESIAN_POINT ( 'NONE',  ( 18.47106347599999765, 1415.579607678529783, 210.5150304694180079 ) ) ;
#61995=CARTESIAN_POINT ( 'NONE',  ( -18.26759032049999831, 1425.063529675129985, 226.1973866133980096 ) ) ;
#61996=CARTESIAN_POINT ( 'NONE',  ( -22.66323514130000305, 1435.715412731579818, 141.6350653710979941 ) ) ;
#61998=CARTESIAN_POINT ( 'NONE',  ( 0.4536707880366389611, 1408.928902979399936, 232.1183505920600112 ) ) ;
#62002=CARTESIAN_POINT ( 'NONE',  ( 1.555417156611949903, 1415.301705643749983, 191.0707738022140063 ) ) ;
#62004=CARTESIAN_POINT ( 'NONE',  ( -24.07234762469999723, 1436.256975754479981, 211.0558319517779751 ) ) ;
#62007=CARTESIAN_POINT ( 'NONE',  ( -3.498438759191051073, 1426.007621855026855, 185.8749847655367091 ) ) ;
#62008=CARTESIAN_POINT ( 'NONE',  ( -19.57175081134495187, 1452.229599788696760, 144.4156370990241669 ) ) ;
#62017=CARTESIAN_POINT ( 'NONE',  ( 25.78167512749999801, 1509.813387183829946, 195.1140785605980170 ) ) ;
#62021=CARTESIAN_POINT ( 'NONE',  ( 19.91241810695860082, 1508.791614727160095, 229.5527701831059915 ) ) ;
#62025=B_SPLINE_CURVE_WITH_KNOTS ( 'NONE', 5,
 ( #88331, #11624, #31714, #75402, #48545, #100017, #100570, #23851, #15451 ),
 .UNSPECIFIED., .F., .F.,
 ( 6, 3, 6 ),
 ( 0.000000000000000000, 0.5459884364902550802, 1.000000000000000000 ),
 .UNSPECIFIED. ) ;
#62026=CARTESIAN_POINT ( 'NONE',  ( 18.03151512659999867, 1424.669534113930013, 225.2917716953979834 ) ) ;
#62028=CARTESIAN_POINT ( 'NONE',  ( 18.95069757339999938, 1434.818091166489921, 209.1678375094830074 ) ) ;
#62029=CARTESIAN_POINT ( 'NONE',  ( -14.25478685789999922, 1474.931945797630078, 267.1909358522980256 ) ) ;
#62031=CARTESIAN_POINT ( 'NONE',  ( -11.13407163250000131, 1433.980143678790000, 151.6624242815980210 ) ) ;
#62032=CARTESIAN_POINT ( 'NONE',  ( 24.02854436560000195, 1507.902905841229767, 195.9321017799980211 ) ) ;
#62034=CARTESIAN_POINT ( 'NONE',  ( 6.015966285260000213, 1410.497582365630024, 186.7561560874980273 ) ) ;
#62035=CARTESIAN_POINT ( 'NONE',  ( 5.243795696529999439, 1423.891122896129900, 185.6630549162979946 ) ) ;
#62036=CARTESIAN_POINT ( 'NONE',  ( -10.37614202680000020, 1435.190620644159935, 152.2457775527979891 ) ) ;
#62037=CARTESIAN_POINT ( 'NONE',  ( 8.766760964599999539, 1437.289887157169915, 153.2969297041979928 ) ) ;
#62041=ORIENTED_EDGE ( 'NONE', *, *, #22062, .T. ) ;
#62042=CARTESIAN_POINT ( 'NONE',  ( 1.861700016370000164E-09, 1407.650947845630071, 270.1377426662980383 ) ) ;
#62044=CARTESIAN_POINT ( 'NONE',  ( -42.86216812819999689, 1450.287397759410169, 270.1125555652979529 ) ) ;
#62046=CARTESIAN_POINT ( 'NONE',  ( 6.620521211799999861, 1440.451554611820029, 154.8188655977980090 ) ) ;
#62048=EDGE_CURVE ( 'NONE', #80209, #51888, #53558, .T. ) ;
#62050=EDGE_CURVE ( 'NONE', #65298, #51033, #69250, .T. ) ;
#62051=CARTESIAN_POINT ( 'NONE',  ( 2.927258396572999910, 1410.119448063770278, 231.5909967517320069 ) ) ;
#62052=CARTESIAN_POINT ( 'NONE',  ( 1.862958190160000083, 1508.877376266829970, 238.0546627234980122 ) ) ;
#62053=CARTESIAN_POINT ( 'NONE',  ( -7.934490975959999304, 1418.851980705729829, 233.0693007919979891 ) ) ;
#62056=CARTESIAN_POINT ( 'NONE',  ( -43.43515788656559806, 1430.093275174819837, 266.2527815779079674 ) ) ;
#62057=CARTESIAN_POINT ( 'NONE',  ( -2.500000000000000000, 1428.666845053830002, 184.0221679455979995 ) ) ;
#62059=CARTESIAN_POINT ( 'NONE',  ( 26.41103520988268016, 1435.419834908374014, 135.2945580757277639 ) ) ;
#62062=DIRECTION ( 'NONE',  ( -1.000000000000000000, 0.000000000000000000, 0.000000000000000000 ) ) ;
#62063=CARTESIAN_POINT ( 'NONE',  ( 17.60627508980000044, 1410.895669370830092, 224.8086596393980017 ) ) ;
#62064=CARTESIAN_POINT ( 'NONE',  ( -14.07411318249999965, 1410.402452814530079, 190.2626066483979912 ) ) ;
#62065=CIRCLE ( 'NONE', #92380, 2.000000000000072387 ) ;
#62069=CARTESIAN_POINT ( 'NONE',  ( -14.47990272989999916, 1470.812340170329890, 194.5754142818979915 ) ) ;
#62070=CARTESIAN_POINT ( 'NONE',  ( 0.3483522942510000053, 1452.334144580529937, 183.2984807459980061 ) ) ;
#62076=ORIENTED_EDGE ( 'NONE', *, *, #40652, .T. ) ;
#62077=CARTESIAN_POINT ( 'NONE',  ( -8.584304488529250321, 1409.159098409799981, 270.4209911071269516 ) ) ;
#62079=CARTESIAN_POINT ( 'NONE',  ( -1.525139958810000085, 1427.692446166030095, 112.4493539157979995 ) ) ;
#62084=CARTESIAN_POINT ( 'NONE',  ( 44.97774548475524625, 1446.717870710880106, 268.9931714851094284 ) ) ;
#62086=CARTESIAN_POINT ( 'NONE',  ( 3.632694880006927640, 1424.801563358291560, 184.7977647149654956 ) ) ;
#62087=CARTESIAN_POINT ( 'NONE',  ( -0.01853033842224269950, 1408.987905777800052, 186.0079448517529954 ) ) ;
#62089=EDGE_CURVE ( 'NONE', #27091, #60488, #49102, .T. ) ;
#62090=CARTESIAN_POINT ( 'NONE',  ( -18.43253908699789889, 1415.651572961160127, 207.5692543878770095 ) ) ;
#62091=CARTESIAN_POINT ( 'NONE',  ( -17.50642310480000319, 1415.863568519329874, 225.9737455361980096 ) ) ;
#62092=CARTESIAN_POINT ( 'NONE',  ( 22.25458370657720053, 1471.079518017990040, 269.4963396272059981 ) ) ;
#62093=CARTESIAN_POINT ( 'NONE',  ( -4.778891795048164859, 1466.453819146259320, 234.5096049691970848 ) ) ;
#62094=CARTESIAN_POINT ( 'NONE',  ( 5.861641773170000569, 1445.997555159400008, 183.2089869270980103 ) ) ;
#62096=EDGE_CURVE ( 'NONE', #10122, #92390, #9753, .T. ) ;
#62097=VERTEX_POINT ( 'NONE', #52449 ) ;
#62098=CARTESIAN_POINT ( 'NONE',  ( 23.33541660002344287, 1411.088284388518787, 212.4521946157103116 ) ) ;
#62099=CARTESIAN_POINT ( 'NONE',  ( 1.508487166569379978, 1461.824335589909879, 183.0899350828030094 ) ) ;
#62102=CARTESIAN_POINT ( 'NONE',  ( 25.61519007770650092, 1452.018576294739887, 135.1698835824450100 ) ) ;
#62103=CARTESIAN_POINT ( 'NONE',  ( -22.74352257909999864, 1409.874439094229956, 210.5210124972680035 ) ) ;
#62105=CARTESIAN_POINT ( 'NONE',  ( -18.70459388414779767, 1509.566239243649989, 231.7064163625079800 ) ) ;
#62106=CARTESIAN_POINT ( 'NONE',  ( 16.87335319769999842, 1409.502290865030091, 193.5015210144979960 ) ) ;
#62108=CARTESIAN_POINT ( 'NONE',  ( 16.63506069319999980, 1409.493969507229849, 224.8086549762979871 ) ) ;
#62109=CARTESIAN_POINT ( 'NONE',  ( 0.7618663611100000566, 1416.510331848630130, 233.5782494407980039 ) ) ;
#62110=CARTESIAN_POINT ( 'NONE',  ( -18.86156570322403780, 1424.747429002025456, 224.4550601468019977 ) ) ;
#62111=CARTESIAN_POINT ( 'NONE',  ( 0.3569283261391170137, 1452.331401915339939, 183.2344466057309944 ) ) ;
#62112=CIRCLE ( 'NONE', #26330, 30.65926195008838562 ) ;
#62119=CARTESIAN_POINT ( 'NONE',  ( -0.5052195027655379533, 1409.815383004930027, 233.0624941665790004 ) ) ;
#62120=CARTESIAN_POINT ( 'NONE',  ( 8535.261851439174279, 2833.596074015790236, 11230.49242346789651 ) ) ;
#62121=CARTESIAN_POINT ( 'NONE',  ( -39.75209972814790405, 1446.403744002959911, 136.7362441017349965 ) ) ;
#62123=CARTESIAN_POINT ( 'NONE',  ( -23.42675388609999843, 1443.575607731430182, 234.3916895697979612 ) ) ;
#62124=FACE_OUTER_BOUND ( 'NONE', #107846, .T. ) ;
#62125=CARTESIAN_POINT ( 'NONE',  ( 11.85885706300000031, 1433.132861810290024, 150.3130965059980042 ) ) ;
#62127=CARTESIAN_POINT ( 'NONE',  ( 27.24318804543259986, 1440.913060389329758, 227.9385435188879683 ) ) ;
#62130=ORIENTED_EDGE ( 'NONE', *, *, #68063, .T. ) ;
#62131=B_SPLINE_CURVE_WITH_KNOTS ( 'NONE', 3,
 ( #76850, #68463, #15793, #24213, #103124, #43251, #58400, #84129, #101464, #92524, #9624, #16353, #49994, #51100 ),
 .UNSPECIFIED., .F., .F.,
 ( 4, 2, 2, 1, 2, 2, 1, 4 ),
 ( 0.000000000000000000, 0.3416613661786893630, 0.4270767077233605380, 0.4697843784956968749, 0.4911382138818642384, 0.5018151315749493913, 0.5124920492680344886, 0.6833227323573606293 ),
 .UNSPECIFIED. ) ;
#62135=CARTESIAN_POINT ( 'NONE',  ( -13.52118962660000001, 1485.980279578529917, 185.5139189508979882 ) ) ;
#62137=CARTESIAN_POINT ( 'NONE',  ( 2.139180587729999861, 1474.716718025229966, 234.7298911498980090 ) ) ;
#62138=CARTESIAN_POINT ( 'NONE',  ( 25.05872055529999898, 1449.799157988799834, 212.4667254601980062 ) ) ;
#62140=CARTESIAN_POINT ( 'NONE',  ( -15.66010638180000214, 1508.960088055129972, 231.8745902587980083 ) ) ;
#62144=CARTESIAN_POINT ( 'NONE',  ( -25.11187825681734509, 1509.789986500208670, 193.4229894714747218 ) ) ;
#62145=CARTESIAN_POINT ( 'NONE',  ( 0.1608976399961470072, 1485.726857135249929, 181.8483459938640010 ) ) ;
#62147=ORIENTED_EDGE ( 'NONE', *, *, #95973, .T. ) ;
#62148=CARTESIAN_POINT ( 'NONE',  ( -1.342027840399999894, 1416.827520120730014, 228.0802440864979985 ) ) ;
#62156=CARTESIAN_POINT ( 'NONE',  ( -16.96258621739999839, 1415.088016306429836, 209.3926059833199815 ) ) ;
#62157=CARTESIAN_POINT ( 'NONE',  ( -2.706144844479429157, 1509.031773379787637, 238.5943737788366548 ) ) ;
#62158=CARTESIAN_POINT ( 'NONE',  ( 18.61829529775840086, 1507.564341563429934, 227.6679763394169811 ) ) ;
#62162=CARTESIAN_POINT ( 'NONE',  ( 8.995981003084148497, 1409.227206965499818, 221.0723839244040221 ) ) ;
#62163=CARTESIAN_POINT ( 'NONE',  ( 18.29112916889999951, 1425.477396046229842, 224.8880732489979835 ) ) ;
#62165=CARTESIAN_POINT ( 'NONE',  ( -17.10576414770000042, 1413.991245370330034, 191.8646404599980144 ) ) ;
#62171=ORIENTED_EDGE ( 'NONE', *, *, #27647, .F. ) ;
#62173=CARTESIAN_POINT ( 'NONE',  ( -12.18885905889360011, 1416.259629948840029, 194.7430301466939966 ) ) ;
#62175=CARTESIAN_POINT ( 'NONE',  ( -11.93399382900000028, 1433.811405297789861, 150.6808762289980166 ) ) ;
#62176=CARTESIAN_POINT ( 'NONE',  ( 17.58886893820438857, 1468.615884927995467, 269.3766193917544456 ) ) ;
#62178=CARTESIAN_POINT ( 'NONE',  ( 1.113913563919999961, 1395.951959106130062, 220.1286928646979959 ) ) ;
#62179=CARTESIAN_POINT ( 'NONE',  ( 22.39107469191120359, 1501.813592075909810, 209.7187615008220121 ) ) ;
#62181=CARTESIAN_POINT ( 'NONE',  ( -0.8956140690670000293, 1476.679333595129947, 182.3599195072980024 ) ) ;
#62183=CARTESIAN_POINT ( 'NONE',  ( -25.89297068493667808, 1436.665709121180498, 137.0068548018288084 ) ) ;
#62186=CARTESIAN_POINT ( 'NONE',  ( -12.94285051013109999, 1434.751085630199896, 149.1919155958750025 ) ) ;
#62190=CARTESIAN_POINT ( 'NONE',  ( 41.60066495211719939, 1444.057103930600078, 136.0676697147460175 ) ) ;
#62192=EDGE_CURVE ( 'NONE', #33885, #104546, #61570, .T. ) ;
#62193=CARTESIAN_POINT ( 'NONE',  ( 45.31148016700000625, 1435.337548181589909, 266.2043215618979843 ) ) ;
#62194=CARTESIAN_POINT ( 'NONE',  ( -26.05067190950000011, 1469.243640235329849, 206.2660147011979745 ) ) ;
#62195=CARTESIAN_POINT ( 'NONE',  ( -11.06188711399999924, 1426.914830454830053, 95.14035786269791117 ) ) ;
#62196=CARTESIAN_POINT ( 'NONE',  ( -1.278194139027049925, 1507.616839994659813, 232.0618046316060088 ) ) ;
#62198=CARTESIAN_POINT ( 'NONE',  ( -21.35837619870000026, 1471.309462467329922, 208.0048516116980295 ) ) ;
#62199=CARTESIAN_POINT ( 'NONE',  ( -33.93598214789999901, 1424.339496380530136, 259.3467867270979923 ) ) ;
#62201=CARTESIAN_POINT ( 'NONE',  ( 28.91692647261170279, 1509.557647286829933, 209.5387477244159982 ) ) ;
#62202=EDGE_CURVE ( 'NONE', #44739, #102101, #11791, .T. ) ;
#62204=CARTESIAN_POINT ( 'NONE',  ( 33.92643312500000263, 1450.868062273570104, 136.1711485282980050 ) ) ;
#62205=ORIENTED_EDGE ( 'NONE', *, *, #99420, .F. ) ;
#62206=CARTESIAN_POINT ( 'NONE',  ( -2.500000000000000000, 1432.353968296120001, 157.4944290049979827 ) ) ;
#62208=CARTESIAN_POINT ( 'NONE',  ( -18.01357308700000104, 1458.773660595129968, 228.0936931546980020 ) ) ;
#62215=CARTESIAN_POINT ( 'NONE',  ( -0.2626479354700000379, 1424.305209145230037, 227.7945639678980285 ) ) ;
#62216=CARTESIAN_POINT ( 'NONE',  ( 7.837683663321347360, 1446.693895632879048, 154.0817846991284910 ) ) ;
#62219=CARTESIAN_POINT ( 'NONE',  ( -3.883780448710000055, 1489.060101785230017, 235.7933154220980043 ) ) ;
#62222=CARTESIAN_POINT ( 'NONE',  ( 45.63098875785350117, 1442.771072822339875, 266.1895104264430074 ) ) ;
#62224=CARTESIAN_POINT ( 'NONE',  ( 0.05774186599319999780, 1420.439312890830251, 183.3105440342980046 ) ) ;
#62228=ORIENTED_EDGE ( 'NONE', *, *, #62414, .F. ) ;
#62229=CARTESIAN_POINT ( 'NONE',  ( 11.85801740980349983, 1431.772258989899910, 149.9533191514260011 ) ) ;
#62232=CARTESIAN_POINT ( 'NONE',  ( 6.325886374943740620, 1422.669378755508660, 139.1419511335710695 ) ) ;
#62233=CARTESIAN_POINT ( 'NONE',  ( -13.51812398686054451, 1443.501467202828962, 169.4008117781592375 ) ) ;
#62234=CARTESIAN_POINT ( 'NONE',  ( 5.043681905660000631, 1508.915672638330079, 236.8001211188980051 ) ) ;
#62236=CARTESIAN_POINT ( 'NONE',  ( 16.50977420799199891, 1452.336526367869965, 146.7133680455360150 ) ) ;
#62237=CARTESIAN_POINT ( 'NONE',  ( 3.182038384110000173, 1408.010183206830106, 270.2907995557980598 ) ) ;
#62242=CARTESIAN_POINT ( 'NONE',  ( 0.02672782265863862458, 1410.277270240254211, 233.2211595074259378 ) ) ;
#62250=CARTESIAN_POINT ( 'NONE',  ( 23.42675388609999843, 1440.913060387330006, 234.3916895593979746 ) ) ;
#62251=CARTESIAN_POINT ( 'NONE',  ( -8.301987938657498844, 1512.913060387330006, 185.0111222839169898 ) ) ;
#62253=CARTESIAN_POINT ( 'NONE',  ( -13.51610093809999924, 1443.913060387330006, 169.3501091259980171 ) ) ;
#62255=DIRECTION ( 'NONE',  ( 0.9076935351921801010, 0.1286034085550979977, -0.3994416221155894786 ) ) ;
#62257=EDGE_LOOP ( 'NONE', ( #87349, #64348, #100436, #108438 ) ) ;
#62259=CARTESIAN_POINT ( 'NONE',  ( -24.15795475150000016, 1443.642594450309844, 212.0312900464880101 ) ) ;
#62260=CARTESIAN_POINT ( 'NONE',  ( -0.5717982397045180409, 1450.893092752919983, 154.2461502927169761 ) ) ;
#62263=CARTESIAN_POINT ( 'NONE',  ( 5.360823395318768725, 1422.262019483632912, 143.3077198672117163 ) ) ;
#62264=CARTESIAN_POINT ( 'NONE',  ( 30.10957446088429990, 1509.964507489280095, 213.6424367098229880 ) ) ;
#62266=CARTESIAN_POINT ( 'NONE',  ( -13.91344329490000042, 1453.313060387329870, 223.0352892571980021 ) ) ;
#62267=CARTESIAN_POINT ( 'NONE',  ( 9.365061209729999447, 1417.415607571329929, 230.4107670011979678 ) ) ;
#62270=CARTESIAN_POINT ( 'NONE',  ( -16.27761471759999878, 1460.158989628929930, 228.4983889328979956 ) ) ;
#62272=CARTESIAN_POINT ( 'NONE',  ( 45.59816521089999952, 1434.873519021199854, 266.9907516340980465 ) ) ;
#62273=CARTESIAN_POINT ( 'NONE',  ( 38.49765372689370224, 1444.525112227430100, 137.1053225086949681 ) ) ;
#62274=CARTESIAN_POINT ( 'NONE',  ( 18.99827228379999866, 1436.394236938839867, 146.4527104209979882 ) ) ;
#62275=CARTESIAN_POINT ( 'NONE',  ( 19.30811431869999950, 1488.591121188929947, 189.5534381757979929 ) ) ;
#62276=CARTESIAN_POINT ( 'NONE',  ( 29.75998665772953444, 1509.996183727615517, 208.5887809057482798 ) ) ;
#62278=CARTESIAN_POINT ( 'NONE',  ( 12.26996142119999966, 1416.831925149330118, 223.5794496915980005 ) ) ;
#62279=EDGE_CURVE ( 'NONE', #102287, #104433, #36063, .T. ) ;
#62281=CARTESIAN_POINT ( 'NONE',  ( -38.57261905365100318, 1437.400638483769853, 135.9606806742719982 ) ) ;
#62282=CARTESIAN_POINT ( 'NONE',  ( -8.524719538440001187, 1409.210750153330082, 197.0779234733980161 ) ) ;
#62283=CARTESIAN_POINT ( 'NONE',  ( -17.17379625170000423, 1415.087974639930053, 205.5614638525080125 ) ) ;
#62284=CARTESIAN_POINT ( 'NONE',  ( -12.76843643930000027, 1441.647446156619935, 188.0548363060980250 ) ) ;
#62285=EDGE_CURVE ( 'NONE', #35225, #88507, #21462, .T. ) ;
#62287=EDGE_CURVE ( 'NONE', #47969, #31004, #56271, .T. ) ;
#62288=CARTESIAN_POINT ( 'NONE',  ( -33.54530754720000374, 1436.144128905479874, 136.3106138590979981 ) ) ;
#62292=CARTESIAN_POINT ( 'NONE',  ( 28.02579834570000017, 1443.109842421789835, 137.4877371059980078 ) ) ;
#62293=AXIS2_PLACEMENT_3D ( 'NONE', #41852, #100641, #102298 ) ;
#62295=CARTESIAN_POINT ( 'NONE',  ( -33.79457713422360854, 1443.086052842850677, 154.8159889477085756 ) ) ;
#62296=CARTESIAN_POINT ( 'NONE',  ( -44.39744386319999592, 1450.996159658330043, 269.0084819576979953 ) ) ;
#62297=CARTESIAN_POINT ( 'NONE',  ( -15.81122951014150146, 1460.391797869179982, 222.7693532890990014 ) ) ;
#62298=CIRCLE ( 'NONE', #8619, 1.999994853189497102 ) ;
#62299=CARTESIAN_POINT ( 'NONE',  ( 0.1982234778270909881, 1420.450287161010010, 183.1181652783670017 ) ) ;
#62303=CARTESIAN_POINT ( 'NONE',  ( 17.60455211062490122, 1424.145611629559880, 228.5323410459380113 ) ) ;
#62304=CARTESIAN_POINT ( 'NONE',  ( 20.85715831889999805, 1508.960610664029900, 227.8108771944980049 ) ) ;
#62306=CARTESIAN_POINT ( 'NONE',  ( 13.96291724000000123, 1452.419068613830177, 222.9619438482979774 ) ) ;
#62308=B_SPLINE_CURVE_WITH_KNOTS ( 'NONE', 3,
 ( #31245, #44634, #34002, #87172, #60325, #19393, #27820, #96119, #85490, #436, #86612, #42971, #8235, #69288 ),
 .UNSPECIFIED., .F., .F.,
 ( 4, 2, 2, 2, 2, 2, 4 ),
 ( 0.000000000000000000, 0.1250000000000107969, 0.2500000000000215938, 0.3750000000000324185, 0.5000000000000431877, 0.7500000000000215383, 1.000000000000000000 ),
 .UNSPECIFIED. ) ;
#62309=DIRECTION ( 'NONE',  ( 0.000000000000000000, 0.000000000000000000, -1.000000000000000000 ) ) ;
#62312=VECTOR ( 'NONE', #92343, 1000.000000000000000 ) ;
#62313=CARTESIAN_POINT ( 'NONE',  ( 3.280305111311562882, 1420.304449242272540, 137.1408355299612083 ) ) ;
#62314=CARTESIAN_POINT ( 'NONE',  ( 15.47007019100000136, 1415.932617989529945, 199.1349231852080095 ) ) ;
#62315=CARTESIAN_POINT ( 'NONE',  ( -11.76272948489999948, 1415.263254653229978, 195.3313732026979892 ) ) ;
#62317=CARTESIAN_POINT ( 'NONE',  ( 23.13869945629999947, 1409.885570435330010, 211.1617192280779989 ) ) ;
#62322=CARTESIAN_POINT ( 'NONE',  ( -11.71629925696549890, 1426.709133827190044, 142.6847339683789926 ) ) ;
#62323=CARTESIAN_POINT ( 'NONE',  ( -0.5000711780859999900, 1414.384141482430095, 233.3460081316979995 ) ) ;
#62331=CARTESIAN_POINT ( 'NONE',  ( -18.09406587330949634, 1485.999646426020036, 188.6973973258030242 ) ) ;
#62333=CARTESIAN_POINT ( 'NONE',  ( -4.251699738499429948, 1441.330574127689943, 160.8255607727610084 ) ) ;
#62336=ORIENTED_EDGE ( 'NONE', *, *, #26145, .T. ) ;
#62340=CARTESIAN_POINT ( 'NONE',  ( 1.270728227940000066, 1414.996442546130083, 191.7853923321980005 ) ) ;
#62341=CARTESIAN_POINT ( 'NONE',  ( 15.97151636080159776, 1420.696294072290129, 191.2129961429930063 ) ) ;
#62342=CARTESIAN_POINT ( 'NONE',  ( 0.6486754834729999697, 1508.983017796130071, 179.4114288221979905 ) ) ;
#62343=CARTESIAN_POINT ( 'NONE',  ( 11.91388749740000108, 1435.945967586000052, 151.0354243678980026 ) ) ;
#62345=CARTESIAN_POINT ( 'NONE',  ( -24.50899199022319763, 1451.899203611129906, 137.2765321853150056 ) ) ;
#62347=CARTESIAN_POINT ( 'NONE',  ( 10.73243676400000091, 1409.287845338830039, 228.4682584063980073 ) ) ;
#62350=CARTESIAN_POINT ( 'NONE',  ( 40.94560254887699813, 1440.384112706230098, 134.0999999980729740 ) ) ;
#62356=ORIENTED_EDGE ( 'NONE', *, *, #93859, .F. ) ;
#62358=ORIENTED_EDGE ( 'NONE', *, *, #38617, .F. ) ;
#62359=CARTESIAN_POINT ( 'NONE',  ( 12.82869999662352001, 1444.968790463791493, 169.4459206408119485 ) ) ;
#62361=CARTESIAN_POINT ( 'NONE',  ( 23.08678647408801154, 1450.877676292979459, 141.6717762082134300 ) ) ;
#62364=CARTESIAN_POINT ( 'NONE',  ( -18.53455667172896426, 1445.620152175496969, 214.4552813252731198 ) ) ;
#62366=CARTESIAN_POINT ( 'NONE',  ( 4.235647993021450119, 1446.341752434789896, 163.6975868290139999 ) ) ;
#62370=ORIENTED_EDGE ( 'NONE', *, *, #104913, .T. ) ;
#62371=CARTESIAN_POINT ( 'NONE',  ( 23.72057897983120256, 1440.913060387330006, 234.6026702862579896 ) ) ;
#62372=CARTESIAN_POINT ( 'NONE',  ( -1.247677516857949989E-10, 1452.913060387320002, 152.5211338456990120 ) ) ;
#62373=ORIENTED_EDGE ( 'NONE', *, *, #9057, .F. ) ;
#62374=CARTESIAN_POINT ( 'NONE',  ( 26.53635440841820170, 1450.860531430359970, 136.4336726719780017 ) ) ;
#62375=CARTESIAN_POINT ( 'NONE',  ( -14.62400382660000098, 1410.796324103030202, 190.5396985440980018 ) ) ;
#62377=CARTESIAN_POINT ( 'NONE',  ( -24.41180956639999877, 1441.164382444379953, 212.0429753022879993 ) ) ;
#62380=CARTESIAN_POINT ( 'NONE',  ( -1.116585105924089969E-07, 1397.914279478820163, 196.1218459578329885 ) ) ;
#62385=CARTESIAN_POINT ( 'NONE',  ( 6.763640255447179445E-10, 1465.118916387369836, 238.1343321182859825 ) ) ;
#62387=CIRCLE ( 'NONE', #96311, 24.00543915299668640 ) ;
#62393=CARTESIAN_POINT ( 'NONE',  ( 28.49020452800000314, 1509.161987680929997, 209.1165913312309783 ) ) ;
#62399=CARTESIAN_POINT ( 'NONE',  ( -18.49117142422373306, 1508.844092023391795, 229.9893364342464963 ) ) ;
#62400=CARTESIAN_POINT ( 'NONE',  ( 5.038677020569999776, 1466.838857910729985, 244.5742075766979724 ) ) ;
#62401=CARTESIAN_POINT ( 'NONE',  ( -19.16951723229999871, 1456.627470220629903, 228.8719212425980061 ) ) ;
#62403=CARTESIAN_POINT ( 'NONE',  ( 2.922921630359999856, 1411.762167022229960, 231.6921255610980097 ) ) ;
#62404=CARTESIAN_POINT ( 'NONE',  ( -18.51604897450000209, 1457.427690017329951, 227.8249311441979899 ) ) ;
#62405=CARTESIAN_POINT ( 'NONE',  ( -23.24262678208922850, 1411.085038142911571, 205.4946917536888122 ) ) ;
#62406=CARTESIAN_POINT ( 'NONE',  ( 2.500000000000000000, 1424.377232884329942, 154.7346221771979913 ) ) ;
#62412=CARTESIAN_POINT ( 'NONE',  ( 0.5563350144439999090, 1406.068590282230161, 269.0455876907979587 ) ) ;
#62414=EDGE_CURVE ( 'NONE', #86711, #16155, #3966, .T. ) ;
#62415=CARTESIAN_POINT ( 'NONE',  ( 18.94924769094170358, 1469.137992140839970, 269.8899230648469825 ) ) ;
#62416=EDGE_CURVE ( 'NONE', #20182, #84728, #32080, .T. ) ;
#62417=CARTESIAN_POINT ( 'NONE',  ( 5.492221782479999703, 1439.600215925509929, 154.7521915351979942 ) ) ;
#62418=CARTESIAN_POINT ( 'NONE',  ( -27.65015241038279825, 1446.921110007989910, 137.0757170956930224 ) ) ;
#62420=CARTESIAN_POINT ( 'NONE',  ( -41.11110488297649823, 1440.913060408669935, 260.8062336396970409 ) ) ;
#62421=CARTESIAN_POINT ( 'NONE',  ( -26.88188727640000053, 1446.276387282099904, 137.3361927622979977 ) ) ;
#62422=CARTESIAN_POINT ( 'NONE',  ( 2.096062236828794667, 1450.108350418862301, 154.3469676365364762 ) ) ;
#62423=CARTESIAN_POINT ( 'NONE',  ( -2.500000000000000000, 1448.894380601670036, 183.1110194938549967 ) ) ;
#62424=EDGE_CURVE ( 'NONE', #36324, #66046, #100928, .T. ) ;
#62425=CARTESIAN_POINT ( 'NONE',  ( 2.307020818445200128, 1449.832034875119916, 154.5197330722639890 ) ) ;
#62427=CARTESIAN_POINT ( 'NONE',  ( 25.61394260045869942, 1439.706797436489978, 138.2743463228129883 ) ) ;
#62428=CARTESIAN_POINT ( 'NONE',  ( 19.87032293674588956, 1498.069103587679137, 189.6526576822627987 ) ) ;
#62429=ORIENTED_EDGE ( 'NONE', *, *, #60455, .F. ) ;
#62430=CARTESIAN_POINT ( 'NONE',  ( -13.66603629819999810, 1410.384381565130070, 271.1218459616979999 ) ) ;
#62433=DIRECTION ( 'NONE',  ( 0.000000000000000000, 1.000000000000000000, 0.000000000000000000 ) ) ;
#62434=CARTESIAN_POINT ( 'NONE',  ( -0.8750415373510000983, 1475.042296104029901, 269.6498237395979913 ) ) ;
#62435=CARTESIAN_POINT ( 'NONE',  ( -27.01382282590000017, 1451.969727051930022, 134.9184453750980026 ) ) ;
#62436=CARTESIAN_POINT ( 'NONE',  ( -28.66654242860000323, 1509.598009360030119, 210.2644538831880254 ) ) ;
#62437=CARTESIAN_POINT ( 'NONE',  ( -3.520715165324825424, 1448.288866220005502, 184.8838926225799071 ) ) ;
#62440=B_SPLINE_SURFACE_WITH_KNOTS ( 'NONE', 5, 5, ( 
 ( #79646, #44387, #10776, #3494, #71825, #45504 ),
 ( #27022, #70166, #96432, #37622, #105945, #44948 ),
 ( #29224, #87489, #2948, #95871, #46046, #54455 ),
 ( #11874, #104278, #20798, #55000, #19137, #79095 ),
 ( #105386, #2403, #9646, #36521, #77967, #1275 ),
 ( #88048, #70714, #28674, #62306, #61211, #11333 ) ),
 .UNSPECIFIED., .F., .F., .F.,
 ( 6, 6 ),
 ( 6, 6 ),
 ( 30.32814661849999993, 107.3223151649999920 ),
 ( -5.551115123129999410E-17, 1.000000000000000000 ),
 .UNSPECIFIED. ) ;
#62441=CARTESIAN_POINT ( 'NONE',  ( -18.76751273909999895, 1416.021639799829927, 207.7595312934080312 ) ) ;
#62442=LINE ( 'NONE', #88171, #91210 ) ;
#62443=CARTESIAN_POINT ( 'NONE',  ( 26.51151404034260040, 1435.625518892859873, 136.0790046155120194 ) ) ;
#62444=CARTESIAN_POINT ( 'NONE',  ( -6.860236169661860117, 1396.152625115059891, 217.7799412713499976 ) ) ;
#62446=CARTESIAN_POINT ( 'NONE',  ( -15.07723704620000049, 1422.393407695729820, 228.4053989051980125 ) ) ;
#62448=CARTESIAN_POINT ( 'NONE',  ( -16.86826392510550221, 1409.748713083289886, 225.5163491958089992 ) ) ;
#62449=CARTESIAN_POINT ( 'NONE',  ( 9.690208402899999740, 1434.541746329560056, 148.7586030823979968 ) ) ;
#62450=ORIENTED_EDGE ( 'NONE', *, *, #55672, .F. ) ;
#62452=CARTESIAN_POINT ( 'NONE',  ( 1.137528735100000077, 1408.952783766029825, 230.8528660165980000 ) ) ;
#62453=ADVANCED_FACE ( 'NONE', ( #8079 ), #25093, .F. ) ;
#62455=CARTESIAN_POINT ( 'NONE',  ( 11.19049484690000007, 1426.041365595529896, 112.6496013507980081 ) ) ;
#62457=DIRECTION ( 'NONE',  ( 0.000000000000000000, 0.000000000000000000, -1.000000000000000000 ) ) ;
#62467=AXIS2_PLACEMENT_3D ( 'NONE', #86582, #61972, #76525 ) ;
#62468=EDGE_CURVE ( 'NONE', #98527, #65089, #48184, .T. ) ;
#62470=CARTESIAN_POINT ( 'NONE',  ( -14.92438923741863732, 1460.034730685946442, 231.4439063516318527 ) ) ;
#62471=VERTEX_POINT ( 'NONE', #15093 ) ;
#62475=CARTESIAN_POINT ( 'NONE',  ( -15.60376662210000198, 1409.457955924729958, 192.7658650750980200 ) ) ;
#62476=CARTESIAN_POINT ( 'NONE',  ( 10.78330898009999927, 1453.313060387329870, 226.3563104863980016 ) ) ;
#62479=CARTESIAN_POINT ( 'NONE',  ( -0.2876053136995322945, 1410.303643378096240, 185.0329637903212188 ) ) ;
#62480=CARTESIAN_POINT ( 'NONE',  ( 22.97053994450000047, 1507.867546928429874, 193.7497404625980266 ) ) ;
#62482=CARTESIAN_POINT ( 'NONE',  ( 21.20068119730000333, 1409.653404488529986, 206.8526477052579935 ) ) ;
#62485=CARTESIAN_POINT ( 'NONE',  ( 6.873845516911429421, 1396.153100362309942, 217.7692040646560088 ) ) ;
#62486=CARTESIAN_POINT ( 'NONE',  ( 3.118363024329799948, 1407.662358049740078, 196.0555615279870096 ) ) ;
#62487=CARTESIAN_POINT ( 'NONE',  ( -6.051417934638940288, 1406.798915588060026, 269.4859423177459803 ) ) ;
#62488=DIRECTION ( 'NONE',  ( 0.000000000000000000, 1.000000000000000000, 0.000000000000000000 ) ) ;
#62490=CARTESIAN_POINT ( 'NONE',  ( -11.30129387189999868, 1432.307760205480008, 151.5220333356979836 ) ) ;
#62491=CARTESIAN_POINT ( 'NONE',  ( 12.70666910289999940, 1441.123310893239932, 188.6801198206979961 ) ) ;
#62499=ADVANCED_FACE ( 'NONE', ( #5622 ), #66240, .F. ) ;
#62500=ORIENTED_EDGE ( 'NONE', *, *, #76302, .T. ) ;
#62506=CARTESIAN_POINT ( 'NONE',  ( -20.49387964680000351, 1440.913060387330006, 220.0331557225980248 ) ) ;
#62509=CARTESIAN_POINT ( 'NONE',  ( -5.193270068679999518, 1409.597742502030087, 231.5844012271980148 ) ) ;
#62510=CARTESIAN_POINT ( 'NONE',  ( -11.95969313620000207, 1446.500039657790012, 187.4450217382979815 ) ) ;
#62512=CARTESIAN_POINT ( 'NONE',  ( -14.45326777613875358, 1435.576065321126180, 149.6094576131308429 ) ) ;
#62517=CARTESIAN_POINT ( 'NONE',  ( 43.83783482102600004, 1431.613819724010000, 269.7043230160370513 ) ) ;
#62521=CARTESIAN_POINT ( 'NONE',  ( 0.002486211556402507725, 1508.917723295689939, 238.6614435536396286 ) ) ;
#62525=ORIENTED_EDGE ( 'NONE', *, *, #42808, .F. ) ;
#62526=CARTESIAN_POINT ( 'NONE',  ( 2.500000000000000000, 1438.230658608039903, 157.6902399668979911 ) ) ;
#62527=CARTESIAN_POINT ( 'NONE',  ( -5.228345434639999567, 1420.444146442230021, 232.2530053203980174 ) ) ;
#62532=AXIS2_PLACEMENT_3D ( 'NONE', #85111, #100801, #15677 ) ;
#62535=CARTESIAN_POINT ( 'NONE',  ( 17.10527938397160241, 1469.008053439460127, 229.1126572397060102 ) ) ;
#62536=CARTESIAN_POINT ( 'NONE',  ( -25.50992329942920023, 1509.803886753590177, 223.6772097800239862 ) ) ;
#62538=CARTESIAN_POINT ( 'NONE',  ( -24.91159428870000170, 1442.158245878219759, 210.4732786028779969 ) ) ;
#62539=CARTESIAN_POINT ( 'NONE',  ( 0.1426546239810000116, 1409.853703253230151, 233.2022054432979985 ) ) ;
#62542=CARTESIAN_POINT ( 'NONE',  ( 21.03123203779729877, 1507.789098030329797, 226.0655639048319756 ) ) ;
#62543=CARTESIAN_POINT ( 'NONE',  ( 19.06717825319999804, 1508.525021977130109, 188.3911631520979881 ) ) ;
#62546=CARTESIAN_POINT ( 'NONE',  ( -12.74994028582299954, 1415.933499560010205, 196.6186742867360238 ) ) ;
#62547=FACE_OUTER_BOUND ( 'NONE', #40865, .T. ) ;
#62548=ORIENTED_EDGE ( 'NONE', *, *, #38173, .T. ) ;
#62550=CARTESIAN_POINT ( 'NONE',  ( 3.175611140780000063, 1421.547207231229777, 184.0610320840980307 ) ) ;
#62553=CARTESIAN_POINT ( 'NONE',  ( 18.90950544697915703, 1416.818673806273864, 209.9484509850840084 ) ) ;
#62558=CARTESIAN_POINT ( 'NONE',  ( 17.40764059099999628, 1414.996444526030018, 210.6782161193179945 ) ) ;
#62559=CARTESIAN_POINT ( 'NONE',  ( -18.96495392289999771, 1425.684290752429888, 226.5179610041979856 ) ) ;
#62561=CARTESIAN_POINT ( 'NONE',  ( -20.19975713530000050, 1435.203085175510068, 142.9756137166980068 ) ) ;
#62565=DIRECTION ( 'NONE',  ( -0.000000000000000000, -0.000000000000000000, 1.000000000000000000 ) ) ;
#62566=CARTESIAN_POINT ( 'NONE',  ( 27.09589979614590050, 1438.319408107809977, 136.9553273407819916 ) ) ;
#62569=CARTESIAN_POINT ( 'NONE',  ( 27.04494987192744659, 1509.634160115218492, 216.9800109594045523 ) ) ;
#62576=CARTESIAN_POINT ( 'NONE',  ( 11.77972227726102616, 1435.190141807486953, 151.2912773572372487 ) ) ;
#62579=CARTESIAN_POINT ( 'NONE',  ( -18.59026783009990069, 1509.562244740590131, 185.7097730471209900 ) ) ;
#62580=EDGE_CURVE ( 'NONE', #10196, #104308, #3317, .T. ) ;
#62588=CARTESIAN_POINT ( 'NONE',  ( 22.79519389169999855, 1509.727640877830027, 190.2016567581979984 ) ) ;
#62592=CARTESIAN_POINT ( 'NONE',  ( -0.8945946638535250406, 1417.298095655010002, 235.8147265033050246 ) ) ;
#62595=CARTESIAN_POINT ( 'NONE',  ( 13.12363690099999936, 1441.384603101129869, 188.9419487780980091 ) ) ;
#62597=CARTESIAN_POINT ( 'NONE',  ( 13.11628250257718520, 1443.038395467839564, 169.4035201152188108 ) ) ;
#62598=CARTESIAN_POINT ( 'NONE',  ( 35.04047526790853340, 1424.095413727867026, 269.5320722744115756 ) ) ;
#62599=CARTESIAN_POINT ( 'NONE',  ( -11.55307712329999958, 1469.479397749430063, 255.2309127613979740 ) ) ;
#62602=CARTESIAN_POINT ( 'NONE',  ( -11.90370000490000102, 1433.409417285139853, 150.2262481879979816 ) ) ;
#62604=CARTESIAN_POINT ( 'NONE',  ( -19.05006020489999941, 1485.976765364930088, 189.5158719427979861 ) ) ;
#62605=CARTESIAN_POINT ( 'NONE',  ( 11.42864686989999967, 1410.242058359229986, 189.4498630199979914 ) ) ;
#62606=CARTESIAN_POINT ( 'NONE',  ( 4.908548385079999576, 1422.370476885929975, 184.3612921802979940 ) ) ;
#62608=EDGE_CURVE ( 'NONE', #79161, #80182, #54803, .T. ) ;
#62614=ORIENTED_EDGE ( 'NONE', *, *, #8081, .F. ) ;
#62617=CARTESIAN_POINT ( 'NONE',  ( -15.45910334130000052, 1472.202164814229945, 270.0849031532980007 ) ) ;
#62619=CARTESIAN_POINT ( 'NONE',  ( 3.364556988579999963, 1443.913060387330006, 155.8032249175980155 ) ) ;
#62620=CARTESIAN_POINT ( 'NONE',  ( -15.18343130929999951, 1495.928917307730217, 224.4314295560979815 ) ) ;
#62622=CARTESIAN_POINT ( 'NONE',  ( 14.59882275830000076, 1475.513060387329915, 194.5230232028980026 ) ) ;
#62623=CARTESIAN_POINT ( 'NONE',  ( -12.36841580329999779, 1419.558714398729990, 228.6604469819980068 ) ) ;
#62624=DIRECTION ( 'NONE',  ( 5.364597654988746180E-15, -0.5877852522921409584, 0.8090169943751888137 ) ) ;
#62626=CARTESIAN_POINT ( 'NONE',  ( -44.92397794980949755, 1433.724551782629987, 266.4419929911069858 ) ) ;
#62632=CARTESIAN_POINT ( 'NONE',  ( 15.20184466319999927, 1507.442701412029919, 192.3795476405979912 ) ) ;
#62633=CARTESIAN_POINT ( 'NONE',  ( -20.86058274790000056, 1508.959351158429854, 190.3690864228979933 ) ) ;
#62634=CARTESIAN_POINT ( 'NONE',  ( -14.56904612549999989, 1425.418745057229899, 189.7987151475979886 ) ) ;
#62642=CARTESIAN_POINT ( 'NONE',  ( -13.09932316763100069, 1411.200286183310027, 270.0791247197240068 ) ) ;
#62644=CARTESIAN_POINT ( 'NONE',  ( -1.496858517070000172, 1428.056401037730211, 101.8807690336980016 ) ) ;
#62647=VERTEX_POINT ( 'NONE', #87291 ) ;
#62648=ORIENTED_EDGE ( 'NONE', *, *, #76302, .F. ) ;
#62649=CARTESIAN_POINT ( 'NONE',  ( 45.60270269536359677, 1442.242646908569441, 268.9756891917134567 ) ) ;
#62651=CARTESIAN_POINT ( 'NONE',  ( 3.627217813073119856, 1424.534510419196295, 184.5254139637974617 ) ) ;
#62654=CARTESIAN_POINT ( 'NONE',  ( -20.66004298134364348, 1506.560172258414468, 216.9379300855220265 ) ) ;
#62655=CARTESIAN_POINT ( 'NONE',  ( 2.560290627914949990, 1439.616563506700004, 157.6871905427350100 ) ) ;
#62656=CARTESIAN_POINT ( 'NONE',  ( -0.0001242829754057280032, 1476.076625553489748, 267.5369961020650749 ) ) ;
#62657=CARTESIAN_POINT ( 'NONE',  ( 12.61566532500000015, 1416.819756528530206, 223.3235035255980279 ) ) ;
#62658=CARTESIAN_POINT ( 'NONE',  ( 7.451360406109999168, 1445.833858733300076, 184.1298986146979928 ) ) ;
#62660=EDGE_LOOP ( 'NONE', ( #47196, #27964, #41336 ) ) ;
#62662=CARTESIAN_POINT ( 'NONE',  ( 1.520870652216739893, 1456.386238873960110, 183.3280966458629848 ) ) ;
#62663=ORIENTED_EDGE ( 'NONE', *, *, #22699, .F. ) ;
#62664=CARTESIAN_POINT ( 'NONE',  ( 11.86629848729999992, 1432.349867583790001, 149.9824242020979739 ) ) ;
#62667=CARTESIAN_POINT ( 'NONE',  ( 24.88563714215300138, 1451.888913396479893, 136.5992973529910159 ) ) ;
#62668=CARTESIAN_POINT ( 'NONE',  ( 14.44947381900000138, 1416.568813549730066, 196.8603287955980079 ) ) ;
#62670=CARTESIAN_POINT ( 'NONE',  ( -18.65451756193940014, 1507.632629711779828, 229.7110761618599781 ) ) ;
#62671=CARTESIAN_POINT ( 'NONE',  ( 17.65747903809999997, 1409.529673141430067, 194.8433731264979940 ) ) ;
#62672=CARTESIAN_POINT ( 'NONE',  ( 22.12674011680000064, 1409.685743178530174, 208.3470065124739676 ) ) ;
#62673=CARTESIAN_POINT ( 'NONE',  ( 17.41346922039999967, 1410.020394367130166, 224.8086586025980012 ) ) ;
#62674=CARTESIAN_POINT ( 'NONE',  ( -20.22025100119805074, 1426.743699746497214, 222.0673968628566968 ) ) ;
#62675=CARTESIAN_POINT ( 'NONE',  ( 0.3900490083317569301, 1451.467585376839907, 182.7676827736779899 ) ) ;
#62682=CARTESIAN_POINT ( 'NONE',  ( -0.4378591917222510177, 1409.291352615860205, 232.6949995814360364 ) ) ;
#62684=CARTESIAN_POINT ( 'NONE',  ( -37.55592389275750520, 1449.175610547529914, 136.3350282757720038 ) ) ;
#62686=CARTESIAN_POINT ( 'NONE',  ( -19.62446893450000118, 1440.913060387330006, 214.3676144200779845 ) ) ;
#62687=CIRCLE ( 'NONE', #28683, 4.003638137702854038 ) ;
#62688=CARTESIAN_POINT ( 'NONE',  ( -1.749739496465730015, 1458.392920694240047, 183.8987760949310086 ) ) ;
#62691=CARTESIAN_POINT ( 'NONE',  ( -0.3022264190282230034, 1475.058218936390176, 269.6445798187899641 ) ) ;
#62694=CARTESIAN_POINT ( 'NONE',  ( -20.90646223069999721, 1508.014129115030073, 227.8602063216980014 ) ) ;
#62698=CIRCLE ( 'NONE', #57252, 2.000000000000000000 ) ;
#62699=CARTESIAN_POINT ( 'NONE',  ( -26.60753696249999933, 1509.169818246329896, 201.4350730330979786 ) ) ;
#62702=EDGE_CURVE ( 'NONE', #106344, #3400, #85521, .T. ) ;
#62703=CARTESIAN_POINT ( 'NONE',  ( -6.940787512450000030, 1485.992914485530264, 182.8505493415979970 ) ) ;
#62707=CARTESIAN_POINT ( 'NONE',  ( 24.93712286909999776, 1430.363841012629791, 209.4446161091190106 ) ) ;
#62708=ADVANCED_FACE ( 'NONE', ( #24465 ), #41189, .F. ) ;
#62713=CARTESIAN_POINT ( 'NONE',  ( -16.81223434880759982, 1414.913060387349788, 207.5743820648510223 ) ) ;
#62718=CARTESIAN_POINT ( 'NONE',  ( -1.342110535129999782, 1416.822692871130130, 228.0800075106980103 ) ) ;
#62724=ORIENTED_EDGE ( 'NONE', *, *, #4250, .F. ) ;
#62726=CARTESIAN_POINT ( 'NONE',  ( -17.97082668629999702, 1416.218047894730262, 209.4769668406679841 ) ) ;
#62730=CIRCLE ( 'NONE', #5535, 4.014131127992580872 ) ;
#62732=CARTESIAN_POINT ( 'NONE',  ( 14.92368822464059974, 1409.434207063760141, 209.5555605250399935 ) ) ;
#62737=CARTESIAN_POINT ( 'NONE',  ( -18.01647495410000133, 1424.182360087930192, 192.6480262483979971 ) ) ;
#62742=ADVANCED_FACE ( 'NONE', ( #33984 ), #99237, .F. ) ;
#62743=CARTESIAN_POINT ( 'NONE',  ( -11.94034776685189847, 1415.658863692659907, 194.9858853494239952 ) ) ;
#62746=CARTESIAN_POINT ( 'NONE',  ( 35.09256191701995675, 1457.673633888417044, 269.5327811216627083 ) ) ;
#62748=CARTESIAN_POINT ( 'NONE',  ( 1.171355130469999839, 1396.015413588030015, 220.7560819512980004 ) ) ;
#62750=CARTESIAN_POINT ( 'NONE',  ( 0.2101337101240000060, 1457.272896011530293, 183.0700940124980036 ) ) ;
#62755=CARTESIAN_POINT ( 'NONE',  ( -13.17405550470000186, 1435.081114633759853, 149.9571693888979951 ) ) ;
#62756=CARTESIAN_POINT ( 'NONE',  ( 1.121350905119999908, 1416.825532216630108, 190.1588586452979825 ) ) ;
#62757=CARTESIAN_POINT ( 'NONE',  ( -0.3791074914540970009, 1489.809295140069935, 187.8701616902860110 ) ) ;
#62759=CARTESIAN_POINT ( 'NONE',  ( 41.61456305172699643, 1444.048090539929944, 136.0122178056329858 ) ) ;
#62761=CARTESIAN_POINT ( 'NONE',  ( 38.63859240729999556, 1428.253853516829849, 261.7057271117980122 ) ) ;
#62762=CARTESIAN_POINT ( 'NONE',  ( -25.57394744089999961, 1488.682087795429879, 201.8621879095979921 ) ) ;
#62763=CARTESIAN_POINT ( 'NONE',  ( -2.553569726430000131, 1507.269243784629907, 180.8456350314980057 ) ) ;
#62764=CARTESIAN_POINT ( 'NONE',  ( 3.399097891949999726E-14, 1411.680853644829995, 266.9202418608980452 ) ) ;
#62768=CARTESIAN_POINT ( 'NONE',  ( -31.69751081790000313, 1436.813883499979966, 244.1892870165980014 ) ) ;
#62769=CARTESIAN_POINT ( 'NONE',  ( 19.55529463106600119, 1509.624433752180039, 231.4241880222230066 ) ) ;
#62770=CARTESIAN_POINT ( 'NONE',  ( 4.046387026569544076, 1446.994266134431655, 154.8289846805161005 ) ) ;
#62771=CARTESIAN_POINT ( 'NONE',  ( 33.92643251289999995, 1451.728352207130001, 135.1493744902979870 ) ) ;
#62773=CARTESIAN_POINT ( 'NONE',  ( -5.377564849545230174, 1430.035755479769932, 154.3918570002599893 ) ) ;
#62775=CARTESIAN_POINT ( 'NONE',  ( 16.19087789078229989, 1409.478458302130093, 193.2334102746530107 ) ) ;
#62780=CARTESIAN_POINT ( 'NONE',  ( -23.02675208173420174, 1409.747009289400012, 208.9090590340030076 ) ) ;
#62785=CARTESIAN_POINT ( 'NONE',  ( 0.3570154777189999962, 1451.680777065829943, 183.0662967611979752 ) ) ;
#62786=CARTESIAN_POINT ( 'NONE',  ( -2.007783359929999900, 1479.773924900330030, 235.8303969823979855 ) ) ;
#62789=CARTESIAN_POINT ( 'NONE',  ( 11.15477664960000048, 1425.160652183429875, 144.1598853320980140 ) ) ;
#62791=CARTESIAN_POINT ( 'NONE',  ( 14.41941774000000009, 1474.742523832529969, 225.1206985227979942 ) ) ;
#62796=CARTESIAN_POINT ( 'NONE',  ( 11.86283928301630120, 1432.108153224739908, 149.9775622573939984 ) ) ;
#62797=CARTESIAN_POINT ( 'NONE',  ( 12.75800579317462891, 1444.997181870303393, 186.4738022370279396 ) ) ;
#62799=ORIENTED_EDGE ( 'NONE', *, *, #71313, .F. ) ;
#62805=CARTESIAN_POINT ( 'NONE',  ( 19.21825364151619908, 1452.241944181910185, 144.1553783344959925 ) ) ;
#62806=CARTESIAN_POINT ( 'NONE',  ( 0.9556514315352180322, 1409.785933179500034, 270.0714045367960239 ) ) ;
#62813=CARTESIAN_POINT ( 'NONE',  ( 14.15593876370000004, 1435.008643399779885, 195.7735139947980088 ) ) ;
#62818=B_SPLINE_CURVE_WITH_KNOTS ( 'NONE', 5,
 ( #43795, #53890, #704, #77946, #60064, #51650 ),
 .UNSPECIFIED., .F., .F.,
 ( 6, 6 ),
 ( -0.9267553667292389719, 5.517427126029999407 ),
 .UNSPECIFIED. ) ;
#62821=CARTESIAN_POINT ( 'NONE',  ( 28.02005515429999960, 1437.694013773219922, 248.0989693021979861 ) ) ;
#62822=CARTESIAN_POINT ( 'NONE',  ( 18.63787275302323465, 1508.244465050627696, 188.4525138201056507 ) ) ;
#62828=ORIENTED_EDGE ( 'NONE', *, *, #30904, .F. ) ;
#62838=CARTESIAN_POINT ( 'NONE',  ( 27.28440919872599935, 1509.865850533680032, 222.5516304213150249 ) ) ;
#62841=CARTESIAN_POINT ( 'NONE',  ( 14.74268596870000003, 1415.084640305229868, 227.8479518795979857 ) ) ;
#62843=CARTESIAN_POINT ( 'NONE',  ( -17.15058533566899968, 1460.897024810804169, 228.2718108823579826 ) ) ;
#62845=CARTESIAN_POINT ( 'NONE',  ( 45.27970250219999571, 1434.949994644049866, 268.7737451221979654 ) ) ;
#62846=CARTESIAN_POINT ( 'NONE',  ( -17.82654646940000021, 1409.700512582729971, 223.9827240008980027 ) ) ;
#62847=CARTESIAN_POINT ( 'NONE',  ( 15.62192944049999888, 1435.060616691779842, 147.8543328025979804 ) ) ;
#62849=CARTESIAN_POINT ( 'NONE',  ( 20.25069675820000015, 1488.587216004930042, 190.8938461704979943 ) ) ;
#62850=CARTESIAN_POINT ( 'NONE',  ( -16.66259792569089981, 1410.427225285170152, 191.7596848084640158 ) ) ;
#62853=CARTESIAN_POINT ( 'NONE',  ( -18.29970625680000040, 1473.000870360929866, 266.8291869051980143 ) ) ;
#62857=DIRECTION ( 'NONE',  ( 1.000000000000000000, -2.740606396879999932E-15, 3.772597702940000410E-15 ) ) ;
#62859=CARTESIAN_POINT ( 'NONE',  ( -12.06734954289999884, 1442.226007087160042, 187.2421031291980000 ) ) ;
#62861=CARTESIAN_POINT ( 'NONE',  ( -27.90835392674980042, 1508.762510115379882, 210.5978890894100175 ) ) ;
#62862=CARTESIAN_POINT ( 'NONE',  ( 11.87595595069999987, 1433.006363244350268, 146.4341592748980077 ) ) ;
#62863=CARTESIAN_POINT ( 'NONE',  ( -30.21734179830000144, 1436.028192106169854, 136.4151164768979925 ) ) ;
#62867=CARTESIAN_POINT ( 'NONE',  ( -5.774656115207120521, 1409.114715822440075, 222.9363759656519903 ) ) ;
#62870=CARTESIAN_POINT ( 'NONE',  ( -37.71859155314457013, 1442.773887286370382, 136.8575361162813238 ) ) ;
#62871=CARTESIAN_POINT ( 'NONE',  ( -46.05260025390000322, 1446.035358659930125, 266.6770541026980368 ) ) ;
#62872=CARTESIAN_POINT ( 'NONE',  ( -16.37398935204720019, 1478.527142925449880, 223.3409276542839734 ) ) ;
#62873=CARTESIAN_POINT ( 'NONE',  ( 0.1601292279041169886, 1420.232911783010195, 183.6671598589649932 ) ) ;
#62874=CARTESIAN_POINT ( 'NONE',  ( -27.34968394090000032, 1509.645410702830077, 214.2836711016779816 ) ) ;
#62879=CARTESIAN_POINT ( 'NONE',  ( 16.05891525850000079, 1416.823418193329871, 217.6350310302879905 ) ) ;
#62880=CARTESIAN_POINT ( 'NONE',  ( 18.11157395349999888, 1509.545530486529969, 186.5307135875980009 ) ) ;
#62883=ORIENTED_EDGE ( 'NONE', *, *, #69860, .F. ) ;
#62884=CARTESIAN_POINT ( 'NONE',  ( -3.535396145210000007, 1507.776748965729894, 180.9473349428980100 ) ) ;
#62885=CARTESIAN_POINT ( 'NONE',  ( -24.02116941819999951, 1411.112860734130209, 208.3416100540740103 ) ) ;
#62886=AXIS2_PLACEMENT_3D ( 'NONE', #14392, #91666, #101150 ) ;
#62887=EDGE_CURVE ( 'NONE', #94000, #61499, #97435, .T. ) ;
#62889=CARTESIAN_POINT ( 'NONE',  ( -11.41983032799999975, 1415.048591094029916, 195.6129360477979731 ) ) ;
#62891=CARTESIAN_POINT ( 'NONE',  ( 22.42609733799999816, 1409.696196963129978, 212.0712440230379912 ) ) ;
#62892=CARTESIAN_POINT ( 'NONE',  ( -12.17235240719999823, 1434.042297368109985, 149.7137827380979900 ) ) ;
#62897=CARTESIAN_POINT ( 'NONE',  ( -0.1099389607409999997, 1413.018602985929874, 233.3789693115979844 ) ) ;
#62904=CARTESIAN_POINT ( 'NONE',  ( 13.37364840053160187, 1507.560048672190078, 233.0513862518880046 ) ) ;
#62905=CARTESIAN_POINT ( 'NONE',  ( -18.13105147114099935, 1486.178406859650067, 188.5764279912840209 ) ) ;
#62909=VERTEX_POINT ( 'NONE', #28176 ) ;
#62911=CARTESIAN_POINT ( 'NONE',  ( 27.73048959930000024, 1508.610947985129997, 212.2558594092780027 ) ) ;
#62912=ORIENTED_EDGE ( 'NONE', *, *, #90736, .T. ) ;
#62915=CARTESIAN_POINT ( 'NONE',  ( -3.677837710089999800E-15, 1426.566393376330097, 144.1938086916980239 ) ) ;
#62916=CARTESIAN_POINT ( 'NONE',  ( 15.76697546804739858, 1409.471978965290191, 192.7550041694750007 ) ) ;
#62919=CARTESIAN_POINT ( 'NONE',  ( -24.43436514662279890, 1452.059797509780083, 135.9947029744789972 ) ) ;
#62920=CARTESIAN_POINT ( 'NONE',  ( 10.69300205652376690, 1438.695736345125624, 152.5084499697617559 ) ) ;
#62921=CARTESIAN_POINT ( 'NONE',  ( 12.52547985540000042, 1410.283479796730035, 228.7537008404979986 ) ) ;
#62922=PRESENTATION_STYLE_ASSIGNMENT (( #46641 ) ) ;
#62924=CARTESIAN_POINT ( 'NONE',  ( 41.46889560158410148, 1441.954934106449855, 134.0999999980859911 ) ) ;
#62926=ORIENTED_EDGE ( 'NONE', *, *, #95207, .F. ) ;
#62931=VERTEX_POINT ( 'NONE', #10834 ) ;
#62934=CARTESIAN_POINT ( 'NONE',  ( 14.09811198787718389, 1451.182526868617742, 150.3098712486240345 ) ) ;
#62935=CARTESIAN_POINT ( 'NONE',  ( 0.000000000000000000, 1519.913060387329779, 209.1218459616979999 ) ) ;
#62941=CARTESIAN_POINT ( 'NONE',  ( 1.118067181730000081, 1508.368074802429874, 237.6116800887979821 ) ) ;
#62942=EDGE_LOOP ( 'NONE', ( #2436, #25936, #13400, #105930 ) ) ;
#62944=VERTEX_POINT ( 'NONE', #106533 ) ;
#62945=CARTESIAN_POINT ( 'NONE',  ( 23.39958255221609917, 1440.913060387330006, 233.3680888324570049 ) ) ;
#62946=CARTESIAN_POINT ( 'NONE',  ( -16.42304823919999990, 1508.244897181629995, 185.8512656781980183 ) ) ;
#62948=CARTESIAN_POINT ( 'NONE',  ( 26.97427084300169753, 1450.930614134690131, 136.4066763474399977 ) ) ;
#62949=CARTESIAN_POINT ( 'NONE',  ( -14.76096091410000000, 1409.595176565530210, 191.2496112059980078 ) ) ;
#62951=CARTESIAN_POINT ( 'NONE',  ( -24.41204057910000103, 1440.938895779720042, 212.0297384891179888 ) ) ;
#62954=CARTESIAN_POINT ( 'NONE',  ( 15.70021604296872830, 1414.913060387330006, 214.2279672958994183 ) ) ;
#62955=CARTESIAN_POINT ( 'NONE',  ( -1.417434298042890006, 1448.552296757619843, 227.8906923748210147 ) ) ;
#62958=CARTESIAN_POINT ( 'NONE',  ( 4.477818878069999897, 1465.350087406130115, 234.1438911684979871 ) ) ;
#62968=EDGE_LOOP ( 'NONE', ( #47537, #38455, #17805, #40428 ) ) ;
#62970=CARTESIAN_POINT ( 'NONE',  ( 29.79081509959999607, 1446.796541106770064, 240.1465591158980146 ) ) ;
#62971=CARTESIAN_POINT ( 'NONE',  ( -11.30248206070000094, 1432.393890462980153, 151.5218268353980022 ) ) ;
#62973=CARTESIAN_POINT ( 'NONE',  ( 2.669715429490000069, 1413.149521960129960, 231.7915367626979730 ) ) ;
#62974=CARTESIAN_POINT ( 'NONE',  ( -19.33162846839999816, 1457.452151859230071, 226.3466835555979912 ) ) ;
#62976=CARTESIAN_POINT ( 'NONE',  ( 11.30116471560000058, 1432.303966848209939, 151.5220940858980043 ) ) ;
#62977=LINE ( 'NONE', #97089, #47956 ) ;
#62983=CARTESIAN_POINT ( 'NONE',  ( 0.7748160517030000527, 1405.993929547030120, 266.9609161638979913 ) ) ;
#62985=CARTESIAN_POINT ( 'NONE',  ( 13.02735688232990086, 1471.728350752560118, 270.3681568976120388 ) ) ;
#62986=CARTESIAN_POINT ( 'NONE',  ( 2.478578393939999902, 1437.039673764719964, 157.6668020507979975 ) ) ;
#62987=CARTESIAN_POINT ( 'NONE',  ( 11.60004869885203682, 1423.972964970261728, 135.9380568969748708 ) ) ;
#62989=CARTESIAN_POINT ( 'NONE',  ( -38.68338032125110004, 1440.913060393820160, 257.3519283540039737 ) ) ;
#62990=CARTESIAN_POINT ( 'NONE',  ( 36.00227838366810573, 1442.549544120750170, 137.1411661020360100 ) ) ;
#62991=CARTESIAN_POINT ( 'NONE',  ( 2.440646991155576373, 1449.387360343648879, 154.4793733419271859 ) ) ;
#62992=B_SPLINE_CURVE_WITH_KNOTS ( 'NONE', 3,
 ( #1638, #68849, #77780, #27926, #95130, #60440, #1090, #52036, #94558, #10016, #26252, #11674, #71066, #27367, #78326, #86725, #78897, #105188, #35776, #9465, #61549, #2203, #18948, #35216, #20064, #69402, #18392, #70514, #26817, #102951, #53143, #10576, #104072, #44747, #36317, #104629, #17833, #53714, #52591, #69958 ),
 .UNSPECIFIED., .F., .F.,
 ( 4, 2, 2, 2, 1, 1, 2, 2, 2, 2, 1, 1, 1, 2, 2, 2, 2, 1, 1, 1, 2, 2, 2, 4 ),
 ( 0.000000000000000000, 0.1249999999996785072, 0.1874999999995110578, 0.2187499999994365618, 0.2343749999994061695, 0.2421874999993911537, 0.2460937499993812727, 0.2499999999993713917, 0.3749999999997545297, 0.4374999999999461542, 0.4687500000000272005, 0.4843750000000677236, 0.4921875000000839329, 0.4960937500000920375, 0.5000000000001001421, 0.6250000000007530643, 0.6875000000010847989, 0.7187500000012642110, 0.7343750000013491430, 0.7421875000013915535, 0.7460937500014258594, 0.7500000000014600543, 0.8750000000007300827, 1.000000000000000000 ),
 .UNSPECIFIED. ) ;
#62994=CARTESIAN_POINT ( 'NONE',  ( 0.8729611875899290219, 1450.882575902080134, 154.5162442169400094 ) ) ;
#62996=DIRECTION ( 'NONE',  ( 0.000000000000000000, 0.7071067811865198172, -0.7071067811865753283 ) ) ;
#62999=CARTESIAN_POINT ( 'NONE',  ( -5.757839681930000175, 1413.763055107629953, 262.6648722463980334 ) ) ;
#63001=CARTESIAN_POINT ( 'NONE',  ( -0.7721454155100000438, 1475.556447494730037, 269.2944986523980333 ) ) ;
#63002=CARTESIAN_POINT ( 'NONE',  ( -4.282859847165069844, 1446.856630987190101, 156.0743107980160005 ) ) ;
#63009=CARTESIAN_POINT ( 'NONE',  ( 26.36150907684390177, 1435.617380069360024, 136.0950546535589751 ) ) ;
#63010=CARTESIAN_POINT ( 'NONE',  ( -7.067966366155039815, 1396.159879213149907, 217.6086540106699942 ) ) ;
#63012=CARTESIAN_POINT ( 'NONE',  ( -15.07865052128000016, 1422.394146857109945, 228.4054231139910200 ) ) ;
#63013=CARTESIAN_POINT ( 'NONE',  ( -16.69321520597850039, 1410.132469723700069, 226.2257568831570040 ) ) ;
#63014=CARTESIAN_POINT ( 'NONE',  ( -45.63527004870000070, 1440.521702456270077, 268.9748019413980273 ) ) ;
#63018=FACE_OUTER_BOUND ( 'NONE', #37099, .T. ) ;
#63019=CARTESIAN_POINT ( 'NONE',  ( 11.17628604429999939, 1426.885039317430255, 103.4432774836980116 ) ) ;
#63022=CARTESIAN_POINT ( 'NONE',  ( -12.37499353609999986, 1442.762691980110048, 205.2217743980949933 ) ) ;
#63027=CARTESIAN_POINT ( 'NONE',  ( 3.211749723379999644, 1507.435849901630036, 181.4459671118979998 ) ) ;
#63028=CARTESIAN_POINT ( 'NONE',  ( -0.08492873674538491124, 1416.830086716310007, 191.0182577611500108 ) ) ;
#63032=VERTEX_POINT ( 'NONE', #63467 ) ;
#63033=ORIENTED_EDGE ( 'NONE', *, *, #24074, .T. ) ;
#63035=CARTESIAN_POINT ( 'NONE',  ( 0.8611642483871809750, 1507.132556045299907, 237.2366988190680104 ) ) ;
#63036=CARTESIAN_POINT ( 'NONE',  ( 13.15726447020000123, 1414.996442546130083, 197.7616625855980033 ) ) ;
#63039=CARTESIAN_POINT ( 'NONE',  ( 12.32904923398311325, 1414.913060387329779, 198.2898876794709224 ) ) ;
#63045=CARTESIAN_POINT ( 'NONE',  ( 33.93535975524210357, 1435.841728338589974, 135.9422392606320216 ) ) ;
#63046=CARTESIAN_POINT ( 'NONE',  ( -6.122330375623380228, 1406.076006365369949, 268.4678845349259859 ) ) ;
#63047=CARTESIAN_POINT ( 'NONE',  ( 41.14740357920000235, 1443.969947807379867, 136.9302553032979972 ) ) ;
#63048=ORIENTED_EDGE ( 'NONE', *, *, #89984, .F. ) ;
#63050=CARTESIAN_POINT ( 'NONE',  ( 11.76268527979999945, 1441.457099483779757, 188.0189021094980149 ) ) ;
#63052=ORIENTED_EDGE ( 'NONE', *, *, #98759, .T. ) ;
#63058=CARTESIAN_POINT ( 'NONE',  ( 2.500000000000000000, 1448.437146640389983, 161.5787848790610326 ) ) ;
#63061=ADVANCED_FACE ( 'NONE', ( #12473 ), #7218, .F. ) ;
#63063=CARTESIAN_POINT ( 'NONE',  ( 16.90152335259999816, 1414.971339025629959, 212.5779198278579827 ) ) ;
#63069=CARTESIAN_POINT ( 'NONE',  ( -5.237765362120001100, 1410.471163508729887, 231.7868085280980210 ) ) ;
#63070=CARTESIAN_POINT ( 'NONE',  ( -15.96958168569999970, 1519.913060387329779, 191.7668369663979888 ) ) ;
#63072=CARTESIAN_POINT ( 'NONE',  ( 31.77002005290000142, 1451.803664145230186, 134.7784598387979997 ) ) ;
#63073=CARTESIAN_POINT ( 'NONE',  ( -26.43364689489139963, 1440.913060452569880, 224.1083565477900095 ) ) ;
#63075=DIRECTION ( 'NONE',  ( 0.3892484888175031799, -0.9211327884476211425, 0.000000000000000000 ) ) ;
#63076=CARTESIAN_POINT ( 'NONE',  ( 35.41142118405590367, 1421.645479188649915, 270.3426747825220104 ) ) ;
#63080=CARTESIAN_POINT ( 'NONE',  ( -7.766142847955903150, 1425.761605071012127, 225.8812321164998025 ) ) ;
#63082=CARTESIAN_POINT ( 'NONE',  ( 21.04378882164967379, 1411.007238685950597, 200.0432284193734915 ) ) ;
#63085=CARTESIAN_POINT ( 'NONE',  ( 22.79764478813683581, 1411.075395668607598, 207.0126141096596371 ) ) ;
#63086=CARTESIAN_POINT ( 'NONE',  ( -2.816706472479999945, 1415.376295151229897, 232.8007527343979746 ) ) ;
#63087=ADVANCED_FACE ( 'NONE', ( #24692 ), #17393, .F. ) ;
#63093=CARTESIAN_POINT ( 'NONE',  ( -24.15153490410000359, 1438.063247892820073, 212.1983423404379892 ) ) ;
#63094=CARTESIAN_POINT ( 'NONE',  ( -24.90943706210489950, 1441.448768262790054, 210.4417431393899847 ) ) ;
#63097=CARTESIAN_POINT ( 'NONE',  ( -0.1262818449771200280, 1420.460208507500056, 182.7273227126599977 ) ) ;
#63103=CARTESIAN_POINT ( 'NONE',  ( -11.84669589607570117, 1415.088506334930116, 196.8357868303870077 ) ) ;
#63104=CARTESIAN_POINT ( 'NONE',  ( -0.7142343592189999146, 1485.913060387329779, 181.6617165099980014 ) ) ;
#63106=CARTESIAN_POINT ( 'NONE',  ( 0.3822502236720000113, 1506.811133769929938, 231.1177528848980103 ) ) ;
#63107=CARTESIAN_POINT ( 'NONE',  ( 11.14671379024469999, 1434.019377051509991, 151.6529839732360188 ) ) ;
#63110=CARTESIAN_POINT ( 'NONE',  ( 16.33841777375469562, 1421.565078431612619, 227.2260880633069178 ) ) ;
#63111=CARTESIAN_POINT ( 'NONE',  ( -3.653657264520000059, 1446.290935081919997, 168.9981087857980242 ) ) ;
#63112=CARTESIAN_POINT ( 'NONE',  ( -5.731937517950226990, 1432.353341358200169, 149.9895731141591000 ) ) ;
#63113=CARTESIAN_POINT ( 'NONE',  ( -15.70342473219999846, 1435.191803117289965, 148.3090083168980016 ) ) ;
#63117=CARTESIAN_POINT ( 'NONE',  ( -18.95277575333325615, 1439.030827722083131, 210.3414025166298131 ) ) ;
#63118=CARTESIAN_POINT ( 'NONE',  ( -0.1847390196904469817, 1457.875415826569906, 229.1891656909159849 ) ) ;
#63123=CARTESIAN_POINT ( 'NONE',  ( -24.42533947069999911, 1437.817911553419890, 210.7709913334879843 ) ) ;
#63125=CARTESIAN_POINT ( 'NONE',  ( -18.65451768850000036, 1507.632629712929884, 229.7110761578979918 ) ) ;
#63127=CARTESIAN_POINT ( 'NONE',  ( 11.46781549567650593, 1434.775379691847320, 151.4529278985016845 ) ) ;
#63131=PRODUCT_DEFINITION ( 'UNKNOWN', '', #24370, #37868 ) ;
#63135=LINE ( 'NONE', #50698, #104743 ) ;
#63136=CARTESIAN_POINT ( 'NONE',  ( 22.34603363939999809, 1509.636789321229799, 190.4959359729979838 ) ) ;
#63142=CARTESIAN_POINT ( 'NONE',  ( 11.78238356083980065, 1440.882651838439870, 188.1224447589279976 ) ) ;
#63144=CARTESIAN_POINT ( 'NONE',  ( 12.57606862101337519, 1442.780661812642620, 169.4711452238722416 ) ) ;
#63145=CARTESIAN_POINT ( 'NONE',  ( 29.80102004019969897, 1419.431233126144662, 269.4687009151867301 ) ) ;
#63146=CARTESIAN_POINT ( 'NONE',  ( -29.14244563990000003, 1446.680133300080115, 238.0755268643980003 ) ) ;
#63147=CARTESIAN_POINT ( 'NONE',  ( -19.71969760489999857, 1491.250796832030119, 189.6734715901979769 ) ) ;
#63148=CARTESIAN_POINT ( 'NONE',  ( -11.93616985209999903, 1433.496130944540027, 150.0979445124980032 ) ) ;
#63150=CARTESIAN_POINT ( 'NONE',  ( 26.93106841620000225, 1509.630720109830008, 201.7989744196580091 ) ) ;
#63151=CARTESIAN_POINT ( 'NONE',  ( -18.97833546889999923, 1485.957402666529788, 189.4643713726979684 ) ) ;
#63154=CARTESIAN_POINT ( 'NONE',  ( 4.923253753420000933, 1424.943525846130115, 185.6775012255980073 ) ) ;
#63156=CARTESIAN_POINT ( 'NONE',  ( 6.218421307649999896, 1442.637438617560065, 154.8383831848980208 ) ) ;
#63158=CARTESIAN_POINT ( 'NONE',  ( -19.97163517270000099, 1451.785673805730084, 145.5354985206979848 ) ) ;
#63161=VERTEX_POINT ( 'NONE', #54905 ) ;
#63162=CARTESIAN_POINT ( 'NONE',  ( -11.86392824893790099, 1432.184205469619883, 149.9802395947019988 ) ) ;
#63164=CARTESIAN_POINT ( 'NONE',  ( -34.72211068080000018, 1462.213514433730097, 270.0646873488980191 ) ) ;
#63166=CARTESIAN_POINT ( 'NONE',  ( 9.624350592200000776, 1441.605633920840091, 153.1179271311979733 ) ) ;
#63167=CARTESIAN_POINT ( 'NONE',  ( -15.80679508490000273, 1506.802866820429927, 224.6866773128980128 ) ) ;
#63170=CARTESIAN_POINT ( 'NONE',  ( -12.26257701979999837, 1420.531538507830192, 229.3828047662979941 ) ) ;
#63173=CARTESIAN_POINT ( 'NONE',  ( -45.53644742934309875, 1435.582664252089899, 266.6938170526619842 ) ) ;
#63175=CARTESIAN_POINT ( 'NONE',  ( -3.540994294616410354, 1498.936809983509875, 181.3258807172460081 ) ) ;
#63176=ORIENTED_EDGE ( 'NONE', *, *, #63800, .T. ) ;
#63180=CARTESIAN_POINT ( 'NONE',  ( 4.500000000000000000, 1425.929641636930000, 183.3886486283980162 ) ) ;
#63182=ORIENTED_EDGE ( 'NONE', *, *, #30904, .T. ) ;
#63183=CARTESIAN_POINT ( 'NONE',  ( -4.026786250540000722, 1415.442497638829991, 163.1427597075980032 ) ) ;
#63191=CARTESIAN_POINT ( 'NONE',  ( -13.59643806539980027, 1409.123878638069982, 270.0979091653910018 ) ) ;
#63195=EDGE_LOOP ( 'NONE', ( #66774, #9580, #93571, #21660, #47876 ) ) ;
#63197=CARTESIAN_POINT ( 'NONE',  ( 44.72660186364661428, 1447.710275772193654, 269.0002519517747714 ) ) ;
#63198=ADVANCED_FACE ( 'NONE', ( #106392 ), #70077, .F. ) ;
#63200=CARTESIAN_POINT ( 'NONE',  ( 3.674553501219381069, 1424.234175143221591, 184.0560900496116972 ) ) ;
#63201=CARTESIAN_POINT ( 'NONE',  ( -33.44263403534804269, 1416.839417735997131, 266.5283828626972991 ) ) ;
#63202=EDGE_CURVE ( 'NONE', #45986, #106196, #49463, .T. ) ;
#63203=DIRECTION ( 'NONE',  ( 1.000000000000000000, 0.000000000000000000, 2.004237160840000101E-13 ) ) ;
#63205=CARTESIAN_POINT ( 'NONE',  ( -14.56125758019999950, 1423.490991497129926, 221.7880315116979943 ) ) ;
#63206=CARTESIAN_POINT ( 'NONE',  ( 11.80119706069999985, 1415.163755984229965, 222.4114065333980079 ) ) ;
#63210=PLANE ( 'NONE',  #40203 ) ;
#63211=CARTESIAN_POINT ( 'NONE',  ( -24.04659120089169733, 1444.796772349889807, 212.0316830080810178 ) ) ;
#63213=CARTESIAN_POINT ( 'NONE',  ( 10.48296864959158192, 1455.202037190736291, 226.3317574583255407 ) ) ;
#63214=CARTESIAN_POINT ( 'NONE',  ( -27.85007289616701698, 1509.193792693449723, 210.7874565944711378 ) ) ;
#63217=CARTESIAN_POINT ( 'NONE',  ( -2.919621720534709919, 1419.522956690290130, 186.2043860719099939 ) ) ;
#63219=CARTESIAN_POINT ( 'NONE',  ( 23.10442914280000082, 1411.095127664230176, 207.3185324329880075 ) ) ;
#63220=CARTESIAN_POINT ( 'NONE',  ( -0.02516806119179999801, 1415.404723302029879, 233.4400559027980080 ) ) ;
#63223=CARTESIAN_POINT ( 'NONE',  ( 0.5501147289262610096, 1452.327375750520105, 183.2609232956120024 ) ) ;
#63224=CARTESIAN_POINT ( 'NONE',  ( 2.500000000000000000, 1439.569237558239820, 165.5254318433829894 ) ) ;
#63230=B_SPLINE_SURFACE_WITH_KNOTS ( 'NONE', 5, 5, ( 
 ( #87603, #26565, #62421, #104943, #18705, #25995 ),
 ( #85930, #87032, #61869, #28234, #78080, #60761 ),
 ( #95987, #94884, #45064, #79207, #96547, #69719 ),
 ( #19820, #103837, #43936, #51790, #14020, #31934 ),
 ( #22403, #24067, #11443, #14577, #58260, #97100 ),
 ( #99124, #81779, #45618, #3065, #23530, #39232 ) ),
 .UNSPECIFIED., .F., .F., .F.,
 ( 6, 6 ),
 ( 6, 6 ),
 ( 6.877177566609999460, 14.96017628310000092 ),
 ( 0.000000000000000000, 2.000000000000000000 ),
 .UNSPECIFIED. ) ;
#63232=CARTESIAN_POINT ( 'NONE',  ( -18.16418870590820234, 1416.835419214280137, 209.0763567938479923 ) ) ;
#63234=CARTESIAN_POINT ( 'NONE',  ( -39.78974365313739270, 1446.312716817450109, 136.7506402475469827 ) ) ;
#63235=CARTESIAN_POINT ( 'NONE',  ( 11.60004869885203860, 1425.208448849134129, 137.9974123457472501 ) ) ;
#63237=CARTESIAN_POINT ( 'NONE',  ( 41.65772607930001215, 1455.325942033426145, 266.3040522087976569 ) ) ;
#63238=CARTESIAN_POINT ( 'NONE',  ( 11.59187693560000021, 1433.125071996289989, 151.1000449916980131 ) ) ;
#63240=CARTESIAN_POINT ( 'NONE',  ( 24.59498489902570029, 1440.913044926110160, 213.3385239659299941 ) ) ;
#63243=ORIENTED_EDGE ( 'NONE', *, *, #74134, .T. ) ;
#63247=CARTESIAN_POINT ( 'NONE',  ( 12.53380665967529950, 1445.052233242549846, 186.0874955919830143 ) ) ;
#63250=CARTESIAN_POINT ( 'NONE',  ( -17.56617790150000147, 1509.356465178830149, 231.0161195107979779 ) ) ;
#63253=CARTESIAN_POINT ( 'NONE',  ( 5.407433588731190177, 1422.540975204839924, 131.0095517816550057 ) ) ;
#63255=CARTESIAN_POINT ( 'NONE',  ( 1.971096436429999654, 1464.814372936629979, 236.1963158674979866 ) ) ;
#63258=CARTESIAN_POINT ( 'NONE',  ( -0.6412295605840000468, 1451.094351508330192, 182.3047427481980094 ) ) ;
#63260=CARTESIAN_POINT ( 'NONE',  ( 3.462090701198914822, 1432.317094223078811, 156.5315814253846156 ) ) ;
#63262=ORIENTED_EDGE ( 'NONE', *, *, #59272, .F. ) ;
#63267=CARTESIAN_POINT ( 'NONE',  ( 11.56380544704854962, 1426.103149140334381, 138.8483449811455159 ) ) ;
#63271=CYLINDRICAL_SURFACE ( 'NONE', #20929, 0.5000000000000005551 ) ;
#63272=CARTESIAN_POINT ( 'NONE',  ( 9.760933975314660671, 1409.253919710149830, 220.4514879604030000 ) ) ;
#63275=CARTESIAN_POINT ( 'NONE',  ( -19.38280343810000161, 1485.637741855729928, 189.8313757130979980 ) ) ;
#63276=CARTESIAN_POINT ( 'NONE',  ( 10.96892109620000078, 1432.312127152960102, 151.7701099976980004 ) ) ;
#63278=EDGE_LOOP ( 'NONE', ( #80458, #87627, #96297, #58620, #109876 ) ) ;
#63281=CARTESIAN_POINT ( 'NONE',  ( -12.06130973530630079, 1415.890045859420070, 194.8674313123640047 ) ) ;
#63284=CARTESIAN_POINT ( 'NONE',  ( 35.04437474502410055, 1457.726427851593144, 269.5321128390857552 ) ) ;
#63285=DIRECTION ( 'NONE',  ( -0.7067700363769180427, 0.03085824620774344287, -0.7067700363772875249 ) ) ;
#63287=CARTESIAN_POINT ( 'NONE',  ( 22.15347900851059748, 1496.414301113179818, 209.7169039519030207 ) ) ;
#63288=CARTESIAN_POINT ( 'NONE',  ( 0.2167502149440000137, 1453.575579519030043, 183.2287056930980214 ) ) ;
#63290=CARTESIAN_POINT ( 'NONE',  ( 0.3740406207303079711, 1452.976564550639978, 183.2744760995269928 ) ) ;
#63294=CARTESIAN_POINT ( 'NONE',  ( 1.121465680670000076, 1416.819759739430083, 190.1591349339979899 ) ) ;
#63297=CARTESIAN_POINT ( 'NONE',  ( 41.36548120546149931, 1444.128165951429992, 136.5310689808069924 ) ) ;
#63298=ORIENTED_EDGE ( 'NONE', *, *, #66255, .T. ) ;
#63299=CARTESIAN_POINT ( 'NONE',  ( 42.46017295210000242, 1427.243201938829998, 266.3334799472979739 ) ) ;
#63300=CARTESIAN_POINT ( 'NONE',  ( -19.72588041030000028, 1469.237837320530161, 193.2706619289980097 ) ) ;
#63301=FACE_OUTER_BOUND ( 'NONE', #65039, .T. ) ;
#63302=CARTESIAN_POINT ( 'NONE',  ( -17.22540132880000030, 1409.514584658930062, 195.8673741195979687 ) ) ;
#63303=CARTESIAN_POINT ( 'NONE',  ( 20.58544670569870760, 1506.578946199305392, 201.0686405472372087 ) ) ;
#63304=CARTESIAN_POINT ( 'NONE',  ( -31.44036050960000139, 1425.375771789929786, 254.7811623578979834 ) ) ;
#63308=CARTESIAN_POINT ( 'NONE',  ( -22.81026925195165944, 1409.709605436964466, 208.9207937587944741 ) ) ;
#63309=ORIENTED_EDGE ( 'NONE', *, *, #61635, .F. ) ;
#63315=EDGE_LOOP ( 'NONE', ( #48628, #15616, #79990, #51586 ) ) ;
#63319=ORIENTED_EDGE ( 'NONE', *, *, #57615, .T. ) ;
#63320=CARTESIAN_POINT ( 'NONE',  ( -0.7235648542570000119, 1417.479220455729774, 184.8026998982980160 ) ) ;
#63324=CARTESIAN_POINT ( 'NONE',  ( -0.2559295722590000377, 1479.777904972630040, 236.1640397496979915 ) ) ;
#63325=CARTESIAN_POINT ( 'NONE',  ( 5.389719913101400195, 1440.971386073809981, 154.8246291173960003 ) ) ;
#63327=CARTESIAN_POINT ( 'NONE',  ( 46.16774997373190104, 1440.912967117140170, 266.9713874478409821 ) ) ;
#63328=CARTESIAN_POINT ( 'NONE',  ( -13.15726442949999964, 1415.948532225030021, 221.7037513481980113 ) ) ;
#63329=CARTESIAN_POINT ( 'NONE',  ( 15.44132444849999786, 1507.624369749529933, 226.1399349509979970 ) ) ;
#63330=ORIENTED_EDGE ( 'NONE', *, *, #89921, .F. ) ;
#63333=CARTESIAN_POINT ( 'NONE',  ( 11.83960237644440028, 1430.521195547569960, 149.6755224652310119 ) ) ;
#63334=CARTESIAN_POINT ( 'NONE',  ( 12.90355812175348404, 1444.932587894390736, 186.7378586203405462 ) ) ;
#63336=ORIENTED_EDGE ( 'NONE', *, *, #84985, .T. ) ;
#63339=CARTESIAN_POINT ( 'NONE',  ( -22.57962297529999773, 1409.701558196430142, 208.4161775753709946 ) ) ;
#63341=CARTESIAN_POINT ( 'NONE',  ( 19.88079262212649923, 1452.218807810889984, 143.3936228603050154 ) ) ;
#63348=CARTESIAN_POINT ( 'NONE',  ( 0.02218773269636665699, 1410.258021740021150, 233.2201378621269896 ) ) ;
#63356=CARTESIAN_POINT ( 'NONE',  ( 20.63825565839999854, 1425.387366209430184, 248.0989693021979861 ) ) ;
#63360=B_SPLINE_SURFACE_WITH_KNOTS ( 'NONE', 5, 5, ( 
 ( #70535, #71089, #28502, #62699, #77613, #16558 ),
 ( #59717, #26076, #94964, #86005, #61391, #85434 ),
 ( #69791, #84887, #59176, #51868, #60838, #102783 ),
 ( #42347, #93296, #35599, #34501, #93834, #50750 ),
 ( #60268, #94387, #924, #101679, #8180, #76502 ),
 ( #27210, #18233, #110651, #95511, #77070, #78154 ),
 ( #69227, #52428, #103910, #18781, #43468, #8732 ),
 ( #44018, #33941, #86554, #68136, #102248, #110105 ),
 ( #17667, #52979, #25527, #9304, #87111, #10401 ),
 ( #68678, #1463, #35048, #9849, #103338, #42914 ),
 ( #75953, #33378, #67574, #24968, #17106, #51297 ),
 ( #380, #26641, #97167, #89868, #87681, #20989 ) ),
 .UNSPECIFIED., .F., .F., .F.,
 ( 6, 3, 3, 6 ),
 ( 6, 6 ),
 ( 52.58344481930000569, 57.38609284729999871, 62.18874087540000062, 65.18198166130000004 ),
 ( 0.000000000000000000, 2.000000000000000000 ),
 .UNSPECIFIED. ) ;
#63364=CARTESIAN_POINT ( 'NONE',  ( 30.48816909598289726, 1414.062251626520037, 269.3695147698609844 ) ) ;
#63368=B_SPLINE_CURVE_WITH_KNOTS ( 'NONE', 3,
 ( #104084, #68861, #11683, #26264, #27379, #52601, #96804, #26830, #87294, #61015, #62119, #36327, #95693, #95142, #18959, #9475, #53155, #10588, #60451, #78340, #44759, #62682, #104639, #11150, #27936, #53725, #54268, #45860, #96246, #94571, #17843, #77791, #18403, #1100, #86737, #35228, #10027, #81084, #31233, #63762 ),
 .UNSPECIFIED., .F., .F.,
 ( 4, 3, 3, 3, 3, 3, 3, 3, 3, 3, 3, 3, 3, 4 ),
 ( -1.435063413027759971, -1.364066038576970064, -1.253444982554889897, -1.141100129978610100, -1.027733815200259970, -0.9128813494742499257, -0.7973539268154259396, -0.6814611664271418290, -0.5655430835226159525, -0.4502876605942469634, -0.3358911414603549250, -0.2226055258251640190, -0.1106062959119480382, -2.220446049250313081E-16 ),
 .UNSPECIFIED. ) ;
#63369=CARTESIAN_POINT ( 'NONE',  ( -24.23120024909999870, 1444.178062262649973, 211.3705830899779983 ) ) ;
#63370=CARTESIAN_POINT ( 'NONE',  ( -2.096033132107356423, 1450.108388725817122, 154.3469607748115493 ) ) ;
#63374=CARTESIAN_POINT ( 'NONE',  ( 27.41738420279390098, 1509.883512505909948, 222.6174317186479925 ) ) ;
#63376=CARTESIAN_POINT ( 'NONE',  ( 12.80306059919530171, 1434.672636252922302, 149.2816584392911352 ) ) ;
#63377=CARTESIAN_POINT ( 'NONE',  ( 2.927772224839999993, 1417.416557252929806, 231.9440355153979851 ) ) ;
#63381=CARTESIAN_POINT ( 'NONE',  ( 45.88375197359999902, 1438.918372143629995, 266.4124103407979760 ) ) ;
#63382=CARTESIAN_POINT ( 'NONE',  ( -18.71691417810000146, 1410.062790051930051, 223.0812584992980021 ) ) ;
#63383=CARTESIAN_POINT ( 'NONE',  ( 23.46567568339999710, 1436.545700739849963, 140.9406085994980060 ) ) ;
#63384=CARTESIAN_POINT ( 'NONE',  ( 23.63314310590000034, 1508.007761069829940, 195.0461405673979982 ) ) ;
#63385=CARTESIAN_POINT ( 'NONE',  ( 21.88687337236331487, 1430.321363104666261, 220.0073771757959378 ) ) ;
#63387=CARTESIAN_POINT ( 'NONE',  ( -2.102271589710000388, 1475.801440029330024, 266.9594147012980443 ) ) ;
#63389=CARTESIAN_POINT ( 'NONE',  ( -34.87346161656260080, 1436.196920817200180, 136.2719409395089940 ) ) ;
#63391=CARTESIAN_POINT ( 'NONE',  ( -14.63963062230000034, 1409.365349618529990, 210.6960423599879846 ) ) ;
#63395=CARTESIAN_POINT ( 'NONE',  ( 11.87587044680000048, 1433.006446481710100, 146.7587676086979798 ) ) ;
#63396=CARTESIAN_POINT ( 'NONE',  ( -35.12295699405159866, 1435.816162438429956, 134.0999999976959884 ) ) ;
#63397=DIRECTION ( 'NONE',  ( -0.9211327884476211425, -0.3892484888175031799, 0.000000000000000000 ) ) ;
#63399=CARTESIAN_POINT ( 'NONE',  ( 5.511665417999469900E-05, 1508.970066526555001, 238.8757070596369942 ) ) ;
#63400=CARTESIAN_POINT ( 'NONE',  ( -3.860068541672339926, 1409.047856951109907, 223.5979342058130044 ) ) ;
#63405=CARTESIAN_POINT ( 'NONE',  ( -30.12637356810000355, 1467.407322974130011, 268.6828795483979775 ) ) ;
#63408=CARTESIAN_POINT ( 'NONE',  ( -26.19919347095130036, 1509.827956409970056, 209.1562360456119904 ) ) ;
#63412=CARTESIAN_POINT ( 'NONE',  ( 15.10946924899999999, 1415.087745006229852, 217.0735260779379701 ) ) ;
#63413=CARTESIAN_POINT ( 'NONE',  ( 1.110223024630000146E-16, 1435.943783413959864, 155.5249316174979981 ) ) ;
#63422=CARTESIAN_POINT ( 'NONE',  ( 23.62603012550000159, 1410.659706541129935, 211.3817606496579913 ) ) ;
#63425=CARTESIAN_POINT ( 'NONE',  ( -5.359903627183280506, 1422.348471699870061, 145.8522681477809897 ) ) ;
#63426=CARTESIAN_POINT ( 'NONE',  ( 11.90000415720300175, 1434.913060496859998, 147.6452464505769910 ) ) ;
#63432=AXIS2_PLACEMENT_3D ( 'NONE', #15370, #7537, #50111 ) ;
#63433=CARTESIAN_POINT ( 'NONE',  ( -1.153787697646769805, 1420.825136633349985, 183.6905923417640167 ) ) ;
#63435=CARTESIAN_POINT ( 'NONE',  ( -18.48452897440000342, 1425.095849964330000, 227.3281627736979829 ) ) ;
#63436=CARTESIAN_POINT ( 'NONE',  ( -18.68115160533190178, 1485.891698176000091, 189.2421416268200005 ) ) ;
#63438=CARTESIAN_POINT ( 'NONE',  ( -4.280709431791439812, 1440.997461520010120, 156.3948438198679867 ) ) ;
#63443=CARTESIAN_POINT ( 'NONE',  ( 29.71730764810000025, 1509.987350273330094, 210.0545273362199907 ) ) ;
#63444=ORIENTED_EDGE ( 'NONE', *, *, #36136, .T. ) ;
#63447=CARTESIAN_POINT ( 'NONE',  ( 15.68557540059999766, 1410.853897593529837, 191.5168599455980143 ) ) ;
#63448=CARTESIAN_POINT ( 'NONE',  ( 23.99815499239999994, 1446.810867530319911, 216.6209177652979747 ) ) ;
#63449=CARTESIAN_POINT ( 'NONE',  ( 5.386185205460879644, 1432.347042709529887, 154.6076275981190236 ) ) ;
#63450=CARTESIAN_POINT ( 'NONE',  ( -25.79081092570330114, 1450.963662666099935, 136.8144486713130163 ) ) ;
#63452=CARTESIAN_POINT ( 'NONE',  ( 4.388734291479999605, 1410.444832901329846, 231.4150274050980158 ) ) ;
#63456=CARTESIAN_POINT ( 'NONE',  ( 41.02967923190390565, 1440.575676734689978, 134.0999999980680002 ) ) ;
#63458=ORIENTED_EDGE ( 'NONE', *, *, #46825, .F. ) ;
#63462=ORIENTED_EDGE ( 'NONE', *, *, #78836, .T. ) ;
#63463=ORIENTED_EDGE ( 'NONE', *, *, #9459, .F. ) ;
#63466=CARTESIAN_POINT ( 'NONE',  ( 7.876852879565064747, 1451.393553377243506, 152.9815231998884428 ) ) ;
#63467=CARTESIAN_POINT ( 'NONE',  ( 1.705087066220000169, 1507.082462650630077, 236.5153987699980007 ) ) ;
#63473=ADVANCED_FACE ( 'NONE', ( #75566 ), #519, .F. ) ;
#63474=CARTESIAN_POINT ( 'NONE',  ( -0.7347961819880001189, 1487.759023923330005, 231.0371655964979709 ) ) ;
#63475=CARTESIAN_POINT ( 'NONE',  ( 6.288099950509999481, 1416.823872462129884, 191.8704827068980308 ) ) ;
#63481=CARTESIAN_POINT ( 'NONE',  ( 27.65997673997260264, 1440.913060387330006, 246.7466754288900006 ) ) ;
#63482=CARTESIAN_POINT ( 'NONE',  ( -15.17209163809999950, 1508.688025133729980, 184.8363905680980110 ) ) ;
#63485=CARTESIAN_POINT ( 'NONE',  ( -14.27950570660000018, 1410.344120410830101, 190.3743234292979878 ) ) ;
#63487=CARTESIAN_POINT ( 'NONE',  ( -24.67319088250000192, 1441.246434465200082, 210.6951902311179765 ) ) ;
#63490=CARTESIAN_POINT ( 'NONE',  ( 0.2153512683669999983, 1405.989301470729970, 266.9611412585979906 ) ) ;
#63493=CARTESIAN_POINT ( 'NONE',  ( 4.509664962759999618, 1465.693492029729896, 233.9834801382980061 ) ) ;
#63499=DIRECTION ( 'NONE',  ( 0.000000000000000000, 0.000000000000000000, -1.000000000000000000 ) ) ;
#63500=CARTESIAN_POINT ( 'NONE',  ( 18.27523319681197833, 1446.550731797170101, 215.9569883731650748 ) ) ;
#63502=CARTESIAN_POINT ( 'NONE',  ( -21.99590692660000002, 1506.811133727630022, 209.5040961443579874 ) ) ;
#63503=( BOUNDED_CURVE ( )  B_SPLINE_CURVE ( 3, ( #94163, #17433, #43236, #68447 ),
 .UNSPECIFIED., .F., .F. ) 
 B_SPLINE_CURVE_WITH_KNOTS ( ( 4, 4 ),
 ( 1.036305746500566061, 2.105308905912994799 ),
 .UNSPECIFIED. ) 
 CURVE ( )  GEOMETRIC_REPRESENTATION_ITEM ( )  RATIONAL_B_SPLINE_CURVE ( ( 1.000000000000000000, 0.9070150916864841983, 0.9070150916864841983, 1.000000000000000000 ) ) 
 REPRESENTATION_ITEM ( '' )  );
#63504=ADVANCED_FACE ( 'NONE', ( #76645 ), #59111, .T. ) ;
#63508=CARTESIAN_POINT ( 'NONE',  ( -18.46505095605026270, 1509.557874174373865, 231.0973782675585255 ) ) ;
#63509=CARTESIAN_POINT ( 'NONE',  ( 18.33597341320000140, 1458.591204236030080, 232.0308503239980098 ) ) ;
#63512=CARTESIAN_POINT ( 'NONE',  ( -1.480417309695410077, 1508.374054581489872, 237.5951421557219874 ) ) ;
#63516=CARTESIAN_POINT ( 'NONE',  ( -20.81941094909999990, 1457.442873729829898, 223.8287928082980045 ) ) ;
#63517=CARTESIAN_POINT ( 'NONE',  ( 2.500000000000000000, 1419.365153366229833, 145.1079871556979981 ) ) ;
#63520=ORIENTED_EDGE ( 'NONE', *, *, #103593, .T. ) ;
#63522=CARTESIAN_POINT ( 'NONE',  ( 2.086239376750000041, 1406.540766230330064, 269.4971845159980148 ) ) ;
#63525=CARTESIAN_POINT ( 'NONE',  ( 6.625222801663490202, 1473.589452326439869, 270.3925718229160111 ) ) ;
#63526=DIRECTION ( 'NONE',  ( -0.5600256381126521577, -0.8284752770339720573, 0.000000000000000000 ) ) ;
#63527=CARTESIAN_POINT ( 'NONE',  ( 10.23376715243824897, 1422.709367747187798, 137.1241318772909779 ) ) ;
#63530=DIRECTION ( 'NONE',  ( -0.04448252661992505713, -0.9990097882110241523, -0.0008648029096898162240 ) ) ;
#63532=CARTESIAN_POINT ( 'NONE',  ( 14.38276615817169635, 1509.537722092532931, 235.4493228184925897 ) ) ;
#63533=CARTESIAN_POINT ( 'NONE',  ( -14.02570581375069914, 1415.492117401580117, 220.9500074586500205 ) ) ;
#63535=ORIENTED_EDGE ( 'NONE', *, *, #100623, .T. ) ;
#63536=CARTESIAN_POINT ( 'NONE',  ( -17.26713005559999914, 1428.027535766330175, 234.3916895593979746 ) ) ;
#63538=CARTESIAN_POINT ( 'NONE',  ( -0.7691164859940000653, 1475.314785482929892, 269.4984833451979966 ) ) ;
#63541=CARTESIAN_POINT ( 'NONE',  ( -3.089550218706188733, 1448.274272998623474, 184.5587172890779186 ) ) ;
#63545=CARTESIAN_POINT ( 'NONE',  ( 26.79919712355280126, 1436.600546571140057, 136.7629453747840103 ) ) ;
#63547=CARTESIAN_POINT ( 'NONE',  ( -10.11703718938549912, 1396.266355110979930, 213.6078271767569845 ) ) ;
#63548=CARTESIAN_POINT ( 'NONE',  ( -15.03157878520000068, 1422.458659762129855, 229.1221048155979929 ) ) ;
#63549=CARTESIAN_POINT ( 'NONE',  ( -44.92382433299999889, 1440.723416683769983, 269.6913831256979961 ) ) ;
#63551=CARTESIAN_POINT ( 'NONE',  ( -16.81223434880759982, 1414.913060387349788, 207.5743820648510223 ) ) ;
#63552=CARTESIAN_POINT ( 'NONE',  ( 2.923263585169999956, 1409.521015940530106, 231.4220185117980009 ) ) ;
#63555=CARTESIAN_POINT ( 'NONE',  ( 10.35419722570000012, 1425.138650036730041, 115.7291061860980079 ) ) ;
#63557=CARTESIAN_POINT ( 'NONE',  ( -16.14705515586277329, 1409.476923469505209, 225.0742284443501546 ) ) ;
#63558=CARTESIAN_POINT ( 'NONE',  ( 4.268211237764689692, 1423.922164383429845, 183.9128890805280037 ) ) ;
#63561=CARTESIAN_POINT ( 'NONE',  ( -2.446787376320000096, 1432.353341358199941, 150.2884730787980061 ) ) ;
#63562=CARTESIAN_POINT ( 'NONE',  ( 1.454856650950000052, 1507.661996469930045, 181.0451578312979848 ) ) ;
#63563=PLANE ( 'NONE',  #88338 ) ;
#63569=CARTESIAN_POINT ( 'NONE',  ( -8.264168053159998806, 1396.728728318830008, 199.4337832187279957 ) ) ;
#63570=CARTESIAN_POINT ( 'NONE',  ( 0.4780929317929359934, 1499.039778920739991, 237.0126458204609889 ) ) ;
#63571=CARTESIAN_POINT ( 'NONE',  ( -16.53869145193961288, 1435.074985393188399, 146.6152319182869803 ) ) ;
#63576=CARTESIAN_POINT ( 'NONE',  ( 3.363175565480000184, 1429.769277944529904, 184.9623219864980115 ) ) ;
#63579=CARTESIAN_POINT ( 'NONE',  ( 40.09012238588890398, 1439.133113879990105, 136.1039124235030044 ) ) ;
#63581=CARTESIAN_POINT ( 'NONE',  ( -40.41548887560000480, 1443.621016936120213, 137.1123791864980035 ) ) ;
#63582=CARTESIAN_POINT ( 'NONE',  ( -6.075257814475249596, 1406.559263763209856, 269.2809304965529691 ) ) ;
#63583=CARTESIAN_POINT ( 'NONE',  ( 41.66135186410000557, 1443.796891309130160, 135.6885248007979783 ) ) ;
#63586=CARTESIAN_POINT ( 'NONE',  ( 11.91277487560000026, 1442.215011169370200, 187.5867736087979836 ) ) ;
#63589=DIRECTION ( 'NONE',  ( -0.9993779840598802089, -0.0009463129492438572803, -0.03525265193161980504 ) ) ;
#63590=CARTESIAN_POINT ( 'NONE',  ( -13.63106836819999934, 1462.228096604230132, 230.1036610636979844 ) ) ;
#63593=ORIENTED_EDGE ( 'NONE', *, *, #79156, .F. ) ;
#63594=CARTESIAN_POINT ( 'NONE',  ( -14.35118438041689970, 1509.480705576550008, 182.9751542011199774 ) ) ;
#63596=EDGE_CURVE ( 'NONE', #41404, #6924, #22634, .T. ) ;
#63598=CARTESIAN_POINT ( 'NONE',  ( 18.81809407629999953, 1416.219761279530076, 210.6452591561279917 ) ) ;
#63602=B_SPLINE_SURFACE_WITH_KNOTS ( 'NONE', 5, 4, ( 
 ( #64252, #59695, #51848, #41776, #101656 ),
 ( #94365, #50203, #76481, #16000, #24944 ),
 ( #93275, #84328, #110633, #68657, #75404 ),
 ( #33361, #67001, #34482, #355, #67554 ),
 ( #8160, #92182, #25505, #42891, #17647 ),
 ( #85985, #35026, #68113, #9283, #33918 ) ),
 .UNSPECIFIED., .F., .F., .F.,
 ( 6, 6 ),
 ( 5, 5 ),
 ( 0.000000000000000000, 111.1101480259999903 ),
 ( 25.81581217359999769, 39.03307591160000101 ),
 .UNSPECIFIED. ) ;
#63603=CARTESIAN_POINT ( 'NONE',  ( 11.06154325740661015, 1433.015924775765143, 151.7088343760975704 ) ) ;
#63604=CARTESIAN_POINT ( 'NONE',  ( -3.069376825600000025, 1409.187778979130144, 231.9248983289979833 ) ) ;
#63605=CARTESIAN_POINT ( 'NONE',  ( -7.326859461719999800, 1453.313060387329870, 190.4665504513979783 ) ) ;
#63607=CARTESIAN_POINT ( 'NONE',  ( -13.85778478534841263, 1434.981447914178034, 148.6210686895626054 ) ) ;
#63612=CARTESIAN_POINT ( 'NONE',  ( 25.61285747430000015, 1414.331920139429940, 270.3573890238980084 ) ) ;
#63615=CARTESIAN_POINT ( 'NONE',  ( 23.43132253519999963, 1410.390761240029860, 207.9091969211580135 ) ) ;
#63616=CARTESIAN_POINT ( 'NONE',  ( 0.008003304918488279504, 1508.487575044294545, 237.9830183513317365 ) ) ;
#63622=CARTESIAN_POINT ( 'NONE',  ( 4.185430511625449768, 1421.177391087800061, 185.2742621543330017 ) ) ;
#63623=CARTESIAN_POINT ( 'NONE',  ( -1.332234214539999906, 1417.916672854830040, 233.3009772848979821 ) ) ;
#63625=ORIENTED_EDGE ( 'NONE', *, *, #94010, .F. ) ;
#63631=CARTESIAN_POINT ( 'NONE',  ( -11.60004869885203682, 1411.254281879943164, 135.5999999980979851 ) ) ;
#63633=CARTESIAN_POINT ( 'NONE',  ( 0.02358223654491949789, 1420.444546422549820, 182.6733859946079974 ) ) ;
#63636=CARTESIAN_POINT ( 'NONE',  ( 19.34325791780000259, 1509.569025932029945, 187.1036586203979937 ) ) ;
#63642=CARTESIAN_POINT ( 'NONE',  ( 0.08925506140130000376, 1497.012273211330012, 230.7310177360980106 ) ) ;
#63646=CARTESIAN_POINT ( 'NONE',  ( -26.43747909245940164, 1508.499208940789913, 201.5081742940070058 ) ) ;
#63647=CARTESIAN_POINT ( 'NONE',  ( -2.710413728979999881, 1447.398499818599930, 159.5173236502980103 ) ) ;
#63648=CARTESIAN_POINT ( 'NONE',  ( -18.43681981810000181, 1425.072882130230028, 225.4380530597979941 ) ) ;
#63649=CARTESIAN_POINT ( 'NONE',  ( -18.81929060680000276, 1436.388221856100245, 146.6704585558979943 ) ) ;
#63650=CARTESIAN_POINT ( 'NONE',  ( 33.92643251289999995, 1451.728352207130001, 135.1493744902979870 ) ) ;
#63651=CARTESIAN_POINT ( 'NONE',  ( 17.04970435369999748, 1508.515036628130019, 187.9166768603979847 ) ) ;
#63652=CARTESIAN_POINT ( 'NONE',  ( 1.137641289866240024, 1410.327604111319943, 232.8584434023429992 ) ) ;
#63653=CARTESIAN_POINT ( 'NONE',  ( -18.67271768969374435, 1437.373477116879258, 211.9268211480253683 ) ) ;
#63655=ORIENTED_EDGE ( 'NONE', *, *, #61432, .T. ) ;
#63657=CARTESIAN_POINT ( 'NONE',  ( 11.90008666459999986, 1434.920851464509951, 147.6452002888979962 ) ) ;
#63662=CARTESIAN_POINT ( 'NONE',  ( 18.37215797060000000, 1453.313060387329870, 217.1322599118979895 ) ) ;
#63667=B_SPLINE_CURVE_WITH_KNOTS ( 'NONE', 3,
 ( #14385, #73215, #108466, #107359, #48579, #31749, #30655, #100058, #3836, #72674, #98949, #98404, #54777, #37964, #21676, #56422, #29549, #80519, #81054, #21123, #106263, #55328, #12194, #46387, #63735, #4368, #38497, #55882, #13829, #48016, #82153, #67585, #16034, #77083, #8192, #7652, #42358, #102259, #16569, #23345, #83810, #75437, #58078 ),
 .UNSPECIFIED., .F., .F.,
 ( 4, 3, 3, 3, 3, 3, 3, 3, 3, 3, 3, 3, 3, 3, 4 ),
 ( -8.338949519795640697, -8.327257911908940713, -8.213231001270830944, -8.087512482746008757, -7.836075445696390140, -7.703760222490700471, -7.408891911687140563, -7.099196593615670459, -6.815814698362330226, -6.550724326761839578, -6.491399922859719673, -6.353894249153509755, -6.157064171545170161, -6.019682015367260774, -5.901461776375070301 ),
 .UNSPECIFIED. ) ;
#63673=ORIENTED_EDGE ( 'NONE', *, *, #105531, .T. ) ;
#63678=ORIENTED_EDGE ( 'NONE', *, *, #82224, .F. ) ;
#63679=CARTESIAN_POINT ( 'NONE',  ( 17.94598849933589690, 1415.434635989099888, 209.7830392791789791 ) ) ;
#63682=CARTESIAN_POINT ( 'NONE',  ( 32.04160921650328930, 1421.195714791004548, 269.4938129757199476 ) ) ;
#63683=CARTESIAN_POINT ( 'NONE',  ( -29.63060422040000219, 1444.770720791339954, 238.0637335945980055 ) ) ;
#63684=CARTESIAN_POINT ( 'NONE',  ( -19.88543994140000137, 1484.719660939830192, 190.7434707760979791 ) ) ;
#63685=CARTESIAN_POINT ( 'NONE',  ( -11.71863204979999828, 1433.641944146899959, 150.9519096011979684 ) ) ;
#63686=CARTESIAN_POINT ( 'NONE',  ( 26.71146732620000108, 1509.845845380629953, 197.1819887268980267 ) ) ;
#63687=CARTESIAN_POINT ( 'NONE',  ( -19.52684841499999990, 1485.866921902229933, 190.0057045620980034 ) ) ;
#63689=CARTESIAN_POINT ( 'NONE',  ( 5.020440211750000437, 1420.408409142929941, 185.9185919516980334 ) ) ;
#63693=B_SPLINE_CURVE_WITH_KNOTS ( 'NONE', 3,
 ( #95407, #35490, #78043, #1923, #70247, #264, #69684 ),
 .UNSPECIFIED., .F., .F.,
 ( 4, 3, 4 ),
 ( -167.5289128729999959, -132.8626999427419833, -78.04659677155639486 ),
 .UNSPECIFIED. ) ;
#63695=CARTESIAN_POINT ( 'NONE',  ( -7.506254784382560023E-12, 1411.829882030230010, 254.0148294673659848 ) ) ;
#63699=VECTOR ( 'NONE', #60238, 1000.000000000000000 ) ;
#63701=CARTESIAN_POINT ( 'NONE',  ( -8.283412045740000451, 1473.335056111630138, 270.2796699741979864 ) ) ;
#63704=CARTESIAN_POINT ( 'NONE',  ( 38.16624314905799764, 1450.366968005889930, 135.2278820825040100 ) ) ;
#63705=CARTESIAN_POINT ( 'NONE',  ( 0.3657425961662950087, 1450.911939891260090, 181.4846316853029862 ) ) ;
#63706=CARTESIAN_POINT ( 'NONE',  ( -11.36250926159999963, 1420.040572322430080, 229.9329963247979833 ) ) ;
#63709=CARTESIAN_POINT ( 'NONE',  ( -1.465793917108519917, 1484.360957496709943, 182.4810413606819850 ) ) ;
#63711=CARTESIAN_POINT ( 'NONE',  ( -46.00814008725180315, 1437.084982451890028, 267.5989046568349750 ) ) ;
#63713=CARTESIAN_POINT ( 'NONE',  ( -3.535156810759120027, 1493.450694636509979, 181.5593925653629981 ) ) ;
#63715=VERTEX_POINT ( 'NONE', #9995 ) ;
#63717=DIRECTION ( 'NONE',  ( -0.03489949670247723124, 0.9993908270190966503, 2.775557561563011889E-14 ) ) ;
#63718=FACE_OUTER_BOUND ( 'NONE', #79694, .T. ) ;
#63719=CARTESIAN_POINT ( 'NONE',  ( -13.69820349629999967, 1410.401525690029985, 190.0660059053979865 ) ) ;
#63720=CARTESIAN_POINT ( 'NONE',  ( -16.42379639758739884, 1461.170146474039939, 228.2802429533950033 ) ) ;
#63721=ORIENTED_EDGE ( 'NONE', *, *, #75552, .F. ) ;
#63723=EDGE_CURVE ( 'NONE', #33631, #22102, #65534, .T. ) ;
#63727=CARTESIAN_POINT ( 'NONE',  ( -8.310284128760839550, 1410.978277515770060, 269.3433025615229894 ) ) ;
#63728=CARTESIAN_POINT ( 'NONE',  ( 1.077847364669999991E-15, 1428.043997280830126, 101.8807690336980016 ) ) ;
#63733=CARTESIAN_POINT ( 'NONE',  ( 44.22871283554869848, 1449.420066736412309, 269.0143090413143909 ) ) ;
#63735=CARTESIAN_POINT ( 'NONE',  ( -13.52034949347279991, 1436.166343023079889, 150.4953566056409784 ) ) ;
#63737=CARTESIAN_POINT ( 'NONE',  ( -17.74486107192629802, 1415.124054205860148, 207.5653927723479910 ) ) ;
#63738=CARTESIAN_POINT ( 'NONE',  ( -451.6393500377540136, 1435.141463851319713, 155.5900692994430017 ) ) ;
#63739=CARTESIAN_POINT ( 'NONE',  ( -13.79270780340000080, 1423.505142977830019, 222.1150309489979691 ) ) ;
#63740=CARTESIAN_POINT ( 'NONE',  ( 11.27186231780000014, 1414.983773854429955, 222.4323527839979988 ) ) ;
#63741=CARTESIAN_POINT ( 'NONE',  ( 7.356463438449999614, 1445.970468545179983, 184.4044459342979962 ) ) ;
#63743=EDGE_LOOP ( 'NONE', ( #72064, #89154, #32381, #61783 ) ) ;
#63745=CARTESIAN_POINT ( 'NONE',  ( -23.65802091397744178, 1447.576292128232353, 214.9099903041857544 ) ) ;
#63747=DIRECTION ( 'NONE',  ( 0.0003696129200224610584, 0.001489947240871160403, -0.9999988217210601382 ) ) ;
#63748=CARTESIAN_POINT ( 'NONE',  ( 11.60004869885203682, 1425.894332500278097, 137.5113157688821275 ) ) ;
#63750=CARTESIAN_POINT ( 'NONE',  ( 19.38627076359999890, 1409.590043883829821, 198.4190663087979942 ) ) ;
#63751=CARTESIAN_POINT ( 'NONE',  ( 20.12133088869999753, 1445.052233488290085, 161.1306464489979930 ) ) ;
#63752=CARTESIAN_POINT ( 'NONE',  ( -23.69915799640000031, 1435.325095724740095, 137.0907082570979867 ) ) ;
#63753=CARTESIAN_POINT ( 'NONE',  ( -23.55087667009999919, 1411.110693366829764, 210.4794020521279947 ) ) ;
#63761=CARTESIAN_POINT ( 'NONE',  ( -6.501109238009999736, 1473.833204323429982, 270.1283629013980203 ) ) ;
#63762=CARTESIAN_POINT ( 'NONE',  ( -0.2331143941452460122, 1408.921200921389982, 231.7611568498559791 ) ) ;
#63765=CARTESIAN_POINT ( 'NONE',  ( -39.76489443428390302, 1446.373445015949983, 136.7410265875109872 ) ) ;
#63767=CARTESIAN_POINT ( 'NONE',  ( 2.051044940784851889, 1417.316251708583195, 233.1624096844531095 ) ) ;
#63768=CARTESIAN_POINT ( 'NONE',  ( -2.900311661485640347, 1477.802570806589756, 183.6038988494130137 ) ) ;
#63770=CARTESIAN_POINT ( 'NONE',  ( -1.511827936991389842, 1475.041441224169830, 269.6439064326379480 ) ) ;
#63771=CARTESIAN_POINT ( 'NONE',  ( 31.38711126342669999, 1440.913060383769789, 242.4731588227919872 ) ) ;
#63772=CARTESIAN_POINT ( 'NONE',  ( -20.22596394560000022, 1508.016461165629835, 228.8175828582979818 ) ) ;
#63773=CIRCLE ( 'NONE', #38727, 7.975189853890007896 ) ;
#63777=CARTESIAN_POINT ( 'NONE',  ( -19.42349535385465131, 1485.589659117401425, 189.9324232024657135 ) ) ;
#63779=CARTESIAN_POINT ( 'NONE',  ( 2.897247639040000156, 1482.822904283830212, 234.8636011151980085 ) ) ;
#63781=CARTESIAN_POINT ( 'NONE',  ( -17.66471548549609949, 1420.877322952379927, 226.1084292698919853 ) ) ;
#63782=CARTESIAN_POINT ( 'NONE',  ( -15.36908788890000110, 1507.577581067430174, 231.3915608676979900 ) ) ;
#63787=CARTESIAN_POINT ( 'NONE',  ( 9.547743298340000351, 1407.913147213329921, 218.7935598638979968 ) ) ;
#63788=CARTESIAN_POINT ( 'NONE',  ( -11.89193436319930086, 1434.276600524120113, 147.6498533934650084 ) ) ;
#63789=CARTESIAN_POINT ( 'NONE',  ( 1.720386059670000023, 1465.121410839730061, 235.5820274437980117 ) ) ;
#63790=ADVANCED_FACE ( 'NONE', ( #107908 ), #82265, .T. ) ;
#63791=CARTESIAN_POINT ( 'NONE',  ( -5.519906363166400709, 1440.499855196290127, 154.7645174855159951 ) ) ;
#63793=CARTESIAN_POINT ( 'NONE',  ( -0.5431364122140001083, 1451.469100220230075, 182.8070713969979977 ) ) ;
#63796=CARTESIAN_POINT ( 'NONE',  ( -17.36791971707869919, 1414.972329067380088, 207.8825838234459980 ) ) ;
#63799=ORIENTED_EDGE ( 'NONE', *, *, #78695, .F. ) ;
#63800=EDGE_CURVE ( 'NONE', #43874, #95045, #75795, .T. ) ;
#63805=ADVANCED_FACE ( 'NONE', ( #86437 ), #98329, .F. ) ;
#63807=DIRECTION ( 'NONE',  ( 0.3363363969979655810, -0.9417419115949056119, 0.000000000000000000 ) ) ;
#63808=CARTESIAN_POINT ( 'NONE',  ( 14.43128343706390027, 1409.417011909710027, 205.2710633763729788 ) ) ;
#63812=DIRECTION ( 'NONE',  ( 0.8771707529291777883, 0.03063147767459039120, -0.4792005663405778937 ) ) ;
#63813=EDGE_CURVE ( 'NONE', #60488, #19532, #34772, .T. ) ;
#63817=ORIENTED_EDGE ( 'NONE', *, *, #99437, .F. ) ;
#63820=CARTESIAN_POINT ( 'NONE',  ( -12.26778636215339979, 1416.765224586759814, 194.6662842786359988 ) ) ;
#63821=( BOUNDED_CURVE ( )  B_SPLINE_CURVE ( 3, ( #65669, #38789, #89752, #57285 ),
 .UNSPECIFIED., .F., .F. ) 
 B_SPLINE_CURVE_WITH_KNOTS ( ( 4, 4 ),
 ( 4.233974059277724855, 5.191467434861920083 ),
 .UNSPECIFIED. ) 
 CURVE ( )  GEOMETRIC_REPRESENTATION_ITEM ( )  RATIONAL_B_SPLINE_CURVE ( ( 1.000000000000000000, 0.9250486529759208709, 0.9250486529759208709, 1.000000000000000000 ) ) 
 REPRESENTATION_ITEM ( '' )  );
#63823=CARTESIAN_POINT ( 'NONE',  ( 1.685908120830160076E-11, 1466.195288505810140, 242.1879250690809897 ) ) ;
#63824=CARTESIAN_POINT ( 'NONE',  ( -20.37857258470070221, 1500.692629429460112, 190.5974988396959873 ) ) ;
#63825=CARTESIAN_POINT ( 'NONE',  ( 6.232532001850000114, 1398.098440471829917, 220.5304192662980256 ) ) ;
#63828=CARTESIAN_POINT ( 'NONE',  ( 13.58268853708210067, 1416.851343896850040, 196.3340833727469885 ) ) ;
#63830=CARTESIAN_POINT ( 'NONE',  ( -22.28696231330000188, 1506.798305107829947, 208.8466800722590051 ) ) ;
#63831=CARTESIAN_POINT ( 'NONE',  ( -22.62861454470000311, 1507.212883763329955, 208.5231287359179930 ) ) ;
#63834=CARTESIAN_POINT ( 'NONE',  ( 11.39017366564850242, 1433.914938483480000, 151.4359183571540086 ) ) ;
#63835=CARTESIAN_POINT ( 'NONE',  ( -13.83305622877970009, 1436.229965305390124, 150.3316969671570007 ) ) ;
#63837=CARTESIAN_POINT ( 'NONE',  ( 18.59403002570000041, 1409.562378223829910, 197.6450396516979993 ) ) ;
#63842=CARTESIAN_POINT ( 'NONE',  ( 10.82132307049999831, 1413.960774641330090, 250.5360043972979440 ) ) ;
#63843=CARTESIAN_POINT ( 'NONE',  ( -26.14369035850000245, 1488.683671329329854, 203.4812363805280029 ) ) ;
#63844=CARTESIAN_POINT ( 'NONE',  ( -1.542474001980000065, 1502.014794158629911, 181.0193620746979946 ) ) ;
#63845=CARTESIAN_POINT ( 'NONE',  ( -17.67654380129999936, 1410.026337406529819, 195.1650949151980114 ) ) ;
#63847=CARTESIAN_POINT ( 'NONE',  ( 5.465011822930000053E-09, 1419.727281558630011, 225.2064029046980238 ) ) ;
#63850=CARTESIAN_POINT ( 'NONE',  ( 33.91369266730000476, 1450.440660192670066, 136.2454535554979884 ) ) ;
#63851=VERTEX_POINT ( 'NONE', #100350 ) ;
#63852=CARTESIAN_POINT ( 'NONE',  ( 7.620902379277350036, 1398.139480053939906, 197.4921199094770259 ) ) ;
#63855=ORIENTED_EDGE ( 'NONE', *, *, #16691, .T. ) ;
#63856=CARTESIAN_POINT ( 'NONE',  ( 2.897985082046180327, 1480.124455445799867, 234.7435789289370121 ) ) ;
#63857=CARTESIAN_POINT ( 'NONE',  ( -22.70984874270769893, 1409.706099204690190, 208.9686739919200136 ) ) ;
#63859=CARTESIAN_POINT ( 'NONE',  ( 0.08478249716650000656, 1419.321047202629870, 227.3343309334979949 ) ) ;
#63862=CARTESIAN_POINT ( 'NONE',  ( -3.371383657610000029, 1479.771743941129898, 235.5096298670979991 ) ) ;
#63865=VERTEX_POINT ( 'NONE', #107653 ) ;
#63866=CARTESIAN_POINT ( 'NONE',  ( 46.05252857291980462, 1440.912967510329963, 266.6768989187639818 ) ) ;
#63869=CARTESIAN_POINT ( 'NONE',  ( 0.4435022942679999747, 1418.672171181530075, 184.7048927422980000 ) ) ;
#63873=CARTESIAN_POINT ( 'NONE',  ( 13.08298364061185559, 1443.010872789425321, 187.3424311853700317 ) ) ;
#63878=CARTESIAN_POINT ( 'NONE',  ( -22.30007645030000063, 1409.691796216729927, 207.3274002725380285 ) ) ;
#63881=CARTESIAN_POINT ( 'NONE',  ( 21.69567490921269837, 1452.155430724869802, 140.9671523504339916 ) ) ;
#63886=CARTESIAN_POINT ( 'NONE',  ( 0.03589260184548991733, 1409.889651789088475, 233.1454190195690330 ) ) ;
#63887=CARTESIAN_POINT ( 'NONE',  ( -18.79435929301390118, 1476.960500850449762, 189.8610087135640185 ) ) ;
#63890=EDGE_CURVE ( 'NONE', #87917, #80584, #54826, .T. ) ;
#63891=CARTESIAN_POINT ( 'NONE',  ( -25.01122921334119908, 1509.595256063680154, 222.7800201234539941 ) ) ;
#63894=CARTESIAN_POINT ( 'NONE',  ( 26.42894384599999924, 1421.320559242730042, 262.6648722463980334 ) ) ;
#63895=CARTESIAN_POINT ( 'NONE',  ( 12.95221149940000060, 1434.756340029210151, 149.1862543735979898 ) ) ;
#63905=CARTESIAN_POINT ( 'NONE',  ( -13.58235848260000012, 1416.828044885930012, 221.9087532849979709 ) ) ;
#63908=CARTESIAN_POINT ( 'NONE',  ( 5.365940947776590697, 1422.323282697306922, 140.6189186885637525 ) ) ;
#63912=CARTESIAN_POINT ( 'NONE',  ( 15.73276775970000330, 1419.767728771030079, 227.5061845221979979 ) ) ;
#63916=CARTESIAN_POINT ( 'NONE',  ( 45.83772369860000140, 1436.897828481359966, 268.5019638271979829 ) ) ;
#63917=CARTESIAN_POINT ( 'NONE',  ( -17.65294392160000214, 1409.529514773629899, 223.4064738432979880 ) ) ;
#63918=CARTESIAN_POINT ( 'NONE',  ( 15.86562505229999864, 1435.238789513250140, 148.1955696700979956 ) ) ;
#63919=CARTESIAN_POINT ( 'NONE',  ( -0.7156054891749999980, 1424.187899035330020, 228.2423996515980207 ) ) ;
#63920=CARTESIAN_POINT ( 'NONE',  ( 5.385044978479859523, 1432.007840264780043, 154.5986929186840086 ) ) ;
#63921=CARTESIAN_POINT ( 'NONE',  ( -12.67256029850000054, 1474.517343106330145, 266.8981073570980129 ) ) ;
#63924=CARTESIAN_POINT ( 'NONE',  ( -38.69039280719189833, 1437.284833695140151, 135.5234525068720188 ) ) ;
#63925=CARTESIAN_POINT ( 'NONE',  ( 0.2160969567860719920, 1453.936780232339970, 183.2132073708449980 ) ) ;
#63926=CARTESIAN_POINT ( 'NONE',  ( -13.88567141579999920, 1409.397958718129985, 203.2213914723980110 ) ) ;
#63927=CARTESIAN_POINT ( 'NONE',  ( -11.49747567979999907, 1414.913060387329779, 197.9009878688979995 ) ) ;
#63931=CARTESIAN_POINT ( 'NONE',  ( -28.35296704552279934, 1509.521797104740017, 211.0041094760910028 ) ) ;
#63932=CARTESIAN_POINT ( 'NONE',  ( 13.80512448200000009, 1434.979588684790087, 149.6997163784980103 ) ) ;
#63933=CARTESIAN_POINT ( 'NONE',  ( -38.36650730484889493, 1437.217469519499900, 134.0999999970779868 ) ) ;
#63937=CARTESIAN_POINT ( 'NONE',  ( -8.740751882428300590, 1409.218294169019828, 221.2666971587190119 ) ) ;
#63944=CARTESIAN_POINT ( 'NONE',  ( -37.78661183750000419, 1461.804245060129915, 266.9502806207980257 ) ) ;
#63945=CARTESIAN_POINT ( 'NONE',  ( -2.500000000000000000, 1425.929641636930000, 172.2701767054979882 ) ) ;
#63947=CARTESIAN_POINT ( 'NONE',  ( -25.16173584180000233, 1509.119668852230234, 220.4671678159979820 ) ) ;
#63952=CARTESIAN_POINT ( 'NONE',  ( -27.03405935059999976, 1451.816840469730096, 135.7882905775979907 ) ) ;
#63960=CARTESIAN_POINT ( 'NONE',  ( -12.18103061950000132, 1415.553739809529816, 195.2061824783980342 ) ) ;
#63962=CARTESIAN_POINT ( 'NONE',  ( 22.84076229929999968, 1409.875136994729928, 212.1997148582279920 ) ) ;
#63965=CARTESIAN_POINT ( 'NONE',  ( -3.611923541125130033, 1508.978184271700002, 180.0004877964609875 ) ) ;
#63966=CARTESIAN_POINT ( 'NONE',  ( -11.87300260940000030, 1432.863468416260048, 150.3956790681980067 ) ) ;
#63968=CARTESIAN_POINT ( 'NONE',  ( 24.37269502358340034, 1430.523498792699911, 207.7385376608809793 ) ) ;
#63971=EDGE_CURVE ( 'NONE', #105306, #43307, #74854, .T. ) ;
#63972=CARTESIAN_POINT ( 'NONE',  ( -1.424810123350000124, 1415.524860511530051, 233.1780344959979914 ) ) ;
#63976=CARTESIAN_POINT ( 'NONE',  ( -4.340483865352609882, 1484.701310027739964, 183.4883394036949937 ) ) ;
#63977=ORIENTED_EDGE ( 'NONE', *, *, #91352, .T. ) ;
#63980=CARTESIAN_POINT ( 'NONE',  ( 18.88752285780000051, 1416.568813549730066, 210.6689649478780098 ) ) ;
#63985=CARTESIAN_POINT ( 'NONE',  ( 28.34445795850000138, 1509.155937278929969, 210.1751191034680062 ) ) ;
#63988=CARTESIAN_POINT ( 'NONE',  ( 1.556370308520000023, 1414.996442553730049, 191.7142053419979959 ) ) ;
#63989=CARTESIAN_POINT ( 'NONE',  ( 2.329729395510000245, 1427.373795049630189, 123.0297916884979941 ) ) ;
#63990=CARTESIAN_POINT ( 'NONE',  ( 24.55110742759999809, 1443.479132512090018, 214.0305984285579939 ) ) ;
#63992=CARTESIAN_POINT ( 'NONE',  ( -24.91466702467300109, 1452.043047651259940, 135.6639804502279958 ) ) ;
#63994=CARTESIAN_POINT ( 'NONE',  ( 7.280053280969999818, 1410.543619424229973, 230.7511305521980205 ) ) ;
#63997=CARTESIAN_POINT ( 'NONE',  ( 41.42406817588610579, 1441.754257787119741, 134.0999999980809889 ) ) ;
#63999=ORIENTED_EDGE ( 'NONE', *, *, #36144, .T. ) ;
#64007=CARTESIAN_POINT ( 'NONE',  ( 7.867369012536836514, 1451.393875050238648, 152.9843002031269350 ) ) ;
#64008=CIRCLE ( 'NONE', #106876, 1.999999954377493783 ) ;
#64010=CARTESIAN_POINT ( 'NONE',  ( -17.49148533773131931, 1448.272215950228656, 218.1393388027306059 ) ) ;
#64014=CARTESIAN_POINT ( 'NONE',  ( 10.26243806819999982, 1415.425644477329797, 194.9508951275979882 ) ) ;
#64016=ORIENTED_EDGE ( 'NONE', *, *, #43172, .T. ) ;
#64018=ORIENTED_EDGE ( 'NONE', *, *, #56320, .T. ) ;
#64019=CARTESIAN_POINT ( 'NONE',  ( 23.79195804607689624, 1440.913060387330006, 234.8714593546470155 ) ) ;
#64020=CARTESIAN_POINT ( 'NONE',  ( -0.002360575507425215300, 1451.791349640477847, 154.0466420352841794 ) ) ;
#64022=CARTESIAN_POINT ( 'NONE',  ( -0.2934977098714270372, 1451.161884857989889, 182.5468558900879827 ) ) ;
#64023=CARTESIAN_POINT ( 'NONE',  ( -16.00480266779999994, 1409.471960401030174, 192.4949821169979884 ) ) ;
#64025=CARTESIAN_POINT ( 'NONE',  ( -24.37563666778019922, 1439.900544325036890, 212.0182502291069682 ) ) ;
#64028=FACE_OUTER_BOUND ( 'NONE', #31172, .T. ) ;
#64029=CARTESIAN_POINT ( 'NONE',  ( -13.80599399759999990, 1434.979619872719923, 146.4346930356980181 ) ) ;
#64031=CARTESIAN_POINT ( 'NONE',  ( 4.523181926059999469, 1464.418891312029928, 235.2759163622980054 ) ) ;
#64032=DIRECTION ( 'NONE',  ( 1.000000000000000000, 7.763588443397869512E-10, 4.457073426249340046E-10 ) ) ;
#64035=CARTESIAN_POINT ( 'NONE',  ( 11.15490121449999883, 1425.160561550830153, 144.1688093938980160 ) ) ;
#64036=CARTESIAN_POINT ( 'NONE',  ( -0.1400231725758700196, 1507.707667440369960, 180.7851207917099998 ) ) ;
#64037=CARTESIAN_POINT ( 'NONE',  ( 19.16976238839742308, 1443.680783661108762, 213.5402241685004299 ) ) ;
#64044=CARTESIAN_POINT ( 'NONE',  ( 25.18985267180000065, 1440.913060401160010, 217.4969598257980010 ) ) ;
#64047=CARTESIAN_POINT ( 'NONE',  ( 1.984553072930000051, 1410.354529030129925, 232.0126999757980002 ) ) ;
#64049=AXIS2_PLACEMENT_3D ( 'NONE', #17167, #20920, #12541 ) ;
#64051=CARTESIAN_POINT ( 'NONE',  ( -22.30354652620000167, 1470.081838450430041, 222.1003071029979878 ) ) ;
#64052=CARTESIAN_POINT ( 'NONE',  ( 5.362073334248089296, 1423.991816925989951, 150.1582991024129967 ) ) ;
#64053=CARTESIAN_POINT ( 'NONE',  ( -1.570312491960000001, 1484.305737421829917, 182.5879718789979904 ) ) ;
#64056=AXIS2_PLACEMENT_3D ( 'NONE', #92552, #59531, #67943 ) ;
#64057=CARTESIAN_POINT ( 'NONE',  ( 2.107306259280000038, 1405.878280305930048, 267.2331469757979789 ) ) ;
#64059=AXIS2_PLACEMENT_3D ( 'NONE', #102558, #16343, #7419 ) ;
#64060=CARTESIAN_POINT ( 'NONE',  ( 20.81489508609670835, 1427.812437954155030, 220.0757061899427924 ) ) ;
#64066=CARTESIAN_POINT ( 'NONE',  ( -12.89832111469999987, 1444.960415658079910, 186.1351309691980020 ) ) ;
#64071=CARTESIAN_POINT ( 'NONE',  ( -21.37693747720000204, 1440.913060387330006, 224.8635562088979896 ) ) ;
#64072=FACE_OUTER_BOUND ( 'NONE', #9378, .T. ) ;
#64073=CARTESIAN_POINT ( 'NONE',  ( 4.276646838899999636, 1441.052817498070226, 157.0212001317980253 ) ) ;
#64074=CARTESIAN_POINT ( 'NONE',  ( -0.8892692271930000558, 1476.043852980030124, 268.4834379751979441 ) ) ;
#64077=DIRECTION ( 'NONE',  ( -0.9993902469236100039, -0.03489947644259129567, 0.001077449766195760121 ) ) ;
#64078=CARTESIAN_POINT ( 'NONE',  ( -2.884443514848614498, 1448.263804016322638, 184.3271468657659966 ) ) ;
#64084=CARTESIAN_POINT ( 'NONE',  ( 0.1681674884180490159, 1420.473121907760060, 182.7464979049940155 ) ) ;
#64085=CARTESIAN_POINT ( 'NONE',  ( -9.061987881421931235, 1396.229511977310040, 215.4630778420020079 ) ) ;
#64086=CARTESIAN_POINT ( 'NONE',  ( -15.35035202399999932, 1421.192170133330137, 227.1237052556980132 ) ) ;
#64087=CARTESIAN_POINT ( 'NONE',  ( 19.74164504280149757, 1455.376031929259852, 226.0788368184279875 ) ) ;
#64088=ORIENTED_EDGE ( 'NONE', *, *, #43476, .F. ) ;
#64090=CARTESIAN_POINT ( 'NONE',  ( 1.408975827199999920, 1408.962262904629824, 231.2047468183979788 ) ) ;
#64092=CARTESIAN_POINT ( 'NONE',  ( 11.51898438939999991, 1425.941348201630035, 135.9196790177979892 ) ) ;
#64094=CARTESIAN_POINT ( 'NONE',  ( -9859.020463813496463, 54.07981494722837823, 1360.877155230279641 ) ) ;
#64099=CARTESIAN_POINT ( 'NONE',  ( -2.431412526649999961, 1428.647745098929818, 149.4227846719979880 ) ) ;
#64100=CARTESIAN_POINT ( 'NONE',  ( 2.537844286819999517, 1508.894213628730085, 180.1480057510979975 ) ) ;
#64103=EDGE_CURVE ( 'NONE', #28737, #71735, #25215, .T. ) ;
#64108=CARTESIAN_POINT ( 'NONE',  ( -12.02002121700249937, 1447.120365805550136, 187.5076542713389927 ) ) ;
#64110=CARTESIAN_POINT ( 'NONE',  ( 2.688591569480000221, 1509.006950921329917, 238.2845073959980198 ) ) ;
#64111=CARTESIAN_POINT ( 'NONE',  ( -13.44670203181539492, 1444.308220740991374, 169.3633618578503217 ) ) ;
#64112=CARTESIAN_POINT ( 'NONE',  ( 7.713339349770000020, 1475.513060387329915, 228.7257818846979944 ) ) ;
#64115=CARTESIAN_POINT ( 'NONE',  ( -1.358297888627590044, 1411.672670050000079, 185.5471854834340206 ) ) ;
#64119=CARTESIAN_POINT ( 'NONE',  ( -39.13294756354380155, 1449.732214584349776, 134.8601900050019822 ) ) ;
#64120=CARTESIAN_POINT ( 'NONE',  ( 41.15111780865080249, 1443.645529726370114, 136.9181479281729992 ) ) ;
#64121=CARTESIAN_POINT ( 'NONE',  ( 8.582644122214238891, 1396.212772926450043, 216.0935766074430262 ) ) ;
#64122=CARTESIAN_POINT ( 'NONE',  ( -39.08794880019009810, 1436.812182271670054, 136.3558420284400086 ) ) ;
#64123=FACE_OUTER_BOUND ( 'NONE', #108631, .T. ) ;
#64128=ORIENTED_EDGE ( 'NONE', *, *, #96652, .T. ) ;
#64129=ORIENTED_EDGE ( 'NONE', *, *, #83766, .F. ) ;
#64130=CARTESIAN_POINT ( 'NONE',  ( -19.29280426250840108, 1478.092759466889902, 227.9528384731270023 ) ) ;
#64133=CARTESIAN_POINT ( 'NONE',  ( -13.92379579760000041, 1452.815214893629900, 195.1322242606980240 ) ) ;
#64134=CARTESIAN_POINT ( 'NONE',  ( 8.881784196999999612E-15, 1441.261220175949802, 126.8032249175980155 ) ) ;
#64138=ORIENTED_EDGE ( 'NONE', *, *, #60455, .T. ) ;
#64139=CARTESIAN_POINT ( 'NONE',  ( -11.60004869885202083, 1426.267714527815315, 138.3561744208223274 ) ) ;
#64140=CARTESIAN_POINT ( 'NONE',  ( 2.500000000000000000, 1448.712186460370049, 157.7132982831409720 ) ) ;
#64142=CIRCLE ( 'NONE', #22910, 10.00000000000000000 ) ;
#64144=CARTESIAN_POINT ( 'NONE',  ( 15.71890336570000102, 1414.913060387229962, 214.6699778313279978 ) ) ;
#64148=CARTESIAN_POINT ( 'NONE',  ( -36.69969584994223766, 1426.055895651937817, 269.5559544832055394 ) ) ;
#64149=CARTESIAN_POINT ( 'NONE',  ( -8.354921657429999371, 1410.136853626930133, 230.4734767913980136 ) ) ;
#64150=CARTESIAN_POINT ( 'NONE',  ( -13.22806383159999832, 1431.113060387329824, 194.5140223583980230 ) ) ;
#64152=CARTESIAN_POINT ( 'NONE',  ( -0.004457925198051789981, 1451.027869956220002, 181.9225055831719828 ) ) ;
#64153=CARTESIAN_POINT ( 'NONE',  ( -28.88351707065390173, 1440.913060387269979, 234.5452952734219991 ) ) ;
#64157=CARTESIAN_POINT ( 'NONE',  ( 25.02520634413389899, 1415.439183875560047, 270.1035392086070033 ) ) ;
#64160=CARTESIAN_POINT ( 'NONE',  ( 23.59717156689999840, 1410.840126738630033, 207.8450998541779882 ) ) ;
#64165=CARTESIAN_POINT ( 'NONE',  ( 4.218374993917859861, 1420.932961763340245, 185.4447900071560014 ) ) ;
#64166=CARTESIAN_POINT ( 'NONE',  ( -10.34676626709999780, 1420.438686667429920, 229.9603813012979856 ) ) ;
#64171=CARTESIAN_POINT ( 'NONE',  ( 0.5260898116900000199, 1417.366494600629949, 235.1724886678979942 ) ) ;
#64172=CARTESIAN_POINT ( 'NONE',  ( -21.39771622935050033, 1509.704956904690107, 229.7894228794980052 ) ) ;
#64180=VERTEX_POINT ( 'NONE', #28475 ) ;
#64184=CARTESIAN_POINT ( 'NONE',  ( 11.60004869885204215, 1426.320646328452540, 137.6121508069457207 ) ) ;
#64188=CARTESIAN_POINT ( 'NONE',  ( -26.40049011798170042, 1508.358675285229992, 201.5240040975259888 ) ) ;
#64189=CARTESIAN_POINT ( 'NONE',  ( -2.500000000000000000, 1448.210448412289907, 170.5244215879980061 ) ) ;
#64190=CARTESIAN_POINT ( 'NONE',  ( -20.35065116390000028, 1427.808792947530037, 223.1463981920979904 ) ) ;
#64193=CARTESIAN_POINT ( 'NONE',  ( 19.87072075760000089, 1498.082836619830005, 189.6522194475979859 ) ) ;
#64195=CARTESIAN_POINT ( 'NONE',  ( 29.75012120190000076, 1509.993914123429931, 209.6841247587719863 ) ) ;
#64203=CARTESIAN_POINT ( 'NONE',  ( -18.47399050599999626, 1509.320896585530136, 230.4813978294980075 ) ) ;
#64205=CARTESIAN_POINT ( 'NONE',  ( -13.25797267067026475, 1444.641804557892556, 186.6667489211167776 ) ) ;
#64206=CARTESIAN_POINT ( 'NONE',  ( -17.36801837519999836, 1414.983771848829747, 207.7378529488679817 ) ) ;
#64219=EDGE_CURVE ( 'NONE', #25603, #91513, #60540, .T. ) ;
#64222=CARTESIAN_POINT ( 'NONE',  ( 26.10691348580380122, 1471.192541839159958, 207.6971073565250094 ) ) ;
#64223=CARTESIAN_POINT ( 'NONE',  ( 13.53422276719999928, 1509.381727759229989, 234.4599784456980274 ) ) ;
#64225=CARTESIAN_POINT ( 'NONE',  ( 33.44398265167041728, 1422.464213849851376, 269.5109561759928738 ) ) ;
#64226=CARTESIAN_POINT ( 'NONE',  ( -34.48978217849999339, 1440.913060389249949, 250.0021841876980488 ) ) ;
#64227=CARTESIAN_POINT ( 'NONE',  ( -19.51711174489999934, 1484.705571712129768, 189.8616710270979979 ) ) ;
#64228=CARTESIAN_POINT ( 'NONE',  ( -11.80297485880000075, 1433.621679574930113, 150.7677425477979796 ) ) ;
#64230=CARTESIAN_POINT ( 'NONE',  ( -19.61483391129999987, 1485.816994056529893, 190.1275648953979953 ) ) ;
#64231=CIRCLE ( 'NONE', #39171, 2.000055272426020991 ) ;
#64240=CARTESIAN_POINT ( 'NONE',  ( 2.409488808553320245E-09, 1410.450358379310046, 257.5163489258059712 ) ) ;
#64241=ORIENTED_EDGE ( 'NONE', *, *, #69020, .T. ) ;
#64243=CARTESIAN_POINT ( 'NONE',  ( -11.86504885435570067, 1432.262511493439888, 149.9818936695930063 ) ) ;
#64245=CARTESIAN_POINT ( 'NONE',  ( -24.70945393470000084, 1465.793440313629844, 269.4189447651980345 ) ) ;
#64248=CARTESIAN_POINT ( 'NONE',  ( 33.92638623454369906, 1450.868589251249887, 136.1710234410380167 ) ) ;
#64249=CARTESIAN_POINT ( 'NONE',  ( 0.2603518607207219726, 1451.283950821710050, 182.4357641078530037 ) ) ;
#64252=CARTESIAN_POINT ( 'NONE',  ( -12.54268436849999979, 1408.913060387329779, 196.5791615931979948 ) ) ;
#64254=CARTESIAN_POINT ( 'NONE',  ( -33.48176124307740764, 1416.813162719589855, 268.8725262323869742 ) ) ;
#64255=ORIENTED_EDGE ( 'NONE', *, *, #105614, .F. ) ;
#64256=CARTESIAN_POINT ( 'NONE',  ( -3.533922947849859941, 1492.310067042970104, 181.6079149013590097 ) ) ;
#64260=CARTESIAN_POINT ( 'NONE',  ( 4.778748612485856029, 1423.572762554393194, 184.0460358434518469 ) ) ;
#64263=CARTESIAN_POINT ( 'NONE',  ( -4.345522541100000247, 1440.427655379589851, 185.4586955749979893 ) ) ;
#64266=B_SPLINE_SURFACE_WITH_KNOTS ( 'NONE', 5, 5, ( 
 ( #31639, #99937, #23232, #68035, #18141, #60744, #69135, #94866, #59620 ),
 ( #61305, #52338, #53442, #9214, #69702, #85909, #87587, #95971, #60178 ),
 ( #61852, #86460, #35509, #94295, #44478, #95423, #70261, #34406, #104369 ),
 ( #280, #10876, #17573, #93731, #27665, #19232, #25979, #9751, #45047 ),
 ( #52884, #79192, #17010, #34952, #10304, #1939, #43374, #51773, #25425 ),
 ( #33844, #87012, #77522, #822, #102144, #103239, #26550, #103821, #78624 ),
 ( #51209, #36076, #85339, #8636, #43917, #42811, #78063, #76971, #18686 ),
 ( #68579, #1366, #27120, #102683, #63512, #28214, #88689, #29861, #97630 ),
 ( #11968, #38260, #54555, #21980, #64601, #28773, #46152, #30412, #55097 ) ),
 .UNSPECIFIED., .F., .F., .F.,
 ( 6, 3, 6 ),
 ( 6, 3, 6 ),
 ( 51.29329440469999923, 55.70673016509999798, 65.19347039801400001 ),
 ( -8.782821396822089466E-05, 1.000000000000000000, 2.000000000000000000 ),
 .UNSPECIFIED. ) ;
#64267=ORIENTED_EDGE ( 'NONE', *, *, #55126, .F. ) ;
#64268=CARTESIAN_POINT ( 'NONE',  ( -26.79919838190000192, 1436.600005541920154, 136.7628791570980127 ) ) ;
#64273=CARTESIAN_POINT ( 'NONE',  ( 1.854736326702351557, 1508.995493199552357, 238.6295539663279612 ) ) ;
#64274=( BOUNDED_CURVE ( )  B_SPLINE_CURVE ( 3, ( #6584, #20205, #74908, #12357 ),
 .UNSPECIFIED., .F., .T. ) 
 B_SPLINE_CURVE_WITH_KNOTS ( ( 4, 4 ),
 ( 4.033485614218559334, 4.137218124529905339 ),
 .UNSPECIFIED. ) 
 CURVE ( )  GEOMETRIC_REPRESENTATION_ITEM ( )  RATIONAL_B_SPLINE_CURVE ( ( 1.000000000000000000, 0.9991034981929989289, 0.9991034981929989289, 1.000000000000000000 ) ) 
 REPRESENTATION_ITEM ( '' )  );
#64275=CARTESIAN_POINT ( 'NONE',  ( -26.64547680037770405, 1415.060613070530053, 270.3501199617340376 ) ) ;
#64276=CARTESIAN_POINT ( 'NONE',  ( -26.79413315976150045, 1435.433175095809929, 135.2874648155150226 ) ) ;
#64281=CARTESIAN_POINT ( 'NONE',  ( 34.06334320139256988, 1463.667877587127350, 269.2714786605345125 ) ) ;
#64283=CARTESIAN_POINT ( 'NONE',  ( -2.500000000000000000, 1419.383100980419840, 144.1003751433630100 ) ) ;
#64284=CARTESIAN_POINT ( 'NONE',  ( -1.326721101379999990, 1486.243302057330084, 181.7592321280980059 ) ) ;
#64287=CARTESIAN_POINT ( 'NONE',  ( -17.92173952435889817, 1415.219159633810023, 207.5658729395169928 ) ) ;
#64290=CARTESIAN_POINT ( 'NONE',  ( -14.51195731179999981, 1426.817867355729959, 222.0493599474980044 ) ) ;
#64291=CARTESIAN_POINT ( 'NONE',  ( 12.30733358380000020, 1416.021639799829927, 223.3557834255979913 ) ) ;
#64295=ORIENTED_EDGE ( 'NONE', *, *, #5680, .T. ) ;
#64297=CARTESIAN_POINT ( 'NONE',  ( -22.44240218647486529, 1451.734269296826824, 219.6387502286748088 ) ) ;
#64299=CARTESIAN_POINT ( 'NONE',  ( 0.3722769099684289928, 1457.826255237599980, 228.9731060096619899 ) ) ;
#64301=CARTESIAN_POINT ( 'NONE',  ( 13.22475641109999955, 1415.063410489729904, 197.5370647170979623 ) ) ;
#64303=CARTESIAN_POINT ( 'NONE',  ( 21.78252905899999803, 1409.837820636329980, 204.8395344835479932 ) ) ;
#64304=CARTESIAN_POINT ( 'NONE',  ( 28.06188869160000010, 1444.994950788469851, 168.7697867250980153 ) ) ;
#64305=CARTESIAN_POINT ( 'NONE',  ( 16.03391504160000025, 1409.472977038530189, 225.2054435686980014 ) ) ;
#64307=CARTESIAN_POINT ( 'NONE',  ( 2.398688105316478580, 1426.758990796949320, 141.3562649765487436 ) ) ;
#64308=CARTESIAN_POINT ( 'NONE',  ( 23.32143419377827698, 1449.605800993310140, 217.2891594252025982 ) ) ;
#64312=EDGE_LOOP ( 'NONE', ( #68516, #108318, #51601, #61430 ) ) ;
#64315=CARTESIAN_POINT ( 'NONE',  ( -2.500000000000000000, 1448.210448412289907, 183.1418046153980015 ) ) ;
#64317=CARTESIAN_POINT ( 'NONE',  ( -38.85669708052029847, 1447.921392184620117, 136.5057008105069940 ) ) ;
#64318=CARTESIAN_POINT ( 'NONE',  ( 11.60004869885203682, 1425.908350318139355, 137.5340513747880777 ) ) ;
#64319=CARTESIAN_POINT ( 'NONE',  ( 2.493582918933280101, 1417.705059006696047, 233.7388004561698551 ) ) ;
#64320=AXIS2_PLACEMENT_3D ( 'NONE', #13779, #72620, #82666 ) ;
#64321=CARTESIAN_POINT ( 'NONE',  ( -1.923670262848290013, 1471.323487510810082, 183.5084292385340063 ) ) ;
#64323=CARTESIAN_POINT ( 'NONE',  ( -15.18874088736159855, 1472.514660487180208, 270.0929918628660289 ) ) ;
#64324=CARTESIAN_POINT ( 'NONE',  ( 28.59384819061660110, 1440.913060387340010, 233.4742120170059820 ) ) ;
#64330=CARTESIAN_POINT ( 'NONE',  ( -29.06854782859999986, 1509.928156445530021, 211.9488907393379975 ) ) ;
#64331=CARTESIAN_POINT ( 'NONE',  ( 2.380922373579999807, 1474.722219450530019, 234.6118303102979894 ) ) ;
#64332=B_SPLINE_CURVE_WITH_KNOTS ( 'NONE', 5,
 ( #32626, #14710, #66259, #100377, #100903, #101448, #23662, #57845, #81911, #39370, #16884, #43782 ),
 .UNSPECIFIED., .F., .F.,
 ( 6, 3, 3, 6 ),
 ( 0.000000000000000000, 0.4215567365674310341, 0.8072018686246260621, 1.000000000000000000 ),
 .UNSPECIFIED. ) ;
#64337=CARTESIAN_POINT ( 'NONE',  ( 6.972733162820000885, 1409.156553594830029, 222.0127823373979936 ) ) ;
#64339=CARTESIAN_POINT ( 'NONE',  ( 2.689345562130000200, 1464.716346730230043, 236.9361815678979895 ) ) ;
#64342=CARTESIAN_POINT ( 'NONE',  ( -1.322994767380000214, 1450.726806844560087, 182.2564604496979825 ) ) ;
#64344=B_SPLINE_CURVE_WITH_KNOTS ( 'NONE', 5,
 ( #20998, #19346, #37282, #3702, #88237, #78728 ),
 .UNSPECIFIED., .F., .F.,
 ( 6, 6 ),
 ( 0.000000000000000000, 1.000000000000000000 ),
 .UNSPECIFIED. ) ;
#64348=ORIENTED_EDGE ( 'NONE', *, *, #33855, .T. ) ;
#64357=CARTESIAN_POINT ( 'NONE',  ( 20.06206385248925272, 1509.646645313393947, 187.2373516834030625 ) ) ;
#64358=CARTESIAN_POINT ( 'NONE',  ( 13.15931087223109941, 1409.372593648980001, 202.0512334247140132 ) ) ;
#64360=CARTESIAN_POINT ( 'NONE',  ( 3.410503593230000074, 1419.799443580629941, 185.4204322456980094 ) ) ;
#64362=FACE_OUTER_BOUND ( 'NONE', #71622, .T. ) ;
#64363=CIRCLE ( 'NONE', #53666, 1.988474534702024066 ) ;
#64365=ORIENTED_EDGE ( 'NONE', *, *, #72139, .T. ) ;
#64366=ORIENTED_EDGE ( 'NONE', *, *, #46758, .F. ) ;
#64368=CARTESIAN_POINT ( 'NONE',  ( -11.23669755706080053, 1415.007830323640064, 195.6839844364440069 ) ) ;
#64369=CARTESIAN_POINT ( 'NONE',  ( -12.50048419760000051, 1435.331243516640143, 150.8675838421980018 ) ) ;
#64371=CARTESIAN_POINT ( 'NONE',  ( -20.34485088181780199, 1499.600355960500110, 190.6291793570229913 ) ) ;
#64374=CARTESIAN_POINT ( 'NONE',  ( -0.5583389695640000872, 1486.508398414630165, 181.8176688025980070 ) ) ;
#64377=CARTESIAN_POINT ( 'NONE',  ( -13.10742788030691663, 1414.941152333605260, 220.2965691509508588 ) ) ;
#64382=CARTESIAN_POINT ( 'NONE',  ( 6.232532001951379463, 1407.162969925759853, 220.5304192662420064 ) ) ;
#64383=CARTESIAN_POINT ( 'NONE',  ( -13.20760688286200057, 1434.870232751160074, 149.1307101172629928 ) ) ;
#64386=B_SPLINE_SURFACE_WITH_KNOTS ( 'NONE', 5, 5, ( 
 ( #93481, #42543, #94040, #17305, #9489, #43655 ),
 ( #45877, #80012, #64331, #62137, #11704, #4418 ),
 ( #63779, #29595, #37459, #96262, #3335, #19538 ),
 ( #21168, #71094, #53745, #98454, #12245, #12799 ),
 ( #21724, #96825, #55376, #55926, #97896, #97356 ),
 ( #27954, #20094, #20625, #46434, #105781, #90046 ) ),
 .UNSPECIFIED., .F., .F., .F.,
 ( 6, 6 ),
 ( 6, 6 ),
 ( 29.77037649420000065, 87.06999293180000166 ),
 ( 0.000000000000000000, 2.000000000000000000 ),
 .UNSPECIFIED. ) ;
#64390=CARTESIAN_POINT ( 'NONE',  ( 36.92073955249999528, 1428.724883233329820, 259.2254644156980135 ) ) ;
#64391=CARTESIAN_POINT ( 'NONE',  ( -0.5262109480990000421, 1494.207478666230145, 181.3805628087980040 ) ) ;
#64392=CARTESIAN_POINT ( 'NONE',  ( -16.40068023219999915, 1409.485784761229979, 195.3783929211979853 ) ) ;
#64393=CARTESIAN_POINT ( 'NONE',  ( 20.62320342492137470, 1506.569407720647177, 201.1880884098677029 ) ) ;
#64395=CARTESIAN_POINT ( 'NONE',  ( -19.86631883729999970, 1428.969954335329930, 216.3509643007580223 ) ) ;
#64398=CARTESIAN_POINT ( 'NONE',  ( 30.24135515959999765, 1450.996674463330010, 136.2805541580979991 ) ) ;
#64400=CARTESIAN_POINT ( 'NONE',  ( -0.001991372178490000491, 1395.912990847029960, 197.8078701673980220 ) ) ;
#64402=CARTESIAN_POINT ( 'NONE',  ( 2.946467845570000410, 1509.056494393530102, 238.8527705038980002 ) ) ;
#64403=ORIENTED_EDGE ( 'NONE', *, *, #13025, .T. ) ;
#64404=EDGE_LOOP ( 'NONE', ( #31515, #80277, #83928, #21945 ) ) ;
#64406=CARTESIAN_POINT ( 'NONE',  ( -23.94289775954100108, 1410.422078863890192, 208.8148502979400121 ) ) ;
#64407=VERTEX_POINT ( 'NONE', #95675 ) ;
#64410=CARTESIAN_POINT ( 'NONE',  ( -3.874466659299999893, 1479.770995650030045, 235.3786624194979709 ) ) ;
#64411=CARTESIAN_POINT ( 'NONE',  ( -1.328200906410177184, 1420.347247853201225, 184.8989557469041074 ) ) ;
#64414=CARTESIAN_POINT ( 'NONE',  ( 46.05253185105119229, 1441.852346002359809, 266.6768988155079683 ) ) ;
#64415=EDGE_CURVE ( 'NONE', #31992, #93336, #18467, .T. ) ;
#64416=CARTESIAN_POINT ( 'NONE',  ( -11.41805403388689832, 1414.913057862230062, 220.8525437052670100 ) ) ;
#64423=CARTESIAN_POINT ( 'NONE',  ( 13.09408958547385460, 1443.019840760110583, 187.3616399427167494 ) ) ;
#64427=EDGE_CURVE ( 'NONE', #104141, #19775, #89305, .T. ) ;
#64428=DIRECTION ( 'NONE',  ( -0.7067700363771036720, 0.03085824620770448792, -0.7067700363771036720 ) ) ;
#64430=EDGE_CURVE ( 'NONE', #81429, #4737, #96227, .T. ) ;
#64431=CARTESIAN_POINT ( 'NONE',  ( -4.370116291996360758, 1424.878943209489535, 185.9531288255872425 ) ) ;
#64432=CARTESIAN_POINT ( 'NONE',  ( 11.45277010228440062, 1452.513120842550052, 149.9488700328180073 ) ) ;
#64436=DIRECTION ( 'NONE',  ( 0.000000000000000000, 1.000000000000000000, 0.000000000000000000 ) ) ;
#64438=DIRECTION ( 'NONE',  ( 1.000000000000000000, 0.000000000000000000, 0.000000000000000000 ) ) ;
#64443=CARTESIAN_POINT ( 'NONE',  ( 11.30500403589999792, 1428.976642997429963, 112.4493539157979995 ) ) ;
#64445=CARTESIAN_POINT ( 'NONE',  ( 10.05164999069999965, 1426.487183120430245, 224.8635561722979901 ) ) ;
#64447=CARTESIAN_POINT ( 'NONE',  ( -11.15489169059993735, 1425.160568487430055, 144.1681086605935604 ) ) ;
#64452=ADVANCED_FACE ( 'NONE', ( #105746 ), #67141, .F. ) ;
#64454=VERTEX_POINT ( 'NONE', #21693 ) ;
#64455=CARTESIAN_POINT ( 'NONE',  ( 3.947090874974254149, 1427.113278099589934, 137.0999999980980704 ) ) ;
#64456=CARTESIAN_POINT ( 'NONE',  ( -2.560278795423229781, 1439.616515393840018, 157.6872015775370244 ) ) ;
#64457=CARTESIAN_POINT ( 'NONE',  ( -14.45771163659999914, 1416.835808398129984, 221.3919539477980152 ) ) ;
#64458=CARTESIAN_POINT ( 'NONE',  ( 11.93801661799999891, 1433.480575387579847, 150.0148646725980086 ) ) ;
#64460=CARTESIAN_POINT ( 'NONE',  ( 13.15726448920050018, 1414.913060387399810, 198.3331475907570223 ) ) ;
#64461=EDGE_CURVE ( 'NONE', #8198, #68958, #65327, .T. ) ;
#64464=ADVANCED_FACE ( 'NONE', ( #41825 ), #42115, .F. ) ;
#64465=CARTESIAN_POINT ( 'NONE',  ( 7.459553558550000574, 1422.095603715230027, 231.2386102329980133 ) ) ;
#64467=AXIS2_PLACEMENT_3D ( 'NONE', #110467, #93640, #85248 ) ;
#64469=CARTESIAN_POINT ( 'NONE',  ( 3.512785867830420180E-12, 1395.913060387330006, 198.1220674046479928 ) ) ;
#64470=CARTESIAN_POINT ( 'NONE',  ( -18.41342271589999768, 1409.720851141630192, 222.9148940093980116 ) ) ;
#64471=CARTESIAN_POINT ( 'NONE',  ( 15.28398915819999893, 1435.448478077710206, 149.0740643685979876 ) ) ;
#64473=CARTESIAN_POINT ( 'NONE',  ( -1.543830048049999792, 1424.182865445729703, 228.3475006505979934 ) ) ;
#64474=CARTESIAN_POINT ( 'NONE',  ( 24.46211382750000141, 1438.319209241250064, 213.4123708239580139 ) ) ;
#64477=CARTESIAN_POINT ( 'NONE',  ( -35.82176637796790430, 1436.379724471920099, 136.2603715204670038 ) ) ;
#64478=CARTESIAN_POINT ( 'NONE',  ( 0.2097987188493439792, 1457.461435332639894, 183.0619989796059883 ) ) ;
#64479=CARTESIAN_POINT ( 'NONE',  ( -8.191952444756632090, 1407.860267943719919, 219.8961961182280049 ) ) ;
#64480=CARTESIAN_POINT ( 'NONE',  ( -17.17404474450000151, 1416.216596894529857, 202.8710369035879921 ) ) ;
#64483=CARTESIAN_POINT ( 'NONE',  ( -28.11107467879419985, 1509.207378190189957, 210.7860757214999978 ) ) ;
#64484=CARTESIAN_POINT ( 'NONE',  ( 12.06130614719999983, 1433.903343712190235, 147.2729309238979738 ) ) ;
#64485=CARTESIAN_POINT ( 'NONE',  ( -27.69670551879999820, 1435.466977414309895, 135.6947802121979976 ) ) ;
#64490=CARTESIAN_POINT ( 'NONE',  ( -4.508178739127020940, 1409.070489457920075, 223.4101744795629827 ) ) ;
#64493=CARTESIAN_POINT ( 'NONE',  ( 14.64585795956600123, 1509.424984143169922, 234.5789104686880080 ) ) ;
#64494=CARTESIAN_POINT ( 'NONE',  ( 5.730844508220573452, 1406.977338306732236, 269.6419569788193940 ) ) ;
#64495=CARTESIAN_POINT ( 'NONE',  ( 20.51078616439999891, 1453.154034703029993, 210.6541330983779972 ) ) ;
#64501=CARTESIAN_POINT ( 'NONE',  ( -29.34423976567429904, 1509.844966209650011, 208.6282038019159870 ) ) ;
#64502=CARTESIAN_POINT ( 'NONE',  ( 0.5007497712181619987, 1414.173381217940005, 184.9066978159829944 ) ) ;
#64504=DIRECTION ( 'NONE',  ( -0.1837295255851838782, -0.06561766200247082237, -0.9807842697869766369 ) ) ;
#64507=CARTESIAN_POINT ( 'NONE',  ( -0.1120303467899630145, 1420.419502555939744, 183.1208681730079775 ) ) ;
#64508=AXIS2_PLACEMENT_3D ( 'NONE', #103437, #26743, #3236 ) ;
#64510=CARTESIAN_POINT ( 'NONE',  ( 22.21106947969999723, 1410.183783044429902, 215.0444402526979957 ) ) ;
#64511=B_SPLINE_SURFACE_WITH_KNOTS ( 'NONE', 4, 5, ( 
 ( #80196, #29239, #28693, #86380, #70183, #3514 ),
 ( #27580, #52254, #1290, #37638, #18602, #62323 ),
 ( #45520, #95891, #2418, #37083, #62897, #10793 ),
 ( #52802, #71287, #53358, #71843, #36535, #95341 ),
 ( #86933, #70732, #105400, #44963, #19727, #97007 ) ),
 .UNSPECIFIED., .F., .F., .F.,
 ( 5, 5 ),
 ( 6, 6 ),
 ( 13.35596682890000153, 21.06373553689999767 ),
 ( 0.000000000000000000, 2.000000835909999886 ),
 .UNSPECIFIED. ) ;
#64512=DIRECTION ( 'NONE',  ( -1.986951185180850528E-13, 0.03085824620771311644, 0.9995237709234254808 ) ) ;
#64514=CARTESIAN_POINT ( 'NONE',  ( -16.46007637289999792, 1423.318218959529986, 228.6067745784980048 ) ) ;
#64516=CARTESIAN_POINT ( 'NONE',  ( -11.63691600037451401, 1426.763110590993392, 137.0152515069076742 ) ) ;
#64517=CARTESIAN_POINT ( 'NONE',  ( 25.47490434202370224, 1449.924909233149947, 207.9936631072650073 ) ) ;
#64520=CARTESIAN_POINT ( 'NONE',  ( -0.4667865956230000668, 1416.135524792730166, 233.5066666412979828 ) ) ;
#64524=CARTESIAN_POINT ( 'NONE',  ( -4.527446633101839701, 1485.996829922820098, 182.3396792648729843 ) ) ;
#64525=VERTEX_POINT ( 'NONE', #88631 ) ;
#64526=AXIS2_PLACEMENT_3D ( 'NONE', #20787, #28103, #96421 ) ;
#64528=CARTESIAN_POINT ( 'NONE',  ( -4.262072192076889365, 1441.213750638199826, 159.1103247205799960 ) ) ;
#64536=CARTESIAN_POINT ( 'NONE',  ( 15.80295874793040056, 1414.899199519979902, 191.3919695463190180 ) ) ;
#64537=FACE_OUTER_BOUND ( 'NONE', #80076, .T. ) ;
#64539=EDGE_CURVE ( 'NONE', #104987, #105027, #32848, .T. ) ;
#64540=CARTESIAN_POINT ( 'NONE',  ( -25.34177650560360107, 1450.805395652589823, 137.4212134988369769 ) ) ;
#64541=CARTESIAN_POINT ( 'NONE',  ( -11.43740528939999912, 1425.481182534629852, 144.1672625331979987 ) ) ;
#64542=CARTESIAN_POINT ( 'NONE',  ( 11.07372907340000090, 1410.233410434930192, 229.3828206623979895 ) ) ;
#64545=CARTESIAN_POINT ( 'NONE',  ( 39.18506236152150279, 1437.902641089279996, 134.0999999975959724 ) ) ;
#64548=VERTEX_POINT ( 'NONE', #63449 ) ;
#64549=CARTESIAN_POINT ( 'NONE',  ( 14.43150070665419982, 1435.522629004720102, 149.5715662318340264 ) ) ;
#64550=ORIENTED_EDGE ( 'NONE', *, *, #79417, .F. ) ;
#64551=ORIENTED_EDGE ( 'NONE', *, *, #91819, .T. ) ;
#64554=VECTOR ( 'NONE', #88796, 1000.000000000000000 ) ;
#64555=CARTESIAN_POINT ( 'NONE',  ( 0.05443591761330000139, 1451.171040272929758, 182.5324322684980132 ) ) ;
#64556=B_SPLINE_CURVE_WITH_KNOTS ( 'NONE', 5,
 ( #77126, #86608, #9358, #102838, #92801, #42967 ),
 .UNSPECIFIED., .F., .F.,
 ( 6, 6 ),
 ( -157.9969979290000026, -29.50720980500000223 ),
 .UNSPECIFIED. ) ;
#64557=CARTESIAN_POINT ( 'NONE',  ( -3.380492229449999719, 1485.523073118029970, 182.9528005117980172 ) ) ;
#64560=CARTESIAN_POINT ( 'NONE',  ( 5399.190729149044273, 50.28429875041807406, -8134.791976860689829 ) ) ;
#64561=EDGE_CURVE ( 'NONE', #65361, #97932, #61507, .T. ) ;
#64562=CARTESIAN_POINT ( 'NONE',  ( 27.78452742954910093, 1508.000976259739900, 207.7754991261529938 ) ) ;
#64563=CARTESIAN_POINT ( 'NONE',  ( 8.403208615350001409, 1415.931391677429929, 193.2488689964980040 ) ) ;
#64565=ORIENTED_EDGE ( 'NONE', *, *, #34974, .F. ) ;
#64566=CARTESIAN_POINT ( 'NONE',  ( -1.085894894499999928E-15, 1432.353341358199941, 150.3995506339979897 ) ) ;
#64569=CARTESIAN_POINT ( 'NONE',  ( 40.43917225116809533, 1440.913060387330006, 267.8759699188719878 ) ) ;
#64571=CARTESIAN_POINT ( 'NONE',  ( -0.0008084625836226779893, 1451.918325721145493, 154.0009410478433551 ) ) ;
#64572=ADVANCED_FACE ( 'NONE', ( #61790 ), #85008, .F. ) ;
#64573=ORIENTED_EDGE ( 'NONE', *, *, #62424, .T. ) ;
#64574=CARTESIAN_POINT ( 'NONE',  ( -0.05864779970183610358, 1450.911012361030089, 181.2397301690949973 ) ) ;
#64578=CARTESIAN_POINT ( 'NONE',  ( 22.49732387063940209, 1410.763224758360138, 206.2063201444890126 ) ) ;
#64580=CARTESIAN_POINT ( 'NONE',  ( 9.884505093230000483, 1406.768685218130031, 266.9235441556980390 ) ) ;
#64583=EDGE_CURVE ( 'NONE', #94550, #80209, #54401, .T. ) ;
#64584=CARTESIAN_POINT ( 'NONE',  ( 16.95715696330000100, 1458.910017354530055, 229.2965042560980180 ) ) ;
#64585=CARTESIAN_POINT ( 'NONE',  ( 0.000000000000000000, 1508.913060387330006, 224.7618459619980058 ) ) ;
#64589=CARTESIAN_POINT ( 'NONE',  ( -0.1525074781070819840, 1507.411687413830123, 180.8672947283149881 ) ) ;
#64590=CARTESIAN_POINT ( 'NONE',  ( 15.11448291366340158, 1451.479646069887622, 221.5393396382719970 ) ) ;
#64596=CARTESIAN_POINT ( 'NONE',  ( -19.28393528680000202, 1507.737928445829994, 229.5896611176980002 ) ) ;
#64597=CARTESIAN_POINT ( 'NONE',  ( 3.672212372280000192, 1459.726867865030044, 213.1264975034980296 ) ) ;
#64598=CARTESIAN_POINT ( 'NONE',  ( -11.76451447100000003, 1431.952785265209968, 150.8015324768979895 ) ) ;
#64601=CARTESIAN_POINT ( 'NONE',  ( -0.3285102747869809714, 1508.336848181169898, 237.7487632055650124 ) ) ;
#64602=EDGE_CURVE ( 'NONE', #22249, #65067, #7777, .T. ) ;
#64604=CARTESIAN_POINT ( 'NONE',  ( -23.82798562378626883, 1411.105473243607321, 207.5387497735277407 ) ) ;
#64605=CARTESIAN_POINT ( 'NONE',  ( 5.360003288404429966, 1422.228637084189813, 144.9391265021819777 ) ) ;
#64606=CARTESIAN_POINT ( 'NONE',  ( 0.2612701249639999834, 1416.813004075630033, 190.7776225037979714 ) ) ;
#64609=CARTESIAN_POINT ( 'NONE',  ( 3.441247510289999756, 1405.871390642129882, 268.4787024712979928 ) ) ;
#64612=FACE_OUTER_BOUND ( 'NONE', #91397, .T. ) ;
#64613=CARTESIAN_POINT ( 'NONE',  ( 21.32599293744084434, 1428.684983583262920, 219.2409462215593408 ) ) ;
#64615=CARTESIAN_POINT ( 'NONE',  ( 11.60004869885203682, 1423.462011167306855, 135.7646888042274327 ) ) ;
#64617=CARTESIAN_POINT ( 'NONE',  ( -0.5697989932908550381, 1450.893162568030220, 155.3351454289200149 ) ) ;
#64618=CARTESIAN_POINT ( 'NONE',  ( -1.726873275417834197, 1450.480600349099859, 182.9637712753274457 ) ) ;
#64619=CARTESIAN_POINT ( 'NONE',  ( 1.179291408672469732, 1450.813351935780020, 155.3354828870230051 ) ) ;
#64620=CARTESIAN_POINT ( 'NONE',  ( -14.27868134598659999, 1415.948038442679945, 221.2079983884039791 ) ) ;
#64622=CARTESIAN_POINT ( 'NONE',  ( -20.63825566599999917, 1425.387366209430184, 248.0989693021979861 ) ) ;
#64623=CARTESIAN_POINT ( 'NONE',  ( -27.05015830627079865, 1507.998384514670079, 211.3652037525360186 ) ) ;
#64624=CARTESIAN_POINT ( 'NONE',  ( 3.143814751020000298, 1440.618483647659787, 155.9530253030979736 ) ) ;
#64626=CARTESIAN_POINT ( 'NONE',  ( -2.107599154099999872, 1475.947830574629961, 267.2331464721979728 ) ) ;
#64627=PLANE ( 'NONE',  #6782 ) ;
#64628=CARTESIAN_POINT ( 'NONE',  ( -17.67071593990000267, 1412.982943450030007, 193.3745006087980016 ) ) ;
#64629=CARTESIAN_POINT ( 'NONE',  ( 17.60549899623140035, 1410.870509167670207, 224.1774152648420113 ) ) ;
#64631=CARTESIAN_POINT ( 'NONE',  ( 7.105427357599999217E-15, 1420.413060387330006, 188.2701767054980166 ) ) ;
#64632=CARTESIAN_POINT ( 'NONE',  ( 17.01536232022260009, 1507.593738162509908, 193.7118019646590028 ) ) ;
#64636=CARTESIAN_POINT ( 'NONE',  ( -8.579552460874170450, 1396.212664961330120, 216.0972139694970338 ) ) ;
#64638=CARTESIAN_POINT ( 'NONE',  ( -14.60687332829999896, 1422.240656693330038, 229.1148143803980020 ) ) ;
#64639=CARTESIAN_POINT ( 'NONE',  ( -45.59060096559999664, 1439.350741641819923, 268.9760078171979671 ) ) ;
#64640=ORIENTED_EDGE ( 'NONE', *, *, #42540, .F. ) ;
#64641=CARTESIAN_POINT ( 'NONE',  ( -9.758366233290264091, 1410.624983480943683, 229.7348544036108535 ) ) ;
#64645=CARTESIAN_POINT ( 'NONE',  ( 10.30253573629999941, 1425.145685828329988, 112.6579331979979912 ) ) ;
#64648=CARTESIAN_POINT ( 'NONE',  ( -16.17746047354429351, 1409.477984536645408, 225.0323634634132759 ) ) ;
#64662=VERTEX_POINT ( 'NONE', #53948 ) ;
#64663=CARTESIAN_POINT ( 'NONE',  ( -9.041387868970000241, 1396.228792609030052, 202.1530002182580006 ) ) ;
#64664=CARTESIAN_POINT ( 'NONE',  ( -21.45557649069999684, 1410.156571378229728, 216.3485480334879867 ) ) ;
#64665=CARTESIAN_POINT ( 'NONE',  ( -1.237038659479999803, 1415.048591087029763, 226.6890547777979918 ) ) ;
#64666=CARTESIAN_POINT ( 'NONE',  ( -13.50348581488808364, 1444.084003877494069, 169.3539515139137279 ) ) ;
#64670=CARTESIAN_POINT ( 'NONE',  ( 16.83667419020000011, 1416.263768433330142, 226.6570821373980209 ) ) ;
#64672=CARTESIAN_POINT ( 'NONE',  ( 2.709355696829999882, 1410.303802397230129, 185.6373498539979892 ) ) ;
#64674=CARTESIAN_POINT ( 'NONE',  ( -40.08938852926480223, 1445.470329989359925, 136.8855892427959873 ) ) ;
#64676=CARTESIAN_POINT ( 'NONE',  ( 7.298542379600410079, 1396.167931181390031, 200.8262254698040010 ) ) ;
#64677=CARTESIAN_POINT ( 'NONE',  ( -28.02579834269999992, 1443.109842421779831, 137.4877371060980238 ) ) ;
#64678=CARTESIAN_POINT ( 'NONE',  ( 11.76733812390000011, 1426.911783682829991, 146.2965758568979879 ) ) ;
#64680=ORIENTED_EDGE ( 'NONE', *, *, #72762, .F. ) ;
#64681=CARTESIAN_POINT ( 'NONE',  ( 4.408900587259999782, 1425.824676780029904, 185.4670178510979781 ) ) ;
#64682=CARTESIAN_POINT ( 'NONE',  ( 2.499999996433849070, 1449.068978386697381, 182.3376700388170661 ) ) ;
#64685=CARTESIAN_POINT ( 'NONE',  ( -18.20796897385059765, 1458.243120258429826, 227.9056602949669923 ) ) ;
#64686=CARTESIAN_POINT ( 'NONE',  ( -15.16833389349999983, 1459.965360397030054, 229.4811956966979949 ) ) ;
#64687=CARTESIAN_POINT ( 'NONE',  ( -6.232532106187401055, 1407.162969929529936, 197.7132727037109987 ) ) ;
#64688=DIRECTION ( 'NONE',  ( -1.000000000000000000, -1.947392753017155135E-14, -3.090046365888145414E-15 ) ) ;
#64693=CARTESIAN_POINT ( 'NONE',  ( -8.914143057620970367, 1509.305272612319868, 180.3769903018060177 ) ) ;
#64695=B_SPLINE_CURVE_WITH_KNOTS ( 'NONE', 5,
 ( #96124, #88282, #69852, #9910, #53040, #79890 ),
 .UNSPECIFIED., .F., .F.,
 ( 6, 6 ),
 ( 0.000000000000000000, 1.000000000000000000 ),
 .UNSPECIFIED. ) ;
#64696=CARTESIAN_POINT ( 'NONE',  ( 0.1955981716400000125, 1414.913060387329779, 225.1861338294980044 ) ) ;
#64698=VERTEX_POINT ( 'NONE', #107287 ) ;
#64702=CARTESIAN_POINT ( 'NONE',  ( -29.83607553919204491, 1419.456892885304342, 269.4690664095026591 ) ) ;
#64707=CARTESIAN_POINT ( 'NONE',  ( 2.500000000000000000, 1430.041878304429929, 157.3252622477980083 ) ) ;
#64708=CARTESIAN_POINT ( 'NONE',  ( -35.83479613928479779, 1440.913060387619907, 252.5442945837890250 ) ) ;
#64710=CARTESIAN_POINT ( 'NONE',  ( -0.1917209389985229939, 1466.035524394150116, 235.8475842902419970 ) ) ;
#64713=CARTESIAN_POINT ( 'NONE',  ( 42.54895236168549388, 1436.706489006040101, 270.0692006931200240 ) ) ;
#64716=ADVANCED_FACE ( 'NONE', ( #99419 ), #73713, .F. ) ;
#64717=CARTESIAN_POINT ( 'NONE',  ( 23.02067909570000026, 1409.743111324829897, 209.2425273049379939 ) ) ;
#64722=CARTESIAN_POINT ( 'NONE',  ( 4.196391599596410060, 1421.708143655280082, 184.6451467733209881 ) ) ;
#64723=CARTESIAN_POINT ( 'NONE',  ( -5.208257314369999946, 1415.371260711229979, 232.0253136197979984 ) ) ;
#64724=CARTESIAN_POINT ( 'NONE',  ( 8.160856992992099990, 1423.395965121194195, 139.1420365292543408 ) ) ;
#64728=B_SPLINE_CURVE_WITH_KNOTS ( 'NONE', 3,
 ( #41953, #32453, #92894, #7787, #14525, #6131, #66629, #59327, #67170, #82840 ),
 .UNSPECIFIED., .F., .F.,
 ( 4, 2, 2, 2, 4 ),
 ( -0.1063667421838040000, -0.07694718867315308852, -0.05063894887267449824, -0.02539707194426270298, -1.064426199959278563E-09 ),
 .UNSPECIFIED. ) ;
#64730=CARTESIAN_POINT ( 'NONE',  ( 1.237116821750000151, 1417.438760711529994, 234.9523517504979964 ) ) ;
#64732=CARTESIAN_POINT ( 'NONE',  ( -24.90078896885400184, 1441.036975948020199, 210.4313365108669984 ) ) ;
#64734=CARTESIAN_POINT ( 'NONE',  ( -11.88915037982130052, 1434.057645910959991, 147.6474571075829658 ) ) ;
#64736=CYLINDRICAL_SURFACE ( 'NONE', #13959, 1.500000000000001332 ) ;
#64737=CARTESIAN_POINT ( 'NONE',  ( 11.60004869885203682, 0.000000000000000000, 137.0999999980979851 ) ) ;
#64741=EDGE_CURVE ( 'NONE', #109512, #9799, #34558, .T. ) ;
#64743=CONICAL_SURFACE ( 'NONE', #66499, 21.50000000000000355, 0.3430239404209998177 ) ;
#64744=CARTESIAN_POINT ( 'NONE',  ( 11.60004869885203327, 1426.371423827809394, 136.9558871456979148 ) ) ;
#64745=CARTESIAN_POINT ( 'NONE',  ( 19.74167487489999928, 1455.375968942129930, 226.0788140436979745 ) ) ;
#64746=CARTESIAN_POINT ( 'NONE',  ( 7.136348315603505910, 1439.003107248918923, 154.1041582727210368 ) ) ;
#64751=CARTESIAN_POINT ( 'NONE',  ( 16.36816379095389706, 1421.588183160469725, 227.2088594400390491 ) ) ;
#64752=CARTESIAN_POINT ( 'NONE',  ( -3.654206553410000335, 1446.297061082940218, 167.4573427789980258 ) ) ;
#64753=CARTESIAN_POINT ( 'NONE',  ( -19.53863231420000446, 1425.698533139729989, 223.3134001096979944 ) ) ;
#64756=CARTESIAN_POINT ( 'NONE',  ( 17.08559277830000056, 1445.364338547270108, 190.4514208886979816 ) ) ;
#64758=CARTESIAN_POINT ( 'NONE',  ( 28.83583421379999834, 1509.587522266130009, 209.1233664437740174 ) ) ;
#64766=CARTESIAN_POINT ( 'NONE',  ( 1.451115179245930031, 1504.682986288419897, 181.2193327503090075 ) ) ;
#64768=B_SPLINE_CURVE_WITH_KNOTS ( 'NONE', 3,
 ( #105753, #28482, #3858, #88929, #89484, #96796, #46957, #20067, #88386, #11676, #97329, #98428, #109054, #39060, #91132, #73805, #91682, #22797, #57559, #92232, #64308, #15503, #83284, #14957, #90575, #49152, #108490, #48602, #21700, #65408, #23906, #40180, #6027, #74362, #107934, #65960, #31774, #30113, #55905, #40731, #4919, #90023, #74905, #81617, #13300, #47493, #6582, #13855, #98972, #48038, #32340, #30677 ),
 .UNSPECIFIED., .F., .F.,
 ( 4, 2, 2, 1, 1, 1, 2, 2, 2, 2, 1, 1, 1, 1, 1, 2, 2, 2, 2, 1, 1, 1, 1, 1, 2, 2, 2, 2, 1, 1, 1, 2, 2, 4 ),
 ( 0.000000000000000000, 0.1249999999996153077, 0.1874999999994217403, 0.2187499999993249566, 0.2343749999992864319, 0.2421874999992573163, 0.2460937499992527366, 0.2499999999992481570, 0.3749999999992578159, 0.4374999999992638666, 0.4687499999992769673, 0.4843749999992835731, 0.4921874999992881250, 0.4960937499993025024, 0.4980468749993096633, 0.4990234374993119948, 0.4999999999993143263, 0.6249999999997680744, 0.6874999999999948930, 0.7187500000001071365, 0.7343750000001494360, 0.7421875000001550982, 0.7460937500001577627, 0.7480468750001444400, 0.7490234375001525446, 0.7500000000001606493, 0.8125000000005421219, 0.8437500000007338574, 0.8593750000008296697, 0.8671875000008767431, 0.8710937500009010570, 0.8730468750008952838, 0.8750000000008895107, 1.000000000000000000 ),
 .UNSPECIFIED. ) ;
#64769=CARTESIAN_POINT ( 'NONE',  ( -13.45091335949210176, 1444.296404058437247, 186.9862568266497078 ) ) ;
#64771=CARTESIAN_POINT ( 'NONE',  ( -7.828115350939239825, 1507.298737064408897, 235.3518802339874583 ) ) ;
#64776=CARTESIAN_POINT ( 'NONE',  ( 20.17495212240000058, 1508.361596599530003, 189.3322781249979982 ) ) ;
#64781=ORIENTED_EDGE ( 'NONE', *, *, #36883, .F. ) ;
#64783=CARTESIAN_POINT ( 'NONE',  ( 13.36396446440000041, 1509.377767200929839, 234.5402373753979930 ) ) ;
#64785=CARTESIAN_POINT ( 'NONE',  ( 34.38405749794775801, 1423.397540913143985, 269.5231537529844559 ) ) ;
#64786=CARTESIAN_POINT ( 'NONE',  ( 3.980216533449999712E-09, 1468.084175534530004, 248.5896189557980165 ) ) ;
#64787=CARTESIAN_POINT ( 'NONE',  ( -19.73850182230000172, 1499.093133259129900, 189.2250669414979996 ) ) ;
#64788=CARTESIAN_POINT ( 'NONE',  ( -11.83876387009999931, 1433.336427731999947, 150.5404244326980177 ) ) ;
#64791=CARTESIAN_POINT ( 'NONE',  ( 11.68510097434900175, 1426.730240608209897, 140.4555551319089943 ) ) ;
#64792=DIRECTION ( 'NONE',  ( -0.8529428551538207337, 0.5214727017401559195, 0.02355222244016309113 ) ) ;
#64793=LINE ( 'NONE', #22719, #50000 ) ;
#64795=DIRECTION ( 'NONE',  ( -1.000000000000000000, 0.000000000000000000, 0.000000000000000000 ) ) ;
#64798=CARTESIAN_POINT ( 'NONE',  ( -4.852802044422932504, 1509.212694702193176, 238.7485159040689950 ) ) ;
#64799=CARTESIAN_POINT ( 'NONE',  ( 1.073572097657399993E-09, 1410.789257220119907, 256.6870931748030102 ) ) ;
#64804=CARTESIAN_POINT ( 'NONE',  ( -13.58968549449999941, 1472.672770405929896, 270.0972160539979541 ) ) ;
#64810=CARTESIAN_POINT ( 'NONE',  ( 0.3919100467378520136, 1450.899374586919976, 181.2708617675390030 ) ) ;
#64811=CARTESIAN_POINT ( 'NONE',  ( -20.50000000000000000, 1445.052233488290085, 169.0968414572980123 ) ) ;
#64813=B_SPLINE_CURVE_WITH_KNOTS ( 'NONE', 3,
 ( #39127, #106887, #29096, #97394 ),
 .UNSPECIFIED., .F., .F.,
 ( 4, 4 ),
 ( 0.000000000000000000, 0.0003467901758445098839 ),
 .UNSPECIFIED. ) ;
#64816=CARTESIAN_POINT ( 'NONE',  ( -24.04206359393009862, 1411.123105596929918, 266.7326845484290061 ) ) ;
#64818=CARTESIAN_POINT ( 'NONE',  ( -3.544577584565780093, 1502.375471873259812, 181.1794101401630144 ) ) ;
#64819=ORIENTED_EDGE ( 'NONE', *, *, #26714, .T. ) ;
#64822=CARTESIAN_POINT ( 'NONE',  ( 4.847717379287757922, 1423.484125437993725, 184.1362136828789176 ) ) ;
#64824=CARTESIAN_POINT ( 'NONE',  ( -12.15287379559999970, 1455.446570946329985, 187.1561056955980007 ) ) ;
#64826=CARTESIAN_POINT ( 'NONE',  ( -2.500000000000000444, 1449.021333099697358, 183.0995997157531576 ) ) ;
#64828=CARTESIAN_POINT ( 'NONE',  ( -26.15575153829999877, 1435.490056906990048, 135.8696537409980181 ) ) ;
#64831=CARTESIAN_POINT ( 'NONE',  ( -1.600048698852036821, 1401.254281879943164, 134.0999999980979851 ) ) ;
#64833=CARTESIAN_POINT ( 'NONE',  ( -38.60728422249630398, 1426.656195254630120, 270.0188047174270309 ) ) ;
#64835=CARTESIAN_POINT ( 'NONE',  ( -4.365829376490000691, 1396.065518508630021, 198.9343448857979979 ) ) ;
#64837=ORIENTED_EDGE ( 'NONE', *, *, #57084, .F. ) ;
#64844=CARTESIAN_POINT ( 'NONE',  ( 2.953701937874160244, 1440.359118138959957, 157.3263569013780057 ) ) ;
#64847=FACE_OUTER_BOUND ( 'NONE', #56417, .T. ) ;
#64851=CARTESIAN_POINT ( 'NONE',  ( -38.81202641437909762, 1450.612734560829949, 135.3761647280269926 ) ) ;
#64852=CARTESIAN_POINT ( 'NONE',  ( -23.49479895857739464, 1448.333498076887736, 215.7494633260788817 ) ) ;
#64857=CARTESIAN_POINT ( 'NONE',  ( 13.76682154080000053, 1416.274718422629803, 196.4072499923979933 ) ) ;
#64861=CARTESIAN_POINT ( 'NONE',  ( 16.40119948470000111, 1409.652464919530075, 226.0181189845979759 ) ) ;
#64864=CARTESIAN_POINT ( 'NONE',  ( 4.255617697982819969, 1441.290921029950141, 160.2176512041789920 ) ) ;
#64869=CARTESIAN_POINT ( 'NONE',  ( -8.322172262500000528, 1473.608514543630008, 270.1222559170979594 ) ) ;
#64871=CARTESIAN_POINT ( 'NONE',  ( -6.305026483082059485, 1422.156206029339955, 144.1470533162859908 ) ) ;
#64874=CARTESIAN_POINT ( 'NONE',  ( 11.36480844366392517, 1425.604749195035765, 138.8039940692290486 ) ) ;
#64875=CARTESIAN_POINT ( 'NONE',  ( 2.290177320370077485, 1417.585464588979448, 233.4942916757924820 ) ) ;
#64876=CARTESIAN_POINT ( 'NONE',  ( 17.98285126925155808, 1424.103838246010582, 225.5445409078726016 ) ) ;
#64878=LINE ( 'NONE', #75479, #43383 ) ;
#64879=CARTESIAN_POINT ( 'NONE',  ( 33.54441201048500432, 1440.913060383900074, 247.8471729086510038 ) ) ;
#64881=DIRECTION ( 'NONE',  ( 1.000000000000000000, 0.000000000000000000, 0.000000000000000000 ) ) ;
#64884=CARTESIAN_POINT ( 'NONE',  ( 13.51610093808349866, 1443.913060387330006, 150.6358704321320090 ) ) ;
#64886=B_SPLINE_CURVE_WITH_KNOTS ( 'NONE', 3,
 ( #38711, #54456, #72886, #46048 ),
 .UNSPECIFIED., .F., .F.,
 ( 4, 4 ),
 ( 0.003723731023023103479, 0.004070443920417508681 ),
 .UNSPECIFIED. ) ;
#64887=CARTESIAN_POINT ( 'NONE',  ( -29.02628104849999957, 1509.926680457029988, 211.9910930718879740 ) ) ;
#64889=DIRECTION ( 'NONE',  ( 1.000000000000000000, 0.000000000000000000, 0.000000000000000000 ) ) ;
#64893=CARTESIAN_POINT ( 'NONE',  ( -15.02984757429999974, 1489.474306033729817, 193.0520931039979757 ) ) ;
#64895=CARTESIAN_POINT ( 'NONE',  ( 2.194850040300000416, 1464.708290688329953, 236.4512987645979933 ) ) ;
#64897=ORIENTED_EDGE ( 'NONE', *, *, #109085, .F. ) ;
#64898=CARTESIAN_POINT ( 'NONE',  ( -0.9007582589660000361, 1450.862954789030027, 181.4326571169980014 ) ) ;
#64901=CARTESIAN_POINT ( 'NONE',  ( 1.556370309037290012, 1414.996442620790276, 191.7142051069610034 ) ) ;
#64907=LINE ( 'NONE', #39112, #40480 ) ;
#64908=CARTESIAN_POINT ( 'NONE',  ( -11.60004869884790679, 1426.654320091513227, 134.6710072971295915 ) ) ;
#64909=APPLICATION_CONTEXT ( 'automotive_design' ) ;
#64911=CARTESIAN_POINT ( 'NONE',  ( 1.313206738690460007, 1408.958918577119903, 194.1820485240640153 ) ) ;
#64912=CARTESIAN_POINT ( 'NONE',  ( 1.133107404670000040, 1409.891086916829863, 185.2370129161979833 ) ) ;
#64914=CARTESIAN_POINT ( 'NONE',  ( -17.51076275510000002, 1437.054563566370007, 191.0009178520979845 ) ) ;
#64915=CARTESIAN_POINT ( 'NONE',  ( 11.30152483799999885, 1432.323726532349838, 151.5220244154980094 ) ) ;
#64919=CARTESIAN_POINT ( 'NONE',  ( 18.49724510411089895, 1458.837717710030120, 227.6444223862160072 ) ) ;
#64922=CARTESIAN_POINT ( 'NONE',  ( -20.48903499640979931, 1504.270597067930112, 190.4936467704999927 ) ) ;
#64931=CARTESIAN_POINT ( 'NONE',  ( 1.430133918726229858, 1408.963001764240062, 224.1218459596319974 ) ) ;
#64932=CARTESIAN_POINT ( 'NONE',  ( -13.19741843239559920, 1434.958471197750214, 149.6694188718060161 ) ) ;
#64936=ORIENTED_EDGE ( 'NONE', *, *, #14464, .F. ) ;
#64937=CARTESIAN_POINT ( 'NONE',  ( 34.21122890170000375, 1429.487523075830040, 254.6787130006979964 ) ) ;
#64938=CARTESIAN_POINT ( 'NONE',  ( -25.47381561740000322, 1508.124471598029913, 199.2434219609179991 ) ) ;
#64940=CARTESIAN_POINT ( 'NONE',  ( -17.11609476099999583, 1409.675656833430139, 194.7256359347979924 ) ) ;
#64941=CARTESIAN_POINT ( 'NONE',  ( 20.90608034670421489, 1506.501081260929141, 202.1326028675541124 ) ) ;
#64942=B_SPLINE_CURVE_WITH_KNOTS ( 'NONE', 3,
 ( #68856, #50934, #77245, #24587, #84520, #76674, #110824, #26260, #41976, #25697, #101291, #1096, #59350, #59896, #95138, #16190, #545, #102959, #60447, #17283, #51477, #69411, #85607, #52597 ),
 .UNSPECIFIED., .F., .F.,
 ( 4, 1, 1, 1, 1, 1, 1, 1, 1, 1, 1, 1, 1, 1, 1, 1, 1, 1, 1, 1, 1, 4 ),
 ( 0.000000000000000000, 0.03678250764465099826, 0.07385281888605636780, 0.1111996474769267329, 0.1487830646126913348, 0.1865181366940833751, 0.2243518957215068221, 0.2622984075178853014, 0.3003633763990504746, 0.3385433752522598039, 0.3768295913742388814, 0.4152115393309738778, 0.4536807115451020334, 0.4922340963814919035, 0.5605612547399086987, 0.7446199554937297238, 0.7613094231601892359, 0.7882927121057347053, 0.8256044977319447753, 0.8732899491329376707, 0.9314021484345864632, 1.000000000000000000 ),
 .UNSPECIFIED. ) ;
#64943=CARTESIAN_POINT ( 'NONE',  ( -27.31509605250000305, 1435.476323111060083, 231.6984297931980166 ) ) ;
#64945=CARTESIAN_POINT ( 'NONE',  ( -11.67164634742229978, 1452.505477515639996, 149.8358995112070033 ) ) ;
#64946=CARTESIAN_POINT ( 'NONE',  ( 22.86388144384979881, 1435.295931049420005, 134.1000000033949959 ) ) ;
#64950=CARTESIAN_POINT ( 'NONE',  ( 14.36093106826099941, 1421.078536739219999, 228.5629966840699865 ) ) ;
#64952=VERTEX_POINT ( 'NONE', #6482 ) ;
#64956=CARTESIAN_POINT ( 'NONE',  ( 0.2228126134860000107, 1419.322656201930158, 227.2982164590980005 ) ) ;
#64958=CARTESIAN_POINT ( 'NONE',  ( -3.370431671830000031, 1507.639056475829875, 236.7514476338979819 ) ) ;
#64962=CARTESIAN_POINT ( 'NONE',  ( 45.55029481160520533, 1443.690934598179865, 266.1917672049960402 ) ) ;
#64963=CARTESIAN_POINT ( 'NONE',  ( -13.15726447900050111, 1414.913057819769847, 220.2185343040899852 ) ) ;
#64964=CARTESIAN_POINT ( 'NONE',  ( 0.01268070879549999981, 1420.208146125329904, 183.8974516564980206 ) ) ;
#64966=VERTEX_POINT ( 'NONE', #42850 ) ;
#64968=CARTESIAN_POINT ( 'NONE',  ( 13.14730852243417125, 1443.066035680741606, 187.4537189246333071 ) ) ;
#64974=CARTESIAN_POINT ( 'NONE',  ( 2.364810563598290116, 1452.830479382759904, 152.4381100973169794 ) ) ;
#64976=DIRECTION ( 'NONE',  ( 5.569232340736249362E-09, 0.03085823662921604107, -0.9995237712191418211 ) ) ;
#64977=CARTESIAN_POINT ( 'NONE',  ( 10.98347131258903531, 1433.186512253130104, 151.7693442413542186 ) ) ;
#64979=CARTESIAN_POINT ( 'NONE',  ( 0.03404605193919440359, 1409.337710408478870, 232.7998981013873561 ) ) ;
#64981=CARTESIAN_POINT ( 'NONE',  ( 17.16792148770000281, 1507.624001450029937, 193.8207119598980057 ) ) ;
#64983=CARTESIAN_POINT ( 'NONE',  ( -24.06019813578369693, 1508.205534045840068, 222.3305738533050260 ) ) ;
#64984=CARTESIAN_POINT ( 'NONE',  ( 4.852453529149999945, 1427.440084250629980, 147.7756948909979826 ) ) ;
#64985=ORIENTED_EDGE ( 'NONE', *, *, #48750, .F. ) ;
#64986=CARTESIAN_POINT ( 'NONE',  ( 19.62446893450000118, 1440.913060387330006, 214.3676144200779845 ) ) ;
#64987=FACE_OUTER_BOUND ( 'NONE', #43875, .T. ) ;
#64994=CARTESIAN_POINT ( 'NONE',  ( -2.927701378049999713E-15, 1442.756953654919926, 150.7628527808980152 ) ) ;
#64996=CARTESIAN_POINT ( 'NONE',  ( 11.93044055110000023, 1433.480854295200061, 150.1316028450980298 ) ) ;
#64997=CARTESIAN_POINT ( 'NONE',  ( 17.87874079019999840, 1466.750581349630238, 265.6112250856980381 ) ) ;
#64998=CARTESIAN_POINT ( 'NONE',  ( 13.15726445890019924, 1415.090956648730071, 197.4244024782210261 ) ) ;
#65002=CARTESIAN_POINT ( 'NONE',  ( 16.78081809529999902, 1422.111771137829919, 226.9773849540979995 ) ) ;
#65005=CARTESIAN_POINT ( 'NONE',  ( -12.27023110815660090, 1416.839692126590080, 194.6640136892829958 ) ) ;
#65006=CARTESIAN_POINT ( 'NONE',  ( 14.03282286439999993, 1434.988470873060123, 148.9022279828979833 ) ) ;
#65007=CARTESIAN_POINT ( 'NONE',  ( -1.545334783909999787, 1420.511277924829983, 228.1845102176980049 ) ) ;
#65013=CARTESIAN_POINT ( 'NONE',  ( 4.602958218326069779E-16, 1426.918876943007945, 134.0999999980979851 ) ) ;
#65014=CARTESIAN_POINT ( 'NONE',  ( 0.2146574046981659933, 1454.739073199480117, 183.1787909047579888 ) ) ;
#65015=CARTESIAN_POINT ( 'NONE',  ( -14.97927429840000002, 1409.436148172130061, 207.8035683059279961 ) ) ;
#65016=CARTESIAN_POINT ( 'NONE',  ( -14.57172186309999873, 1416.216739748630062, 198.5744135584980086 ) ) ;
#65018=CARTESIAN_POINT ( 'NONE',  ( 13.50105822729999971, 1434.968970759619879, 148.5019007266980111 ) ) ;
#65019=CARTESIAN_POINT ( 'NONE',  ( -34.72084050082580120, 1435.748200648189822, 134.0999999979019890 ) ) ;
#65028=CARTESIAN_POINT ( 'NONE',  ( 19.73997541995389327, 1410.042412248772507, 269.5249961499508800 ) ) ;
#65029=CARTESIAN_POINT ( 'NONE',  ( 20.24918891140000099, 1453.165958253830013, 209.7008772832169825 ) ) ;
#65035=CARTESIAN_POINT ( 'NONE',  ( -27.02655812420000103, 1451.969196582630047, 135.3522152283979949 ) ) ;
#65037=CARTESIAN_POINT ( 'NONE',  ( -15.84999874720450030, 1409.466461689740072, 225.3744910454719843 ) ) ;
#65039=EDGE_LOOP ( 'NONE', ( #54920, #69175, #96081, #20390, #78396, #56682, #100888, #63330 ) ) ;
#65044=CARTESIAN_POINT ( 'NONE',  ( -22.35793875571175704, 1411.052089644072339, 213.2600881478184078 ) ) ;
#65047=CARTESIAN_POINT ( 'NONE',  ( 0.9807047822899999101, 1465.891021135629899, 235.6257849829979989 ) ) ;
#65049=CARTESIAN_POINT ( 'NONE',  ( 21.38088874639999659, 1410.581319675330178, 217.4617667072079996 ) ) ;
#65053=CARTESIAN_POINT ( 'NONE',  ( -17.07859384879999709, 1422.557183082329857, 226.8334922828980211 ) ) ;
#65055=CARTESIAN_POINT ( 'NONE',  ( 22.06116865624104051, 1506.527232287948436, 209.0797454662948383 ) ) ;
#65056=CARTESIAN_POINT ( 'NONE',  ( 24.17539452729910110, 1411.086234962870094, 209.2386321558909685 ) ) ;
#65059=CARTESIAN_POINT ( 'NONE',  ( -0.5401129779459999947, 1417.004128308830104, 234.1403188875979708 ) ) ;
#65062=CARTESIAN_POINT ( 'NONE',  ( -18.11291060900000005, 1424.770096122030054, 227.5276574296979959 ) ) ;
#65063=EDGE_LOOP ( 'NONE', ( #36045, #37748, #2866, #1728, #16243, #45277, #75941, #3591, #46871, #49913, #34070, #18789, #18643, #60134, #23760, #104935, #54947, #75724, #82214, #95500 ) ) ;
#65065=CARTESIAN_POINT ( 'NONE',  ( -4.225717896591520528, 1441.570140337609928, 166.2107877269230016 ) ) ;
#65067=VERTEX_POINT ( 'NONE', #105941 ) ;
#65073=CARTESIAN_POINT ( 'NONE',  ( -20.59664500270120158, 1507.763472350329948, 190.3621299389660066 ) ) ;
#65074=CARTESIAN_POINT ( 'NONE',  ( 19.74164504280149757, 1455.376031929259852, 226.0788368184279875 ) ) ;
#65077=CARTESIAN_POINT ( 'NONE',  ( -25.55040591486629964, 1450.975945474709988, 137.0378106854079761 ) ) ;
#65078=CARTESIAN_POINT ( 'NONE',  ( -10.81518740880000173, 1424.921099675630103, 144.1705347732979874 ) ) ;
#65083=CARTESIAN_POINT ( 'NONE',  ( 35.35021333609370231, 1451.550776711799926, 134.0999999984329918 ) ) ;
#65084=CARTESIAN_POINT ( 'NONE',  ( -39.71338550447469373, 1440.957585935580028, 136.8228776063639884 ) ) ;
#65085=VERTEX_POINT ( 'NONE', #33059 ) ;
#65087=CARTESIAN_POINT ( 'NONE',  ( -16.36071930985236023, 1410.862894828049775, 226.6398529266253945 ) ) ;
#65089=VERTEX_POINT ( 'NONE', #67247 ) ;
#65092=CARTESIAN_POINT ( 'NONE',  ( 14.74339714404158386, 1410.800272255869004, 227.6397578307206970 ) ) ;
#65094=CARTESIAN_POINT ( 'NONE',  ( 0.08037848105579999125, 1450.910253508570122, 181.8884884461979823 ) ) ;
#65096=CARTESIAN_POINT ( 'NONE',  ( -2.500000000000000000, 1439.336915393649861, 160.7446411339429915 ) ) ;
#65100=CARTESIAN_POINT ( 'NONE',  ( -1.520741264619999811, 1487.753241046729954, 231.1621170213979894 ) ) ;
#65101=( BOUNDED_SURFACE ( )  B_SPLINE_SURFACE ( 1, 2, ( 
 ( #38306, #4710, #64094 ),
 ( #89270, #29902, #73032 ) ),
 .UNSPECIFIED., .F., .F., .F. ) 
 B_SPLINE_SURFACE_WITH_KNOTS ( ( 2, 2 ),
 ( 3, 3 ),
 ( -10000.00000000000000, 10000.00000000000000 ),
 ( 5.300753508068390296, 6.148747966412170030 ),
 .UNSPECIFIED. ) 
 GEOMETRIC_REPRESENTATION_ITEM ( )  RATIONAL_B_SPLINE_SURFACE ( (
 ( 0.8627701935022100699, 0.8231028658293879641, 0.9541560038375069830),
 ( 0.8627701935022100699, 0.8231028658293879641, 0.9541560038375069830) ) ) 
 REPRESENTATION_ITEM ( '' )  SURFACE ( )  );
#65102=CARTESIAN_POINT ( 'NONE',  ( 12.50239388149999975, 1416.520646107730045, 196.1087965155979873 ) ) ;
#65104=ORIENTED_EDGE ( 'NONE', *, *, #85947, .F. ) ;
#65108=CARTESIAN_POINT ( 'NONE',  ( 11.01884469525210086, 1414.913527275050001, 222.3009101210830067 ) ) ;
#65109=CARTESIAN_POINT ( 'NONE',  ( -0.0002367882524984884097, 1452.632826069514067, 153.4248884296770825 ) ) ;
#65110=ORIENTED_EDGE ( 'NONE', *, *, #25126, .T. ) ;
#65111=CARTESIAN_POINT ( 'NONE',  ( -0.1807640977892359946, 1452.343039199269924, 183.2709366604759964 ) ) ;
#65112=EDGE_CURVE ( 'NONE', #60117, #68958, #22993, .T. ) ;
#65113=CARTESIAN_POINT ( 'NONE',  ( -14.82206140629999958, 1409.430658177129999, 192.2978730262979923 ) ) ;
#65118=CARTESIAN_POINT ( 'NONE',  ( 45.11781007811134003, 1434.982686472060777, 266.2041965797337753 ) ) ;
#65121=CARTESIAN_POINT ( 'NONE',  ( 15.80576098240000071, 1459.642315333929901, 231.7528682457979983 ) ) ;
#65122=CARTESIAN_POINT ( 'NONE',  ( -11.60004869883236900, 1424.991221944704876, 137.7502973972462712 ) ) ;
#65123=CARTESIAN_POINT ( 'NONE',  ( -4.999961604102280077, 1422.677871151950740, 184.8425649944229576 ) ) ;
#65127=CARTESIAN_POINT ( 'NONE',  ( -0.1099879671840549994, 1508.188471773840092, 180.5321450717350160 ) ) ;
#65128=CARTESIAN_POINT ( 'NONE',  ( 16.68655976294136423, 1449.426786541504725, 219.0859720786843354 ) ) ;
#65130=CARTESIAN_POINT ( 'NONE',  ( 18.57349583820000305, 1508.241272126429976, 188.5096420841980205 ) ) ;
#65131=CARTESIAN_POINT ( 'NONE',  ( -11.60004869885203682, 1426.235585318013136, 138.1668353689006778 ) ) ;
#65133=ORIENTED_EDGE ( 'NONE', *, *, #7569, .T. ) ;
#65134=CARTESIAN_POINT ( 'NONE',  ( -18.87980335319999625, 1507.654596516530091, 229.6982590054979880 ) ) ;
#65136=CARTESIAN_POINT ( 'NONE',  ( -11.84293662189999807, 1430.740907695629858, 149.7515331920980088 ) ) ;
#65139=CARTESIAN_POINT ( 'NONE',  ( 9.364590546472930654, 1429.570614365610027, 153.1245137695219967 ) ) ;
#65143=CARTESIAN_POINT ( 'NONE',  ( -18.98990496860000121, 1457.449620047930011, 226.8627260498979865 ) ) ;
#65145=CARTESIAN_POINT ( 'NONE',  ( -2.646145475300000438, 1485.849692937330019, 182.4222346857980313 ) ) ;
#65148=CARTESIAN_POINT ( 'NONE',  ( 9.934322565360000468, 1406.490945014630142, 267.8131979194979522 ) ) ;
#65150=CARTESIAN_POINT ( 'NONE',  ( 38.64250925720489960, 1443.812098352220119, 137.1879208744120149 ) ) ;
#65152=CARTESIAN_POINT ( 'NONE',  ( 24.24851111099502177, 1436.811212231015816, 213.2345827942206427 ) ) ;
#65154=CARTESIAN_POINT ( 'NONE',  ( 11.60004869885203682, 1422.719466699653367, 136.9994304497845405 ) ) ;
#65155=EDGE_CURVE ( 'NONE', #47913, #27899, #23967, .T. ) ;
#65156=CARTESIAN_POINT ( 'NONE',  ( -1.469498567789999877, 1450.684669993949910, 155.6080925168980116 ) ) ;
#65158=CARTESIAN_POINT ( 'NONE',  ( 2.437740546411169884, 1449.518193510780065, 155.3362082612889878 ) ) ;
#65161=CARTESIAN_POINT ( 'NONE',  ( -16.86383896459999931, 1416.370072266829993, 262.6648722463980334 ) ) ;
#65163=CARTESIAN_POINT ( 'NONE',  ( 20.00300104875735485, 1507.847453148246132, 229.0979941101246595 ) ) ;
#65164=CARTESIAN_POINT ( 'NONE',  ( 2.500000000000000000, 1439.162612134750134, 158.2752953368980116 ) ) ;
#65165=CARTESIAN_POINT ( 'NONE',  ( -6.157771320920000235, 1475.261075526229888, 269.2805908171979468 ) ) ;
#65166=DIRECTION ( 'NONE',  ( -0.7071067811865475727, 0.000000000000000000, 0.7071067811865475727 ) ) ;
#65168=ADVANCED_FACE ( 'NONE', ( #84017 ), #31302, .F. ) ;
#65169=CARTESIAN_POINT ( 'NONE',  ( 17.95365621164559755, 1414.298405984240162, 223.3003528621370037 ) ) ;
#65173=CARTESIAN_POINT ( 'NONE',  ( 12.23023785385239925, 1416.449138228889979, 223.5409194945380023 ) ) ;
#65177=CARTESIAN_POINT ( 'NONE',  ( 25.23672735205020956, 1509.794346327565336, 195.3594086562886787 ) ) ;
#65179=CARTESIAN_POINT ( 'NONE',  ( -21.29937734410000161, 1409.656851037430215, 203.0292493083479712 ) ) ;
#65181=CARTESIAN_POINT ( 'NONE',  ( -15.08147747143999950, 1422.395625179872013, 228.4054715315770068 ) ) ;
#65182=CARTESIAN_POINT ( 'NONE',  ( 19.43004901905829840, 1455.649281546792963, 225.6093494351993058 ) ) ;
#65183=ORIENTED_EDGE ( 'NONE', *, *, #3636, .T. ) ;
#65185=CARTESIAN_POINT ( 'NONE',  ( -3.018679138473939094, 1410.395947885577925, 232.5197392892935397 ) ) ;
#65188=CARTESIAN_POINT ( 'NONE',  ( 11.62665903299999925, 1425.870842608729845, 143.4637069816980102 ) ) ;
#65195=CARTESIAN_POINT ( 'NONE',  ( -4.852453529149999945, 1427.440084250629980, 147.7756948909979826 ) ) ;
#65200=EDGE_CURVE ( 'NONE', #14800, #70574, #96049, .T. ) ;
#65202=ORIENTED_EDGE ( 'NONE', *, *, #41297, .F. ) ;
#65204=CARTESIAN_POINT ( 'NONE',  ( -11.13078726520000039, 1396.479398862830067, 203.7609886355280082 ) ) ;
#65205=CARTESIAN_POINT ( 'NONE',  ( -22.00494421760000208, 1410.601295256730054, 214.9637058440179942 ) ) ;
#65206=CARTESIAN_POINT ( 'NONE',  ( -1.556370157619999972, 1414.996444526030018, 226.5294865527980051 ) ) ;
#65207=CARTESIAN_POINT ( 'NONE',  ( -13.02693512829444700, 1444.857299289932826, 169.4172639506946325 ) ) ;
#65210=CYLINDRICAL_SURFACE ( 'NONE', #103250, 1.999999999999982014 ) ;
#65211=FACE_OUTER_BOUND ( 'NONE', #77206, .T. ) ;
#65212=AXIS2_PLACEMENT_3D ( 'NONE', #17138, #51328, #13164 ) ;
#65213=CARTESIAN_POINT ( 'NONE',  ( 4.204230650730000463, 1410.300354822230247, 186.1030492174980111 ) ) ;
#65214=CARTESIAN_POINT ( 'NONE',  ( -11.74107623939999989, 1415.088275290029969, 195.6245027881980150 ) ) ;
#65215=CARTESIAN_POINT ( 'NONE',  ( -40.18287292922800447, 1445.042548787329906, 136.9561948773950064 ) ) ;
#65216=CARTESIAN_POINT ( 'NONE',  ( 10.37381255510450018, 1396.275321906710133, 205.2617250521719825 ) ) ;
#65217=ADVANCED_FACE ( 'NONE', ( #72749 ), #47004, .T. ) ;
#65218=CARTESIAN_POINT ( 'NONE',  ( 33.29224916083880004, 1436.556216818010171, 136.5296164106590027 ) ) ;
#65219=CARTESIAN_POINT ( 'NONE',  ( 10.84999101200000204, 1425.206555810429791, 146.9406714080979839 ) ) ;
#65221=ORIENTED_EDGE ( 'NONE', *, *, #43723, .T. ) ;
#65222=CARTESIAN_POINT ( 'NONE',  ( 3.827442175440000316, 1424.287716995130040, 184.6276801873979991 ) ) ;
#65226=ORIENTED_EDGE ( 'NONE', *, *, #85613, .T. ) ;
#65232=EDGE_CURVE ( 'NONE', #66863, #12979, #78956, .T. ) ;
#65235=CARTESIAN_POINT ( 'NONE',  ( -11.79167011069929849, 1509.456730339710020, 181.3501055891659917 ) ) ;
#65237=CARTESIAN_POINT ( 'NONE',  ( 0.3610880125729999390, 1416.520646107730045, 227.1639889635980296 ) ) ;
#65241=CARTESIAN_POINT ( 'NONE',  ( -20.07643676080000006, 1508.105275053929972, 229.0283142729980170 ) ) ;
#65242=CARTESIAN_POINT ( 'NONE',  ( -25.36365838169201226, 1416.527675838791311, 269.4265581229172994 ) ) ;
#65243=CARTESIAN_POINT ( 'NONE',  ( -1.241688091069999889, 1409.462072764129971, 232.7892660792980166 ) ) ;
#65244=CARTESIAN_POINT ( 'NONE',  ( -12.45610846519999981, 1519.913060387329779, 189.3614993990980224 ) ) ;
#65246=CARTESIAN_POINT ( 'NONE',  ( -0.01303797444059440029, 1452.990214026840022, 183.2388976015689934 ) ) ;
#65247=CARTESIAN_POINT ( 'NONE',  ( -28.56580625744389934, 1440.913060387279984, 233.3672108470599937 ) ) ;
#65250=CARTESIAN_POINT ( 'NONE',  ( -0.3216917231897860052, 1465.013453958230002, 237.3752535225130202 ) ) ;
#65251=CARTESIAN_POINT ( 'NONE',  ( 6.266567495659089992, 1410.110873601029880, 270.0731530804650333 ) ) ;
#65255=VECTOR ( 'NONE', #15805, 1000.000000000000000 ) ;
#65256=CARTESIAN_POINT ( 'NONE',  ( 23.86480761299999998, 1410.397258296229893, 208.6144169840580105 ) ) ;
#65257=ADVANCED_FACE ( 'NONE', ( #3908 ), #83059, .T. ) ;
#65265=CARTESIAN_POINT ( 'NONE',  ( 11.86965601189266728, 1423.326342551363041, 137.0999999980981272 ) ) ;
#65267=ORIENTED_EDGE ( 'NONE', *, *, #100041, .T. ) ;
#65269=CARTESIAN_POINT ( 'NONE',  ( 18.96298731639999602, 1416.825532216530064, 210.2431968665279953 ) ) ;
#65276=FACE_OUTER_BOUND ( 'NONE', #75842, .T. ) ;
#65282=VERTEX_POINT ( 'NONE', #70566 ) ;
#65284=CARTESIAN_POINT ( 'NONE',  ( 24.35915060720000014, 1445.179795648890149, 214.1348656310980232 ) ) ;
#65285=CARTESIAN_POINT ( 'NONE',  ( 7.873429467257136771, 1438.236320869735664, 153.7470637502197519 ) ) ;
#65288=CARTESIAN_POINT ( 'NONE',  ( -26.63926297338899829, 1508.969960717049844, 201.4257229170909795 ) ) ;
#65290=CARTESIAN_POINT ( 'NONE',  ( -2.500000004229999906, 1447.770735518889978, 162.7884840773980102 ) ) ;
#65291=CARTESIAN_POINT ( 'NONE',  ( -19.05289845549999939, 1425.496478449930009, 224.1872183716980089 ) ) ;
#65292=CARTESIAN_POINT ( 'NONE',  ( -24.92720726409999799, 1436.178261884299900, 137.8894286862980039 ) ) ;
#65294=CARTESIAN_POINT ( 'NONE',  ( 19.64936965250000256, 1498.079962482629981, 189.3459704154979875 ) ) ;
#65297=CARTESIAN_POINT ( 'NONE',  ( 26.79413740735880367, 1436.761939593030093, 136.7822073642480234 ) ) ;
#65298=VERTEX_POINT ( 'NONE', #81127 ) ;
#65300=ADVANCED_FACE ( 'NONE', ( #4445 ), #72428, .F. ) ;
#65304=CARTESIAN_POINT ( 'NONE',  ( -0.1245423319220000102, 1416.981664566430027, 234.1917870246980158 ) ) ;
#65305=CARTESIAN_POINT ( 'NONE',  ( -13.44509113387912613, 1444.312623396357594, 186.9757151702101794 ) ) ;
#65306=B_SPLINE_SURFACE_WITH_KNOTS ( 'NONE', 3, 5, ( 
 ( #13395, #83368, #6113, #74454, #65499, #6669 ),
 ( #108582, #75000, #109150, #106918, #32434, #107469 ),
 ( #55989, #5013, #99060, #56539, #90667, #13951 ),
 ( #48140, #59312, #49794, #51437, #50893, #51999 ) ),
 .UNSPECIFIED., .F., .F., .F.,
 ( 4, 4 ),
 ( 6, 6 ),
 ( 5.479561967589999583, 5.505632813710000129 ),
 ( 0.000000000000000000, 1.000000000000000000 ),
 .UNSPECIFIED. ) ;
#65309=CARTESIAN_POINT ( 'NONE',  ( 12.53380499174499896, 1442.773887286369927, 169.4755105688890069 ) ) ;
#65311=DIRECTION ( 'NONE',  ( 0.9417419115949053898, -0.3363363969979660806, 0.000000000000000000 ) ) ;
#65312=CARTESIAN_POINT ( 'NONE',  ( -13.17497928872374402, 1443.091744202487234, 169.3947364813658680 ) ) ;
#65314=CARTESIAN_POINT ( 'NONE',  ( -14.44229636320000054, 1409.585625700530045, 226.2125909719979973 ) ) ;
#65318=EDGE_CURVE ( 'NONE', #75143, #103585, #835, .T. ) ;
#65325=CARTESIAN_POINT ( 'NONE',  ( -5.442004251730000242, 1468.737548879730184, 250.5651368667980421 ) ) ;
#65326=ADVANCED_FACE ( 'NONE', ( #66019 ), #55427, .F. ) ;
#65327=B_SPLINE_CURVE_WITH_KNOTS ( 'NONE', 3,
 ( #23363, #91676, #40175, #46950, #82170, #73233, #56438, #107376, #30106, #57553, #5470, #109048, #38513, #98421, #55899, #81610, #4914, #30671, #59204, #75980, #59746, #25554, #49696, #32861, #23901, #68167, #9335, #33971, #93322, #16584, #68708, #100616, #86036, #58641, #102274, #93866, #17135, #110132, #109591, #67052, #102812, #24453, #41282, #26106, #76528, #110680, #51324, #16050, #85460, #84914 ),
 .UNSPECIFIED., .F., .F.,
 ( 4, 2, 2, 2, 1, 2, 2, 2, 2, 1, 1, 2, 2, 2, 2, 2, 1, 1, 2, 2, 2, 2, 1, 1, 1, 2, 2, 2, 4 ),
 ( 0.000000000000000000, 0.06250000000014811763, 0.09375000000033439918, 0.1093750000004250211, 0.1171875000004729828, 0.1210937500004969636, 0.1250000000005209444, 0.1874999999982666643, 0.2187499999971440900, 0.2343749999966805442, 0.2421874999963559427, 0.2460937499961080022, 0.2499999999958600894, 0.3749999999961667885, 0.4374999999963201658, 0.4687499999963219977, 0.4843749999963902209, 0.4921874999964880315, 0.4960937499966067699, 0.4999999999967255082, 0.6249999999975833775, 0.6874999999980123677, 0.7187499999982158716, 0.7343749999983176791, 0.7421874999983686383, 0.7460937499983835153, 0.7499999999983983923, 0.8749999999991993072, 1.000000000000000000 ),
 .UNSPECIFIED. ) ;
#65329=CARTESIAN_POINT ( 'NONE',  ( -11.25663278669999912, 1433.724203657259977, 151.5578573542979939 ) ) ;
#65333=CARTESIAN_POINT ( 'NONE',  ( 16.06428792994640276, 1414.913060387329779, 208.9262477894010033 ) ) ;
#65340=CARTESIAN_POINT ( 'NONE',  ( -7.587845399210802810, 1509.305955895972602, 238.1603715047018852 ) ) ;
#65341=CARTESIAN_POINT ( 'NONE',  ( 7.547424700377989516E-09, 1409.628684922620096, 259.4492681075740279 ) ) ;
#65342=ORIENTED_EDGE ( 'NONE', *, *, #2908, .T. ) ;
#65344=CARTESIAN_POINT ( 'NONE',  ( -11.85978036263550095, 1431.894859516819906, 149.9645931322949934 ) ) ;
#65347=CARTESIAN_POINT ( 'NONE',  ( -6.238302164579999420, 1471.462343947730005, 269.8685151816979442 ) ) ;
#65349=CARTESIAN_POINT ( 'NONE',  ( 3.218260492609999801, 1432.346960983880081, 155.4230413404980027 ) ) ;
#65350=CARTESIAN_POINT ( 'NONE',  ( 33.92637545789110476, 1451.728355673910073, 135.1498132472949862 ) ) ;
#65351=CARTESIAN_POINT ( 'NONE',  ( 0.2864299555745510317, 1451.125108261750029, 182.1816743638030118 ) ) ;
#65356=CARTESIAN_POINT ( 'NONE',  ( -27.50386026148250096, 1412.567279178109857, 267.5294091190150425 ) ) ;
#65358=CARTESIAN_POINT ( 'NONE',  ( -3.543960468857640045, 1501.780698723729984, 181.2047494549660200 ) ) ;
#65360=EDGE_LOOP ( 'NONE', ( #96782, #48010, #23987, #19596 ) ) ;
#65361=VERTEX_POINT ( 'NONE', #56781 ) ;
#65363=CARTESIAN_POINT ( 'NONE',  ( 4.583195184658291232, 1423.744221409726151, 183.8097901654739985 ) ) ;
#65364=CARTESIAN_POINT ( 'NONE',  ( 41.39923983940850150, 1444.121112939410068, 136.4829021321949938 ) ) ;
#65368=CARTESIAN_POINT ( 'NONE',  ( -16.22390639470000195, 1455.453005806130022, 189.2659189164979807 ) ) ;
#65369=CARTESIAN_POINT ( 'NONE',  ( -2.182017354322035807, 1449.976583366785462, 182.9105004910145169 ) ) ;
#65370=ORIENTED_EDGE ( 'NONE', *, *, #34944, .F. ) ;
#65371=DIRECTION ( 'NONE',  ( 1.000000000000000000, -0.000000000000000000, -0.000000000000000000 ) ) ;
#65374=CARTESIAN_POINT ( 'NONE',  ( -40.60082915980000706, 1447.775075536270379, 135.1193778666983292 ) ) ;
#65377=CARTESIAN_POINT ( 'NONE',  ( -42.85030160454469694, 1440.913048488810091, 270.2009464246669950 ) ) ;
#65379=CARTESIAN_POINT ( 'NONE',  ( -3.412833957800000206, 1396.032239175229961, 198.2233776492980155 ) ) ;
#65384=CARTESIAN_POINT ( 'NONE',  ( 3.747137648998505544, 1425.479684836872821, 185.1860802519873062 ) ) ;
#65386=CARTESIAN_POINT ( 'NONE',  ( -2.500000000000000000, 1419.471702562262180, 139.8968355505663794 ) ) ;
#65387=CARTESIAN_POINT ( 'NONE',  ( -0.03395478378652629775, 1410.184876381479853, 185.0299449505969847 ) ) ;
#65392=CARTESIAN_POINT ( 'NONE',  ( 18.80400139965103889, 1425.877415487390863, 225.3118880953776966 ) ) ;
#65396=CARTESIAN_POINT ( 'NONE',  ( -33.91369114127179785, 1451.728768196330066, 134.7398512173020038 ) ) ;
#65398=CARTESIAN_POINT ( 'NONE',  ( -23.50846456196114431, 1448.274227622677017, 215.6832531493611782 ) ) ;
#65401=CARTESIAN_POINT ( 'NONE',  ( 25.07770885454710097, 1451.593447514730087, 137.0505554713550112 ) ) ;
#65402=CARTESIAN_POINT ( 'NONE',  ( 13.57591587739999994, 1415.063410501330054, 197.7477002572979927 ) ) ;
#65404=CARTESIAN_POINT ( 'NONE',  ( -10.85852385830536448, 1424.794007418652882, 138.1924915167475660 ) ) ;
#65408=CARTESIAN_POINT ( 'NONE',  ( 24.20724779095554879, 1446.232668714965484, 214.6598422090904705 ) ) ;
#65409=CARTESIAN_POINT ( 'NONE',  ( 2.500000000000079936, 1439.283171039279978, 159.9469904227869961 ) ) ;
#65414=CARTESIAN_POINT ( 'NONE',  ( -1.476727087160000007, 1474.160226259529963, 270.1373298219979802 ) ) ;
#65415=CARTESIAN_POINT ( 'NONE',  ( 15.56469051819999905, 1506.798305132829910, 225.0756798403980099 ) ) ;
#65417=CIRCLE ( 'NONE', #13580, 26.99999999999999645 ) ;
#65419=CARTESIAN_POINT ( 'NONE',  ( 21.61286264580910199, 1509.680930481669975, 229.7181273278760045 ) ) ;
#65420=CARTESIAN_POINT ( 'NONE',  ( 11.44767209065952684, 1425.800566880429642, 139.0551406208118124 ) ) ;
#65421=DIRECTION ( 'NONE',  ( 0.08338001035575019759, 5.083217065477059319E-13, 0.9965178241622549837 ) ) ;
#65422=CARTESIAN_POINT ( 'NONE',  ( -1.730624838930999942, 1477.776000856039900, 183.0333778651980197 ) ) ;
#65426=CARTESIAN_POINT ( 'NONE',  ( 30.55220783223240133, 1440.913060385000108, 240.0655027828689754 ) ) ;
#65429=CARTESIAN_POINT ( 'NONE',  ( 13.02322702449999881, 1416.825784017130218, 221.6328457789979893 ) ) ;
#65431=ORIENTED_EDGE ( 'NONE', *, *, #30273, .F. ) ;
#65432=CARTESIAN_POINT ( 'NONE',  ( 11.23388613411650105, 1443.913060387330006, 207.0699376370760092 ) ) ;
#65436=CARTESIAN_POINT ( 'NONE',  ( 1.399926847669999974, 1507.072115598929940, 236.8180522793980174 ) ) ;
#65437=CARTESIAN_POINT ( 'NONE',  ( -10.81507089441019964, 1424.921187596680056, 144.1620444830689962 ) ) ;
#65442=CARTESIAN_POINT ( 'NONE',  ( 2.499944985410900156, 1419.419865434090070, 142.4063531947399781 ) ) ;
#65444=( BOUNDED_CURVE ( )  B_SPLINE_CURVE ( 3, ( #1029, #86658, #68238, #8284 ),
 .UNSPECIFIED., .F., .F. ) 
 B_SPLINE_CURVE_WITH_KNOTS ( ( 4, 4 ),
 ( 3.097740324398939649, 3.109955547998598746 ),
 .UNSPECIFIED. ) 
 CURVE ( )  GEOMETRIC_REPRESENTATION_ITEM ( )  RATIONAL_B_SPLINE_CURVE ( ( 1.000000000000000000, 0.9999875657313538335, 0.9999875657313538335, 1.000000000000000000 ) ) 
 REPRESENTATION_ITEM ( '' )  );
#65445=CARTESIAN_POINT ( 'NONE',  ( 2.933761806229999713, 1464.631290085030059, 236.6723689097979673 ) ) ;
#65448=CARTESIAN_POINT ( 'NONE',  ( -1.033934541210000058, 1452.678099303230056, 183.5143811305979966 ) ) ;
#65453=CARTESIAN_POINT ( 'NONE',  ( -16.36863935783290103, 1414.913057862230062, 209.3429184488039709 ) ) ;
#65454=ORIENTED_EDGE ( 'NONE', *, *, #46604, .T. ) ;
#65456=CIRCLE ( 'NONE', #36823, 1.999999999999911182 ) ;
#65458=CARTESIAN_POINT ( 'NONE',  ( 35.50394988412039510, 1437.266775526519950, 136.5354948351899793 ) ) ;
#65459=CARTESIAN_POINT ( 'NONE',  ( -0.5620977654635980203, 1416.851343899799986, 227.7685710128770040 ) ) ;
#65460=CARTESIAN_POINT ( 'NONE',  ( -11.60004869884791212, 1426.686844843452036, 134.5518989175760396 ) ) ;
#65464=CARTESIAN_POINT ( 'NONE',  ( 12.83740251975140012, 1409.361352361609988, 201.4721406717710011 ) ) ;
#65465=CARTESIAN_POINT ( 'NONE',  ( 18.03151512659999867, 1424.669534113930013, 225.2917716953979834 ) ) ;
#65467=CARTESIAN_POINT ( 'NONE',  ( -19.17357988869999730, 1470.688427666330199, 190.5575023379979882 ) ) ;
#65468=DIRECTION ( 'NONE',  ( 0.4794255386025446652, -1.809663530140880534E-11, 0.8775825618912787007 ) ) ;
#65470=CARTESIAN_POINT ( 'NONE',  ( -2.499996183066730104, 1449.218566323959976, 183.0817960734219696 ) ) ;
#65474=CARTESIAN_POINT ( 'NONE',  ( 13.86092937120000101, 1410.765486813630105, 191.1266627561979874 ) ) ;
#65475=CARTESIAN_POINT ( 'NONE',  ( 2.029578523264960108E-10, 1465.856113608230089, 240.9469248189070072 ) ) ;
#65476=CARTESIAN_POINT ( 'NONE',  ( -20.28392256243369829, 1497.626837986160126, 190.6863869125700148 ) ) ;
#65477=CARTESIAN_POINT ( 'NONE',  ( 0.000000000000000000, 1414.913060387329779, 221.6218459616979999 ) ) ;
#65479=CARTESIAN_POINT ( 'NONE',  ( -1.212266992759999829, 1483.398284593029985, 182.2695464371980165 ) ) ;
#65481=CARTESIAN_POINT ( 'NONE',  ( -46.15015871273919856, 1440.464460849770148, 268.2045569567199550 ) ) ;
#65482=CARTESIAN_POINT ( 'NONE',  ( 13.39710138444150012, 1508.017386564119988, 233.1392620568510097 ) ) ;
#65483=CARTESIAN_POINT ( 'NONE',  ( -21.33942536743590068, 1477.920010453090072, 208.5333634439200239 ) ) ;
#65485=CARTESIAN_POINT ( 'NONE',  ( 5.082258451441009406, 1407.428259223129999, 221.1577315719200101 ) ) ;
#65486=EDGE_CURVE ( 'NONE', #99871, #32822, #2603, .T. ) ;
#65490=CARTESIAN_POINT ( 'NONE',  ( 27.90885394449999879, 1424.419860138930062, 250.2249407727979928 ) ) ;
#65492=CARTESIAN_POINT ( 'NONE',  ( -2.545491131529999951, 1499.389042279630075, 181.1800920301980113 ) ) ;
#65495=CARTESIAN_POINT ( 'NONE',  ( 1.469929971929456070, 1507.915326702531047, 180.9459708344064666 ) ) ;
#65496=CARTESIAN_POINT ( 'NONE',  ( -27.70845745580000141, 1431.442878273549923, 238.1060641559980127 ) ) ;
#65497=CARTESIAN_POINT ( 'NONE',  ( -29.43798506786606950, 1509.956740567253064, 206.0314242323168230 ) ) ;
#65498=CARTESIAN_POINT ( 'NONE',  ( -10.75854853582960047, 1452.537363593840155, 150.2728578400229935 ) ) ;
#65499=CARTESIAN_POINT ( 'NONE',  ( -18.79734781009999978, 1416.844618635330107, 208.4088319070980049 ) ) ;
#65502=CARTESIAN_POINT ( 'NONE',  ( 6.480125363573969479E-05, 1410.239966284670118, 269.6149245224239621 ) ) ;
#65503=CARTESIAN_POINT ( 'NONE',  ( 16.89525345604750228, 1422.350075462329869, 226.9164778485460090 ) ) ;
#65504=CARTESIAN_POINT ( 'NONE',  ( -4.161595075237580765, 1448.982995846620042, 185.0801961897900298 ) ) ;
#65508=CARTESIAN_POINT ( 'NONE',  ( -22.93660144289669844, 1409.723673488970007, 209.0949845260039979 ) ) ;
#65509=ORIENTED_EDGE ( 'NONE', *, *, #14612, .F. ) ;
#65510=CARTESIAN_POINT ( 'NONE',  ( 0.08461443304019999889, 1416.823634022930037, 227.2251189671980001 ) ) ;
#65512=CARTESIAN_POINT ( 'NONE',  ( -2.907264515414449857, 1451.960119877520128, 184.7556101994359778 ) ) ;
#65513=CARTESIAN_POINT ( 'NONE',  ( -1.368191914778909890, 1419.344528075180278, 185.2221190139939893 ) ) ;
#65517=CARTESIAN_POINT ( 'NONE',  ( 41.65757230853200355, 1455.325850625539942, 266.3038443812790206 ) ) ;
#65518=CARTESIAN_POINT ( 'NONE',  ( -11.80289467576660023, 1415.088012641449950, 221.3076621094219831 ) ) ;
#65524=CARTESIAN_POINT ( 'NONE',  ( 13.28675557712670674, 1443.221090981650377, 187.6942237735384253 ) ) ;
#65534=B_SPLINE_CURVE_WITH_KNOTS ( 'NONE', 3,
 ( #44165, #11655, #54239, #96214, #18373, #105731, #12196, #53692, #86701, #27904, #53123, #104611, #10553, #1616, #79964, #62087, #61530, #95658, #45831, #18925, #19488, #87833, #11121, #56423, #38498, #21124, #5454, #29550, #12754, #3837, #48017, #100059, #13830, #39037, #73216, #48580, #80521, #65936, #72675, #82154, #39613, #46936, #81055, #65387, #90004, #90553 ),
 .UNSPECIFIED., .F., .F.,
 ( 4, 3, 3, 3, 3, 3, 3, 3, 3, 3, 3, 3, 3, 3, 3, 4 ),
 ( 0.000000000000000000, 0.09251053440245410320, 0.1819424025277689982, 0.2703167020720390057, 0.3599760602905189844, 0.4496354185090000177, 0.6562016036042499501, 0.8628455277292459424, 1.069372843309620125, 1.260326837218950002, 1.275900158890000080, 1.435752599818300057, 1.593630893054559960, 1.750171058644690136, 1.905888283666149929, 2.061605508687600175 ),
 .UNSPECIFIED. ) ;
#65536=FACE_OUTER_BOUND ( 'NONE', #96877, .T. ) ;
#65537=CARTESIAN_POINT ( 'NONE',  ( -16.79695581410840077, 1415.044791756060022, 191.6206649154599688 ) ) ;
#65540=CARTESIAN_POINT ( 'NONE',  ( -24.34259636588380005, 1508.950977677119909, 222.4692572808739897 ) ) ;
#65544=CARTESIAN_POINT ( 'NONE',  ( -1.347412987175396371, 1395.960113085665398, 201.1218459616979999 ) ) ;
#65553=CARTESIAN_POINT ( 'NONE',  ( 11.77548435589999976, 1433.640636952740124, 150.8383593496980097 ) ) ;
#65554=CARTESIAN_POINT ( 'NONE',  ( 36.06124926539999365, 1440.913060387330006, 262.6648722463980334 ) ) ;
#65556=CARTESIAN_POINT ( 'NONE',  ( 11.81707110430000007, 1430.266231075130008, 147.2485970657980090 ) ) ;
#65557=CARTESIAN_POINT ( 'NONE',  ( 0.2576823252080000515, 1419.224537961029910, 184.6439154818979773 ) ) ;
#65561=CARTESIAN_POINT ( 'NONE',  ( -4.500000000000000000, 1425.929641636930000, 184.1455913746980002 ) ) ;
#65562=B_SPLINE_CURVE_WITH_KNOTS ( 'NONE', 5,
 ( #105088, #36780, #46315, #106188, #88287, #89929 ),
 .UNSPECIFIED., .F., .F.,
 ( 6, 6 ),
 ( 0.000000000000000000, 1.000000000000000000 ),
 .UNSPECIFIED. ) ;
#65563=CARTESIAN_POINT ( 'NONE',  ( 5.021037906353149616, 1440.968375784319960, 155.1907003990020257 ) ) ;
#65565=CARTESIAN_POINT ( 'NONE',  ( -16.63500958477349911, 1409.493940183780069, 193.4350317777050066 ) ) ;
#65567=CARTESIAN_POINT ( 'NONE',  ( 4.026786250540000722, 1408.413060387330006, 146.1721969590979882 ) ) ;
#65569=CARTESIAN_POINT ( 'NONE',  ( -9.612666206359998355, 1414.913060387329779, 222.3789311915979852 ) ) ;
#65570=CARTESIAN_POINT ( 'NONE',  ( 0.2088027491384900070, 1458.021659680169932, 183.0379629500139913 ) ) ;
#65571=CARTESIAN_POINT ( 'NONE',  ( -12.86051124159999937, 1409.184418768930072, 216.3873131214179750 ) ) ;
#65572=ORIENTED_EDGE ( 'NONE', *, *, #109978, .F. ) ;
#65575=CARTESIAN_POINT ( 'NONE',  ( 13.80544311399999913, 1434.979600114139885, 148.5019818398979794 ) ) ;
#65576=CARTESIAN_POINT ( 'NONE',  ( -26.80766422789999837, 1435.433722594319988, 135.7240085096979954 ) ) ;
#65577=CARTESIAN_POINT ( 'NONE',  ( 10.24908546679999866, 1441.239651135290160, 187.1830758738979910 ) ) ;
#65584=CARTESIAN_POINT ( 'NONE',  ( 13.37404851082409962, 1507.496393256099964, 233.0472755390670159 ) ) ;
#65585=CARTESIAN_POINT ( 'NONE',  ( 39.19951531957330104, 1423.398545273861146, 269.1491992711760872 ) ) ;
#65587=CARTESIAN_POINT ( 'NONE',  ( 20.32975030060803334, 1508.870389961778528, 189.2250207761221930 ) ) ;
#65588=CARTESIAN_POINT ( 'NONE',  ( 2.661634141329999537, 1431.451308766379952, 184.1577198843980057 ) ) ;
#65591=CARTESIAN_POINT ( 'NONE',  ( -26.80425587306198310, 1435.467044139958489, 135.6517718923794575 ) ) ;
#65592=ORIENTED_EDGE ( 'NONE', *, *, #86576, .F. ) ;
#65593=CARTESIAN_POINT ( 'NONE',  ( -28.49886664254099600, 1509.035040377790210, 208.7883124179550123 ) ) ;
#65594=CARTESIAN_POINT ( 'NONE',  ( -16.03783333616070195, 1409.473006842159975, 225.3014575052910118 ) ) ;
#65602=CARTESIAN_POINT ( 'NONE',  ( -11.30241272700000010, 1414.983773852829927, 195.8621715883979846 ) ) ;
#65603=CARTESIAN_POINT ( 'NONE',  ( 0.4070099242259999639, 1465.094834125830175, 236.9943866744980028 ) ) ;
#65604=EDGE_CURVE ( 'NONE', #99690, #30233, #58993, .T. ) ;
#65605=CARTESIAN_POINT ( 'NONE',  ( 23.01300307269999834, 1410.211808750929777, 212.8080261142179666 ) ) ;
#65608=CARTESIAN_POINT ( 'NONE',  ( -16.55421215910000043, 1423.367941342530003, 228.9006519623980012 ) ) ;
#65610=CARTESIAN_POINT ( 'NONE',  ( 21.99231067417252206, 1506.446781340372127, 208.8672818357590018 ) ) ;
#65613=CARTESIAN_POINT ( 'NONE',  ( 13.91344329460000040, 1453.313060387329870, 224.4164659125979995 ) ) ;
#65614=CARTESIAN_POINT ( 'NONE',  ( -0.7334337980199999718, 1417.382035507929913, 235.1308628909980030 ) ) ;
#65617=CARTESIAN_POINT ( 'NONE',  ( -12.70480096745579957, 1484.837292199019885, 185.9669015828420129 ) ) ;
#65618=ORIENTED_EDGE ( 'NONE', *, *, #58614, .F. ) ;
#65620=CARTESIAN_POINT ( 'NONE',  ( -4.225202376359490586, 1441.574362862340195, 166.3910519188600006 ) ) ;
#65623=EDGE_LOOP ( 'NONE', ( #56280, #99259, #14812, #9605 ) ) ;
#65629=CARTESIAN_POINT ( 'NONE',  ( -11.44354861750966279, 1425.477604805352030, 144.5838835533737381 ) ) ;
#65630=CARTESIAN_POINT ( 'NONE',  ( 15.84154831066869917, 1409.491884921769952, 192.6660917361010092 ) ) ;
#65632=FACE_OUTER_BOUND ( 'NONE', #63315, .T. ) ;
#65634=CARTESIAN_POINT ( 'NONE',  ( 16.86259531663306532, 1460.525699792653995, 228.8369507918937700 ) ) ;
#65635=CARTESIAN_POINT ( 'NONE',  ( 8.921631616102885687, 1502.413060387330006, 225.4527830926159595 ) ) ;
#65636=CARTESIAN_POINT ( 'NONE',  ( 44.93136303390000563, 1440.913033067569813, 269.6838066906980202 ) ) ;
#65640=ORIENTED_EDGE ( 'NONE', *, *, #66585, .T. ) ;
#65642=CARTESIAN_POINT ( 'NONE',  ( 10.06505727382652715, 1410.639190484854907, 229.7922706876150301 ) ) ;
#65643=CYLINDRICAL_SURFACE ( 'NONE', #106428, 1.999999999999902967 ) ;
#65644=CARTESIAN_POINT ( 'NONE',  ( 0.1475592169000000120, 1451.689388021529794, 183.0405803991980065 ) ) ;
#65649=CARTESIAN_POINT ( 'NONE',  ( 40.71747595459699909, 1448.637563191980007, 135.6938357208099717 ) ) ;
#65650=CARTESIAN_POINT ( 'NONE',  ( -5426.659240077532559, 2833.746317950420234, 8449.939303199314963 ) ) ;
#65651=CARTESIAN_POINT ( 'NONE',  ( 26.64405787239999768, 1440.573177016219915, 137.3591247521979994 ) ) ;
#65658=CARTESIAN_POINT ( 'NONE',  ( 41.96952434445400115, 1440.913060387330006, 269.5508532369769910 ) ) ;
#65659=CARTESIAN_POINT ( 'NONE',  ( -0.002355423392913324858, 1451.792606406385175, 154.0462491319130436 ) ) ;
#65661=CARTESIAN_POINT ( 'NONE',  ( -0.2565269630447720162, 1450.904102268370025, 181.8958596656970030 ) ) ;
#65665=CARTESIAN_POINT ( 'NONE',  ( -4.288575270049999943, 1421.887819494029827, 185.0877211516979912 ) ) ;
#65667=CARTESIAN_POINT ( 'NONE',  ( -0.7082213409149999972, 1508.873178418929911, 179.8394376137979975 ) ) ;
#65669=CARTESIAN_POINT ( 'NONE',  ( 10.81507089421240053, 1424.921187596799882, 144.1620444706739761 ) ) ;
#65670=CARTESIAN_POINT ( 'NONE',  ( 13.76459360349999983, 1460.937369267029908, 231.9016751017979914 ) ) ;
#65671=CARTESIAN_POINT ( 'NONE',  ( -11.60004869885203860, 1423.522019188771310, 137.0424394678681210 ) ) ;
#65672=CARTESIAN_POINT ( 'NONE',  ( -4.572909471579259311, 1422.074987962655996, 184.6258731943378280 ) ) ;
#65678=CARTESIAN_POINT ( 'NONE',  ( 17.06845921355082041, 1448.846822804656540, 218.4183351126684727 ) ) ;
#65680=CARTESIAN_POINT ( 'NONE',  ( 18.60392304109999984, 1508.243836144429906, 188.5101919634980163 ) ) ;
#65683=VERTEX_POINT ( 'NONE', #93121 ) ;
#65685=CARTESIAN_POINT ( 'NONE',  ( 11.20759482449999922, 1458.854746706030028, 217.3836589402779964 ) ) ;
#65686=CARTESIAN_POINT ( 'NONE',  ( -10.94598488280000126, 1430.643605498629995, 151.5761596627980055 ) ) ;
#65687=CARTESIAN_POINT ( 'NONE',  ( 19.07077998173900113, 1456.927795362189954, 225.2567787181259860 ) ) ;
#65688=EDGE_CURVE ( 'NONE', #104987, #68277, #48946, .T. ) ;
#65690=FACE_OUTER_BOUND ( 'NONE', #85879, .T. ) ;
#65692=CARTESIAN_POINT ( 'NONE',  ( 12.69201959859999995, 1445.029817614240073, 186.3520294606980201 ) ) ;
#65693=CARTESIAN_POINT ( 'NONE',  ( -19.37516407789999917, 1457.447849671029871, 226.2756290344979959 ) ) ;
#65696=CARTESIAN_POINT ( 'NONE',  ( -3.054816022670000297, 1485.996906138130043, 182.1538610966980229 ) ) ;
#65699=CARTESIAN_POINT ( 'NONE',  ( 7.002505146659999902, 1406.898447550930086, 269.4815251353980443 ) ) ;
#65700=CARTESIAN_POINT ( 'NONE',  ( -0.05604939685589999804, 1409.080516226629925, 185.5803113818979853 ) ) ;
#65702=CARTESIAN_POINT ( 'NONE',  ( 23.41305660651092424, 1433.448859892850123, 215.2039121327621274 ) ) ;
#65704=CARTESIAN_POINT ( 'NONE',  ( 28.19408364699999936, 1508.123162656630029, 209.7484684564449822 ) ) ;
#65706=CARTESIAN_POINT ( 'NONE',  ( -2.491511770217889943, 1449.258138113479845, 154.2481093272120063 ) ) ;
#65707=CARTESIAN_POINT ( 'NONE',  ( -1.641945290704282190, 1450.652787028681360, 183.1941434156354660 ) ) ;
#65708=CARTESIAN_POINT ( 'NONE',  ( -19.86849070297746067, 1485.435531518196740, 190.6411886671614582 ) ) ;
#65709=CARTESIAN_POINT ( 'NONE',  ( -14.36283523570150145, 1416.196255300880011, 221.2942896565629951 ) ) ;
#65711=CARTESIAN_POINT ( 'NONE',  ( -8.827869491105628796, 1409.221336382960317, 197.0457684614559923 ) ) ;
#65712=AXIS2_PLACEMENT_3D ( 'NONE', #52343, #61311, #18692 ) ;
#65713=CARTESIAN_POINT ( 'NONE',  ( 4.363119589138680254, 1423.854801764450031, 183.5697712894070150 ) ) ;
#65714=CARTESIAN_POINT ( 'NONE',  ( 3.685495795909999650, 1441.157097705729939, 159.2182474352979966 ) ) ;
#65715=CARTESIAN_POINT ( 'NONE',  ( -3.774051438349999898, 1475.935069928129906, 268.4776602676979564 ) ) ;
#65716=B_SPLINE_CURVE_WITH_KNOTS ( 'NONE', 5,
 ( #59076, #14280, #57968, #75326, #67479, #90991, #14832, #32200, #42257, #7547, #92103, #15379, #57431, #48471, #66926 ),
 .UNSPECIFIED., .F., .F.,
 ( 6, 3, 3, 3, 6 ),
 ( 0.000000000000000000, 0.1467687781236080569, 0.3860735318475042033, 0.6253782855714004052, 1.000000000000000000 ),
 .UNSPECIFIED. ) ;
#65717=CARTESIAN_POINT ( 'NONE',  ( -4.240750497009450726, 1446.388360617959961, 162.7103197369740144 ) ) ;
#65721=CARTESIAN_POINT ( 'NONE',  ( 2.370878938589389140, 1508.995853304402544, 237.7496061730882673 ) ) ;
#65727=CARTESIAN_POINT ( 'NONE',  ( -17.98939367079999840, 1410.465183412730084, 195.2754043712980092 ) ) ;
#65729=CARTESIAN_POINT ( 'NONE',  ( -22.40611913229999885, 1411.902937806130012, 270.0285353679980176 ) ) ;
#65732=CARTESIAN_POINT ( 'NONE',  ( -1.709547000564935804, 1410.351682048799603, 232.8846474005925415 ) ) ;
#65735=CARTESIAN_POINT ( 'NONE',  ( 11.64281719679999938, 1426.759312292029790, 137.4371925635979892 ) ) ;
#65737=FACE_OUTER_BOUND ( 'NONE', #71752, .T. ) ;
#65739=CARTESIAN_POINT ( 'NONE',  ( 40.32490366350000244, 1444.177947227670074, 137.1005529477980076 ) ) ;
#65740=B_SPLINE_CURVE_WITH_KNOTS ( 'NONE', 3,
 ( #57822, #66780, #101986, #84641, #7938, #42107, #51063, #76254, #93583, #85193, #9043, #25824, #42654, #60025 ),
 .UNSPECIFIED., .F., .F.,
 ( 4, 2, 1, 1, 1, 1, 2, 2, 4 ),
 ( 0.000000000000000000, 0.2499999999999296119, 0.3749999999998988587, 0.4374999999998812616, 0.4687499999998721023, 0.4843749999998657740, 0.4921874999998628319, 0.4999999999998597788, 1.000000000000000000 ),
 .UNSPECIFIED. ) ;
#65743=AXIS2_PLACEMENT_3D ( 'NONE', #39075, #99528, #47505 ) ;
#65744=CARTESIAN_POINT ( 'NONE',  ( -13.56343219680000090, 1416.311719779230089, 221.8446948800979897 ) ) ;
#65748=CARTESIAN_POINT ( 'NONE',  ( 19.77968988581690013, 1507.818078778149811, 229.2755617519239877 ) ) ;
#65750=ORIENTED_EDGE ( 'NONE', *, *, #7769, .T. ) ;
#65752=CARTESIAN_POINT ( 'NONE',  ( -10.98463078130000170, 1397.930555569230137, 216.8780141624080215 ) ) ;
#65753=CARTESIAN_POINT ( 'NONE',  ( -21.49107218889999871, 1409.827664247030043, 214.8354072608880188 ) ) ;
#65755=CARTESIAN_POINT ( 'NONE',  ( -13.01504163501136802, 1444.865561423528334, 169.4190877585964472 ) ) ;
#65756=CARTESIAN_POINT ( 'NONE',  ( 21.64833465062206841, 1509.708313661343936, 229.4903290947612504 ) ) ;
#65759=CARTESIAN_POINT ( 'NONE',  ( -2.253566441613126910E-10, 1426.918876941764893, 134.0999999980980135 ) ) ;
#65760=CARTESIAN_POINT ( 'NONE',  ( -14.19446170199559987, 1509.352195767969761, 183.2680670197790107 ) ) ;
#65761=CARTESIAN_POINT ( 'NONE',  ( 3.344599308599999876, 1449.236580124219927, 184.0881402263979965 ) ) ;
#65764=CARTESIAN_POINT ( 'NONE',  ( 7.695515934043100081, 1396.181793810000045, 201.1942046015250014 ) ) ;
#65765=CARTESIAN_POINT ( 'NONE',  ( 0.6414547015549999509, 1416.067629290630066, 190.6212042380979881 ) ) ;
#65766=CARTESIAN_POINT ( 'NONE',  ( 11.68304837730000045, 1426.648785231629972, 147.7179971800979956 ) ) ;
#65767=CARTESIAN_POINT ( 'NONE',  ( 8.590023996720262289, 1509.213085694760821, 181.0924370714511440 ) ) ;
#65769=CARTESIAN_POINT ( 'NONE',  ( 12.97954183294099906, 1434.770645735859944, 149.2712075224750095 ) ) ;
#65770=CARTESIAN_POINT ( 'NONE',  ( 2.500000195207620290, 1448.894380947069976, 182.3534016008459844 ) ) ;
#65774=CARTESIAN_POINT ( 'NONE',  ( -17.07194142410000026, 1458.267783243329859, 228.1906384420979919 ) ) ;
#65775=CARTESIAN_POINT ( 'NONE',  ( -13.48270089159999863, 1461.679658884430182, 230.3973540560979814 ) ) ;
#65782=CARTESIAN_POINT ( 'NONE',  ( 2.500000000000000000, 1448.216386378729794, 167.2100391009490181 ) ) ;
#65788=CARTESIAN_POINT ( 'NONE',  ( -20.11539149109999869, 1508.359231761630099, 229.0631537309980104 ) ) ;
#65789=CARTESIAN_POINT ( 'NONE',  ( -29.98137141540891903, 1419.563817194629792, 269.4706080157307042 ) ) ;
#65791=CARTESIAN_POINT ( 'NONE',  ( -0.3266950887954889748, 1415.429375168339902, 226.7788835740809930 ) ) ;
#65793=CARTESIAN_POINT ( 'NONE',  ( 24.56509548029999834, 1440.948408367609773, 213.0043227547379843 ) ) ;
#65794=CARTESIAN_POINT ( 'NONE',  ( -27.22136134539860208, 1440.913060408979845, 227.8408515943710029 ) ) ;
#65797=CARTESIAN_POINT ( 'NONE',  ( -0.4726113425640879884, 1465.085982962939852, 236.9699332437729993 ) ) ;
#65798=CARTESIAN_POINT ( 'NONE',  ( 8.322172261349999545, 1408.217606231929949, 270.1222559176979416 ) ) ;
#65801=CARTESIAN_POINT ( 'NONE',  ( 24.10111531969999987, 1410.845843824029998, 208.8643776631820117 ) ) ;
#65810=CARTESIAN_POINT ( 'NONE',  ( 0.4542301007209999519, 1418.679722665129930, 184.7067504190980003 ) ) ;
#65811=CARTESIAN_POINT ( 'NONE',  ( 10.97799415081370000, 1432.849868510099896, 151.7696862706320076 ) ) ;
#65816=FACE_OUTER_BOUND ( 'NONE', #107355, .T. ) ;
#65826=CARTESIAN_POINT ( 'NONE',  ( -29.31378141421994599, 1450.601296382764986, 136.3806906879467249 ) ) ;
#65828=VECTOR ( 'NONE', #20637, 1000.000000000000000 ) ;
#65832=CARTESIAN_POINT ( 'NONE',  ( 0.08771972261379999691, 1467.621255356930078, 229.4461896818980051 ) ) ;
#65837=CARTESIAN_POINT ( 'NONE',  ( 25.97508195616575577, 1450.776908619160849, 136.7573643306957933 ) ) ;
#65838=CARTESIAN_POINT ( 'NONE',  ( 15.21669680536202485, 1420.730405204549470, 227.8538932186329191 ) ) ;
#65839=CARTESIAN_POINT ( 'NONE',  ( 40.26396420611710170, 1444.186530323160014, 137.1012295353969819 ) ) ;
#65840=CARTESIAN_POINT ( 'NONE',  ( -19.52413277859999852, 1426.414269502929756, 225.5212833970979887 ) ) ;
#65843=CARTESIAN_POINT ( 'NONE',  ( 18.72056918370000034, 1488.305367430329852, 189.2161702103979906 ) ) ;
#65846=CARTESIAN_POINT ( 'NONE',  ( -29.77122833299150173, 1462.416651616063064, 269.4683881299069412 ) ) ;
#65847=ORIENTED_EDGE ( 'NONE', *, *, #18037, .T. ) ;
#65849=CARTESIAN_POINT ( 'NONE',  ( 10.26696809936899513, 1506.473666147782524, 189.6435125623585520 ) ) ;
#65852=CARTESIAN_POINT ( 'NONE',  ( -5.164876290100000489, 1519.913060387329779, 231.9023197776979828 ) ) ;
#65854=CARTESIAN_POINT ( 'NONE',  ( -12.63725134787329196, 1442.793345748885940, 186.0969688226275593 ) ) ;
#65860=CARTESIAN_POINT ( 'NONE',  ( 18.27452169968656293, 1424.830735475889469, 227.7277621568871098 ) ) ;
#65861=B_SPLINE_CURVE_WITH_KNOTS ( 'NONE', 5,
 ( #27267, #20496, #96691, #12118, #78780, #104527, #11026, #36775, #26703, #36223, #87178, #61450 ),
 .UNSPECIFIED., .F., .F.,
 ( 6, 3, 3, 6 ),
 ( 0.000000000000000000, 0.2059268257605248176, 0.6177804772432864411, 1.000000000000000000 ),
 .UNSPECIFIED. ) ;
#65862=CARTESIAN_POINT ( 'NONE',  ( -13.14393378692782299, 1443.063090240467091, 169.3993137622184690 ) ) ;
#65863=CARTESIAN_POINT ( 'NONE',  ( 18.02077237764099849, 1424.321284042770003, 225.1939596517550228 ) ) ;
#65865=CARTESIAN_POINT ( 'NONE',  ( -0.2707663694140940436, 1415.088012641449950, 192.1592658664270061 ) ) ;
#65866=CARTESIAN_POINT ( 'NONE',  ( 21.91509308718912763, 1509.516311612268055, 226.8168978660500841 ) ) ;
#65869=CARTESIAN_POINT ( 'NONE',  ( 16.20819593131900049, 1414.913060387399810, 209.7580636464409736 ) ) ;
#65872=CARTESIAN_POINT ( 'NONE',  ( -21.29700444710000085, 1453.723742755830017, 225.2777522932979934 ) ) ;
#65876=CARTESIAN_POINT ( 'NONE',  ( -11.17646686400000000, 1433.232109516899982, 151.6158427537980060 ) ) ;
#65879=CIRCLE ( 'NONE', #17557, 1.999994602259498100 ) ;
#65880=CARTESIAN_POINT ( 'NONE',  ( -25.39849853130000312, 1438.598112496549902, 138.1525938156979976 ) ) ;
#65881=CARTESIAN_POINT ( 'NONE',  ( -24.88010259380000022, 1440.326081558280066, 210.4197093850879980 ) ) ;
#65887=EDGE_CURVE ( 'NONE', #27055, #18369, #15674, .T. ) ;
#65888=CARTESIAN_POINT ( 'NONE',  ( 1.509834891803940062E-08, 1407.459576716519905, 264.1073148544030005 ) ) ;
#65889=ORIENTED_EDGE ( 'NONE', *, *, #83766, .T. ) ;
#65891=CARTESIAN_POINT ( 'NONE',  ( -11.78481361938159999, 1427.587923050230074, 147.3447378541869739 ) ) ;
#65895=CARTESIAN_POINT ( 'NONE',  ( -4.259181586709999578, 1473.442099373829933, 270.3898288651980124 ) ) ;
#65896=DIRECTION ( 'NONE',  ( 0.4794255386042040601, 0.000000000000000000, 0.8775825618903722036 ) ) ;
#65898=CARTESIAN_POINT ( 'NONE',  ( -13.71487111490000110, 1452.409042808630147, 223.1592556243980141 ) ) ;
#65899=CARTESIAN_POINT ( 'NONE',  ( 0.2795316912186849856, 1451.161107430230004, 182.2471984510860068 ) ) ;
#65904=CARTESIAN_POINT ( 'NONE',  ( -28.99670781314710055, 1413.665506641640150, 266.8891590342930158 ) ) ;
#65905=VERTEX_POINT ( 'NONE', #82402 ) ;
#65910=ADVANCED_FACE ( 'NONE', ( #33079 ), #13382, .T. ) ;
#65911=CARTESIAN_POINT ( 'NONE',  ( 34.00753574056176376, 1443.913060387329097, 154.9193549732159454 ) ) ;
#65912=CARTESIAN_POINT ( 'NONE',  ( 41.43280085394450651, 1444.114101214960101, 136.4350172471320093 ) ) ;
#65915=CARTESIAN_POINT ( 'NONE',  ( -3.869313214925711897, 1441.524545288032868, 170.5363236963821123 ) ) ;
#65916=CARTESIAN_POINT ( 'NONE',  ( -17.59820799470000097, 1455.456540126329855, 190.1371769522980060 ) ) ;
#65917=CARTESIAN_POINT ( 'NONE',  ( -2.230120725627048994, 1449.898333919053584, 182.9323432209308464 ) ) ;
#65919=CARTESIAN_POINT ( 'NONE',  ( -26.79956309869999842, 1435.440280005279874, 135.4702187632980213 ) ) ;
#65925=CARTESIAN_POINT ( 'NONE',  ( -42.28242862210569797, 1440.913046154859785, 269.8809742447210169 ) ) ;
#65927=CARTESIAN_POINT ( 'NONE',  ( -4.487375328049999723, 1396.069762987030117, 198.6459191643980091 ) ) ;
#65928=EDGE_CURVE ( 'NONE', #67449, #15423, #12040, .T. ) ;
#65930=ORIENTED_EDGE ( 'NONE', *, *, #72276, .F. ) ;
#65931=ORIENTED_EDGE ( 'NONE', *, *, #78971, .F. ) ;
#65932=CARTESIAN_POINT ( 'NONE',  ( 0.4061596876509999676, 1451.157747844730238, 182.5691048874980140 ) ) ;
#65936=CARTESIAN_POINT ( 'NONE',  ( -0.03698025251986000739, 1409.854707136450088, 185.1104546373300082 ) ) ;
#65939=CARTESIAN_POINT ( 'NONE',  ( -10.10004869885203682, 1411.254281879943164, 137.0999999980979851 ) ) ;
#65942=EDGE_CURVE ( 'NONE', #47384, #81952, #25004, .T. ) ;
#65943=CARTESIAN_POINT ( 'NONE',  ( 11.75111438890000137, 1446.815402695709963, 187.7955925520979861 ) ) ;
#65945=EDGE_LOOP ( 'NONE', ( #27467, #37688, #91104, #103610 ) ) ;
#65946=CARTESIAN_POINT ( 'NONE',  ( -38.81202644819489933, 1450.612734570859857, 134.4203407196499995 ) ) ;
#65952=CARTESIAN_POINT ( 'NONE',  ( 12.89586781552239891, 1434.724716683040242, 149.2198538527470077 ) ) ;
#65954=CARTESIAN_POINT ( 'NONE',  ( 13.38213216230000135, 1415.140114695929924, 197.3646947084980070 ) ) ;
#65955=CARTESIAN_POINT ( 'NONE',  ( -1.517310924280000028, 1507.186118470329802, 180.8246499599979984 ) ) ;
#65956=CARTESIAN_POINT ( 'NONE',  ( 2.461716435160000049, 1435.943783413959864, 150.4083956814980070 ) ) ;
#65957=CARTESIAN_POINT ( 'NONE',  ( 3.491631218259470426, 1450.859992781919573, 184.0578325456160655 ) ) ;
#65960=CARTESIAN_POINT ( 'NONE',  ( 24.34104170635332665, 1445.460888148215190, 214.1669348561839001 ) ) ;
#65961=EDGE_CURVE ( 'NONE', #66906, #57154, #81150, .T. ) ;
#65962=CARTESIAN_POINT ( 'NONE',  ( 41.52362078918107358, 1442.051295106819907, 135.5055851492039380 ) ) ;
#65968=CARTESIAN_POINT ( 'NONE',  ( -5.402393449050000740, 1473.936434490630063, 270.1311850751980046 ) ) ;
#65970=CARTESIAN_POINT ( 'NONE',  ( 0.1115023623899999983, 1420.227194636330069, 183.9075503089979975 ) ) ;
#65971=EDGE_CURVE ( 'NONE', #50244, #90113, #37152, .T. ) ;
#65973=CIRCLE ( 'NONE', #15887, 2.000006069085131344 ) ;
#65976=CARTESIAN_POINT ( 'NONE',  ( 30.54124909559969936, 1510.057079062230059, 213.7077286667680198 ) ) ;
#65977=CARTESIAN_POINT ( 'NONE',  ( 3.835404308833624043, 1405.413060387330006, 216.1425064568209677 ) ) ;
#65979=CARTESIAN_POINT ( 'NONE',  ( 17.90582816991177495, 1423.855356620343855, 225.8115124795609745 ) ) ;
#65982=CARTESIAN_POINT ( 'NONE',  ( 33.88603162083069975, 1440.913060384309802, 248.6081570316809746 ) ) ;
#65986=CARTESIAN_POINT ( 'NONE',  ( 12.88143820049999810, 1419.885573380330015, 222.2329351837979914 ) ) ;
#65987=VERTEX_POINT ( 'NONE', #8589 ) ;
#65990=CARTESIAN_POINT ( 'NONE',  ( -19.63429367885367682, 1485.335955380609221, 190.2453589707047286 ) ) ;
#65991=CARTESIAN_POINT ( 'NONE',  ( -28.17856942739999937, 1509.667335739730106, 211.1330165365179994 ) ) ;
#65996=CARTESIAN_POINT ( 'NONE',  ( 20.29103523386016050, 1509.739352328666428, 231.2885314561093253 ) ) ;
#66001=CARTESIAN_POINT ( 'NONE',  ( 5.361946547511959871, 1422.281156908029971, 142.4701046725139975 ) ) ;
#66006=CARTESIAN_POINT ( 'NONE',  ( -1.676216080179999901, 1450.511945511729891, 182.4451616703979937 ) ) ;
#66018=CARTESIAN_POINT ( 'NONE',  ( 7.067760138535259529, 1409.159872009930041, 195.9246175589510131 ) ) ;
#66019=FACE_OUTER_BOUND ( 'NONE', #47345, .T. ) ;
#66022=CARTESIAN_POINT ( 'NONE',  ( -3.655277279608119656, 1441.526510731130202, 166.9096038968010021 ) ) ;
#66024=CARTESIAN_POINT ( 'NONE',  ( -3.827327156165859723, 1424.046157831530081, 184.1455916618039907 ) ) ;
#66026=CARTESIAN_POINT ( 'NONE',  ( -1.608351468689999786, 1426.598937817530214, 144.1938086916980239 ) ) ;
#66027=CARTESIAN_POINT ( 'NONE',  ( 18.65411303873779758, 1457.703406872730056, 227.4352212818459975 ) ) ;
#66028=CARTESIAN_POINT ( 'NONE',  ( -12.19455143910000139, 1434.284752744940079, 150.5224356719979824 ) ) ;
#66030=CARTESIAN_POINT ( 'NONE',  ( -3.063324380877089998E-10, 1466.672023398390138, 243.8770760458830011 ) ) ;
#66035=B_SPLINE_CURVE_WITH_KNOTS ( 'NONE', 3,
 ( #95760, #80060, #47031, #87368, #79524, #106906, #89560 ),
 .UNSPECIFIED., .F., .F.,
 ( 4, 3, 4 ),
 ( -89.03555611550000037, -57.33326531478269317, -17.24302739680000229 ),
 .UNSPECIFIED. ) ;
#66038=CARTESIAN_POINT ( 'NONE',  ( 13.48944867574859963, 1508.549640178079926, 233.3847123851280116 ) ) ;
#66041=CARTESIAN_POINT ( 'NONE',  ( 6.825986730469999486, 1409.091027440530070, 221.7399762292980085 ) ) ;
#66042=SURFACE_STYLE_FILL_AREA ( #5564 ) ;
#66043=CARTESIAN_POINT ( 'NONE',  ( 5.553848058839999879, 1423.191816860230119, 91.03168606369779070 ) ) ;
#66046=VERTEX_POINT ( 'NONE', #50069 ) ;
#66048=CARTESIAN_POINT ( 'NONE',  ( 23.87826881430000014, 1432.672873845370077, 221.5017660107979793 ) ) ;
#66050=CARTESIAN_POINT ( 'NONE',  ( -1.515746652750000312, 1478.158358440429765, 182.0299493565979958 ) ) ;
#66051=CARTESIAN_POINT ( 'NONE',  ( -16.63178664779999849, 1409.493855175129966, 194.4517206995979848 ) ) ;
#66053=CARTESIAN_POINT ( 'NONE',  ( -24.09667674930000203, 1426.479304371029912, 238.1639134735980008 ) ) ;
#66056=CARTESIAN_POINT ( 'NONE',  ( -22.24479823131389722, 1452.136254915900054, 140.1071540872370065 ) ) ;
#66059=CARTESIAN_POINT ( 'NONE',  ( -2.500000000000000000, 1422.798905948130141, 153.2868469301980099 ) ) ;
#66060=CARTESIAN_POINT ( 'NONE',  ( 13.95553492442098431, 1416.818673872114459, 196.3353044460132537 ) ) ;
#66064=ORIENTED_EDGE ( 'NONE', *, *, #82880, .T. ) ;
#66066=CARTESIAN_POINT ( 'NONE',  ( -22.77796388237689840, 1409.708471313090058, 209.3294552566549669 ) ) ;
#66071=DIRECTION ( 'NONE',  ( -0.03489949673788425577, -0.9993908270178603059, 4.843886099300351310E-10 ) ) ;
#66072=CARTESIAN_POINT ( 'NONE',  ( -19.53416072559999961, 1415.852625093730012, 222.3903674702980027 ) ) ;
#66073=CARTESIAN_POINT ( 'NONE',  ( 42.12374111126599985, 1455.597911166439872, 267.7355564021549412 ) ) ;
#66078=CARTESIAN_POINT ( 'NONE',  ( -2.500000000000000000, 1411.429641636930000, 146.1721969575970093 ) ) ;
#66080=CARTESIAN_POINT ( 'NONE',  ( 13.18440430809449460, 1443.101454830199145, 187.5179277441473005 ) ) ;
#66083=ADVANCED_FACE ( 'NONE', ( #40891 ), #74261, .T. ) ;
#66084=CARTESIAN_POINT ( 'NONE',  ( 26.75523174175490126, 1451.912001146919920, 135.4172217544110026 ) ) ;
#66085=CARTESIAN_POINT ( 'NONE',  ( -4.363123796622770278, 1423.854800546939941, 184.2546035468919854 ) ) ;
#66086=CARTESIAN_POINT ( 'NONE',  ( 10.53235956273399943, 1452.545262286839943, 150.3730426087770127 ) ) ;
#66087=EDGE_CURVE ( 'NONE', #49285, #24021, #110515, .T. ) ;
#66093=CARTESIAN_POINT ( 'NONE',  ( 13.04207810306199988, 1409.368499790489750, 192.3005055522939983 ) ) ;
#66094=CARTESIAN_POINT ( 'NONE',  ( -13.07075687411459874, 1434.811948465909836, 149.1083925370589895 ) ) ;
#66097=EDGE_CURVE ( 'NONE', #44736, #28853, #24041, .T. ) ;
#66099=CARTESIAN_POINT ( 'NONE',  ( 9.534219445089998857, 1428.030197386430018, 144.1938086916980239 ) ) ;
#66100=ORIENTED_EDGE ( 'NONE', *, *, #34757, .F. ) ;
#66101=CARTESIAN_POINT ( 'NONE',  ( 2.331468351709999880E-15, 1427.913060387330006, 209.1218459616979999 ) ) ;
#66102=AXIS2_PLACEMENT_3D ( 'NONE', #14544, #48733, #31905 ) ;
#66103=CARTESIAN_POINT ( 'NONE',  ( -0.09233079908728399066, 1424.283549355850027, 227.6553671107380126 ) ) ;
#66106=B_SPLINE_SURFACE_WITH_KNOTS ( 'NONE', 5, 5, ( 
 ( #17765, #69336, #79377, #44681, #18334, #60938, #70449, #2693, #51969 ),
 ( #95067, #102886, #78826, #86110, #78259, #34600, #36817, #9404, #102347 ),
 ( #26183, #2137, #19446, #25630, #43566, #104569, #59822, #93942, #77717 ),
 ( #44124, #17208, #60372, #85536, #86657, #87219, #27864, #95616, #1028 ),
 ( #35152, #27306, #62044, #103444, #8831, #52525, #51404, #26749, #69894 ),
 ( #96170, #9952, #18883, #43016, #77173, #53081, #35705, #36260, #53644 ),
 ( #1572, #104009, #476, #61487, #87788, #10509, #11070, #68786, #94493 ),
 ( #45239, #63164, #106763, #98913, #21640, #38460, #81554, #105693, #97811 ),
 ( #11619, #21090, #3245, #89967, #56383, #4330, #28976, #30054, #55845 ),
 ( #55293, #13241, #13790, #96734, #72110, #47431, #39001, #46350, #64245 ),
 ( #72634, #89423, #97265, #98367, #20541, #37371, #12713, #4856, #22185 ),
 ( #62617, #20005, #73178, #106224, #107322, #46897, #30617, #105128, #5413 ),
 ( #64804, #90515, #47974, #81021, #82114, #71007, #28419, #54745, #54199 ),
 ( #88875, #45796, #79929, #29508, #12160, #80479, #88324, #71572, #3797 ),
 ( #37928, #63701, #66452, #73745, #91064, #100565, #82677, #58587, #24937 ),
 ( #108427, #75395, #24403, #22733, #56935, #5968, #14348, #6515, #40113 ),
 ( #84321, #15993, #91622, #50195, #109534, #49637, #65347, #23846, #59149 ),
 ( #7068, #41224, #108985, #66993, #32808, #31157, #99455, #41768, #101103 ),
 ( #40668, #92175, #74841, #92717, #58037, #93270, #33353, #48539, #32270 ),
 ( #75925, #74296, #65895, #15446, #16533, #7612, #83774, #110078, #67548 ),
 ( #100012, #31709, #101650, #23302, #50724, #57497, #84855, #14898, #39572 ),
 ( #49089, #83225, #107869, #17079, #25499, #61917, #102220, #69198, #94934 ),
 ( #51274, #60809, #19305, #77040, #59690, #103305, #103882, #87084, #1428 ),
 ( #26046, #17638, #43989, #10368, #51840, #93802, #895, #8155, #85977 ),
 ( #86526, #78124, #27182, #27729, #77588, #69765, #35019, #26613, #68650 ),
 ( #85406, #44542, #35570, #2003, #8705, #33911, #34475, #42883, #348 ),
 ( #18206, #102751, #60239, #96034, #94358, #52403, #9820, #9277, #61365 ) ),
 .UNSPECIFIED., .F., .F., .F.,
 ( 6, 3, 3, 3, 3, 3, 3, 3, 6 ),
 ( 6, 3, 6 ),
 ( 24.02324320159999971, 42.68733206409999781, 75.98967771649999747, 109.6146260670000032, 126.4768870990000096, 132.7991108720000000, 135.9602227580000147, 139.1213346450000188, 143.3324205490000054 ),
 ( 0.000000000000000000, 1.000000000000000000, 2.000000000000000000 ),
 .UNSPECIFIED. ) ;
#66109=( BOUNDED_CURVE ( )  B_SPLINE_CURVE ( 3, ( #16660, #57070, #75525, #91197 ),
 .UNSPECIFIED., .F., .T. ) 
 B_SPLINE_CURVE_WITH_KNOTS ( ( 4, 4 ),
 ( 2.768156387931280271, 3.267547937231884969 ),
 .UNSPECIFIED. ) 
 CURVE ( )  GEOMETRIC_REPRESENTATION_ITEM ( )  RATIONAL_B_SPLINE_CURVE ( ( 1.000000000000000000, 0.9793250956183989775, 0.9793250956183989775, 1.000000000000000000 ) ) 
 REPRESENTATION_ITEM ( '' )  );
#66111=CARTESIAN_POINT ( 'NONE',  ( 16.81223226430000039, 1414.913060387329779, 210.6693098017280192 ) ) ;
#66113=AXIS2_PLACEMENT_3D ( 'NONE', #77944, #71234, #35390 ) ;
#66115=CARTESIAN_POINT ( 'NONE',  ( 11.88903768390000160, 1433.614055813610094, 150.5325803792979968 ) ) ;
#66116=CARTESIAN_POINT ( 'NONE',  ( 10.79382269979189957, 1414.913060387349788, 222.1041130917409987 ) ) ;
#66117=B_SPLINE_SURFACE_WITH_KNOTS ( 'NONE', 5, 5, ( 
 ( #32241, #83740, #73148, #99980, #83197, #15417, #108396, #107291, #106731, #98884, #14320, #82649 ),
 ( #22151, #31129, #56352, #90484, #13759, #99424, #74266, #22702, #56900, #91033, #23272, #48510 ),
 ( #5940, #57469, #94333, #8675, #85380, #16507, #50166, #17050, #41740, #50696, #18182, #58558 ),
 ( #84827, #15963, #33325, #84294, #17611, #103279, #67520, #26586, #51813, #102724, #75366, #60215 ),
 ( #43412, #8128, #102189, #110600, #60783, #66965, #51247, #24373, #101075, #101621, #85953, #321 ),
 ( #24909, #9254, #867, #52377, #92687, #34446, #77562, #94908, #77015, #75899, #7037, #59117 ),
 ( #42855, #34992, #41195, #42294, #110051, #109505, #7585, #32781, #68622, #93241, #76446, #33883 ),
 ( #68077, #25469, #59663, #69173, #93771, #26018, #54045, #96005, #18723, #96568, #10340, #19274 ),
 ( #27156, #105521, #53479, #52920, #97116, #63009, #87622, #104962, #88172, #20385, #44513, #80317 ),
 ( #10909, #2534, #28251, #19840, #3632, #62443, #61341, #79225, #3084, #11463, #36655, #45638 ),
 ( #70852, #45083, #78660, #71406, #79777, #1977, #43958, #37211, #28810, #95461, #54587, #104409 ),
 ( #88723, #12005, #46186, #37762, #71955, #86497, #106066, #27702, #87053, #29346, #63545, #97661 ) ),
 .UNSPECIFIED., .F., .F., .F.,
 ( 6, 3, 3, 6 ),
 ( 6, 3, 3, 6 ),
 ( 12.92362791200000061, 14.22782209820000077, 16.13066607289999865, 17.24295068607450077 ),
 ( 0.000000000000000000, 0.3306909445339999976, 0.9920728336020000482, 1.580619590369999994 ),
 .UNSPECIFIED. ) ;
#66118=CARTESIAN_POINT ( 'NONE',  ( 1.168363032481170016, 1450.780489601989984, 181.5091470336249984 ) ) ;
#66120=AXIS2_PLACEMENT_3D ( 'NONE', #103896, #77055, #77600 ) ;
#66123=CARTESIAN_POINT ( 'NONE',  ( -5.360152366205530150, 1422.242722016050038, 144.1549655170190078 ) ) ;
#66125=CARTESIAN_POINT ( 'NONE',  ( -16.48212676430000201, 1409.488628936830082, 224.5375981998979853 ) ) ;
#66128=CARTESIAN_POINT ( 'NONE',  ( -0.7143255590409999245, 1420.516258837929854, 228.0808124483980066 ) ) ;
#66131=CARTESIAN_POINT ( 'NONE',  ( -3.172147559474420109E-06, 1406.917453532339778, 196.1218398979460176 ) ) ;
#66135=CARTESIAN_POINT ( 'NONE',  ( -11.22085809270000034, 1414.913060387329779, 220.6193216414980043 ) ) ;
#66136=CARTESIAN_POINT ( 'NONE',  ( 0.1840937434512019966, 1472.115685549119917, 182.4330042628529895 ) ) ;
#66138=ORIENTED_EDGE ( 'NONE', *, *, #62424, .F. ) ;
#66139=CARTESIAN_POINT ( 'NONE',  ( -16.90742463042001376, 1444.994950788469623, 162.4348201727408991 ) ) ;
#66140=CARTESIAN_POINT ( 'NONE',  ( -27.95614485608019706, 1508.896726002669993, 210.6431370344629954 ) ) ;
#66141=CARTESIAN_POINT ( 'NONE',  ( 11.87916569230000086, 1433.311660768669981, 149.4775962793980000 ) ) ;
#66142=CARTESIAN_POINT ( 'NONE',  ( -41.66188030070000536, 1443.681299836830021, 134.0999999982049928 ) ) ;
#66150=CARTESIAN_POINT ( 'NONE',  ( 31.97075719519320458, 1416.524385823295688, 269.3163262971341396 ) ) ;
#66151=VECTOR ( 'NONE', #23288, 1000.000000000000114 ) ;
#66152=CARTESIAN_POINT ( 'NONE',  ( 4.500000000000000000, 1439.615672362369878, 182.7715282920979973 ) ) ;
#66153=B_SPLINE_CURVE_WITH_KNOTS ( 'NONE', 3,
 ( #83964, #57695, #58232, #40309, #23503, #15089, #40861, #15628, #7264, #41427 ),
 .UNSPECIFIED., .F., .F.,
 ( 4, 2, 2, 2, 4 ),
 ( 0.000000000000000000, 0.2500000000000000000, 0.5000000000000000000, 0.7500000000000000000, 1.000000000000000000 ),
 .UNSPECIFIED. ) ;
#66155=CARTESIAN_POINT ( 'NONE',  ( 2.500000000000000000, 1428.667732478729931, 183.2651393807979900 ) ) ;
#66157=CARTESIAN_POINT ( 'NONE',  ( 12.87618670774100060, 1416.835419214280137, 196.3099906520550064 ) ) ;
#66160=CARTESIAN_POINT ( 'NONE',  ( -28.70934402958750198, 1509.343126753840124, 208.7447959780810152 ) ) ;
#66161=CARTESIAN_POINT ( 'NONE',  ( -15.93050487141630178, 1409.571762620169920, 225.8570170024219976 ) ) ;
#66163=ORIENTED_EDGE ( 'NONE', *, *, #51073, .F. ) ;
#66166=CARTESIAN_POINT ( 'NONE',  ( -18.96565013588459792, 1410.937324021512723, 223.0483911484982400 ) ) ;
#66168=CARTESIAN_POINT ( 'NONE',  ( -0.1424279854816119795, 1419.609337117080031, 184.3401574130290044 ) ) ;
#66170=CARTESIAN_POINT ( 'NONE',  ( 17.84692647500000007, 1410.032952999730014, 222.8512867949980318 ) ) ;
#66172=CARTESIAN_POINT ( 'NONE',  ( -17.64168070010000022, 1423.919165630929911, 226.5634843356980070 ) ) ;
#66174=CARTESIAN_POINT ( 'NONE',  ( 2.500000000000000000, 1428.667732465049994, 183.2651393814149969 ) ) ;
#66182=DIRECTION ( 'NONE',  ( -0.3363363969979660806, -0.9417419115949053898, 0.000000000000000000 ) ) ;
#66184=ORIENTED_EDGE ( 'NONE', *, *, #20659, .F. ) ;
#66187=ORIENTED_EDGE ( 'NONE', *, *, #25860, .T. ) ;
#66189=CARTESIAN_POINT ( 'NONE',  ( -22.66911695520000336, 1410.908238445129882, 203.8386702287579908 ) ) ;
#66190=CARTESIAN_POINT ( 'NONE',  ( -11.63809698065658438, 1425.864003583440081, 144.2671358013096778 ) ) ;
#66191=CARTESIAN_POINT ( 'NONE',  ( 15.86082858073990032, 1410.114303850130000, 191.7269226526290140 ) ) ;
#66193=CARTESIAN_POINT ( 'NONE',  ( 41.49264608937420462, 1443.127563515339943, 136.5039589477979973 ) ) ;
#66195=CARTESIAN_POINT ( 'NONE',  ( -10.81512807170000023, 1424.921141247430114, 144.1662922870979742 ) ) ;
#66196=FACE_OUTER_BOUND ( 'NONE', #15190, .T. ) ;
#66199=CARTESIAN_POINT ( 'NONE',  ( 35.54866228602229938, 1451.502040174259946, 134.0999999984919668 ) ) ;
#66203=CIRCLE ( 'NONE', #60845, 1.000002393159192371 ) ;
#66205=ORIENTED_EDGE ( 'NONE', *, *, #98178, .F. ) ;
#66206=VERTEX_POINT ( 'NONE', #78786 ) ;
#66208=CARTESIAN_POINT ( 'NONE',  ( -16.19492410612830113, 1409.478599598990058, 194.0661808939520085 ) ) ;
#66209=CARTESIAN_POINT ( 'NONE',  ( 19.19535387687943029, 1456.080104641030175, 225.8939609127118047 ) ) ;
#66215=CARTESIAN_POINT ( 'NONE',  ( 33.91369120209999721, 1435.681798817170147, 134.0999984767980209 ) ) ;
#66217=CARTESIAN_POINT ( 'NONE',  ( 26.46046307870000192, 1441.626270307079949, 137.7338459176980336 ) ) ;
#66220=ORIENTED_EDGE ( 'NONE', *, *, #108387, .T. ) ;
#66224=CARTESIAN_POINT ( 'NONE',  ( 41.87718344479209520, 1440.913060387330006, 269.4528669971400063 ) ) ;
#66225=CARTESIAN_POINT ( 'NONE',  ( -0.0002536599424906319715, 1452.586836000080439, 153.4883541576832329 ) ) ;
#66226=ORIENTED_EDGE ( 'NONE', *, *, #104640, .T. ) ;
#66236=CARTESIAN_POINT ( 'NONE',  ( 26.40325702796710061, 1497.690506021000147, 206.2288011628740207 ) ) ;
#66237=CARTESIAN_POINT ( 'NONE',  ( 17.37740683730000057, 1460.085864807530015, 228.4865696861979814 ) ) ;
#66238=CARTESIAN_POINT ( 'NONE',  ( -10.85852385072151449, 1424.794007429657313, 138.1924915429941905 ) ) ;
#66239=CARTESIAN_POINT ( 'NONE',  ( -4.632166985597920394, 1422.117103908413128, 184.6589626825009418 ) ) ;
#66240=B_SPLINE_SURFACE_WITH_KNOTS ( 'NONE', 5, 5, ( 
 ( #72834, #73933, #39204, #108063, #47084, #31359, #91815, #6710, #66651 ),
 ( #100753, #106968, #94569, #93460, #24040, #109729, #51479, #17285, #42517 ),
 ( #77247, #60449, #59898, #16731, #41432, #7811, #75599, #26262, #58236 ),
 ( #52044, #110826, #43637, #17841, #25147, #547, #67193, #49839, #68858 ),
 ( #7268, #33547, #68309, #102417, #76129, #67745, #69413, #9473, #50394 ),
 ( #34671, #101854, #92360, #85609, #15632, #83968, #33007, #59352, #101293 ) ),
 .UNSPECIFIED., .F., .F., .F.,
 ( 6, 6 ),
 ( 6, 3, 6 ),
 ( 0.4666582265090000181, 2.797885342447860246 ),
 ( -1.082961785764040044E-05, 1.000000000000000000, 2.000000000000000000 ),
 .UNSPECIFIED. ) ;
#66242=ORIENTED_EDGE ( 'NONE', *, *, #6974, .T. ) ;
#66243=CARTESIAN_POINT ( 'NONE',  ( -1.210324586182019546, 1486.266221086842961, 181.7930448816870523 ) ) ;
#66249=FACE_OUTER_BOUND ( 'NONE', #37841, .T. ) ;
#66252=CYLINDRICAL_SURFACE ( 'NONE', #79986, 2.000000000000022204 ) ;
#66255=EDGE_CURVE ( 'NONE', #42031, #65361, #58061, .T. ) ;
#66256=CARTESIAN_POINT ( 'NONE',  ( -11.86004383289999886, 1431.913113693130072, 149.9670089978980059 ) ) ;
#66259=CARTESIAN_POINT ( 'NONE',  ( 27.02366939970098159, 1451.038188054575812, 136.3589578157976803 ) ) ;
#66260=B_SPLINE_CURVE_WITH_KNOTS ( 'NONE', 3,
 ( #107141, #108242, #13061, #66279, #98739, #31532, #4687, #5801, #100395, #74663, #30433, #82500, #107699, #91991, #47246, #83581, #99273, #5235, #74112, #65708, #90889, #6880, #100922, #39390, #73566, #75213, #99830, #48918 ),
 .UNSPECIFIED., .F., .F.,
 ( 4, 2, 1, 1, 1, 2, 2, 2, 1, 1, 2, 2, 1, 1, 1, 2, 2, 4 ),
 ( 0.000000000000000000, 0.1249999999971333209, 0.1874999999956837582, 0.2187499999949452933, 0.2343749999945753670, 0.2421874999943897933, 0.2499999999942042195, 0.3749999999947117857, 0.4374999999949656382, 0.4687499999949767404, 0.4843749999949823470, 0.4999999999949878982, 0.6249999999956661334, 0.6874999999958667507, 0.7187499999961025621, 0.7343749999962204678, 0.7499999999963383734, 1.000000000000000000 ),
 .UNSPECIFIED. ) ;
#66262=CARTESIAN_POINT ( 'NONE',  ( 12.86833609579999838, 1444.979730008290062, 187.1048578417980082 ) ) ;
#66263=CARTESIAN_POINT ( 'NONE',  ( -26.86204968839999907, 1508.007394745430020, 212.0120969969080136 ) ) ;
#66264=CARTESIAN_POINT ( 'NONE',  ( -5.940831854492779840, 1420.421544355079959, 137.0999999980978430 ) ) ;
#66265=CARTESIAN_POINT ( 'NONE',  ( -16.12806753298000473, 1459.080126285580036, 229.9878173539649993 ) ) ;
#66268=CARTESIAN_POINT ( 'NONE',  ( 14.57541043219999999, 1407.789481095929887, 268.9619740390979814 ) ) ;
#66269=CARTESIAN_POINT ( 'NONE',  ( 38.62063633891679615, 1443.662372577139877, 137.1803698152800166 ) ) ;
#66271=CARTESIAN_POINT ( 'NONE',  ( 22.07708618635539466, 1430.125185735898640, 217.9172516584410744 ) ) ;
#66273=CARTESIAN_POINT ( 'NONE',  ( 27.70972759929999896, 1508.058934375229910, 212.2396871123379753 ) ) ;
#66274=ADVANCED_FACE ( 'NONE', ( #103975 ), #21422, .T. ) ;
#66275=CARTESIAN_POINT ( 'NONE',  ( 13.99649777436419917, 1443.814619143300206, 195.5016475565269900 ) ) ;
#66276=AXIS2_PLACEMENT_3D ( 'NONE', #100432, #23715, #102075 ) ;
#66277=CARTESIAN_POINT ( 'NONE',  ( -0.8736373970091440011, 1450.882552293999879, 154.7893752771190066 ) ) ;
#66278=CARTESIAN_POINT ( 'NONE',  ( -12.03594224589999939, 1445.662096867079981, 187.0019513043980055 ) ) ;
#66279=CARTESIAN_POINT ( 'NONE',  ( -19.69953526152687928, 1486.120311317603864, 190.0890748500791290 ) ) ;
#66282=CARTESIAN_POINT ( 'NONE',  ( -19.00000000000000000, 1440.913060387330006, 209.1218459616979999 ) ) ;
#66283=CARTESIAN_POINT ( 'NONE',  ( 20.10171188468166292, 1507.852758503362338, 228.9948063811727934 ) ) ;
#66284=CARTESIAN_POINT ( 'NONE',  ( 3.134096205239999655, 1440.879545174999976, 159.2386616682979934 ) ) ;
#66285=CARTESIAN_POINT ( 'NONE',  ( -2.077244269789999986, 1475.014520942230092, 269.6487028165980178 ) ) ;
#66286=CARTESIAN_POINT ( 'NONE',  ( -11.45157208071476695, 1425.808262388908815, 139.1344810667301601 ) ) ;
#66293=CARTESIAN_POINT ( 'NONE',  ( -24.27560546558390087, 1444.785062312789933, 211.2846025609280218 ) ) ;
#66296=CARTESIAN_POINT ( 'NONE',  ( -20.91134631659999599, 1409.807790057629745, 201.0288384400980135 ) ) ;
#66297=B_SPLINE_CURVE_WITH_KNOTS ( 'NONE', 3,
 ( #45637, #70296, #79224, #27155, #10339, #12004, #2533, #78659, #46185, #80316 ),
 .UNSPECIFIED., .F., .F.,
 ( 4, 3, 3, 4 ),
 ( 2.231733318449370174, 2.693712400684689978, 2.992882853181570102, 3.155691482920000013 ),
 .UNSPECIFIED. ) ;
#66298=CARTESIAN_POINT ( 'NONE',  ( -15.03850872322399823, 1422.463411162540069, 228.7611157286099797 ) ) ;
#66301=LINE ( 'NONE', #56775, #23065 ) ;
#66304=CARTESIAN_POINT ( 'NONE',  ( 11.72729116660000059, 1426.702026288230172, 143.4717466479980033 ) ) ;
#66307=CARTESIAN_POINT ( 'NONE',  ( -1.600048698852036821, 1401.254281879943164, 135.5999999980979851 ) ) ;
#66311=CARTESIAN_POINT ( 'NONE',  ( 11.54436744337454002, 1432.352362330610049, 151.3410663384053976 ) ) ;
#66312=DIRECTION ( 'NONE',  ( 1.988618688120850357E-13, 0.03085824620771311644, -0.9995237709234254808 ) ) ;
#66315=CYLINDRICAL_SURFACE ( 'NONE', #66276, 2.000000000000001776 ) ;
#66316=CARTESIAN_POINT ( 'NONE',  ( 21.68605459302450100, 1509.621532965099959, 228.4776040847019942 ) ) ;
#66320=CARTESIAN_POINT ( 'NONE',  ( 12.02669875993479920, 1433.747065677280034, 149.9298205679299940 ) ) ;
#66321=CARTESIAN_POINT ( 'NONE',  ( -4.661545375210000230, 1396.075845138829891, 219.5353638017980131 ) ) ;
#66322=CARTESIAN_POINT ( 'NONE',  ( -20.28107068739999974, 1410.981495019129852, 220.2339880788979940 ) ) ;
#66324=CARTESIAN_POINT ( 'NONE',  ( -13.36916045171295053, 1444.478176240853372, 169.3716993028445472 ) ) ;
#66325=CARTESIAN_POINT ( 'NONE',  ( 22.51756156282889876, 1509.699390964210124, 227.9212218486820234 ) ) ;
#66326=CARTESIAN_POINT ( 'NONE',  ( -0.1613635714646410035, 1507.107001889669846, 180.9028745560509890 ) ) ;
#66328=CARTESIAN_POINT ( 'NONE',  ( -13.70772824027479864, 1507.648153509909889, 184.2587339175119894 ) ) ;
#66329=CIRCLE ( 'NONE', #75189, 1.999994602351848672 ) ;
#66330=CARTESIAN_POINT ( 'NONE',  ( 7.083309374099999722, 1468.699157173630056, 184.4250794663979889 ) ) ;
#66334=CARTESIAN_POINT ( 'NONE',  ( 9.833610268327619863, 1396.256457636480036, 204.0482078523459677 ) ) ;
#66335=CARTESIAN_POINT ( 'NONE',  ( 0.7890062529840000671, 1416.021639796329964, 190.5012297770979899 ) ) ;
#66336=CARTESIAN_POINT ( 'NONE',  ( 10.91629673539999956, 1428.582341354329856, 150.7594233110980042 ) ) ;
#66337=CARTESIAN_POINT ( 'NONE',  ( 7.960834073489841067, 1509.191483305627116, 180.8814468251773064 ) ) ;
#66338=ORIENTED_EDGE ( 'NONE', *, *, #100084, .F. ) ;
#66339=CARTESIAN_POINT ( 'NONE',  ( 13.29115197908729940, 1435.192795144800129, 149.9986224416759910 ) ) ;
#66342=CARTESIAN_POINT ( 'NONE',  ( 12.92773491524689078, 1444.920201159182170, 169.4324473822623816 ) ) ;
#66343=CARTESIAN_POINT ( 'NONE',  ( -9.049861655339999089, 1463.472726760930072, 233.4465893264980139 ) ) ;
#66344=CARTESIAN_POINT ( 'NONE',  ( -12.86077854309999857, 1416.823634022829992, 196.3807302971979993 ) ) ;
#66349=CARTESIAN_POINT ( 'NONE',  ( 2.500000000000000000, 1448.203020940240094, 169.6834909796610020 ) ) ;
#66355=CARTESIAN_POINT ( 'NONE',  ( -20.25110114130000127, 1509.046039793229966, 229.4394552683979782 ) ) ;
#66356=CARTESIAN_POINT ( 'NONE',  ( -20.74384221371932924, 1414.376127513459551, 269.3942681799695151 ) ) ;
#66358=CARTESIAN_POINT ( 'NONE',  ( -0.05152562430163110108, 1416.529254608160045, 227.2755757173690085 ) ) ;
#66360=CARTESIAN_POINT ( 'NONE',  ( 2.500000000000000000, 1425.201036443130079, 155.3321294796979828 ) ) ;
#66361=CARTESIAN_POINT ( 'NONE',  ( -27.45330484456810183, 1440.913060400619997, 228.8604962196139923 ) ) ;
#66364=CARTESIAN_POINT ( 'NONE',  ( 14.88997449063399969, 1411.680983156579941, 270.0818248018620693 ) ) ;
#66367=CARTESIAN_POINT ( 'NONE',  ( 24.12740820519999829, 1411.115144176130116, 208.8584871057929888 ) ) ;
#66368=CARTESIAN_POINT ( 'NONE',  ( -20.13638283970000131, 1507.886205248129954, 189.0953426691980042 ) ) ;
#66373=CARTESIAN_POINT ( 'NONE',  ( 0.1114963473639999925, 1420.227192211030115, 183.9075558398980093 ) ) ;
#66375=CARTESIAN_POINT ( 'NONE',  ( -8.473904872574415492, 1486.003588610487441, 183.3063149312824294 ) ) ;
#66384=CARTESIAN_POINT ( 'NONE',  ( -23.40333288369999920, 1448.250072204309845, 217.2337772597779804 ) ) ;
#66388=CARTESIAN_POINT ( 'NONE',  ( -25.32446257976238968, 1450.806899494430354, 137.4427265456963880 ) ) ;
#66390=EDGE_LOOP ( 'NONE', ( #37293, #97832, #96706, #26977 ) ) ;
#66393=CARTESIAN_POINT ( 'NONE',  ( -27.02655704100176592, 1451.108971386630174, 136.3738572239980158 ) ) ;
#66394=CARTESIAN_POINT ( 'NONE',  ( 20.06570944619999963, 1454.764211563430081, 224.8152366716980168 ) ) ;
#66398=DIRECTION ( 'NONE',  ( 0.000000000000000000, 0.000000000000000000, -1.000000000000000000 ) ) ;
#66399=AXIS2_PLACEMENT_3D ( 'NONE', #69720, #63530, #3616 ) ;
#66401=CARTESIAN_POINT ( 'NONE',  ( -23.63309344749999852, 1435.875959318670084, 212.1442856114379936 ) ) ;
#66404=CARTESIAN_POINT ( 'NONE',  ( -16.56636285579999779, 1413.296451893629865, 226.6997547370980044 ) ) ;
#66407=CARTESIAN_POINT ( 'NONE',  ( -30.00386682649119763, 1462.246334517119067, 269.4708284355384080 ) ) ;
#66409=CARTESIAN_POINT ( 'NONE',  ( 2.439001525050000119, 1430.488531030629929, 150.2249694046979869 ) ) ;
#66410=CARTESIAN_POINT ( 'NONE',  ( -42.06510204283767962, 1427.649616927324587, 269.0740259319668439 ) ) ;
#66411=ADVANCED_FACE ( 'NONE', ( #52616 ), #64386, .T. ) ;
#66413=CARTESIAN_POINT ( 'NONE',  ( -0.9756374909739999879, 1431.113060387329824, 228.8047907271979966 ) ) ;
#66414=CARTESIAN_POINT ( 'NONE',  ( -0.1798688738929999642, 1417.261861208530263, 235.9169760632979944 ) ) ;
#66415=CARTESIAN_POINT ( 'NONE',  ( -13.46697063184865151, 1444.247415097991052, 187.0159000695805673 ) ) ;
#66418=CIRCLE ( 'NONE', #18104, 17.74083438352840503 ) ;
#66420=CARTESIAN_POINT ( 'NONE',  ( -15.07584010957818954, 1451.149360461914966, 149.6732302036660656 ) ) ;
#66422=( BOUNDED_CURVE ( )  B_SPLINE_CURVE ( 3, ( #40932, #25766, #32541, #77307 ),
 .UNSPECIFIED., .F., .F. ) 
 B_SPLINE_CURVE_WITH_KNOTS ( ( 4, 4 ),
 ( 1.555588359660764919, 1.573006934440774884 ),
 .UNSPECIFIED. ) 
 CURVE ( )  GEOMETRIC_REPRESENTATION_ITEM ( )  RATIONAL_B_SPLINE_CURVE ( ( 1.000000000000000000, 0.9999747162642045328, 0.9999747162642045328, 1.000000000000000000 ) ) 
 REPRESENTATION_ITEM ( '' )  );
#66423=CARTESIAN_POINT ( 'NONE',  ( -12.60679465157404167, 1442.786628925963214, 169.4683254417570026 ) ) ;
#66424=CARTESIAN_POINT ( 'NONE',  ( -14.33610927549999836, 1409.413688348330197, 225.7799880264979890 ) ) ;
#66425=VERTEX_POINT ( 'NONE', #38545 ) ;
#66426=CARTESIAN_POINT ( 'NONE',  ( -0.09392264339291689357, 1415.426561690370136, 191.6203292375940066 ) ) ;
#66427=CARTESIAN_POINT ( 'NONE',  ( 22.01759343194246910, 1509.573295641457435, 226.9000235256352767 ) ) ;
#66430=CARTESIAN_POINT ( 'NONE',  ( 16.98743823132990016, 1415.088136167450102, 209.1445283149309944 ) ) ;
#66433=CARTESIAN_POINT ( 'NONE',  ( -24.18530732099999980, 1444.140951279559886, 212.0278258309579940 ) ) ;
#66435=CARTESIAN_POINT ( 'NONE',  ( -11.75646471859999842, 1433.433141379730159, 150.8109742706980114 ) ) ;
#66437=CARTESIAN_POINT ( 'NONE',  ( 251.6799247787360230, 1855.634424228300077, 173.9675981348009941 ) ) ;
#66439=CARTESIAN_POINT ( 'NONE',  ( -14.32882045604760357, 1429.651770908837989, 222.2483748908982761 ) ) ;
#66444=CARTESIAN_POINT ( 'NONE',  ( -28.97640022888837663, 1510.035890305760176, 216.8925410192303218 ) ) ;
#66448=CARTESIAN_POINT ( 'NONE',  ( -11.75158851103499913, 1426.771919862610048, 145.1867488865719906 ) ) ;
#66450=EDGE_CURVE ( 'NONE', #89981, #66046, #104657, .T. ) ;
#66452=CARTESIAN_POINT ( 'NONE',  ( -8.240145092400000593, 1473.030649236130103, 270.3822351584980197 ) ) ;
#66457=CARTESIAN_POINT ( 'NONE',  ( 37.85868654299600422, 1450.015328435070160, 136.0234584287910025 ) ) ;
#66458=CARTESIAN_POINT ( 'NONE',  ( 18.70730727500000157, 1431.113060387329824, 209.1218459615069776 ) ) ;
#66459=EDGE_CURVE ( 'NONE', #20723, #110373, #56937, .T. ) ;
#66465=CARTESIAN_POINT ( 'NONE',  ( -43.77342332416050397, 1429.948824217480023, 266.7521212402160131 ) ) ;
#66468=ORIENTED_EDGE ( 'NONE', *, *, #100925, .F. ) ;
#66472=CARTESIAN_POINT ( 'NONE',  ( 4.619879510139068834, 1423.718273955572158, 183.8526073848954638 ) ) ;
#66476=CARTESIAN_POINT ( 'NONE',  ( -16.58606811730000175, 1455.453783750930143, 189.4873228618979795 ) ) ;
#66479=CARTESIAN_POINT ( 'NONE',  ( -26.29948081250000058, 1435.416034970859982, 135.3926350979980100 ) ) ;
#66484=EDGE_CURVE ( 'NONE', #81651, #13362, #31256, .T. ) ;
#66486=CARTESIAN_POINT ( 'NONE',  ( -33.74129728029610220, 1421.399541067400150, 269.9732882242340111 ) ) ;
#66487=DIRECTION ( 'NONE',  ( -0.7067700464262639537, 0.03085823069700149510, -0.7067700270051548994 ) ) ;
#66488=CARTESIAN_POINT ( 'NONE',  ( -1.143643780430000145, 1395.952997308129852, 197.8013073227980101 ) ) ;
#66493=EDGE_CURVE ( 'NONE', #9890, #9209, #68390, .T. ) ;
#66496=CARTESIAN_POINT ( 'NONE',  ( -25.11421028039999825, 1436.601945934859941, 137.7221587483980159 ) ) ;
#66497=CARTESIAN_POINT ( 'NONE',  ( -24.49558118859999922, 1441.433152052330115, 211.0117683613680128 ) ) ;
#66499=AXIS2_PLACEMENT_3D ( 'NONE', #37850, #107802, #82036 ) ;
#66501=CARTESIAN_POINT ( 'NONE',  ( -2.293592999468180071, 1484.254952969489977, 183.1434726039850034 ) ) ;
#66503=CARTESIAN_POINT ( 'NONE',  ( -13.15471227499809892, 1414.913526845469960, 220.1561254705790134 ) ) ;
#66506=CARTESIAN_POINT ( 'NONE',  ( -2.907264515414449857, 1451.960119877520128, 184.7556101994359778 ) ) ;
#66509=ORIENTED_EDGE ( 'NONE', *, *, #80952, .F. ) ;
#66511=B_SPLINE_CURVE_WITH_KNOTS ( 'NONE', 3,
 ( #94189, #17458, #51658, #85797, #9095, #105369, #35961, #88574, #11317, #11857, #37050, #69587, #53898, #36504, #61194, #79629 ),
 .UNSPECIFIED., .F., .F.,
 ( 4, 2, 2, 1, 1, 1, 1, 2, 2, 4 ),
 ( 0.000000000000000000, 0.2499999999999679146, 0.3749999999999507616, 0.4374999999999422129, 0.4687499999999449329, 0.4843749999999474865, 0.4921874999999487632, 0.4960937499999555356, 0.4999999999999622524, 1.000000000000000000 ),
 .UNSPECIFIED. ) ;
#66512=CARTESIAN_POINT ( 'NONE',  ( -22.64739172320458849, 1509.725407825014599, 228.2189809371752460 ) ) ;
#66513=CARTESIAN_POINT ( 'NONE',  ( 18.22865577494500045, 1459.310763497099970, 227.8759328773050186 ) ) ;
#66515=CARTESIAN_POINT ( 'NONE',  ( 12.62835224979999893, 1416.067629290630066, 222.6573521500980064 ) ) ;
#66516=CARTESIAN_POINT ( 'NONE',  ( 2.830001175615096454, 1451.807281766560891, 183.8374670539779174 ) ) ;
#66519=CARTESIAN_POINT ( 'NONE',  ( 4.278374243669960109, 1441.027869772839949, 156.7540461662579787 ) ) ;
#66521=DIRECTION ( 'NONE',  ( -2.513978196838388281E-18, -0.7071067811865475727, -0.7071067811865475727 ) ) ;
#66524=CARTESIAN_POINT ( 'NONE',  ( -12.77825866169999891, 1416.543503932829935, 195.9645815386980132 ) ) ;
#66525=CARTESIAN_POINT ( 'NONE',  ( 16.16926794620007257, 1409.477699224023809, 193.1978555737975682 ) ) ;
#66526=CARTESIAN_POINT ( 'NONE',  ( 2.250225901099999870, 1421.216712495730008, 183.8152323106979793 ) ) ;
#66531=CARTESIAN_POINT ( 'NONE',  ( 18.76751273909999895, 1416.021639799829927, 210.4841606299879970 ) ) ;
#66538=VERTEX_POINT ( 'NONE', #49728 ) ;
#66539=ORIENTED_EDGE ( 'NONE', *, *, #49364, .T. ) ;
#66542=CARTESIAN_POINT ( 'NONE',  ( 16.34617637888406705, 1409.483876603966110, 193.1367303227071659 ) ) ;
#66553=CARTESIAN_POINT ( 'NONE',  ( -13.85509113240000012, 1453.154616238129847, 193.9807013630980066 ) ) ;
#66554=CARTESIAN_POINT ( 'NONE',  ( -27.44229999310290680, 1509.334241622238778, 212.0840502660885249 ) ) ;
#66559=AXIS2_PLACEMENT_3D ( 'NONE', #87884, #71664, #45335 ) ;
#66563=ORIENTED_EDGE ( 'NONE', *, *, #61940, .F. ) ;
#66565=( BOUNDED_CURVE ( )  B_SPLINE_CURVE ( 3, ( #58202, #50366, #42488, #84492 ),
 .UNSPECIFIED., .F., .T. ) 
 B_SPLINE_CURVE_WITH_KNOTS ( ( 4, 4 ),
 ( 5.330947148644519906, 5.979513181285929235 ),
 .UNSPECIFIED. ) 
 CURVE ( )  GEOMETRIC_REPRESENTATION_ITEM ( )  RATIONAL_B_SPLINE_CURVE ( ( 1.000000000000000000, 0.9652529480040055176, 0.9652529480040055176, 1.000000000000000000 ) ) 
 REPRESENTATION_ITEM ( '' )  );
#66567=CARTESIAN_POINT ( 'NONE',  ( 35.81700442754009828, 1437.367486095130062, 136.5363678219200096 ) ) ;
#66575=CARTESIAN_POINT ( 'NONE',  ( 0.5133706386020000512, 1410.311097227529899, 185.0719932622980082 ) ) ;
#66578=CARTESIAN_POINT ( 'NONE',  ( 11.76945428880000044, 1432.334073542720034, 150.8119095935979885 ) ) ;
#66580=CARTESIAN_POINT ( 'NONE',  ( -2.101005067686500194, 1450.237514968539699, 183.4561686731089765 ) ) ;
#66584=CARTESIAN_POINT ( 'NONE',  ( 18.24783257861880159, 1458.395086229769959, 227.8518626438460046 ) ) ;
#66585=EDGE_CURVE ( 'NONE', #63161, #12743, #22421, .T. ) ;
#66587=CARTESIAN_POINT ( 'NONE',  ( -1.634883190284829911E-09, 1471.268413604999978, 257.2557666294709975 ) ) ;
#66588=CARTESIAN_POINT ( 'NONE',  ( 16.96608709051594488, 1436.324541078401126, 148.2478660041307990 ) ) ;
#66589=PLANE ( 'NONE',  #1768 ) ;
#66591=CARTESIAN_POINT ( 'NONE',  ( -0.9064963533630000514, 1486.513385844430104, 181.9403208173980033 ) ) ;
#66594=CARTESIAN_POINT ( 'NONE',  ( 13.97271228624649986, 1509.364740696860054, 234.5129875352629938 ) ) ;
#66598=DIRECTION ( 'NONE',  ( 0.000000000000000000, -1.000000000000000000, 0.000000000000000000 ) ) ;
#66601=EDGE_CURVE ( 'NONE', #64966, #31041, #72005, .T. ) ;
#66603=CARTESIAN_POINT ( 'NONE',  ( 28.07850872979999934, 1439.094797578370162, 231.9053043656980151 ) ) ;
#66604=CARTESIAN_POINT ( 'NONE',  ( -2.531548701460000217, 1486.446787100029951, 181.7283458845979851 ) ) ;
#66608=CARTESIAN_POINT ( 'NONE',  ( -28.81229682350082300, 1509.921425474858097, 203.0494097711116410 ) ) ;
#66610=CARTESIAN_POINT ( 'NONE',  ( 9859.020463722770728, 54.07981494723821925, 1360.877155955070066 ) ) ;
#66612=CARTESIAN_POINT ( 'NONE',  ( -5.370353317006889782, 1427.592827902419913, 153.4505299550590109 ) ) ;
#66613=CARTESIAN_POINT ( 'NONE',  ( 13.58235846979999906, 1416.828040475229955, 196.3349388281980055 ) ) ;
#66614=CARTESIAN_POINT ( 'NONE',  ( 14.59153218112539996, 1421.962858571700053, 230.0979270886319910 ) ) ;
#66617=ORIENTED_EDGE ( 'NONE', *, *, #106213, .F. ) ;
#66620=CARTESIAN_POINT ( 'NONE',  ( -22.71590553989589978, 1409.706312905169852, 209.0156571623660113 ) ) ;
#66623=CARTESIAN_POINT ( 'NONE',  ( -4.496878417739999634, 1428.155750001629940, 101.8807690336980016 ) ) ;
#66624=EDGE_CURVE ( 'NONE', #62944, #39452, #28372, .T. ) ;
#66625=CARTESIAN_POINT ( 'NONE',  ( -0.4200920693160000163, 1507.643922758529925, 237.3276516554979878 ) ) ;
#66628=CARTESIAN_POINT ( 'NONE',  ( 44.13469765186309957, 1449.794459338159868, 269.0171759414279791 ) ) ;
#66629=CARTESIAN_POINT ( 'NONE',  ( -1.210427285455619950, 1424.150940588480125, 228.3852517110850044 ) ) ;
#66630=CARTESIAN_POINT ( 'NONE',  ( -0.3973369724709999717, 1418.672808243929921, 184.7148013090980214 ) ) ;
#66632=ORIENTED_EDGE ( 'NONE', *, *, #95252, .F. ) ;
#66633=CARTESIAN_POINT ( 'NONE',  ( 18.94672925339437342, 1457.565180153704205, 226.7986852134035871 ) ) ;
#66638=CARTESIAN_POINT ( 'NONE',  ( 26.79276161880000018, 1451.726218324329693, 135.7942559489979999 ) ) ;
#66640=CARTESIAN_POINT ( 'NONE',  ( 0.3648627223273580023, 1452.900319100310071, 152.5217687494670145 ) ) ;
#66642=CARTESIAN_POINT ( 'NONE',  ( 16.87240902346729854, 1409.502257893559772, 222.1138755377239988 ) ) ;
#66644=CARTESIAN_POINT ( 'NONE',  ( 12.20337053245270020, 1409.339211476720038, 191.6948814310479747 ) ) ;
#66645=CARTESIAN_POINT ( 'NONE',  ( -13.11275527770450111, 1434.829963905530121, 149.0799834946710121 ) ) ;
#66646=CARTESIAN_POINT ( 'NONE',  ( -11.22085813611739979, 1414.913060387329779, 220.6193216859199993 ) ) ;
#66651=CARTESIAN_POINT ( 'NONE',  ( 12.78776258890000150, 1416.851343897030119, 222.2791103843980238 ) ) ;
#66657=B_SPLINE_CURVE_WITH_KNOTS ( 'NONE', 3,
 ( #59475, #60027, #25274, #24717, #42109, #49959, #50519, #25826, #94145, #101425, #34249, #17416, #103089, #92489, #41561, #669, #8482, #109322, #68988, #93045, #34800, #126, #109862, #84095 ),
 .UNSPECIFIED., .F., .F.,
 ( 4, 2, 2, 1, 1, 1, 1, 1, 1, 2, 2, 2, 2, 2, 4 ),
 ( 0.000000000000000000, 0.2499999999998854805, 0.3749999999998297473, 0.4374999999998017697, 0.4687499999997883360, 0.4843749999997818412, 0.4921874999997785660, 0.4960937499997771227, 0.4980468749997753464, 0.4990234374997746247, 0.4999999999997739586, 0.7499999999998890887, 0.8124999999999159561, 0.8749999999999427125, 1.000000000000000000 ),
 .UNSPECIFIED. ) ;
#66659=CARTESIAN_POINT ( 'NONE',  ( -2.451271202390000070, 1433.447543843880112, 150.3250444719979839 ) ) ;
#66660=CARTESIAN_POINT ( 'NONE',  ( -21.95659415135585846, 1509.539901157007534, 191.3931345191016931 ) ) ;
#66661=CARTESIAN_POINT ( 'NONE',  ( -12.87561223598270033, 1428.667272998819954, 222.5140706137790119 ) ) ;
#66662=CARTESIAN_POINT ( 'NONE',  ( 29.75208676419999776, 1462.665512622030064, 268.3665355201979992 ) ) ;
#66663=CARTESIAN_POINT ( 'NONE',  ( 13.15726442270000085, 1416.851343897030119, 196.3340833727979771 ) ) ;
#66664=CARTESIAN_POINT ( 'NONE',  ( 1.213697692988580545, 1466.857525291594811, 235.2505294708204246 ) ) ;
#66665=CARTESIAN_POINT ( 'NONE',  ( -9.202936508599998788, 1519.913060387329779, 230.3262217860979888 ) ) ;
#66668=CARTESIAN_POINT ( 'NONE',  ( -19.61825196109999681, 1486.333718774929821, 189.8690818786980117 ) ) ;
#66670=CARTESIAN_POINT ( 'NONE',  ( 17.54299231450000107, 1415.063410489729904, 210.2814835228880099 ) ) ;
#66671=CARTESIAN_POINT ( 'NONE',  ( 23.70212955589999737, 1410.915617627129905, 211.1403328626279858 ) ) ;
#66674=CARTESIAN_POINT ( 'NONE',  ( 12.45642912959999826, 1416.822692871130130, 223.4763060122980107 ) ) ;
#66677=CARTESIAN_POINT ( 'NONE',  ( -11.41806921110000062, 1414.913060387329779, 220.8525480562979908 ) ) ;
#66678=CARTESIAN_POINT ( 'NONE',  ( 0.2023891958416690062, 1461.642228596550012, 182.8826039181769829 ) ) ;
#66679=CARTESIAN_POINT ( 'NONE',  ( -5.619561408211779963, 1407.449627137000107, 221.3655341017839930 ) ) ;
#66684=CARTESIAN_POINT ( 'NONE',  ( 11.87905392670000104, 1433.311775745339901, 149.9804763676980031 ) ) ;
#66685=CARTESIAN_POINT ( 'NONE',  ( -41.63323805074259809, 1443.027121606309947, 134.0999999981200119 ) ) ;
#66686=DIRECTION ( 'NONE',  ( -0.7067700477543440440, -0.03085664260726115465, 0.7067700950127487891 ) ) ;
#66687=ORIENTED_EDGE ( 'NONE', *, *, #59018, .F. ) ;
#66696=CARTESIAN_POINT ( 'NONE',  ( 3.500000000000000000, 1420.857604035629947, 170.3256330572980062 ) ) ;
#66697=CARTESIAN_POINT ( 'NONE',  ( 2.662604276420000193, 1436.925442033910031, 183.9139560369979733 ) ) ;
#66701=CARTESIAN_POINT ( 'NONE',  ( -30.93305786360000198, 1450.544576909440138, 136.3330928348979967 ) ) ;
#66702=CARTESIAN_POINT ( 'NONE',  ( -15.91753217932039632, 1410.856834153720001, 226.7185307615260115 ) ) ;
#66703=CARTESIAN_POINT ( 'NONE',  ( 11.60004869885203682, 1428.983126981193436, 137.0999999980966777 ) ) ;
#66707=B_SPLINE_CURVE_WITH_KNOTS ( 'NONE', 3,
 ( #68137, #84889, #33379, #26078, #51298, #75955 ),
 .UNSPECIFIED., .F., .F.,
 ( 4, 2, 4 ),
 ( 0.000000000000000000, 0.5000000000000001110, 1.000000000000000000 ),
 .UNSPECIFIED. ) ;
#66708=CARTESIAN_POINT ( 'NONE',  ( -20.22565842890162813, 1410.979628444421451, 220.3650596930099823 ) ) ;
#66710=CARTESIAN_POINT ( 'NONE',  ( -0.3936502047466580168, 1418.683933865910149, 184.7134515189369779 ) ) ;
#66713=CARTESIAN_POINT ( 'NONE',  ( 21.48911905780000353, 1409.663476963630046, 214.7487920242479902 ) ) ;
#66715=CARTESIAN_POINT ( 'NONE',  ( -17.36099134979999903, 1423.305661865730144, 226.7048953899980006 ) ) ;
#66716=CARTESIAN_POINT ( 'NONE',  ( -10.96878236979999954, 1432.307827591499972, 151.7701597093980013 ) ) ;
#66721=B_SPLINE_CURVE_WITH_KNOTS ( 'NONE', 5,
 ( #36133, #62470, #28276, #88192, #11485, #77583, #10363, #61910, #61361, #17631, #79246, #28835, #18747, #9272, #70318 ),
 .UNSPECIFIED., .F., .F.,
 ( 6, 3, 3, 3, 6 ),
 ( 0.000000000000000000, 0.3593463541239135250, 0.6253129843951757971, 0.8912796146636228212, 1.000000000000000000 ),
 .UNSPECIFIED. ) ;
#66723=EDGE_CURVE ( 'NONE', #52165, #12260, #95610, .T. ) ;
#66725=CARTESIAN_POINT ( 'NONE',  ( 2.500000000000000000, 1448.197706736549890, 167.4845663187979881 ) ) ;
#66728=CARTESIAN_POINT ( 'NONE',  ( -4.226271147029579289, 1441.565518713930032, 166.0303910921570036 ) ) ;
#66733=ORIENTED_EDGE ( 'NONE', *, *, #58323, .F. ) ;
#66736=CARTESIAN_POINT ( 'NONE',  ( -11.44511274162072922, 1425.476693466300048, 144.6899562955641727 ) ) ;
#66737=CARTESIAN_POINT ( 'NONE',  ( 16.01538719336489791, 1409.574438585999815, 192.4055768128030195 ) ) ;
#66739=CARTESIAN_POINT ( 'NONE',  ( 41.33979271583219628, 1441.992233827169912, 136.3820788539130149 ) ) ;
#66742=CARTESIAN_POINT ( 'NONE',  ( 16.20733605427863466, 1461.062281268581728, 229.2672831881708646 ) ) ;
#66745=CARTESIAN_POINT ( 'NONE',  ( 35.94635777376459629, 1451.396212934409959, 134.0999999986040052 ) ) ;
#66747=ORIENTED_EDGE ( 'NONE', *, *, #59412, .F. ) ;
#66750=CARTESIAN_POINT ( 'NONE',  ( 4.500000000000000000, 1417.575542696430148, 161.0097146498980010 ) ) ;
#66751=ORIENTED_EDGE ( 'NONE', *, *, #110155, .T. ) ;
#66753=CARTESIAN_POINT ( 'NONE',  ( -29.73446499118736241, 1509.991171415641929, 209.9271895720580119 ) ) ;
#66755=CARTESIAN_POINT ( 'NONE',  ( 0.2353718297500000112, 1450.904841021550055, 181.9002531089979868 ) ) ;
#66757=CARTESIAN_POINT ( 'NONE',  ( -2.500000000000000000, 1439.450741932119854, 162.6867559029170138 ) ) ;
#66758=ADVANCED_FACE ( 'NONE', ( #98876 ), #73321, .T. ) ;
#66759=CARTESIAN_POINT ( 'NONE',  ( -15.81201443571409904, 1506.433683733589987, 193.8503163142329981 ) ) ;
#66761=CARTESIAN_POINT ( 'NONE',  ( 36.37832870499009630, 1435.767865672110020, 135.0591074476149913 ) ) ;
#66767=EDGE_LOOP ( 'NONE', ( #88761, #30474, #4911, #11920, #50835 ) ) ;
#66772=CARTESIAN_POINT ( 'NONE',  ( 11.81027685177540043, 1428.753867292769883, 148.6741505271899939 ) ) ;
#66773=CARTESIAN_POINT ( 'NONE',  ( 19.44271374779999917, 1487.524084985929903, 228.4659268090980220 ) ) ;
#66774=ORIENTED_EDGE ( 'NONE', *, *, #69348, .T. ) ;
#66775=CARTESIAN_POINT ( 'NONE',  ( -14.45750869480000134, 1416.828040475729949, 221.3916373288979855 ) ) ;
#66779=CARTESIAN_POINT ( 'NONE',  ( -12.90256217089999957, 1426.055024770130103, 222.3411140444979992 ) ) ;
#66780=CARTESIAN_POINT ( 'NONE',  ( -10.29555775080639002, 1446.577085899077929, 153.2855484792325171 ) ) ;
#66782=CARTESIAN_POINT ( 'NONE',  ( 7.229059247251790943, 1441.096153942899946, 154.2643636836130270 ) ) ;
#66783=CARTESIAN_POINT ( 'NONE',  ( -17.16792151400000321, 1507.624001480129891, 224.4229799719980178 ) ) ;
#66784=CARTESIAN_POINT ( 'NONE',  ( 12.17526685459999847, 1461.764631763230000, 233.4497560276980153 ) ) ;
#66785=CARTESIAN_POINT ( 'NONE',  ( -3.045280019940000305, 1464.258769156330118, 184.9382089438980188 ) ) ;
#66789=DIRECTION ( 'NONE',  ( 0.000000000000000000, 0.000000000000000000, 1.000000000000000000 ) ) ;
#66790=CARTESIAN_POINT ( 'NONE',  ( -0.01329177500952799865, 1508.926402960789801, 179.5289494733509912 ) ) ;
#66799=CARTESIAN_POINT ( 'NONE',  ( -11.76893999620000031, 1432.294269540009964, 150.8119674620979822 ) ) ;
#66802=CARTESIAN_POINT ( 'NONE',  ( 11.81421920076309995, 1428.091863512399868, 150.2203696085690012 ) ) ;
#66804=CARTESIAN_POINT ( 'NONE',  ( -2.446787376320000096, 1432.353341358199941, 150.2884730787980061 ) ) ;
#66805=CARTESIAN_POINT ( 'NONE',  ( -25.53892276620000246, 1482.721804240530219, 213.6785391664080009 ) ) ;
#66810=CARTESIAN_POINT ( 'NONE',  ( 9.852114434889999828, 1407.017073787930030, 269.2595063332979635 ) ) ;
#66811=CARTESIAN_POINT ( 'NONE',  ( 0.009290522623869999774, 1410.298660454629953, 185.0095042931980061 ) ) ;
#66813=CARTESIAN_POINT ( 'NONE',  ( 14.45783227242900004, 1416.839692127189892, 196.8516148535319985 ) ) ;
#66814=CARTESIAN_POINT ( 'NONE',  ( -0.2730513641314620266, 1508.977834863310136, 238.8681177356729961 ) ) ;
#66817=CARTESIAN_POINT ( 'NONE',  ( 14.14095063499999938, 1460.769213631630237, 232.7918287509980075 ) ) ;
#66819=CARTESIAN_POINT ( 'NONE',  ( -13.05435892270000053, 1444.863344029789914, 186.3556100537979887 ) ) ;
#66820=CARTESIAN_POINT ( 'NONE',  ( 1.469498570049999842, 1450.684669992949921, 155.6080914330979965 ) ) ;
#66821=DIRECTION ( 'NONE',  ( 0.9417419115949662300, -0.2378257470769920556, 0.2378257470769920556 ) ) ;
#66822=CARTESIAN_POINT ( 'NONE',  ( 15.45910333959999861, 1409.623955960430067, 270.0849031534979758 ) ) ;
#66823=CARTESIAN_POINT ( 'NONE',  ( 1.455936843708680151, 1499.898551737820071, 181.4280194235350052 ) ) ;
#66825=CARTESIAN_POINT ( 'NONE',  ( 11.44337041098931884, 1425.811177062257002, 138.6327568690129510 ) ) ;
#66827=CARTESIAN_POINT ( 'NONE',  ( -4.991700414389999452, 1475.854790790129982, 268.4734068006980579 ) ) ;
#66829=CARTESIAN_POINT ( 'NONE',  ( -20.99782421929999643, 1509.712776153829964, 187.9222525847980023 ) ) ;
#66833=CARTESIAN_POINT ( 'NONE',  ( 12.06130973522970073, 1415.890045859200200, 223.3762606109779938 ) ) ;
#66834=CARTESIAN_POINT ( 'NONE',  ( -25.74355351751919940, 1470.054056054910006, 210.8602373093899871 ) ) ;
#66837=CARTESIAN_POINT ( 'NONE',  ( -21.69939614430000319, 1409.835269271030029, 202.8599322941780088 ) ) ;
#66839=CARTESIAN_POINT ( 'NONE',  ( -15.49863863286799948, 1421.635490484141883, 227.2930321168060175 ) ) ;
#66840=CARTESIAN_POINT ( 'NONE',  ( -37.66082768700000116, 1421.358466341330086, 269.1862046009979395 ) ) ;
#66843=CARTESIAN_POINT ( 'NONE',  ( -3.460923246345533943, 1410.410939174867508, 232.3865415841924857 ) ) ;
#66847=PLANE ( 'NONE',  #19243 ) ;
#66848=CARTESIAN_POINT ( 'NONE',  ( 13.89554995500000167, 1452.733480491630189, 223.3956528723979886 ) ) ;
#66851=CARTESIAN_POINT ( 'NONE',  ( 39.63966549301360232, 1448.134706967000056, 136.4410930580840215 ) ) ;
#66853=CARTESIAN_POINT ( 'NONE',  ( -0.4331437097091430100, 1420.567764534569960, 183.4025247420120195 ) ) ;
#66856=CARTESIAN_POINT ( 'NONE',  ( -13.22475641109999955, 1415.063410489829948, 220.7066272063979966 ) ) ;
#66858=CARTESIAN_POINT ( 'NONE',  ( -20.86040077545140647, 1508.959081886482636, 190.3921826379178128 ) ) ;
#66860=CARTESIAN_POINT ( 'NONE',  ( 20.49664126143500198, 1509.564783478530217, 230.0195525190269734 ) ) ;
#66863=VERTEX_POINT ( 'NONE', #103266 ) ;
#66864=ORIENTED_EDGE ( 'NONE', *, *, #3034, .F. ) ;
#66865=CARTESIAN_POINT ( 'NONE',  ( 11.71402527498609913, 1434.165202139100074, 151.1281046944980062 ) ) ;
#66867=CARTESIAN_POINT ( 'NONE',  ( -4.791785870520000046, 1396.080393236430155, 219.8298651381980164 ) ) ;
#66873=CARTESIAN_POINT ( 'NONE',  ( -14.22567049866490052, 1509.383945902550067, 183.2093469327639923 ) ) ;
#66874=CARTESIAN_POINT ( 'NONE',  ( 15.83539164919999997, 1468.698963289930134, 189.4138077346979969 ) ) ;
#66876=DIRECTION ( 'NONE',  ( -0.03489949670258984948, -0.9993908270190926535, 0.000000000000000000 ) ) ;
#66879=CARTESIAN_POINT ( 'NONE',  ( 1.064544241010000114, 1415.263254644529979, 191.1462797974980106 ) ) ;
#66880=CARTESIAN_POINT ( 'NONE',  ( 10.96948772520000048, 1432.349142915770017, 151.7703043505979963 ) ) ;
#66881=CARTESIAN_POINT ( 'NONE',  ( 5.450092238964659330, 1509.109689566522320, 180.1788934176617261 ) ) ;
#66883=CARTESIAN_POINT ( 'NONE',  ( 13.30485551143830136, 1434.923289955479959, 149.2654130802310135 ) ) ;
#66886=VERTEX_POINT ( 'NONE', #59653 ) ;
#66887=CARTESIAN_POINT ( 'NONE',  ( -19.00201092185649898, 1497.942407030830054, 229.3262107436430028 ) ) ;
#66888=CARTESIAN_POINT ( 'NONE',  ( -4.015348745509998984, 1465.563087846730014, 234.9746089298979825 ) ) ;
#66892=ADVANCED_FACE ( 'NONE', ( #93231 ), #68610, .F. ) ;
#66893=ORIENTED_EDGE ( 'NONE', *, *, #107778, .T. ) ;
#66902=CARTESIAN_POINT ( 'NONE',  ( -21.01954463430000430, 1509.698214774029793, 230.2158738807979717 ) ) ;
#66903=CARTESIAN_POINT ( 'NONE',  ( -11.54610603179999906, 1410.690116826029907, 189.0374836358980133 ) ) ;
#66905=CARTESIAN_POINT ( 'NONE',  ( -0.02268235318324710037, 1415.088136167450102, 226.1092841930270083 ) ) ;
#66906=VERTEX_POINT ( 'NONE', #77003 ) ;
#66907=CARTESIAN_POINT ( 'NONE',  ( 19.90855454129999913, 1426.369513873829874, 221.4890869410980088 ) ) ;
#66908=CARTESIAN_POINT ( 'NONE',  ( 4.363122647530000009, 1419.257904667329967, 165.6263425522979844 ) ) ;
#66911=CARTESIAN_POINT ( 'NONE',  ( 5.260635151189210212, 1409.438182731229972, 270.3705377465669812 ) ) ;
#66913=CARTESIAN_POINT ( 'NONE',  ( 24.13962150589999922, 1410.980605758129968, 209.1808452922209938 ) ) ;
#66918=CARTESIAN_POINT ( 'NONE',  ( 13.66603629819999810, 1410.384381565130070, 271.1218459616979999 ) ) ;
#66920=CARTESIAN_POINT ( 'NONE',  ( 3.912681475688819521, 1422.009998005289162, 137.0999999980402038 ) ) ;
#66924=CARTESIAN_POINT ( 'NONE',  ( 43.50124903029999501, 1440.913060358479925, 263.8967010685980199 ) ) ;
#66926=CARTESIAN_POINT ( 'NONE',  ( -14.49383181622579997, 1422.099016211560183, 229.4564907068830166 ) ) ;
#66929=CARTESIAN_POINT ( 'NONE',  ( 1.530052826864370052, 1452.704406626560058, 183.4894965714629791 ) ) ;
#66932=LINE ( 'NONE', #50662, #98325 ) ;
#66936=ORIENTED_EDGE ( 'NONE', *, *, #33674, .T. ) ;
#66938=CARTESIAN_POINT ( 'NONE',  ( 1.600048698852036821, 1402.754281879943164, 137.0999999980979851 ) ) ;
#66940=CARTESIAN_POINT ( 'NONE',  ( 22.10609025900000191, 1451.545546232430070, 221.1255554720980001 ) ) ;
#66944=CARTESIAN_POINT ( 'NONE',  ( 14.56058096671784696, 1420.278162403178612, 228.1987085794017389 ) ) ;
#66945=CARTESIAN_POINT ( 'NONE',  ( 30.84777211902780181, 1435.574755141710057, 135.1614299696309729 ) ) ;
#66946=CARTESIAN_POINT ( 'NONE',  ( 38.06107368031250360, 1448.769205308820119, 136.3873687041340190 ) ) ;
#66947=CARTESIAN_POINT ( 'NONE',  ( 18.97170715521336959, 1506.426094403162324, 220.2326835074680105 ) ) ;
#66948=CARTESIAN_POINT ( 'NONE',  ( -42.03398950740197648, 1454.231940949233831, 269.0747901792028642 ) ) ;
#66950=CARTESIAN_POINT ( 'NONE',  ( 8.365518969610000966, 1508.201463035029974, 182.8802338420979936 ) ) ;
#66954=ORIENTED_EDGE ( 'NONE', *, *, #44527, .F. ) ;
#66956=CARTESIAN_POINT ( 'NONE',  ( -32.91875957721972412, 1417.237689351310792, 269.2963688217181470 ) ) ;
#66958=CARTESIAN_POINT ( 'NONE',  ( 14.71671434821139890, 1437.593839606849997, 190.2862900904850108 ) ) ;
#66959=CARTESIAN_POINT ( 'NONE',  ( -0.02064597189409999797, 1416.982031923930208, 234.1905971974979934 ) ) ;
#66960=CARTESIAN_POINT ( 'NONE',  ( -12.96700364194406063, 1444.896546755032659, 186.2391592067185115 ) ) ;
#66961=DIRECTION ( 'NONE',  ( 0.000000000000000000, 0.000000000000000000, 1.000000000000000000 ) ) ;
#66964=CARTESIAN_POINT ( 'NONE',  ( -25.25200574389469921, 1450.804213008409988, 137.6134964715130025 ) ) ;
#66965=CARTESIAN_POINT ( 'NONE',  ( 24.93753932649999783, 1435.554748705289967, 136.7196437487980063 ) ) ;
#66966=CARTESIAN_POINT ( 'NONE',  ( -12.54032227232971941, 1442.774810664047664, 169.4746785633205377 ) ) ;
#66967=CARTESIAN_POINT ( 'NONE',  ( -13.82592499520000118, 1409.562390380129955, 226.4595049929980064 ) ) ;
#66968=ORIENTED_EDGE ( 'NONE', *, *, #65961, .T. ) ;
#66969=CARTESIAN_POINT ( 'NONE',  ( 0.1558546717571289986, 1414.913057860449953, 192.7215652979920151 ) ) ;
#66970=CARTESIAN_POINT ( 'NONE',  ( -1.331498055899999811, 1408.959557324029902, 231.4960598541979948 ) ) ;
#66971=ORIENTED_EDGE ( 'NONE', *, *, #57100, .F. ) ;
#66974=CARTESIAN_POINT ( 'NONE',  ( 12.71038950080000163, 1507.471771860230092, 233.3404623603979928 ) ) ;
#66975=CARTESIAN_POINT ( 'NONE',  ( -11.71230443242549057, 1428.980197708463947, 142.1750151601944196 ) ) ;
#66976=CARTESIAN_POINT ( 'NONE',  ( -8.693754259799998607, 1462.836994988729884, 231.7886756190980009 ) ) ;
#66978=CARTESIAN_POINT ( 'NONE',  ( -11.87682048279999947, 1433.080538608139932, 149.9786578666980006 ) ) ;
#66982=CARTESIAN_POINT ( 'NONE',  ( -24.11734200909999970, 1437.967381767040024, 211.4545393857079887 ) ) ;
#66984=CARTESIAN_POINT ( 'NONE',  ( 2.208852557009999718, 1450.292621906749901, 182.8591303368980050 ) ) ;
#66987=CARTESIAN_POINT ( 'NONE',  ( -2.613846493977370076E-09, 1415.477284282600067, 242.7389708432399971 ) ) ;
#66990=EDGE_CURVE ( 'NONE', #75001, #63161, #38307, .T. ) ;
#66991=CARTESIAN_POINT ( 'NONE',  ( -11.85313930576219832, 1431.434453636790067, 149.9099107531910136 ) ) ;
#66993=CARTESIAN_POINT ( 'NONE',  ( -5.319674814159999876, 1473.030992683929981, 270.4258975184980613 ) ) ;
#66996=CARTESIAN_POINT ( 'NONE',  ( 38.60868605548520094, 1450.040723184470153, 135.2652482427139944 ) ) ;
#67000=CARTESIAN_POINT ( 'NONE',  ( 12.78743207240877844, 1416.839570626248587, 223.0777679028553280 ) ) ;
#67001=CARTESIAN_POINT ( 'NONE',  ( -17.20730882039999798, 1475.513060387329915, 197.3895399271980011 ) ) ;
#67005=CARTESIAN_POINT ( 'NONE',  ( -20.31811729283709766, 1410.278425004400106, 269.5165023367199524 ) ) ;
#67006=CARTESIAN_POINT ( 'NONE',  ( -13.03512055435489891, 1436.019541896100236, 150.7289522397179837 ) ) ;
#67007=EDGE_LOOP ( 'NONE', ( #85559, #7403, #15420, #17799 ) ) ;
#67009=B_SPLINE_SURFACE_WITH_KNOTS ( 'NONE', 5, 5, ( 
 ( #43921, #10309, #97090, #61856, #88694, #78068 ),
 ( #78628, #11975, #46156, #80286, #3602, #1371 ),
 ( #79196, #52889, #37725, #44482, #71929, #69706 ),
 ( #35513, #36081, #27671, #95976, #19237, #53446 ),
 ( #10880, #45052, #70821, #2502, #104933, #28220 ),
 ( #64606, #81917, #82486, #47783, #47234, #107127 ) ),
 .UNSPECIFIED., .F., .F., .F.,
 ( 6, 6 ),
 ( 6, 6 ),
 ( 30.40177460600000003, 157.7844419379999863 ),
 ( 0.000000000000000000, 1.000000000000000000 ),
 .UNSPECIFIED. ) ;
#67013=CARTESIAN_POINT ( 'NONE',  ( 4.998158967913196804, 1422.670539410961510, 184.4254624145364119 ) ) ;
#67018=CARTESIAN_POINT ( 'NONE',  ( -17.60022530830000065, 1470.471392115730168, 189.3785151195980063 ) ) ;
#67020=CARTESIAN_POINT ( 'NONE',  ( -18.18137326301040346, 1507.608478571330124, 229.7139312028679967 ) ) ;
#67021=B_SPLINE_SURFACE_WITH_KNOTS ( 'NONE', 5, 5, ( 
 ( #47714, #5148, #107609, #6247, #40397, #74573, #32001, #66189, #100309, #23594, #95218, #24668, #102493, #17370, #50475, #71, #109816, #9545, #25227, #33095, #103615, #26913, #94658, #85150, #101939, #61101, #8436 ),
 ( #43715, #51015, #58867, #34202, #41513, #42609, #8997, #76762, #77866, #59981, #34753, #75672, #86812, #68941, #85701, #17929, #52127, #25783, #51568, #43169, #18479, #67828, #69493, #77323, #59430, #16273, #84599 ),
 ( #16815, #52676, #94099, #622, #93542, #92997, #103042, #26339, #1176, #60536, #68386, #86255, #35306, #67284, #101376, #7890, #42061, #76212, #110357, #33634, #88476, #45391, #12299, #28564, #3387, #44277, #55433 ),
 ( #63300, #97418, #71149, #96879, #11760, #97954, #36405, #38066, #20148, #70597, #95766, #19033, #11229, #62194, #2294, #45930, #72243, #71718, #80065, #20688, #44836, #36953, #78421, #61636, #105272, #53234, #29114 ),
 ( #54885, #3938, #104713, #54345, #21224, #62762, #89010, #63843, #35871, #79530, #46491, #80624, #96321, #37515, #105836, #106370, #29657, #28006, #10104, #19598, #87376, #1732, #70055, #104166, #27452, #10670, #78991 ),
 ( #53801, #87938, #2832, #82271, #64938, #108012, #13943, #100172, #108572, #4475, #22331, #39720, #40263, #81160, #13387, #30757, #57651, #14500, #56532, #90660, #6107, #91763, #47574, #106911, #48133, #21779, #48690 ) ),
 .UNSPECIFIED., .F., .F., .F.,
 ( 6, 6 ),
 ( 6, 3, 3, 3, 3, 3, 3, 3, 6 ),
 ( 2.214628081880000376, 99.53245534100000214 ),
 ( 27.66703433360000020, 34.17017220330000526, 36.60162405750000403, 37.81734998450000518, 38.42521294809999688, 39.03307591160000101, 39.44313445199999535, 39.85319299230000212, 40.67331007300000323 ),
 .UNSPECIFIED. ) ;
#67025=B_SPLINE_SURFACE_WITH_KNOTS ( 'NONE', 3, 5, ( 
 ( #19924, #54123, #105612, #80950, #21565, #90989 ),
 ( #108354, #23778, #89890, #99934, #73672, #109466 ),
 ( #40594, #14277, #65269, #47347, #57428, #81475 ),
 ( #13161, #99380, #48468, #30537, #39498, #98843 ) ),
 .UNSPECIFIED., .F., .F., .F.,
 ( 4, 4 ),
 ( 6, 6 ),
 ( 5.479561967899999608, 5.505632814020000154 ),
 ( 0.000000000000000000, 1.000000000000000000 ),
 .UNSPECIFIED. ) ;
#67028=CARTESIAN_POINT ( 'NONE',  ( -2.807027225260000147, 1408.949922547829829, 194.9270130112979871 ) ) ;
#67033=CARTESIAN_POINT ( 'NONE',  ( 27.78146449860000189, 1508.131230137430066, 211.9290048573379863 ) ) ;
#67036=CARTESIAN_POINT ( 'NONE',  ( -23.93699678040000123, 1435.351892431589931, 137.2158235772980106 ) ) ;
#67037=CARTESIAN_POINT ( 'NONE',  ( -24.39131474979999936, 1441.263362519649945, 211.3484880528980057 ) ) ;
#67040=CARTESIAN_POINT ( 'NONE',  ( -1.858959159852470178, 1484.242442314900018, 182.8691889360869993 ) ) ;
#67042=CARTESIAN_POINT ( 'NONE',  ( -12.98226561589999939, 1414.913060387329779, 219.9156672276980089 ) ) ;
#67045=ORIENTED_EDGE ( 'NONE', *, *, #62468, .F. ) ;
#67046=CARTESIAN_POINT ( 'NONE',  ( -2.639044490659959941, 1451.958037943090176, 184.7018172437709893 ) ) ;
#67048=CARTESIAN_POINT ( 'NONE',  ( -19.50204366554770274, 1457.206926615194106, 226.0571257576273183 ) ) ;
#67049=VERTEX_POINT ( 'NONE', #54036 ) ;
#67051=FACE_OUTER_BOUND ( 'NONE', #109408, .T. ) ;
#67052=CARTESIAN_POINT ( 'NONE',  ( -4.107056636162540464, 1441.387641401842757, 184.3702559431454233 ) ) ;
#67055=CARTESIAN_POINT ( 'NONE',  ( -10.98289517778636792, 1424.968082807670953, 138.3353964325996515 ) ) ;
#67058=CARTESIAN_POINT ( 'NONE',  ( 4.224932291032190257, 1441.576670139289718, 166.5005718325089958 ) ) ;
#67061=CARTESIAN_POINT ( 'NONE',  ( 21.02506697189999940, 1509.639958400629894, 188.3976031865980190 ) ) ;
#67064=CARTESIAN_POINT ( 'NONE',  ( -18.53418666356940037, 1507.620785846770104, 229.7143111648900060 ) ) ;
#67066=CARTESIAN_POINT ( 'NONE',  ( 0.1469571361719999858, 1420.465545067329913, 183.3355639602979750 ) ) ;
#67075=CARTESIAN_POINT ( 'NONE',  ( 17.38836599616480427, 1422.723741091718466, 226.5637347084151259 ) ) ;
#67077=CARTESIAN_POINT ( 'NONE',  ( 18.80339027203730140, 1425.953307585449693, 225.0197318394450008 ) ) ;
#67078=CARTESIAN_POINT ( 'NONE',  ( -8.661115458674929329E-07, 1407.922920414400096, 222.3762974436029936 ) ) ;
#67079=CARTESIAN_POINT ( 'NONE',  ( 42.85777160514339812, 1440.913060354170057, 263.0145395452340153 ) ) ;
#67080=EDGE_CURVE ( 'NONE', #85866, #109412, #70844, .T. ) ;
#67083=CARTESIAN_POINT ( 'NONE',  ( 12.78671360849999772, 1416.817366564930126, 222.1376795749980033 ) ) ;
#67085=VERTEX_POINT ( 'NONE', #90896 ) ;
#67087=AXIS2_PLACEMENT_3D ( 'NONE', #37536, #61126, #95239 ) ;
#67089=CARTESIAN_POINT ( 'NONE',  ( -27.87492310950000274, 1509.195406832029903, 210.7637215495180101 ) ) ;
#67092=CARTESIAN_POINT ( 'NONE',  ( 27.56820608061211075, 1509.987796949902304, 220.9537938550800220 ) ) ;
#67093=CARTESIAN_POINT ( 'NONE',  ( -5.473890262062679923, 1440.659206222230068, 154.7842680559549819 ) ) ;
#67100=VERTEX_POINT ( 'NONE', #91999 ) ;
#67102=B_SPLINE_SURFACE_WITH_KNOTS ( 'NONE', 5, 4, ( 
 ( #58420, #16373, #16919, #69045, #34857 ),
 ( #60642, #26449, #7997, #34304, #50571 ),
 ( #41049, #8544, #109379, #42162, #32656 ),
 ( #110465, #33742, #17474, #102587, #59526 ),
 ( #42718, #100941, #92546, #15814, #68486 ),
 ( #25886, #50018, #41614, #104828, #63413 ),
 ( #43821, #71266, #97528, #18587, #103720 ),
 ( #28114, #20255, #27565, #78530, #88591 ),
 ( #19710, #53913, #80179, #35415, #53342 ) ),
 .UNSPECIFIED., .F., .F., .F.,
 ( 6, 3, 6 ),
 ( 5, 5 ),
 ( -1.776356839400000001E-15, 5.782490304330000441, 11.25975508159999983 ),
 ( 25.78146411700000229, 39.23969207129999859 ),
 .UNSPECIFIED. ) ;
#67105=VERTEX_POINT ( 'NONE', #22555 ) ;
#67110=CARTESIAN_POINT ( 'NONE',  ( -38.60856581307790236, 1443.613625294319945, 137.1750438966080026 ) ) ;
#67114=CARTESIAN_POINT ( 'NONE',  ( 41.66021864449999867, 1443.875655612860101, 135.6929158170979974 ) ) ;
#67116=CARTESIAN_POINT ( 'NONE',  ( 23.84533589473599946, 1452.080362908450070, 136.9869410992479857 ) ) ;
#67117=CARTESIAN_POINT ( 'NONE',  ( 0.9336696193000000310, 1408.945664848729848, 186.1949048084980234 ) ) ;
#67120=CARTESIAN_POINT ( 'NONE',  ( -3.134579720209279774, 1440.880072796180002, 159.2383936985540061 ) ) ;
#67124=CARTESIAN_POINT ( 'NONE',  ( -0.8167354255590000278, 1432.353341358199941, 150.3995506339979897 ) ) ;
#67125=CARTESIAN_POINT ( 'NONE',  ( -9.736852438091474937, 1428.340212313232087, 134.0999999980979567 ) ) ;
#67126=CARTESIAN_POINT ( 'NONE',  ( 14.91777843120000036, 1430.152623513529988, 190.7961912442980008 ) ) ;
#67127=CARTESIAN_POINT ( 'NONE',  ( -8.598089374990029619E-11, 1469.758488426850136, 253.3729536691440387 ) ) ;
#67129=CARTESIAN_POINT ( 'NONE',  ( -1.547118986179999878, 1416.568813549730066, 228.0093688194979791 ) ) ;
#67130=ADVANCED_FACE ( 'NONE', ( #48366 ), #22325, .T. ) ;
#67133=AXIS2_PLACEMENT_3D ( 'NONE', #79013, #61660, #28582 ) ;
#67136=CARTESIAN_POINT ( 'NONE',  ( -46.27883891992610188, 1440.696393458320017, 267.5894411246799791 ) ) ;
#67140=CARTESIAN_POINT ( 'NONE',  ( -2.478627793510000288, 1436.625092229730171, 157.6517990276980186 ) ) ;
#67141=B_SPLINE_SURFACE_WITH_KNOTS ( 'NONE', 5, 5, ( 
 ( #61544, #53708, #44742, #78892, #2198, #2747 ),
 ( #62668, #96789, #20059, #32332, #106815, #14951 ),
 ( #83278, #13294, #6576, #108484, #64857, #97862 ),
 ( #55344, #21137, #89478, #98966, #12773, #22240 ),
 ( #49146, #22791, #81070, #91126, #40725, #90017 ),
 ( #99508, #107927, #73798, #74356, #39053, #90569 ),
 ( #31767, #6021, #82730, #39630, #65954, #31220 ),
 ( #65402, #47487, #72692, #56996, #4385, #64301 ),
 ( #14403, #74898, #48596, #13847, #48032, #100078 ) ),
 .UNSPECIFIED., .F., .F., .F.,
 ( 6, 3, 6 ),
 ( 6, 6 ),
 ( 0.7655572723400000390, 2.316155491850000026, 3.835724788489999870 ),
 ( 0.000000000000000000, 1.000000000000000000 ),
 .UNSPECIFIED. ) ;
#67144=CARTESIAN_POINT ( 'NONE',  ( -26.62605130868620051, 1450.898279949580001, 136.4493292573559984 ) ) ;
#67146=CARTESIAN_POINT ( 'NONE',  ( -3.034064455719999779E-09, 1416.682256071730080, 238.2947578363979915 ) ) ;
#67152=CARTESIAN_POINT ( 'NONE',  ( 0.4666204826262328464, 1415.437692837088889, 233.3904393389156269 ) ) ;
#67153=CARTESIAN_POINT ( 'NONE',  ( 20.59684415639999955, 1507.762623716630060, 209.5602205471840023 ) ) ;
#67154=EDGE_LOOP ( 'NONE', ( #8772, #47864, #45554, #6956 ) ) ;
#67155=CARTESIAN_POINT ( 'NONE',  ( 14.27715652531434820, 1416.818673809773600, 196.5253453210812609 ) ) ;
#67159=ORIENTED_EDGE ( 'NONE', *, *, #69252, .T. ) ;
#67161=CARTESIAN_POINT ( 'NONE',  ( -22.97501113406280382, 1409.745379998360249, 209.4185639539470003 ) ) ;
#67166=CARTESIAN_POINT ( 'NONE',  ( -12.32958673350000112, 1507.632494499530139, 233.3296017327979825 ) ) ;
#67167=FACE_OUTER_BOUND ( 'NONE', #88532, .T. ) ;
#67168=CARTESIAN_POINT ( 'NONE',  ( 46.11011654448370223, 1442.803748059199961, 268.2059351147869961 ) ) ;
#67170=CARTESIAN_POINT ( 'NONE',  ( -1.462741316680280068, 1424.166085031260081, 228.3696464465570273 ) ) ;
#67171=CARTESIAN_POINT ( 'NONE',  ( -17.05655558861789345, 1422.119710870798144, 226.7808225676212430 ) ) ;
#67173=ORIENTED_EDGE ( 'NONE', *, *, #43218, .T. ) ;
#67174=CARTESIAN_POINT ( 'NONE',  ( 18.36669116892507958, 1459.044192910584343, 227.7581707921801524 ) ) ;
#67177=ORIENTED_EDGE ( 'NONE', *, *, #37186, .T. ) ;
#67178=CARTESIAN_POINT ( 'NONE',  ( 2.994866067409999832, 1448.618510723430063, 183.8359025843979850 ) ) ;
#67179=CARTESIAN_POINT ( 'NONE',  ( 26.71026096653610082, 1451.513660524960187, 136.0795779202579752 ) ) ;
#67181=CARTESIAN_POINT ( 'NONE',  ( 0.8647627281377370245, 1452.882862207440212, 152.5191013288349779 ) ) ;
#67185=CARTESIAN_POINT ( 'NONE',  ( 2.038497153056070044, 1408.984246276509793, 186.9383856488950073 ) ) ;
#67186=CARTESIAN_POINT ( 'NONE',  ( 1.324323477659999915, 1416.409446159829940, 233.0341864379980166 ) ) ;
#67187=PLANE ( 'NONE',  #45802 ) ;
#67190=ADVANCED_FACE ( 'NONE', ( #98745 ), #9100, .F. ) ;
#67191=DIRECTION ( 'NONE',  ( 0.3282391760791589785, -0.000000000000000000, 0.9445946449598763284 ) ) ;
#67193=CARTESIAN_POINT ( 'NONE',  ( 12.78353013627689982, 1416.221314539589912, 221.8283297262470057 ) ) ;
#67194=CARTESIAN_POINT ( 'NONE',  ( -4.500000000000000000, 1411.429641636930000, 127.2892455880980123 ) ) ;
#67203=CARTESIAN_POINT ( 'NONE',  ( 6.661338147749999709E-15, 1470.874276671130019, 268.3665355202980436 ) ) ;
#67204=CARTESIAN_POINT ( 'NONE',  ( -21.46027262497062793, 1509.101876609105830, 191.8002388787112693 ) ) ;
#67206=CARTESIAN_POINT ( 'NONE',  ( 11.16482994470000101, 1433.388395248510051, 151.6286288133979951 ) ) ;
#67207=CARTESIAN_POINT ( 'NONE',  ( 6.092217245739999676, 1469.463552837929910, 265.6112250856980381 ) ) ;
#67208=CARTESIAN_POINT ( 'NONE',  ( 11.70695556603179988, 1414.913057860449953, 197.6353021862890103 ) ) ;
#67212=CARTESIAN_POINT ( 'NONE',  ( -22.86388141640000171, 1443.913060387330006, 134.0999999980979851 ) ) ;
#67215=EDGE_CURVE ( 'NONE', #69697, #61631, #18034, .T. ) ;
#67218=CARTESIAN_POINT ( 'NONE',  ( -17.02454731339999938, 1409.507570680530080, 224.4911189336980044 ) ) ;
#67219=CARTESIAN_POINT ( 'NONE',  ( 23.88743783590000191, 1410.917949436429808, 210.4190463509079905 ) ) ;
#67225=CARTESIAN_POINT ( 'NONE',  ( -12.45618503170000047, 1416.218047894730262, 222.0802477567980304 ) ) ;
#67228=CARTESIAN_POINT ( 'NONE',  ( 0.1994830306498499850, 1463.291321531269887, 182.8118295327159899 ) ) ;
#67229=CARTESIAN_POINT ( 'NONE',  ( 0.03232803809133739242, 1407.837594165099972, 222.3069522204950204 ) ) ;
#67231=CARTESIAN_POINT ( 'NONE',  ( -13.76936860679999874, 1444.324653571829003, 176.3340081878980641 ) ) ;
#67234=CARTESIAN_POINT ( 'NONE',  ( -40.80783872826999925, 1447.308166564250087, 134.0999999984899773 ) ) ;
#67239=DIRECTION ( 'NONE',  ( -0.7067700363769178207, -0.03085824620771834489, -0.7067700363772886352 ) ) ;
#67244=CARTESIAN_POINT ( 'NONE',  ( 0.4578175030638683696, 1418.682250877671322, 184.7073717525739482 ) ) ;
#67247=CARTESIAN_POINT ( 'NONE',  ( -0.1681676274470000065, 1420.473121337229941, 182.7663689088979879 ) ) ;
#67251=VERTEX_POINT ( 'NONE', #67379 ) ;
#67253=CARTESIAN_POINT ( 'NONE',  ( -33.29550038720000060, 1451.750386302530160, 134.7337860542980081 ) ) ;
#67254=CARTESIAN_POINT ( 'NONE',  ( -15.81239927484159935, 1409.848076597319960, 226.2976557237249722 ) ) ;
#67255=VECTOR ( 'NONE', #103067, 1000.000000000000000 ) ;
#67261=CARTESIAN_POINT ( 'NONE',  ( -20.72940845510794361, 1410.996615820652323, 219.0750059994481092 ) ) ;
#67266=CARTESIAN_POINT ( 'NONE',  ( 17.06090267708677644, 1433.319433169794138, 217.0403965233522854 ) ) ;
#67267=CARTESIAN_POINT ( 'NONE',  ( 2.879377773099999871, 1417.724437854929874, 234.4927649805979968 ) ) ;
#67270=CARTESIAN_POINT ( 'NONE',  ( 3.820241900599999510E-10, 1475.513060387329915, 229.7676991014980104 ) ) ;
#67273=CARTESIAN_POINT ( 'NONE',  ( 3.138402309729999562, 1447.047508311479987, 157.7990817848980214 ) ) ;
#67274=ORIENTED_EDGE ( 'NONE', *, *, #48895, .T. ) ;
#67276=CARTESIAN_POINT ( 'NONE',  ( 13.79590917850000054, 1416.844618635429924, 196.3342909300980068 ) ) ;
#67278=VERTEX_POINT ( 'NONE', #85802 ) ;
#67282=ORIENTED_EDGE ( 'NONE', *, *, #18644, .F. ) ;
#67284=CARTESIAN_POINT ( 'NONE',  ( -25.18172488869999981, 1449.799985351279929, 206.2325939675880022 ) ) ;
#67285=CARTESIAN_POINT ( 'NONE',  ( -11.74236480618606926, 1426.276761585844952, 144.5884759014079464 ) ) ;
#67286=CARTESIAN_POINT ( 'NONE',  ( 15.84346258294009857, 1409.719321388350181, 192.1077202728040163 ) ) ;
#67289=CARTESIAN_POINT ( 'NONE',  ( 39.77278037070129812, 1440.034032915139960, 136.7118410945930123 ) ) ;
#67290=CARTESIAN_POINT ( 'NONE',  ( 5.408518632609999834E-10, 1408.296887868130170, 262.4989398460980397 ) ) ;
#67291=DIRECTION ( 'NONE',  ( 1.000000000000000000, 0.000000000000000000, 0.000000000000000000 ) ) ;
#67294=CARTESIAN_POINT ( 'NONE',  ( 36.72650137404210113, 1451.114006374460132, 134.0999999987039644 ) ) ;
#67295=CARTESIAN_POINT ( 'NONE',  ( -35.70801268710279430, 1437.331117183020069, 136.5359098274630014 ) ) ;
#67298=DIRECTION ( 'NONE',  ( 0.000000000000000000, -0.7071067811865475727, -0.7071067811865475727 ) ) ;
#67302=ADVANCED_FACE ( 'NONE', ( #2939 ), #83391, .T. ) ;
#67307=CARTESIAN_POINT ( 'NONE',  ( 36.37832872589339672, 1435.767865734180077, 134.7402661757760143 ) ) ;
#67309=CARTESIAN_POINT ( 'NONE',  ( 27.30844321330000213, 1439.416619586579827, 137.0772895148980126 ) ) ;
#67315=ORIENTED_EDGE ( 'NONE', *, *, #74694, .F. ) ;
#67316=CARTESIAN_POINT ( 'NONE',  ( 10.79382126600000014, 1414.913060387329779, 222.1041115775979904 ) ) ;
#67320=CARTESIAN_POINT ( 'NONE',  ( -13.91566348329999947, 1415.553739809529816, 221.3028765811980065 ) ) ;
#67321=CARTESIAN_POINT ( 'NONE',  ( -12.53380499169999851, 1442.773887286369927, 169.4755105685979970 ) ) ;
#67324=CARTESIAN_POINT ( 'NONE',  ( -12.74111566449999877, 1416.823634022930037, 221.9826245047979967 ) ) ;
#67325=EDGE_CURVE ( 'NONE', #80757, #57302, #103776, .T. ) ;
#67330=CARTESIAN_POINT ( 'NONE',  ( -16.47067245780000277, 1485.103171130329883, 223.7192837535979777 ) ) ;
#67331=CARTESIAN_POINT ( 'NONE',  ( 17.94899309970000090, 1459.572665234330088, 228.0797701638979902 ) ) ;
#67334=B_SPLINE_CURVE_WITH_KNOTS ( 'NONE', 5,
 ( #44630, #80973, #10456, #79882, #71518, #36215 ),
 .UNSPECIFIED., .F., .F.,
 ( 6, 6 ),
 ( -92.88478189117469697, -23.15748665169219578 ),
 .UNSPECIFIED. ) ;
#67337=CARTESIAN_POINT ( 'NONE',  ( -1.924560002181862739, 1486.146552202361818, 181.8515281887476362 ) ) ;
#67342=CARTESIAN_POINT ( 'NONE',  ( -11.60004869885204037, 1426.058235232188963, 138.8694919005308179 ) ) ;
#67347=EDGE_CURVE ( 'NONE', #71735, #67105, #78507, .T. ) ;
#67348=CARTESIAN_POINT ( 'NONE',  ( -11.75953795439999894, 1426.408695322430049, 145.8957383316979985 ) ) ;
#67351=CARTESIAN_POINT ( 'NONE',  ( -1.010302820291719810E-14, 1421.486528639720063, 147.6331986621470094 ) ) ;
#67353=CARTESIAN_POINT ( 'NONE',  ( 7.105427357599999217E-15, 1432.413060387330006, 146.1721969590979882 ) ) ;
#67355=CARTESIAN_POINT ( 'NONE',  ( -19.02532173170000007, 1470.092591092030034, 227.7517131706979967 ) ) ;
#67356=CARTESIAN_POINT ( 'NONE',  ( -3.515242004654977492, 1419.856981650250191, 137.0999999980978430 ) ) ;
#67357=DIRECTION ( 'NONE',  ( 0.1261098496724238627, 0.9885420249951558658, -0.08295161622340639640 ) ) ;
#67360=CARTESIAN_POINT ( 'NONE',  ( 3.756404312819999980, 1406.179919416030089, 269.0400515133979980 ) ) ;
#67362=CARTESIAN_POINT ( 'NONE',  ( 19.84704116899999704, 1449.730418169799805, 193.3609370523980147 ) ) ;
#67365=CARTESIAN_POINT ( 'NONE',  ( -0.1579380382326590060, 1508.143587606610026, 237.5556629045009913 ) ) ;
#67367=CARTESIAN_POINT ( 'NONE',  ( -1.757532404670000048, 1451.933574905729756, 184.1885909310980196 ) ) ;
#67368=CARTESIAN_POINT ( 'NONE',  ( 16.63395377013535636, 1459.015803111507921, 231.1847133987910468 ) ) ;
#67370=CARTESIAN_POINT ( 'NONE',  ( -13.02484207390000037, 1445.915793797939841, 187.8647291817979976 ) ) ;
#67371=CARTESIAN_POINT ( 'NONE',  ( -15.98141629860000101, 1475.513060387329915, 223.7206687197979988 ) ) ;
#67376=CARTESIAN_POINT ( 'NONE',  ( -18.57221558799999883, 1434.150321635919909, 219.6133835466979747 ) ) ;
#67379=CARTESIAN_POINT ( 'NONE',  ( -14.49383181622579997, 1422.099016211560183, 229.4564907068830166 ) ) ;
#67380=CARTESIAN_POINT ( 'NONE',  ( -9.911219186020000294, 1475.204444335230164, 267.1956757164980445 ) ) ;
#67381=CARTESIAN_POINT ( 'NONE',  ( 1.361307284737899970, 1413.955589619809871, 232.7931714649010075 ) ) ;
#67387=CARTESIAN_POINT ( 'NONE',  ( 11.53151684852190151, 1415.184612916159949, 222.8541440776940021 ) ) ;
#67389=CARTESIAN_POINT ( 'NONE',  ( 2.500000000000000000, 1440.913060387330006, 137.0999999980979851 ) ) ;
#67390=CARTESIAN_POINT ( 'NONE',  ( -45.88374309256568750, 1440.913026864722724, 266.4124039852627561 ) ) ;
#67391=( BOUNDED_SURFACE ( )  B_SPLINE_SURFACE ( 4, 2, ( 
 ( #43121, #33584, #25734 ),
 ( #77280, #34703, #51515 ),
 ( #93496, #15665, #85648 ),
 ( #577, #68895, #50970 ),
 ( #9503, #102997, #7303 ) ),
 .UNSPECIFIED., .F., .F., .F. ) 
 B_SPLINE_SURFACE_WITH_KNOTS ( ( 5, 5 ),
 ( 3, 3 ),
 ( 3.613988937040000238, 5.260361675040000407 ),
 ( 5.300753508049940166, 6.150222949633159963 ),
 .UNSPECIFIED. ) 
 GEOMETRIC_REPRESENTATION_ITEM ( )  RATIONAL_B_SPLINE_SURFACE ( (
 ( 0.8627701935039370218, 0.8230338693346749279, 0.9546124223293859234),
 ( 0.8627701935039370218, 0.8230338693346749279, 0.9546124223293859234),
 ( 0.8627701935039370218, 0.8230338693346749279, 0.9546124223293859234),
 ( 0.8627701935039370218, 0.8230338693346749279, 0.9546124223293859234),
 ( 0.8627701935039370218, 0.8230338693346749279, 0.9546124223293859234) ) ) 
 REPRESENTATION_ITEM ( '' )  SURFACE ( )  );
#67392=CARTESIAN_POINT ( 'NONE',  ( -22.19955145049999956, 1411.048519434129958, 202.6338174844580067 ) ) ;
#67396=CARTESIAN_POINT ( 'NONE',  ( 2.500000000000000000, 1443.913060387330006, 150.6726614421979775 ) ) ;
#67402=CARTESIAN_POINT ( 'NONE',  ( 11.73199753003260071, 1426.699139563339941, 143.8094287576769830 ) ) ;
#67406=CARTESIAN_POINT ( 'NONE',  ( -0.06052882951021919949, 1420.434688371959965, 183.3377468054080168 ) ) ;
#67408=DIRECTION ( 'NONE',  ( -0.08330058268155800250, -0.04363816682463637214, -0.9955685427538869536 ) ) ;
#67409=FACE_OUTER_BOUND ( 'NONE', #108550, .T. ) ;
#67413=CARTESIAN_POINT ( 'NONE',  ( 19.99715769724119951, 1508.853444755030068, 229.3809204472839838 ) ) ;
#67414=AXIS2_PLACEMENT_3D ( 'NONE', #66152, #31960, #34167 ) ;
#67418=CARTESIAN_POINT ( 'NONE',  ( 11.98355472118069898, 1433.631889606809864, 149.9631560847739706 ) ) ;
#67419=CARTESIAN_POINT ( 'NONE',  ( -11.29356329139999993, 1396.307440307529987, 211.1970805475479835 ) ) ;
#67426=CARTESIAN_POINT ( 'NONE',  ( 18.73044736589999815, 1507.815472637730181, 230.0234365859979846 ) ) ;
#67427=( BOUNDED_CURVE ( )  B_SPLINE_CURVE ( 3, ( #91090, #42345, #60265, #9299 ),
 .UNSPECIFIED., .F., .T. ) 
 B_SPLINE_CURVE_WITH_KNOTS ( ( 4, 4 ),
 ( 1.268017761107936181, 1.928411118409885106 ),
 .UNSPECIFIED. ) 
 CURVE ( )  GEOMETRIC_REPRESENTATION_ITEM ( )  RATIONAL_B_SPLINE_CURVE ( ( 1.000000000000000000, 0.9639857285903185025, 0.9639857285903185025, 1.000000000000000000 ) ) 
 REPRESENTATION_ITEM ( '' )  );
#67428=CARTESIAN_POINT ( 'NONE',  ( 0.6876992757690000291, 1429.776213807130034, 184.2878479203979794 ) ) ;
#67430=CARTESIAN_POINT ( 'NONE',  ( 42.06232107069909887, 1440.913053860320133, 269.6487541118979721 ) ) ;
#67433=CARTESIAN_POINT ( 'NONE',  ( -1.547462741870939906, 1414.913060391199906, 225.9340804956229931 ) ) ;
#67434=CARTESIAN_POINT ( 'NONE',  ( 11.76160536819999969, 1431.728708710070123, 150.7840645346979898 ) ) ;
#67437=CARTESIAN_POINT ( 'NONE',  ( 13.06529732548069944, 1434.818778377569970, 149.3188580375970105 ) ) ;
#67440=CARTESIAN_POINT ( 'NONE',  ( 13.44971459290628601, 1444.299826105456532, 169.3629876352260055 ) ) ;
#67441=CARTESIAN_POINT ( 'NONE',  ( -4.894696787210000011, 1465.369418360130112, 234.6993435765979825 ) ) ;
#67442=CARTESIAN_POINT ( 'NONE',  ( -8.866214871307620982, 1407.269089423789865, 199.4203128504979929 ) ) ;
#67449=VERTEX_POINT ( 'NONE', #39256 ) ;
#67451=ORIENTED_EDGE ( 'NONE', *, *, #16679, .F. ) ;
#67452=CARTESIAN_POINT ( 'NONE',  ( 20.33301140202129886, 1440.913060387330006, 218.5204036554350182 ) ) ;
#67454=CARTESIAN_POINT ( 'NONE',  ( -11.89919548239999969, 1409.328589449730089, 190.2794074207979804 ) ) ;
#67456=CARTESIAN_POINT ( 'NONE',  ( -0.7266101759396799142, 1414.971717244350202, 226.0555041422940121 ) ) ;
#67458=CARTESIAN_POINT ( 'NONE',  ( 22.72408229139999847, 1432.100443994239868, 218.1715127473280234 ) ) ;
#67461=FACE_OUTER_BOUND ( 'NONE', #97558, .T. ) ;
#67463=CIRCLE ( 'NONE', #85324, 1.638701816490922836 ) ;
#67470=CARTESIAN_POINT ( 'NONE',  ( 14.29520360740000129, 1410.788278508630128, 191.3967167922980082 ) ) ;
#67471=DIRECTION ( 'NONE',  ( 0.7067699325522937004, 0.03085807370314938569, -0.7067701477335875948 ) ) ;
#67475=EDGE_CURVE ( 'NONE', #85422, #65987, #93044, .T. ) ;
#67476=CARTESIAN_POINT ( 'NONE',  ( 34.48978216820000142, 1440.913060384829805, 250.0021841762979875 ) ) ;
#67479=CARTESIAN_POINT ( 'NONE',  ( -3.454294121580000265, 1417.605600631229890, 235.1430308038980002 ) ) ;
#67481=CARTESIAN_POINT ( 'NONE',  ( -24.02240277289999781, 1444.576888666170134, 212.2493134410879918 ) ) ;
#67490=CARTESIAN_POINT ( 'NONE',  ( 0.2341451561260000092, 1497.013800431029949, 230.6965820202980240 ) ) ;
#67491=VECTOR ( 'NONE', #10497, 1000.000000000000114 ) ;
#67497=CARTESIAN_POINT ( 'NONE',  ( 14.94073065363653008, 1420.536355086338062, 228.0011852406256025 ) ) ;
#67498=CARTESIAN_POINT ( 'NONE',  ( 32.00873930189860062, 1435.615230547090050, 135.1257559928430112 ) ) ;
#67499=CARTESIAN_POINT ( 'NONE',  ( 38.29258608828820343, 1448.551925925989963, 136.4167175071939937 ) ) ;
#67502=CARTESIAN_POINT ( 'NONE',  ( 10.23468988059999951, 1508.269291830929888, 183.6304174551979997 ) ) ;
#67504=CARTESIAN_POINT ( 'NONE',  ( -27.06221056512304912, 1464.234489086119765, 269.4420994688821338 ) ) ;
#67507=CARTESIAN_POINT ( 'NONE',  ( -11.29656894142413037, 1407.765265707235130, 269.6109022948709253 ) ) ;
#67509=CARTESIAN_POINT ( 'NONE',  ( 16.12453495796710001, 1481.913039286089997, 188.8995036690789959 ) ) ;
#67510=CARTESIAN_POINT ( 'NONE',  ( 10.91296393538931220, 1424.870198133627355, 138.2545201306494960 ) ) ;
#67513=CARTESIAN_POINT ( 'NONE',  ( -28.25086640909999858, 1508.135711191930113, 208.8579954691720104 ) ) ;
#67518=CARTESIAN_POINT ( 'NONE',  ( -14.65103220135884499, 1451.163773513072101, 149.9447318886720382 ) ) ;
#67520=CARTESIAN_POINT ( 'NONE',  ( 24.74089786250000245, 1435.642227076270046, 137.1785840707979958 ) ) ;
#67521=CARTESIAN_POINT ( 'NONE',  ( -12.95651626014300639, 1442.923275661127491, 169.4280452214743775 ) ) ;
#67522=ADVANCED_FACE ( 'NONE', ( #98609 ), #26012, .F. ) ;
#67526=ORIENTED_EDGE ( 'NONE', *, *, #73287, .T. ) ;
#67527=VERTEX_POINT ( 'NONE', #2117 ) ;
#67531=CARTESIAN_POINT ( 'NONE',  ( -16.00255113769999937, 1456.293564252130182, 216.3706747924380238 ) ) ;
#67533=CARTESIAN_POINT ( 'NONE',  ( 4.292760611305180163, 1425.438012504090239, 185.4035972331899984 ) ) ;
#67536=CARTESIAN_POINT ( 'NONE',  ( -2.656119403435029280, 1420.364487350997479, 185.9144866987654154 ) ) ;
#67538=CARTESIAN_POINT ( 'NONE',  ( -24.23237730770000198, 1438.888001088869942, 211.7327264377979645 ) ) ;
#67540=CARTESIAN_POINT ( 'NONE',  ( 0.003568499702431209702, 1467.142144108200000, 235.6416276161930057 ) ) ;
#67543=CARTESIAN_POINT ( 'NONE',  ( -6.317740384107130598E-10, 1416.973155798829794, 237.0820494564949854 ) ) ;
#67548=CARTESIAN_POINT ( 'NONE',  ( -4.101685208650000192, 1471.292125227329961, 269.3367844517979961 ) ) ;
#67549=CARTESIAN_POINT ( 'NONE',  ( 11.87563351815570023, 1433.006677199550040, 147.6591432317509884 ) ) ;
#67551=CARTESIAN_POINT ( 'NONE',  ( 19.67658020740000069, 1453.313060387329870, 209.1218459613160121 ) ) ;
#67554=CARTESIAN_POINT ( 'NONE',  ( -21.62349440730000083, 1475.513060387329915, 208.1442046935659960 ) ) ;
#67557=CARTESIAN_POINT ( 'NONE',  ( -15.46812277936250091, 1408.003561489749927, 268.9519026408210038 ) ) ;
#67558=CARTESIAN_POINT ( 'NONE',  ( -13.51745720335679835, 1434.977168586970038, 149.1397909361569987 ) ) ;
#67561=ORIENTED_EDGE ( 'NONE', *, *, #65318, .T. ) ;
#67564=CARTESIAN_POINT ( 'NONE',  ( -21.99231067425982999, 1506.446781340468078, 209.3764100870739355 ) ) ;
#67567=CARTESIAN_POINT ( 'NONE',  ( -19.10795447410000136, 1485.490635589229896, 189.6432606092980109 ) ) ;
#67569=CARTESIAN_POINT ( 'NONE',  ( -16.98603930835629683, 1470.451025123820045, 228.5667710449559991 ) ) ;
#67574=CARTESIAN_POINT ( 'NONE',  ( -28.75306173559999579, 1509.589359939629958, 208.3584206130200016 ) ) ;
#67575=CARTESIAN_POINT ( 'NONE',  ( 11.60004869885204570, 1426.273943615695998, 138.2686089212693332 ) ) ;
#67581=CARTESIAN_POINT ( 'NONE',  ( -26.85728217208029989, 1488.762426835850192, 210.5633333958139701 ) ) ;
#67582=CARTESIAN_POINT ( 'NONE',  ( 26.47779523700000226, 1469.247571737029830, 210.0128041243490031 ) ) ;
#67585=CARTESIAN_POINT ( 'NONE',  ( -13.24677860586930045, 1436.091658137889908, 150.6304371349799851 ) ) ;
#67586=CARTESIAN_POINT ( 'NONE',  ( -24.47138174589999693, 1442.190446117989950, 211.0555081549980230 ) ) ;
#67591=CARTESIAN_POINT ( 'NONE',  ( -12.98226561589999939, 1414.913060387329779, 219.9156672276980089 ) ) ;
#67594=DIRECTION ( 'NONE',  ( 6.546194519182246997E-06, 0.000000000000000000, 0.9999999999785736948 ) ) ;
#67596=DIRECTION ( 'NONE',  ( -3.334807482003173289E-08, 5.770116306383727380E-11, -0.9999999999999995559 ) ) ;
#67597=EDGE_LOOP ( 'NONE', ( #39640, #67974, #22588, #82759, #88451, #72120 ) ) ;
#67599=CARTESIAN_POINT ( 'NONE',  ( 12.74071504291650037, 1434.633262964860023, 149.4353413572609952 ) ) ;
#67600=CARTESIAN_POINT ( 'NONE',  ( 17.21575504016569980, 1459.307510025329975, 228.5504449505849891 ) ) ;
#67602=CARTESIAN_POINT ( 'NONE',  ( 26.07120187149999779, 1452.002625937929906, 135.0137028555979839 ) ) ;
#67606=CIRCLE ( 'NONE', #53309, 29.83173541461230727 ) ;
#67608=FACE_OUTER_BOUND ( 'NONE', #43731, .T. ) ;
#67614=ORIENTED_EDGE ( 'NONE', *, *, #100669, .F. ) ;
#67616=ADVANCED_FACE ( 'NONE', ( #1551 ), #95594, .F. ) ;
#67621=CARTESIAN_POINT ( 'NONE',  ( 17.41395121031547788, 1422.770471704767260, 226.5406294010037413 ) ) ;
#67623=DIRECTION ( 'NONE',  ( 1.000000000000000000, 0.000000000000000000, 0.000000000000000000 ) ) ;
#67625=CARTESIAN_POINT ( 'NONE',  ( -2.461716435160000049, 1435.943783413959864, 150.4083956814980070 ) ) ;
#67626=CARTESIAN_POINT ( 'NONE',  ( 44.10764275524749678, 1440.913060362949864, 264.4775968722539687 ) ) ;
#67629=DIRECTION ( 'NONE',  ( -0.7074300732371815448, 0.02470400256250997878, 0.7063514732320074208 ) ) ;
#67632=ORIENTED_EDGE ( 'NONE', *, *, #9021, .T. ) ;
#67636=CARTESIAN_POINT ( 'NONE',  ( -29.15071157469999719, 1509.931025666729965, 211.8621304569779795 ) ) ;
#67637=CARTESIAN_POINT ( 'NONE',  ( 2.352760052573430016, 1410.373437767319956, 185.5341168253151523 ) ) ;
#67639=CARTESIAN_POINT ( 'NONE',  ( 11.78238356083980065, 1440.882651838439870, 188.1224447589279976 ) ) ;
#67642=B_SPLINE_CURVE_WITH_KNOTS ( 'NONE', 3,
 ( #67077, #93892, #101181, #41848, #83849, #41305, #75478, #109611, #24476, #16072, #58664, #50274, #84404, #76003, #33426, #25025, #59227 ),
 .UNSPECIFIED., .F., .F.,
 ( 4, 2, 2, 1, 1, 1, 2, 2, 2, 4 ),
 ( 0.000000000000000000, 0.2499999999972815079, 0.3749999999959241492, 0.4374999999953910201, 0.4687499999951194596, 0.4843749999949900076, 0.4921874999949239493, 0.4999999999948580021, 0.7499999999974289455, 1.000000000000000000 ),
 .UNSPECIFIED. ) ;
#67647=CARTESIAN_POINT ( 'NONE',  ( 24.18195368869999839, 1450.840504138970118, 140.0925686386979976 ) ) ;
#67648=CARTESIAN_POINT ( 'NONE',  ( -27.12970500513406336, 1508.933968740432874, 212.0467364469421909 ) ) ;
#67654=CARTESIAN_POINT ( 'NONE',  ( -16.38529656942809964, 1409.485247551910106, 224.6959546567310042 ) ) ;
#67655=VERTEX_POINT ( 'NONE', #69874 ) ;
#67659=CARTESIAN_POINT ( 'NONE',  ( 40.09667693707910274, 1442.092650259239917, 136.9432980588629789 ) ) ;
#67661=CARTESIAN_POINT ( 'NONE',  ( 1.682318894840000079, 1409.475163267829885, 232.0401757884979759 ) ) ;
#67668=CARTESIAN_POINT ( 'NONE',  ( 3.642177762369999794, 1409.207669089330011, 186.4969686919980063 ) ) ;
#67671=CARTESIAN_POINT ( 'NONE',  ( 11.86614525289999911, 1432.349253981680022, 150.3971727848980038 ) ) ;
#67672=CARTESIAN_POINT ( 'NONE',  ( -22.65242742670000098, 1452.122020190730154, 139.7531684575980080 ) ) ;
#67673=CARTESIAN_POINT ( 'NONE',  ( 0.2762028305379999882, 1466.385324525529995, 235.6853349533979838 ) ) ;
#67677=CARTESIAN_POINT ( 'NONE',  ( -2.409586283469999923, 1426.663880916129983, 144.1938086916980239 ) ) ;
#67678=CARTESIAN_POINT ( 'NONE',  ( -27.74152896854549866, 1446.393007474169963, 137.1637341980870133 ) ) ;
#67680=CARTESIAN_POINT ( 'NONE',  ( 17.14891132210000180, 1507.633349707429943, 188.2623345620979762 ) ) ;
#67681=CARTESIAN_POINT ( 'NONE',  ( -7.045284513412829670E-09, 1472.436258976460067, 259.9932842362949827 ) ) ;
#67682=CARTESIAN_POINT ( 'NONE',  ( -20.00399723164029808, 1488.559828140339960, 190.9486810803579999 ) ) ;
#67684=CARTESIAN_POINT ( 'NONE',  ( -0.4967073768120000010, 1415.438070335630073, 233.3911243366979988 ) ) ;
#67689=CARTESIAN_POINT ( 'NONE',  ( -45.97429859279590403, 1438.843789423260205, 266.6795026073090185 ) ) ;
#67696=CARTESIAN_POINT ( 'NONE',  ( -26.72416512552139878, 1451.509345559029953, 136.0758556284789904 ) ) ;
#67698=CARTESIAN_POINT ( 'NONE',  ( 24.66839858290000009, 1432.416040610029995, 225.6916884349980137 ) ) ;
#67700=CARTESIAN_POINT ( 'NONE',  ( 15.39496762990000001, 1488.801231227030030, 194.1127781847980032 ) ) ;
#67702=CARTESIAN_POINT ( 'NONE',  ( -19.16951723229999871, 1456.627470220629903, 228.8719212425980061 ) ) ;
#67704=CARTESIAN_POINT ( 'NONE',  ( -23.84533141485470153, 1452.080363065020038, 136.9869391916130041 ) ) ;
#67705=CARTESIAN_POINT ( 'NONE',  ( -9794.298952052929963, 2837.541834147239570, -1088.485032349865833 ) ) ;
#67707=CARTESIAN_POINT ( 'NONE',  ( -0.6132286398022869234, 1408.236656115740061, 270.3925693042170337 ) ) ;
#67708=CARTESIAN_POINT ( 'NONE',  ( 10.54373566122539962, 1419.511555201090005, 230.6885890306220119 ) ) ;
#67712=CARTESIAN_POINT ( 'NONE',  ( -22.73045215911909978, 1409.706683828489986, 209.4201699003199906 ) ) ;
#67714=DIRECTION ( 'NONE',  ( -2.513978196838388281E-18, -0.7071067811865475727, -0.7071067811865475727 ) ) ;
#67715=CARTESIAN_POINT ( 'NONE',  ( -6.742596065479999901, 1428.329919402730184, 101.8807690336980016 ) ) ;
#67718=CARTESIAN_POINT ( 'NONE',  ( -18.78618306029910201, 1416.259629939410161, 207.5733126889130062 ) ) ;
#67720=CIRCLE ( 'NONE', #40924, 0.5866484772300107897 ) ;
#67721=CARTESIAN_POINT ( 'NONE',  ( 22.61737647487870007, 1471.968567494569925, 267.6424710453320017 ) ) ;
#67723=CARTESIAN_POINT ( 'NONE',  ( -17.15598988914259238, 1422.277001189961311, 226.7238155055327411 ) ) ;
#67727=CARTESIAN_POINT ( 'NONE',  ( 18.34455336298703543, 1459.088291602529353, 227.7786510797382959 ) ) ;
#67730=ORIENTED_EDGE ( 'NONE', *, *, #70167, .T. ) ;
#67732=CARTESIAN_POINT ( 'NONE',  ( 26.92792935968680013, 1450.870610057039812, 136.4174504459710136 ) ) ;
#67734=CARTESIAN_POINT ( 'NONE',  ( -1.546867746862319981, 1416.839692133689823, 228.0214409764060122 ) ) ;
#67738=CARTESIAN_POINT ( 'NONE',  ( 1.185993768368289958, 1408.954476202319938, 186.7131526092149727 ) ) ;
#67739=CARTESIAN_POINT ( 'NONE',  ( 2.004290588779999993, 1417.602443405030044, 234.4383503574979954 ) ) ;
#67745=CARTESIAN_POINT ( 'NONE',  ( 12.74994028582560013, 1415.933499560010205, 221.6250176366550022 ) ) ;
#67746=FACE_OUTER_BOUND ( 'NONE', #39856, .T. ) ;
#67751=CARTESIAN_POINT ( 'NONE',  ( 13.08154635940000077, 1418.696939362130024, 221.6904558216980092 ) ) ;
#67752=CARTESIAN_POINT ( 'NONE',  ( -6.438546668579999910, 1470.874276671330108, 268.3665355204980187 ) ) ;
#67754=CARTESIAN_POINT ( 'NONE',  ( 11.47665303230000156, 1433.538822946230084, 151.3125183399980074 ) ) ;
#67755=CARTESIAN_POINT ( 'NONE',  ( 3.444929440920000197, 1456.909266848530024, 224.8635561966979708 ) ) ;
#67756=CARTESIAN_POINT ( 'NONE',  ( 12.45618235599049939, 1416.218047878440075, 196.1634418539379965 ) ) ;
#67761=FACE_OUTER_BOUND ( 'NONE', #101979, .T. ) ;
#67762=CARTESIAN_POINT ( 'NONE',  ( -28.08216322107800167, 1509.932735855700003, 222.4427074788879963 ) ) ;
#67763=AXIS2_PLACEMENT_3D ( 'NONE', #11529, #63075, #2043 ) ;
#67764=CARTESIAN_POINT ( 'NONE',  ( 24.22746707339999972, 1430.355866414130105, 212.3409394264880063 ) ) ;
#67766=CARTESIAN_POINT ( 'NONE',  ( 26.79413740735880367, 1436.761939593030093, 136.7822073642480234 ) ) ;
#67772=CARTESIAN_POINT ( 'NONE',  ( 0.2069650299334150068, 1459.057086511930038, 182.9935364721550002 ) ) ;
#67777=CARTESIAN_POINT ( 'NONE',  ( 10.10004869885203682, 0.000000000000000000, 135.5999999980979851 ) ) ;
#67778=CARTESIAN_POINT ( 'NONE',  ( 12.91282902989999926, 1434.774388673019985, 149.7891053277979836 ) ) ;
#67779=CARTESIAN_POINT ( 'NONE',  ( -41.28347186119889756, 1446.141341654479902, 134.0999999985599800 ) ) ;
#67781=ORIENTED_EDGE ( 'NONE', *, *, #95252, .T. ) ;
#67782=B_SPLINE_SURFACE_WITH_KNOTS ( 'NONE', 5, 5, ( 
 ( #49214, #22304, #22861, #4449, #6638, #40793, #6087, #97930, #90635 ),
 ( #65470, #74970, #40238, #73302, #90078, #91194, #39694, #99578, #14474 ),
 ( #48102, #38576, #82242, #21198, #13360, #89539, #81133, #81672, #39122 ),
 ( #107436, #73861, #107989, #31285, #102341, #83894, #34596, #102881, #51400 ),
 ( #7199, #26179, #66580, #41355, #85532, #59818, #50854, #15563, #77713 ),
 ( #75523, #33472, #8827, #100684, #9399, #110752, #23968, #101779, #109656 ) ),
 .UNSPECIFIED., .F., .F., .F.,
 ( 6, 6 ),
 ( 6, 3, 6 ),
 ( 7.509787108449399895, 11.13865211956250079 ),
 ( -3.527284231174740019E-05, 1.000000000000000000, 2.000000000000000000 ),
 .UNSPECIFIED. ) ;
#67787=EDGE_CURVE ( 'NONE', #31041, #43965, #12918, .T. ) ;
#67789=CARTESIAN_POINT ( 'NONE',  ( -2.021663551027474082, 1408.983658434181052, 187.9413203637166987 ) ) ;
#67792=CARTESIAN_POINT ( 'NONE',  ( -5.367207161296789764, 1422.334098476926783, 140.1444612193151897 ) ) ;
#67797=ORIENTED_EDGE ( 'NONE', *, *, #92401, .F. ) ;
#67798=AXIS2_PLACEMENT_3D ( 'NONE', #103526, #44198, #28490 ) ;
#67799=CARTESIAN_POINT ( 'NONE',  ( -33.92643244749999809, 1451.728353150429939, 135.1493689542980121 ) ) ;
#67800=CARTESIAN_POINT ( 'NONE',  ( 13.51610093809999924, 1443.501467202829872, 169.3501091259980171 ) ) ;
#67805=DIRECTION ( 'NONE',  ( -0.7071068048275286344, 1.153083735983437180E-10, -0.7071067575455656229 ) ) ;
#67810=CARTESIAN_POINT ( 'NONE',  ( 16.64291266002331326, 1432.692105207829854, 217.7214433012767358 ) ) ;
#67811=CARTESIAN_POINT ( 'NONE',  ( 1.707043585809999930, 1416.544879546130005, 232.5604860032980241 ) ) ;
#67812=CARTESIAN_POINT ( 'NONE',  ( 2.500000000000000000, 1431.405490181040022, 183.1416673786320075 ) ) ;
#67813=DIRECTION ( 'NONE',  ( -0.4874171250595387694, 0.8731692540388111823, 0.000000000000000000 ) ) ;
#67814=CARTESIAN_POINT ( 'NONE',  ( 22.17671526344968314, 1509.715724164745325, 189.3973745417270038 ) ) ;
#67824=CARTESIAN_POINT ( 'NONE',  ( 40.65896460247470401, 1444.188686613040090, 137.0313705377079998 ) ) ;
#67828=CARTESIAN_POINT ( 'NONE',  ( -24.69009492209999834, 1430.360063187129981, 207.6875836211879971 ) ) ;
#67829=CARTESIAN_POINT ( 'NONE',  ( -11.67474245070000016, 1426.737381196229762, 139.7158479479979860 ) ) ;
#67830=CARTESIAN_POINT ( 'NONE',  ( 16.50452789831379974, 1410.127611398650060, 191.9106860492449869 ) ) ;
#67833=CARTESIAN_POINT ( 'NONE',  ( 16.28988456800818341, 1509.602866217699102, 183.9209087581965321 ) ) ;
#67834=EDGE_CURVE ( 'NONE', #99393, #80584, #71684, .T. ) ;
#67836=CARTESIAN_POINT ( 'NONE',  ( -37.00344541100000129, 1420.039541595830087, 266.5575487690979912 ) ) ;
#67839=CARTESIAN_POINT ( 'NONE',  ( 11.36622730368661038, 1464.114352876782277, 231.8218590705467932 ) ) ;
#67841=CARTESIAN_POINT ( 'NONE',  ( -39.32574430968750079, 1440.209197080029980, 136.7482234617440042 ) ) ;
#67842=ORIENTED_EDGE ( 'NONE', *, *, #1598, .F. ) ;
#67843=CARTESIAN_POINT ( 'NONE',  ( 12.14532673125249929, 1396.857034010459984, 213.7755067647490250 ) ) ;
#67848=CARTESIAN_POINT ( 'NONE',  ( -29.60477471821983642, 1509.968944135829588, 210.6717049192871514 ) ) ;
#67854=CARTESIAN_POINT ( 'NONE',  ( 15.13342375178309851, 1507.606285622089899, 226.3974328904010065 ) ) ;
#67855=CARTESIAN_POINT ( 'NONE',  ( 33.91369104887559871, 1435.681798505150027, 135.6938344556039908 ) ) ;
#67857=CARTESIAN_POINT ( 'NONE',  ( 27.26752121369999671, 1441.515264365290022, 137.3262971963980021 ) ) ;
#67858=FACE_OUTER_BOUND ( 'NONE', #81207, .T. ) ;
#67865=CARTESIAN_POINT ( 'NONE',  ( 11.75520567813219941, 1426.817959112909875, 145.4357449278519994 ) ) ;
#67870=CARTESIAN_POINT ( 'NONE',  ( -12.93929867839810122, 1442.831169986189252, 169.4513495753611210 ) ) ;
#67872=ADVANCED_FACE ( 'NONE', ( #11048 ), #60033, .F. ) ;
#67875=CARTESIAN_POINT ( 'NONE',  ( -13.34764978429999971, 1422.966168412730212, 222.0983912147980277 ) ) ;
#67879=CARTESIAN_POINT ( 'NONE',  ( 7.701966595568799256, 1441.125018358639863, 154.1230950460079896 ) ) ;
#67881=CARTESIAN_POINT ( 'NONE',  ( -16.13533334829999788, 1485.106086671430148, 223.9657626398980028 ) ) ;
#67882=CARTESIAN_POINT ( 'NONE',  ( 17.60092044200000316, 1458.856313947630042, 228.4764048559979983 ) ) ;
#67884=CARTESIAN_POINT ( 'NONE',  ( -5.012111505640171494, 1423.085453659650284, 184.7955982197375420 ) ) ;
#67885=CARTESIAN_POINT ( 'NONE',  ( -2.499957339885570118, 1419.383124631570126, 144.0983870681699841 ) ) ;
#67898=CARTESIAN_POINT ( 'NONE',  ( -11.81835065930000006, 1428.979157509329980, 149.3874597924980208 ) ) ;
#67900=CARTESIAN_POINT ( 'NONE',  ( 31.61373788305444421, 1450.520975417251975, 136.3130673618244941 ) ) ;
#67902=B_SPLINE_CURVE_WITH_KNOTS ( 'NONE', 5,
 ( #58864, #91898, #101373, #40947, #90800, #75124, #57232, #16270, #109272 ),
 .UNSPECIFIED., .F., .F.,
 ( 6, 3, 6 ),
 ( 0.000000000000000000, 0.7318475515115363539, 1.000000000000000000 ),
 .UNSPECIFIED. ) ;
#67903=DIRECTION ( 'NONE',  ( 1.000000000000000000, 0.000000000000000000, 0.000000000000000000 ) ) ;
#67904=CARTESIAN_POINT ( 'NONE',  ( -20.65050755260000059, 1470.086394453330058, 225.2399685796980293 ) ) ;
#67906=CARTESIAN_POINT ( 'NONE',  ( -16.32520297863799996, 1459.451184924540030, 228.9510746369849983 ) ) ;
#67908=ORIENTED_EDGE ( 'NONE', *, *, #106963, .T. ) ;
#67910=CARTESIAN_POINT ( 'NONE',  ( 26.80873977519999940, 1412.873887987429953, 269.2446989046979979 ) ) ;
#67912=B_SPLINE_SURFACE_WITH_KNOTS ( 'NONE', 5, 5, ( 
 ( #94417, #36744, #43499, #34528, #53569, #17694 ),
 ( #94997, #2064, #78186, #78748, #2618, #85463 ),
 ( #36195, #27788, #35080, #53010, #35630, #27239 ),
 ( #51898, #87146, #9337, #77643, #86588, #104496 ),
 ( #93871, #69261, #103368, #9879, #87715, #69823 ),
 ( #10995, #102815, #68711, #26671, #79307, #60870 ) ),
 .UNSPECIFIED., .F., .F., .F.,
 ( 6, 6 ),
 ( 6, 6 ),
 ( 8.883702454569998963, 11.85812885390000027 ),
 ( 0.000000000000000000, 1.447371157720000134 ),
 .UNSPECIFIED. ) ;
#67913=CARTESIAN_POINT ( 'NONE',  ( 19.11094363509999994, 1430.303984236330052, 193.7458470186979866 ) ) ;
#67914=CARTESIAN_POINT ( 'NONE',  ( -0.03650439547260889844, 1507.115325378910029, 237.3518449088199986 ) ) ;
#67920=CARTESIAN_POINT ( 'NONE',  ( -12.69395104490000037, 1446.088563078959851, 187.6870124384980159 ) ) ;
#67923=ORIENTED_EDGE ( 'NONE', *, *, #89991, .T. ) ;
#67924=CARTESIAN_POINT ( 'NONE',  ( 1.462963723040370034, 1493.088310213640170, 181.7250244461219779 ) ) ;
#67929=DIRECTION ( 'NONE',  ( 0.000000000000000000, 1.000000000000000000, 0.000000000000000000 ) ) ;
#67930=CARTESIAN_POINT ( 'NONE',  ( -9.885589491230001968, 1475.057254907329934, 266.9235355597979833 ) ) ;
#67932=CARTESIAN_POINT ( 'NONE',  ( -21.68903860500000036, 1509.722673403329964, 188.7015949552979919 ) ) ;
#67934=CARTESIAN_POINT ( 'NONE',  ( 17.92070293022930016, 1421.080221703320149, 224.5097658201460149 ) ) ;
#67937=CARTESIAN_POINT ( 'NONE',  ( 11.90198537394640077, 1415.595619977620117, 223.2201660334189910 ) ) ;
#67938=B_SPLINE_SURFACE_WITH_KNOTS ( 'NONE', 5, 5, ( 
 ( #27787, #78747, #53568, #17693, #87714, #61975 ),
 ( #62536, #955, #77102, #10994, #45165, #9336 ),
 ( #17136, #1497, #36194, #70936, #42943, #18263 ),
 ( #19365, #103367, #44605, #35629, #87144, #69822 ),
 ( #2063, #35079, #26108, #9878, #85461, #79306 ),
 ( #8762, #2617, #36743, #70378, #60869, #26670 ),
 ( #52457, #44046, #104495, #51326, #410, #34527 ),
 ( #68709, #102814, #78185, #60298, #27238, #94415 ),
 ( #61419, #51897, #86038, #12643, #21015, #46821 ),
 ( #72036, #13163, #80951, #5342, #106152, #21568 ),
 ( #39501, #47901, #12084, #29431, #13715, #38385 ),
 ( #64172, #107247, #20464, #4251, #19928, #37301 ) ),
 .UNSPECIFIED., .F., .F., .F.,
 ( 6, 3, 3, 6 ),
 ( 6, 6 ),
 ( 52.42854093907030233, 57.31387688920000301, 62.19918898450000455, 65.17288249872970596 ),
 ( 0.000000000000000000, 2.000023854729739980 ),
 .UNSPECIFIED. ) ;
#67939=CARTESIAN_POINT ( 'NONE',  ( -25.20740283234720280, 1470.078870519829934, 211.7617687522999859 ) ) ;
#67942=CARTESIAN_POINT ( 'NONE',  ( -23.69114534980000286, 1411.100850862329935, 207.0316896202280361 ) ) ;
#67943=DIRECTION ( 'NONE',  ( 0.000000000000000000, 0.000000000000000000, -1.000000000000000000 ) ) ;
#67947=CARTESIAN_POINT ( 'NONE',  ( -16.35645674180000242, 1409.677081954430150, 270.0833092963979993 ) ) ;
#67948=B_SPLINE_SURFACE_WITH_KNOTS ( 'NONE', 5, 5, ( 
 ( #83318, #15538, #6613, #40766, #100657, #109630 ),
 ( #55932, #90051, #92818, #93910, #86078, #67647 ),
 ( #1540, #85505, #94460, #93364, #51370, #41868 ),
 ( #69303, #78228, #101755, #9374, #43537, #26716 ),
 ( #26152, #101199, #102312, #76573, #103411, #35674 ),
 ( #8250, #60908, #76024, #16629, #24495, #16089 ),
 ( #110725, #34014, #58685, #110174, #42416, #34568 ),
 ( #95035, #60340, #18303, #68209, #25599, #50296 ),
 ( #84424, #68753, #7709, #25043, #59245, #77682 ) ),
 .UNSPECIFIED., .F., .F., .F.,
 ( 6, 3, 6 ),
 ( 6, 6 ),
 ( 17.98526101469999716, 36.72584873329999766, 62.49779112240000245 ),
 ( 0.000000000000000000, 1.596925542399999953 ),
 .UNSPECIFIED. ) ;
#67949=DIRECTION ( 'NONE',  ( -0.7067700363771035610, 0.03085824620770448445, 0.7067700363771036720 ) ) ;
#67952=CARTESIAN_POINT ( 'NONE',  ( -36.00227781734899679, 1442.549544043670039, 137.1411661128690014 ) ) ;
#67953=CARTESIAN_POINT ( 'NONE',  ( -22.60520452300000116, 1410.200391382629959, 211.1984955222980034 ) ) ;
#67955=CARTESIAN_POINT ( 'NONE',  ( 11.72881690059139892, 1426.701155718149948, 143.5815159837019905 ) ) ;
#67960=CARTESIAN_POINT ( 'NONE',  ( 11.60004869885203149, 1428.971947790928198, 136.1000015555673315 ) ) ;
#67962=CARTESIAN_POINT ( 'NONE',  ( 22.59589169820000265, 1507.700907224229923, 227.3081670307980175 ) ) ;
#67966=CARTESIAN_POINT ( 'NONE',  ( 1.607042714549999918, 1508.277410111030122, 236.9905385516979948 ) ) ;
#67968=CARTESIAN_POINT ( 'NONE',  ( 20.31245813560099833, 1507.850129543419825, 228.7302837791660295 ) ) ;
#67972=CARTESIAN_POINT ( 'NONE',  ( 11.64843754084820127, 1434.007725651600140, 151.1673272559080203 ) ) ;
#67973=CARTESIAN_POINT ( 'NONE',  ( -5.436310085770000633, 1397.763550466030210, 221.4241563309980165 ) ) ;
#67974=ORIENTED_EDGE ( 'NONE', *, *, #46601, .T. ) ;
#67976=EDGE_CURVE ( 'NONE', #80118, #90450, #2005, .T. ) ;
#67977=CARTESIAN_POINT ( 'NONE',  ( -22.52609275360000041, 1509.699688879929909, 190.9355249643979846 ) ) ;
#67979=CARTESIAN_POINT ( 'NONE',  ( -2.500000000000529798, 1448.894380907979894, 155.6080925131469996 ) ) ;
#67981=CARTESIAN_POINT ( 'NONE',  ( 18.41333652109999974, 1507.814877555129897, 230.2405691312980025 ) ) ;
#67982=CARTESIAN_POINT ( 'NONE',  ( 12.99461696440000047, 1468.696672636130188, 187.3355539092980280 ) ) ;
#67983=CARTESIAN_POINT ( 'NONE',  ( 6.632916768162448129, 1509.144686944858449, 237.5225686160735847 ) ) ;
#67984=CARTESIAN_POINT ( 'NONE',  ( -4.500000000000000000, 1439.615672362369878, 128.3512065685980019 ) ) ;
#67985=CARTESIAN_POINT ( 'NONE',  ( 2.468689065161279839, 1395.999268909109787, 198.3831816525220120 ) ) ;
#67986=CARTESIAN_POINT ( 'NONE',  ( 14.40791762927999997, 1416.384967875050052, 196.9030818062619801 ) ) ;
#67987=CARTESIAN_POINT ( 'NONE',  ( 11.29023540169999862, 1431.477258515079939, 151.4697263553979951 ) ) ;
#67990=CARTESIAN_POINT ( 'NONE',  ( 13.42353523596650078, 1434.939809150270094, 149.0761011451980096 ) ) ;
#67993=EDGE_CURVE ( 'NONE', #110792, #94174, #43420, .T. ) ;
#67994=CARTESIAN_POINT ( 'NONE',  ( 13.32446307317308154, 1444.551246767114890, 169.3762330793057913 ) ) ;
#67995=CARTESIAN_POINT ( 'NONE',  ( -6.651410363940000181, 1465.239839440230071, 233.9266418807979733 ) ) ;
#68002=CARTESIAN_POINT ( 'NONE',  ( 2.500000000000000000, 1448.204674875420096, 169.9458606413469965 ) ) ;
#68007=CARTESIAN_POINT ( 'NONE',  ( 21.96624934842110122, 1440.913060387330006, 227.2068459464609873 ) ) ;
#68009=CARTESIAN_POINT ( 'NONE',  ( -19.75308352559999747, 1509.626197081729970, 231.2246848602980265 ) ) ;
#68010=CARTESIAN_POINT ( 'NONE',  ( -8.912128646530000253, 1409.224278777129939, 189.0536454187979984 ) ) ;
#68012=CARTESIAN_POINT ( 'NONE',  ( -0.08631495460232219141, 1416.225364278609959, 227.2130314078410152 ) ) ;
#68014=CARTESIAN_POINT ( 'NONE',  ( 20.41137819500000106, 1427.953452258230072, 221.0141490875980139 ) ) ;
#68016=EDGE_CURVE ( 'NONE', #54755, #96843, #51613, .T. ) ;
#68022=CARTESIAN_POINT ( 'NONE',  ( 23.89892804850000019, 1410.398181719029935, 209.5833347769950024 ) ) ;
#68023=CARTESIAN_POINT ( 'NONE',  ( 23.69134403178578907, 1410.129789052333081, 209.5325411534778084 ) ) ;
#68028=CARTESIAN_POINT ( 'NONE',  ( -4.982512062026007271, 1485.996114690913828, 182.4005058417187968 ) ) ;
#68030=ORIENTED_EDGE ( 'NONE', *, *, #52876, .F. ) ;
#68033=CARTESIAN_POINT ( 'NONE',  ( 6.526381463449999920, 1473.529262900630101, 262.4990045935979879 ) ) ;
#68034=CARTESIAN_POINT ( 'NONE',  ( -27.16116926167260104, 1509.861549318230118, 220.2428113040780318 ) ) ;
#68035=CARTESIAN_POINT ( 'NONE',  ( -8.664662764387241367, 1509.043723808620143, 236.1803171092909963 ) ) ;
#68038=CARTESIAN_POINT ( 'NONE',  ( 0.7059648962766970071, 1452.945346370949892, 183.3242576825529966 ) ) ;
#68040=CARTESIAN_POINT ( 'NONE',  ( 17.40660825725099770, 1409.684622116380069, 222.5152860288629881 ) ) ;
#68046=AXIS2_PLACEMENT_3D ( 'NONE', #84470, #9421, #43584 ) ;
#68048=CARTESIAN_POINT ( 'NONE',  ( 12.61640438689999932, 1416.837080256829950, 223.3238927095979989 ) ) ;
#68050=CARTESIAN_POINT ( 'NONE',  ( -6.451353027019999686, 1421.812455514629846, 186.8014209383979960 ) ) ;
#68052=CARTESIAN_POINT ( 'NONE',  ( 0.3919100467378520136, 1450.899374586919976, 181.2708617675390030 ) ) ;
#68053=CARTESIAN_POINT ( 'NONE',  ( 27.05706720676449706, 1435.442239277179851, 135.2793738133329953 ) ) ;
#68055=FACE_OUTER_BOUND ( 'NONE', #76366, .T. ) ;
#68057=CARTESIAN_POINT ( 'NONE',  ( 10.58064693039999860, 1509.111078008130107, 182.8327862588980111 ) ) ;
#68062=CARTESIAN_POINT ( 'NONE',  ( -34.06505905677735768, 1418.159631727885198, 269.2714297548777154 ) ) ;
#68063=EDGE_CURVE ( 'NONE', #28836, #94675, #59219, .T. ) ;
#68065=CARTESIAN_POINT ( 'NONE',  ( 14.00412664368519877, 1415.247667709120151, 190.9862133854840351 ) ) ;
#68067=CARTESIAN_POINT ( 'NONE',  ( 10.85845406881951192, 1424.793774302243946, 138.1921923613813590 ) ) ;
#68070=CARTESIAN_POINT ( 'NONE',  ( -13.09898176730286146, 1444.802254457625395, 186.4275170488816684 ) ) ;
#68074=DIRECTION ( 'NONE',  ( -0.1294182776648229727, -0.05003219150570591828, -0.9903270617424362321 ) ) ;
#68075=CARTESIAN_POINT ( 'NONE',  ( -38.41729418502210081, 1444.641748168739923, 137.0880170107530205 ) ) ;
#68076=CARTESIAN_POINT ( 'NONE',  ( -21.25708629881845368, 1435.239819464369702, 139.1347687532081636 ) ) ;
#68077=CARTESIAN_POINT ( 'NONE',  ( 25.70089172607919892, 1435.395012783340235, 135.4164353173910058 ) ) ;
#68078=CARTESIAN_POINT ( 'NONE',  ( -13.38944205750223126, 1443.385879950765684, 169.3692234598943287 ) ) ;
#68079=VERTEX_POINT ( 'NONE', #27708 ) ;
#68082=CARTESIAN_POINT ( 'NONE',  ( 0.1222452018807889951, 1415.427621830080170, 191.5619203254349827 ) ) ;
#68083=CARTESIAN_POINT ( 'NONE',  ( 21.72816364826307378, 1509.385241731590213, 226.6647666414965840 ) ) ;
#68085=VERTEX_POINT ( 'NONE', #107165 ) ;
#68088=CARTESIAN_POINT ( 'NONE',  ( 9.983193396660000829, 1425.227045000729959, 93.46322213869791540 ) ) ;
#68089=CARTESIAN_POINT ( 'NONE',  ( -18.28461450430000212, 1458.543868107529988, 231.7753221004980162 ) ) ;
#68091=CARTESIAN_POINT ( 'NONE',  ( 4.372068842044389392, 1425.711177915499775, 185.4562312974719873 ) ) ;
#68093=CARTESIAN_POINT ( 'NONE',  ( -2.706452301512094039, 1420.190219406222923, 186.0099876176680027 ) ) ;
#68095=CARTESIAN_POINT ( 'NONE',  ( -24.77772770919999701, 1438.702763892639950, 210.4551298550980221 ) ) ;
#68097=CARTESIAN_POINT ( 'NONE',  ( 2.706438817270000019, 1450.839219090760025, 183.6941181407979968 ) ) ;
#68099=CARTESIAN_POINT ( 'NONE',  ( -28.93059565662124299, 1510.034316939833616, 201.1399980697655963 ) ) ;
#68100=CARTESIAN_POINT ( 'NONE',  ( -1.079296730995619915E-09, 1416.674463692480231, 238.2624803028730014 ) ) ;
#68103=CARTESIAN_POINT ( 'NONE',  ( -11.75870877344729948, 1426.873346726019918, 145.6745198646130177 ) ) ;
#68104=CARTESIAN_POINT ( 'NONE',  ( -2.500000000000000000, 1448.210448412289907, 176.8331131016979896 ) ) ;
#68105=CARTESIAN_POINT ( 'NONE',  ( -5.551115123129999164E-16, 1408.913060387329779, 226.8598803041980148 ) ) ;
#68109=CYLINDRICAL_SURFACE ( 'NONE', #105518, 13.00000000000000355 ) ;
#68110=EDGE_CURVE ( 'NONE', #46740, #100339, #51717, .T. ) ;
#68113=CARTESIAN_POINT ( 'NONE',  ( -21.20437582439999957, 1519.913060387329779, 199.9189094530979958 ) ) ;
#68116=CARTESIAN_POINT ( 'NONE',  ( -6.122247995272200427, 1406.053493193089935, 267.5211899804779705 ) ) ;
#68118=CARTESIAN_POINT ( 'NONE',  ( -14.30322175442669952, 1435.879355932359886, 149.9105199582620287 ) ) ;
#68121=CARTESIAN_POINT ( 'NONE',  ( 13.86472875750000000, 1443.323743473050172, 189.2628177551980286 ) ) ;
#68122=B_SPLINE_CURVE_WITH_KNOTS ( 'NONE', 3,
 ( #29076, #63260, #87894, #44230 ),
 .UNSPECIFIED., .F., .F.,
 ( 4, 4 ),
 ( 0.000000000000000000, 1.000000000000000000 ),
 .UNSPECIFIED. ) ;
#68124=ORIENTED_EDGE ( 'NONE', *, *, #95913, .F. ) ;
#68126=CARTESIAN_POINT ( 'NONE',  ( 4.680157983689395174, 1422.155807250380803, 184.1346165008071694 ) ) ;
#68129=CARTESIAN_POINT ( 'NONE',  ( -10.61951293090000092, 1485.478317074230063, 185.0532574409980100 ) ) ;
#68131=EDGE_CURVE ( 'NONE', #45774, #64698, #66301, .T. ) ;
#68132=CARTESIAN_POINT ( 'NONE',  ( 7.121584085660000341, 1409.161751583630121, 222.2855843900980233 ) ) ;
#68133=ORIENTED_EDGE ( 'NONE', *, *, #5003, .F. ) ;
#68136=CARTESIAN_POINT ( 'NONE',  ( -28.12061240270000084, 1509.153472191830133, 206.7763965112779943 ) ) ;
#68137=CARTESIAN_POINT ( 'NONE',  ( 11.60004869885203682, 1428.983126981193436, 134.0999999980966777 ) ) ;
#68140=DIRECTION ( 'NONE',  ( -0.3363363879354877017, -0.9417419148315043786, -3.002409420756286433E-08 ) ) ;
#68144=VERTEX_POINT ( 'NONE', #13630 ) ;
#68145=CARTESIAN_POINT ( 'NONE',  ( -24.17543378828390033, 1411.086233064730095, 209.0052275329530005 ) ) ;
#68146=CARTESIAN_POINT ( 'NONE',  ( 27.09023322280000201, 1488.688618553730066, 211.1670471512279903 ) ) ;
#68149=CARTESIAN_POINT ( 'NONE',  ( 14.12038737319999804, 1509.406339941330089, 234.8413163218980060 ) ) ;
#68159=CARTESIAN_POINT ( 'NONE',  ( -2.798509278424440083, 1451.959363124020001, 184.7388509875849820 ) ) ;
#68160=CARTESIAN_POINT ( 'NONE',  ( -10.16202339710000047, 1410.292653515729853, 229.5428569793980103 ) ) ;
#68166=CARTESIAN_POINT ( 'NONE',  ( -23.88501998544221294, 1509.754567424550487, 226.4501273782086059 ) ) ;
#68167=CARTESIAN_POINT ( 'NONE',  ( -4.069498839565195425, 1440.810691400258065, 185.0753115836025984 ) ) ;
#68169=CARTESIAN_POINT ( 'NONE',  ( -18.46438761643240056, 1509.557851011080174, 231.7133587057680018 ) ) ;
#68171=DIRECTION ( 'NONE',  ( -0.7074300732391541890, 0.02470400240461650618, 0.7063514732355541392 ) ) ;
#68175=CARTESIAN_POINT ( 'NONE',  ( 20.84357890140000080, 1509.537325846329850, 188.5527488798980187 ) ) ;
#68177=ORIENTED_EDGE ( 'NONE', *, *, #32170, .T. ) ;
#68178=CARTESIAN_POINT ( 'NONE',  ( -10.78869837093980166, 1414.913060387399810, 195.9645814724970023 ) ) ;
#68188=CARTESIAN_POINT ( 'NONE',  ( 17.61970473800957038, 1423.169058096252002, 226.3196634091193289 ) ) ;
#68191=CARTESIAN_POINT ( 'NONE',  ( -9.740283752330000766, 1438.194204504490017, 148.7998369308980102 ) ) ;
#68192=CARTESIAN_POINT ( 'NONE',  ( 40.87114964212709367, 1440.913060358009943, 260.4862142944329548 ) ) ;
#68194=PLANE ( 'NONE',  #62293 ) ;
#68195=CARTESIAN_POINT ( 'NONE',  ( 11.94272607768921368, 1433.497737235805744, 149.9957492810318627 ) ) ;
#68196=ORIENTED_EDGE ( 'NONE', *, *, #5143, .T. ) ;
#68198=B_SPLINE_CURVE_WITH_KNOTS ( 'NONE', 5,
 ( #80262, #3578, #55079, #12499, #61289, #95405 ),
 .UNSPECIFIED., .F., .F.,
 ( 6, 6 ),
 ( -157.9969979290000026, -29.50720980489998624 ),
 .UNSPECIFIED. ) ;
#68201=CARTESIAN_POINT ( 'NONE',  ( -27.74968902340000199, 1508.601238165030054, 210.5367534243380021 ) ) ;
#68202=CARTESIAN_POINT ( 'NONE',  ( 4.040293861182902013, 1410.430566701483258, 186.0441672988231971 ) ) ;
#68203=CARTESIAN_POINT ( 'NONE',  ( -3.083506393234342724, 1425.993302487229357, 185.5564644828080532 ) ) ;
#68209=CARTESIAN_POINT ( 'NONE',  ( 3.623662524359999804, 1452.348591074630122, 153.7833281135980030 ) ) ;
#68211=FACE_OUTER_BOUND ( 'NONE', #84111, .T. ) ;
#68215=CARTESIAN_POINT ( 'NONE',  ( 19.77866157937050318, 1507.866340390989990, 229.2788407071620043 ) ) ;
#68218=CARTESIAN_POINT ( 'NONE',  ( 19.72812719659350122, 1509.538929610160039, 230.6333991359829838 ) ) ;
#68219=CARTESIAN_POINT ( 'NONE',  ( 1.467768375174040179E-06, 1443.913060387330006, 126.8032257208279958 ) ) ;
#68220=CARTESIAN_POINT ( 'NONE',  ( 37.86301218237910149, 1438.513682760549955, 136.5996409465739987 ) ) ;
#68221=CARTESIAN_POINT ( 'NONE',  ( 18.24515611230000189, 1416.817366564930126, 209.2838582706760064 ) ) ;
#68227=CARTESIAN_POINT ( 'NONE',  ( -12.83843010853493283, 1435.934049928529475, 150.8131814970956270 ) ) ;
#68228=CARTESIAN_POINT ( 'NONE',  ( -18.96814374670399772, 1466.784892475500101, 227.5901968024730024 ) ) ;
#68229=CARTESIAN_POINT ( 'NONE',  ( 3.236814144259999804, 1409.530546742930028, 186.0023276647980026 ) ) ;
#68230=CARTESIAN_POINT ( 'NONE',  ( 4.661455296369999779, 1424.482000793030011, 185.3998824713980014 ) ) ;
#68232=CARTESIAN_POINT ( 'NONE',  ( -3.671612586564420244, 1441.354008908910146, 162.1785783326109822 ) ) ;
#68233=CARTESIAN_POINT ( 'NONE',  ( 11.81421903917279970, 1428.091851616979966, 150.2203617970459959 ) ) ;
#68234=CARTESIAN_POINT ( 'NONE',  ( 0.2305905531100000128, 1465.018788707330032, 237.3910730024980182 ) ) ;
#68235=EDGE_LOOP ( 'NONE', ( #16402, #20240, #88493, #93882 ) ) ;
#68238=CARTESIAN_POINT ( 'NONE',  ( -12.26996133465255845, 1416.831922878780688, 194.6642422945479325 ) ) ;
#68240=CARTESIAN_POINT ( 'NONE',  ( 15.30440149880000078, 1449.517001060780103, 190.0710924244979765 ) ) ;
#68242=CARTESIAN_POINT ( 'NONE',  ( -9.057141760850039745E-09, 1474.953449740560018, 265.2715189222170125 ) ) ;
#68243=EDGE_CURVE ( 'NONE', #102730, #52385, #56973, .T. ) ;
#68244=CARTESIAN_POINT ( 'NONE',  ( -19.98564276653569749, 1487.965312040789968, 190.9658536150159875 ) ) ;
#68246=CARTESIAN_POINT ( 'NONE',  ( -4.398754361689999115, 1417.887151154330013, 234.1121797774980280 ) ) ;
#68252=CARTESIAN_POINT ( 'NONE',  ( -45.84352532457269547, 1439.431483318510118, 266.4135387465440203 ) ) ;
#68261=CARTESIAN_POINT ( 'NONE',  ( -26.44085854399180135, 1451.923913589589802, 135.4526211769480142 ) ) ;
#68264=CARTESIAN_POINT ( 'NONE',  ( 12.80168991080000040, 1420.300675106630024, 231.9932541996980149 ) ) ;
#68267=CARTESIAN_POINT ( 'NONE',  ( -2.919621720534709919, 1419.522956690290130, 186.2043860719099939 ) ) ;
#68270=ADVANCED_FACE ( 'NONE', ( #15826 ), #133, .F. ) ;
#68271=CARTESIAN_POINT ( 'NONE',  ( -23.64739862777970103, 1452.087275030800129, 137.4458378415889968 ) ) ;
#68274=CARTESIAN_POINT ( 'NONE',  ( -1.789119454972039946, 1410.413094933679986, 269.3349920968730089 ) ) ;
#68275=CARTESIAN_POINT ( 'NONE',  ( 4.752796431384060938, 1418.054332079780124, 232.9684996267220072 ) ) ;
#68277=VERTEX_POINT ( 'NONE', #92557 ) ;
#68279=CARTESIAN_POINT ( 'NONE',  ( -23.53967062633439866, 1410.852811126989991, 210.4592016816770013 ) ) ;
#68280=CARTESIAN_POINT ( 'NONE',  ( -0.4537698790271669780, 1408.928907069390107, 186.1253897045490078 ) ) ;
#68281=DIRECTION ( 'NONE',  ( -0.6456859403403140130, -3.014380202827815434E-11, 0.7636030817426319173 ) ) ;
#68282=CARTESIAN_POINT ( 'NONE',  ( -44.72199813584910544, 1433.780093884953658, 266.2156661089638874 ) ) ;
#68283=CARTESIAN_POINT ( 'NONE',  ( -20.93296107774385462, 1436.459762213529984, 144.3971198658650792 ) ) ;
#68285=CARTESIAN_POINT ( 'NONE',  ( 35.63549790119169813, 1463.085316031469802, 266.7196555065800112 ) ) ;
#68289=ADVANCED_FACE ( 'NONE', ( #110474 ), #33752, .F. ) ;
#68290=VERTEX_POINT ( 'NONE', #7460 ) ;
#68291=CARTESIAN_POINT ( 'NONE',  ( 18.75812740016049318, 1458.154557397180952, 227.2553891438375331 ) ) ;
#68295=CARTESIAN_POINT ( 'NONE',  ( 2.664554167959999997, 1448.256636474130119, 183.4094032644979677 ) ) ;
#68296=CARTESIAN_POINT ( 'NONE',  ( 27.01619435114130141, 1451.969645972749959, 135.0017328818020133 ) ) ;
#68301=CARTESIAN_POINT ( 'NONE',  ( 3.780176498421650155, 1409.045067059440044, 187.4689532811570132 ) ) ;
#68302=CARTESIAN_POINT ( 'NONE',  ( 1.116230662139999996, 1415.987376048129818, 233.0984228107980130 ) ) ;
#68303=CARTESIAN_POINT ( 'NONE',  ( -17.93227703497376524, 1423.574558478578865, 225.8942140318575582 ) ) ;
#68304=CARTESIAN_POINT ( 'NONE',  ( 1.420887417485810156, 1452.418213911920247, 183.4780521848920216 ) ) ;
#68305=VECTOR ( 'NONE', #35970, 1000.000000000000000 ) ;
#68309=CARTESIAN_POINT ( 'NONE',  ( 11.74757148146339958, 1414.971390223319986, 220.9933141604269906 ) ) ;
#68311=CARTESIAN_POINT ( 'NONE',  ( 19.02704169900689735, 1456.915441405320053, 225.6706379604710264 ) ) ;
#68314=CARTESIAN_POINT ( 'NONE',  ( -35.24640315935789658, 1450.253616403709884, 136.2305448810739961 ) ) ;
#68317=CARTESIAN_POINT ( 'NONE',  ( -36.06124927489999976, 1440.913060387330006, 262.6648722463980334 ) ) ;
#68318=CARTESIAN_POINT ( 'NONE',  ( -21.46972948204773601, 1509.114287412469821, 191.7923745190988711 ) ) ;
#68319=CARTESIAN_POINT ( 'NONE',  ( 11.91481860790000091, 1433.381974997530051, 150.0448548111979790 ) ) ;
#68320=CARTESIAN_POINT ( 'NONE',  ( 6.509745749769999534, 1455.357238104129920, 219.6133833021979740 ) ) ;
#68321=CARTESIAN_POINT ( 'NONE',  ( 12.74111629471100038, 1416.830086716310007, 196.2606222955850228 ) ) ;
#68324=CARTESIAN_POINT ( 'NONE',  ( 9.726491193908251375E-12, 1408.913060387299993, 194.1220083575990145 ) ) ;
#68325=CARTESIAN_POINT ( 'NONE',  ( -19.58697162420000382, 1486.201721251429944, 189.8983747997980061 ) ) ;
#68326=CARTESIAN_POINT ( 'NONE',  ( 12.60638609191129156, 1398.286777232254053, 205.9470198407383066 ) ) ;
#68327=CARTESIAN_POINT ( 'NONE',  ( -28.21231394539000092, 1509.976025385810090, 222.5052518413109794 ) ) ;
#68329=CARTESIAN_POINT ( 'NONE',  ( 20.32611051209999786, 1410.902622695729860, 219.5117589930979989 ) ) ;
#68330=DIRECTION ( 'NONE',  ( -1.987897879952545076E-13, 0.000000000000000000, 1.000000000000000000 ) ) ;
#68331=FACE_OUTER_BOUND ( 'NONE', #81050, .T. ) ;
#68337=VECTOR ( 'NONE', #53509, 1000.000000000000000 ) ;
#68338=CARTESIAN_POINT ( 'NONE',  ( 0.1964394189208260033, 1465.025380390069813, 182.7374004966019925 ) ) ;
#68339=CARTESIAN_POINT ( 'NONE',  ( 4.821407917150390210E-08, 1406.911841293459929, 222.1218459631980124 ) ) ;
#68340=VERTEX_POINT ( 'NONE', #102057 ) ;
#68343=CARTESIAN_POINT ( 'NONE',  ( 11.87509769129999881, 1433.007199317849881, 149.6991846015980059 ) ) ;
#68344=CARTESIAN_POINT ( 'NONE',  ( -39.19204896935080029, 1449.501219045460175, 134.0999999980739688 ) ) ;
#68345=CARTESIAN_POINT ( 'NONE',  ( -37.66849514949689848, 1445.052233488579986, 137.0436250779820000 ) ) ;
#68346=ORIENTED_EDGE ( 'NONE', *, *, #38464, .T. ) ;
#68349=CARTESIAN_POINT ( 'NONE',  ( -16.17135632760000163, 1414.913060387329779, 211.6988393313379788 ) ) ;
#68352=CARTESIAN_POINT ( 'NONE',  ( -15.05526703829680102, 1490.297662996039890, 193.6804093798809845 ) ) ;
#68353=CARTESIAN_POINT ( 'NONE',  ( 21.35837619879999849, 1471.309462468929951, 210.2388403116680138 ) ) ;
#68354=CARTESIAN_POINT ( 'NONE',  ( 8.735814283539220071, 1409.218121743860138, 221.2697303220529932 ) ) ;
#68357=CARTESIAN_POINT ( 'NONE',  ( 12.61823209568870041, 1416.826860677879949, 196.1892328963569980 ) ) ;
#68360=CARTESIAN_POINT ( 'NONE',  ( -32.69005633750000328, 1450.911397438570020, 136.2076752502979673 ) ) ;
#68361=CARTESIAN_POINT ( 'NONE',  ( 16.68533971102617741, 1442.773887286371291, 162.0931267225411148 ) ) ;
#68363=EDGE_LOOP ( 'NONE', ( #54380, #88947, #56659, #10079 ) ) ;
#68365=CARTESIAN_POINT ( 'NONE',  ( 25.31820978150000201, 1509.573487416829948, 221.0603481741979692 ) ) ;
#68368=CARTESIAN_POINT ( 'NONE',  ( -4.652381700140650445, 1440.963318135419968, 155.5568945814929975 ) ) ;
#68370=FACE_OUTER_BOUND ( 'NONE', #87594, .T. ) ;
#68377=CARTESIAN_POINT ( 'NONE',  ( 2.500000000000000000, 1448.346004463229974, 162.8188077318980334 ) ) ;
#68379=CARTESIAN_POINT ( 'NONE',  ( 45.63713230869999649, 1440.913060384009896, 268.9747493906979798 ) ) ;
#68381=ORIENTED_EDGE ( 'NONE', *, *, #32172, .F. ) ;
#68383=ORIENTED_EDGE ( 'NONE', *, *, #72916, .T. ) ;
#68386=CARTESIAN_POINT ( 'NONE',  ( -24.93139309809999915, 1449.798359909379997, 205.3225103653480232 ) ) ;
#68387=CARTESIAN_POINT ( 'NONE',  ( -11.37160906494359836, 1425.522438667359893, 139.7055457720969969 ) ) ;
#68388=CARTESIAN_POINT ( 'NONE',  ( 16.11681422559630050, 1409.475865535250250, 193.1327842899079883 ) ) ;
#68390=( BOUNDED_CURVE ( )  B_SPLINE_CURVE ( 3, ( #74935, #83859, #23934, #22828 ),
 .UNSPECIFIED., .F., .F. ) 
 B_SPLINE_CURVE_WITH_KNOTS ( ( 4, 4 ),
 ( 1.036132084875134307, 2.105460515756535145 ),
 .UNSPECIFIED. ) 
 CURVE ( )  GEOMETRIC_REPRESENTATION_ITEM ( )  RATIONAL_B_SPLINE_CURVE ( ( 1.000000000000000000, 0.9069598516813908162, 0.9069598516813908162, 1.000000000000000000 ) ) 
 REPRESENTATION_ITEM ( '' )  );
#68391=CARTESIAN_POINT ( 'NONE',  ( 27.67506469288673898, 1509.991447327714695, 220.7024101144958763 ) ) ;
#68392=CARTESIAN_POINT ( 'NONE',  ( 1.546867617820790075, 1416.839692126689897, 190.2222510973109877 ) ) ;
#68393=CARTESIAN_POINT ( 'NONE',  ( 2.299422874330000137E-10, 1405.830933579830116, 267.2558761554980151 ) ) ;
#68395=CARTESIAN_POINT ( 'NONE',  ( 28.29378357456099735, 1508.482245359879926, 209.4043078930619970 ) ) ;
#68399=CARTESIAN_POINT ( 'NONE',  ( -38.43658860624190510, 1439.043532485229889, 136.6419780607560028 ) ) ;
#68401=CARTESIAN_POINT ( 'NONE',  ( 12.64817333528600152, 1398.288027439289863, 213.9887766886679970 ) ) ;
#68403=CARTESIAN_POINT ( 'NONE',  ( -18.34469986919999940, 1457.405375599930039, 229.1958636041979958 ) ) ;
#68406=CARTESIAN_POINT ( 'NONE',  ( 11.60004869885204570, 1426.273943615695998, 138.2686089212693332 ) ) ;
#68408=CARTESIAN_POINT ( 'NONE',  ( -0.5000000000000000000, 1448.894380913990062, 169.5117309619979835 ) ) ;
#68413=CARTESIAN_POINT ( 'NONE',  ( -4.338666831039999394, 1461.192105632430184, 234.4075396365979884 ) ) ;
#68421=ORIENTED_EDGE ( 'NONE', *, *, #39908, .F. ) ;
#68422=CARTESIAN_POINT ( 'NONE',  ( 11.77484973565070092, 1427.254610112360069, 146.7344958145999954 ) ) ;
#68423=CARTESIAN_POINT ( 'NONE',  ( 20.60026074440000343, 1507.873289787829890, 228.0392264067980364 ) ) ;
#68424=VERTEX_POINT ( 'NONE', #96443 ) ;
#68425=CARTESIAN_POINT ( 'NONE',  ( -13.22475641109999955, 1415.063410489829948, 220.7066272063979966 ) ) ;
#68426=CARTESIAN_POINT ( 'NONE',  ( -11.77504666877200101, 1432.336839525429923, 150.6178357199280242 ) ) ;
#68429=CARTESIAN_POINT ( 'NONE',  ( -4.556667256680000833, 1420.452533403130019, 186.4400355392980089 ) ) ;
#68434=CARTESIAN_POINT ( 'NONE',  ( -14.87670423429999822, 1451.329521634429966, 222.9740515411980084 ) ) ;
#68435=CARTESIAN_POINT ( 'NONE',  ( 18.22804834760000148, 1459.311383086529759, 227.8763781793979888 ) ) ;
#68437=CARTESIAN_POINT ( 'NONE',  ( -4.881429273560958570, 1423.432558903203699, 184.6511038030233465 ) ) ;
#68438=CARTESIAN_POINT ( 'NONE',  ( -2.499957339842320270, 1419.383212207730139, 144.0944162744979735 ) ) ;
#68439=VERTEX_POINT ( 'NONE', #3508 ) ;
#68440=CARTESIAN_POINT ( 'NONE',  ( 18.02920443208860135, 1424.486262421390165, 224.5040309780439998 ) ) ;
#68442=CARTESIAN_POINT ( 'NONE',  ( -2.899297689372634323, 1484.395568125579302, 183.3060837819314202 ) ) ;
#68446=CARTESIAN_POINT ( 'NONE',  ( 1.115901143310000121, 1489.466917449630046, 186.9663283330980050 ) ) ;
#68447=CARTESIAN_POINT ( 'NONE',  ( -12.26979726809049964, 1416.828039266780024, 194.6643405733680083 ) ) ;
#68448=CARTESIAN_POINT ( 'NONE',  ( -10.82836173039999927, 1424.910041191229993, 145.2218151137980158 ) ) ;
#68449=CARTESIAN_POINT ( 'NONE',  ( -10.86693375039079079, 1425.933726053461669, 148.0815712597264735 ) ) ;
#68451=DIRECTION ( 'NONE',  ( 1.225338022780404242E-19, -0.5877852522921362954, 0.8090169943751921444 ) ) ;
#68454=CARTESIAN_POINT ( 'NONE',  ( 11.61695163049999913, 1410.397346041930177, 229.1624418486979948 ) ) ;
#68455=CARTESIAN_POINT ( 'NONE',  ( -19.72763672960000036, 1470.089429620230021, 226.7169729388979817 ) ) ;
#68458=VERTEX_POINT ( 'NONE', #88058 ) ;
#68460=CARTESIAN_POINT ( 'NONE',  ( 23.72341811100000086, 1410.667716130429881, 268.2433620527979770 ) ) ;
#68462=CARTESIAN_POINT ( 'NONE',  ( 17.38485634039999894, 1410.884445771429910, 192.4603913046979926 ) ) ;
#68463=CARTESIAN_POINT ( 'NONE',  ( 2.161903390967117922, 1506.361658163160655, 231.0098389382108337 ) ) ;
#68464=EDGE_CURVE ( 'NONE', #81952, #109869, #7365, .T. ) ;
#68469=CARTESIAN_POINT ( 'NONE',  ( -13.84069052210000095, 1443.989035751789970, 188.2135015426979976 ) ) ;
#68472=EDGE_CURVE ( 'NONE', #75409, #48999, #94219, .T. ) ;
#68474=CARTESIAN_POINT ( 'NONE',  ( 41.65085711740252350, 1427.189773105231097, 269.7492452597979877 ) ) ;
#68475=ORIENTED_EDGE ( 'NONE', *, *, #85308, .F. ) ;
#68476=CARTESIAN_POINT ( 'NONE',  ( 1.457290784524640115, 1498.568683518979924, 181.4860206734340125 ) ) ;
#68477=CARTESIAN_POINT ( 'NONE',  ( -14.62787175408529983, 1409.423876925000059, 206.1255987914319974 ) ) ;
#68480=CARTESIAN_POINT ( 'NONE',  ( -12.70598598470000162, 1474.665014927529910, 267.1690917002979972 ) ) ;
#68481=DIRECTION ( 'NONE',  ( 0.09872124640252573358, 0.9946467452574913048, -0.03052814533198805816 ) ) ;
#68483=CARTESIAN_POINT ( 'NONE',  ( -24.07284968513953061, 1444.387198279564927, 212.0163994439685951 ) ) ;
#68485=CARTESIAN_POINT ( 'NONE',  ( 13.58245575526007443, 1416.835806643160140, 196.3346083899895120 ) ) ;
#68486=CARTESIAN_POINT ( 'NONE',  ( -1.887379141860000372E-15, 1438.194204504490017, 155.6035180864980134 ) ) ;
#68487=CARTESIAN_POINT ( 'NONE',  ( -24.08134052106170131, 1444.794274679859882, 211.7743307240010040 ) ) ;
#68490=CARTESIAN_POINT ( 'NONE',  ( -22.32273759649999789, 1409.692587561330129, 207.4115339668879869 ) ) ;
#68491=EDGE_CURVE ( 'NONE', #108306, #80118, #44599, .T. ) ;
#68492=CARTESIAN_POINT ( 'NONE',  ( 17.36177572460000107, 1416.518532928429977, 203.7896239905979883 ) ) ;
#68493=B_SPLINE_CURVE_WITH_KNOTS ( 'NONE', 3,
 ( #22401, #47648, #81777, #73955 ),
 .UNSPECIFIED., .F., .F.,
 ( 4, 4 ),
 ( 0.000000000000000000, 1.000000000000000000 ),
 .UNSPECIFIED. ) ;
#68496=DIRECTION ( 'NONE',  ( 0.04361938736533144123, 0.9990482215818579093, 0.000000000000000000 ) ) ;
#68501=CARTESIAN_POINT ( 'NONE',  ( -21.56891622590000068, 1409.666263542329943, 211.8934861044880051 ) ) ;
#68503=CARTESIAN_POINT ( 'NONE',  ( 11.72712749186690040, 1426.702236078659780, 143.4605025666630240 ) ) ;
#68507=CARTESIAN_POINT ( 'NONE',  ( -16.42420382550000113, 1507.212883782629888, 224.6993357452979865 ) ) ;
#68509=B_SPLINE_CURVE_WITH_KNOTS ( 'NONE', 5,
 ( #83279, #6577, #100617, #40726, #74899, #109049 ),
 .UNSPECIFIED., .F., .F.,
 ( 6, 6 ),
 ( -168.5477119569999900, -31.28316115780000928 ),
 .UNSPECIFIED. ) ;
#68510=CARTESIAN_POINT ( 'NONE',  ( -4.536954624239665890, 1398.048335974680867, 221.3051406648845045 ) ) ;
#68511=CARTESIAN_POINT ( 'NONE',  ( -3.607350949321984412, 1440.817088961761328, 156.6135841830677293 ) ) ;
#68513=CARTESIAN_POINT ( 'NONE',  ( -18.60709431639999778, 1430.292579561230013, 194.6369243821980035 ) ) ;
#68516=ORIENTED_EDGE ( 'NONE', *, *, #104508, .T. ) ;
#68518=CARTESIAN_POINT ( 'NONE',  ( 11.86099846289999959, 1433.814634837920039, 150.7353243123980064 ) ) ;
#68521=CARTESIAN_POINT ( 'NONE',  ( -0.0002529968379770906732, 1396.150242178169037, 221.0765849288899574 ) ) ;
#68522=CARTESIAN_POINT ( 'NONE',  ( -21.04382066049999978, 1508.388118462830107, 192.1514652868980022 ) ) ;
#68524=CARTESIAN_POINT ( 'NONE',  ( 17.36735080831220301, 1468.293338259049960, 189.7435350345869836 ) ) ;
#68525=CARTESIAN_POINT ( 'NONE',  ( 0.5620975284970839425, 1416.851343896850040, 190.4751211475700075 ) ) ;
#68526=CARTESIAN_POINT ( 'NONE',  ( 16.39757969585189912, 1498.110351991700099, 231.0166114906680264 ) ) ;
#68527=CARTESIAN_POINT ( 'NONE',  ( 0.02470720775370000011, 1488.177913144229933, 181.6829962196979977 ) ) ;
#68528=CARTESIAN_POINT ( 'NONE',  ( -5.335636987560000044, 1416.823418193329871, 191.7467471926979954 ) ) ;
#68529=CARTESIAN_POINT ( 'NONE',  ( -24.24870063226580186, 1444.787720494630094, 211.3850291965160011 ) ) ;
#68534=CARTESIAN_POINT ( 'NONE',  ( 14.31665923840910004, 1416.051481378869994, 196.9967738469869971 ) ) ;
#68535=CARTESIAN_POINT ( 'NONE',  ( 11.85510997289999935, 1431.526737989079948, 150.3422258050980247 ) ) ;
#68538=CARTESIAN_POINT ( 'NONE',  ( 13.90979721639719990, 1435.199138253310139, 149.4519102904939984 ) ) ;
#68539=ORIENTED_EDGE ( 'NONE', *, *, #96912, .T. ) ;
#68540=ORIENTED_EDGE ( 'NONE', *, *, #68491, .F. ) ;
#68541=CARTESIAN_POINT ( 'NONE',  ( 13.43766692883458269, 1444.332322004376692, 169.3644260008774438 ) ) ;
#68542=CARTESIAN_POINT ( 'NONE',  ( -4.363122647530000009, 1417.926080483629903, 166.9581667359979917 ) ) ;
#68543=CARTESIAN_POINT ( 'NONE',  ( -2.814434489400770012, 1407.025243844600027, 222.1218459754350363 ) ) ;
#68552=CARTESIAN_POINT ( 'NONE',  ( 20.08821595115609782, 1440.913060387330006, 216.9936666811269959 ) ) ;
#68554=EDGE_LOOP ( 'NONE', ( #83506, #27340, #3620, #80024 ) ) ;
#68555=CARTESIAN_POINT ( 'NONE',  ( -4.323257523719999718, 1409.231785804929814, 187.3862315473980118 ) ) ;
#68560=CARTESIAN_POINT ( 'NONE',  ( 21.56408335959999789, 1429.453335383130025, 218.9472881200579764 ) ) ;
#68562=DIRECTION ( 'NONE',  ( 0.6831251091958939758, -0.2299220283779639940, -0.6931637224008919684 ) ) ;
#68563=CARTESIAN_POINT ( 'NONE',  ( 0.003579571106766400116, 1467.142144048650152, 235.6416276143629887 ) ) ;
#68566=EDGE_CURVE ( 'NONE', #44537, #80100, #49949, .T. ) ;
#68569=CARTESIAN_POINT ( 'NONE',  ( -20.58126087740000187, 1507.779106712530165, 190.0921675882979969 ) ) ;
#68572=CARTESIAN_POINT ( 'NONE',  ( 14.24543712669999884, 1409.914297001830164, 191.5991055419980000 ) ) ;
#68576=CARTESIAN_POINT ( 'NONE',  ( 39.40334551520000161, 1445.870380880999846, 259.1105671997980266 ) ) ;
#68577=CARTESIAN_POINT ( 'NONE',  ( 2.611439748538543437, 1452.027163526197228, 183.7718830791166340 ) ) ;
#68579=CARTESIAN_POINT ( 'NONE',  ( -1.673272949882680161, 1509.003834942280037, 238.7500911974470057 ) ) ;
#68580=CARTESIAN_POINT ( 'NONE',  ( -24.09814616339999915, 1444.255785636859855, 212.5772553282479862 ) ) ;
#68582=CARTESIAN_POINT ( 'NONE',  ( 17.00957473938450093, 1409.517103885259985, 222.2161159761519968 ) ) ;
#68587=EDGE_CURVE ( 'NONE', #19422, #89981, #52018, .T. ) ;
#68588=CARTESIAN_POINT ( 'NONE',  ( 0.2151019729850000006, 1406.066550330029941, 269.0456880831980016 ) ) ;
#68589=CARTESIAN_POINT ( 'NONE',  ( 28.20849540440000069, 1509.668627050129771, 207.1396464727879732 ) ) ;
#68590=ADVANCED_FACE ( 'NONE', ( #38721 ), #72358, .F. ) ;
#68591=CARTESIAN_POINT ( 'NONE',  ( 24.65284882109999742, 1440.998884811290054, 212.5088486048679783 ) ) ;
#68596=CARTESIAN_POINT ( 'NONE',  ( 33.27875429775290428, 1435.659579155510073, 135.0862773368370142 ) ) ;
#68598=CARTESIAN_POINT ( 'NONE',  ( -12.78743204916831822, 1416.839570625586930, 195.1659244036679866 ) ) ;
#68600=CARTESIAN_POINT ( 'NONE',  ( 10.16713191040000019, 1507.687633808930059, 183.8172474484979944 ) ) ;
#68604=EDGE_LOOP ( 'NONE', ( #56555, #107627, #83220, #29832 ) ) ;
#68605=CARTESIAN_POINT ( 'NONE',  ( 1.613214857710000061, 1426.534415841129885, 146.0564723340980038 ) ) ;
#68606=CARTESIAN_POINT ( 'NONE',  ( -33.91369269983620427, 1450.440666099120108, 136.2454419983430114 ) ) ;
#68607=AXIS2_PLACEMENT_3D ( 'NONE', #32011, #108721, #5724 ) ;
#68608=ADVANCED_FACE ( 'NONE', ( #72896 ), #110720, .T. ) ;
#68610=SPHERICAL_SURFACE ( 'NONE', #41979, 2.000000000000000000 ) ;
#68611=CARTESIAN_POINT ( 'NONE',  ( -0.7176848839889999887, 1417.283279384530033, 235.8571367780980097 ) ) ;
#68614=CARTESIAN_POINT ( 'NONE',  ( 25.25200551730000242, 1450.804230319249882, 137.6134878989979882 ) ) ;
#68619=CARTESIAN_POINT ( 'NONE',  ( 42.54897258395909176, 1440.913021756910211, 270.0691962208189807 ) ) ;
#68620=CARTESIAN_POINT ( 'NONE',  ( -14.87261298220626848, 1451.156254727674877, 149.8042946858963944 ) ) ;
#68622=CARTESIAN_POINT ( 'NONE',  ( 25.82385068980000042, 1436.204139849239937, 136.8568693873980067 ) ) ;
#68623=CARTESIAN_POINT ( 'NONE',  ( -10.96840289711549943, 1396.296085456599940, 207.6085868023199907 ) ) ;
#68626=CARTESIAN_POINT ( 'NONE',  ( -16.99375006173600156, 1409.880053590220086, 225.6062263545040025 ) ) ;
#68630=CARTESIAN_POINT ( 'NONE',  ( 9.921670129709269759, 1445.422324508452675, 184.5085384531410568 ) ) ;
#68633=CARTESIAN_POINT ( 'NONE',  ( 10.68580243010000075, 1425.706269979529907, 93.45797665869790194 ) ) ;
#68635=CARTESIAN_POINT ( 'NONE',  ( 23.82311388440000144, 1410.240487848430121, 209.8684836133409704 ) ) ;
#68637=CARTESIAN_POINT ( 'NONE',  ( 4.181971434956770040, 1424.905875537870088, 185.1749942703449960 ) ) ;
#68638=CARTESIAN_POINT ( 'NONE',  ( -2.500591765228052044, 1421.109708633257696, 185.0623077226939017 ) ) ;
#68641=CARTESIAN_POINT ( 'NONE',  ( 8.365522723199999788, 1508.201466091430120, 182.8802321776979909 ) ) ;
#68642=CARTESIAN_POINT ( 'NONE',  ( 3.920714864009999356, 1449.393300602180261, 184.2471769888979907 ) ) ;
#68643=EDGE_CURVE ( 'NONE', #59669, #29227, #68875, .T. ) ;
#68650=CARTESIAN_POINT ( 'NONE',  ( -0.9453320770299999953, 1471.431441225329991, 269.3347421566979847 ) ) ;
#68651=CARTESIAN_POINT ( 'NONE',  ( 13.68849417913788535, 1434.975516646386268, 146.5173254893715011 ) ) ;
#68653=CARTESIAN_POINT ( 'NONE',  ( 15.98141629860000101, 1475.513060387329915, 194.5230232035980293 ) ) ;
#68657=CARTESIAN_POINT ( 'NONE',  ( -19.81155763900000011, 1453.313060387329870, 204.5601901296680012 ) ) ;
#68659=CARTESIAN_POINT ( 'NONE',  ( -0.05087731996257439937, 1408.368774903450003, 195.5796676407180144 ) ) ;
#68660=CARTESIAN_POINT ( 'NONE',  ( -24.08411849022170159, 1411.068933507980091, 268.8151254836839712 ) ) ;
#68661=CARTESIAN_POINT ( 'NONE',  ( -14.24203721301430114, 1435.591090021740001, 149.7553460124620131 ) ) ;
#68664=CARTESIAN_POINT ( 'NONE',  ( 14.09542765070000137, 1445.387346742360023, 189.3996806953979899 ) ) ;
#68671=CARTESIAN_POINT ( 'NONE',  ( -17.32570511339999797, 1470.470731013029990, 189.1993959853980130 ) ) ;
#68673=VERTEX_POINT ( 'NONE', #59965 ) ;
#68676=CARTESIAN_POINT ( 'NONE',  ( -5.359822931069220253, 1422.298725726440125, 145.8185784961330000 ) ) ;
#68678=CARTESIAN_POINT ( 'NONE',  ( -29.68011195740000119, 1509.981398976430228, 207.8176008383179862 ) ) ;
#68680=CARTESIAN_POINT ( 'NONE',  ( -7.478246699966769384, 1428.083861423860071, 222.0822691923259811 ) ) ;
#68682=CARTESIAN_POINT ( 'NONE',  ( -10.44739388110000000, 1446.724320542959958, 186.7828859559980117 ) ) ;
#68683=EDGE_LOOP ( 'NONE', ( #22136, #3526, #97432, #19501 ) ) ;
#68684=CARTESIAN_POINT ( 'NONE',  ( -24.91361132602320083, 1430.502641201929919, 208.6735168275199612 ) ) ;
#68685=CARTESIAN_POINT ( 'NONE',  ( 27.16947874219999903, 1488.689296588730031, 210.7748653152779923 ) ) ;
#68687=CARTESIAN_POINT ( 'NONE',  ( 19.34098968424050113, 1467.084471247349938, 225.9997439510970025 ) ) ;
#68688=EDGE_CURVE ( 'NONE', #96843, #101763, #66422, .T. ) ;
#68689=CARTESIAN_POINT ( 'NONE',  ( -24.25710768520000116, 1435.418799296620136, 137.1797428065980000 ) ) ;
#68693=CARTESIAN_POINT ( 'NONE',  ( -14.87415096680000026, 1413.165999674329896, 226.7982133869979862 ) ) ;
#68695=( BOUNDED_CURVE ( )  B_SPLINE_CURVE ( 3, ( #34991, #22845, #68076, #59116 ),
 .UNSPECIFIED., .F., .F. ) 
 B_SPLINE_CURVE_WITH_KNOTS ( ( 4, 4 ),
 ( 2.183705749549460062, 2.832670179246489894 ),
 .UNSPECIFIED. ) 
 CURVE ( )  GEOMETRIC_REPRESENTATION_ITEM ( )  RATIONAL_B_SPLINE_CURVE ( ( 1.000000000000000000, 0.9652106218148086558, 0.9652106218148086558, 1.000000000000000000 ) ) 
 REPRESENTATION_ITEM ( '' )  );
#68698=CARTESIAN_POINT ( 'NONE',  ( -1.948088825686169923, 1451.942038968990119, 184.3567259028899912 ) ) ;
#68699=CARTESIAN_POINT ( 'NONE',  ( -0.8591407147159999536, 1410.309640657729915, 233.0900045620979881 ) ) ;
#68702=B_SPLINE_CURVE_WITH_KNOTS ( 'NONE', 5,
 ( #29576, #98434, #63232, #14417, #48047, #12225 ),
 .UNSPECIFIED., .F., .F.,
 ( 6, 6 ),
 ( 0.000000000000000000, 1.000000000000000000 ),
 .UNSPECIFIED. ) ;
#68706=CARTESIAN_POINT ( 'NONE',  ( 12.22857413548589989, 1435.233796397459855, 150.9813450485239912 ) ) ;
#68707=B_SPLINE_SURFACE_WITH_KNOTS ( 'NONE', 5, 4, ( 
 ( #15630, #73379, #56578, #108061, #58234 ),
 ( #83413, #5620, #107517, #99100, #91813 ),
 ( #75597, #47624, #100751, #7266, #14551 ),
 ( #6708, #64984, #98560, #92358, #90711 ),
 ( #13997, #48182, #82321, #39771, #48739 ),
 ( #73931, #82864, #6156, #66099, #49284 ) ),
 .UNSPECIFIED., .F., .F., .F.,
 ( 6, 6 ),
 ( 5, 5 ),
 ( 0.000000000000000000, 11.48858425020000062 ),
 ( 40.20365518519999881, 50.26548245740000453 ),
 .UNSPECIFIED. ) ;
#68708=CARTESIAN_POINT ( 'NONE',  ( -4.071675667009562183, 1441.007006124126065, 184.9002666288488683 ) ) ;
#68709=CARTESIAN_POINT ( 'NONE',  ( -22.71192893796499845, 1509.726026642720171, 228.1488050769010272 ) ) ;
#68711=CARTESIAN_POINT ( 'NONE',  ( -1.443308691599999971, 1409.130619234930009, 186.4549414153979683 ) ) ;
#68713=CARTESIAN_POINT ( 'NONE',  ( 4.238435005652729792, 1441.459264359959889, 163.1404339353370005 ) ) ;
#68715=CARTESIAN_POINT ( 'NONE',  ( -2.473077522879999712, 1421.063464807129776, 185.4030335298980106 ) ) ;
#68716=CARTESIAN_POINT ( 'NONE',  ( 19.94169889329999990, 1509.369061810729818, 188.0276712769979781 ) ) ;
#68719=CARTESIAN_POINT ( 'NONE',  ( -12.26996141999999956, 1416.831925117829996, 194.6642422325980135 ) ) ;
#68724=CARTESIAN_POINT ( 'NONE',  ( 4.209031986870000352, 1421.916286088630159, 184.3722574647979968 ) ) ;
#68730=CARTESIAN_POINT ( 'NONE',  ( 17.36591816528652643, 1422.683100631737943, 226.5834436581721434 ) ) ;
#68734=CARTESIAN_POINT ( 'NONE',  ( 7.105427357599999217E-15, 1410.913060387329779, 137.0999999980979851 ) ) ;
#68735=CARTESIAN_POINT ( 'NONE',  ( 43.69322311477699827, 1440.913060359309839, 264.0012025825540150 ) ) ;
#68738=CARTESIAN_POINT ( 'NONE',  ( 11.39042046171206835, 1433.915048304869288, 151.4356557148368552 ) ) ;
#68740=CARTESIAN_POINT ( 'NONE',  ( 1.553898488376879827, 1415.492117401580117, 190.8404010663989823 ) ) ;
#68741=CARTESIAN_POINT ( 'NONE',  ( 22.53878404599999641, 1411.058442739730026, 206.1986151668880041 ) ) ;
#68742=EDGE_CURVE ( 'NONE', #52693, #67085, #44172, .T. ) ;
#68743=B_SPLINE_CURVE_WITH_KNOTS ( 'NONE', 3,
 ( #65839, #84270, #32219, #14850, #24353, #51225, #40617, #93750, #41720, #32763, #59639, #110578, #74788, #99957, #108930, #74246, #8107, #50675, #75880, #23798, #110028, #6467, #42274, #33304, #57989, #93219, #101055, #24888, #31659, #23251, #84808, #15399, #49041, #83177, #67499, #7015, #41172, #66946, #101603, #92665, #59095, #36637, #102701, #1383, #52902, #52358, #88155, #104388, #54027, #9233, #19252, #10891, #844, #43390, #70833, #27137, #297, #78640, #2513, #94312, #10321, #42830, #17591, #44495, #18161, #34969, #76991, #34424, #53458, #69151, #86475, #36093, #27685, #70279, #61323, #1955 ),
 .UNSPECIFIED., .F., .F.,
 ( 4, 3, 3, 3, 3, 3, 3, 3, 3, 3, 3, 3, 3, 3, 3, 3, 3, 3, 3, 3, 3, 3, 3, 3, 3, 4 ),
 ( -32.41280709890000367, -32.04800627787870582, -31.23028833932220039, -30.40294656779999727, -29.97571463615929943, -29.17405848693029924, -28.39797230597359956, -27.64057875201519821, -26.91504384857509891, -26.20815561766710289, -25.51808413167499978, -24.82024664080000065, -24.40663526596280164, -23.87734799550889875, -23.33898530432950125, -22.80091041601890112, -22.27434435385609746, -21.75967651710000084, -21.56181898327110247, -21.07938793902939878, -20.58798065129229826, -20.09329540484139898, -19.59996587401529666, -19.11219011100000031, -18.70494888627219865, -18.22829625880000037 ),
 .UNSPECIFIED. ) ;
#68744=CARTESIAN_POINT ( 'NONE',  ( -27.74496046000000149, 1507.996570526829828, 210.5130752751180125 ) ) ;
#68745=CARTESIAN_POINT ( 'NONE',  ( 2.640159921366920681, 1410.383150405935567, 185.6143680615537335 ) ) ;
#68748=CARTESIAN_POINT ( 'NONE',  ( 6.232532001850000114, 1407.162969929529936, 220.5304192662980256 ) ) ;
#68753=CARTESIAN_POINT ( 'NONE',  ( -0.004285587994040000043, 1452.913210043629988, 152.9532950659979917 ) ) ;
#68754=CARTESIAN_POINT ( 'NONE',  ( -28.77730029287999969, 1509.917985857419808, 212.2396942430650029 ) ) ;
#68758=CARTESIAN_POINT ( 'NONE',  ( -18.41476513140925064, 1458.949142990964219, 227.7116331479677740 ) ) ;
#68760=CARTESIAN_POINT ( 'NONE',  ( -16.81208394469999945, 1409.500151295429987, 223.9875056278980026 ) ) ;
#68762=ORIENTED_EDGE ( 'NONE', *, *, #108978, .T. ) ;
#68763=CARTESIAN_POINT ( 'NONE',  ( 19.26614117215169841, 1508.824729876830133, 229.9165145868500133 ) ) ;
#68766=CARTESIAN_POINT ( 'NONE',  ( 39.65501738910209895, 1440.824868566870009, 136.8092738732900102 ) ) ;
#68768=CARTESIAN_POINT ( 'NONE',  ( -43.15848718719999511, 1446.267105529279888, 263.9122466480980620 ) ) ;
#68773=CARTESIAN_POINT ( 'NONE',  ( -12.71745976146490342, 1435.880823605873275, 150.8653729509765355 ) ) ;
#68774=CARTESIAN_POINT ( 'NONE',  ( -20.93293658309999827, 1485.999516591429938, 191.6309104264979908 ) ) ;
#68775=CARTESIAN_POINT ( 'NONE',  ( 1.629670625839999998, 1408.969969738429882, 186.3700264965980011 ) ) ;
#68777=CARTESIAN_POINT ( 'NONE',  ( -8.002862407569999448, 1439.449515582499998, 153.7646872161979843 ) ) ;
#68778=EDGE_CURVE ( 'NONE', #1325, #12333, #24840, .T. ) ;
#68779=CARTESIAN_POINT ( 'NONE',  ( 12.84239758539999876, 1435.935717715699866, 150.8114787689980005 ) ) ;
#68782=FACE_OUTER_BOUND ( 'NONE', #58512, .T. ) ;
#68783=CARTESIAN_POINT ( 'NONE',  ( 2.004165785690000146, 1464.806852714229990, 237.1135893016980276 ) ) ;
#68786=CARTESIAN_POINT ( 'NONE',  ( -37.16667942899999844, 1455.848356743629893, 269.8045258284980150 ) ) ;
#68787=CARTESIAN_POINT ( 'NONE',  ( -26.92291386341319992, 1446.493256825939852, 137.3410762857710097 ) ) ;
#68790=CARTESIAN_POINT ( 'NONE',  ( -7.626016305360259571E-09, 1472.553150102269910, 260.2551601210919898 ) ) ;
#68792=CARTESIAN_POINT ( 'NONE',  ( -0.9088213736110000163, 1416.535385209229844, 228.0150015372980192 ) ) ;
#68793=CARTESIAN_POINT ( 'NONE',  ( -9.980081002260000389, 1419.601693820030050, 231.3438068025980101 ) ) ;
#68796=CARTESIAN_POINT ( 'NONE',  ( -0.2368219676957374342, 1485.961491073400111, 181.8351824008125561 ) ) ;
#68798=CARTESIAN_POINT ( 'NONE',  ( -46.11102460466209862, 1439.417470722359894, 268.2058513100960226 ) ) ;
#68799=CARTESIAN_POINT ( 'NONE',  ( -3.600923890900000313, 1431.488321968289938, 185.7685271587979798 ) ) ;
#68801=ORIENTED_EDGE ( 'NONE', *, *, #6539, .T. ) ;
#68804=CARTESIAN_POINT ( 'NONE',  ( -26.07583950859109834, 1441.264734016169996, 138.1452376982360022 ) ) ;
#68806=CARTESIAN_POINT ( 'NONE',  ( -26.81127850451720107, 1451.960562951069960, 135.1661831948950123 ) ) ;
#68808=CARTESIAN_POINT ( 'NONE',  ( -15.59201085679999998, 1506.806593688130079, 193.4620896933980134 ) ) ;
#68810=CARTESIAN_POINT ( 'NONE',  ( 15.65975626840000068, 1506.806593688130079, 193.5298351049979999 ) ) ;
#68813=CARTESIAN_POINT ( 'NONE',  ( -23.83765245656579879, 1446.530553801166661, 215.3656821588423611 ) ) ;
#68818=CARTESIAN_POINT ( 'NONE',  ( -1.210091630371270099, 1409.788755468769750, 270.0714238039610109 ) ) ;
#68820=CARTESIAN_POINT ( 'NONE',  ( 13.36103377078690002, 1421.223394105900070, 230.7424813387619906 ) ) ;
#68823=ORIENTED_EDGE ( 'NONE', *, *, #5131, .T. ) ;
#68824=ORIENTED_EDGE ( 'NONE', *, *, #20739, .T. ) ;
#68825=CARTESIAN_POINT ( 'NONE',  ( -23.64789126648100037, 1411.111376611279866, 210.3824361856959797 ) ) ;
#68826=CARTESIAN_POINT ( 'NONE',  ( -3.985554679939999900, 1423.989648005430126, 184.8079733748980118 ) ) ;
#68828=CARTESIAN_POINT ( 'NONE',  ( -11.01124415049999961, 1428.984115384829920, 91.31218443469779800 ) ) ;
#68829=CARTESIAN_POINT ( 'NONE',  ( -18.21027245059960009, 1417.630028607339909, 195.0416608005989758 ) ) ;
#68830=CARTESIAN_POINT ( 'NONE',  ( -17.60168979070000006, 1415.862843299730002, 225.8220616334979809 ) ) ;
#68831=CARTESIAN_POINT ( 'NONE',  ( 35.28102380709319874, 1462.674111978580186, 269.2449631940870063 ) ) ;
#68832=CARTESIAN_POINT ( 'NONE',  ( -2.627082428580422846, 1466.871129784743061, 235.1219302449402448 ) ) ;
#68833=CARTESIAN_POINT ( 'NONE',  ( -16.37191349014004516, 1421.177096782927265, 227.0079739609353737 ) ) ;
#68835=VERTEX_POINT ( 'NONE', #29099 ) ;
#68836=CARTESIAN_POINT ( 'NONE',  ( 18.75318093336727898, 1458.167641362951599, 227.2642414340100743 ) ) ;
#68838=CARTESIAN_POINT ( 'NONE',  ( 0.000000000000000000, 1395.913060387330006, 215.6218459616979999 ) ) ;
#68839=VERTEX_POINT ( 'NONE', #9529 ) ;
#68841=CARTESIAN_POINT ( 'NONE',  ( 26.44176926394449723, 1451.249329871009877, 136.3297133206949923 ) ) ;
#68845=CARTESIAN_POINT ( 'NONE',  ( 17.95574905190000337, 1409.540088961029824, 195.3910318465979969 ) ) ;
#68847=CARTESIAN_POINT ( 'NONE',  ( 20.75326766870000128, 1443.913060387330006, 176.0807405191980024 ) ) ;
#68849=CARTESIAN_POINT ( 'NONE',  ( 3.854469939346678142, 1439.700967340914303, 184.6638362761631527 ) ) ;
#68850=CARTESIAN_POINT ( 'NONE',  ( 1.157712740350000047, 1416.622647982630042, 233.3632169813980113 ) ) ;
#68851=CARTESIAN_POINT ( 'NONE',  ( -22.48437655502024057, 1431.424403463011231, 216.6260149409388305 ) ) ;
#68852=CARTESIAN_POINT ( 'NONE',  ( 0.9798719467442907893, 1451.400798846600082, 182.8910064217580214 ) ) ;
#68853=CARTESIAN_POINT ( 'NONE',  ( -0.02546055715129019736, 1508.875231489110092, 179.6647779767779980 ) ) ;
#68856=CARTESIAN_POINT ( 'NONE',  ( 17.04824238339829634, 1423.676546790900147, 228.9394188427949928 ) ) ;
#68858=CARTESIAN_POINT ( 'NONE',  ( 12.86122366611430046, 1416.830086716310007, 221.8629622564060071 ) ) ;
#68861=CARTESIAN_POINT ( 'NONE',  ( -0.5142297307823490149, 1410.274753841589927, 233.1699704715869927 ) ) ;
#68867=CARTESIAN_POINT ( 'NONE',  ( -39.47393889809999479, 1455.502555575530096, 271.1218459616979999 ) ) ;
#68869=CARTESIAN_POINT ( 'NONE',  ( 11.05013786159999967, 1433.657746916940141, 151.7238025743979790 ) ) ;
#68870=ADVANCED_FACE ( 'NONE', ( #80049 ), #10085, .F. ) ;
#68871=CARTESIAN_POINT ( 'NONE',  ( 22.74199303559999663, 1446.314437877210139, 234.3916895436979928 ) ) ;
#68872=B_SPLINE_SURFACE_WITH_KNOTS ( 'NONE', 5, 5, ( 
 ( #88008, #45998, #28070, #2358, #2903, #29178 ),
 ( #87440, #44908, #54411, #63369, #43778, #104232 ),
 ( #36473, #62259, #20752, #79599, #9607, #96387 ),
 ( #97484, #86875, #1235, #11290, #86323, #19664 ),
 ( #10169, #53869, #45457, #71215, #105337, #28628 ),
 ( #96946, #20212, #18547, #11828, #44342, #80129 ) ),
 .UNSPECIFIED., .F., .F., .F.,
 ( 6, 6 ),
 ( 6, 6 ),
 ( 118.7831216769999969, 123.7287573859999981 ),
 ( 0.000000000000000000, 2.000000000000000000 ),
 .UNSPECIFIED. ) ;
#68873=CARTESIAN_POINT ( 'NONE',  ( 12.85343379848070100, 1416.225364278609959, 196.3904799426800025 ) ) ;
#68875=B_SPLINE_CURVE_WITH_KNOTS ( 'NONE', 3,
 ( #85682, #24107, #34184, #26322, #33074, #17350, #102477 ),
 .UNSPECIFIED., .F., .F.,
 ( 4, 3, 4 ),
 ( 0.000000000000000000, 0.0008424868321600594316, 0.002213898725977839644 ),
 .UNSPECIFIED. ) ;
#68877=CARTESIAN_POINT ( 'NONE',  ( -15.06279246576909259, 1422.388300736680321, 229.4662110716209327 ) ) ;
#68878=CARTESIAN_POINT ( 'NONE',  ( -3.511104830509999886, 1486.134592826630069, 181.9823189358980073 ) ) ;
#68879=CARTESIAN_POINT ( 'NONE',  ( 12.73679432148881574, 1398.290618096285471, 206.5085731043449755 ) ) ;
#68880=CARTESIAN_POINT ( 'NONE',  ( 0.05322450152090000414, 1509.045416624730024, 239.1217102979979643 ) ) ;
#68883=CARTESIAN_POINT ( 'NONE',  ( 3.503070653725943284, 1446.464826921931717, 170.5350607410328507 ) ) ;
#68884=CARTESIAN_POINT ( 'NONE',  ( 26.72339292633054342, 1436.753392519305862, 136.7836805358251411 ) ) ;
#68886=FACE_OUTER_BOUND ( 'NONE', #254, .T. ) ;
#68891=CARTESIAN_POINT ( 'NONE',  ( 0.1631646649216179912, 1484.369741073460091, 181.9066623653069996 ) ) ;
#68892=DIRECTION ( 'NONE',  ( 0.6212649842969746317, 0.04409479819909335047, -0.7823589125575685088 ) ) ;
#68893=ORIENTED_EDGE ( 'NONE', *, *, #107785, .F. ) ;
#68895=CARTESIAN_POINT ( 'NONE',  ( -33.46247258405923475, 1444.994950788469168, 154.5793418554282539 ) ) ;
#68896=CARTESIAN_POINT ( 'NONE',  ( -9.258583944369999847E-15, 1443.913060387330006, 150.8032249175980155 ) ) ;
#68901=AXIS2_PLACEMENT_3D ( 'NONE', #103469, #95638, #19470 ) ;
#68903=CARTESIAN_POINT ( 'NONE',  ( -12.97490759070000088, 1414.913060387329779, 220.5751958562979951 ) ) ;
#68912=CARTESIAN_POINT ( 'NONE',  ( -17.60565864420000182, 1410.875688248029974, 193.0296143146979944 ) ) ;
#68915=CARTESIAN_POINT ( 'NONE',  ( 17.22592482065197927, 1443.501467202829190, 162.9227486220069920 ) ) ;
#68916=CARTESIAN_POINT ( 'NONE',  ( -2.370970874524634286, 1427.002265528474027, 137.0999999980979567 ) ) ;
#68918=CARTESIAN_POINT ( 'NONE',  ( -11.41961239078290191, 1507.432264719158638, 233.9077293063710385 ) ) ;
#68926=CARTESIAN_POINT ( 'NONE',  ( 5.776215007970000315, 1396.296062261630141, 219.5799249200979943 ) ) ;
#68927=CARTESIAN_POINT ( 'NONE',  ( 2.797255426280000012, 1417.697071498429978, 234.5789349732979758 ) ) ;
#68931=CARTESIAN_POINT ( 'NONE',  ( -2.409586283469999923, 1426.663880916129983, 144.1938086916980239 ) ) ;
#68934=CARTESIAN_POINT ( 'NONE',  ( -2.500000000000000000, 1438.970653384089928, 157.7201897330980103 ) ) ;
#68935=CARTESIAN_POINT ( 'NONE',  ( 43.39686093150000090, 1451.895030900229813, 269.7191771298979575 ) ) ;
#68937=ORIENTED_EDGE ( 'NONE', *, *, #109189, .F. ) ;
#68938=CARTESIAN_POINT ( 'NONE',  ( 10.79382269979189957, 1414.913060387349788, 222.1041130917409987 ) ) ;
#68941=CARTESIAN_POINT ( 'NONE',  ( -24.30946323690000099, 1430.356462489929982, 206.1914330134380009 ) ) ;
#68942=CARTESIAN_POINT ( 'NONE',  ( -11.30626018579999936, 1426.878239686230017, 113.0072544287980065 ) ) ;
#68944=CARTESIAN_POINT ( 'NONE',  ( 17.25149442856769610, 1410.459880232700243, 192.3767002299429976 ) ) ;
#68946=CARTESIAN_POINT ( 'NONE',  ( 29.87053939714199657, 1510.066426918421257, 204.8311492353107894 ) ) ;
#68947=CARTESIAN_POINT ( 'NONE',  ( -21.19319384159999942, 1471.316885392730001, 208.3912962420869803 ) ) ;
#68948=CARTESIAN_POINT ( 'NONE',  ( -14.25478412350000212, 1406.894180200230267, 267.1909259577980151 ) ) ;
#68949=CARTESIAN_POINT ( 'NONE',  ( 19.39560819206040065, 1509.616854481060045, 231.5472923800719798 ) ) ;
#68950=CARTESIAN_POINT ( 'NONE',  ( 28.43277596785110006, 1508.901247230659919, 209.4404433710649869 ) ) ;
#68952=CARTESIAN_POINT ( 'NONE',  ( -39.00494972961689655, 1439.722668488820091, 136.7021091258499723 ) ) ;
#68954=FACE_OUTER_BOUND ( 'NONE', #92695, .T. ) ;
#68956=CARTESIAN_POINT ( 'NONE',  ( -17.39471470580000201, 1458.587118211430152, 228.8964261825979918 ) ) ;
#68958=VERTEX_POINT ( 'NONE', #108555 ) ;
#68959=CARTESIAN_POINT ( 'NONE',  ( -29.36423093692776121, 1509.941268890160018, 211.4558441758299523 ) ) ;
#68960=CARTESIAN_POINT ( 'NONE',  ( -6.305024129259999555, 1422.156209412130011, 144.1468801376980196 ) ) ;
#68966=CARTESIAN_POINT ( 'NONE',  ( 26.87217692225963361, 1508.240760517084027, 206.2294961738559778 ) ) ;
#68967=CARTESIAN_POINT ( 'NONE',  ( 1.435143914157240186, 1420.925611785209867, 183.0242435332739888 ) ) ;
#68968=VECTOR ( 'NONE', #67629, 1000.000000000000114 ) ;
#68972=EDGE_LOOP ( 'NONE', ( #103895, #45943, #44194, #101001 ) ) ;
#68976=CARTESIAN_POINT ( 'NONE',  ( 11.81097173189579941, 1428.791000847919804, 148.7051997554240188 ) ) ;
#68981=CARTESIAN_POINT ( 'NONE',  ( 11.45019036429999915, 1509.312909845629974, 236.0262225088980017 ) ) ;
#68984=CARTESIAN_POINT ( 'NONE',  ( -5.528991355650000550, 1423.112510947830060, 186.1101815182979919 ) ) ;
#68985=CARTESIAN_POINT ( 'NONE',  ( 10.57863187995810073, 1410.707288523929947, 270.0764058261560194 ) ) ;
#68986=CARTESIAN_POINT ( 'NONE',  ( -8.991629940588330427, 1509.227055023859975, 237.0095830223739881 ) ) ;
#68988=CARTESIAN_POINT ( 'NONE',  ( -14.46866624055838990, 1410.791144959253643, 190.4540876299275283 ) ) ;
#68990=CARTESIAN_POINT ( 'NONE',  ( -16.57804597599999852, 1485.105086709729903, 223.5480764049980280 ) ) ;
#68991=CARTESIAN_POINT ( 'NONE',  ( 17.68181829800000315, 1459.090084424630277, 228.3014959847979810 ) ) ;
#68993=CARTESIAN_POINT ( 'NONE',  ( -4.871044490860866105, 1423.449036601908119, 184.6413674952053441 ) ) ;
#68999=CARTESIAN_POINT ( 'NONE',  ( -2.986641160691798191, 1485.642120341665077, 182.6840798815813685 ) ) ;
#69002=VERTEX_POINT ( 'NONE', #55963 ) ;
#69003=CARTESIAN_POINT ( 'NONE',  ( 1.327504031670000195, 1471.309244717329875, 187.7603546987980110 ) ) ;
#69004=CARTESIAN_POINT ( 'NONE',  ( -15.21149315567410021, 1507.619498552399818, 191.9000986313440364 ) ) ;
#69005=CARTESIAN_POINT ( 'NONE',  ( -11.23092292039999940, 1427.419555970229794, 149.5756494223980155 ) ) ;
#69006=CARTESIAN_POINT ( 'NONE',  ( -12.53380580351000084, 1442.773887400870080, 185.9733686700720057 ) ) ;
#69010=FACE_OUTER_BOUND ( 'NONE', #48159, .T. ) ;
#69011=CARTESIAN_POINT ( 'NONE',  ( -22.49156919629999862, 1508.010176357929822, 225.3481774520980139 ) ) ;
#69013=CARTESIAN_POINT ( 'NONE',  ( -16.78409198796899915, 1460.264608996595825, 228.3353229335820060 ) ) ;
#69015=CARTESIAN_POINT ( 'NONE',  ( 18.18323680749999838, 1409.226845187329900, 269.3834355279979604 ) ) ;
#69016=CARTESIAN_POINT ( 'NONE',  ( 23.93773119740000155, 1435.477561280669761, 138.6590435606979952 ) ) ;
#69017=CARTESIAN_POINT ( 'NONE',  ( 18.31698807710000310, 1430.307821480030043, 192.4318916728979900 ) ) ;
#69018=CARTESIAN_POINT ( 'NONE',  ( 21.41666166824317585, 1506.776553316454283, 215.7211524448117359 ) ) ;
#69020=EDGE_CURVE ( 'NONE', #110792, #49383, #11352, .T. ) ;
#69021=CARTESIAN_POINT ( 'NONE',  ( -0.08826310995340809484, 1508.140386909309882, 237.5604311155479706 ) ) ;
#69024=CARTESIAN_POINT ( 'NONE',  ( -41.66768437117050183, 1443.241400757599877, 135.6286676937990023 ) ) ;
#69025=CARTESIAN_POINT ( 'NONE',  ( -18.61615538203637854, 1506.404057884007671, 197.4600136827062613 ) ) ;
#69027=CARTESIAN_POINT ( 'NONE',  ( -13.39006534200000154, 1443.300441888700107, 187.2669796394979755 ) ) ;
#69029=CARTESIAN_POINT ( 'NONE',  ( -14.60782360329999996, 1431.113060387329824, 222.3499097932980249 ) ) ;
#69030=B_SPLINE_SURFACE_WITH_KNOTS ( 'NONE', 5, 5, ( 
 ( #24241, #50023, #39409, #15819, #65727, #24776 ),
 ( #101490, #90909, #5819, #92014, #48379, #13626 ),
 ( #6357, #48936, #58424, #41618, #107716, #99847 ),
 ( #39958, #23140, #73585, #57344, #23696, #90346 ),
 ( #91468, #75772, #66296, #83600, #83066, #84155 ),
 ( #109922, #65179, #66837, #100412, #6898, #67392 ),
 ( #31000, #33202, #14192, #41054, #40505, #47814 ),
 ( #109383, #81949, #5253, #75233, #99291, #22566 ),
 ( #56771, #93642, #8002, #25334, #50575, #730 ),
 ( #42167, #76320, #94205, #188, #86369, #8550 ),
 ( #43280, #77973, #1845, #84701, #60090, #35420 ),
 ( #58974, #76877, #16377, #42722, #110470, #85816 ),
 ( #60646, #26453, #94770, #17479, #9652, #69050 ),
 ( #93106, #34309, #59530, #77427, #16924, #51126 ),
 ( #103725, #69607, #18591, #52787, #33747, #51679 ),
 ( #68490, #104282, #43826, #70171, #9114, #67942 ),
 ( #102050, #27027, #95330, #34862, #102591, #25891 ),
 ( #103151, #85250, #18047, #52241, #1279, #61215 ),
 ( #86923, #10214, #44392, #78534, #35980, #88052 ),
 ( #27570, #36525, #97534, #53917, #47140, #62885 ),
 ( #55549, #89673, #80736, #71272, #11337, #28119 ) ),
 .UNSPECIFIED., .F., .F., .F.,
 ( 6, 3, 3, 3, 3, 3, 6 ),
 ( 6, 6 ),
 ( 39.80009957240000062, 49.32247488090000331, 52.79489999459999439, 54.53111255139999969, 56.26732510819999789, 56.97897492249999374, 58.84485018950000068 ),
 ( 0.000000000000000000, 1.469182821640000025 ),
 .UNSPECIFIED. ) ;
#69031=CARTESIAN_POINT ( 'NONE',  ( -30.80659297389999907, 1435.733914001370067, 136.0405333270979895 ) ) ;
#69035=CARTESIAN_POINT ( 'NONE',  ( -12.85845572773480150, 1409.362087555840162, 216.7356519297030104 ) ) ;
#69038=CARTESIAN_POINT ( 'NONE',  ( -12.72837614330000022, 1474.761265398429941, 267.4694132100979687 ) ) ;
#69041=CARTESIAN_POINT ( 'NONE',  ( -24.27333433320000111, 1509.087578212329845, 222.4402611466979920 ) ) ;
#69044=CARTESIAN_POINT ( 'NONE',  ( 18.80671126632940116, 1425.657109644339926, 226.1563198364650020 ) ) ;
#69045=CARTESIAN_POINT ( 'NONE',  ( -3.364556988579999963, 1443.913060387330006, 155.8032249175980155 ) ) ;
#69048=CARTESIAN_POINT ( 'NONE',  ( -46.02998242119897299, 1440.913029505377381, 268.4959138949732278 ) ) ;
#69050=CARTESIAN_POINT ( 'NONE',  ( -23.46122789450000212, 1411.092679750530124, 206.2085811050380073 ) ) ;
#69052=CARTESIAN_POINT ( 'NONE',  ( 14.74831652169999963, 1414.913060387329779, 202.0310540578979897 ) ) ;
#69055=CARTESIAN_POINT ( 'NONE',  ( 2.493947715939999643, 1442.756953654919926, 150.6345094620980092 ) ) ;
#69059=CARTESIAN_POINT ( 'NONE',  ( -21.74753855979999884, 1409.672501167229939, 211.1389744297880213 ) ) ;
#69064=CARTESIAN_POINT ( 'NONE',  ( -18.26675480510339966, 1424.840341062940070, 227.6848255537819909 ) ) ;
#69066=B_SPLINE_CURVE_WITH_KNOTS ( 'NONE', 5,
 ( #53303, #104237, #11294, #45462, #63908, #29182, #37026, #62263, #54955 ),
 .UNSPECIFIED., .F., .F.,
 ( 6, 3, 6 ),
 ( 0.9063219059076105255, 0.9212159755548054996, 1.000000000000000000 ),
 .UNSPECIFIED. ) ;
#69068=CARTESIAN_POINT ( 'NONE',  ( -1.783433545534589104, 1397.966851194222954, 222.0187806250839060 ) ) ;
#69070=CARTESIAN_POINT ( 'NONE',  ( 4.500000000000000000, 1432.413060387330006, 146.1721969590979882 ) ) ;
#69072=CARTESIAN_POINT ( 'NONE',  ( 37.61621548944700066, 1449.688575227499996, 136.2442305511190170 ) ) ;
#69076=CARTESIAN_POINT ( 'NONE',  ( 0.2751658889820000065, 1506.798305107329952, 186.8348836488979998 ) ) ;
#69077=CARTESIAN_POINT ( 'NONE',  ( 0.08248983565340001212, 1397.911842041330146, 222.1215842506979925 ) ) ;
#69079=CARTESIAN_POINT ( 'NONE',  ( -0.0001938387787944162953, 1397.283789131768117, 222.0379186164004466 ) ) ;
#69080=CARTESIAN_POINT ( 'NONE',  ( 17.04824238339829634, 1423.676546790900147, 228.9394188427949928 ) ) ;
#69082=CARTESIAN_POINT ( 'NONE',  ( 16.01295443681960151, 1422.119564716039804, 191.1690555812749892 ) ) ;
#69083=CARTESIAN_POINT ( 'NONE',  ( 8.968501251859999357, 1428.602659895330135, 101.8807690336980016 ) ) ;
#69084=CARTESIAN_POINT ( 'NONE',  ( 18.08856701439330195, 1498.113134534269875, 229.9575450159010188 ) ) ;
#69085=CARTESIAN_POINT ( 'NONE',  ( 2.458572921189999594, 1507.640305379429947, 181.2872115462979821 ) ) ;
#69089=CARTESIAN_POINT ( 'NONE',  ( 36.51516363007900168, 1436.208852635709945, 134.0999999969979797 ) ) ;
#69090=CARTESIAN_POINT ( 'NONE',  ( 11.86176063160000105, 1432.032830640380098, 149.9745659136979725 ) ) ;
#69093=CARTESIAN_POINT ( 'NONE',  ( 14.06744947489100106, 1435.197734885789941, 149.3372217745049966 ) ) ;
#69097=CARTESIAN_POINT ( 'NONE',  ( 12.64457216002790574, 1445.030948195889323, 169.4649751935023119 ) ) ;
#69098=CARTESIAN_POINT ( 'NONE',  ( -1.296202833079999950, 1464.946618178429844, 237.1878767853979753 ) ) ;
#69106=CARTESIAN_POINT ( 'NONE',  ( 0.8957163599030000256, 1507.375187373130075, 237.2105928541979836 ) ) ;
#69110=CARTESIAN_POINT ( 'NONE',  ( 19.42500282749999840, 1440.913060387330006, 212.4633492400480179 ) ) ;
#69111=CARTESIAN_POINT ( 'NONE',  ( -20.17745077670000242, 1509.606869791130066, 230.6312312576980048 ) ) ;
#69113=CARTESIAN_POINT ( 'NONE',  ( -9.153149079460000337, 1409.735973916530156, 188.2996874139979866 ) ) ;
#69115=CARTESIAN_POINT ( 'NONE',  ( -9.380124768717641004, 1428.163396101657781, 137.0999999980979851 ) ) ;
#69117=CARTESIAN_POINT ( 'NONE',  ( 24.50256053759999730, 1438.051362122639830, 212.5740290884979800 ) ) ;
#69123=CIRCLE ( 'NONE', #4680, 2.000000000000000000 ) ;
#69124=CARTESIAN_POINT ( 'NONE',  ( -21.92423686380000092, 1509.678671609130106, 190.3411753256980035 ) ) ;
#69126=CARTESIAN_POINT ( 'NONE',  ( -16.90742456150000095, 1442.831169986189934, 162.4348202098979925 ) ) ;
#69132=CARTESIAN_POINT ( 'NONE',  ( 35.93745672850000261, 1447.859703060729998, 254.6053128065979934 ) ) ;
#69133=CARTESIAN_POINT ( 'NONE',  ( 3.490272952469018364, 1450.862712094549352, 184.0573294561584134 ) ) ;
#69134=CARTESIAN_POINT ( 'NONE',  ( -28.74419454077009917, 1509.916829779089994, 215.0463914455240229 ) ) ;
#69135=CARTESIAN_POINT ( 'NONE',  ( -8.326540575840001068, 1507.918730918930123, 235.2420017123980074 ) ) ;
#69138=CARTESIAN_POINT ( 'NONE',  ( 11.57592109439999994, 1432.301060653729792, 151.1967999008980144 ) ) ;
#69139=CARTESIAN_POINT ( 'NONE',  ( 19.09164403609999994, 1456.344937430229947, 226.3477507761979837 ) ) ;
#69144=CARTESIAN_POINT ( 'NONE',  ( 3.780309398849999084E-14, 1406.777728848529932, 269.6500679732980075 ) ) ;
#69145=CARTESIAN_POINT ( 'NONE',  ( 27.72858359559999997, 1508.599279870730015, 207.6849852067780091 ) ) ;
#69146=CARTESIAN_POINT ( 'NONE',  ( 24.59137937210000047, 1442.248894770099923, 213.3251317051179967 ) ) ;
#69147=CARTESIAN_POINT ( 'NONE',  ( 5.386093888109999561, 1432.347042751149957, 154.6076556448980170 ) ) ;
#69150=CARTESIAN_POINT ( 'NONE',  ( 26.80760470685860142, 1436.328554475559940, 136.7304320938700073 ) ) ;
#69151=CARTESIAN_POINT ( 'NONE',  ( 34.60210436545990120, 1450.378017727679890, 136.2318747066630067 ) ) ;
#69152=CARTESIAN_POINT ( 'NONE',  ( -34.13334863075944270, 1463.712688128719037, 269.2713322011451851 ) ) ;
#69157=CARTESIAN_POINT ( 'NONE',  ( -42.06231930236405248, 1442.702167343311658, 269.6487547253948378 ) ) ;
#69160=CARTESIAN_POINT ( 'NONE',  ( 13.50151513640000189, 1434.968987195889895, 146.5972134562979932 ) ) ;
#69163=CARTESIAN_POINT ( 'NONE',  ( 11.44665326297827335, 1425.798162341591706, 139.1345266541928538 ) ) ;
#69166=CARTESIAN_POINT ( 'NONE',  ( 19.26928223589375833, 1455.917628554740986, 225.9370567887913808 ) ) ;
#69171=CARTESIAN_POINT ( 'NONE',  ( -18.45314936670000350, 1415.553739809529816, 207.8952753008079810 ) ) ;
#69173=CARTESIAN_POINT ( 'NONE',  ( 25.79054002703109916, 1435.417905869039942, 135.6747449796359888 ) ) ;
#69174=CARTESIAN_POINT ( 'NONE',  ( -13.51610093808349866, 1443.887577857937458, 169.3501091255429856 ) ) ;
#69175=ORIENTED_EDGE ( 'NONE', *, *, #69995, .T. ) ;
#69176=CARTESIAN_POINT ( 'NONE',  ( -16.39775370592910164, 1409.510809139110052, 225.2343662999429910 ) ) ;
#69177=CARTESIAN_POINT ( 'NONE',  ( 9.771922359260001301, 1440.444625599219989, 148.8200729295979841 ) ) ;
#69178=EDGE_LOOP ( 'NONE', ( #28471, #79709, #52222, #3240 ) ) ;
#69182=CARTESIAN_POINT ( 'NONE',  ( 10.03329442769999957, 1425.203965949929852, 96.53732743869790056 ) ) ;
#69184=DIRECTION ( 'NONE',  ( 0.9846671174924281900, -0.1149361401860498344, -0.1312263365650570279 ) ) ;
#69185=CARTESIAN_POINT ( 'NONE',  ( 4.350626057107779054, 1425.642856625690001, 185.4477024701949972 ) ) ;
#69187=CARTESIAN_POINT ( 'NONE',  ( -2.901771220848202937, 1419.574541655020312, 186.1989676290672264 ) ) ;
#69190=CARTESIAN_POINT ( 'NONE',  ( 7.925631312170001053, 1509.190094470230179, 180.8627748357979783 ) ) ;
#69191=CARTESIAN_POINT ( 'NONE',  ( 2.531379128109999765, 1449.143641694869984, 182.8453065789979917 ) ) ;
#69196=CARTESIAN_POINT ( 'NONE',  ( -41.66194525459999909, 1443.744937001919880, 136.1277553619979699 ) ) ;
#69198=CARTESIAN_POINT ( 'NONE',  ( -3.056877442999999861, 1471.506820614530170, 269.6159236013979807 ) ) ;
#69199=CARTESIAN_POINT ( 'NONE',  ( 12.74692502376422176, 1434.633369486244646, 147.1384066575065219 ) ) ;
#69200=CARTESIAN_POINT ( 'NONE',  ( 0.1420983796599999682, 1486.103412518930099, 181.9585633641979996 ) ) ;
#69201=CARTESIAN_POINT ( 'NONE',  ( 21.00523825079999796, 1507.839072599329711, 190.5229776796980161 ) ) ;
#69203=CARTESIAN_POINT ( 'NONE',  ( -36.39519410782710196, 1451.404435322049949, 135.1209920990980038 ) ) ;
#69204=CARTESIAN_POINT ( 'NONE',  ( -11.60004869885203682, -0.000000000000000000, 137.0999999980979851 ) ) ;
#69205=CARTESIAN_POINT ( 'NONE',  ( 38.62863167664609421, 1444.143249097809985, 137.1666610355499927 ) ) ;
#69207=CARTESIAN_POINT ( 'NONE',  ( 8.993528449059150276, 1407.583683456149856, 198.9375600053470237 ) ) ;
#69208=CARTESIAN_POINT ( 'NONE',  ( -20.64901375512450343, 1409.367826505309949, 267.6706922366469712 ) ) ;
#69209=CARTESIAN_POINT ( 'NONE',  ( -13.86043986179080001, 1435.008531462659903, 148.8737775447249874 ) ) ;
#69211=CARTESIAN_POINT ( 'NONE',  ( -11.30175580989999951, 1432.339690393880119, 151.5220148440980097 ) ) ;
#69212=CARTESIAN_POINT ( 'NONE',  ( 13.28241350259999898, 1445.641312562420126, 188.6965274455980079 ) ) ;
#69219=CARTESIAN_POINT ( 'NONE',  ( -16.02210698220000040, 1470.468178375529988, 188.3958660763979935 ) ) ;
#69222=EDGE_CURVE ( 'NONE', #103324, #36366, #16646, .T. ) ;
#69225=CARTESIAN_POINT ( 'NONE',  ( 9.626138668350000316, 1415.087974640030097, 223.7831235720980203 ) ) ;
#69227=CARTESIAN_POINT ( 'NONE',  ( -29.35556035689999987, 1509.949879406430000, 205.5028565010079831 ) ) ;
#69229=CARTESIAN_POINT ( 'NONE',  ( 1.436979206307143375, 1507.073228327747302, 236.7831034515724014 ) ) ;
#69232=ADVANCED_FACE ( 'NONE', ( #21499 ), #78833, .F. ) ;
#69234=CARTESIAN_POINT ( 'NONE',  ( -1.286178515069999806, 1407.887987576529895, 195.9343300142979842 ) ) ;
#69235=CARTESIAN_POINT ( 'NONE',  ( -12.38733338750000179, 1409.511671407230097, 227.5189851686980091 ) ) ;
#69236=CARTESIAN_POINT ( 'NONE',  ( -4.164625339459999687, 1446.237990885560066, 183.4551341185980107 ) ) ;
#69237=ORIENTED_EDGE ( 'NONE', *, *, #6835, .T. ) ;
#69239=CARTESIAN_POINT ( 'NONE',  ( 27.53546928359999768, 1508.129852616029893, 212.9718660772680039 ) ) ;
#69242=CARTESIAN_POINT ( 'NONE',  ( -24.72639760740000270, 1435.360974979420007, 136.0074239971980035 ) ) ;
#69250=LINE ( 'NONE', #9870, #90229 ) ;
#69251=CARTESIAN_POINT ( 'NONE',  ( 5.401672926506360106, 1440.924418278400026, 154.8182599678980012 ) ) ;
#69252=EDGE_CURVE ( 'NONE', #25299, #49915, #31350, .T. ) ;
#69254=ORIENTED_EDGE ( 'NONE', *, *, #93787, .T. ) ;
#69256=LINE ( 'NONE', #103363, #92405 ) ;
#69257=CARTESIAN_POINT ( 'NONE',  ( 12.23184522910000105, 1434.618918689169959, 150.6553485564980122 ) ) ;
#69258=CARTESIAN_POINT ( 'NONE',  ( 16.24562813123679561, 1478.707530004980072, 230.1287771015380201 ) ) ;
#69261=CARTESIAN_POINT ( 'NONE',  ( -1.408971986799999909, 1408.962262773329940, 187.0389398893979944 ) ) ;
#69267=CARTESIAN_POINT ( 'NONE',  ( 19.63615699109999824, 1508.568590227029972, 188.6353561189980041 ) ) ;
#69272=CARTESIAN_POINT ( 'NONE',  ( -20.34835314180000054, 1499.713795797229977, 189.8114522981980201 ) ) ;
#69273=VERTEX_POINT ( 'NONE', #27311 ) ;
#69274=ADVANCED_FACE ( 'NONE', ( #95622 ), #77676, .T. ) ;
#69275=CARTESIAN_POINT ( 'NONE',  ( 3.521117552959999841, 1421.670602369330027, 184.1604385248979838 ) ) ;
#69279=CARTESIAN_POINT ( 'NONE',  ( -3.819157230050550598E-10, 1415.320034473050100, 235.4381035424730158 ) ) ;
#69280=B_SPLINE_CURVE_WITH_KNOTS ( 'NONE', 5,
 ( #13722, #47907, #82615, #48477, #82043, #56867 ),
 .UNSPECIFIED., .F., .F.,
 ( 6, 6 ),
 ( -1.468559632160000072, -1.438859269287107168E-06 ),
 .UNSPECIFIED. ) ;
#69281=CARTESIAN_POINT ( 'NONE',  ( -4.283010808509999379, 1446.850643219170024, 156.0812219214980132 ) ) ;
#69282=CARTESIAN_POINT ( 'NONE',  ( 15.87566767260028833, 1507.597642236632055, 231.8003891413981421 ) ) ;
#69284=DIRECTION ( 'NONE',  ( 0.7074300731457748848, -0.02470400237811459093, 0.7063514733300028103 ) ) ;
#69285=CARTESIAN_POINT ( 'NONE',  ( 17.01771828639999740, 1416.204137079330167, 191.6576494061979758 ) ) ;
#69287=CARTESIAN_POINT ( 'NONE',  ( 0.5987183461865049905, 1507.212886145319999, 186.4932301926239688 ) ) ;
#69288=CARTESIAN_POINT ( 'NONE',  ( 10.96946812545280103, 1432.347663862999980, 151.7701354189910035 ) ) ;
#69289=ORIENTED_EDGE ( 'NONE', *, *, #96325, .T. ) ;
#69290=CARTESIAN_POINT ( 'NONE',  ( 1.553484637916519917, 1415.542389211330146, 190.7873441232580092 ) ) ;
#69292=CARTESIAN_POINT ( 'NONE',  ( 26.86204974310000182, 1508.007394749430205, 206.2315949334080187 ) ) ;
#69297=CARTESIAN_POINT ( 'NONE',  ( -3.549608351769999892, 1507.276797637930031, 180.9704965309979912 ) ) ;
#69303=CARTESIAN_POINT ( 'NONE',  ( 19.97872766260000077, 1452.215387843930102, 143.5714034319979930 ) ) ;
#69304=EDGE_CURVE ( 'NONE', #22078, #13046, #59543, .T. ) ;
#69305=CARTESIAN_POINT ( 'NONE',  ( -15.37090796494357825, 1506.446781329460464, 224.8527620067033297 ) ) ;
#69307=CARTESIAN_POINT ( 'NONE',  ( 24.27343742149999883, 1509.087597399430024, 195.8036337447979918 ) ) ;
#69309=CARTESIAN_POINT ( 'NONE',  ( -18.38172408721423068, 1459.016642225524038, 227.7444303527029774 ) ) ;
#69312=VERTEX_POINT ( 'NONE', #65005 ) ;
#69314=CARTESIAN_POINT ( 'NONE',  ( 13.63158477449999850, 1446.168541001489984, 189.0290012264979964 ) ) ;
#69317=CARTESIAN_POINT ( 'NONE',  ( 19.03312855989999974, 1434.814457747880169, 209.2860607477259975 ) ) ;
#69318=CARTESIAN_POINT ( 'NONE',  ( -33.67852042730000761, 1460.266105628030118, 261.9077679340980467 ) ) ;
#69322=ADVANCED_FACE ( 'NONE', ( #110294 ), #73954, .F. ) ;
#69323=CARTESIAN_POINT ( 'NONE',  ( -12.45548913970438853, 1435.744143842510539, 150.9793205285649265 ) ) ;
#69324=CARTESIAN_POINT ( 'NONE',  ( -18.49631469930000094, 1416.851343894929869, 208.7101585479910000 ) ) ;
#69325=CARTESIAN_POINT ( 'NONE',  ( 4.237847613999999652, 1409.564918727129907, 186.3248662794979964 ) ) ;
#69326=CARTESIAN_POINT ( 'NONE',  ( 4.363111636370000213, 1423.854804604630090, 183.5697630181979889 ) ) ;
#69327=CARTESIAN_POINT ( 'NONE',  ( -9.836119169070000723, 1438.961854973259960, 152.9388125716980085 ) ) ;
#69328=CARTESIAN_POINT ( 'NONE',  ( 10.37614134790000087, 1435.190621590189949, 152.2457780280979875 ) ) ;
#69331=CARTESIAN_POINT ( 'NONE',  ( -9.270813479730000140, 1452.444632404429967, 152.0931890696979849 ) ) ;
#69336=CARTESIAN_POINT ( 'NONE',  ( -44.70563246039999683, 1440.913062630770128, 269.9105894055979888 ) ) ;
#69337=DIRECTION ( 'NONE',  ( 0.9483721503360844629, -0.1343667288060120535, 0.2872905265700261279 ) ) ;
#69338=CARTESIAN_POINT ( 'NONE',  ( 17.41030305009999779, 1410.018619230629838, 223.8936866133980175 ) ) ;
#69339=EDGE_CURVE ( 'NONE', #69349, #39470, #107509, .T. ) ;
#69341=CARTESIAN_POINT ( 'NONE',  ( 2.897498764350990186, 1409.458680991969914, 231.2323409181370266 ) ) ;
#69343=CARTESIAN_POINT ( 'NONE',  ( -7.560007814519999592, 1417.633148021330044, 231.2533292727980268 ) ) ;
#69346=CARTESIAN_POINT ( 'NONE',  ( -46.16525872307749978, 1438.439294611029709, 267.5933863983919991 ) ) ;
#69348=EDGE_CURVE ( 'NONE', #93667, #107006, #62131, .T. ) ;
#69349=VERTEX_POINT ( 'NONE', #702 ) ;
#69355=DIRECTION ( 'NONE',  ( 0.3363363966051478027, 0.9417419117351976121, -2.812289527534883684E-09 ) ) ;
#69357=CARTESIAN_POINT ( 'NONE',  ( -25.74067306890999873, 1452.014159533350039, 135.1052487677340253 ) ) ;
#69359=CARTESIAN_POINT ( 'NONE',  ( -17.33016184879966204, 1410.462515310626713, 225.7401866622987541 ) ) ;
#69363=( BOUNDED_CURVE ( )  B_SPLINE_CURVE ( 3, ( #86788, #72619, #68918, #18452 ),
 .UNSPECIFIED., .F., .F. ) 
 B_SPLINE_CURVE_WITH_KNOTS ( ( 4, 4 ),
 ( 3.284991966284695142, 3.571871965064760346 ),
 .UNSPECIFIED. ) 
 CURVE ( )  GEOMETRIC_REPRESENTATION_ITEM ( )  RATIONAL_B_SPLINE_CURVE ( ( 1.000000000000000000, 0.9931534066853130449, 0.9931534066853130449, 1.000000000000000000 ) ) 
 REPRESENTATION_ITEM ( '' )  );
#69364=CARTESIAN_POINT ( 'NONE',  ( -10.96966273854589957, 1432.359729197300112, 151.7701366752919796 ) ) ;
#69369=ORIENTED_EDGE ( 'NONE', *, *, #75380, .T. ) ;
#69370=CARTESIAN_POINT ( 'NONE',  ( -4.172734005785669886, 1410.537251115530125, 269.3368119707569690 ) ) ;
#69372=CARTESIAN_POINT ( 'NONE',  ( 7.957816838496420964, 1418.901444373749882, 232.5320780446629954 ) ) ;
#69373=CARTESIAN_POINT ( 'NONE',  ( -0.4599830242969941141, 1508.922867521862145, 238.6015126468603569 ) ) ;
#69375=EDGE_LOOP ( 'NONE', ( #47065, #7810, #33433, #104456 ) ) ;
#69377=CARTESIAN_POINT ( 'NONE',  ( -23.06575186558750090, 1409.834430086540124, 209.8350140253269842 ) ) ;
#69378=ADVANCED_FACE ( 'NONE', ( #33173 ), #88468, .F. ) ;
#69379=CARTESIAN_POINT ( 'NONE',  ( -1.137698304267330096, 1410.327606596320265, 185.3853181447140059 ) ) ;
#69380=CARTESIAN_POINT ( 'NONE',  ( 3.727927280429065515, 1425.399814015164338, 185.1578063585167513 ) ) ;
#69382=CARTESIAN_POINT ( 'NONE',  ( -8.363327067911551893, 1406.549745658205438, 266.9340124281022213 ) ) ;
#69384=CARTESIAN_POINT ( 'NONE',  ( -18.75340623979260002, 1434.970300145230112, 194.4886870813739961 ) ) ;
#69385=CARTESIAN_POINT ( 'NONE',  ( -21.83928577469999865, 1430.785017815930132, 218.7203724610579911 ) ) ;
#69386=CARTESIAN_POINT ( 'NONE',  ( 22.48834728391410209, 1471.669847397150079, 266.7671210210439767 ) ) ;
#69387=CARTESIAN_POINT ( 'NONE',  ( -6.430339621037643560, 1466.008313631039528, 233.9307461128825878 ) ) ;
#69390=VERTEX_POINT ( 'NONE', #53888 ) ;
#69391=CARTESIAN_POINT ( 'NONE',  ( 21.70910712195382430, 1411.031551472956380, 216.7158344536642574 ) ) ;
#69393=CARTESIAN_POINT ( 'NONE',  ( 23.57286938940000098, 1410.708643128529957, 207.8716802985080108 ) ) ;
#69396=CARTESIAN_POINT ( 'NONE',  ( 26.31673506719999978, 1451.748965920229921, 135.8560917224979789 ) ) ;
#69400=CARTESIAN_POINT ( 'NONE',  ( 18.31811527990000243, 1410.915650460429788, 194.0164629065979796 ) ) ;
#69402=CARTESIAN_POINT ( 'NONE',  ( 2.789113515896739948, 1439.662583475943393, 183.8117166454382811 ) ) ;
#69404=CARTESIAN_POINT ( 'NONE',  ( -18.67702562490066498, 1424.502089277812502, 224.7510542254474331 ) ) ;
#69407=CARTESIAN_POINT ( 'NONE',  ( -0.2751659207381170202, 1506.798305148240161, 231.4088083080649767 ) ) ;
#69408=CARTESIAN_POINT ( 'NONE',  ( 28.59841869927651103, 1509.911739174257491, 206.6816370879510316 ) ) ;
#69411=CARTESIAN_POINT ( 'NONE',  ( 4.087631528831106920, 1417.919639086681173, 234.1544686792272785 ) ) ;
#69413=CARTESIAN_POINT ( 'NONE',  ( 12.86029672966080106, 1416.218865267220053, 221.6945511805459716 ) ) ;
#69421=CARTESIAN_POINT ( 'NONE',  ( -21.37693747720000204, 1440.913060387330006, 224.8635562088979896 ) ) ;
#69422=CARTESIAN_POINT ( 'NONE',  ( 10.62380629660010101, 1475.245810864669011, 266.9323113450542451 ) ) ;
#69423=CARTESIAN_POINT ( 'NONE',  ( 11.69923102470000131, 1433.280222705429878, 150.9071057001980023 ) ) ;
#69424=CARTESIAN_POINT ( 'NONE',  ( 19.62446893450000118, 1440.913060387330006, 214.3676144200779845 ) ) ;
#69429=CARTESIAN_POINT ( 'NONE',  ( -5.797154954569999852, 1485.993502122029895, 182.5750687759980337 ) ) ;
#69430=CARTESIAN_POINT ( 'NONE',  ( 11.17483157899774859, 1398.244322891364391, 215.7730490302998874 ) ) ;
#69432=CIRCLE ( 'NONE', #1478, 95.87906057922711511 ) ;
#69433=CARTESIAN_POINT ( 'NONE',  ( 24.57539793370000325, 1430.358747812230149, 211.0346440933479926 ) ) ;
#69434=CARTESIAN_POINT ( 'NONE',  ( 4.222531898828509433, 1446.229786520979815, 170.5365406785500113 ) ) ;
#69435=CARTESIAN_POINT ( 'NONE',  ( 25.73763176173297396, 1436.650863761621849, 137.0965057394066378 ) ) ;
#69440=CARTESIAN_POINT ( 'NONE',  ( 0.1651937675056289745, 1483.163554816820124, 181.9584872145249790 ) ) ;
#69441=DIRECTION ( 'NONE',  ( 0.000000000000000000, 1.000000000000000000, 0.000000000000000000 ) ) ;
#69443=CARTESIAN_POINT ( 'NONE',  ( -18.29245442332561566, 1445.052233488289403, 161.2175811807110506 ) ) ;
#69452=CARTESIAN_POINT ( 'NONE',  ( -13.83520620040000004, 1414.913060387329779, 218.3795407500680312 ) ) ;
#69453=CARTESIAN_POINT ( 'NONE',  ( 11.60004869885205459, 1426.267709371766387, 138.3562380925339994 ) ) ;
#69455=EDGE_CURVE ( 'NONE', #99393, #80494, #103696, .T. ) ;
#69462=CARTESIAN_POINT ( 'NONE',  ( -17.70224057689999952, 1414.004052165529856, 192.9401193470979763 ) ) ;
#69464=ORIENTED_EDGE ( 'NONE', *, *, #80331, .F. ) ;
#69465=CARTESIAN_POINT ( 'NONE',  ( 13.31869796660000027, 1443.086052842849995, 169.3753098992980028 ) ) ;
#69467=EDGE_LOOP ( 'NONE', ( #88392, #52316, #64366, #73703 ) ) ;
#69473=EDGE_CURVE ( 'NONE', #32914, #51052, #71490, .T. ) ;
#69474=CARTESIAN_POINT ( 'NONE',  ( 30.77169378701360003, 1461.664014259019268, 269.4792440743883617 ) ) ;
#69476=CARTESIAN_POINT ( 'NONE',  ( 18.74698803448425366, 1436.847809687247036, 213.8123656996561408 ) ) ;
#69484=CARTESIAN_POINT ( 'NONE',  ( -0.0002840614181677549835, 1443.913060387330006, 126.7977857662820043 ) ) ;
#69486=CIRCLE ( 'NONE', #74913, 2.000000020766222075 ) ;
#69488=EDGE_LOOP ( 'NONE', ( #79024, #38493, #83748, #67282, #6622 ) ) ;
#69490=ORIENTED_EDGE ( 'NONE', *, *, #80331, .T. ) ;
#69492=CARTESIAN_POINT ( 'NONE',  ( 30.10637292080000194, 1413.645514435030009, 266.8104572860979715 ) ) ;
#69493=CARTESIAN_POINT ( 'NONE',  ( -24.75581127569999751, 1430.360917255730101, 207.9708729454779927 ) ) ;
#69494=CARTESIAN_POINT ( 'NONE',  ( -11.30596056951389983, 1425.565231672570008, 135.2551855802589955 ) ) ;
#69495=CARTESIAN_POINT ( 'NONE',  ( 16.16892249492000033, 1409.485760428959793, 192.9099775984909968 ) ) ;
#69497=CARTESIAN_POINT ( 'NONE',  ( 29.03576926601821029, 1510.037895104773270, 201.5770025554943459 ) ) ;
#69498=CARTESIAN_POINT ( 'NONE',  ( -22.95227133490000071, 1507.624369720630057, 208.0069050751279747 ) ) ;
#69499=CARTESIAN_POINT ( 'NONE',  ( -43.15848075010000429, 1435.559015939599931, 263.9122388061979905 ) ) ;
#69500=CARTESIAN_POINT ( 'NONE',  ( 19.18955701931950131, 1509.607256104009821, 231.7035876696010064 ) ) ;
#69501=CARTESIAN_POINT ( 'NONE',  ( 17.39313975581298521, 1460.068489132931745, 228.4728633170865351 ) ) ;
#69504=CARTESIAN_POINT ( 'NONE',  ( -37.00411130546480365, 1437.912636928700067, 136.5589373068169721 ) ) ;
#69506=CARTESIAN_POINT ( 'NONE',  ( 11.64773666870840074, 1396.497100933559750, 213.5793525411820042 ) ) ;
#69509=CARTESIAN_POINT ( 'NONE',  ( -17.59666625160000208, 1458.100482827429914, 230.0625289195980088 ) ) ;
#69510=ORIENTED_EDGE ( 'NONE', *, *, #65971, .F. ) ;
#69512=CARTESIAN_POINT ( 'NONE',  ( -2.446787376320000096, 1432.353341358199941, 150.2884730787980061 ) ) ;
#69513=CARTESIAN_POINT ( 'NONE',  ( -11.81421925085510161, 1428.091866732929930, 150.2203729037190101 ) ) ;
#69516=CARTESIAN_POINT ( 'NONE',  ( 0.2232360794380000291, 1421.820066533229920, 227.4074839354979929 ) ) ;
#69521=CARTESIAN_POINT ( 'NONE',  ( 27.44229968044188439, 1509.334241250234754, 206.1596417527201197 ) ) ;
#69522=CARTESIAN_POINT ( 'NONE',  ( 1.597238071469150089, 1420.983502555679934, 183.0619176556710102 ) ) ;
#69530=CARTESIAN_POINT ( 'NONE',  ( 11.86506748840099945, 1432.263814426909903, 149.9818949723999992 ) ) ;
#69534=CARTESIAN_POINT ( 'NONE',  ( -17.22623662315568893, 1443.501467202830781, 162.9225832754749490 ) ) ;
#69535=CARTESIAN_POINT ( 'NONE',  ( 11.24596261149999954, 1509.248420230330112, 235.4555975505980143 ) ) ;
#69537=CARTESIAN_POINT ( 'NONE',  ( -5.273497523000000520, 1420.712481594430074, 186.5671558910979968 ) ) ;
#69538=CARTESIAN_POINT ( 'NONE',  ( 3.549205703259999733, 1408.030536462830014, 270.2903253923980174 ) ) ;
#69543=CARTESIAN_POINT ( 'NONE',  ( -3.500000000000000000, 1409.663060387330006, 146.1721969590979882 ) ) ;
#69546=CARTESIAN_POINT ( 'NONE',  ( -4.619247800516277813, 1423.719106761370995, 184.4314750194308488 ) ) ;
#69547=CARTESIAN_POINT ( 'NONE',  ( 17.68653785626990071, 1413.495428231110054, 224.8840759871750095 ) ) ;
#69548=EDGE_CURVE ( 'NONE', #43965, #75409, #97143, .T. ) ;
#69551=CARTESIAN_POINT ( 'NONE',  ( 18.02578551396119977, 1424.483936704789812, 224.5809757487189984 ) ) ;
#69554=CARTESIAN_POINT ( 'NONE',  ( -2.983004277789705228, 1485.615614723739100, 182.7116838820144267 ) ) ;
#69560=CARTESIAN_POINT ( 'NONE',  ( -2.446787376320000096, 1432.353341358199941, 150.2884730787980061 ) ) ;
#69561=B_SPLINE_CURVE_WITH_KNOTS ( 'NONE', 5,
 ( #87089, #28287, #2009, #36689, #19310, #17645 ),
 .UNSPECIFIED., .F., .F.,
 ( 6, 6 ),
 ( -22.82719364450599997, -6.734755223259998758 ),
 .UNSPECIFIED. ) ;
#69562=CARTESIAN_POINT ( 'NONE',  ( -11.54804583780000193, 1430.179206417029945, 150.8480334790980066 ) ) ;
#69563=CARTESIAN_POINT ( 'NONE',  ( -10.96946876072200006, 1432.347663854339999, 151.7701362700559855 ) ) ;
#69565=CARTESIAN_POINT ( 'NONE',  ( 1.190307662709999936E-15, 1432.413060387330006, 146.1721969590979882 ) ) ;
#69568=CARTESIAN_POINT ( 'NONE',  ( 16.49337488880000180, 1410.410615523229808, 226.5881202531979852 ) ) ;
#69570=CARTESIAN_POINT ( 'NONE',  ( -16.61244015609999991, 1459.967035441530015, 228.4924331886979871 ) ) ;
#69573=CARTESIAN_POINT ( 'NONE',  ( 35.72701205430000471, 1418.844138006729963, 266.4694652101980523 ) ) ;
#69574=CARTESIAN_POINT ( 'NONE',  ( 22.68396052030000121, 1435.289475021379985, 139.2169948456979967 ) ) ;
#69575=CIRCLE ( 'NONE', #6866, 27.48039236454309275 ) ;
#69576=CARTESIAN_POINT ( 'NONE',  ( 23.44272364520000096, 1430.296227159529963, 206.5262785095279696 ) ) ;
#69577=CARTESIAN_POINT ( 'NONE',  ( -22.43751286540000223, 1431.503785808020211, 216.9270791274780095 ) ) ;
#69578=CIRCLE ( 'NONE', #21222, 28.99999999999999645 ) ;
#69579=DIRECTION ( 'NONE',  ( -0.7074300732239336975, -0.02470400246746228684, -0.7063514732485997039 ) ) ;
#69580=CARTESIAN_POINT ( 'NONE',  ( 3.827327205999999649, 1409.546157813730133, 126.8043280305979863 ) ) ;
#69581=CARTESIAN_POINT ( 'NONE',  ( -1.464544818259999825, 1451.650746978230018, 183.9079519998980174 ) ) ;
#69582=DIRECTION ( 'NONE',  ( 0.02307773700814929468, -0.7475172611785151355, -0.6638413683213441052 ) ) ;
#69584=CARTESIAN_POINT ( 'NONE',  ( -12.28185623160000084, 1441.208366488439879, 187.9047578019979881 ) ) ;
#69585=CARTESIAN_POINT ( 'NONE',  ( -15.29461995089999959, 1453.313060387329870, 223.0352892562980003 ) ) ;
#69586=CARTESIAN_POINT ( 'NONE',  ( -30.20925992649999969, 1436.447313216129942, 136.6262449664980068 ) ) ;
#69587=CARTESIAN_POINT ( 'NONE',  ( -8.178650747341842830, 1456.230684632761040, 227.1998168167369840 ) ) ;
#69588=ORIENTED_EDGE ( 'NONE', *, *, #58846, .F. ) ;
#69590=CARTESIAN_POINT ( 'NONE',  ( -14.20386470660680089, 1409.409070272629833, 204.4985088955900210 ) ) ;
#69593=CARTESIAN_POINT ( 'NONE',  ( -21.24668275234344250, 1409.655010898162118, 211.0876053273857735 ) ) ;
#69594=CARTESIAN_POINT ( 'NONE',  ( -21.91923426869999858, 1471.782736223630081, 267.0360668916979989 ) ) ;
#69596=CARTESIAN_POINT ( 'NONE',  ( 0.2081566899150210093, 1419.757203975580069, 184.2452808931809898 ) ) ;
#69597=CARTESIAN_POINT ( 'NONE',  ( -24.19977663905823562, 1444.537531331827950, 211.5031488161932032 ) ) ;
#69600=CARTESIAN_POINT ( 'NONE',  ( 16.82531969527569871, 1423.253125815850126, 227.2938718802809888 ) ) ;
#69601=CARTESIAN_POINT ( 'NONE',  ( 14.59411311889999929, 1414.913060387329779, 216.7687570508280146 ) ) ;
#69602=CARTESIAN_POINT ( 'NONE',  ( -28.25086642335310216, 1508.135711581739997, 208.8579954535609886 ) ) ;
#69607=CARTESIAN_POINT ( 'NONE',  ( -22.72436476140000039, 1409.706612691029704, 207.2124451185780174 ) ) ;
#69608=FACE_OUTER_BOUND ( 'NONE', #58943, .T. ) ;
#69611=CARTESIAN_POINT ( 'NONE',  ( 0.8182520991989999937, 1433.447543843880112, 150.4377610267980003 ) ) ;
#69620=CARTESIAN_POINT ( 'NONE',  ( -22.98095509850000084, 1420.941332502029809, 212.0408358815379870 ) ) ;
#69626=CARTESIAN_POINT ( 'NONE',  ( -17.84734352359999932, 1410.892954231429940, 195.0519780797979763 ) ) ;
#69628=AXIS2_PLACEMENT_3D ( 'NONE', #102662, #25405, #17555 ) ;
#69629=CARTESIAN_POINT ( 'NONE',  ( 38.26972034215779672, 1449.715126992240130, 136.0601146782780120 ) ) ;
#69633=CARTESIAN_POINT ( 'NONE',  ( 11.94173468258579973, 1433.516563288440011, 150.0939282449400025 ) ) ;
#69635=ORIENTED_EDGE ( 'NONE', *, *, #71060, .T. ) ;
#69639=CARTESIAN_POINT ( 'NONE',  ( 16.08972158192780100, 1424.754442430379868, 191.0877091364910143 ) ) ;
#69640=CARTESIAN_POINT ( 'NONE',  ( 9.253402716490001012, 1428.330636036430178, 123.0297916884979941 ) ) ;
#69641=CARTESIAN_POINT ( 'NONE',  ( 19.21540365814130169, 1507.816561716200113, 229.6838698100480087 ) ) ;
#69643=CARTESIAN_POINT ( 'NONE',  ( 3.826470069039999977, 1488.170811478430096, 182.4750432301979970 ) ) ;
#69645=CARTESIAN_POINT ( 'NONE',  ( 16.57640676229999954, 1409.993768047430194, 226.3203803305979704 ) ) ;
#69647=B_SPLINE_SURFACE_WITH_KNOTS ( 'NONE', 5, 5, ( 
 ( #84766, #33265, #84221, #41120, #101010, #34382 ),
 ( #50635, #24309, #68555, #75299, #8064, #110531 ),
 ( #9187, #60150, #51749, #42234, #50094, #75839 ),
 ( #76382, #77497, #33816, #25399, #94841, #51185 ),
 ( #85314, #68010, #16985, #69113, #83669, #102120 ),
 ( #59592, #43349, #85884, #109443, #32723, #18117 ),
 ( #797, #58490, #25955, #17547, #8609, #66903 ),
 ( #59049, #67454, #102655, #6966, #15894, #41679 ),
 ( #92617, #7520, #101554, #24846, #93170, #16440 ),
 ( #42786, #34926, #76946, #94271, #103214, #26522 ),
 ( #60719, #97604, #20325, #95399, #53409, #28744 ),
 ( #54530, #45573, #96501, #1344, #104900, #18662 ),
 ( #45021, #3570, #37144, #71341, #19207, #37694 ),
 ( #79715, #103799, #27639, #52861, #63485, #70788 ),
 ( #19781, #78598, #2474, #28189, #1916, #35483 ),
 ( #29289, #86988, #11942, #71897, #10277, #62375 ),
 ( #44454, #43892, #27098, #95947, #87560, #70239 ),
 ( #53982, #46123, #52313, #78036, #10849, #104346 ),
 ( #105455, #3022, #62949, #97060, #88116, #79166 ),
 ( #36052, #9727, #61824, #88664, #61283, #36591 ),
 ( #11405, #80252, #106013, #69677, #86436, #98136 ),
 ( #65113, #99224, #108748, #108192, #99779, #21953 ),
 ( #12489, #40437, #56146, #90282, #98693, #106549 ),
 ( #55621, #46672, #80804, #107095, #38234, #29837 ),
 ( #81329, #5187, #13563, #4644, #39342, #4110 ),
 ( #23071, #64023, #47749, #31481, #89197, #22502 ),
 ( #20874, #81884, #21412, #56703, #90839, #14124 ) ),
 .UNSPECIFIED., .F., .F., .F.,
 ( 6, 3, 3, 3, 3, 3, 3, 3, 6 ),
 ( 6, 6 ),
 ( 10.40199318109999993, 19.90315615969999996, 23.28476991740000202, 24.97557679630000038, 25.82098023580000046, 26.66638367519999875, 26.99360131220000270, 28.03535140669999848, 29.40431913829999999 ),
 ( 0.000000000000000000, 1.455169987240000129 ),
 .UNSPECIFIED. ) ;
#69649=CARTESIAN_POINT ( 'NONE',  ( 14.17422268772769911, 1415.724942525210054, 197.1424870051829998 ) ) ;
#69652=ORIENTED_EDGE ( 'NONE', *, *, #28887, .F. ) ;
#69653=CARTESIAN_POINT ( 'NONE',  ( 14.19348081423260055, 1435.301921962149891, 149.4341381306140022 ) ) ;
#69655=ORIENTED_EDGE ( 'NONE', *, *, #94079, .T. ) ;
#69656=ORIENTED_EDGE ( 'NONE', *, *, #40545, .F. ) ;
#69658=DIRECTION ( 'NONE',  ( 0.000000000000000000, -0.7071067811865474617, -0.7071067811865474617 ) ) ;
#69665=CARTESIAN_POINT ( 'NONE',  ( 4.265655661611780225, 1446.644466445230137, 158.6693615694720165 ) ) ;
#69666=EDGE_CURVE ( 'NONE', #104566, #18861, #90042, .T. ) ;
#69668=CARTESIAN_POINT ( 'NONE',  ( 0.6067091484059999873, 1507.391323370129840, 237.3179893959980120 ) ) ;
#69673=CARTESIAN_POINT ( 'NONE',  ( -19.35070331030000190, 1509.010601545330019, 230.0701437765980018 ) ) ;
#69676=EDGE_CURVE ( 'NONE', #66886, #75744, #88690, .T. ) ;
#69677=CARTESIAN_POINT ( 'NONE',  ( -15.29119482810000008, 1409.948801712029990, 191.1498944753979856 ) ) ;
#69678=CARTESIAN_POINT ( 'NONE',  ( -24.49292865060000324, 1441.580045819019915, 211.0188571790179992 ) ) ;
#69681=DIRECTION ( 'NONE',  ( -0.4632728134665660691, -0.8857936774813760517, -0.02734705170200765062 ) ) ;
#69684=CARTESIAN_POINT ( 'NONE',  ( -24.04659120089169733, 1444.796772349889807, 212.0316830080810178 ) ) ;
#69685=CARTESIAN_POINT ( 'NONE',  ( 0.3722769099684289928, 1457.826255237599980, 228.9731060096619899 ) ) ;
#69689=CARTESIAN_POINT ( 'NONE',  ( 24.02347744240000083, 1410.714002832030019, 209.6150577782879907 ) ) ;
#69691=CARTESIAN_POINT ( 'NONE',  ( 28.83249087089999918, 1509.587594255930071, 208.9222957011619997 ) ) ;
#69697=VERTEX_POINT ( 'NONE', #82764 ) ;
#69698=AXIS2_PLACEMENT_3D ( 'NONE', #42161, #25884, #76313 ) ;
#69699=CARTESIAN_POINT ( 'NONE',  ( 26.00754374179999928, 1454.033399689230009, 240.2274373035980091 ) ) ;
#69702=CARTESIAN_POINT ( 'NONE',  ( -7.988150404321079812, 1508.679516143240107, 235.8900466699099923 ) ) ;
#69703=CARTESIAN_POINT ( 'NONE',  ( -18.92998585080000140, 1456.923645639730012, 227.1748017144979883 ) ) ;
#69704=CARTESIAN_POINT ( 'NONE',  ( 11.86547437279999961, 1432.299053485889999, 150.3973020406980083 ) ) ;
#69705=CARTESIAN_POINT ( 'NONE',  ( 17.79684371365149786, 1410.125370365290109, 222.8164932182040161 ) ) ;
#69706=CARTESIAN_POINT ( 'NONE',  ( -0.3753211829319999526, 1470.816980702529918, 188.7016457681980057 ) ) ;
#69710=CARTESIAN_POINT ( 'NONE',  ( 0.2126091594639999971, 1406.777959006730043, 269.6500587044980648 ) ) ;
#69711=CARTESIAN_POINT ( 'NONE',  ( 28.73878200240000069, 1509.916640768729849, 206.8280204061180143 ) ) ;
#69712=CARTESIAN_POINT ( 'NONE',  ( 12.45702690739999952, 1416.837177099529754, 223.4766769987980126 ) ) ;
#69713=CARTESIAN_POINT ( 'NONE',  ( 2.478650075360000038, 1436.419591246580012, 157.6446810035980093 ) ) ;
#69714=( BOUNDED_CURVE ( )  B_SPLINE_CURVE ( 3, ( #98010, #72835, #65544, #108065 ),
 .UNSPECIFIED., .F., .T. ) 
 B_SPLINE_CURVE_WITH_KNOTS ( ( 4, 4 ),
 ( 4.212388980384758952, 4.712388980384758952 ),
 .UNSPECIFIED. ) 
 CURVE ( )  GEOMETRIC_REPRESENTATION_ITEM ( )  RATIONAL_B_SPLINE_CURVE ( ( 1.000000000000000000, 0.9792749478070963409, 0.9792749478070963409, 1.000000000000000000 ) ) 
 REPRESENTATION_ITEM ( '' )  );
#69717=CARTESIAN_POINT ( 'NONE',  ( -41.89974302683250329, 1440.913060410779963, 261.8273974356069971 ) ) ;
#69719=CARTESIAN_POINT ( 'NONE',  ( -25.71518287839999672, 1448.115169621710038, 138.0481613422979876 ) ) ;
#69720=CARTESIAN_POINT ( 'NONE',  ( 28.84710513917680075, 1507.919203931609900, 206.0039949767749761 ) ) ;
#69724=CARTESIAN_POINT ( 'NONE',  ( -38.87775330991500766, 1452.503265736994535, 269.5910503552404975 ) ) ;
#69727=B_SPLINE_CURVE_WITH_KNOTS ( 'NONE', 5,
 ( #101861, #553, #40873, #67751, #24595, #100235, #93466, #25155, #59358 ),
 .UNSPECIFIED., .F., .F.,
 ( 6, 3, 6 ),
 ( -157.7108139780000045, -153.2961530439999933, -140.3375013407610084 ),
 .UNSPECIFIED. ) ;
#69730=CARTESIAN_POINT ( 'NONE',  ( -0.3788211479479999810, 1416.124142285029848, 233.5244129845979728 ) ) ;
#69736=CARTESIAN_POINT ( 'NONE',  ( -17.85311748929999709, 1415.140114704729967, 207.6665950678980153 ) ) ;
#69739=CARTESIAN_POINT ( 'NONE',  ( -10.47578755381780091, 1396.278882950810157, 205.5458655290329943 ) ) ;
#69741=CARTESIAN_POINT ( 'NONE',  ( -16.35908613486439833, 1409.492693367569927, 225.1152296089470042 ) ) ;
#69742=CARTESIAN_POINT ( 'NONE',  ( 7.333237907140000900, 1433.447543843880112, 149.5704065546979962 ) ) ;
#69745=CARTESIAN_POINT ( 'NONE',  ( -20.59684415639999955, 1507.762623716630060, 208.9176257130860108 ) ) ;
#69747=CARTESIAN_POINT ( 'NONE',  ( 10.88730574250000060, 1426.101986003629918, 91.15062687669779962 ) ) ;
#69750=CARTESIAN_POINT ( 'NONE',  ( -11.46220264589999971, 1433.073555843209988, 151.3007702552979765 ) ) ;
#69752=CARTESIAN_POINT ( 'NONE',  ( -2.866286648406546345, 1419.680164975547541, 186.1825321117389933 ) ) ;
#69756=CARTESIAN_POINT ( 'NONE',  ( 7.466351093540000150, 1508.652853213030085, 182.1636783160980144 ) ) ;
#69757=CARTESIAN_POINT ( 'NONE',  ( 2.500000726750000180, 1448.905931065010009, 182.6097889574979831 ) ) ;
#69758=B_SPLINE_SURFACE_WITH_KNOTS ( 'NONE', 5, 5, ( 
 ( #59325, #32450, #50369, #75570, #101264, #109703, #49261, #92891, #6685, #100197, #24563, #84495, #50907, #91243, #100727, #91786, #7785, #16705, #41951, #48713, #22909 ),
 ( #6127, #33517, #40283, #108597, #31885, #92333, #110243, #24011, #66072, #23480, #40840, #15605, #44731, #18375, #60985, #59867, #94540, #103495, #17259, #68830, #62091 ),
 ( #95110, #77219, #51450, #17814, #34646, #43060, #86155, #52570, #521, #8878, #45283, #85583, #86704, #95661, #9997, #27347, #87836, #70495, #9446, #93994, #53695 ),
 ( #104613, #18928, #102392, #52013, #61532, #69941, #27907, #1070, #102931, #44168, #36855, #43611, #77761, #11124, #53126, #96216, #78305, #1621, #25675, #87263, #35757 ),
 ( #78881, #35198, #10557, #79424, #69385, #19492, #104055, #2185, #26797, #36300, #26234, #2734, #60423, #106804, #98954, #21680, #38502, #81597, #105734, #97851, #105171 ),
 ( #37415, #48021, #54780, #20047, #30660, #71614, #12759, #106267, #13283, #55332, #90006, #13836, #96777, #29553, #55887, #21126, #29018, #3840, #82158, #71048, #54242 ) ),
 .UNSPECIFIED., .F., .F., .F.,
 ( 6, 6 ),
 ( 6, 3, 3, 3, 3, 3, 6 ),
 ( 2.177956466309999950, 27.10020543639999957 ),
 ( 27.90569345569999982, 34.29022120999999856, 36.66164856079999623, 37.84736223619999862, 39.03307591160000101, 39.85391243800000183, 40.67474896430000086 ),
 .UNSPECIFIED. ) ;
#69761=ORIENTED_EDGE ( 'NONE', *, *, #97339, .T. ) ;
#69763=CARTESIAN_POINT ( 'NONE',  ( -41.14066536589999856, 1444.183253557760054, 136.8991340996980171 ) ) ;
#69765=CARTESIAN_POINT ( 'NONE',  ( -0.9556612664140000657, 1472.040204376429983, 270.0714134045979904 ) ) ;
#69767=CARTESIAN_POINT ( 'NONE',  ( -0.9862637779436296270, 1410.322815402584638, 185.2948817930962662 ) ) ;
#69770=CARTESIAN_POINT ( 'NONE',  ( -33.93389154554730425, 1451.270658457710169, 135.9469627738999975 ) ) ;
#69772=CARTESIAN_POINT ( 'NONE',  ( -2.500000000000000000, 1448.210448412289907, 170.5244215879980061 ) ) ;
#69774=CARTESIAN_POINT ( 'NONE',  ( 12.31782521489999915, 1408.309306176930022, 215.8722587012880183 ) ) ;
#69775=CARTESIAN_POINT ( 'NONE',  ( -1.532158170363220107, 1405.788062017090169, 268.4831340189729758 ) ) ;
#69776=CARTESIAN_POINT ( 'NONE',  ( -13.71232569032570048, 1434.975555795949958, 148.7451008170540092 ) ) ;
#69778=CARTESIAN_POINT ( 'NONE',  ( -11.86529746090000081, 1432.285507951989985, 150.3971901167980150 ) ) ;
#69779=CARTESIAN_POINT ( 'NONE',  ( 13.52955335139999882, 1444.423027347819925, 188.5011656169979801 ) ) ;
#69786=ORIENTED_EDGE ( 'NONE', *, *, #37831, .F. ) ;
#69788=CARTESIAN_POINT ( 'NONE',  ( 11.60080558210000135, 1414.971439108430104, 222.3644924952979807 ) ) ;
#69791=CARTESIAN_POINT ( 'NONE',  ( -28.52408420809999967, 1509.909458608030263, 201.9849479314579810 ) ) ;
#69793=CARTESIAN_POINT ( 'NONE',  ( -1.114940899219999837, 1507.624369749730022, 232.0741173169980129 ) ) ;
#69794=CARTESIAN_POINT ( 'NONE',  ( -41.29476677764731818, 1435.144711064243438, 269.6341300601254147 ) ) ;
#69797=CARTESIAN_POINT ( 'NONE',  ( -24.91457825792770109, 1430.518871130359912, 208.6748305930140077 ) ) ;
#69798=AXIS2_PLACEMENT_3D ( 'NONE', #53647, #27867, #44127 ) ;
#69799=CARTESIAN_POINT ( 'NONE',  ( -5.865704164809999455, 1445.996979593550122, 183.7573955461979835 ) ) ;
#69800=ORIENTED_EDGE ( 'NONE', *, *, #52901, .F. ) ;
#69801=CARTESIAN_POINT ( 'NONE',  ( 33.91369968912619726, 1451.728767897860052, 134.7155302171979940 ) ) ;
#69802=CARTESIAN_POINT ( 'NONE',  ( -24.41186848580399982, 1440.913060429360030, 212.0284777848129920 ) ) ;
#69803=CARTESIAN_POINT ( 'NONE',  ( 19.65495273042400370, 1477.253990450800075, 226.3277939041599893 ) ) ;
#69804=CARTESIAN_POINT ( 'NONE',  ( -25.30535122030000039, 1436.307508284910227, 137.3140542664980046 ) ) ;
#69808=B_SPLINE_CURVE_WITH_KNOTS ( 'NONE', 3,
 ( #4334, #39005, #21644, #38465, #73182, #37934, #100016, #22737, #89428, #55851, #31160, #12164, #56387, #106767, #54749, #13245, #46902, #22189, #47979, #82118, #5972, #48544, #89971, #56941, #81025, #4860, #40117, #106229, #64249, #98372, #82682, #65899, #65351, #81559, #29513, #72114, #91069, #88879, #107328, #3802, #46354, #80485, #63705, #99459, #5419, #64810 ),
 .UNSPECIFIED., .F., .F.,
 ( 4, 3, 3, 3, 3, 3, 3, 3, 3, 3, 3, 3, 3, 3, 3, 4 ),
 ( -2.000000000000000000, -1.940228845006789937, -1.806436809266960042, -1.670720477943769877, -1.533764895268459938, -1.394888271458489815, -1.254958854399230050, -1.114243059651710110, -0.9730594466478950100, -0.8263536533118798211, -0.6856755233809810335, -0.5458629076362540022, -0.4072070084870209605, -0.2699245238820009440, -0.1341607992937359217, 0.000000000000000000 ),
 .UNSPECIFIED. ) ;
#69809=CARTESIAN_POINT ( 'NONE',  ( -14.69695073940000007, 1415.591872390730032, 226.9139971760980075 ) ) ;
#69810=PLANE ( 'NONE',  #28868 ) ;
#69813=VERTEX_POINT ( 'NONE', #6056 ) ;
#69814=CARTESIAN_POINT ( 'NONE',  ( 2.500000000000000000, 1439.002693873140061, 157.7215435580980056 ) ) ;
#69815=CARTESIAN_POINT ( 'NONE',  ( -3.621823104480000222, 1410.301613452430047, 232.3323923370979855 ) ) ;
#69819=DIRECTION ( 'NONE',  ( 0.000000000000000000, -1.000000000000000000, 0.000000000000000000 ) ) ;
#69820=CARTESIAN_POINT ( 'NONE',  ( 12.11419479737319804, 1434.101768081229920, 150.3426090226449787 ) ) ;
#69821=CARTESIAN_POINT ( 'NONE',  ( 15.93672166378249777, 1469.005798317469953, 229.8246201197470100 ) ) ;
#69822=CARTESIAN_POINT ( 'NONE',  ( -23.28153440269690222, 1507.876989814209992, 223.8845409149209900 ) ) ;
#69823=CARTESIAN_POINT ( 'NONE',  ( -1.984533605359999564, 1410.356878505129998, 186.2308698998980105 ) ) ;
#69824=CARTESIAN_POINT ( 'NONE',  ( 0.1600673621120000112, 1410.295025425230051, 233.2191648330980058 ) ) ;
#69825=CARTESIAN_POINT ( 'NONE',  ( -13.58268883541719951, 1416.851343898680170, 221.9096085506480165 ) ) ;
#69828=CARTESIAN_POINT ( 'NONE',  ( -4.363122371700000279, 1421.971318377230091, 184.5104922129979741 ) ) ;
#69829=CARTESIAN_POINT ( 'NONE',  ( 19.21159273369999809, 1509.355098208629897, 187.6258791606980196 ) ) ;
#69832=CARTESIAN_POINT ( 'NONE',  ( -12.18581614772419996, 1415.088012641449950, 197.3189512858170076 ) ) ;
#69834=VERTEX_POINT ( 'NONE', #50289 ) ;
#69835=CARTESIAN_POINT ( 'NONE',  ( 0.2612772751870610088, 1416.851343895820037, 190.7759414009450154 ) ) ;
#69839=B_SPLINE_CURVE_WITH_KNOTS ( 'NONE', 3,
 ( #31275, #97377, #40228, #74411, #20649, #54851 ),
 .UNSPECIFIED., .F., .F.,
 ( 4, 2, 4 ),
 ( -0.1904887807602000105, -0.09529849760486289179, -1.010125272010720110E-06 ),
 .UNSPECIFIED. ) ;
#69841=CARTESIAN_POINT ( 'NONE',  ( 17.83233393729999960, 1415.128105759529944, 210.4741431536880043 ) ) ;
#69842=CARTESIAN_POINT ( 'NONE',  ( -18.78018960140000360, 1425.453421275130040, 226.8344281414980230 ) ) ;
#69843=CARTESIAN_POINT ( 'NONE',  ( -21.31715047099999794, 1436.055628343680155, 143.9063927194979726 ) ) ;
#69844=CARTESIAN_POINT ( 'NONE',  ( -11.97724519069999971, 1441.600846913620217, 147.6096801420980000 ) ) ;
#69848=CARTESIAN_POINT ( 'NONE',  ( 11.81532904971749254, 1433.677431381189763, 150.7649965429154406 ) ) ;
#69850=CARTESIAN_POINT ( 'NONE',  ( 12.91878488757420129, 1430.070686061380002, 195.6857951094069961 ) ) ;
#69852=CARTESIAN_POINT ( 'NONE',  ( -11.90002773584334683, 1434.916176828660127, 147.6452132258590382 ) ) ;
#69853=CARTESIAN_POINT ( 'NONE',  ( 13.86092937120069912, 1410.765486813650114, 191.1266627561969926 ) ) ;
#69858=CARTESIAN_POINT ( 'NONE',  ( 13.40958072579999971, 1414.996442553730049, 197.9133052342980079 ) ) ;
#69860=EDGE_CURVE ( 'NONE', #91513, #85568, #7703, .T. ) ;
#69862=CARTESIAN_POINT ( 'NONE',  ( -7.628773448420000491, 1416.913060387330006, 216.7506196533379921 ) ) ;
#69863=PLANE ( 'NONE',  #82189 ) ;
#69865=CARTESIAN_POINT ( 'NONE',  ( 22.98967036120000174, 1508.444085606630097, 193.7320087538980147 ) ) ;
#69867=CARTESIAN_POINT ( 'NONE',  ( -1.547463840030000037, 1414.913060387329779, 225.9340782259980074 ) ) ;
#69872=ORIENTED_EDGE ( 'NONE', *, *, #55761, .F. ) ;
#69873=ORIENTED_EDGE ( 'NONE', *, *, #9305, .T. ) ;
#69874=CARTESIAN_POINT ( 'NONE',  ( 33.91369120165509798, 1451.728768194249824, 134.0999999980979851 ) ) ;
#69876=CARTESIAN_POINT ( 'NONE',  ( 40.26850195192459836, 1443.374941825310088, 137.0885199844659894 ) ) ;
#69877=CARTESIAN_POINT ( 'NONE',  ( 21.25073931209999856, 1488.812149332829904, 209.0329839582499858 ) ) ;
#69878=CARTESIAN_POINT ( 'NONE',  ( -18.32011812489999869, 1469.450906033330057, 259.8063372729980074 ) ) ;
#69881=CARTESIAN_POINT ( 'NONE',  ( 24.93047652359999944, 1508.532778672029963, 197.8716724273980105 ) ) ;
#69882=CARTESIAN_POINT ( 'NONE',  ( -20.45667992530000134, 1485.851243504329886, 191.2933074961979969 ) ) ;
#69883=CARTESIAN_POINT ( 'NONE',  ( 2.104012799200000394, 1408.986534133630130, 186.4985688927979766 ) ) ;
#69884=CARTESIAN_POINT ( 'NONE',  ( 6.313072733930000346, 1422.316561012229840, 186.3238498068980107 ) ) ;
#69885=CARTESIAN_POINT ( 'NONE',  ( -11.83477905770000049, 1434.684743416989932, 151.1661213938980097 ) ) ;
#69892=CARTESIAN_POINT ( 'NONE',  ( -2.393268998928310687, 1426.806556743500096, 139.9374969045731518 ) ) ;
#69894=CARTESIAN_POINT ( 'NONE',  ( -40.64494809139999631, 1449.406402974629827, 269.6215796247980165 ) ) ;
#69897=CARTESIAN_POINT ( 'NONE',  ( 1.110223024629999949E-15, 1434.541756592460160, 155.4759165859979930 ) ) ;
#69898=B_SPLINE_CURVE_WITH_KNOTS ( 'NONE', 3,
 ( #71116, #37482, #2803, #61598, #10631, #18439, #45899, #52639, #71685, #44238 ),
 .UNSPECIFIED., .F., .F.,
 ( 4, 2, 2, 2, 4 ),
 ( 0.000000000000000000, 0.2500000000000000000, 0.5000000000000000000, 0.7500000000000000000, 1.000000000000000000 ),
 .UNSPECIFIED. ) ;
#69902=CARTESIAN_POINT ( 'NONE',  ( -3.349453590340000009, 1417.674249932829980, 234.8202870076979991 ) ) ;
#69905=CARTESIAN_POINT ( 'NONE',  ( -1.258566612072725688, 1484.609298652428606, 182.2899128876086081 ) ) ;
#69907=CARTESIAN_POINT ( 'NONE',  ( -45.72953638603589610, 1436.732522043369954, 266.6874787479000020 ) ) ;
#69910=CARTESIAN_POINT ( 'NONE',  ( 23.84671661830000033, 1435.330256084430175, 136.8235927701979904 ) ) ;
#69912=VERTEX_POINT ( 'NONE', #61452 ) ;
#69914=TOROIDAL_SURFACE ( 'NONE', #75249, 24.00000000000000000, 1.000000000000000000 ) ;
#69917=CARTESIAN_POINT ( 'NONE',  ( -16.34177352999999755, 1410.409901485429828, 191.5622047604979912 ) ) ;
#69919=VERTEX_POINT ( 'NONE', #95027 ) ;
#69920=CARTESIAN_POINT ( 'NONE',  ( 22.57734580500000021, 1433.084083961730130, 213.0699815576180072 ) ) ;
#69922=CARTESIAN_POINT ( 'NONE',  ( 13.57457166070000021, 1434.814457747740107, 195.7795090784979948 ) ) ;
#69924=CIRCLE ( 'NONE', #66399, 2.000006071546453157 ) ;
#69929=CARTESIAN_POINT ( 'NONE',  ( -1.875969534053839816, 1407.674994227130128, 270.1370502786999737 ) ) ;
#69931=CARTESIAN_POINT ( 'NONE',  ( 7.876066647220000938, 1417.703921191229938, 230.9570592481979929 ) ) ;
#69934=ORIENTED_EDGE ( 'NONE', *, *, #109828, .F. ) ;
#69936=CARTESIAN_POINT ( 'NONE',  ( 13.40958089240390017, 1414.996442620800053, 197.9133050684260127 ) ) ;
#69937=CARTESIAN_POINT ( 'NONE',  ( -0.003606333971295369849, 1409.082051554400095, 185.5805092309179827 ) ) ;
#69938=CARTESIAN_POINT ( 'NONE',  ( 3.664318114120971970, 1425.064796927145153, 184.9869177022372639 ) ) ;
#69940=CARTESIAN_POINT ( 'NONE',  ( -18.51001488987260046, 1427.198549858980186, 194.7363669604100096 ) ) ;
#69941=CARTESIAN_POINT ( 'NONE',  ( -20.83663208060000116, 1425.807880000829982, 220.5952949419979916 ) ) ;
#69942=CARTESIAN_POINT ( 'NONE',  ( 28.54163408408160052, 1468.582989030339832, 267.1922970806700732 ) ) ;
#69944=CARTESIAN_POINT ( 'NONE',  ( 3.887502411549999870, 1447.985170383209834, 184.3007615236979859 ) ) ;
#69947=CARTESIAN_POINT ( 'NONE',  ( -13.62133678120479985, 1452.879579795280051, 223.2680741433150047 ) ) ;
#69949=CARTESIAN_POINT ( 'NONE',  ( 22.86785504970000105, 1409.720132996430038, 208.8870272755499968 ) ) ;
#69952=CARTESIAN_POINT ( 'NONE',  ( 26.21289084844420003, 1451.932721288379980, 135.4906490382789741 ) ) ;
#69953=CARTESIAN_POINT ( 'NONE',  ( -14.77824381598609982, 1473.184986518139794, 194.8749861038550080 ) ) ;
#69956=CARTESIAN_POINT ( 'NONE',  ( 17.56784546119999746, 1409.526543069129957, 195.5982376816980093 ) ) ;
#69958=CARTESIAN_POINT ( 'NONE',  ( 2.500000000000039968, 1439.615672328189930, 182.7715275322960053 ) ) ;
#69959=CARTESIAN_POINT ( 'NONE',  ( 0.2946311075390000145, 1417.347637901529879, 235.5671102051979915 ) ) ;
#69960=CARTESIAN_POINT ( 'NONE',  ( -18.77412637462996159, 1424.630488750686936, 224.5960567574681193 ) ) ;
#69961=CARTESIAN_POINT ( 'NONE',  ( 0.7128917335112240350, 1452.003216656849872, 183.1721099556629895 ) ) ;
#69962=EDGE_CURVE ( 'NONE', #68439, #50075, #44665, .T. ) ;
#69963=CARTESIAN_POINT ( 'NONE',  ( -0.2751659207381170202, 1506.798305148240161, 231.4088083080649767 ) ) ;
#69976=CARTESIAN_POINT ( 'NONE',  ( -28.02005515429999960, 1444.132106999520147, 248.0989693021979861 ) ) ;
#69977=EDGE_CURVE ( 'NONE', #25667, #70841, #82082, .T. ) ;
#69978=CARTESIAN_POINT ( 'NONE',  ( 45.67177335919998171, 1441.839097175249435, 266.1885934058977909 ) ) ;
#69979=CARTESIAN_POINT ( 'NONE',  ( 11.06154325740000033, 1433.015924775339954, 151.7088343760979967 ) ) ;
#69980=CARTESIAN_POINT ( 'NONE',  ( 4.290289619920000241, 1461.407663422529822, 243.9198229428980085 ) ) ;
#69981=CARTESIAN_POINT ( 'NONE',  ( 27.02044944551220240, 1440.913060390540068, 226.9243301018659906 ) ) ;
#69984=CARTESIAN_POINT ( 'NONE',  ( 14.22937790979999839, 1463.546440309030004, 223.7319135734979909 ) ) ;
#69985=CARTESIAN_POINT ( 'NONE',  ( -4.642927288299999233, 1485.993600593529891, 182.3621085484980142 ) ) ;
#69987=CIRCLE ( 'NONE', #3815, 1.999999999999982458 ) ;
#69989=CARTESIAN_POINT ( 'NONE',  ( -28.86589449839050303, 1509.921079635449814, 200.7492878960630094 ) ) ;
#69991=CARTESIAN_POINT ( 'NONE',  ( 25.67898337129999931, 1449.805023455629907, 209.8444692255790187 ) ) ;
#69993=CARTESIAN_POINT ( 'NONE',  ( -38.70772189830101695, 1437.296230298083174, 135.0862444309819921 ) ) ;
#69995=EDGE_CURVE ( 'NONE', #61056, #39980, #104732, .T. ) ;
#69999=EDGE_CURVE ( 'NONE', #107054, #100575, #13876, .T. ) ;
#70002=CARTESIAN_POINT ( 'NONE',  ( 16.11867488194040732, 1414.913060387329779, 209.5777220539784480 ) ) ;
#70006=CARTESIAN_POINT ( 'NONE',  ( -36.91977620350599665, 1451.033275236189866, 134.0999999987079718 ) ) ;
#70012=CARTESIAN_POINT ( 'NONE',  ( -15.47006972390000001, 1415.932617990029939, 219.1087698475380137 ) ) ;
#70015=EDGE_CURVE ( 'NONE', #46489, #98890, #80751, .T. ) ;
#70017=FACE_OUTER_BOUND ( 'NONE', #102470, .T. ) ;
#70018=CARTESIAN_POINT ( 'NONE',  ( 12.67571009042330132, 1409.355705931530110, 217.0370738725129911 ) ) ;
#70021=CARTESIAN_POINT ( 'NONE',  ( -17.81762806769999941, 1417.741547129829996, 192.8330553043980160 ) ) ;
#70024=VECTOR ( 'NONE', #432, 1000.000000000000114 ) ;
#70027=CARTESIAN_POINT ( 'NONE',  ( -1.556099498820364024, 1414.941240534605186, 226.3359606419509760 ) ) ;
#70028=ORIENTED_EDGE ( 'NONE', *, *, #31840, .F. ) ;
#70031=( BOUNDED_CURVE ( )  B_SPLINE_CURVE ( 3, ( #6606, #73830, #31803, #107404 ),
 .UNSPECIFIED., .F., .F. ) 
 B_SPLINE_CURVE_WITH_KNOTS ( ( 4, 4 ),
 ( 6.031750335428980314, 6.430153915118459906 ),
 .UNSPECIFIED. ) 
 CURVE ( )  GEOMETRIC_REPRESENTATION_ITEM ( )  RATIONAL_B_SPLINE_CURVE ( ( 1.000000000000000000, 0.9868165636548378306, 0.9868165636548378306, 1.000000000000000000 ) ) 
 REPRESENTATION_ITEM ( '' )  );
#70032=CARTESIAN_POINT ( 'NONE',  ( 26.37683526749999885, 1508.582706265930028, 216.7137036938680126 ) ) ;
#70035=CARTESIAN_POINT ( 'NONE',  ( 17.16188218510789909, 1468.758169019195520, 269.3744713492412188 ) ) ;
#70037=CARTESIAN_POINT ( 'NONE',  ( 3.841758412219999475, 1398.027797085529983, 221.6465661679980030 ) ) ;
#70040=CARTESIAN_POINT ( 'NONE',  ( -1.443364724160000057, 1457.295863107529840, 183.6403006915980143 ) ) ;
#70043=EDGE_CURVE ( 'NONE', #35617, #56560, #8532, .T. ) ;
#70044=CARTESIAN_POINT ( 'NONE',  ( 3.439931081351653042, 1448.290196154458272, 184.1542931849176910 ) ) ;
#70046=CARTESIAN_POINT ( 'NONE',  ( -13.01309165946850044, 1435.753263066840191, 150.6599531705490165 ) ) ;
#70048=CARTESIAN_POINT ( 'NONE',  ( -7.228663065755881689, 1511.163060387329779, 183.1074954935087646 ) ) ;
#70049=CARTESIAN_POINT ( 'NONE',  ( 13.79555441699999996, 1416.822694190629818, 196.3351662185980047 ) ) ;
#70052=CARTESIAN_POINT ( 'NONE',  ( 40.43746183755959578, 1444.189944152170028, 137.0849278640690159 ) ) ;
#70055=CARTESIAN_POINT ( 'NONE',  ( -27.33420534970000304, 1488.691127167430068, 208.3487218773969971 ) ) ;
#70056=CARTESIAN_POINT ( 'NONE',  ( -10.55446544952580012, 1425.080811231209964, 127.8430071859979762 ) ) ;
#70057=CARTESIAN_POINT ( 'NONE',  ( 16.19082947937390315, 1409.478451820400096, 193.2334330245300009 ) ) ;
#70061=CARTESIAN_POINT ( 'NONE',  ( -12.45246057309999976, 1410.452083772230026, 259.9009997819980526 ) ) ;
#70062=CARTESIAN_POINT ( 'NONE',  ( 18.83404400785749999, 1509.591035207039795, 231.9679584295540167 ) ) ;
#70063=CARTESIAN_POINT ( 'NONE',  ( 28.25550469550829646, 1508.223393718089937, 209.3894320226199852 ) ) ;
#70065=CARTESIAN_POINT ( 'NONE',  ( 32.74960465840000268, 1450.908762451789926, 136.2057699161979940 ) ) ;
#70066=ORIENTED_EDGE ( 'NONE', *, *, #46601, .F. ) ;
#70067=CARTESIAN_POINT ( 'NONE',  ( 6.170308677738740144, 1397.182086642849981, 220.3579607364119681 ) ) ;
#70069=CARTESIAN_POINT ( 'NONE',  ( -17.95620059730000051, 1457.813590052430072, 229.1786308768979836 ) ) ;
#70070=ORIENTED_EDGE ( 'NONE', *, *, #49688, .T. ) ;
#70072=CARTESIAN_POINT ( 'NONE',  ( -2.409586283469999923, 1426.663880916129983, 144.1938086916980239 ) ) ;
#70076=CARTESIAN_POINT ( 'NONE',  ( -0.7199630763800000111, 1415.645607075230146, 184.8796628268980271 ) ) ;
#70077=SPHERICAL_SURFACE ( 'NONE', #67087, 2.000000000000000000 ) ;
#70078=CARTESIAN_POINT ( 'NONE',  ( 3.500000000000000000, 1409.663060387330006, 146.1721969590979882 ) ) ;
#70079=CARTESIAN_POINT ( 'NONE',  ( 27.42787240605195009, 1509.319615610296296, 206.1613560982198692 ) ) ;
#70080=CARTESIAN_POINT ( 'NONE',  ( 1.991789202884729715, 1421.124413674059952, 183.1574783845820207 ) ) ;
#70083=CARTESIAN_POINT ( 'NONE',  ( 14.91384436259999902, 1485.716867147530138, 224.8720064076979952 ) ) ;
#70088=CARTESIAN_POINT ( 'NONE',  ( 11.86098062413520005, 1431.978481139299902, 149.9706316993390089 ) ) ;
#70090=CARTESIAN_POINT ( 'NONE',  ( 13.20674952220708143, 1444.700630393524307, 187.3249437680643723 ) ) ;
#70094=CARTESIAN_POINT ( 'NONE',  ( 23.61230825720000226, 1435.322028862560046, 137.2857987807979896 ) ) ;
#70096=CARTESIAN_POINT ( 'NONE',  ( -6.220537627200000586, 1424.583777295530126, 186.6152486391980005 ) ) ;
#70097=CARTESIAN_POINT ( 'NONE',  ( 3.422118110653599832, 1410.133528635409903, 269.8663509809509833 ) ) ;
#70104=FACE_OUTER_BOUND ( 'NONE', #108120, .T. ) ;
#70105=CARTESIAN_POINT ( 'NONE',  ( -5.023809873749912391, 1422.821914202444304, 184.8408105619813568 ) ) ;
#70107=CARTESIAN_POINT ( 'NONE',  ( 17.79886040655730284, 1417.133647275629983, 224.9897512113339815 ) ) ;
#70109=ORIENTED_EDGE ( 'NONE', *, *, #85776, .F. ) ;
#70110=CARTESIAN_POINT ( 'NONE',  ( 38.34143788450000301, 1440.913060387330006, 265.6112250856980381 ) ) ;
#70112=CARTESIAN_POINT ( 'NONE',  ( 13.80546151116429954, 1434.979654507460054, 148.5370226032280243 ) ) ;
#70120=B_SPLINE_CURVE_WITH_KNOTS ( 'NONE', 3,
 ( #27490, #79571, #10142, #96916, #61678, #95801, #19069, #53273, #87412, #10707, #44878 ),
 .UNSPECIFIED., .F., .F.,
 ( 4, 2, 1, 2, 2, 4 ),
 ( 0.000000000000000000, 0.2499999999997352118, 0.3749999999995330957, 0.4374999999994320654, 0.4999999999993309796, 1.000000000000000000 ),
 .UNSPECIFIED. ) ;
#70122=ADVANCED_FACE ( 'NONE', ( #82642 ), #35667, .F. ) ;
#70123=CARTESIAN_POINT ( 'NONE',  ( -10.81519956420000028, 1424.921090988229935, 144.1714224092980032 ) ) ;
#70124=CARTESIAN_POINT ( 'NONE',  ( -14.62342645192239843, 1422.162688039920113, 221.5608089125659887 ) ) ;
#70127=EDGE_CURVE ( 'NONE', #93336, #84761, #41856, .T. ) ;
#70129=CARTESIAN_POINT ( 'NONE',  ( -13.22806383169999833, 1431.113060387329824, 222.3499097936980036 ) ) ;
#70130=CARTESIAN_POINT ( 'NONE',  ( 13.26154391220000051, 1415.081125743829944, 228.6222406189980063 ) ) ;
#70132=CARTESIAN_POINT ( 'NONE',  ( -16.96734216822699892, 1460.582103501581969, 228.2620883328710022 ) ) ;
#70134=CARTESIAN_POINT ( 'NONE',  ( 18.39250288750000095, 1408.568853042730098, 268.3412086706979949 ) ) ;
#70136=CARTESIAN_POINT ( 'NONE',  ( 24.71638692850000396, 1435.786853257239954, 137.7886294928979964 ) ) ;
#70137=CARTESIAN_POINT ( 'NONE',  ( 19.52745459059999789, 1469.160779044030050, 191.2963237270979846 ) ) ;
#70138=CARTESIAN_POINT ( 'NONE',  ( -23.49218588160000110, 1435.195132014040155, 213.3092087416680158 ) ) ;
#70139=CARTESIAN_POINT ( 'NONE',  ( 27.43355929049999986, 1507.980920698529872, 207.4175378521480013 ) ) ;
#70142=CARTESIAN_POINT ( 'NONE',  ( -22.33217205817994255, 1507.117986396238166, 204.9771641880283823 ) ) ;
#70143=CARTESIAN_POINT ( 'NONE',  ( -16.61533299009999709, 1414.913060387329779, 205.7754145581380101 ) ) ;
#70144=CARTESIAN_POINT ( 'NONE',  ( -13.95628782549999869, 1442.683319114259803, 188.5952711372979991 ) ) ;
#70145=EDGE_CURVE ( 'NONE', #18900, #63032, #8665, .T. ) ;
#70146=CARTESIAN_POINT ( 'NONE',  ( -27.78452750130110260, 1508.000976266860107, 210.4681927182890036 ) ) ;
#70147=CARTESIAN_POINT ( 'NONE',  ( -33.54529832459999739, 1435.829277014980107, 135.9561275551980088 ) ) ;
#70150=ADVANCED_FACE ( 'NONE', ( #42286 ), #85692, .T. ) ;
#70152=CARTESIAN_POINT ( 'NONE',  ( -12.86297904326220021, 1409.362245513460039, 201.5229356212220182 ) ) ;
#70156=CARTESIAN_POINT ( 'NONE',  ( -38.70127719692458612, 1443.501467202840104, 136.9798462687442679 ) ) ;
#70158=CARTESIAN_POINT ( 'NONE',  ( -46.16778036140000552, 1446.056973084060019, 266.9714954301979901 ) ) ;
#70160=CARTESIAN_POINT ( 'NONE',  ( -14.45750500688560081, 1416.828039245989885, 221.3916439204320170 ) ) ;
#70161=CARTESIAN_POINT ( 'NONE',  ( -25.63704141100000200, 1507.963169804229892, 218.3319399335480000 ) ) ;
#70164=CARTESIAN_POINT ( 'NONE',  ( 18.41238929687650128, 1425.273680578170115, 226.4426435738229770 ) ) ;
#70165=CARTESIAN_POINT ( 'NONE',  ( 20.85881780809999952, 1508.960366401729971, 227.7807767123979943 ) ) ;
#70166=CARTESIAN_POINT ( 'NONE',  ( 15.22899453930000035, 1495.924838334530023, 224.5915237618979745 ) ) ;
#70167=EDGE_CURVE ( 'NONE', #19615, #59795, #12520, .T. ) ;
#70170=CARTESIAN_POINT ( 'NONE',  ( -9.837454594919998740, 1508.005995996430102, 182.3419145424980172 ) ) ;
#70171=CARTESIAN_POINT ( 'NONE',  ( -23.49882790210000394, 1410.228905210230096, 207.0913801706779793 ) ) ;
#70172=CARTESIAN_POINT ( 'NONE',  ( 17.84204423069999734, 1415.932840167130053, 208.7775004867189921 ) ) ;
#70178=CARTESIAN_POINT ( 'NONE',  ( 17.60627569411529691, 1410.895669416499913, 224.1775087544040161 ) ) ;
#70179=( BOUNDED_CURVE ( )  B_SPLINE_CURVE ( 3, ( #18430, #45347, #18987, #37472 ),
 .UNSPECIFIED., .F., .T. ) 
 B_SPLINE_CURVE_WITH_KNOTS ( ( 4, 4 ),
 ( 3.108823480124809802, 3.416777941171309951 ),
 .UNSPECIFIED. ) 
 CURVE ( )  GEOMETRIC_REPRESENTATION_ITEM ( )  RATIONAL_B_SPLINE_CURVE ( ( 1.000000000000000000, 0.9921126061611611480, 0.9921126061611611480, 1.000000000000000000 ) ) 
 REPRESENTATION_ITEM ( '' )  );
#70183=CARTESIAN_POINT ( 'NONE',  ( -0.1019954133980000149, 1415.740983310430011, 233.4942065637980306 ) ) ;
#70186=EDGE_CURVE ( 'NONE', #24399, #29251, #36304, .T. ) ;
#70187=CARTESIAN_POINT ( 'NONE',  ( -23.31536538260000313, 1425.877123410529975, 211.5352558136579830 ) ) ;
#70188=CARTESIAN_POINT ( 'NONE',  ( -1.780436306985229811, 1421.048930496699995, 183.4850363039900003 ) ) ;
#70191=CARTESIAN_POINT ( 'NONE',  ( -15.55317322349129938, 1485.870500728060051, 186.9405944658579983 ) ) ;
#70192=CARTESIAN_POINT ( 'NONE',  ( -19.52959706730000278, 1468.975338568629923, 192.9635188021979957 ) ) ;
#70200=CARTESIAN_POINT ( 'NONE',  ( 11.95465844686730073, 1433.562513212249996, 150.0837927613160048 ) ) ;
#70205=LINE ( 'NONE', #104311, #71171 ) ;
#70206=CARTESIAN_POINT ( 'NONE',  ( -0.1042373741590000014, 1508.844537587730201, 179.8773204004980073 ) ) ;
#70208=DIRECTION ( 'NONE',  ( -1.000000000000000000, 0.000000000000000000, -2.775557561562891351E-14 ) ) ;
#70209=CARTESIAN_POINT ( 'NONE',  ( 3.328378719390000295, 1488.171522112329967, 182.3487599890979993 ) ) ;
#70211=CARTESIAN_POINT ( 'NONE',  ( -24.06822806131540204, 1444.795745940579991, 211.8976761515809812 ) ) ;
#70214=CARTESIAN_POINT ( 'NONE',  ( 37.83686684571890169, 1436.862236043870098, 134.0999999968879877 ) ) ;
#70216=CARTESIAN_POINT ( 'NONE',  ( -12.54761498111694884, 1509.351232781885074, 235.8718500083220704 ) ) ;
#70218=CARTESIAN_POINT ( 'NONE',  ( 13.64250267370000103, 1435.175725784029964, 149.6291831842980287 ) ) ;
#70222=VERTEX_POINT ( 'NONE', #84013 ) ;
#70224=CARTESIAN_POINT ( 'NONE',  ( -2.975604897060000198, 1464.763624779529891, 236.8058159536980156 ) ) ;
#70225=CARTESIAN_POINT ( 'NONE',  ( 17.33396934321472926, 1451.072800439867706, 148.0459263477291074 ) ) ;
#70228=CARTESIAN_POINT ( 'NONE',  ( -19.06540802248403565, 1442.452554616592579, 210.7014195594630905 ) ) ;
#70230=CARTESIAN_POINT ( 'NONE',  ( 4.238698726834749131, 1446.369305975439829, 163.0897191397669985 ) ) ;
#70231=CARTESIAN_POINT ( 'NONE',  ( -0.008809588698450001101, 1507.869595074230119, 237.5091932035980165 ) ) ;
#70235=CARTESIAN_POINT ( 'NONE',  ( 32.84806791407179816, 1440.913060387330006, 257.4303453130210073 ) ) ;
#70236=CARTESIAN_POINT ( 'NONE',  ( -20.65862993740000064, 1509.573542409829997, 188.2595545114980098 ) ) ;
#70239=CARTESIAN_POINT ( 'NONE',  ( -14.78404272899999938, 1410.801860023729887, 190.6280328239980122 ) ) ;
#70241=CARTESIAN_POINT ( 'NONE',  ( -24.33264312739999724, 1442.481256506720001, 211.4417695029279685 ) ) ;
#70243=CARTESIAN_POINT ( 'NONE',  ( -3.530668216773314118E-09, 1395.913060387170844, 197.9004239563262217 ) ) ;
#70245=CARTESIAN_POINT ( 'NONE',  ( -12.91279240200000089, 1434.774393157829991, 149.9807649780979943 ) ) ;
#70247=CARTESIAN_POINT ( 'NONE',  ( -25.19798387652940264, 1470.611580667020007, 212.0227933820560224 ) ) ;
#70254=CARTESIAN_POINT ( 'NONE',  ( -17.92791450389482222, 1486.167514923851513, 188.4156298903135962 ) ) ;
#70258=CARTESIAN_POINT ( 'NONE',  ( 14.01630619350000018, 1463.409576321530039, 240.3753821329979985 ) ) ;
#70261=CARTESIAN_POINT ( 'NONE',  ( -7.349614982530000340, 1507.875248142329838, 235.6215898391979806 ) ) ;
#70264=CARTESIAN_POINT ( 'NONE',  ( 11.87124599549999893, 1432.722052905369992, 149.9814473066979872 ) ) ;
#70265=CARTESIAN_POINT ( 'NONE',  ( 19.08933866519999967, 1456.280081694130104, 226.1031454244979955 ) ) ;
#70272=CARTESIAN_POINT ( 'NONE',  ( 12.83854459959200156, 1470.906649396920102, 269.8736685321649702 ) ) ;
#70273=CARTESIAN_POINT ( 'NONE',  ( 2.478743724850000163, 1435.404071181940026, 157.6105368136979905 ) ) ;
#70275=CARTESIAN_POINT ( 'NONE',  ( 1.090037377353519974E-11, 1406.777728848529932, 269.6500679732980075 ) ) ;
#70276=B_SPLINE_CURVE_WITH_KNOTS ( 'NONE', 3,
 ( #46267, #3709, #18250, #44034, #78171, #87131, #10420, #56849, #14822, #55768, #40034, #4771, #56295, #90981 ),
 .UNSPECIFIED., .F., .F.,
 ( 4, 2, 2, 2, 2, 2, 4 ),
 ( 0.000000000000000000, 0.001069581499410647389, 0.001604372249115970867, 0.002139162998821294778, 0.003208744498231351060, 0.003743535247936652637, 0.004278325997641954648 ),
 .UNSPECIFIED. ) ;
#70277=EDGE_CURVE ( 'NONE', #21233, #68144, #101788, .T. ) ;
#70278=CARTESIAN_POINT ( 'NONE',  ( -38.86154762539019458, 1440.913060394929971, 257.6231068593190230 ) ) ;
#70279=CARTESIAN_POINT ( 'NONE',  ( 34.16143226917030518, 1450.427616041969941, 136.2389182185960124 ) ) ;
#70280=CARTESIAN_POINT ( 'NONE',  ( 2.497446428329765489, 1449.075933931984537, 154.5437254066351329 ) ) ;
#70282=ADVANCED_FACE ( 'NONE', ( #49880 ), #7314, .T. ) ;
#70283=CARTESIAN_POINT ( 'NONE',  ( -1.433829657236012523, 1450.688199284849816, 182.8043069926514193 ) ) ;
#70287=CARTESIAN_POINT ( 'NONE',  ( -38.34143788450000301, 1436.524347981669962, 265.6112249940979950 ) ) ;
#70288=CARTESIAN_POINT ( 'NONE',  ( -0.5697963391879999895, 1450.893162800530263, 181.2886238165980046 ) ) ;
#70290=CARTESIAN_POINT ( 'NONE',  ( -0.5500088493020000024, 1475.046162849929942, 269.6499792952980101 ) ) ;
#70295=CARTESIAN_POINT ( 'NONE',  ( -18.96271086799999850, 1416.819756528530206, 208.0003800946280137 ) ) ;
#70296=CARTESIAN_POINT ( 'NONE',  ( 11.86774696298919984, 1432.458695464179982, 149.9821701094620039 ) ) ;
#70298=CARTESIAN_POINT ( 'NONE',  ( -13.48132209962330030, 1443.611916072062741, 169.3589951324157710 ) ) ;
#70299=ORIENTED_EDGE ( 'NONE', *, *, #108978, .F. ) ;
#70300=CARTESIAN_POINT ( 'NONE',  ( 4.408870434958439333, 1425.824683284920184, 185.4670092970000042 ) ) ;
#70301=CARTESIAN_POINT ( 'NONE',  ( 11.98890328080000067, 1442.756953654919926, 147.5994355510979688 ) ) ;
#70304=CARTESIAN_POINT ( 'NONE',  ( 2.242229686229999963, 1409.158574056130192, 231.2133334487979823 ) ) ;
#70306=CARTESIAN_POINT ( 'NONE',  ( 10.74293569890000022, 1425.684509311930242, 97.29932836569790311 ) ) ;
#70315=CARTESIAN_POINT ( 'NONE',  ( 2.541163892419999737, 1448.917481751670039, 182.8661774463979839 ) ) ;
#70316=EDGE_CURVE ( 'NONE', #56560, #11116, #93520, .T. ) ;
#70318=CARTESIAN_POINT ( 'NONE',  ( -0.6774325393469999845, 1465.095555782530027, 238.0673157071979915 ) ) ;
#70321=CARTESIAN_POINT ( 'NONE',  ( -40.27186325100000630, 1443.842159933049970, 137.1351494573980005 ) ) ;
#70322=CARTESIAN_POINT ( 'NONE',  ( 0.02607543431880000179, 1466.687777830830100, 235.6591783243979989 ) ) ;
#70323=FACE_OUTER_BOUND ( 'NONE', #54633, .T. ) ;
#70325=CARTESIAN_POINT ( 'NONE',  ( 12.53380499169999851, 1442.773887286369927, 177.9435428178979919 ) ) ;
#70328=CARTESIAN_POINT ( 'NONE',  ( 14.59277107062129986, 1436.244837967300100, 149.8707660814949918 ) ) ;
#70329=CARTESIAN_POINT ( 'NONE',  ( -36.21674782232960155, 1450.969262370170100, 135.9186764936750080 ) ) ;
#70330=CARTESIAN_POINT ( 'NONE',  ( 33.93525398028069873, 1436.160849851710054, 136.3001642050429894 ) ) ;
#70331=CARTESIAN_POINT ( 'NONE',  ( 9.646161636302020170, 1396.249911776859790, 214.5408828654969966 ) ) ;
#70332=CARTESIAN_POINT ( 'NONE',  ( 13.93304799769729918, 1408.881101324619976, 204.4086770006200027 ) ) ;
#70333=CARTESIAN_POINT ( 'NONE',  ( -5.337764340897860116, 1406.291602267970120, 269.0345653378449811 ) ) ;
#70334=CARTESIAN_POINT ( 'NONE',  ( -14.20723507282459863, 1435.348451359640194, 149.4979282535020104 ) ) ;
#70336=CARTESIAN_POINT ( 'NONE',  ( 3.902542322860000024, 1426.015650169130140, 185.2953858070979720 ) ) ;
#70347=CARTESIAN_POINT ( 'NONE',  ( 7.191822421769999529, 1414.913060387229962, 224.1599105121979960 ) ) ;
#70349=CARTESIAN_POINT ( 'NONE',  ( -4.363122647530000009, 1407.471318475729959, 146.1721969590979882 ) ) ;
#70350=CARTESIAN_POINT ( 'NONE',  ( 10603.70820181224371, 2837.742859962505918, -4739.672918854301315 ) ) ;
#70351=CARTESIAN_POINT ( 'NONE',  ( 11.79467588633447583, 1433.007546482180260, 150.6262872999809019 ) ) ;
#70354=CARTESIAN_POINT ( 'NONE',  ( -10.15115807179999941, 1410.198279941630062, 229.5434800901979884 ) ) ;
#70355=CARTESIAN_POINT ( 'NONE',  ( -10.93884247429999945, 1445.278210069279794, 184.9723926117980284 ) ) ;
#70356=ORIENTED_EDGE ( 'NONE', *, *, #28932, .F. ) ;
#70357=LINE ( 'NONE', #97724, #33258 ) ;
#70358=CARTESIAN_POINT ( 'NONE',  ( -24.49816830492780184, 1440.913060440859908, 212.6606737188390071 ) ) ;
#70360=SPHERICAL_SURFACE ( 'NONE', #67763, 2.000000000000000000 ) ;
#70361=CARTESIAN_POINT ( 'NONE',  ( -24.89417918259999851, 1435.865321316010295, 137.4102906330980147 ) ) ;
#70364=CARTESIAN_POINT ( 'NONE',  ( 0.009483596459017473723, 1508.335432445508786, 237.8375765388574337 ) ) ;
#70369=CARTESIAN_POINT ( 'NONE',  ( 2.500000000000000000, 1435.788807054279914, 157.6019689661980010 ) ) ;
#70370=CARTESIAN_POINT ( 'NONE',  ( -14.02792940870000038, 1415.367714275730123, 227.2463639653980181 ) ) ;
#70375=DIRECTION ( 'NONE',  ( 0.01398399491000389475, 0.01017778245426219710, -0.9998504191281166742 ) ) ;
#70376=CARTESIAN_POINT ( 'NONE',  ( 12.12836356214739908, 1434.009854529710083, 150.0535883806440154 ) ) ;
#70377=CARTESIAN_POINT ( 'NONE',  ( 14.13280191679420028, 1478.704388969779984, 231.2915111619190043 ) ) ;
#70378=CARTESIAN_POINT ( 'NONE',  ( -22.35377295150689747, 1508.960832111700029, 226.0627451311750065 ) ) ;
#70381=CARTESIAN_POINT ( 'NONE',  ( 0.02113572768988940254, 1420.444438332730215, 182.6732129553429900 ) ) ;
#70383=CARTESIAN_POINT ( 'NONE',  ( -3.959162678200000229, 1419.915783653529843, 186.3511350151979968 ) ) ;
#70385=CARTESIAN_POINT ( 'NONE',  ( 18.42577555256999844, 1424.509265906519886, 223.4215472205989954 ) ) ;
#70387=CARTESIAN_POINT ( 'NONE',  ( -12.44185449472369953, 1415.426561690380140, 196.8128181430920165 ) ) ;
#70388=FACE_OUTER_BOUND ( 'NONE', #43166, .T. ) ;
#70389=ORIENTED_EDGE ( 'NONE', *, *, #37285, .T. ) ;
#70395=CARTESIAN_POINT ( 'NONE',  ( -26.35475552313950232, 1507.985742420310089, 201.5462045797129917 ) ) ;
#70397=CARTESIAN_POINT ( 'NONE',  ( -2.499999998559999881, 1448.104721231620033, 157.8850639176980337 ) ) ;
#70399=CARTESIAN_POINT ( 'NONE',  ( -21.65324558190000204, 1435.253471290910056, 140.9571069649979904 ) ) ;
#70400=CARTESIAN_POINT ( 'NONE',  ( -7.333237907140000900, 1433.447543843880112, 149.5704065546979962 ) ) ;
#70401=CARTESIAN_POINT ( 'NONE',  ( 16.72731342339999827, 1418.990981506430217, 191.3670037215980244 ) ) ;
#70403=CARTESIAN_POINT ( 'NONE',  ( -19.00997723749662427, 1439.581593688745215, 210.0041471448513732 ) ) ;
#70404=CARTESIAN_POINT ( 'NONE',  ( -26.79413315976150045, 1435.433175095809929, 135.2874648155150226 ) ) ;
#70407=CARTESIAN_POINT ( 'NONE',  ( 24.38386427640000065, 1449.838343677799912, 206.7258738186879725 ) ) ;
#70408=CARTESIAN_POINT ( 'NONE',  ( -24.04833748900000145, 1437.594120219370097, 211.5101582450080002 ) ) ;
#70412=CARTESIAN_POINT ( 'NONE',  ( -12.53380499169999851, 1442.773887286369927, 169.4755105685979970 ) ) ;
#70417=EDGE_CURVE ( 'NONE', #36273, #23739, #108695, .T. ) ;
#70418=B_SPLINE_CURVE_WITH_KNOTS ( 'NONE', 5,
 ( #64687, #13670, #67442, #18101, #25387, #33802, #59580, #103200, #76370, #26506, #68543, #1328 ),
 .UNSPECIFIED., .F., .F.,
 ( 6, 3, 3, 6 ),
 ( 0.000000000000000000, 0.2278800823983170021, 0.5900544727611899409, 1.000000000000000000 ),
 .UNSPECIFIED. ) ;
#70421=CARTESIAN_POINT ( 'NONE',  ( -22.83134035751703905, 1409.745587068702889, 209.7110239188152150 ) ) ;
#70424=CARTESIAN_POINT ( 'NONE',  ( -18.57177926220356667, 1458.612650609036109, 227.5361665883615387 ) ) ;
#70426=CARTESIAN_POINT ( 'NONE',  ( 19.98048820006079751, 1508.975598045479956, 229.6642444245289880 ) ) ;
#70429=ORIENTED_EDGE ( 'NONE', *, *, #74117, .F. ) ;
#70431=CARTESIAN_POINT ( 'NONE',  ( 18.28847123799999963, 1425.325025442230071, 225.4709929694980133 ) ) ;
#70433=CARTESIAN_POINT ( 'NONE',  ( 20.42020019299999944, 1470.816980701229795, 208.7465247758109967 ) ) ;
#70434=CARTESIAN_POINT ( 'NONE',  ( -41.56052291270000154, 1440.913060434399995, 261.5689799299980223 ) ) ;
#70436=CARTESIAN_POINT ( 'NONE',  ( -11.92876349830000038, 1433.442608765759815, 149.9100308696980051 ) ) ;
#70437=CARTESIAN_POINT ( 'NONE',  ( 24.69949309869999965, 1509.552011340129866, 195.6045197258980011 ) ) ;
#70438=CARTESIAN_POINT ( 'NONE',  ( -20.27111778190000280, 1485.538628530129927, 191.5000650964979911 ) ) ;
#70439=CARTESIAN_POINT ( 'NONE',  ( 10.14794430829999961, 1410.198169809130150, 188.6983266523980092 ) ) ;
#70440=CARTESIAN_POINT ( 'NONE',  ( 4.455748556580000574, 1421.964143777330037, 184.5555025332980108 ) ) ;
#70442=CARTESIAN_POINT ( 'NONE',  ( 10.15459887489999957, 1436.277524974660082, 152.4140740738980071 ) ) ;
#70443=CARTESIAN_POINT ( 'NONE',  ( -3.144306714850350293, 1440.618978642349930, 155.9524017610649764 ) ) ;
#70444=CARTESIAN_POINT ( 'NONE',  ( -6.348459599079999904, 1451.445385983630104, 153.6738296132980111 ) ) ;
#70445=CARTESIAN_POINT ( 'NONE',  ( 1.594477343619999932, 1465.161209020629940, 235.7125686318980229 ) ) ;
#70446=VERTEX_POINT ( 'NONE', #45358 ) ;
#70449=CARTESIAN_POINT ( 'NONE',  ( -42.54899908119999452, 1440.913084212150125, 270.0692079169979820 ) ) ;
#70450=CARTESIAN_POINT ( 'NONE',  ( -23.89984773989923639, 1435.936556201614849, 211.3273771066375843 ) ) ;
#70451=CARTESIAN_POINT ( 'NONE',  ( 9.663014860980000620, 1442.759804623820173, 153.0865865510980086 ) ) ;
#70453=CARTESIAN_POINT ( 'NONE',  ( 4.360582346120001063, 1431.113060387329824, 190.2999270487979970 ) ) ;
#70454=CARTESIAN_POINT ( 'NONE',  ( 2.831208615256320282, 1409.103140891420026, 230.6980589985730035 ) ) ;
#70455=CARTESIAN_POINT ( 'NONE',  ( -1.149035020100000137, 1415.140114695929924, 226.8980037389979998 ) ) ;
#70456=CARTESIAN_POINT ( 'NONE',  ( -7.703814818310000589, 1418.732955197130195, 232.4505356538980152 ) ) ;
#70459=CARTESIAN_POINT ( 'NONE',  ( -45.28153491675919895, 1434.439803511990021, 266.7022297949800418 ) ) ;
#70460=CARTESIAN_POINT ( 'NONE',  ( -3.086273611079999757, 1434.212532904980208, 185.3571854654980200 ) ) ;
#70461=EDGE_LOOP ( 'NONE', ( #5159, #13825, #60977, #83393, #108532, #16422 ) ) ;
#70465=DIRECTION ( 'NONE',  ( -8.117787186050000125E-15, -2.786659791809999935E-14, -1.000000000000000000 ) ) ;
#70470=B_SPLINE_SURFACE_WITH_KNOTS ( 'NONE', 5, 5, ( 
 ( #11402, #45017, #106010, #29286, #1912, #45570 ),
 ( #3018, #10274, #105452, #63482, #80249, #104343 ),
 ( #46669, #28741, #37141, #95395, #62946, #97057 ),
 ( #79163, #52858, #36049, #61821, #36588, #61280 ),
 ( #44451, #19204, #20321, #12486, #3567, #72415 ),
 ( #54527, #70236, #2471, #86985, #53406, #10846 ) ),
 .UNSPECIFIED., .F., .F., .F.,
 ( 6, 6 ),
 ( 6, 6 ),
 ( 26.92148545460000264, 41.10482460869999954 ),
 ( 0.000000000000000000, 2.000000000000000000 ),
 .UNSPECIFIED. ) ;
#70472=CARTESIAN_POINT ( 'NONE',  ( -15.72497962059999921, 1506.810797420529980, 193.7296588674980171 ) ) ;
#70473=CARTESIAN_POINT ( 'NONE',  ( 0.3570154777189999962, 1451.680777065829943, 183.0662967611979752 ) ) ;
#70474=CARTESIAN_POINT ( 'NONE',  ( 13.17272844760000083, 1434.822352678270136, 195.6302333700980114 ) ) ;
#70475=CARTESIAN_POINT ( 'NONE',  ( 11.60004869885203860, 1424.621825572507532, 136.2521570335653678 ) ) ;
#70477=DIRECTION ( 'NONE',  ( -0.6906235816661250304, 0.2466512791670444904, 0.6798545542481230219 ) ) ;
#70480=CARTESIAN_POINT ( 'NONE',  ( -16.50783381592070143, 1412.114139793179902, 270.0842635278900161 ) ) ;
#70483=CARTESIAN_POINT ( 'NONE',  ( 4.249559015328859601, 1418.026146675719929, 233.7825626454939822 ) ) ;
#70489=CARTESIAN_POINT ( 'NONE',  ( 45.47623103552137991, 1443.785048864438522, 268.9791838446159318 ) ) ;
#70490=CARTESIAN_POINT ( 'NONE',  ( -0.3788414990293429985, 1408.926289824029936, 186.6322569618010050 ) ) ;
#70491=CARTESIAN_POINT ( 'NONE',  ( -10.72663399029027964, 1438.657822394603727, 152.4853033122590773 ) ) ;
#70494=CARTESIAN_POINT ( 'NONE',  ( -17.48716113793120286, 1415.020374539339855, 207.5653286189619848 ) ) ;
#70495=CARTESIAN_POINT ( 'NONE',  ( -17.92118525700000120, 1420.840642511729811, 225.6991564338980254 ) ) ;
#70496=CARTESIAN_POINT ( 'NONE',  ( 15.87316543544599945, 1474.349515721750095, 267.7599166360050162 ) ) ;
#70498=CARTESIAN_POINT ( 'NONE',  ( -8.771379158800783671, 1465.168284390142617, 232.9278865296558365 ) ) ;
#70499=CARTESIAN_POINT ( 'NONE',  ( 10.31307702720000030, 1447.342907605319851, 186.9095413067980189 ) ) ;
#70502=CARTESIAN_POINT ( 'NONE',  ( 20.38176113183206439, 1410.985889941965070, 219.3306597827873077 ) ) ;
#70503=CARTESIAN_POINT ( 'NONE',  ( 1.487297559325930107, 1473.104910899560082, 182.5967061028410114 ) ) ;
#70507=CARTESIAN_POINT ( 'NONE',  ( 24.45310709153400097, 1452.054032404549844, 136.2426869603699799 ) ) ;
#70508=EDGE_CURVE ( 'NONE', #52184, #17927, #71362, .T. ) ;
#70509=CARTESIAN_POINT ( 'NONE',  ( -23.10442739037580040, 1411.095127590459924, 210.9251608898400150 ) ) ;
#70512=CARTESIAN_POINT ( 'NONE',  ( 17.81467328779999804, 1409.700101153729975, 194.2398719659980202 ) ) ;
#70514=CARTESIAN_POINT ( 'NONE',  ( 2.688983237145497363, 1439.653997274290305, 183.6213077983770461 ) ) ;
#70515=CARTESIAN_POINT ( 'NONE',  ( 0.5934285380220000183, 1417.359862721729996, 235.5294838487980087 ) ) ;
#70516=CARTESIAN_POINT ( 'NONE',  ( -18.83596995908460059, 1424.713049970400107, 224.4964886877786512 ) ) ;
#70520=CARTESIAN_POINT ( 'NONE',  ( 27.74428279426650334, 1446.393444133639832, 137.1635631392660173 ) ) ;
#70525=CARTESIAN_POINT ( 'NONE',  ( -8576.261851439176098, 2833.596074015790236, -10892.29874055330765 ) ) ;
#70526=CARTESIAN_POINT ( 'NONE',  ( -34.87559606798220813, 1450.334017323499893, 136.2297881972530149 ) ) ;
#70527=CARTESIAN_POINT ( 'NONE',  ( -6.759474677965349620, 1416.948096802409964, 218.8894228273509839 ) ) ;
#70528=CARTESIAN_POINT ( 'NONE',  ( -3.114882401860000094, 1454.846680951630105, 214.3676144192479853 ) ) ;
#70529=CARTESIAN_POINT ( 'NONE',  ( 45.63117166579991135, 1442.771140612856243, 266.1897092273976568 ) ) ;
#70530=CARTESIAN_POINT ( 'NONE',  ( 10.98577627829999948, 1433.173240417669831, 151.7674451195979941 ) ) ;
#70532=CARTESIAN_POINT ( 'NONE',  ( 26.21990212871559933, 1440.913060396030005, 223.0271923088249935 ) ) ;
#70535=CARTESIAN_POINT ( 'NONE',  ( -28.15442807850000051, 1509.896234805130007, 200.8410251444579728 ) ) ;
#70538=CARTESIAN_POINT ( 'NONE',  ( -9.656302321220000096, 1486.131777580530070, 183.4210019581979907 ) ) ;
#70540=CARTESIAN_POINT ( 'NONE',  ( -8.778933807423072722, 1427.705008372408884, 144.1938086916980524 ) ) ;
#70541=CARTESIAN_POINT ( 'NONE',  ( 25.80166435820000004, 1469.242112528930193, 212.9326132565380192 ) ) ;
#70543=CARTESIAN_POINT ( 'NONE',  ( -13.70965915470000063, 1507.817784722230044, 232.5379316308980151 ) ) ;
#70545=CARTESIAN_POINT ( 'NONE',  ( -25.62237252300000279, 1435.677407238350042, 212.3102753037179866 ) ) ;
#70546=CARTESIAN_POINT ( 'NONE',  ( 18.64588652299999794, 1416.828040475229955, 209.6843149956849857 ) ) ;
#70547=FACE_OUTER_BOUND ( 'NONE', #16547, .T. ) ;
#70548=CARTESIAN_POINT ( 'NONE',  ( 0.1618819747345350002, 1485.136375146799764, 181.8737203127180067 ) ) ;
#70550=EDGE_LOOP ( 'NONE', ( #17182, #70637, #110787, #71321 ) ) ;
#70551=CARTESIAN_POINT ( 'NONE',  ( -0.4299350981030000129, 1451.092099702930000, 182.2245401378979750 ) ) ;
#70561=CARTESIAN_POINT ( 'NONE',  ( 12.27010794681469008, 1416.835807157242016, 223.5795575599114500 ) ) ;
#70565=CARTESIAN_POINT ( 'NONE',  ( 14.89108873512989994, 1409.433068664470056, 210.2543917981890047 ) ) ;
#70566=CARTESIAN_POINT ( 'NONE',  ( 6.763640255447179445E-10, 1465.118916387369836, 238.1343321182859825 ) ) ;
#70568=CARTESIAN_POINT ( 'NONE',  ( -17.30242272219999933, 1430.613991027629936, 191.1830775443980031 ) ) ;
#70571=DIRECTION ( 'NONE',  ( 0.9810655946269050132, 0.06469995582470079720, 0.1825492118735090041 ) ) ;
#70572=CARTESIAN_POINT ( 'NONE',  ( -2.370970874524634286, 1427.002265528474027, 134.0999999980979567 ) ) ;
#70574=VERTEX_POINT ( 'NONE', #39686 ) ;
#70576=CIRCLE ( 'NONE', #65212, 2.000000000029146907 ) ;
#70579=CARTESIAN_POINT ( 'NONE',  ( 5.512104717576124635, 1471.237629144492075, 269.3375989710273188 ) ) ;
#70584=CARTESIAN_POINT ( 'NONE',  ( 0.1857455191719999954, 1471.145214114130113, 182.4746948879979982 ) ) ;
#70590=B_SPLINE_SURFACE_WITH_KNOTS ( 'NONE', 5, 5, ( 
 ( #14890, #48529, #58579, #75917, #5960, #109524, #40105, #83763, #7604 ),
 ( #23292, #49081, #108417, #50716, #41215, #110069, #83216, #23837, #84845 ),
 ( #91613, #84312, #108975, #74287, #59139, #6505, #101640, #40659, #93261 ),
 ( #16525, #76467, #110619, #66984, #31701, #68097, #92707, #56924, #50186 ),
 ( #91054, #74832, #100557, #58029, #92164, #7060, #1996, #77579, #78117 ),
 ( #26038, #96026, #27174, #19297, #79244, #9270, #35561, #102742, #61908 ),
 ( #51833, #43430, #69191, #25490, #340, #42876, #52939, #59681, #68642 ),
 ( #10361, #60801, #87076, #36131, #78679, #8695, #17628, #2552, #60231 ),
 ( #93793, #69757, #70315, #102210, #94350, #85970, #887, #35010, #87642 ) ),
 .UNSPECIFIED., .F., .F., .F.,
 ( 6, 3, 6 ),
 ( 6, 3, 6 ),
 ( 4.947986407769999317, 8.870455474829999076, 10.02594095490000115 ),
 ( 0.000000000000000000, 1.000000000000000000, 2.000000000000000000 ),
 .UNSPECIFIED. ) ;
#70595=ORIENTED_EDGE ( 'NONE', *, *, #85022, .T. ) ;
#70596=CARTESIAN_POINT ( 'NONE',  ( 27.41410076250000216, 1415.612337104729932, 262.1295773258979693 ) ) ;
#70597=CARTESIAN_POINT ( 'NONE',  ( -25.66628087289999982, 1469.241412583229931, 204.8365099310479991 ) ) ;
#70598=CARTESIAN_POINT ( 'NONE',  ( -10.89878236088929953, 1426.095048252110246, 91.95250234051970040 ) ) ;
#70599=CARTESIAN_POINT ( 'NONE',  ( 17.21791179325979826, 1410.146180600570005, 192.5803812474509868 ) ) ;
#70602=DIRECTION ( 'NONE',  ( -1.000000000000000000, -2.220446049250313081E-13, 0.000000000000000000 ) ) ;
#70603=CARTESIAN_POINT ( 'NONE',  ( -27.90885395119999757, 1424.419860134829833, 250.2249407852980028 ) ) ;
#70604=CARTESIAN_POINT ( 'NONE',  ( 20.55662018261149981, 1509.675015189930036, 230.6199700381970104 ) ) ;
#70605=CARTESIAN_POINT ( 'NONE',  ( 29.21489664454900037, 1509.775817163060083, 209.5928712634359954 ) ) ;
#70607=CARTESIAN_POINT ( 'NONE',  ( -22.70509189929999749, 1409.705932116229860, 208.9454376012710100 ) ) ;
#70608=ORIENTED_EDGE ( 'NONE', *, *, #103466, .F. ) ;
#70611=CARTESIAN_POINT ( 'NONE',  ( -16.64514777280000146, 1458.767275973729966, 229.9812677959979794 ) ) ;
#70618=CARTESIAN_POINT ( 'NONE',  ( -0.7271388932819999873, 1419.324264331729864, 184.7252148951980075 ) ) ;
#70622=AXIS2_PLACEMENT_3D ( 'NONE', #82641, #41185, #21603 ) ;
#70623=CARTESIAN_POINT ( 'NONE',  ( 27.27513885906573776, 1509.144913387980750, 206.1795252833925929 ) ) ;
#70624=CARTESIAN_POINT ( 'NONE',  ( 1.410687896538389996, 1420.916877493199991, 183.0185646639909862 ) ) ;
#70629=CARTESIAN_POINT ( 'NONE',  ( 13.75454463520000026, 1463.783809604629823, 225.0383857723980157 ) ) ;
#70630=ORIENTED_EDGE ( 'NONE', *, *, #59619, .F. ) ;
#70634=CARTESIAN_POINT ( 'NONE',  ( 11.86610049460949945, 1432.336025080309810, 149.9824239092829998 ) ) ;
#70636=CYLINDRICAL_SURFACE ( 'NONE', #24750, 0.5000000000000005551 ) ;
#70637=ORIENTED_EDGE ( 'NONE', *, *, #67475, .T. ) ;
#70638=CARTESIAN_POINT ( 'NONE',  ( 9.908006808964964662, 1424.402993806118047, 139.1388889620660052 ) ) ;
#70644=CARTESIAN_POINT ( 'NONE',  ( 21.97362714515480064, 1452.145724418900045, 140.5458991228840091 ) ) ;
#70645=CARTESIAN_POINT ( 'NONE',  ( 4.128048954824370398, 1410.178378922490083, 269.8667681920509835 ) ) ;
#70650=DIRECTION ( 'NONE',  ( -0.9417419115949053898, -0.3363363969979660806, -9.559255346349042767E-16 ) ) ;
#70659=CARTESIAN_POINT ( 'NONE',  ( 11.06589456070000033, 1424.668795903030286, 234.3916895905979629 ) ) ;
#70660=CARTESIAN_POINT ( 'NONE',  ( 40.27308693906149273, 1443.611999474700042, 137.1163322506119755 ) ) ;
#70664=AXIS2_PLACEMENT_3D ( 'NONE', #38218, #71881, #47731 ) ;
#70667=EDGE_CURVE ( 'NONE', #74815, #48606, #21746, .T. ) ;
#70674=CARTESIAN_POINT ( 'NONE',  ( 1.804213505530000150, 1410.351307731129964, 232.1928988982980115 ) ) ;
#70676=CARTESIAN_POINT ( 'NONE',  ( 13.05502264250409894, 1509.382255964980004, 181.3091698393539843 ) ) ;
#70678=CARTESIAN_POINT ( 'NONE',  ( -4.561655832029999580, 1453.313060387329870, 228.9334036006980000 ) ) ;
#70680=CARTESIAN_POINT ( 'NONE',  ( 4.387294391120000192, 1412.734080688830090, 231.5195920807979917 ) ) ;
#70682=CARTESIAN_POINT ( 'NONE',  ( -16.16546996768000000, 1459.158286300486225, 229.6201364928280100 ) ) ;
#70684=CARTESIAN_POINT ( 'NONE',  ( 39.36363609779999706, 1422.502404882930023, 266.6143061720980540 ) ) ;
#70686=CARTESIAN_POINT ( 'NONE',  ( 20.76830133009999813, 1436.454188401799911, 144.6138742496980001 ) ) ;
#70688=CARTESIAN_POINT ( 'NONE',  ( 25.79183385109999804, 1488.578147155629949, 204.4850554393780158 ) ) ;
#70689=CARTESIAN_POINT ( 'NONE',  ( 29.64936652346687040, 1509.975957225338334, 207.7724523241800227 ) ) ;
#70691=CARTESIAN_POINT ( 'NONE',  ( 12.73048906530000046, 1416.839648764230105, 223.1309759826980041 ) ) ;
#70694=CARTESIAN_POINT ( 'NONE',  ( -33.92723575372020406, 1435.682266284350135, 135.5036441057579850 ) ) ;
#70695=CARTESIAN_POINT ( 'NONE',  ( -6.232532107092660034, 1407.162969920749902, 197.7132727041200155 ) ) ;
#70696=CARTESIAN_POINT ( 'NONE',  ( -16.32914645889999861, 1414.913060387329779, 205.8850555510879872 ) ) ;
#70697=CARTESIAN_POINT ( 'NONE',  ( -14.11670454040000067, 1442.569783380919944, 188.7198005640980227 ) ) ;
#70698=CARTESIAN_POINT ( 'NONE',  ( -27.82104174381949946, 1508.416260427059797, 210.5121804756579991 ) ) ;
#70699=CARTESIAN_POINT ( 'NONE',  ( -32.75718130879999990, 1436.536627606989896, 136.5459210844979907 ) ) ;
#70701=ORIENTED_EDGE ( 'NONE', *, *, #39094, .F. ) ;
#70703=CARTESIAN_POINT ( 'NONE',  ( -11.51995628840010077, 1409.315346125450105, 218.6443785118009941 ) ) ;
#70705=CARTESIAN_POINT ( 'NONE',  ( -4.785434006952626440, 1421.795252747364430, 137.9170229470215077 ) ) ;
#70706=CARTESIAN_POINT ( 'NONE',  ( -45.88373572799999778, 1440.913038273419943, 266.4124089069979391 ) ) ;
#70707=CARTESIAN_POINT ( 'NONE',  ( -12.87561223598270033, 1428.667272998819954, 222.5140706137790119 ) ) ;
#70708=CARTESIAN_POINT ( 'NONE',  ( 0.3028733268543740142, 1419.325029753159924, 184.5281611957330199 ) ) ;
#70712=CARTESIAN_POINT ( 'NONE',  ( 17.30207205515339908, 1423.280328764439901, 226.7191613964260171 ) ) ;
#70713=CARTESIAN_POINT ( 'NONE',  ( 20.59646478119999813, 1507.764133386629965, 227.7125276174979831 ) ) ;
#70714=CARTESIAN_POINT ( 'NONE',  ( 13.88564761750000009, 1452.412735684230029, 223.2422962839980016 ) ) ;
#70716=CARTESIAN_POINT ( 'NONE',  ( -26.87108745762090223, 1495.338653855599887, 210.8366527536690000 ) ) ;
#70717=CARTESIAN_POINT ( 'NONE',  ( 4.363122683464830232, 1421.971318488559973, 183.8271341761570170 ) ) ;
#70722=CARTESIAN_POINT ( 'NONE',  ( 12.97490827640000077, 1414.913060387329779, 197.6684973124980047 ) ) ;
#70723=CARTESIAN_POINT ( 'NONE',  ( -12.77426335350000031, 1416.547221146729953, 195.3312399645980122 ) ) ;
#70725=CARTESIAN_POINT ( 'NONE',  ( 22.50049573229999922, 1409.698795012430082, 211.8242440451179789 ) ) ;
#70726=B_SPLINE_SURFACE_WITH_KNOTS ( 'NONE', 5, 5, ( 
 ( #2490, #55088, #89216, #72435, #106029, #63502 ),
 ( #37166, #38252, #87578, #98156, #89761, #95963 ),
 ( #71361, #53431, #80820, #13032, #88132, #104921 ),
 ( #46144, #46689, #88681, #47220, #20890, #29853 ),
 ( #81346, #11958, #36068, #19224, #105474, #37712 ),
 ( #28762, #97622, #10866, #79183, #28206, #4127 ) ),
 .UNSPECIFIED., .F., .F., .F.,
 ( 6, 6 ),
 ( 6, 6 ),
 ( 30.32814665369999929, 157.7108139869999945 ),
 ( -1.942890293099999814E-16, 1.000000000000000000 ),
 .UNSPECIFIED. ) ;
#70727=CARTESIAN_POINT ( 'NONE',  ( -12.89608512423069975, 1434.724840024559853, 149.2206170422699927 ) ) ;
#70729=CARTESIAN_POINT ( 'NONE',  ( -5.360152366205530150, 1422.242722016050038, 144.1549655170190078 ) ) ;
#70730=CARTESIAN_POINT ( 'NONE',  ( -11.30788591870000204, 1432.727006032190047, 151.5212569347980036 ) ) ;
#70732=CARTESIAN_POINT ( 'NONE',  ( 1.069243730569999995, 1410.308942135029838, 232.9260189513979924 ) ) ;
#70735=CARTESIAN_POINT ( 'NONE',  ( -23.09493868299999875, 1420.935639543630032, 211.5389171420879961 ) ) ;
#70740=CARTESIAN_POINT ( 'NONE',  ( -21.78276816909999880, 1430.096355600930110, 220.5348153272979914 ) ) ;
#70741=CARTESIAN_POINT ( 'NONE',  ( -19.06789788857610191, 1485.490801430430110, 189.6154567045299757 ) ) ;
#70742=CARTESIAN_POINT ( 'NONE',  ( -4.255035861773739825, 1441.293950967729870, 160.2601193279770087 ) ) ;
#70746=CARTESIAN_POINT ( 'NONE',  ( 11.93532877116399860, 1433.536986264360166, 150.1921723446900216 ) ) ;
#70747=CARTESIAN_POINT ( 'NONE',  ( 26.60746491089999921, 1509.169831192730044, 216.8088406937480102 ) ) ;
#70752=CARTESIAN_POINT ( 'NONE',  ( 13.79159911834929986, 1453.017954755449864, 224.3209708394340112 ) ) ;
#70753=CARTESIAN_POINT ( 'NONE',  ( 11.91321771470000002, 1435.943783413959864, 147.6429393588979906 ) ) ;
#70756=CARTESIAN_POINT ( 'NONE',  ( -24.29770167611630072, 1452.000795570500031, 137.1838091970490154 ) ) ;
#70757=CARTESIAN_POINT ( 'NONE',  ( 10.65455282579233298, 1438.738895160811580, 152.5347921806118734 ) ) ;
#70758=CARTESIAN_POINT ( 'NONE',  ( 14.78239737450000035, 1410.801796610830252, 227.6257754451980020 ) ) ;
#70760=CARTESIAN_POINT ( 'NONE',  ( 40.71250048023939883, 1447.497876396469792, 134.0999999984609872 ) ) ;
#70763=CARTESIAN_POINT ( 'NONE',  ( 5425.877333011740120, 54.28084071072822780, 8448.741457639642249 ) ) ;
#70765=CARTESIAN_POINT ( 'NONE',  ( 13.90749792064180035, 1435.812708943650023, 150.1213536925990297 ) ) ;
#70766=EDGE_CURVE ( 'NONE', #110254, #78256, #1335, .T. ) ;
#70770=ORIENTED_EDGE ( 'NONE', *, *, #83601, .T. ) ;
#70772=CARTESIAN_POINT ( 'NONE',  ( -0.6774325393469999845, 1465.095555782530027, 238.0673157071979915 ) ) ;
#70778=CARTESIAN_POINT ( 'NONE',  ( 4.222531898828509433, 1446.229786520979815, 170.5365406785500113 ) ) ;
#70783=CARTESIAN_POINT ( 'NONE',  ( 23.65006834624189835, 1440.913060387330006, 234.3338484623149895 ) ) ;
#70784=CARTESIAN_POINT ( 'NONE',  ( -8.586954633810537876E-06, 1452.913060687297275, 152.6867136803564335 ) ) ;
#70785=ADVANCED_FACE ( 'NONE', ( #1986 ), #23959, .F. ) ;
#70787=CARTESIAN_POINT ( 'NONE',  ( 26.10257120823780141, 1450.811424229450040, 136.5821829170589865 ) ) ;
#70788=CARTESIAN_POINT ( 'NONE',  ( -14.27637756340000053, 1410.784304046130046, 190.3513780643979771 ) ) ;
#70790=CARTESIAN_POINT ( 'NONE',  ( -24.67346689489999889, 1441.307773655729761, 210.6971997129480201 ) ) ;
#70793=CARTESIAN_POINT ( 'NONE',  ( -18.89959486414000267, 1416.839692127460012, 207.5749783441650038 ) ) ;
#70795=CARTESIAN_POINT ( 'NONE',  ( -11.94116563470000081, 1433.615379977029988, 149.2721031343980087 ) ) ;
#70798=CARTESIAN_POINT ( 'NONE',  ( 4.561144869889999676, 1466.058506330530008, 233.9063445751979771 ) ) ;
#70813=CARTESIAN_POINT ( 'NONE',  ( 31.95512683039999757, 1440.913060382470121, 244.1805851198980122 ) ) ;
#70816=CARTESIAN_POINT ( 'NONE',  ( 2.921131793919999886, 1415.930151872029910, 231.8786077231980016 ) ) ;
#70817=ADVANCED_FACE ( 'NONE', ( #63018 ), #9737, .T. ) ;
#70818=CARTESIAN_POINT ( 'NONE',  ( -19.22340757710000148, 1456.313295594730107, 227.1916260328980002 ) ) ;
#70819=CARTESIAN_POINT ( 'NONE',  ( 11.87111128170000107, 1432.721370721239964, 150.3961584458980099 ) ) ;
#70820=CARTESIAN_POINT ( 'NONE',  ( 19.24165877509999945, 1455.917582588630239, 226.0685302825979761 ) ) ;
#70821=CARTESIAN_POINT ( 'NONE',  ( 0.04599154778319999859, 1434.818091166349859, 190.1711483882980076 ) ) ;
#70825=CARTESIAN_POINT ( 'NONE',  ( 1.333571497619999935, 1405.789322411930016, 268.4830616106980301 ) ) ;
#70829=CARTESIAN_POINT ( 'NONE',  ( 30.41063212992060372, 1463.807241927210043, 269.9433037886050215 ) ) ;
#70830=CARTESIAN_POINT ( 'NONE',  ( 5.388168580889999504, 1432.635621093390000, 154.6140392605979912 ) ) ;
#70832=CARTESIAN_POINT ( 'NONE',  ( -36.99862439799500180, 1440.913060387569885, 254.6224166283950296 ) ) ;
#70833=CARTESIAN_POINT ( 'NONE',  ( 36.42198593292390285, 1449.840865744850134, 136.2602280137270157 ) ) ;
#70834=CARTESIAN_POINT ( 'NONE',  ( 2.397204011594943118, 1449.532271010019485, 154.4508081864954647 ) ) ;
#70837=CARTESIAN_POINT ( 'NONE',  ( 25.00977876991279913, 1436.598012848749931, 137.9330263815630246 ) ) ;
#70841=VERTEX_POINT ( 'NONE', #53486 ) ;
#70844=LINE ( 'NONE', #104953, #88498 ) ;
#70845=CARTESIAN_POINT ( 'NONE',  ( -0.2162292962460000134, 1476.076401974029977, 267.5371521268979791 ) ) ;
#70846=CARTESIAN_POINT ( 'NONE',  ( 10.85845406881951192, 1424.793774302243946, 138.1921923613813590 ) ) ;
#70847=CARTESIAN_POINT ( 'NONE',  ( 15.05358514859999985, 1410.831827802429871, 191.5175413050980069 ) ) ;
#70848=CARTESIAN_POINT ( 'NONE',  ( -3.012147942673290224, 1448.270564837731172, 184.4771857188410138 ) ) ;
#70850=CARTESIAN_POINT ( 'NONE',  ( -17.39559652730000039, 1414.988017874730076, 207.6227087713480159 ) ) ;
#70852=CARTESIAN_POINT ( 'NONE',  ( 26.60255046156829906, 1435.426458939230088, 135.2844108396259912 ) ) ;
#70853=CARTESIAN_POINT ( 'NONE',  ( -10.98175438394980041, 1396.296551700780128, 210.5364588383239948 ) ) ;
#70854=CARTESIAN_POINT ( 'NONE',  ( -15.97230427090000049, 1420.722880863429964, 227.0315165930979902 ) ) ;
#70855=CARTESIAN_POINT ( 'NONE',  ( -16.48341284556989805, 1409.589363928740113, 225.5757014958979880 ) ) ;
#70856=CARTESIAN_POINT ( 'NONE',  ( 9.675350337739999418, 1433.447543843880112, 148.7453054530979841 ) ) ;
#70859=CARTESIAN_POINT ( 'NONE',  ( 1.899651985450000025, 1408.979397696429942, 230.3912746812980004 ) ) ;
#70860=CARTESIAN_POINT ( 'NONE',  ( -5.350997755189996319, 1484.262300443630920, 183.6825286484975095 ) ) ;
#70861=CARTESIAN_POINT ( 'NONE',  ( 10.51778671589999803, 1425.368423570830146, 103.4445267086979925 ) ) ;
#70863=CARTESIAN_POINT ( 'NONE',  ( -15.99169327979993405, 1409.471481020725832, 225.2129679076976174 ) ) ;
#70868=CARTESIAN_POINT ( 'NONE',  ( 5.496790702980000276, 1508.067699050229976, 181.8679897695980117 ) ) ;
#70875=CIRCLE ( 'NONE', #97618, 28.41070217520000440 ) ;
#70877=CARTESIAN_POINT ( 'NONE',  ( -14.68857900839999964, 1409.425996869029859, 192.2200297474979891 ) ) ;
#70878=CARTESIAN_POINT ( 'NONE',  ( 3.820260774390000039E-10, 1453.313060387329870, 228.7984261690980077 ) ) ;
#70881=CARTESIAN_POINT ( 'NONE',  ( -2.056488256989999819, 1486.374418793230006, 181.7138485504979997 ) ) ;
#70884=CARTESIAN_POINT ( 'NONE',  ( 22.47142205740000165, 1410.193803466230065, 206.7884343312579745 ) ) ;
#70885=CARTESIAN_POINT ( 'NONE',  ( 35.07271181893440826, 1436.204584066430016, 136.2659483677949765 ) ) ;
#70886=CARTESIAN_POINT ( 'NONE',  ( 8.750394133592571677, 1396.218630886179881, 215.8835450990220295 ) ) ;
#70887=CARTESIAN_POINT ( 'NONE',  ( 12.20862189049999991, 1408.016881114429907, 215.8065031030079979 ) ) ;
#70888=CARTESIAN_POINT ( 'NONE',  ( 5.741649384740319799E-05, 1405.716795532820015, 267.8539894883900274 ) ) ;
#70889=CARTESIAN_POINT ( 'NONE',  ( 41.65810716170000205, 1443.954329772089977, 135.6863066689980144 ) ) ;
#70891=CARTESIAN_POINT ( 'NONE',  ( -11.57667674939999891, 1432.352206966570066, 151.1966745221979807 ) ) ;
#70892=CARTESIAN_POINT ( 'NONE',  ( 12.36054334989999859, 1442.536702532669779, 187.4076687437979842 ) ) ;
#70902=B_SPLINE_CURVE_WITH_KNOTS ( 'NONE', 5,
 ( #76727, #85666, #66157, #15681, #68357, #83460 ),
 .UNSPECIFIED., .F., .F.,
 ( 6, 6 ),
 ( 0.000000000000000000, 1.000000000000000000 ),
 .UNSPECIFIED. ) ;
#70905=CARTESIAN_POINT ( 'NONE',  ( -21.43608950620000186, 1440.913060387330006, 225.1375979974980055 ) ) ;
#70906=EDGE_CURVE ( 'NONE', #94116, #8387, #105934, .T. ) ;
#70909=CARTESIAN_POINT ( 'NONE',  ( -7.764017288770000746, 1409.184185845429965, 229.1854234257980067 ) ) ;
#70911=CARTESIAN_POINT ( 'NONE',  ( -4.219438975460000130, 1446.230224810899927, 183.1418051739979944 ) ) ;
#70913=CARTESIAN_POINT ( 'NONE',  ( 2.500020115319840031, 1419.382923540379807, 144.1035841389490031 ) ) ;
#70914=CARTESIAN_POINT ( 'NONE',  ( -25.61448129076210023, 1440.913060494739966, 219.7488153746120076 ) ) ;
#70916=CARTESIAN_POINT ( 'NONE',  ( -2.105916231296855123, 1485.584842600218508, 182.5101088624064403 ) ) ;
#70917=FACE_OUTER_BOUND ( 'NONE', #9560, .T. ) ;
#70918=CARTESIAN_POINT ( 'NONE',  ( -25.54523398509999765, 1435.396131125720103, 135.6579912344979846 ) ) ;
#70919=EDGE_CURVE ( 'NONE', #99476, #24021, #93784, .T. ) ;
#70920=CARTESIAN_POINT ( 'NONE',  ( 43.61871776674129819, 1431.697620533069994, 269.9278503807960305 ) ) ;
#70924=CARTESIAN_POINT ( 'NONE',  ( -8.855566472366772857, 1426.236804904744531, 225.2812767048452827 ) ) ;
#70930=CARTESIAN_POINT ( 'NONE',  ( -6.530923115290000247, 1417.905666013130030, 231.6298835945980272 ) ) ;
#70932=ORIENTED_EDGE ( 'NONE', *, *, #21307, .T. ) ;
#70934=FACE_OUTER_BOUND ( 'NONE', #55956, .T. ) ;
#70935=CARTESIAN_POINT ( 'NONE',  ( 14.75922108689939982, 1469.003854007090240, 230.4826721581509901 ) ) ;
#70936=CARTESIAN_POINT ( 'NONE',  ( -23.77573081741120120, 1509.051567791879961, 223.4963634714729892 ) ) ;
#70937=DIRECTION ( 'NONE',  ( 0.000000000000000000, 1.000000000000000000, 0.000000000000000000 ) ) ;
#70938=CARTESIAN_POINT ( 'NONE',  ( -0.1886782460270000072, 1409.088270590330012, 232.6670924473980051 ) ) ;
#70939=CARTESIAN_POINT ( 'NONE',  ( 2.797255426280000012, 1417.697071498429978, 234.5789349732979758 ) ) ;
#70941=CARTESIAN_POINT ( 'NONE',  ( 14.68195088934960069, 1451.730267658390176, 195.2572681451519827 ) ) ;
#70943=EDGE_LOOP ( 'NONE', ( #39022, #78853, #14323, #65618 ) ) ;
#70944=CARTESIAN_POINT ( 'NONE',  ( -11.99589392261009912, 1415.088136167450102, 197.0938743475270201 ) ) ;
#70945=EDGE_CURVE ( 'NONE', #106239, #58739, #37699, .T. ) ;
#70958=CARTESIAN_POINT ( 'NONE',  ( -18.57722710470000038, 1435.146103754619844, 144.7442513582979871 ) ) ;
#70960=CARTESIAN_POINT ( 'NONE',  ( -3.171072485709999889, 1451.871858332230204, 182.7750508701979868 ) ) ;
#70961=CARTESIAN_POINT ( 'NONE',  ( 1.356545997123550062, 1410.335726221229834, 232.6398861002840022 ) ) ;
#70962=CARTESIAN_POINT ( 'NONE',  ( -14.38276615813130022, 1509.537722091349906, 182.7943691049900110 ) ) ;
#70965=CARTESIAN_POINT ( 'NONE',  ( 1.552473713816009848, 1415.666200589839946, 190.6769660270060172 ) ) ;
#70966=CARTESIAN_POINT ( 'NONE',  ( 22.65374460030000137, 1411.052683168629983, 206.6971487888179979 ) ) ;
#70967=CARTESIAN_POINT ( 'NONE',  ( -24.16028618640000047, 1437.513346555010003, 211.1466462160479978 ) ) ;
#70969=DIRECTION ( 'NONE',  ( 0.000000000000000000, 0.000000000000000000, -1.000000000000000000 ) ) ;
#70970=CARTESIAN_POINT ( 'NONE',  ( -2.580627846919146595, 1425.957731743932754, 184.7531624060546562 ) ) ;
#70972=CARTESIAN_POINT ( 'NONE',  ( -24.89623166663279719, 1440.854217278560100, 210.4275088599499952 ) ) ;
#70975=VECTOR ( 'NONE', #30336, 1000.000000000000114 ) ;
#70981=CARTESIAN_POINT ( 'NONE',  ( 22.33903000980000186, 1509.718431408929973, 189.5993525853980088 ) ) ;
#70988=CARTESIAN_POINT ( 'NONE',  ( 26.51636468996370155, 1480.769270085010021, 207.6884295754969969 ) ) ;
#70990=CARTESIAN_POINT ( 'NONE',  ( 12.72540794655758489, 1442.818196233205981, 169.4573749914120526 ) ) ;
#70991=CARTESIAN_POINT ( 'NONE',  ( 34.89652595409791047, 1423.938945117018648, 269.5300863509276041 ) ) ;
#70992=CARTESIAN_POINT ( 'NONE',  ( -39.71667984149999597, 1440.913060391189902, 259.0958842013980075 ) ) ;
#70994=CARTESIAN_POINT ( 'NONE',  ( -11.11051595620000043, 1433.900636542000029, 151.6798721210980148 ) ) ;
#70996=CARTESIAN_POINT ( 'NONE',  ( -18.99761857140000032, 1485.804004457929977, 189.5282822598980204 ) ) ;
#70997=CARTESIAN_POINT ( 'NONE',  ( 5.275011299300000012, 1410.472427662630025, 186.4709616624980129 ) ) ;
#70998=CARTESIAN_POINT ( 'NONE',  ( 5.036045094249999465, 1422.685027075830021, 184.4684357060980062 ) ) ;
#71000=CARTESIAN_POINT ( 'NONE',  ( 7.765022045919999449, 1439.035228149790100, 153.8379896983980188 ) ) ;
#71007=CARTESIAN_POINT ( 'NONE',  ( -13.09237183259999959, 1470.597673365530227, 270.0792996520979727 ) ) ;
#71009=CARTESIAN_POINT ( 'NONE',  ( 3.329166574300000292, 1441.604926038239910, 155.7074624611979914 ) ) ;
#71010=CARTESIAN_POINT ( 'NONE',  ( -15.27799311270000082, 1485.037650874329984, 224.0147209149980085 ) ) ;
#71012=CARTESIAN_POINT ( 'NONE',  ( -13.16208950729999927, 1420.370919692029929, 228.2271380253979771 ) ) ;
#71016=CARTESIAN_POINT ( 'NONE',  ( -45.31040329346470230, 1436.802911717760026, 268.9839291206840244 ) ) ;
#71017=CARTESIAN_POINT ( 'NONE',  ( -4.148575093039999828, 1428.755514565529893, 185.9890542076980182 ) ) ;
#71020=ORIENTED_EDGE ( 'NONE', *, *, #62096, .F. ) ;
#71023=CARTESIAN_POINT ( 'NONE',  ( -20.61542114839999940, 1508.364347659730129, 190.3921826406979960 ) ) ;
#71024=CARTESIAN_POINT ( 'NONE',  ( -13.78890751930000036, 1425.417061756730163, 189.3862953465980183 ) ) ;
#71028=DIRECTION ( 'NONE',  ( 1.000000000000000000, 0.000000000000000000, 0.000000000000000000 ) ) ;
#71030=B_SPLINE_CURVE_WITH_KNOTS ( 'NONE', 3,
 ( #9823, #71441, #80349, #30482, #20963, #97145, #37795, #88750, #20413, #12586, #28843, #14225, #73617, #29924, #46767, #89291, #81418, #107745, #80897, #12034, #64115, #4729, #98236, #46215, #22598 ),
 .UNSPECIFIED., .F., .F.,
 ( 4, 3, 3, 3, 3, 3, 3, 3, 4 ),
 ( -42.69308751009999980, -41.31664050871439997, -39.51470315257619603, -37.85453691144520150, -36.24168671189359969, -34.73070981842659677, -33.26220518797870085, -31.82994285059310258, -30.44684653110000028 ),
 .UNSPECIFIED. ) ;
#71034=EDGE_LOOP ( 'NONE', ( #102401, #29078, #75354, #15310, #58901 ) ) ;
#71035=CARTESIAN_POINT ( 'NONE',  ( -16.97136689889709871, 1410.626141966220075, 270.3495370215860021 ) ) ;
#71037=CARTESIAN_POINT ( 'NONE',  ( -0.7904366496569998901, 1426.935925255829943, 133.6118001900980232 ) ) ;
#71041=ORIENTED_EDGE ( 'NONE', *, *, #74078, .T. ) ;
#71042=CARTESIAN_POINT ( 'NONE',  ( 45.63562816159383573, 1441.199288540710768, 268.9747940734181384 ) ) ;
#71044=CARTESIAN_POINT ( 'NONE',  ( -9.066449906558435856, 1440.400147515658091, 153.5443354344916145 ) ) ;
#71045=CARTESIAN_POINT ( 'NONE',  ( -15.46200339894285847, 1407.981780703992172, 266.8670517912573246 ) ) ;
#71047=CARTESIAN_POINT ( 'NONE',  ( -18.45097462037960057, 1415.673583075490114, 207.5694314020479965 ) ) ;
#71048=CARTESIAN_POINT ( 'NONE',  ( -18.09906091010000040, 1435.779564141970013, 226.5701799449980172 ) ) ;
#71049=EDGE_CURVE ( 'NONE', #109427, #17632, #33755, .T. ) ;
#71050=CARTESIAN_POINT ( 'NONE',  ( 15.79251552625780164, 1474.064138637460019, 266.8741674170499891 ) ) ;
#71051=CARTESIAN_POINT ( 'NONE',  ( 12.07588402680000073, 1415.579607678529783, 223.1679904141980160 ) ) ;
#71055=CARTESIAN_POINT ( 'NONE',  ( 20.68010504029316010, 1410.996119301493081, 218.7905024334752113 ) ) ;
#71056=CARTESIAN_POINT ( 'NONE',  ( 1.503770822449239875, 1464.070697699469974, 182.9916286601730064 ) ) ;
#71057=ORIENTED_EDGE ( 'NONE', *, *, #30538, .T. ) ;
#71059=CARTESIAN_POINT ( 'NONE',  ( 25.24320764742720158, 1451.875638110379896, 136.2233328636380350 ) ) ;
#71060=EDGE_CURVE ( 'NONE', #41855, #10196, #83111, .T. ) ;
#71064=CARTESIAN_POINT ( 'NONE',  ( 17.85287820219999944, 1409.701424983430115, 194.3066436361979754 ) ) ;
#71066=CARTESIAN_POINT ( 'NONE',  ( 3.351449279187751262, 1439.689399315149558, 184.4071940306241117 ) ) ;
#71067=CARTESIAN_POINT ( 'NONE',  ( -19.82422479395705750, 1426.129180672527127, 222.7993382114829046 ) ) ;
#71078=CARTESIAN_POINT ( 'NONE',  ( -37.93102824555499808, 1448.882024444920035, 136.3724781078850015 ) ) ;
#71081=CARTESIAN_POINT ( 'NONE',  ( -14.35418281379999961, 1450.996202461129997, 214.3676144195279676 ) ) ;
#71083=CARTESIAN_POINT ( 'NONE',  ( 11.85425778610000158, 1433.048935507500119, 150.3174848872980078 ) ) ;
#71084=CARTESIAN_POINT ( 'NONE',  ( -4.761695837242630347, 1473.992865699130107, 270.1327791948820050 ) ) ;
#71085=CARTESIAN_POINT ( 'NONE',  ( 25.63907149821320175, 1440.913060399049982, 219.8810537515410033 ) ) ;
#71086=CARTESIAN_POINT ( 'NONE',  ( -20.33900532369999681, 1508.016036090129774, 228.6619146254979853 ) ) ;
#71089=CARTESIAN_POINT ( 'NONE',  ( -27.59578990780000041, 1509.876726736629962, 201.0523533628679616 ) ) ;
#71090=CARTESIAN_POINT ( 'NONE',  ( 24.93050294115990795, 1436.289034237693386, 137.8926071792222672 ) ) ;
#71092=CARTESIAN_POINT ( 'NONE',  ( 22.71325450959999870, 1409.706218420429877, 209.2588089802279967 ) ) ;
#71093=CARTESIAN_POINT ( 'NONE',  ( 7.590703170876726524, 1398.138570740227351, 198.5570256807006047 ) ) ;
#71094=CARTESIAN_POINT ( 'NONE',  ( 2.630527005430000287, 1490.916590196630068, 235.2555692320979972 ) ) ;
#71095=CARTESIAN_POINT ( 'NONE',  ( 24.85895335929999916, 1430.362482292330014, 209.8091488686460195 ) ) ;
#71101=CARTESIAN_POINT ( 'NONE',  ( 2.499936552876079965, 1420.115363462959976, 90.95688517979088772 ) ) ;
#71106=CARTESIAN_POINT ( 'NONE',  ( -0.5623043548920000356, 1416.835809830829930, 227.7680352835980102 ) ) ;
#71109=CARTESIAN_POINT ( 'NONE',  ( -36.72650137420430383, 1451.114006374390101, 134.0999999987039644 ) ) ;
#71112=ORIENTED_EDGE ( 'NONE', *, *, #73287, .F. ) ;
#71114=CARTESIAN_POINT ( 'NONE',  ( -17.76192429420000352, 1416.216739748429973, 211.9674486285379942 ) ) ;
#71116=CARTESIAN_POINT ( 'NONE',  ( 23.55087631299999984, 1411.110694763729953, 207.7642880164279973 ) ) ;
#71117=B_SPLINE_CURVE_WITH_KNOTS ( 'NONE', 3,
 ( #84384, #32864, #6578, #22793, #8209, #59206, #23903, #32335, #100618, #7671, #67055, #65404 ),
 .UNSPECIFIED., .F., .F.,
 ( 4, 2, 2, 2, 2, 4 ),
 ( 4.496430354704500113E-15, 9.667223565493732152E-05, 0.0001933444713053782127, 0.0003866889426061961626, 0.0007733778852078835621, 0.001546755770410726451 ),
 .UNSPECIFIED. ) ;
#71121=CARTESIAN_POINT ( 'NONE',  ( 13.89024821118459840, 1409.398118541669874, 214.6073209033960154 ) ) ;
#71122=DIRECTION ( 'NONE',  ( 1.000000000000000000, 0.000000000000000000, 0.000000000000000000 ) ) ;
#71124=CARTESIAN_POINT ( 'NONE',  ( -17.67056496260000031, 1412.978053172430009, 193.3746425421979893 ) ) ;
#71127=CARTESIAN_POINT ( 'NONE',  ( 3.034148894259999896, 1440.440283194090171, 157.2495476715980089 ) ) ;
#71130=CARTESIAN_POINT ( 'NONE',  ( -12.25049518321329955, 1416.576002138870081, 194.6830814986430198 ) ) ;
#71131=CARTESIAN_POINT ( 'NONE',  ( -11.99985923319999870, 1433.681662988860126, 149.8469377335979971 ) ) ;
#71132=CARTESIAN_POINT ( 'NONE',  ( 16.66598991933063445, 1468.916255155639874, 269.3720935231359022 ) ) ;
#71134=CARTESIAN_POINT ( 'NONE',  ( 1.233953280850000001, 1397.950740760129975, 222.1299377637979831 ) ) ;
#71137=CARTESIAN_POINT ( 'NONE',  ( -19.02802488173782081, 1486.252467685796091, 189.3493767970001898 ) ) ;
#71142=CARTESIAN_POINT ( 'NONE',  ( -13.18323158269999951, 1435.197366603820001, 150.1160888488979879 ) ) ;
#71143=CARTESIAN_POINT ( 'NONE',  ( 18.16369802799999889, 1409.547350699329854, 196.7220820877979861 ) ) ;
#71144=CARTESIAN_POINT ( 'NONE',  ( -18.70459388414779767, 1509.566239243649989, 231.7064163625079800 ) ) ;
#71148=CARTESIAN_POINT ( 'NONE',  ( 45.67178420940000194, 1438.126719075119809, 266.1886048709980059 ) ) ;
#71149=CARTESIAN_POINT ( 'NONE',  ( -21.80621300580000010, 1469.235547604329895, 196.1136359960979973 ) ) ;
#71150=CARTESIAN_POINT ( 'NONE',  ( -10.97801989845739890, 1426.061463023469742, 97.52402582803289022 ) ) ;
#71151=CARTESIAN_POINT ( 'NONE',  ( 13.56343219680000090, 1416.311719779230089, 196.3989970432979817 ) ) ;
#71154=CARTESIAN_POINT ( 'NONE',  ( -32.79493994580000304, 1434.501496568330140, 248.1152222149979991 ) ) ;
#71156=CARTESIAN_POINT ( 'NONE',  ( 3.183012419607803345, 1447.433753094939448, 154.8412150998025538 ) ) ;
#71157=DIRECTION ( 'NONE',  ( 0.3363363969981663093, 0.6659120918162475533, -0.6659120918163308200 ) ) ;
#71159=CARTESIAN_POINT ( 'NONE',  ( -5.385828860609489510, 1432.197383170389912, 154.6045697296559922 ) ) ;
#71161=CARTESIAN_POINT ( 'NONE',  ( -15.36439361150980076, 1376.113480921259907, 247.8666525594929908 ) ) ;
#71168=CARTESIAN_POINT ( 'NONE',  ( -0.1626181647790000129, 1421.812182938429942, 227.5856863222980166 ) ) ;
#71171=VECTOR ( 'NONE', #222, 1000.000000000000114 ) ;
#71172=CARTESIAN_POINT ( 'NONE',  ( -0.3264474814539999881, 1470.489006557829953, 235.7562541381980168 ) ) ;
#71173=CARTESIAN_POINT ( 'NONE',  ( 1.923719469800590165, 1421.100103055099908, 183.1407590705949815 ) ) ;
#71174=ORIENTED_EDGE ( 'NONE', *, *, #66493, .F. ) ;
#71176=CARTESIAN_POINT ( 'NONE',  ( 11.63658410760000095, 1425.864915301529891, 144.1607460163980079 ) ) ;
#71178=CARTESIAN_POINT ( 'NONE',  ( 15.59042067260000053, 1507.631725826930051, 225.7583918763980080 ) ) ;
#71182=CARTESIAN_POINT ( 'NONE',  ( 11.86235724903239941, 1432.074504238270038, 149.9760656271810149 ) ) ;
#71186=CARTESIAN_POINT ( 'NONE',  ( -1.447759218079930132, 1462.381657541340019, 183.4226446050429900 ) ) ;
#71187=CARTESIAN_POINT ( 'NONE',  ( -13.51610093809999924, 1443.913060387330006, 169.3501091259980171 ) ) ;
#71188=CARTESIAN_POINT ( 'NONE',  ( 3.048828140119999919, 1509.019527812029992, 237.9289388369980145 ) ) ;
#71190=CARTESIAN_POINT ( 'NONE',  ( -4.363116875470000267, 1423.854803018830125, 184.2545991611980014 ) ) ;
#71191=CARTESIAN_POINT ( 'NONE',  ( 3.056876074108880292, 1410.319324463180010, 269.6158940089480325 ) ) ;
#71204=CARTESIAN_POINT ( 'NONE',  ( 38.34143784940000188, 1436.524347965420020, 265.6112251771979800 ) ) ;
#71206=CARTESIAN_POINT ( 'NONE',  ( 41.15110440228482958, 1443.645438857304953, 136.9181504661874840 ) ) ;
#71207=B_SPLINE_CURVE_WITH_KNOTS ( 'NONE', 3,
 ( #30988, #108247, #56201, #108802, #13613, #56758, #15272, #81936, #91456, #64623, #14178, #5239, #99834, #83586, #48923, #13066, #48365, #98744, #4691 ),
 .UNSPECIFIED., .F., .F.,
 ( 4, 3, 3, 3, 3, 3, 4 ),
 ( -1.403944690730000167, -1.188125015481449998, -0.9636848121176839754, -0.7385352318536739791, -0.5129228707660121733, -0.2865928050055470688, -0.05981740377519995100 ),
 .UNSPECIFIED. ) ;
#71211=CARTESIAN_POINT ( 'NONE',  ( 43.70825229526830213, 1428.337867259879886, 269.0264340981559599 ) ) ;
#71213=VERTEX_POINT ( 'NONE', #61762 ) ;
#71215=CARTESIAN_POINT ( 'NONE',  ( -24.39954769610000085, 1443.080901239500008, 211.1504982047080148 ) ) ;
#71216=CARTESIAN_POINT ( 'NONE',  ( -1.600048698852036821, 1411.254281879943164, 135.5999999980979851 ) ) ;
#71219=CARTESIAN_POINT ( 'NONE',  ( -12.10873113499999931, 1442.495059057370099, 187.0567141033980079 ) ) ;
#71220=CARTESIAN_POINT ( 'NONE',  ( 21.71631475791559751, 1509.710815674639889, 229.8179829200470010 ) ) ;
#71222=CARTESIAN_POINT ( 'NONE',  ( 12.28535814839943541, 1434.206754551802078, 149.6317592098948808 ) ) ;
#71223=CARTESIAN_POINT ( 'NONE',  ( 14.57860324780000028, 1417.424410125430086, 228.0517902003980169 ) ) ;
#71226=CIRCLE ( 'NONE', #37226, 1.999999999999957589 ) ;
#71227=CARTESIAN_POINT ( 'NONE',  ( -16.12699268032000077, 1459.080750933630043, 229.9878372279760015 ) ) ;
#71229=CARTESIAN_POINT ( 'NONE',  ( 39.35535942429999778, 1422.520539079029959, 268.7089579441980050 ) ) ;
#71230=CARTESIAN_POINT ( 'NONE',  ( -18.81215439969999892, 1410.493119616930244, 223.2931733231980047 ) ) ;
#71231=CARTESIAN_POINT ( 'NONE',  ( 17.05308463140000086, 1435.093823673100133, 146.1608047648980175 ) ) ;
#71232=CARTESIAN_POINT ( 'NONE',  ( 20.43733526010000290, 1469.157605011630039, 192.7233812162979802 ) ) ;
#71233=CARTESIAN_POINT ( 'NONE',  ( 5.362419220542090414, 1424.201140997230141, 150.5224082514530153 ) ) ;
#71234=DIRECTION ( 'NONE',  ( 0.000000000000000000, 0.5259463573989414664, 0.8505177418130589473 ) ) ;
#71235=CARTESIAN_POINT ( 'NONE',  ( -44.47031351537230393, 1451.019434385626482, 266.2216429519685903 ) ) ;
#71238=CARTESIAN_POINT ( 'NONE',  ( -33.93525006893180063, 1435.841462747220021, 135.9408810291510008 ) ) ;
#71239=B_SPLINE_CURVE_WITH_KNOTS ( 'NONE', 5,
 ( #21116, #55321, #89453, #12746, #89996, #46928, #81046, #30082, #36290, #96765, #54230, #64276 ),
 .UNSPECIFIED., .F., .F.,
 ( 6, 3, 3, 6 ),
 ( 0.000000000000000000, 0.2739007385715113152, 0.6877721063829390635, 1.000000000000000000 ),
 .UNSPECIFIED. ) ;
#71240=DIRECTION ( 'NONE',  ( 0.000000000000000000, -1.000000000000000000, 0.000000000000000000 ) ) ;
#71241=CARTESIAN_POINT ( 'NONE',  ( -15.71890336570000102, 1414.913060387229962, 203.5737140920780064 ) ) ;
#71242=CARTESIAN_POINT ( 'NONE',  ( 22.70509004431190192, 1409.705939603270053, 209.2982552845940063 ) ) ;
#71244=CARTESIAN_POINT ( 'NONE',  ( 12.40455451780000118, 1434.419853495000098, 146.4343138086979934 ) ) ;
#71245=CARTESIAN_POINT ( 'NONE',  ( -30.19569412050000068, 1435.551785849099815, 135.1818641824980034 ) ) ;
#71247=ORIENTED_EDGE ( 'NONE', *, *, #20912, .T. ) ;
#71249=CARTESIAN_POINT ( 'NONE',  ( 39.87321672109999326, 1440.876652101590025, 136.8077108269980044 ) ) ;
#71251=VERTEX_POINT ( 'NONE', #70178 ) ;
#71253=DIRECTION ( 'NONE',  ( 0.000000000000000000, -1.000000000000000000, -2.312964634635740689E-15 ) ) ;
#71254=CARTESIAN_POINT ( 'NONE',  ( -4.897370105774945692, 1421.905084353634948, 138.0291448931159550 ) ) ;
#71255=CARTESIAN_POINT ( 'NONE',  ( -37.68243668920000289, 1461.704006605230006, 266.6693340566979487 ) ) ;
#71256=CARTESIAN_POINT ( 'NONE',  ( -13.42305729488690069, 1429.046643101820109, 222.2861133963140219 ) ) ;
#71258=CARTESIAN_POINT ( 'NONE',  ( 0.3556640921540570321, 1419.127793398659833, 184.6118934103729998 ) ) ;
#71264=CARTESIAN_POINT ( 'NONE',  ( 17.17404474450000151, 1416.216596894529857, 215.3726550198079792 ) ) ;
#71266=CARTESIAN_POINT ( 'NONE',  ( -9.443064477949999258, 1434.540978515130064, 153.1670680800980051 ) ) ;
#71271=EDGE_CURVE ( 'NONE', #54363, #5297, #45849, .T. ) ;
#71272=CARTESIAN_POINT ( 'NONE',  ( -23.89076775359999871, 1410.242936723630010, 208.6635434592330114 ) ) ;
#71273=ADVANCED_FACE ( 'NONE', ( #46615 ), #54541, .F. ) ;
#71279=EDGE_CURVE ( 'NONE', #48668, #45161, #40466, .T. ) ;
#71280=CARTESIAN_POINT ( 'NONE',  ( 23.45078998690000205, 1410.227208243830091, 211.3297003749379996 ) ) ;
#71282=ADVANCED_FACE ( 'NONE', ( #68370 ), #10662, .F. ) ;
#71285=CARTESIAN_POINT ( 'NONE',  ( -27.43355922089999765, 1507.980920696029898, 210.8261541407979962 ) ) ;
#71287=CARTESIAN_POINT ( 'NONE',  ( 1.071447408489999864, 1411.670163745530090, 232.9832474924979806 ) ) ;
#71290=CARTESIAN_POINT ( 'NONE',  ( -23.23815859999999844, 1425.880866807129905, 211.7841193188579894 ) ) ;
#71291=CARTESIAN_POINT ( 'NONE',  ( -1.499738582814070131, 1420.769031529490121, 184.5716992340250044 ) ) ;
#71293=CARTESIAN_POINT ( 'NONE',  ( 13.37370059936500155, 1507.528266836789953, 233.0489815920269905 ) ) ;
#71294=CARTESIAN_POINT ( 'NONE',  ( -16.37199061016699986, 1485.898763490840111, 187.4707436738999888 ) ) ;
#71300=CARTESIAN_POINT ( 'NONE',  ( 27.36865155859999987, 1509.161448955630021, 214.5593760264079890 ) ) ;
#71304=CARTESIAN_POINT ( 'NONE',  ( 15.82232452675290091, 1415.565885647649793, 191.3713869796289941 ) ) ;
#71305=CARTESIAN_POINT ( 'NONE',  ( 15.76326814482090199, 1409.463407968690035, 192.8551723846009907 ) ) ;
#71306=CARTESIAN_POINT ( 'NONE',  ( 11.86716023049999968, 1432.353341358199941, 147.6509521729980179 ) ) ;
#71307=EDGE_CURVE ( 'NONE', #96609, #100850, #79171, .T. ) ;
#71309=CARTESIAN_POINT ( 'NONE',  ( -25.40499604889999929, 1451.786406054930239, 136.2913176118979948 ) ) ;
#71311=CARTESIAN_POINT ( 'NONE',  ( 15.60951394679999993, 1410.830427143530187, 227.1466297419979696 ) ) ;
#71313=EDGE_CURVE ( 'NONE', #44698, #48553, #74267, .T. ) ;
#71314=CARTESIAN_POINT ( 'NONE',  ( 41.18215094353789851, 1440.963619928870003, 134.0999999980659823 ) ) ;
#71316=CARTESIAN_POINT ( 'NONE',  ( -0.5620977654635980203, 1416.851343899799986, 227.7685710128770040 ) ) ;
#71321=ORIENTED_EDGE ( 'NONE', *, *, #14450, .F. ) ;
#71326=CARTESIAN_POINT ( 'NONE',  ( 19.34610958727051155, 1451.004559698421644, 146.2861324281605278 ) ) ;
#71327=B_SPLINE_CURVE_WITH_KNOTS ( 'NONE', 5,
 ( #54696, #20486, #87168, #19389, #63650, #28363 ),
 .UNSPECIFIED., .F., .F.,
 ( 6, 6 ),
 ( 0.000000000000000000, 1.000000000000000000 ),
 .UNSPECIFIED. ) ;
#71328=CARTESIAN_POINT ( 'NONE',  ( -2.896892189909999971, 1484.263391075629897, 183.3160938871980079 ) ) ;
#71331=CARTESIAN_POINT ( 'NONE',  ( -3.827327205999999649, 1409.546157813730133, 146.1721969590979882 ) ) ;
#71332=CARTESIAN_POINT ( 'NONE',  ( 4.246950514239129504, 1446.447518977580103, 161.6227665976579715 ) ) ;
#71333=CARTESIAN_POINT ( 'NONE',  ( 0.3572670465939999929, 1508.337857058129885, 237.7796338305979873 ) ) ;
#71337=CARTESIAN_POINT ( 'NONE',  ( 32.06566495267949790, 1440.913060387330006, 256.0678710581919972 ) ) ;
#71340=CARTESIAN_POINT ( 'NONE',  ( -33.91369269983620427, 1450.440666099120108, 136.2454419983430114 ) ) ;
#71341=CARTESIAN_POINT ( 'NONE',  ( -13.97246758180000015, 1409.902985965229846, 190.4217242322980042 ) ) ;
#71343=CARTESIAN_POINT ( 'NONE',  ( -24.67000125460000248, 1440.968500227289951, 210.6876455135279969 ) ) ;
#71345=CARTESIAN_POINT ( 'NONE',  ( 22.53427855600670071, 1410.990232248750090, 206.1996399176450154 ) ) ;
#71347=CARTESIAN_POINT ( 'NONE',  ( 27.69925877688100258, 1441.434395746940027, 137.3015763641899980 ) ) ;
#71349=CARTESIAN_POINT ( 'NONE',  ( 18.17633956390000094, 1435.132278384110123, 145.0981326318980109 ) ) ;
#71350=CARTESIAN_POINT ( 'NONE',  ( 6.314283035290000790, 1463.997681713329939, 235.6565739224980121 ) ) ;
#71353=CIRCLE ( 'NONE', #40909, 1.999999999999942935 ) ;
#71356=CARTESIAN_POINT ( 'NONE',  ( 11.73653109249999993, 1426.280329148629789, 144.1709412064980143 ) ) ;
#71358=AXIS2_PLACEMENT_3D ( 'NONE', #67194, #52600, #87862 ) ;
#71359=CARTESIAN_POINT ( 'NONE',  ( 28.78960601649999873, 1509.588732904530161, 208.4412888571310134 ) ) ;
#71361=CARTESIAN_POINT ( 'NONE',  ( -20.71063674839999891, 1470.804162801530083, 208.8514674448739754 ) ) ;
#71362=( BOUNDED_CURVE ( )  B_SPLINE_CURVE ( 3, ( #4442, #47001, #22854, #57060 ),
 .UNSPECIFIED., .F., .F. ) 
 B_SPLINE_CURVE_WITH_KNOTS ( ( 4, 4 ),
 ( 3.464045754873669836, 3.751191316916064888 ),
 .UNSPECIFIED. ) 
 CURVE ( )  GEOMETRIC_REPRESENTATION_ITEM ( )  RATIONAL_B_SPLINE_CURVE ( ( 1.000000000000000000, 0.9931407469010118394, 0.9931407469010118394, 1.000000000000000000 ) ) 
 REPRESENTATION_ITEM ( '' )  );
#71367=CARTESIAN_POINT ( 'NONE',  ( 4.694071664390000009, 1465.143864797330025, 238.2947585048979988 ) ) ;
#71370=CARTESIAN_POINT ( 'NONE',  ( 11.22085813615770000, 1414.913060387329779, 197.6243702374680140 ) ) ;
#71371=CARTESIAN_POINT ( 'NONE',  ( -20.92345263760000051, 1454.438554760929946, 223.3898966321980026 ) ) ;
#71372=ADVANCED_FACE ( 'NONE', ( #106892 ), #91202, .T. ) ;
#71373=CARTESIAN_POINT ( 'NONE',  ( -21.53807511146743181, 1411.025645835263049, 201.1588749450977218 ) ) ;
#71374=CARTESIAN_POINT ( 'NONE',  ( 5.386491384805029980, 1432.359961415570069, 154.6077504147789909 ) ) ;
#71378=ORIENTED_EDGE ( 'NONE', *, *, #46258, .F. ) ;
#71380=CARTESIAN_POINT ( 'NONE',  ( 1.749310115339999916, 1406.801363622329973, 269.6491151137980182 ) ) ;
#71383=CARTESIAN_POINT ( 'NONE',  ( 39.57252994079590280, 1456.675038565810155, 270.2586952983279502 ) ) ;
#71384=CARTESIAN_POINT ( 'NONE',  ( -23.74108753817469974, 1436.296634041249945, 212.5883363871789982 ) ) ;
#71386=CARTESIAN_POINT ( 'NONE',  ( -42.90581327332729700, 1440.913060410159915, 263.0724741836789917 ) ) ;
#71387=ADVANCED_FACE ( 'NONE', ( #99036, #47018 ), #66589, .T. ) ;
#71388=CARTESIAN_POINT ( 'NONE',  ( -12.53380580351000084, 1442.773887400870080, 185.9733686700720057 ) ) ;
#71389=CARTESIAN_POINT ( 'NONE',  ( 1.367072583474315595, 1450.698607345994787, 154.2613738994832033 ) ) ;
#71390=DIRECTION ( 'NONE',  ( -0.09762373801881200908, -0.1163955094263306178, 0.9883934900436258664 ) ) ;
#71391=CARTESIAN_POINT ( 'NONE',  ( -1.218484030269072260, 1451.352790354969784, 183.4814141672358119 ) ) ;
#71394=EDGE_LOOP ( 'NONE', ( #47314, #49482, #29128, #96710 ) ) ;
#71395=CARTESIAN_POINT ( 'NONE',  ( -9.019386504720001696, 1419.938649402030023, 248.0989693098979956 ) ) ;
#71397=CARTESIAN_POINT ( 'NONE',  ( -1.328227237909999969, 1475.823473844229966, 266.9604901357979543 ) ) ;
#71399=CARTESIAN_POINT ( 'NONE',  ( -28.04656858090000071, 1508.051246290529889, 210.1181873726100093 ) ) ;
#71403=CARTESIAN_POINT ( 'NONE',  ( -17.86855543449999928, 1415.163755998629995, 207.5652616391579954 ) ) ;
#71406=CARTESIAN_POINT ( 'NONE',  ( 26.62473440929639779, 1435.447231379140021, 135.5572024620289824 ) ) ;
#71407=EDGE_CURVE ( 'NONE', #75744, #46325, #13390, .T. ) ;
#71408=CARTESIAN_POINT ( 'NONE',  ( -11.06075986596750127, 1396.299310633010236, 208.6759994649900136 ) ) ;
#71409=CARTESIAN_POINT ( 'NONE',  ( -15.64704939853400134, 1421.345936108949900, 227.1284707070510080 ) ) ;
#71411=CARTESIAN_POINT ( 'NONE',  ( -16.35500113143990220, 1409.585309854400066, 225.6783689361829772 ) ) ;
#71412=CARTESIAN_POINT ( 'NONE',  ( -45.49575511559999796, 1438.180874202940004, 268.9785913983979526 ) ) ;
#71417=CARTESIAN_POINT ( 'NONE',  ( -14.13260639439999977, 1484.576036422829930, 186.6695759715979932 ) ) ;
#71418=CARTESIAN_POINT ( 'NONE',  ( 11.41326510949999928, 1425.999523078630091, 128.4892991212979894 ) ) ;
#71420=CARTESIAN_POINT ( 'NONE',  ( -0.2816376222929999895, 1499.119349190730190, 236.9843354826979862 ) ) ;
#71422=EDGE_CURVE ( 'NONE', #90510, #99871, #82251, .T. ) ;
#71425=CARTESIAN_POINT ( 'NONE',  ( -4.882003189570000679, 1430.559178934629927, 150.0077195948979920 ) ) ;
#71426=CARTESIAN_POINT ( 'NONE',  ( 6.853204512189999598, 1508.129908978229878, 182.3155033407979886 ) ) ;
#71431=EDGE_CURVE ( 'NONE', #66206, #79432, #89850, .T. ) ;
#71435=CARTESIAN_POINT ( 'NONE',  ( -12.51070046275587266, 1447.046588421757406, 187.7237876303275641 ) ) ;
#71436=VECTOR ( 'NONE', #21625, 1000.000000000000000 ) ;
#71437=CARTESIAN_POINT ( 'NONE',  ( -15.94347048536829803, 1409.469818645040050, 192.9752432267480060 ) ) ;
#71438=DIRECTION ( 'NONE',  ( 0.3741247022715693538, 0.04424963817041901309, -0.9263221236006385917 ) ) ;
#71441=CARTESIAN_POINT ( 'NONE',  ( -1.367757481957880161, 1418.999489435819896, 185.2367492338790100 ) ) ;
#71442=CARTESIAN_POINT ( 'NONE',  ( 6.200576079530000229, 1429.764427576630169, 185.9200482557980081 ) ) ;
#71445=CARTESIAN_POINT ( 'NONE',  ( -2.500000000000000000, 1448.206577425080013, 168.0218890593559991 ) ) ;
#71446=CARTESIAN_POINT ( 'NONE',  ( -13.02571899038530567, 1435.353243946824477, 150.4465727419359951 ) ) ;
#71447=PLANE ( 'NONE',  #12246 ) ;
#71449=CARTESIAN_POINT ( 'NONE',  ( 0.000000000000000000, 1405.413060387330006, 209.1218459616979999 ) ) ;
#71453=ORIENTED_EDGE ( 'NONE', *, *, #51655, .F. ) ;
#71462=EDGE_LOOP ( 'NONE', ( #105335, #93156, #46779, #33148, #39293 ) ) ;
#71465=CARTESIAN_POINT ( 'NONE',  ( 12.26986170129999998, 1416.828040559629926, 223.5793159245980064 ) ) ;
#71467=CARTESIAN_POINT ( 'NONE',  ( -39.71894992190000551, 1440.913060387330006, 267.1764892454980327 ) ) ;
#71469=CARTESIAN_POINT ( 'NONE',  ( -4.331002755570000140, 1409.231591811829958, 231.5156777643979922 ) ) ;
#71472=CARTESIAN_POINT ( 'NONE',  ( -27.95545114004499965, 1508.164280454029949, 210.3124796796069802 ) ) ;
#71474=CARTESIAN_POINT ( 'NONE',  ( -1.808737572104399227, 1485.212291744892127, 182.6011977422664927 ) ) ;
#71476=CARTESIAN_POINT ( 'NONE',  ( 20.73365673480000027, 1411.792342831829956, 270.3294707265980037 ) ) ;
#71480=CARTESIAN_POINT ( 'NONE',  ( 0.01553491999268000710, 1507.764438927018546, 237.4914441325955465 ) ) ;
#71485=CARTESIAN_POINT ( 'NONE',  ( 4.199282754958249875, 1421.058089936039778, 185.3644816151839905 ) ) ;
#71486=CARTESIAN_POINT ( 'NONE',  ( -0.9715279139649999340, 1417.917963001030103, 233.3865104881980130 ) ) ;
#71490=CIRCLE ( 'NONE', #66113, 1.500000000000014433 ) ;
#71493=CARTESIAN_POINT ( 'NONE',  ( 12.81251879674629990, 1488.404633894339895, 232.3873005381080077 ) ) ;
#71495=CARTESIAN_POINT ( 'NONE',  ( 19.28393622879999825, 1507.737928638330004, 188.6540313642980209 ) ) ;
#71498=CARTESIAN_POINT ( 'NONE',  ( 2.715010028530000064, 1417.669881552329798, 234.6652376653979957 ) ) ;
#71506=CARTESIAN_POINT ( 'NONE',  ( -11.46637696920000060, 1485.913060386929828, 183.3557477887979985 ) ) ;
#71509=CARTESIAN_POINT ( 'NONE',  ( 3.835404308833624043, 1396.046995657106436, 216.1425064568209677 ) ) ;
#71513=CARTESIAN_POINT ( 'NONE',  ( -26.45794170912690291, 1508.569471461619969, 201.4995158287420054 ) ) ;
#71514=ADVANCED_FACE ( 'NONE', ( #40611 ), #104531, .F. ) ;
#71515=CARTESIAN_POINT ( 'NONE',  ( -2.715357302349999724, 1447.820972450259887, 154.4673902286979796 ) ) ;
#71516=CARTESIAN_POINT ( 'NONE',  ( -18.35233659730000255, 1424.971321547430080, 225.5691796496979862 ) ) ;
#71517=CARTESIAN_POINT ( 'NONE',  ( -15.06148604940000091, 1435.839581580419917, 149.4729251189979777 ) ) ;
#71518=CARTESIAN_POINT ( 'NONE',  ( -0.5845692370331438958, 1467.807727929299972, 230.0158462584300025 ) ) ;
#71519=CARTESIAN_POINT ( 'NONE',  ( 16.32486700269999957, 1418.999550187130126, 191.2653796169979898 ) ) ;
#71520=CARTESIAN_POINT ( 'NONE',  ( 0.1697262053381299873, 1408.918987357010110, 231.7543611685260032 ) ) ;
#71521=CARTESIAN_POINT ( 'NONE',  ( -18.44100721514212537, 1436.486662365291750, 212.9983258236653683 ) ) ;
#71524=CARTESIAN_POINT ( 'NONE',  ( -0.2626388803150430107, 1424.255108698730055, 227.7923674800080107 ) ) ;
#71527=FACE_OUTER_BOUND ( 'NONE', #42424, .T. ) ;
#71530=CARTESIAN_POINT ( 'NONE',  ( -18.58455358810000035, 1509.562047299329834, 231.7122880195979917 ) ) ;
#71531=CARTESIAN_POINT ( 'NONE',  ( 11.60004869885203682, 1426.786827912535728, 134.3786173235958472 ) ) ;
#71532=CARTESIAN_POINT ( 'NONE',  ( 19.68294476550000027, 1431.113060387329824, 210.0974834526720088 ) ) ;
#71535=CARTESIAN_POINT ( 'NONE',  ( -14.24649929728060016, 1509.423840198609923, 183.1703963639310189 ) ) ;
#71545=ADVANCED_FACE ( 'NONE', ( #85352 ), #37507, .T. ) ;
#71546=CARTESIAN_POINT ( 'NONE',  ( 19.93293359290609956, 1508.855319075360057, 229.5871707258750121 ) ) ;
#71548=VERTEX_POINT ( 'NONE', #27131 ) ;
#71549=CARTESIAN_POINT ( 'NONE',  ( 16.63478241967279914, 1414.913060387399810, 210.4991047624779981 ) ) ;
#71550=CARTESIAN_POINT ( 'NONE',  ( 13.45333203899999930, 1508.683642288930059, 233.3158433383979968 ) ) ;
#71551=CARTESIAN_POINT ( 'NONE',  ( 12.60661500655967693, 1442.786586627101997, 169.4683401008484509 ) ) ;
#71552=CARTESIAN_POINT ( 'NONE',  ( 41.21166932550332973, 1434.842932742385074, 269.6325636146803504 ) ) ;
#71553=CARTESIAN_POINT ( 'NONE',  ( -27.70845756829999829, 1450.383242533360090, 238.1060645626980090 ) ) ;
#71555=CARTESIAN_POINT ( 'NONE',  ( -20.51560685680000162, 1505.131281290129891, 190.1532519183979844 ) ) ;
#71556=CARTESIAN_POINT ( 'NONE',  ( -11.91229251400000066, 1433.393972783660047, 150.1287693233979894 ) ) ;
#71557=ADVANCED_FACE ( 'NONE', ( #18155 ), #45584, .F. ) ;
#71558=CARTESIAN_POINT ( 'NONE',  ( 26.64289581539999929, 1508.595173681330152, 204.0920109017480115 ) ) ;
#71559=CARTESIAN_POINT ( 'NONE',  ( -19.06270802089999705, 1485.830083011429906, 189.5716758561979987 ) ) ;
#71561=CARTESIAN_POINT ( 'NONE',  ( 5.174241722320000569, 1423.109489784829975, 185.3707530537979835 ) ) ;
#71562=CARTESIAN_POINT ( 'NONE',  ( -24.39066168639999788, 1440.643119315069953, 211.3250814536579867 ) ) ;
#71563=CARTESIAN_POINT ( 'NONE',  ( 6.017144064880000087, 1442.258634807139970, 154.7968030183980090 ) ) ;
#71564=DIRECTION ( 'NONE',  ( -1.985713488479999930E-13, 1.181721098350000151E-14, 1.000000000000000000 ) ) ;
#71566=CARTESIAN_POINT ( 'NONE',  ( 0.02089856015480650100, 1507.111761549349922, 237.3522809668369860 ) ) ;
#71567=CARTESIAN_POINT ( 'NONE',  ( 2.149988386126029882E-09, 1405.989059316979819, 266.9611530767110139 ) ) ;
#71568=ORIENTED_EDGE ( 'NONE', *, *, #98951, .T. ) ;
#71572=CARTESIAN_POINT ( 'NONE',  ( -10.49063443250000027, 1470.661302036229699, 269.6264949689979744 ) ) ;
#71574=CARTESIAN_POINT ( 'NONE',  ( 2.331468351709999880E-15, 1435.943783413959864, 155.5249316174979981 ) ) ;
#71575=CARTESIAN_POINT ( 'NONE',  ( -22.79764378385881329, 1411.075395676238713, 211.2310797118794596 ) ) ;
#71579=CARTESIAN_POINT ( 'NONE',  ( -1.202518465757487220, 1484.679450086970292, 182.2456923944191374 ) ) ;
#71581=CARTESIAN_POINT ( 'NONE',  ( -44.28103615880979760, 1432.290645226539709, 266.2283159212610144 ) ) ;
#71583=EDGE_LOOP ( 'NONE', ( #97836, #4532, #45734, #66100, #23931 ) ) ;
#71585=EDGE_LOOP ( 'NONE', ( #26061, #75321, #73777, #81362 ) ) ;
#71589=CARTESIAN_POINT ( 'NONE',  ( -21.33083225349999879, 1509.431387662330053, 190.3642105689980042 ) ) ;
#71597=CARTESIAN_POINT ( 'NONE',  ( 18.53418652026280000, 1507.620785850910124, 188.5293807599879869 ) ) ;
#71600=CARTESIAN_POINT ( 'NONE',  ( -19.44407063118980261, 1410.830196386340049, 270.0540648103669810 ) ) ;
#71602=CARTESIAN_POINT ( 'NONE',  ( 3.561272854136539934, 1416.011968391400160, 231.7883711070729760 ) ) ;
#71607=CARTESIAN_POINT ( 'NONE',  ( 42.75061902808843683, 1452.888007040521416, 269.0553722311352658 ) ) ;
#71609=CARTESIAN_POINT ( 'NONE',  ( 3.625945072265513769, 1424.652023359415125, 184.6562347036613403 ) ) ;
#71610=AXIS2_PLACEMENT_3D ( 'NONE', #61888, #20384, #105520 ) ;
#71612=B_SPLINE_SURFACE_WITH_KNOTS ( 'NONE', 5, 5, ( 
 ( #52594, #86728, #44188, #78330, #110265, #77241, #542, #68304, #24585 ),
 ( #33542, #8348, #43633, #34666, #68852, #102954, #94561, #9468, #77783 ),
 ( #29570, #3305, #36874, #45853, #2206, #81077, #19512, #4393, #79443 ),
 ( #80543, #97868, #104075, #96236, #37985, #69961, #27370, #53717, #78900 ),
 ( #61552, #27929, #53146, #54260, #54797, #72167, #63223, #95685, #87855 ),
 ( #37435, #106285, #2754, #87285, #62675, #18951, #62111, #45304, #21143 ) ),
 .UNSPECIFIED., .F., .F., .F.,
 ( 6, 6 ),
 ( 6, 3, 6 ),
 ( 3.271539800728220371, 6.921095641200810000 ),
 ( -3.659009177935479380E-05, 1.000000000000000000, 2.000000000000000000 ),
 .UNSPECIFIED. ) ;
#71614=CARTESIAN_POINT ( 'NONE',  ( -21.20399697579999909, 1435.766733359059799, 220.8510379581979919 ) ) ;
#71615=CARTESIAN_POINT ( 'NONE',  ( -14.11290024180000025, 1420.166582371130062, 221.9553848337980071 ) ) ;
#71616=CARTESIAN_POINT ( 'NONE',  ( -1.697652520239993246, 1466.995205074520072, 235.3380831672032798 ) ) ;
#71617=CARTESIAN_POINT ( 'NONE',  ( -17.53366249653573306, 1422.926247351624397, 226.4414695557952939 ) ) ;
#71622=EDGE_LOOP ( 'NONE', ( #25607, #108062, #96861, #1706 ) ) ;
#71623=CARTESIAN_POINT ( 'NONE',  ( 10.13233719373625696, 1455.383656796513833, 226.4959039531065059 ) ) ;
#71624=CARTESIAN_POINT ( 'NONE',  ( -27.68254001883949655, 1507.989615300039986, 210.5775529569929745 ) ) ;
#71629=CARTESIAN_POINT ( 'NONE',  ( 19.40037511790000124, 1410.512935499930109, 196.1053253185980054 ) ) ;
#71630=CARTESIAN_POINT ( 'NONE',  ( -2.804857515051331074, 1447.114276553103309, 170.5309535041508298 ) ) ;
#71631=CARTESIAN_POINT ( 'NONE',  ( -24.89775120788979734, 1442.835553621690224, 210.5176540011790109 ) ) ;
#71637=ORIENTED_EDGE ( 'NONE', *, *, #99379, .T. ) ;
#71639=CARTESIAN_POINT ( 'NONE',  ( 43.51386715234850300, 1440.913060384299797, 268.2728856686210293 ) ) ;
#71640=CARTESIAN_POINT ( 'NONE',  ( -3.609207719799999659, 1448.636783799939849, 185.0007839605979996 ) ) ;
#71642=PLANE ( 'NONE',  #51986 ) ;
#71643=CARTESIAN_POINT ( 'NONE',  ( -38.57173337800420398, 1448.259622455230101, 136.4573440376570090 ) ) ;
#71644=FACE_OUTER_BOUND ( 'NONE', #94972, .T. ) ;
#71645=CARTESIAN_POINT ( 'NONE',  ( 2.053820611095168669, 1417.320383901196010, 233.1665847537391301 ) ) ;
#71647=CARTESIAN_POINT ( 'NONE',  ( -2.387209960284789823, 1464.875116557210049, 184.0699123369479935 ) ) ;
#71648=CARTESIAN_POINT ( 'NONE',  ( 10.99133036650000150, 1433.251705345969867, 151.7641221038979893 ) ) ;
#71650=B_SPLINE_SURFACE_WITH_KNOTS ( 'NONE', 4, 5, ( 
 ( #61969, #946, #44038, #68160, #53002, #78176, #17128, #95534, #96083, #35071, #69815, #42935, #103359, #102267, #26661, #18807, #42367, #59739, #68699, #94986, #51318 ),
 ( #25547, #103932, #8752, #27231, #87135, #10425, #34520, #60862, #102804, #51890, #26099, #18254, #60289, #94408, #50774, #86026, #61411, #77634, #52450, #78739, #2054 ),
 ( #70370, #76522, #84908, #110672, #4243, #105046, #97185, #64723, #12078, #45159, #36735, #89886, #63086, #2610, #19358, #4774, #30532, #29974, #88247, #81470, #106145 ),
 ( #53559, #3713, #12637, #11540, #80399, #70930, #37843, #98284, #107240, #96650, #38377, #72553, #55771, #55212, #89341, #87705, #63623, #71486, #19918, #73101, #97739 ),
 ( #79299, #28891, #28335, #64166, #38920, #3163, #54119, #62527, #29424, #21561, #72030, #10985, #106683, #13156, #105607, #45715, #21010, #79852, #37295, #20459, #46814 ) ),
 .UNSPECIFIED., .F., .F., .F.,
 ( 5, 5 ),
 ( 6, 3, 3, 3, 3, 3, 6 ),
 ( 1.603979892999999990, 11.76009528039999985 ),
 ( 27.96617286999999763, 34.32222934679999327, 36.67765262920000424, 37.85536427039999552, 39.03307591160000101, 39.85568086760000028, 40.67828582359999956 ),
 .UNSPECIFIED. ) ;
#71652=CARTESIAN_POINT ( 'NONE',  ( -25.03616385470000338, 1508.005457897430006, 220.0251884486980032 ) ) ;
#71656=CARTESIAN_POINT ( 'NONE',  ( 22.90620825975110009, 1507.562497965009925, 210.1669428755749891 ) ) ;
#71659=CARTESIAN_POINT ( 'NONE',  ( -19.37630605257373873, 1485.608798315509375, 189.8785843432788738 ) ) ;
#71661=CARTESIAN_POINT ( 'NONE',  ( 0.5697989934050000649, 1450.893162568020216, 198.0847581318980133 ) ) ;
#71664=DIRECTION ( 'NONE',  ( 0.3527344445857066857, -0.9357193065623196082, -0.002791223628648406563 ) ) ;
#71666=( BOUNDED_CURVE ( )  B_SPLINE_CURVE ( 3, ( #28600, #60577, #17971, #3423 ),
 .UNSPECIFIED., .F., .F. ) 
 B_SPLINE_CURVE_WITH_KNOTS ( ( 4, 4 ),
 ( 0.8955272655465470466, 1.005666413988429930 ),
 .UNSPECIFIED. ) 
 CURVE ( )  GEOMETRIC_REPRESENTATION_ITEM ( )  RATIONAL_B_SPLINE_CURVE ( ( 1.000000000000000000, 0.9989893694451776884, 0.9989893694451776884, 1.000000000000000000 ) ) 
 REPRESENTATION_ITEM ( '' )  );
#71667=DIRECTION ( 'NONE',  ( 0.000000000000000000, 1.000000000000000000, 0.000000000000000000 ) ) ;
#71668=CARTESIAN_POINT ( 'NONE',  ( 2.499944111023190363, 1419.634096732200078, 130.9499281974879921 ) ) ;
#71670=CARTESIAN_POINT ( 'NONE',  ( 1.649680371479999907, 1465.639337990229933, 235.0739432404980107 ) ) ;
#71673=CARTESIAN_POINT ( 'NONE',  ( -1.192591789150000192, 1451.233485826829792, 183.2247612650980102 ) ) ;
#71675=ADVANCED_FACE ( 'NONE', ( #49518 ), #110508, .F. ) ;
#71676=CARTESIAN_POINT ( 'NONE',  ( -5.519891203089999365, 1440.499824919269940, 154.7645185998979969 ) ) ;
#71684=B_SPLINE_CURVE_WITH_KNOTS ( 'NONE', 3,
 ( #3223, #29483, #88304, #3772, #70988, #64222, #46872, #97243, #81000, #20518, #54725, #53625, #46329 ),
 .UNSPECIFIED., .F., .F.,
 ( 4, 3, 3, 3, 4 ),
 ( -167.7240082859999859, -142.7479071452019923, -102.0777101884260105, -65.48876935620850759, -30.58270280209998759 ),
 .UNSPECIFIED. ) ;
#71685=CARTESIAN_POINT ( 'NONE',  ( 22.70290200285219484, 1409.705865383426271, 208.6626894467611919 ) ) ;
#71689=CARTESIAN_POINT ( 'NONE',  ( 14.24591603755999891, 1409.410538736599847, 213.5977365385609801 ) ) ;
#71692=CARTESIAN_POINT ( 'NONE',  ( -19.35957638029999828, 1470.693184109529966, 190.9127711249979882 ) ) ;
#71696=ORIENTED_EDGE ( 'NONE', *, *, #95396, .T. ) ;
#71697=ORIENTED_EDGE ( 'NONE', *, *, #102915, .F. ) ;
#71698=CARTESIAN_POINT ( 'NONE',  ( -11.44693299037050060, 1415.124054205840139, 195.4737557617620212 ) ) ;
#71699=DIRECTION ( 'NONE',  ( 1.000000000000000000, 0.000000000000000000, 0.000000000000000000 ) ) ;
#71702=CARTESIAN_POINT ( 'NONE',  ( 29.83339565102073720, 1462.371191219802768, 269.4690383729464429 ) ) ;
#71704=CARTESIAN_POINT ( 'NONE',  ( 3.586107180329999977, 1396.221082240130045, 220.6064224583979865 ) ) ;
#71706=CARTESIAN_POINT ( 'NONE',  ( -0.8850937001509999735, 1467.455705555530130, 182.7531797504979920 ) ) ;
#71710=CARTESIAN_POINT ( 'NONE',  ( -13.04373921950000081, 1435.024846296409805, 150.0238230700980182 ) ) ;
#71712=CARTESIAN_POINT ( 'NONE',  ( 0.7130140550910000208, 1416.844618635429924, 190.3244981512979734 ) ) ;
#71714=CARTESIAN_POINT ( 'NONE',  ( 4.500000000000000000, 1448.210448412289907, 182.3842140122979743 ) ) ;
#71718=CARTESIAN_POINT ( 'NONE',  ( -26.28495520110000072, 1469.245429239829946, 207.2831767420279903 ) ) ;
#71719=CARTESIAN_POINT ( 'NONE',  ( -10.92148113222090089, 1426.083150769400163, 93.54269902050201324 ) ) ;
#71720=CARTESIAN_POINT ( 'NONE',  ( -0.5987183604784179769, 1507.212886163649955, 231.7504617458309895 ) ) ;
#71721=EDGE_CURVE ( 'NONE', #98568, #28929, #10783, .T. ) ;
#71722=CARTESIAN_POINT ( 'NONE',  ( 1.669890710131026967, 1508.956865050931128, 179.7751757192045261 ) ) ;
#71723=CARTESIAN_POINT ( 'NONE',  ( -10.53938673480000077, 1414.594228658529801, 248.5638781430979805 ) ) ;
#71724=CARTESIAN_POINT ( 'NONE',  ( 20.51326474582850068, 1509.672687637749959, 230.6559570000279962 ) ) ;
#71726=DIRECTION ( 'NONE',  ( 0.5674277338727796716, 0.8234232003241116482, 0.000000000000000000 ) ) ;
#71727=ORIENTED_EDGE ( 'NONE', *, *, #85099, .T. ) ;
#71728=CARTESIAN_POINT ( 'NONE',  ( 3.920879176457659820, 1439.701872010520219, 184.6839060028229937 ) ) ;
#71730=CARTESIAN_POINT ( 'NONE',  ( 11.57433915100000021, 1509.317245216830088, 236.3676525501980166 ) ) ;
#71735=VERTEX_POINT ( 'NONE', #92591 ) ;
#71736=FACE_OUTER_BOUND ( 'NONE', #86950, .T. ) ;
#71739=CARTESIAN_POINT ( 'NONE',  ( -11.86678758501360065, 1432.386623006779928, 149.9823363065619901 ) ) ;
#71740=CARTESIAN_POINT ( 'NONE',  ( -1.436137458879999995, 1489.063931860629964, 236.3499381435979956 ) ) ;
#71743=CARTESIAN_POINT ( 'NONE',  ( 10.81506866279999990, 1424.921186100929845, 144.1620444789979842 ) ) ;
#71744=CARTESIAN_POINT ( 'NONE',  ( -12.03795434196880088, 1414.913057855109855, 220.4160453579169996 ) ) ;
#71745=CARTESIAN_POINT ( 'NONE',  ( 14.78974000539999878, 1496.665265930929991, 226.0583177165980260 ) ) ;
#71749=CARTESIAN_POINT ( 'NONE',  ( 11.86398041411250048, 1432.187849662659801, 149.9803448969269937 ) ) ;
#71752=EDGE_LOOP ( 'NONE', ( #80476, #9838, #60407 ) ) ;
#71754=FACE_OUTER_BOUND ( 'NONE', #25097, .T. ) ;
#71759=CARTESIAN_POINT ( 'NONE',  ( 0.4843704149012760252, 1408.561147827879950, 270.4290818619680294 ) ) ;
#71762=CARTESIAN_POINT ( 'NONE',  ( -20.71991831406684170, 1509.684987494643565, 230.4894327893642867 ) ) ;
#71764=CARTESIAN_POINT ( 'NONE',  ( 14.20204630610000152, 1416.837080254230159, 196.5054416555979913 ) ) ;
#71767=CARTESIAN_POINT ( 'NONE',  ( 17.96527429238589946, 1422.523928809379868, 225.1465795047810161 ) ) ;
#71770=CARTESIAN_POINT ( 'NONE',  ( 16.86383896219999912, 1416.370072266829993, 262.6648722463980334 ) ) ;
#71775=DIRECTION ( 'NONE',  ( 0.3971731930706579039, 0.04395516701092885142, 0.9166904592058866541 ) ) ;
#71785=CARTESIAN_POINT ( 'NONE',  ( 19.19360523492100157, 1509.583315851710040, 231.6001312093189881 ) ) ;
#71787=CARTESIAN_POINT ( 'NONE',  ( -15.28420222199999934, 1497.713060387329961, 224.4060481839979957 ) ) ;
#71788=CARTESIAN_POINT ( 'NONE',  ( 4.426925289939999786, 1417.415159599829849, 231.7246244170979992 ) ) ;
#71790=CARTESIAN_POINT ( 'NONE',  ( 1.356522472024429993, 1410.335674015750101, 232.6399073486850000 ) ) ;
#71792=CARTESIAN_POINT ( 'NONE',  ( 45.06536953950000424, 1434.999718682669936, 268.9906915396979912 ) ) ;
#71793=CARTESIAN_POINT ( 'NONE',  ( -18.33065379749999835, 1410.049607812529985, 223.7945510231980109 ) ) ;
#71794=CARTESIAN_POINT ( 'NONE',  ( 17.98866383510000233, 1435.941952030790162, 147.2730939229980152 ) ) ;
#71796=CARTESIAN_POINT ( 'NONE',  ( 21.20954604569999802, 1488.584398273929992, 192.3846377322979890 ) ) ;
#71797=CARTESIAN_POINT ( 'NONE',  ( 22.72408229139999847, 1432.100443994239868, 218.1715127473280234 ) ) ;
#71799=CARTESIAN_POINT ( 'NONE',  ( -0.7749238296759999312, 1475.832189872029858, 266.9609160975979876 ) ) ;
#71801=CARTESIAN_POINT ( 'NONE',  ( -36.93911259867740426, 1436.285475061979923, 135.0345442704649770 ) ) ;
#71802=CARTESIAN_POINT ( 'NONE',  ( 0.2072761112290929797, 1458.881660194060260, 183.0010636273980253 ) ) ;
#71803=CARTESIAN_POINT ( 'NONE',  ( -12.34781077223220080, 1407.409374063429823, 203.9011771819639876 ) ) ;
#71804=CARTESIAN_POINT ( 'NONE',  ( 0.2417153426969999852, 1418.558758520830224, 184.6769579382979884 ) ) ;
#71805=CARTESIAN_POINT ( 'NONE',  ( -12.45591551270000075, 1442.246608597349905, 187.4685661162980068 ) ) ;
#71807=CARTESIAN_POINT ( 'NONE',  ( 13.50147622419999927, 1434.968985796360130, 146.7592199324979845 ) ) ;
#71808=FACE_OUTER_BOUND ( 'NONE', #22821, .T. ) ;
#71809=CARTESIAN_POINT ( 'NONE',  ( -1.018585033021226938, 1419.107236328670524, 184.9305476069722545 ) ) ;
#71812=CARTESIAN_POINT ( 'NONE',  ( -5.146882827519980275, 1409.092793496169861, 223.1895541711200224 ) ) ;
#71813=CARTESIAN_POINT ( 'NONE',  ( -17.22592475670000312, 1443.913060387330006, 162.9227486557980171 ) ) ;
#71816=CARTESIAN_POINT ( 'NONE',  ( -44.93232737969999135, 1451.209032879530014, 267.0122724004980341 ) ) ;
#71818=CARTESIAN_POINT ( 'NONE',  ( -19.82130876261663133, 1501.765438912635773, 189.1477900679612958 ) ) ;
#71819=CARTESIAN_POINT ( 'NONE',  ( -26.93111412509999880, 1509.630721880230112, 216.4445429101480158 ) ) ;
#71823=CARTESIAN_POINT ( 'NONE',  ( 17.33325820480230206, 1423.906894160079901, 228.7549733049369820 ) ) ;
#71824=CARTESIAN_POINT ( 'NONE',  ( 21.92402930929999982, 1509.678664361430037, 227.7489718475979998 ) ) ;
#71825=CARTESIAN_POINT ( 'NONE',  ( 15.72497962809999983, 1506.810797447130199, 224.5140330397979938 ) ) ;
#71829=ORIENTED_EDGE ( 'NONE', *, *, #4980, .T. ) ;
#71833=CARTESIAN_POINT ( 'NONE',  ( 25.70439233229999942, 1469.175250655529908, 207.3826630381880136 ) ) ;
#71834=CARTESIAN_POINT ( 'NONE',  ( -12.45642902069999991, 1416.822690122629865, 194.7673859876979918 ) ) ;
#71836=EDGE_CURVE ( 'NONE', #107891, #15749, #34899, .T. ) ;
#71837=CARTESIAN_POINT ( 'NONE',  ( 23.99977061020000235, 1410.673205389529812, 209.9141634752309926 ) ) ;
#71841=CARTESIAN_POINT ( 'NONE',  ( -10.97596787830000054, 1432.730999280179958, 151.7698537100980047 ) ) ;
#71842=CARTESIAN_POINT ( 'NONE',  ( -11.61990403848027675, 1426.774261403575565, 135.7993244020507575 ) ) ;
#71843=CARTESIAN_POINT ( 'NONE',  ( 0.3042685152679999727, 1411.657205677930051, 233.3132544252979983 ) ) ;
#71847=FACE_OUTER_BOUND ( 'NONE', #78450, .T. ) ;
#71848=CARTESIAN_POINT ( 'NONE',  ( -0.8190364809989280070, 1418.969067203539907, 184.8287228181580133 ) ) ;
#71851=CARTESIAN_POINT ( 'NONE',  ( 13.40431027868319980, 1508.087536715469696, 233.1606899894430001 ) ) ;
#71852=CARTESIAN_POINT ( 'NONE',  ( -18.39201604218439812, 1486.027299296950105, 188.9270178829710005 ) ) ;
#71858=CARTESIAN_POINT ( 'NONE',  ( 28.60142811679999753, 1509.872226484729936, 213.7037800932280049 ) ) ;
#71862=CARTESIAN_POINT ( 'NONE',  ( -1.077847364669999991E-15, 1428.043997280830126, 101.8807690336980016 ) ) ;
#71863=CARTESIAN_POINT ( 'NONE',  ( 1.129089833999999959, 1507.125633147629969, 181.0548235415979832 ) ) ;
#71866=CARTESIAN_POINT ( 'NONE',  ( -24.24285629885429927, 1452.061333677959965, 136.5609822530450117 ) ) ;
#71868=CARTESIAN_POINT ( 'NONE',  ( 4.247845347069999278, 1409.061398416330121, 230.4234178570980021 ) ) ;
#71872=CARTESIAN_POINT ( 'NONE',  ( 41.49772933728709745, 1445.334750750500007, 134.0999999984909721 ) ) ;
#71875=CARTESIAN_POINT ( 'NONE',  ( 14.59287365574109963, 1436.244834338669989, 149.8708846901989773 ) ) ;
#71878=EDGE_LOOP ( 'NONE', ( #99186, #9990, #49068, #65931, #56085 ) ) ;
#71881=DIRECTION ( 'NONE',  ( 1.000000000000000000, 0.000000000000000000, 0.000000000000000000 ) ) ;
#71882=CARTESIAN_POINT ( 'NONE',  ( 8.737474774033083591, 1451.364372104259473, 152.7144497316307650 ) ) ;
#71889=CARTESIAN_POINT ( 'NONE',  ( 5.808539518960000869, 1415.087797054229895, 192.8637157185980016 ) ) ;
#71890=B_SPLINE_CURVE_WITH_KNOTS ( 'NONE', 3,
 ( #14886, #49077, #47418, #91609, #31145, #13777, #81540, #6501, #99999, #40655, #73166, #107310, #74826 ),
 .UNSPECIFIED., .F., .F.,
 ( 4, 3, 3, 3, 4 ),
 ( -167.9629942519999872, -131.9082348649870085, -95.51900912811341016, -62.09002792079060384, -30.61745639480000136 ),
 .UNSPECIFIED. ) ;
#71893=CARTESIAN_POINT ( 'NONE',  ( 31.96508519263229786, 1440.913060387330006, 255.8875838973339683 ) ) ;
#71897=CARTESIAN_POINT ( 'NONE',  ( -14.54947616759999995, 1409.923023063329993, 190.7312617873979832 ) ) ;
#71901=CARTESIAN_POINT ( 'NONE',  ( 22.04426538949190117, 1410.014371781770024, 206.2776455835269758 ) ) ;
#71903=CARTESIAN_POINT ( 'NONE',  ( -12.10808283629549820, 1433.926313951669499, 147.5251541910231765 ) ) ;
#71904=CARTESIAN_POINT ( 'NONE',  ( -12.91306329870000091, 1434.774359993769849, 148.5639779176980255 ) ) ;
#71906=CARTESIAN_POINT ( 'NONE',  ( 7.696916953700000619, 1464.574746897430032, 233.3918279888980010 ) ) ;
#71911=CARTESIAN_POINT ( 'NONE',  ( 16.67654997235155534, 1449.441375609227862, 219.1029392211832771 ) ) ;
#71917=ORIENTED_EDGE ( 'NONE', *, *, #93872, .T. ) ;
#71919=CARTESIAN_POINT ( 'NONE',  ( 22.59987829099999956, 1454.496478413630030, 232.0087828362979963 ) ) ;
#71921=FACE_OUTER_BOUND ( 'NONE', #7267, .T. ) ;
#71923=EDGE_CURVE ( 'NONE', #52837, #73912, #39056, .T. ) ;
#71924=CARTESIAN_POINT ( 'NONE',  ( 2.193589587269999974, 1410.361569429029942, 231.8614317343979963 ) ) ;
#71926=AXIS2_PLACEMENT_3D ( 'NONE', #45521, #37639, #104846 ) ;
#71927=CARTESIAN_POINT ( 'NONE',  ( -19.29250527829999839, 1444.805202439009918, 225.3992152728980329 ) ) ;
#71928=CARTESIAN_POINT ( 'NONE',  ( 5.382707040917719787, 1431.444277130069850, 154.5902336194710074 ) ) ;
#71929=CARTESIAN_POINT ( 'NONE',  ( -0.2308247287459999908, 1470.816572150329876, 188.6928027695979893 ) ) ;
#71933=CARTESIAN_POINT ( 'NONE',  ( 1.777755710779999943, 1405.800407096930030, 268.4824710471980325 ) ) ;
#71935=CARTESIAN_POINT ( 'NONE',  ( 39.04070846521679528, 1456.280716702200152, 270.3387515494820263 ) ) ;
#71936=CARTESIAN_POINT ( 'NONE',  ( -0.0002122017571388959824, 1432.353341358199941, 123.3907408769529894 ) ) ;
#71937=CARTESIAN_POINT ( 'NONE',  ( 11.60004869883886869, 1424.049974457302142, 137.1751211143046874 ) ) ;
#71939=CARTESIAN_POINT ( 'NONE',  ( 12.53380745427929988, 1442.773887455719887, 186.4115735415020083 ) ) ;
#71940=CARTESIAN_POINT ( 'NONE',  ( 14.39948538648319776, 1509.538292521139510, 235.4401890623756799 ) ) ;
#71942=CARTESIAN_POINT ( 'NONE',  ( 17.38482601099109814, 1410.884446382940041, 192.4603632472940262 ) ) ;
#71945=CARTESIAN_POINT ( 'NONE',  ( 6.439293542829999756E-15, 1420.418457356630142, 243.9198229339980060 ) ) ;
#71947=CARTESIAN_POINT ( 'NONE',  ( -0.3397164161819999917, 1476.075833985229792, 267.5371225513979994 ) ) ;
#71949=CARTESIAN_POINT ( 'NONE',  ( -29.12559713569999786, 1509.873774314229877, 210.4730869765679984 ) ) ;
#71950=CARTESIAN_POINT ( 'NONE',  ( -3.854452527945675389, 1448.295591906145319, 185.0328819066131700 ) ) ;
#71952=CIRCLE ( 'NONE', #75522, 28.41070217520000440 ) ;
#71955=CARTESIAN_POINT ( 'NONE',  ( 26.80802651847389839, 1435.516884147950122, 135.8294075311020208 ) ) ;
#71956=CARTESIAN_POINT ( 'NONE',  ( -2.313829914396530185, 1395.993861108439887, 219.8905569203290042 ) ) ;
#71957=CARTESIAN_POINT ( 'NONE',  ( -14.75316392789999931, 1422.315547878330108, 228.7562151032980182 ) ) ;
#71961=CARTESIAN_POINT ( 'NONE',  ( -13.90496247579444322, 1414.913060387329779, 200.7481815758607411 ) ) ;
#71962=CARTESIAN_POINT ( 'NONE',  ( 1.943617413929999982, 1409.147975478429998, 231.3620511928980079 ) ) ;
#71963=CARTESIAN_POINT ( 'NONE',  ( -11.86590139589999815, 1432.348266868109931, 151.0567667964980103 ) ) ;
#71964=CARTESIAN_POINT ( 'NONE',  ( 11.62168133680000004, 1426.773520508030060, 135.9278380674980156 ) ) ;
#71967=CARTESIAN_POINT ( 'NONE',  ( 4.210524679639359391, 1424.023046679440085, 184.1832055361919913 ) ) ;
#71971=CARTESIAN_POINT ( 'NONE',  ( 1.585275487589999921, 1508.725511249229839, 180.2575163522980120 ) ) ;
#71972=CARTESIAN_POINT ( 'NONE',  ( 7.105427357599999217E-15, 1423.509254465030153, 167.6739826277979830 ) ) ;
#71977=ORIENTED_EDGE ( 'NONE', *, *, #30273, .T. ) ;
#71978=CARTESIAN_POINT ( 'NONE',  ( -10.57949873459999779, 1396.282504623229897, 204.0310317109180005 ) ) ;
#71979=CARTESIAN_POINT ( 'NONE',  ( -11.49359948000000031, 1409.314425725430056, 190.5616205332979973 ) ) ;
#71980=CARTESIAN_POINT ( 'NONE',  ( 8.099819236969999281, 1497.713060387329961, 229.6744222972979799 ) ) ;
#71986=CARTESIAN_POINT ( 'NONE',  ( -41.48253158878969771, 1444.135608968060069, 136.5500586159059822 ) ) ;
#71987=CARTESIAN_POINT ( 'NONE',  ( 37.28638872520870251, 1436.958943370610086, 136.2769035375250155 ) ) ;
#71989=CARTESIAN_POINT ( 'NONE',  ( 33.92729347383400551, 1436.577116162089851, 136.5096455005439964 ) ) ;
#71990=CARTESIAN_POINT ( 'NONE',  ( -3.772679660826560255, 1406.882484426249903, 269.6459227122439870 ) ) ;
#71991=FACE_OUTER_BOUND ( 'NONE', #36459, .T. ) ;
#71993=CARTESIAN_POINT ( 'NONE',  ( 4.087259578919999470, 1424.194160912629968, 184.7150810775980005 ) ) ;
#71994=ORIENTED_EDGE ( 'NONE', *, *, #47610, .F. ) ;
#71996=ADVANCED_FACE ( 'NONE', ( #26491 ), #60730, .F. ) ;
#72002=ORIENTED_EDGE ( 'NONE', *, *, #19527, .F. ) ;
#72003=CARTESIAN_POINT ( 'NONE',  ( -5.985688616083930214, 1509.236238061519771, 179.5306295814190207 ) ) ;
#72005=( BOUNDED_CURVE ( )  B_SPLINE_CURVE ( 3, ( #8241, #59783, #85496, #8795 ),
 .UNSPECIFIED., .F., .F. ) 
 B_SPLINE_CURVE_WITH_KNOTS ( ( 4, 4 ),
 ( 4.621677078022849550, 4.871924224616510202 ),
 .UNSPECIFIED. ) 
 CURVE ( )  GEOMETRIC_REPRESENTATION_ITEM ( )  RATIONAL_B_SPLINE_CURVE ( ( 1.000000000000000000, 0.9947881687906164894, 0.9947881687906164894, 1.000000000000000000 ) ) 
 REPRESENTATION_ITEM ( '' )  );
#72006=CARTESIAN_POINT ( 'NONE',  ( 5.332222640600000396, 1416.518532928330160, 226.4836215587980064 ) ) ;
#72010=CARTESIAN_POINT ( 'NONE',  ( -3.672183373650000249, 1409.545492258829881, 232.1063284713980011 ) ) ;
#72011=CARTESIAN_POINT ( 'NONE',  ( 13.51610093809999924, 1443.913060387330006, 169.3501091259980171 ) ) ;
#72012=EDGE_LOOP ( 'NONE', ( #28350, #75101, #61593, #42299 ) ) ;
#72018=CARTESIAN_POINT ( 'NONE',  ( 40.92984665081159790, 1427.618493474619981, 270.2459107829799905 ) ) ;
#72022=CARTESIAN_POINT ( 'NONE',  ( 23.67748127589999996, 1410.709634711930221, 207.9970578281480016 ) ) ;
#72023=CARTESIAN_POINT ( 'NONE',  ( 0.01564820846407900465, 1507.754288909950901, 237.4874347475621619 ) ) ;
#72029=CARTESIAN_POINT ( 'NONE',  ( 4.291363136070279083, 1421.924736920739861, 184.1044750076529795 ) ) ;
#72030=CARTESIAN_POINT ( 'NONE',  ( -3.615035349779999851, 1420.447245347430226, 232.7901725780979802 ) ) ;
#72036=CARTESIAN_POINT ( 'NONE',  ( -21.87101081987050222, 1509.710974767680000, 229.2198085769670115 ) ) ;
#72038=CARTESIAN_POINT ( 'NONE',  ( 0.2565248355029999816, 1409.415731479529995, 232.9897570089979979 ) ) ;
#72039=CARTESIAN_POINT ( 'NONE',  ( 0.07335717183216540482, 1420.449307609759899, 182.6843235195379975 ) ) ;
#72040=EDGE_CURVE ( 'NONE', #105370, #10196, #73801, .T. ) ;
#72043=CARTESIAN_POINT ( 'NONE',  ( 19.26470018019999841, 1508.010672954829943, 188.6340786004979861 ) ) ;
#72049=CARTESIAN_POINT ( 'NONE',  ( -0.1702787592430000108, 1497.005873238030063, 230.8763743371980013 ) ) ;
#72055=CARTESIAN_POINT ( 'NONE',  ( -26.38747615144840353, 1508.287016310790023, 201.5298666568500039 ) ) ;
#72056=CARTESIAN_POINT ( 'NONE',  ( 4.401092417150000102, 1420.174153566729956, 185.7217845719979721 ) ) ;
#72057=CARTESIAN_POINT ( 'NONE',  ( -13.80537871780000003, 1434.979603129589805, 148.5370412790979913 ) ) ;
#72059=CARTESIAN_POINT ( 'NONE',  ( 18.11157302770000044, 1509.545530454130130, 186.5307135953979980 ) ) ;
#72060=CARTESIAN_POINT ( 'NONE',  ( 1.270728227940000066, 1414.996442546130083, 191.7853923321980005 ) ) ;
#72061=CARTESIAN_POINT ( 'NONE',  ( 28.25086641300000068, 1508.135711190629991, 209.3856964555159834 ) ) ;
#72064=ORIENTED_EDGE ( 'NONE', *, *, #3058, .F. ) ;
#72067=CARTESIAN_POINT ( 'NONE',  ( -45.09884245687089788, 1435.519538208483709, 268.9899558901107071 ) ) ;
#72069=CARTESIAN_POINT ( 'NONE',  ( -23.93221639060000072, 1436.995215223070090, 212.4007312564980055 ) ) ;
#72072=CARTESIAN_POINT ( 'NONE',  ( 12.63891593913163014, 1435.851297268093504, 150.8990495699463565 ) ) ;
#72073=CARTESIAN_POINT ( 'NONE',  ( -17.10420012025889847, 1414.913526845469960, 207.6224735737659728 ) ) ;
#72075=ADVANCED_FACE ( 'NONE', ( #66196 ), #100844, .F. ) ;
#72082=ORIENTED_EDGE ( 'NONE', *, *, #93906, .F. ) ;
#72086=ORIENTED_EDGE ( 'NONE', *, *, #52584, .T. ) ;
#72087=CARTESIAN_POINT ( 'NONE',  ( 17.15013451049770055, 1414.913057819779851, 210.5788933209909715 ) ) ;
#72089=CARTESIAN_POINT ( 'NONE',  ( 13.42574451573709915, 1443.464390912571616, 169.3656144573682241 ) ) ;
#72090=CARTESIAN_POINT ( 'NONE',  ( 40.69310009642936166, 1433.220003743809912, 269.6228712187607357 ) ) ;
#72091=CARTESIAN_POINT ( 'NONE',  ( -29.87496815560000130, 1440.913060384770006, 238.0574314952980046 ) ) ;
#72092=CARTESIAN_POINT ( 'NONE',  ( -19.59580092090000036, 1494.488138752529949, 189.3579594609980177 ) ) ;
#72093=CARTESIAN_POINT ( 'NONE',  ( -11.81944340819999972, 1433.674010844490113, 150.7526810563979893 ) ) ;
#72095=CARTESIAN_POINT ( 'NONE',  ( -19.82947209420000334, 1486.245552723730043, 190.1506153878980001 ) ) ;
#72097=CARTESIAN_POINT ( 'NONE',  ( 6.328983188139999605, 1409.301000327829797, 187.4842807998980163 ) ) ;
#72098=CARTESIAN_POINT ( 'NONE',  ( 5.461421721539999830, 1423.173959525930059, 185.7905159978980123 ) ) ;
#72099=CARTESIAN_POINT ( 'NONE',  ( -24.49316664000000188, 1440.648604759869841, 210.9862992980479817 ) ) ;
#72100=CARTESIAN_POINT ( 'NONE',  ( 7.036086740800000072, 1439.758761535590111, 154.1890769228979821 ) ) ;
#72104=CARTESIAN_POINT ( 'NONE',  ( 2.485998036212079895E-11, 1411.655689664790089, 254.4737176916400188 ) ) ;
#72107=CARTESIAN_POINT ( 'NONE',  ( -11.85761565696060060, 1431.744374585950027, 149.9502556072889945 ) ) ;
#72108=EDGE_CURVE ( 'NONE', #28853, #24977, #88464, .T. ) ;
#72110=CARTESIAN_POINT ( 'NONE',  ( -25.30728195769999900, 1466.918094299930090, 270.3546022141979961 ) ) ;
#72111=CARTESIAN_POINT ( 'NONE',  ( 37.65047687761219919, 1442.773887286080026, 137.1096749932030150 ) ) ;
#72113=CARTESIAN_POINT ( 'NONE',  ( -14.94781368989999848, 1495.930802959929906, 224.6074030012979961 ) ) ;
#72114=CARTESIAN_POINT ( 'NONE',  ( 0.3084180738009330014, 1451.032819945409983, 181.9791184512139921 ) ) ;
#72117=CARTESIAN_POINT ( 'NONE',  ( -1.404759085750468373, 1484.431622893082249, 182.4191754957871296 ) ) ;
#72119=CARTESIAN_POINT ( 'NONE',  ( -44.73938210465490073, 1432.137784287730028, 267.0202877731520061 ) ) ;
#72120=ORIENTED_EDGE ( 'NONE', *, *, #11972, .T. ) ;
#72127=CARTESIAN_POINT ( 'NONE',  ( 16.89684008137831484, 1409.672990159872597, 224.8086551987313726 ) ) ;
#72128=CARTESIAN_POINT ( 'NONE',  ( -15.33845266750000036, 1425.420605040230157, 190.2292057122979827 ) ) ;
#72134=CARTESIAN_POINT ( 'NONE',  ( 0.4649367091635221994, 1508.983694905193943, 238.8636469665097763 ) ) ;
#72136=CARTESIAN_POINT ( 'NONE',  ( -13.38634297238620086, 1410.004322308419887, 270.4097950069890430 ) ) ;
#72137=CARTESIAN_POINT ( 'NONE',  ( 4.017110540329999856E-16, 1428.413060387330006, 91.31218443469779800 ) ) ;
#72139=EDGE_CURVE ( 'NONE', #98647, #101745, #24967, .T. ) ;
#72143=CARTESIAN_POINT ( 'NONE',  ( 45.63156121253045683, 1441.449654500054976, 268.9749044632669666 ) ) ;
#72145=CARTESIAN_POINT ( 'NONE',  ( -23.10442739037580040, 1411.095127590459924, 210.9251608898400150 ) ) ;
#72147=CARTESIAN_POINT ( 'NONE',  ( 2.500000195207620290, 1448.894380947069976, 182.3534016008459844 ) ) ;
#72148=CARTESIAN_POINT ( 'NONE',  ( 5.395424494550000283, 1433.568245638130065, 154.6346167951979851 ) ) ;
#72149=CARTESIAN_POINT ( 'NONE',  ( -14.45805363400000054, 1420.164084007830070, 221.6834749228980002 ) ) ;
#72150=CARTESIAN_POINT ( 'NONE',  ( 11.24049419410000006, 1414.988017874730076, 222.4824403021980004 ) ) ;
#72151=EDGE_CURVE ( 'NONE', #35341, #56358, #60520, .T. ) ;
#72154=VERTEX_POINT ( 'NONE', #75551 ) ;
#72155=CARTESIAN_POINT ( 'NONE',  ( -38.81202640297369300, 1436.797832147450208, 135.6928027013960047 ) ) ;
#72156=CARTESIAN_POINT ( 'NONE',  ( -21.11429705600878393, 1454.601516258118863, 222.9879907867546649 ) ) ;
#72160=CARTESIAN_POINT ( 'NONE',  ( 25.41125599211969899, 1450.806039855719973, 137.2920521431910004 ) ) ;
#72163=CARTESIAN_POINT ( 'NONE',  ( 18.81460391099999896, 1409.734757761829997, 196.1127275027980090 ) ) ;
#72164=CARTESIAN_POINT ( 'NONE',  ( 22.92333831959999557, 1411.083494111930122, 207.1379507454479949 ) ) ;
#72165=CARTESIAN_POINT ( 'NONE',  ( -24.89775082669573081, 1442.835544666243777, 210.5176539913697980 ) ) ;
#72167=CARTESIAN_POINT ( 'NONE',  ( 0.5369751114729359731, 1452.020381932720056, 183.1429488159060099 ) ) ;
#72173=B_SPLINE_SURFACE_WITH_KNOTS ( 'NONE', 5, 5, ( 
 ( #40023, #74744, #108333, #65793, #99915, #91535 ),
 ( #14813, #17551, #15898, #33822, #76950, #50640 ),
 ( #69117, #77501, #102124, #42238, #25403, #109992 ),
 ( #102659, #94275, #101559, #801, #51189, #24313 ),
 ( #60154, #85318, #41683, #34386, #76386, #259 ),
 ( #49548, #25959, #92621, #34930, #103218, #59596 ),
 ( #51753, #58495, #101014, #109447, #85889, #67458 ),
 ( #24850, #68560, #7525, #9191, #110535, #43353 ),
 ( #75843, #26526, #68014, #33269, #59053, #16444 ),
 ( #66907, #93174, #60723, #15355, #16989, #83673 ),
 ( #84770, #6970, #8068, #41124, #75304, #93712 ),
 ( #8613, #42790, #32727, #50098, #84225, #80258 ) ),
 .UNSPECIFIED., .F., .F., .F.,
 ( 6, 3, 3, 6 ),
 ( 6, 6 ),
 ( 256.2762652140000341, 274.6371078000000239, 288.1827336739999623, 303.9584180850000052 ),
 ( 0.000000000000000000, 2.000000000000000000 ),
 .UNSPECIFIED. ) ;
#72174=CARTESIAN_POINT ( 'NONE',  ( -0.4918994192140000443, 1474.175172928430129, 270.1377426665980011 ) ) ;
#72176=ADVANCED_FACE ( 'NONE', ( #14505 ), #6111, .T. ) ;
#72178=CARTESIAN_POINT ( 'NONE',  ( -36.68740469744260224, 1449.713037953679986, 136.2729166271199972 ) ) ;
#72179=CARTESIAN_POINT ( 'NONE',  ( 10.93432276284407578, 1424.900206430952039, 138.2785255352749800 ) ) ;
#72180=CARTESIAN_POINT ( 'NONE',  ( 2.151158825738029190, 1417.448177126915425, 233.3079752067678783 ) ) ;
#72181=CARTESIAN_POINT ( 'NONE',  ( -1.724584671162449956, 1484.237036739869836, 182.7452427733539935 ) ) ;
#72182=CARTESIAN_POINT ( 'NONE',  ( 11.68464665229999966, 1433.115614787020149, 150.9197101507980108 ) ) ;
#72183=CARTESIAN_POINT ( 'NONE',  ( -0.9073772589629539587, 1475.052622579760055, 269.6443551920880282 ) ) ;
#72184=CARTESIAN_POINT ( 'NONE',  ( 25.38699096459989946, 1440.913060399439928, 218.4286271017939782 ) ) ;
#72187=ORIENTED_EDGE ( 'NONE', *, *, #91306, .T. ) ;
#72189=CARTESIAN_POINT ( 'NONE',  ( 12.45478753333600430, 1442.762691980110276, 206.9140754477638779 ) ) ;
#72195=CARTESIAN_POINT ( 'NONE',  ( -12.20547381490000127, 1508.837368717929849, 234.0475190257980103 ) ) ;
#72197=DIRECTION ( 'NONE',  ( 1.000000000000000000, 0.000000000000000000, 0.000000000000000000 ) ) ;
#72198=CARTESIAN_POINT ( 'NONE',  ( 2.499944954983469803, 1419.437547127799917, 141.5609276200659963 ) ) ;
#72200=CARTESIAN_POINT ( 'NONE',  ( -8.776010960647441905, 1437.272641178195499, 153.2877079375153073 ) ) ;
#72202=CARTESIAN_POINT ( 'NONE',  ( -1.126185392460000045, 1452.246737684529990, 183.5926816214980022 ) ) ;
#72205=CARTESIAN_POINT ( 'NONE',  ( -17.36569701797450094, 1415.089948427370018, 208.2953144318539671 ) ) ;
#72210=CARTESIAN_POINT ( 'NONE',  ( -17.83292639989999984, 1416.519106787530063, 211.9794219605880130 ) ) ;
#72212=VECTOR ( 'NONE', #109688, 1000.000000000000000 ) ;
#72215=CARTESIAN_POINT ( 'NONE',  ( 21.02561364274377453, 1509.697797271616992, 188.0382605465152892 ) ) ;
#72216=CARTESIAN_POINT ( 'NONE',  ( 14.81250144069860042, 1409.430324335749901, 207.2165134956449890 ) ) ;
#72217=DIRECTION ( 'NONE',  ( 0.3363363969981225110, -0.6659120918163835556, 0.6659120918162170222 ) ) ;
#72219=CARTESIAN_POINT ( 'NONE',  ( -18.52991418089999698, 1440.813075470910007, 192.5628466259980200 ) ) ;
#72222=ORIENTED_EDGE ( 'NONE', *, *, #57754, .F. ) ;
#72225=CARTESIAN_POINT ( 'NONE',  ( -12.11709951228450066, 1416.029511585980117, 194.8129639842090057 ) ) ;
#72226=CARTESIAN_POINT ( 'NONE',  ( -11.14668889100000193, 1434.019367915380144, 151.6529889640980002 ) ) ;
#72227=CARTESIAN_POINT ( 'NONE',  ( -8.373252022487429826E-10, 1467.972697941590013, 248.1685000166579869 ) ) ;
#72228=CARTESIAN_POINT ( 'NONE',  ( -20.13950479349729861, 1492.949028624929952, 190.8218133787059969 ) ) ;
#72229=CARTESIAN_POINT ( 'NONE',  ( -0.08248982457600000096, 1397.911842041330146, 222.1215842558980000 ) ) ;
#72231=CARTESIAN_POINT ( 'NONE',  ( -19.25953065130653030, 1486.268686617437652, 189.5640820582841855 ) ) ;
#72233=CARTESIAN_POINT ( 'NONE',  ( -26.79413167943010166, 1436.761919080860025, 136.7821860765010058 ) ) ;
#72236=CARTESIAN_POINT ( 'NONE',  ( -13.82697551398640101, 1435.577831593989913, 150.0135038830870258 ) ) ;
#72238=CARTESIAN_POINT ( 'NONE',  ( 16.49791572389999672, 1409.489180299430018, 193.7307885960979945 ) ) ;
#72239=PLANE ( 'NONE',  #51875 ) ;
#72242=CARTESIAN_POINT ( 'NONE',  ( 5.038677013330000065, 1414.987262866129868, 244.5742075695980020 ) ) ;
#72243=CARTESIAN_POINT ( 'NONE',  ( -26.22657672300000087, 1469.244931008629919, 207.0149935993579788 ) ) ;
#72244=CARTESIAN_POINT ( 'NONE',  ( -3.546950034939999608, 1504.656051162229915, 181.0822442398979888 ) ) ;
#72245=CARTESIAN_POINT ( 'NONE',  ( -17.83435983690000270, 1410.458698071030085, 195.0679307497979948 ) ) ;
#72247=CARTESIAN_POINT ( 'NONE',  ( -10.01186952819999831, 1415.800370259029933, 244.5548898303979968 ) ) ;
#72249=CARTESIAN_POINT ( 'NONE',  ( 1.259881505249289102, 1415.704932012589325, 232.9709734747342225 ) ) ;
#72250=CARTESIAN_POINT ( 'NONE',  ( 33.53414239590000534, 1451.742177158130062, 135.1601382658980128 ) ) ;
#72252=CARTESIAN_POINT ( 'NONE',  ( -2.500000000000000000, 1428.057245272730142, 156.8186834866980064 ) ) ;
#72258=CARTESIAN_POINT ( 'NONE',  ( -23.31956537140380092, 1409.842592781089934, 208.8535798542440034 ) ) ;
#72259=ORIENTED_EDGE ( 'NONE', *, *, #85910, .F. ) ;
#72260=CARTESIAN_POINT ( 'NONE',  ( 0.3621993321110000275, 1416.825784017230035, 227.1772709138980133 ) ) ;
#72262=CARTESIAN_POINT ( 'NONE',  ( -2.529530985780000130, 1479.773065607530043, 235.7142106943980195 ) ) ;
#72263=ORIENTED_EDGE ( 'NONE', *, *, #43723, .F. ) ;
#72264=CARTESIAN_POINT ( 'NONE',  ( 11.63666214179999869, 1425.864857562230100, 144.1663263553980130 ) ) ;
#72265=CARTESIAN_POINT ( 'NONE',  ( -12.45618235598599988, 1416.218047878440075, 222.0802500694620107 ) ) ;
#72266=CARTESIAN_POINT ( 'NONE',  ( 0.09323026570510001276, 1419.758325144530090, 184.3752198323979883 ) ) ;
#72272=CARTESIAN_POINT ( 'NONE',  ( 12.91283110541483481, 1442.898483852980235, 187.0493004153197774 ) ) ;
#72273=ORIENTED_EDGE ( 'NONE', *, *, #19568, .T. ) ;
#72274=ORIENTED_EDGE ( 'NONE', *, *, #110707, .T. ) ;
#72276=EDGE_CURVE ( 'NONE', #60533, #110334, #20584, .T. ) ;
#72278=CARTESIAN_POINT ( 'NONE',  ( 13.08557583159999993, 1509.198239579430037, 234.3544144791979988 ) ) ;
#72280=CARTESIAN_POINT ( 'NONE',  ( -4.269482153190000240, 1423.951865566630204, 184.8620142645980025 ) ) ;
#72285=CARTESIAN_POINT ( 'NONE',  ( 0.03361787647180682764, 1409.314441787272244, 232.7761456571624024 ) ) ;
#72291=ORIENTED_EDGE ( 'NONE', *, *, #33553, .T. ) ;
#72292=CARTESIAN_POINT ( 'NONE',  ( 5.757839680740000077, 1413.763055107629953, 262.6648722463980334 ) ) ;
#72294=CARTESIAN_POINT ( 'NONE',  ( 40.71506177431396623, 1443.618738248601403, 137.1015905690878185 ) ) ;
#72304=CARTESIAN_POINT ( 'NONE',  ( -2.493947715939999643, 1442.756953654919926, 150.6345094620980092 ) ) ;
#72309=CARTESIAN_POINT ( 'NONE',  ( 13.17829454071469897, 1509.452805009219901, 181.0409878138019906 ) ) ;
#72311=CARTESIAN_POINT ( 'NONE',  ( 11.96010483130011615, 1433.559153112955300, 149.8793145819948620 ) ) ;
#72312=CARTESIAN_POINT ( 'NONE',  ( 16.13570061800000133, 1417.429050015530038, 227.1491849133979883 ) ) ;
#72313=CARTESIAN_POINT ( 'NONE',  ( 0.2876204004905856815, 1410.303643508743107, 233.2107274150785656 ) ) ;
#72315=CARTESIAN_POINT ( 'NONE',  ( 45.85459148159999643, 1440.913082154319909, 268.7562765770979922 ) ) ;
#72316=CARTESIAN_POINT ( 'NONE',  ( -18.52609349599999788, 1410.056276687730133, 223.4391609856979812 ) ) ;
#72318=CARTESIAN_POINT ( 'NONE',  ( 16.85424017000000063, 1435.512808430289851, 147.9204353908980352 ) ) ;
#72319=CARTESIAN_POINT ( 'NONE',  ( 21.16806657020000060, 1508.013423686629949, 190.7674652822980192 ) ) ;
#72320=CARTESIAN_POINT ( 'NONE',  ( 23.06896861730000126, 1432.937351989309946, 217.3496264744780149 ) ) ;
#72321=CARTESIAN_POINT ( 'NONE',  ( -17.51833969970000027, 1423.339066635030122, 226.5264271338980109 ) ) ;
#72323=CARTESIAN_POINT ( 'NONE',  ( -39.55169151563139707, 1438.906647882520019, 136.4243423413529968 ) ) ;
#72325=CARTESIAN_POINT ( 'NONE',  ( 0.2082676714215480063, 1458.322912406209980, 183.0250375897019808 ) ) ;
#72326=CARTESIAN_POINT ( 'NONE',  ( -9.544533345749998787, 1409.066719050529855, 198.6089048286980017 ) ) ;
#72327=CARTESIAN_POINT ( 'NONE',  ( -13.00742463789999981, 1414.913060387329779, 199.6866883146780083 ) ) ;
#72329=CARTESIAN_POINT ( 'NONE',  ( -27.78906332080140018, 1508.131006276290009, 210.4760188063899875 ) ) ;
#72330=CARTESIAN_POINT ( 'NONE',  ( 13.19913408340000061, 1434.900406177449895, 146.4345303725980045 ) ) ;
#72331=CARTESIAN_POINT ( 'NONE',  ( -37.83686684702099967, 1436.862236044670226, 134.0999999968879877 ) ) ;
#72332=CARTESIAN_POINT ( 'NONE',  ( 5.960845302450000105, 1441.842620914080044, 183.2877535976979857 ) ) ;
#72335=CARTESIAN_POINT ( 'NONE',  ( 28.11559569350000132, 1443.570698335169936, 137.5389433186979886 ) ) ;
#72339=CARTESIAN_POINT ( 'NONE',  ( 17.68492033649999939, 1509.541129174830075, 232.7807741972980011 ) ) ;
#72340=CARTESIAN_POINT ( 'NONE',  ( -30.12632811909999830, 1467.434565237230117, 266.8625626170980354 ) ) ;
#72342=CARTESIAN_POINT ( 'NONE',  ( -19.40402912745183173, 1488.299841789603761, 189.5360758023356027 ) ) ;
#72343=DIRECTION ( 'NONE',  ( -0.7566862579294338920, 0.02642405976598289144, 0.6532439637120530662 ) ) ;
#72347=CARTESIAN_POINT ( 'NONE',  ( 22.52609269779999934, 1509.699688877929930, 227.6602567939980020 ) ) ;
#72350=CARTESIAN_POINT ( 'NONE',  ( 0.4863421998530879642, 1418.702335047680208, 184.7127968358159933 ) ) ;
#72353=CARTESIAN_POINT ( 'NONE',  ( 3.803126312677917120, 1420.824521573977336, 137.2929579002170328 ) ) ;
#72355=CARTESIAN_POINT ( 'NONE',  ( -12.54660221610000193, 1415.996778984329922, 195.2080008646979934 ) ) ;
#72357=CARTESIAN_POINT ( 'NONE',  ( 23.06615049169999665, 1409.718548108430014, 209.6838289468859955 ) ) ;
#72358=PLANE ( 'NONE',  #57073 ) ;
#72360=CARTESIAN_POINT ( 'NONE',  ( -5.381128819750470527, 1430.992662387599921, 154.5043601312420094 ) ) ;
#72363=CARTESIAN_POINT ( 'NONE',  ( 26.85785241404909840, 1488.762402825080017, 207.6809295873910060 ) ) ;
#72364=B_SPLINE_CURVE_WITH_KNOTS ( 'NONE', 3,
 ( #56858, #82607, #57966, #5897, #32196, #40042 ),
 .UNSPECIFIED., .F., .F.,
 ( 4, 2, 4 ),
 ( 0.000000000000000000, 0.5000000000000000000, 1.000000000000000000 ),
 .UNSPECIFIED. ) ;
#72367=CARTESIAN_POINT ( 'NONE',  ( -0.4731238061870000067, 1415.788375264130082, 233.4112679483980060 ) ) ;
#72368=VECTOR ( 'NONE', #12222, 1000.000000000000227 ) ;
#72371=CARTESIAN_POINT ( 'NONE',  ( -18.43681367705789853, 1485.257906025299917, 189.1833959593609791 ) ) ;
#72377=B_SPLINE_CURVE_WITH_KNOTS ( 'NONE', 3,
 ( #57818, #15217, #75709, #15752, #85189, #34793, #24167, #58357, #34242, #58908, #59469, #75166, #102528, #94139, #8475, #23636, #24709, #109315, #25267, #68426, #77361, #49953, #7933, #83534, #100348, #25820, #92481, #101419 ),
 .UNSPECIFIED., .F., .F.,
 ( 4, 3, 3, 3, 3, 3, 3, 3, 3, 4 ),
 ( -1.114100600540000041, -0.9686789198448820803, -0.7108214831117060095, -0.4506324998962669692, -0.1893315385652869498, 0.07294047128922009904, 0.3351094554373470480, 0.5965822039599320004, 0.8568144055465909403, 1.114100600540000041 ),
 .UNSPECIFIED. ) ;
#72379=CARTESIAN_POINT ( 'NONE',  ( 28.40019573429999866, 1509.157491143330162, 209.8143715515469978 ) ) ;
#72380=ORIENTED_EDGE ( 'NONE', *, *, #65887, .T. ) ;
#72383=CARTESIAN_POINT ( 'NONE',  ( -15.73408764137255034, 1409.498451079286042, 225.6596250670369272 ) ) ;
#72384=CARTESIAN_POINT ( 'NONE',  ( 0.4857469785310000177, 1507.117126404930104, 180.9629171623980142 ) ) ;
#72386=CARTESIAN_POINT ( 'NONE',  ( -24.71204467725759812, 1451.893171190130033, 136.8663216757400107 ) ) ;
#72387=DIRECTION ( 'NONE',  ( 1.000000000000000000, 0.000000000000000000, 0.000000000000000000 ) ) ;
#72388=CARTESIAN_POINT ( 'NONE',  ( 8.918237991669998976, 1409.224492122430092, 229.1880316136980014 ) ) ;
#72392=CARTESIAN_POINT ( 'NONE',  ( 40.80783872799189993, 1447.308166564819885, 134.0999999984899773 ) ) ;
#72396=ORIENTED_EDGE ( 'NONE', *, *, #7783, .F. ) ;
#72398=VERTEX_POINT ( 'NONE', #80373 ) ;
#72399=CARTESIAN_POINT ( 'NONE',  ( 9.965445173606990892, 1410.635768303481655, 229.8293632461459879 ) ) ;
#72401=CARTESIAN_POINT ( 'NONE',  ( -5.623474965688048840E-07, 1451.660737107639989, 154.0815186765750013 ) ) ;
#72403=CARTESIAN_POINT ( 'NONE',  ( -18.55485652327908142, 1445.548742844001254, 214.3589705322614805 ) ) ;
#72406=CIRCLE ( 'NONE', #47366, 1.999999999999915623 ) ;
#72407=CARTESIAN_POINT ( 'NONE',  ( -9828.720208194639781, 54.28084076250829781, -1083.674256066600037 ) ) ;
#72408=CARTESIAN_POINT ( 'NONE',  ( 3.923553339340000168, 1416.217772597929979, 190.9999006073979899 ) ) ;
#72411=ORIENTED_EDGE ( 'NONE', *, *, #86512, .T. ) ;
#72414=CARTESIAN_POINT ( 'NONE',  ( 28.19745448794409981, 1440.913060387330006, 248.0707952811780217 ) ) ;
#72415=CARTESIAN_POINT ( 'NONE',  ( -18.88961621640000033, 1507.836736047129989, 187.8591162544979909 ) ) ;
#72418=CARTESIAN_POINT ( 'NONE',  ( -3.034707026709789979, 1440.440247136690004, 157.2489849372729793 ) ) ;
#72420=CARTESIAN_POINT ( 'NONE',  ( -24.49648242109999785, 1440.984241468170012, 210.9954442990479890 ) ) ;
#72422=CARTESIAN_POINT ( 'NONE',  ( 13.74454213900000177, 1436.216140752829915, 150.3798544741980265 ) ) ;
#72423=CARTESIAN_POINT ( 'NONE',  ( 39.21111056970000419, 1422.625647128129913, 266.3742241808980111 ) ) ;
#72425=CARTESIAN_POINT ( 'NONE',  ( 25.82427654007650020, 1484.679466883040050, 206.2250770722999960 ) ) ;
#72426=CARTESIAN_POINT ( 'NONE',  ( 7.744760412899999835, 1463.664893275730037, 234.4935621930980005 ) ) ;
#72427=CARTESIAN_POINT ( 'NONE',  ( -11.60004869885203682, 1423.462184080716270, 135.7647354703441351 ) ) ;
#72428=B_SPLINE_SURFACE_WITH_KNOTS ( 'NONE', 4, 5, ( 
 ( #38572, #97384, #11734, #62163, #97926, #55951 ),
 ( #20655, #30169, #45903, #90073, #53772, #108543 ),
 ( #48097, #5538, #82237, #13912, #109652, #48662 ),
 ( #82788, #101218, #100142, #15558, #58158, #73857 ),
 ( #22299, #65465, #32394, #6082, #57064, #39117 ),
 ( #73297, #15011, #41351, #40234, #107984, #13355 ),
 ( #56501, #74964, #99572, #90630, #39689, #91189 ),
 ( #47547, #57621, #22858, #49759, #81667, #6633 ),
 ( #23428, #32928, #83888, #14470, #74417, #31281 ) ),
 .UNSPECIFIED., .F., .F., .F.,
 ( 5, 4, 5 ),
 ( 6, 6 ),
 ( 36.89059838979999739, 37.78706028239999881, 37.79602490132599968 ),
 ( 0.000000000000000000, 2.000000000000000000 ),
 .UNSPECIFIED. ) ;
#72431=CARTESIAN_POINT ( 'NONE',  ( -0.1594943249209899994, 1507.184524987769919, 180.8985575764880025 ) ) ;
#72433=CARTESIAN_POINT ( 'NONE',  ( 16.81138730642775769, 1449.242716094900288, 218.8724950056246712 ) ) ;
#72435=CARTESIAN_POINT ( 'NONE',  ( -22.03740498310000007, 1506.809279317530127, 209.2115705851809935 ) ) ;
#72437=CARTESIAN_POINT ( 'NONE',  ( -12.94448954231350868, 1519.913060387329779, 185.4271167906579478 ) ) ;
#72438=ORIENTED_EDGE ( 'NONE', *, *, #83607, .F. ) ;
#72440=CARTESIAN_POINT ( 'NONE',  ( 3.814136268639999994, 1460.517119005329960, 217.3476460196580149 ) ) ;
#72441=ADVANCED_FACE ( 'NONE', ( #13677 ), #97409, .T. ) ;
#72444=CARTESIAN_POINT ( 'NONE',  ( 2.923531254659999856, 1410.372839466330106, 231.6299449191980102 ) ) ;
#72447=CARTESIAN_POINT ( 'NONE',  ( 11.75111247159999905, 1446.815402699049855, 187.7955951978979954 ) ) ;
#72448=CARTESIAN_POINT ( 'NONE',  ( -19.47133434590000078, 1457.447441929329898, 226.1258623160980221 ) ) ;
#72449=CARTESIAN_POINT ( 'NONE',  ( 19.74393297489999810, 1455.407987973630043, 226.2017192373979810 ) ) ;
#72450=CARTESIAN_POINT ( 'NONE',  ( -2.897715842900000283, 1486.012679015429967, 182.1056253353979741 ) ) ;
#72453=CARTESIAN_POINT ( 'NONE',  ( 2.778298004749999883, 1405.778071318030015, 267.8507722644980049 ) ) ;
#72456=CARTESIAN_POINT ( 'NONE',  ( 6.422733791020810656, 1471.791680861769919, 269.8654503459380294 ) ) ;
#72462=CARTESIAN_POINT ( 'NONE',  ( 0.5699886612280750109, 1450.893155944679847, 155.0620510323830104 ) ) ;
#72463=CARTESIAN_POINT ( 'NONE',  ( -14.22819488934809939, 1415.834070662929889, 221.1563499966289896 ) ) ;
#72466=CARTESIAN_POINT ( 'NONE',  ( -20.41675352909999930, 1440.913060387330006, 219.6133834379979817 ) ) ;
#72467=CARTESIAN_POINT ( 'NONE',  ( 2.704956093210000301, 1440.760885240010111, 170.5389561584980243 ) ) ;
#72468=CARTESIAN_POINT ( 'NONE',  ( -0.5566428566430000613, 1475.834717975330022, 266.9610393015980208 ) ) ;
#72469=CARTESIAN_POINT ( 'NONE',  ( -29.80701629120000007, 1451.872188912029969, 134.8363203424979986 ) ) ;
#72470=CARTESIAN_POINT ( 'NONE',  ( -9.814778378175621043, 1424.216271979959856, 144.1582897904220033 ) ) ;
#72471=CARTESIAN_POINT ( 'NONE',  ( -3.558031533707346927, 1448.289799212619300, 184.9044431245979183 ) ) ;
#72477=CARTESIAN_POINT ( 'NONE',  ( -10.66105778724350017, 1396.285352728870066, 212.1046978785340116 ) ) ;
#72479=CARTESIAN_POINT ( 'NONE',  ( -44.92200289279999481, 1440.533167347589824, 269.6914162027979955 ) ) ;
#72485=CARTESIAN_POINT ( 'NONE',  ( 11.34308291480000008, 1426.877116246929972, 115.7237209403979961 ) ) ;
#72491=CARTESIAN_POINT ( 'NONE',  ( -11.84242369139999873, 1431.324257919750153, 147.6543138610979895 ) ) ;
#72492=CARTESIAN_POINT ( 'NONE',  ( 2.491448480239999874, 1508.759613064230052, 180.3874124875980272 ) ) ;
#72499=FACE_OUTER_BOUND ( 'NONE', #38433, .T. ) ;
#72500=CARTESIAN_POINT ( 'NONE',  ( 2.892830563952609957, 1409.416455242979964, 231.1906418284260099 ) ) ;
#72502=CARTESIAN_POINT ( 'NONE',  ( -9.251110758310000293, 1409.236116293629948, 189.6234339899980057 ) ) ;
#72503=DIRECTION ( 'NONE',  ( 0.9272802558616994872, -0.03238135539626126047, 0.3729648440694676714 ) ) ;
#72506=CARTESIAN_POINT ( 'NONE',  ( 17.38002308720000144, 1413.529868483829887, 226.0648461332980332 ) ) ;
#72507=CARTESIAN_POINT ( 'NONE',  ( 1.721725048689999760, 1429.772963309329953, 184.5251936066979965 ) ) ;
#72508=CARTESIAN_POINT ( 'NONE',  ( -38.13298815378909978, 1448.843107352490051, 136.3720512951870205 ) ) ;
#72509=B_SPLINE_CURVE_WITH_KNOTS ( 'NONE', 5,
 ( #39328, #100861, #83519, #21938, #82981, #82439, #24151, #58341, #23620, #84076, #56132, #31467 ),
 .UNSPECIFIED., .F., .F.,
 ( 6, 3, 3, 6 ),
 ( 0.000000000000000000, 0.3812068090311336310, 0.7624136180702053567, 1.000000000000000000 ),
 .UNSPECIFIED. ) ;
#72510=CARTESIAN_POINT ( 'NONE',  ( 40.69210606679339293, 1440.912522207950133, 136.6173652597990156 ) ) ;
#72511=CARTESIAN_POINT ( 'NONE',  ( 27.05712719250106701, 1435.442241411316218, 135.2793719061239130 ) ) ;
#72512=CARTESIAN_POINT ( 'NONE',  ( 33.93536013789529449, 1436.159636157269915, 136.2998715483510068 ) ) ;
#72513=CARTESIAN_POINT ( 'NONE',  ( 10.94632149490000117, 1430.668062723530056, 151.5807326048979746 ) ) ;
#72514=CARTESIAN_POINT ( 'NONE',  ( 41.65668456659999919, 1444.003990099839712, 136.1262293497980238 ) ) ;
#72515=ORIENTED_EDGE ( 'NONE', *, *, #95034, .F. ) ;
#72516=LINE ( 'NONE', #46777, #82230 ) ;
#72520=CARTESIAN_POINT ( 'NONE',  ( -14.74939910209999994, 1460.058428731729919, 231.1927315459980150 ) ) ;
#72521=FACE_OUTER_BOUND ( 'NONE', #58192, .T. ) ;
#72527=CARTESIAN_POINT ( 'NONE',  ( 2.500000000000000000, 1448.763411304559895, 157.1038816470399979 ) ) ;
#72530=CARTESIAN_POINT ( 'NONE',  ( 0.2210648319480000012, 1414.913060387329779, 225.4904991280980084 ) ) ;
#72534=B_SPLINE_SURFACE_WITH_KNOTS ( 'NONE', 5, 1, ( 
 ( #99502, #16579 ),
 ( #82165, #23357 ),
 ( #15493, #84375 ),
 ( #31214, #83820 ),
 ( #22785, #40168 ),
 ( #74351, #49140 ) ),
 .UNSPECIFIED., .F., .F., .F.,
 ( 6, 6 ),
 ( 2, 2 ),
 ( 0.000000000000000000, 52.98959944900320096 ),
 ( -1.500000000000000000, 1.500000000000000000 ),
 .UNSPECIFIED. ) ;
#72535=CARTESIAN_POINT ( 'NONE',  ( -30.18855271174454558, 1419.717913747435205, 269.4728395028291743 ) ) ;
#72536=CARTESIAN_POINT ( 'NONE',  ( -5.505226529499999799, 1409.105307133929955, 230.1454130303979753 ) ) ;
#72537=DIRECTION ( 'NONE',  ( 0.000000000000000000, 0.000000000000000000, -1.000000000000000000 ) ) ;
#72540=CARTESIAN_POINT ( 'NONE',  ( -31.87892841237279740, 1440.913060389169914, 243.7976297880429684 ) ) ;
#72541=CARTESIAN_POINT ( 'NONE',  ( 20.28287979410820085, 1497.593060318700054, 226.9821815841060300 ) ) ;
#72543=CARTESIAN_POINT ( 'NONE',  ( 20.37632423397029768, 1412.699084889349933, 270.3601818045660252 ) ) ;
#72546=CARTESIAN_POINT ( 'NONE',  ( 23.72051015330000112, 1411.111939740129856, 207.9527775095279765 ) ) ;
#72547=CARTESIAN_POINT ( 'NONE',  ( 0.01365740389280096709, 1507.932904300896780, 237.5666955293443436 ) ) ;
#72552=CARTESIAN_POINT ( 'NONE',  ( 4.176954718270289746, 1421.290050260260159, 185.1746166876249902 ) ) ;
#72553=CARTESIAN_POINT ( 'NONE',  ( -3.077130052889999856, 1417.912031963829804, 232.8375555567980086 ) ) ;
#72558=EDGE_CURVE ( 'NONE', #36324, #2313, #107099, .T. ) ;
#72559=CARTESIAN_POINT ( 'NONE',  ( -0.009082284558410000028, 1417.355061569330019, 235.2087945027979856 ) ) ;
#72560=CIRCLE ( 'NONE', #4620, 2.000000000000000000 ) ;
#72561=B_SPLINE_CURVE_WITH_KNOTS ( 'NONE', 3,
 ( #99640, #64977, #89604, #29158, #54928, #106416 ),
 .UNSPECIFIED., .F., .F.,
 ( 4, 2, 4 ),
 ( 0.000000000000000000, 0.5000000000000000000, 1.000000000000000000 ),
 .UNSPECIFIED. ) ;
#72570=ORIENTED_EDGE ( 'NONE', *, *, #2794, .F. ) ;
#72573=ORIENTED_EDGE ( 'NONE', *, *, #15031, .T. ) ;
#72579=CARTESIAN_POINT ( 'NONE',  ( -27.00783404025900225, 1509.422393139779842, 201.2804958749899811 ) ) ;
#72580=CARTESIAN_POINT ( 'NONE',  ( -2.500000000000000000, 1448.229591734839914, 165.9681906964980271 ) ) ;
#72581=CARTESIAN_POINT ( 'NONE',  ( -19.91120744939999909, 1427.184642357730127, 223.3904735300980064 ) ) ;
#72584=CARTESIAN_POINT ( 'NONE',  ( 18.78950644500000067, 1478.520229345230064, 189.7031885923980212 ) ) ;
#72585=CARTESIAN_POINT ( 'NONE',  ( 0.08580183426129689428, 1408.916056653429905, 231.7748806593529878 ) ) ;
#72586=CARTESIAN_POINT ( 'NONE',  ( 29.77420891850000118, 1509.998730826829842, 209.4122126407480096 ) ) ;
#72591=EDGE_CURVE ( 'NONE', #42283, #94550, #7510, .T. ) ;
#72594=CARTESIAN_POINT ( 'NONE',  ( -18.49117141179999990, 1508.844092022629866, 229.9893364338979893 ) ) ;
#72596=CARTESIAN_POINT ( 'NONE',  ( -13.29514579968463295, 1443.228841607992308, 186.9064473022689867 ) ) ;
#72597=CARTESIAN_POINT ( 'NONE',  ( -17.39559655639999747, 1414.988015881329829, 207.6227086602179952 ) ) ;
#72613=CARTESIAN_POINT ( 'NONE',  ( 34.22334808525543082, 1423.233184880918998, 269.5210271296780888 ) ) ;
#72614=CARTESIAN_POINT ( 'NONE',  ( -22.71362857400000124, 1462.471423925029967, 250.3594883113980245 ) ) ;
#72615=CARTESIAN_POINT ( 'NONE',  ( -20.08751159799999897, 1491.264926706829783, 190.5547343358980186 ) ) ;
#72616=CARTESIAN_POINT ( 'NONE',  ( -11.20119892960000030, 1433.868452093230189, 151.6098175551980205 ) ) ;
#72617=CARTESIAN_POINT ( 'NONE',  ( -7.082960536665612317, 1445.824516962028611, 183.6528070193931796 ) ) ;
#72618=CARTESIAN_POINT ( 'NONE',  ( -19.69623350909999715, 1485.259879109029953, 190.3329780841980323 ) ) ;
#72619=CARTESIAN_POINT ( 'NONE',  ( -14.31466601544043904, 1507.539053601158457, 232.2266900997976222 ) ) ;
#72620=DIRECTION ( 'NONE',  ( 1.988619772330852129E-13, 0.03085824620771311644, -0.9995237709234254808 ) ) ;
#72622=CARTESIAN_POINT ( 'NONE',  ( 7.492226197380000841, 1440.568647855370045, 154.1013268154979983 ) ) ;
#72623=CARTESIAN_POINT ( 'NONE',  ( 13.14097700228099974, 1428.660233805160033, 223.2339875276319958 ) ) ;
#72626=AXIS2_PLACEMENT_3D ( 'NONE', #55233, #3734, #28914 ) ;
#72627=CARTESIAN_POINT ( 'NONE',  ( 3.013314585799149801E-09, 1410.335667381920075, 257.7916050914839730 ) ) ;
#72634=CARTESIAN_POINT ( 'NONE',  ( -20.94370973279999859, 1470.568016209030020, 270.0430967339979702 ) ) ;
#72636=( BOUNDED_CURVE ( )  B_SPLINE_CURVE ( 3, ( #96510, #95955, #3579, #62385 ),
 .UNSPECIFIED., .F., .T. ) 
 B_SPLINE_CURVE_WITH_KNOTS ( ( 4, 4 ),
 ( 5.908974974280949866, 6.104714675071489793 ),
 .UNSPECIFIED. ) 
 CURVE ( )  GEOMETRIC_REPRESENTATION_ITEM ( )  RATIONAL_B_SPLINE_CURVE ( ( 1.000000000000000000, 0.9968097118645246058, 0.9968097118645246058, 1.000000000000000000 ) ) 
 REPRESENTATION_ITEM ( '' )  );
#72645=FACE_OUTER_BOUND ( 'NONE', #15459, .T. ) ;
#72647=CARTESIAN_POINT ( 'NONE',  ( -39.33011038453689423, 1423.172057499710036, 269.1477809332180300 ) ) ;
#72649=CARTESIAN_POINT ( 'NONE',  ( -3.547294053305450223, 1505.009196866179991, 181.0671712231609831 ) ) ;
#72654=CARTESIAN_POINT ( 'NONE',  ( -22.52594231189999974, 1509.699683626429987, 190.3521444180979927 ) ) ;
#72655=CARTESIAN_POINT ( 'NONE',  ( -5.956347180529999896, 1440.426868644620072, 185.7687637636979900 ) ) ;
#72656=CARTESIAN_POINT ( 'NONE',  ( -15.67479435197149940, 1461.186449370369928, 228.5358082348789992 ) ) ;
#72658=CARTESIAN_POINT ( 'NONE',  ( -26.43469822969999683, 1435.724577353250197, 136.2325690242980158 ) ) ;
#72664=EDGE_LOOP ( 'NONE', ( #58834, #46080, #16061, #40074, #15174, #27691, #30066 ) ) ;
#72665=CARTESIAN_POINT ( 'NONE',  ( -18.91874693594079915, 1412.285123103680007, 270.3614442910130151 ) ) ;
#72666=CARTESIAN_POINT ( 'NONE',  ( -2.244413413239999766, 1428.081157166129969, 101.8807690336980016 ) ) ;
#72671=EDGE_CURVE ( 'NONE', #16982, #35617, #30940, .T. ) ;
#72672=CARTESIAN_POINT ( 'NONE',  ( 39.42853080850703407, 1458.278269001917351, 269.1443194363598082 ) ) ;
#72674=CARTESIAN_POINT ( 'NONE',  ( -14.42367087132340053, 1436.254602620129845, 149.9796175991139933 ) ) ;
#72675=CARTESIAN_POINT ( 'NONE',  ( -0.03669057782753510494, 1409.908510651789811, 185.0915849681089753 ) ) ;
#72678=CARTESIAN_POINT ( 'NONE',  ( -18.72196294886500212, 1507.117986375961891, 221.9823435811830734 ) ) ;
#72681=CARTESIAN_POINT ( 'NONE',  ( -13.79590940549999978, 1416.844618645930041, 221.9094009210980118 ) ) ;
#72682=CARTESIAN_POINT ( 'NONE',  ( 12.26151716610000086, 1416.568813549730066, 223.5713197806979906 ) ) ;
#72687=CARTESIAN_POINT ( 'NONE',  ( -33.91369107984309750, 1435.681798568270096, 135.3761632788110205 ) ) ;
#72688=CARTESIAN_POINT ( 'NONE',  ( -23.85399841774137286, 1446.449082436806748, 213.6949048731282801 ) ) ;
#72690=CARTESIAN_POINT ( 'NONE',  ( 3.840665656060542776, 1457.471497273520299, 228.5188823049041957 ) ) ;
#72691=CARTESIAN_POINT ( 'NONE',  ( -27.68516857330043734, 1508.595246550359661, 210.6013668309819593 ) ) ;
#72692=CARTESIAN_POINT ( 'NONE',  ( 13.43950372030000118, 1415.041103191630100, 197.6576099831980002 ) ) ;
#72694=CARTESIAN_POINT ( 'NONE',  ( 18.14423173670000367, 1409.546670921429950, 196.7317315907980060 ) ) ;
#72695=CARTESIAN_POINT ( 'NONE',  ( -3.503071675944339880, 1446.464826362650228, 170.5350607194175154 ) ) ;
#72696=CARTESIAN_POINT ( 'NONE',  ( -26.53940720459999980, 1435.424242704579910, 135.2833523932980029 ) ) ;
#72698=CARTESIAN_POINT ( 'NONE',  ( 0.1909392970979732207, 1506.691119431691050, 186.9237900612206147 ) ) ;
#72699=CARTESIAN_POINT ( 'NONE',  ( 4.250709873168109887, 1441.341571527049837, 160.9975569674199960 ) ) ;
#72700=CARTESIAN_POINT ( 'NONE',  ( 2.500000000000349942, 1439.188131747740272, 158.6514102456989974 ) ) ;
#72708=EDGE_CURVE ( 'NONE', #63161, #67085, #45651, .T. ) ;
#72709=CARTESIAN_POINT ( 'NONE',  ( -36.20521733875069970, 1449.935881827250114, 136.2514865721049659 ) ) ;
#72710=CARTESIAN_POINT ( 'NONE',  ( 11.60004869885203682, 1425.182052903856402, 137.9775777671608523 ) ) ;
#72712=CARTESIAN_POINT ( 'NONE',  ( -2.500000000000000000, 1424.573971167730178, 154.8453096575980226 ) ) ;
#72714=CARTESIAN_POINT ( 'NONE',  ( -33.03302978810000212, 1464.710710526430148, 269.2927538329980166 ) ) ;
#72715=CARTESIAN_POINT ( 'NONE',  ( 29.11563328215180135, 1440.913060387169935, 235.3779001622630176 ) ) ;
#72716=CARTESIAN_POINT ( 'NONE',  ( -21.83283345040000256, 1508.011745662929798, 226.4479051240980141 ) ) ;
#72719=ORIENTED_EDGE ( 'NONE', *, *, #102706, .F. ) ;
#72724=CARTESIAN_POINT ( 'NONE',  ( -5.639308305133534205, 1426.925666188799596, 144.1938086916980524 ) ) ;
#72726=CARTESIAN_POINT ( 'NONE',  ( -10.37122021030000063, 1508.772071339130207, 234.9411915187980071 ) ) ;
#72729=CARTESIAN_POINT ( 'NONE',  ( 6.224176841629999402, 1407.473636846729960, 220.5349837110979934 ) ) ;
#72730=CARTESIAN_POINT ( 'NONE',  ( 0.000000000000000000, 1395.913060387330006, 209.1218459616979999 ) ) ;
#72731=CARTESIAN_POINT ( 'NONE',  ( 2.500838501690000548, 1464.655874327429956, 236.6367800689979788 ) ) ;
#72733=EDGE_LOOP ( 'NONE', ( #62171, #96059, #30717, #2074 ) ) ;
#72734=CARTESIAN_POINT ( 'NONE',  ( -1.298841827429999984, 1450.798617704459957, 182.5802580294979691 ) ) ;
#72738=CARTESIAN_POINT ( 'NONE',  ( -16.93365818059630001, 1414.971717244350202, 208.3952357857560003 ) ) ;
#72749=FACE_OUTER_BOUND ( 'NONE', #71462, .T. ) ;
#72753=AXIS2_PLACEMENT_3D ( 'NONE', #21312, #28650, #106994 ) ;
#72755=VERTEX_POINT ( 'NONE', #71331 ) ;
#72757=B_SPLINE_CURVE_WITH_KNOTS ( 'NONE', 5,
 ( #73803, #21142, #29036, #4391, #57001, #63753 ),
 .UNSPECIFIED., .F., .F.,
 ( 6, 6 ),
 ( -68.29823909129999038, -30.60719516609999857 ),
 .UNSPECIFIED. ) ;
#72758=ADVANCED_FACE ( 'NONE', ( #75697 ), #76754, .F. ) ;
#72760=CARTESIAN_POINT ( 'NONE',  ( -11.39648213456350057, 1415.089996094060098, 195.5240353112880030 ) ) ;
#72761=CARTESIAN_POINT ( 'NONE',  ( -12.68300523669999968, 1434.599391714779813, 149.8266026369979897 ) ) ;
#72762=EDGE_CURVE ( 'NONE', #43673, #7200, #89289, .T. ) ;
#72763=CARTESIAN_POINT ( 'NONE',  ( -6.811018194030011041E-10, 1468.607607974030088, 250.1015337166009829 ) ) ;
#72764=CARTESIAN_POINT ( 'NONE',  ( -20.44043492644280136, 1502.696401150339852, 190.5393524559290199 ) ) ;
#72774=CARTESIAN_POINT ( 'NONE',  ( 11.96005369018680042, 1433.558984481940115, 149.8785667304369724 ) ) ;
#72775=CARTESIAN_POINT ( 'NONE',  ( -14.07841550641330031, 1435.880379415640164, 150.0502609686649862 ) ) ;
#72778=CARTESIAN_POINT ( 'NONE',  ( 20.63995199495029809, 1409.633823393240164, 203.6085389666449998 ) ) ;
#72780=CARTESIAN_POINT ( 'NONE',  ( -15.46700379407589843, 1461.188231737419756, 228.6959062608830209 ) ) ;
#72781=EDGE_CURVE ( 'NONE', #87520, #85181, #50980, .T. ) ;
#72782=ORIENTED_EDGE ( 'NONE', *, *, #77567, .F. ) ;
#72783=CARTESIAN_POINT ( 'NONE',  ( 29.43658765630000218, 1426.244274388930080, 250.1802633497980253 ) ) ;
#72785=CARTESIAN_POINT ( 'NONE',  ( -3.505536969380000034, 1469.883756972129959, 182.5602054222979973 ) ) ;
#72786=CARTESIAN_POINT ( 'NONE',  ( -17.98939636220000082, 1410.465183404129903, 195.2754017030979981 ) ) ;
#72787=CARTESIAN_POINT ( 'NONE',  ( 21.40977039944027283, 1506.404057884778922, 204.2043969544953086 ) ) ;
#72788=CARTESIAN_POINT ( 'NONE',  ( -23.03273353839999871, 1432.943670924359822, 216.3812418159480160 ) ) ;
#72790=CARTESIAN_POINT ( 'NONE',  ( 2.563011323989787815, 1448.466148586485360, 154.6738348880471960 ) ) ;
#72791=CARTESIAN_POINT ( 'NONE',  ( 27.84004021000000151, 1451.940495779430194, 134.8938502556979984 ) ) ;
#72793=CARTESIAN_POINT ( 'NONE',  ( -5.386608739887719821, 1432.386065917429960, 154.6079987177780026 ) ) ;
#72795=DIRECTION ( 'NONE',  ( -0.7067700396628828763, 0.03085822887489574409, -0.7067700338480908950 ) ) ;
#72800=CARTESIAN_POINT ( 'NONE',  ( -23.74108481809569682, 1410.154262403590110, 208.8447893202840078 ) ) ;
#72804=CARTESIAN_POINT ( 'NONE',  ( 7.666452193948486205, 1446.704586381792069, 154.1277914733520618 ) ) ;
#72806=CARTESIAN_POINT ( 'NONE',  ( -3.866472413419999921, 1470.481908910429866, 234.9634525317979978 ) ) ;
#72809=CARTESIAN_POINT ( 'NONE',  ( -12.50239138351000001, 1416.520646088589956, 222.1348975693170189 ) ) ;
#72810=CARTESIAN_POINT ( 'NONE',  ( -0.1660195018879999929, 1419.189969043630072, 184.6475926504979839 ) ) ;
#72819=CARTESIAN_POINT ( 'NONE',  ( -16.87240959569610155, 1409.502257913620042, 196.1298155364530089 ) ) ;
#72820=CARTESIAN_POINT ( 'NONE',  ( -4.285317720289061327, 1423.936271504486967, 184.7606816147036000 ) ) ;
#72821=CARTESIAN_POINT ( 'NONE',  ( 12.35308117012139917, 1452.481681287280026, 149.4845737701170094 ) ) ;
#72825=CARTESIAN_POINT ( 'NONE',  ( -11.77874533540000002, 1433.007533761370041, 150.8097953740980017 ) ) ;
#72826=CARTESIAN_POINT ( 'NONE',  ( 0.03674529885730881684, 1409.783607822271051, 233.1033682352890253 ) ) ;
#72834=CARTESIAN_POINT ( 'NONE',  ( 10.78869837091210115, 1414.913060387399810, 222.2791104508980027 ) ) ;
#72835=CARTESIAN_POINT ( 'NONE',  ( -2.652938167623882126, 1396.005703029557480, 201.4552012694761629 ) ) ;
#72844=CARTESIAN_POINT ( 'NONE',  ( -14.45783246989999959, 1416.839692131129823, 221.3920770846980020 ) ) ;
#72849=CARTESIAN_POINT ( 'NONE',  ( 0.07204350251990000731, 1420.438792470029966, 183.3235075831980225 ) ) ;
#72850=CARTESIAN_POINT ( 'NONE',  ( 16.75937749040000213, 1417.431709849029858, 226.7626019668980177 ) ) ;
#72851=ADVANCED_FACE ( 'NONE', ( #2317 ), #78608, .F. ) ;
#72855=CARTESIAN_POINT ( 'NONE',  ( -17.33214102919999888, 1409.518312089029905, 223.0780283743980306 ) ) ;
#72856=CARTESIAN_POINT ( 'NONE',  ( 14.84366460950000111, 1435.005722275260041, 148.3982965428979810 ) ) ;
#72857=CARTESIAN_POINT ( 'NONE',  ( -0.9046944608469998927, 1420.511302084529916, 228.1910018231980075 ) ) ;
#72858=CARTESIAN_POINT ( 'NONE',  ( 20.84791299872678394, 1428.606219089622300, 221.9193619309947962 ) ) ;
#72859=CARTESIAN_POINT ( 'NONE',  ( 12.73024473090000086, 1416.833018185029914, 223.1308346796979833 ) ) ;
#72861=CARTESIAN_POINT ( 'NONE',  ( -38.08542200536700051, 1437.973992156650183, 136.5281536927070078 ) ) ;
#72862=CARTESIAN_POINT ( 'NONE',  ( 0.2106922363277919930, 1456.959421693720060, 183.0835369170150102 ) ) ;
#72863=CARTESIAN_POINT ( 'NONE',  ( -10.35371055715830124, 1408.750016124369949, 200.1903725439599953 ) ) ;
#72864=CARTESIAN_POINT ( 'NONE',  ( -17.05693858869999957, 1415.931669658029932, 202.9275732158079961 ) ) ;
#72866=EDGE_CURVE ( 'NONE', #50703, #60010, #87068, .T. ) ;
#72867=CARTESIAN_POINT ( 'NONE',  ( -28.14748610570159926, 1509.264785235030104, 210.8191992312090122 ) ) ;
#72868=CARTESIAN_POINT ( 'NONE',  ( 13.19895467340000117, 1434.900408194780084, 147.2732437339979867 ) ) ;
#72869=CARTESIAN_POINT ( 'NONE',  ( -39.33777288045889975, 1438.052711712020027, 134.0999999977100003 ) ) ;
#72870=FACE_OUTER_BOUND ( 'NONE', #54915, .T. ) ;
#72872=CARTESIAN_POINT ( 'NONE',  ( 1.270728227940000066, 1414.996442546130083, 191.7853923321980005 ) ) ;
#72873=CARTESIAN_POINT ( 'NONE',  ( -9.407086540023099630, 1428.119775475241568, 137.0999999980979567 ) ) ;
#72874=CARTESIAN_POINT ( 'NONE',  ( -7.883119093557859891, 1409.188344972089908, 221.8444256219010242 ) ) ;
#72878=CARTESIAN_POINT ( 'NONE',  ( -45.63712929009999897, 1440.913040511230065, 268.9747524132980061 ) ) ;
#72879=CARTESIAN_POINT ( 'NONE',  ( 19.59664182059999860, 1435.002040243510237, 209.8413840370809851 ) ) ;
#72885=CARTESIAN_POINT ( 'NONE',  ( -28.35149942255360145, 1508.694958915340067, 208.8230497516570381 ) ) ;
#72886=CARTESIAN_POINT ( 'NONE',  ( 2.581714097353351889, 1419.606499247553529, 137.0999999980980135 ) ) ;
#72887=CARTESIAN_POINT ( 'NONE',  ( 0.4891117522232159565, 1417.821273825019944, 184.7505294229070216 ) ) ;
#72889=CARTESIAN_POINT ( 'NONE',  ( -11.87970252420000072, 1508.569810688830103, 183.0303274090979926 ) ) ;
#72890=CARTESIAN_POINT ( 'NONE',  ( 4.897299265963440007, 1421.905024103366259, 138.0290641785962009 ) ) ;
#72892=CARTESIAN_POINT ( 'NONE',  ( -0.07306891522338199163, 1420.163695034950024, 183.7345046574349965 ) ) ;
#72894=EDGE_CURVE ( 'NONE', #80364, #19422, #62687, .T. ) ;
#72895=CARTESIAN_POINT ( 'NONE',  ( 22.02607710719999901, 1409.682227949630033, 213.2973235375779950 ) ) ;
#72896=FACE_OUTER_BOUND ( 'NONE', #58602, .T. ) ;
#72898=CARTESIAN_POINT ( 'NONE',  ( -18.00891941800000140, 1424.550924635830143, 228.0706972725979824 ) ) ;
#72900=CARTESIAN_POINT ( 'NONE',  ( -11.66434316710000019, 1426.744466202629837, 138.9734773543980282 ) ) ;
#72904=CARTESIAN_POINT ( 'NONE',  ( -1.879696342130000142, 1417.130803178230053, 233.8217075207979860 ) ) ;
#72907=EDGE_CURVE ( 'NONE', #66206, #23409, #101712, .T. ) ;
#72909=CARTESIAN_POINT ( 'NONE',  ( -8.525248407514739668, 1485.814754067230069, 183.6819159046639811 ) ) ;
#72913=CIRCLE ( 'NONE', #1451, 13.01015689117599194 ) ;
#72916=EDGE_CURVE ( 'NONE', #22669, #92171, #47023, .T. ) ;
#72918=CARTESIAN_POINT ( 'NONE',  ( 28.65017561800000223, 1509.591492509430054, 210.6114885952979989 ) ) ;
#72922=CARTESIAN_POINT ( 'NONE',  ( 15.72893663209239890, 1412.349048870499928, 191.4707002167729968 ) ) ;
#72923=CARTESIAN_POINT ( 'NONE',  ( 15.72580792003489947, 1409.716081128220139, 192.1010822671919982 ) ) ;
#72925=CARTESIAN_POINT ( 'NONE',  ( -25.06305140060980108, 1451.591299545579886, 137.0985386837109843 ) ) ;
#72926=CARTESIAN_POINT ( 'NONE',  ( -11.73707087880000088, 1426.695959143629807, 144.1731741466979884 ) ) ;
#72927=CARTESIAN_POINT ( 'NONE',  ( 11.55483592659999914, 1410.690417346330150, 229.2024983323979939 ) ) ;
#72930=CARTESIAN_POINT ( 'NONE',  ( 41.65423399716409847, 1444.110307755000122, 134.0999999982789745 ) ) ;
#72931=CARTESIAN_POINT ( 'NONE',  ( -39.90911398472610472, 1441.456692148860157, 136.8748725833579840 ) ) ;
#72933=CARTESIAN_POINT ( 'NONE',  ( 3.746090737668994031, 1425.475261178803976, 185.1844613459034576 ) ) ;
#72938=CARTESIAN_POINT ( 'NONE',  ( 0.2178194638410000106, 1452.982787315429960, 183.2541300742979899 ) ) ;
#72939=CIRCLE ( 'NONE', #46180, 23.05825808840000946 ) ;
#72940=CARTESIAN_POINT ( 'NONE',  ( -2.981888917330000055, 1484.262615835429870, 183.3265128428980120 ) ) ;
#72941=EDGE_CURVE ( 'NONE', #85887, #59575, #8036, .T. ) ;
#72945=CARTESIAN_POINT ( 'NONE',  ( 28.04656794799999986, 1508.051246012029878, 208.1255033510109911 ) ) ;
#72947=EDGE_CURVE ( 'NONE', #33227, #28182, #76275, .T. ) ;
#72948=CARTESIAN_POINT ( 'NONE',  ( 7.646911088080000418, 1414.913060387329779, 194.5277328420979757 ) ) ;
#72954=CARTESIAN_POINT ( 'NONE',  ( 35.98947194835299968, 1440.913060387330006, 262.2736039185940058 ) ) ;
#72955=CARTESIAN_POINT ( 'NONE',  ( 18.74558053519999845, 1457.022375937530114, 227.2948936758980096 ) ) ;
#72963=CARTESIAN_POINT ( 'NONE',  ( -3.540693246070000022, 1508.270058569329876, 180.7688421415979860 ) ) ;
#72964=CARTESIAN_POINT ( 'NONE',  ( -11.87952668650000021, 1433.311289539269865, 147.8551187025980198 ) ) ;
#72965=CARTESIAN_POINT ( 'NONE',  ( 26.80046753784469971, 1506.622207043549906, 206.2312287904520076 ) ) ;
#72966=CARTESIAN_POINT ( 'NONE',  ( 6.084791432159999403, 1464.440196481730027, 234.2785017269980017 ) ) ;
#72970=CARTESIAN_POINT ( 'NONE',  ( -22.59789932822333114, 1409.702173780693784, 209.4225277437891179 ) ) ;
#72972=CARTESIAN_POINT ( 'NONE',  ( 6.232532001850000114, 1407.162969929529936, 220.5304192662980256 ) ) ;
#72974=B_SPLINE_CURVE_WITH_KNOTS ( 'NONE', 5,
 ( #79967, #3284, #20580, #80524, #37967, #72148, #103223, #26532, #92761, #83266, #100064, #40160, #60728, #91664, #74343, #84367, #110121, #99494, #41813, #22777, #14390 ),
 .UNSPECIFIED., .F., .F.,
 ( 6, 3, 3, 3, 3, 3, 6 ),
 ( 37.33063420879999939, 38.00991709350000036, 40.59642292560000243, 43.18292875779999918, 44.87875381330000124, 46.52360639289999966, 48.64583233200000478 ),
 .UNSPECIFIED. ) ;
#72975=CARTESIAN_POINT ( 'NONE',  ( 18.63433765150000099, 1508.246382733229893, 188.5113568914979965 ) ) ;
#72980=CARTESIAN_POINT ( 'NONE',  ( 7.601478266899999170, 1459.957272486130023, 217.3594088466479946 ) ) ;
#72981=CARTESIAN_POINT ( 'NONE',  ( -11.85693426559999963, 1431.696772119709976, 149.9476199621979902 ) ) ;
#72984=FACE_OUTER_BOUND ( 'NONE', #107780, .T. ) ;
#72985=CARTESIAN_POINT ( 'NONE',  ( -19.79581205538870137, 1456.560075471280015, 209.4938375809250033 ) ) ;
#72986=CIRCLE ( 'NONE', #10384, 95.87905590040163872 ) ;
#72987=CARTESIAN_POINT ( 'NONE',  ( 12.53380496490000162, 1445.052233482669862, 186.0874927582979979 ) ) ;
#72988=CARTESIAN_POINT ( 'NONE',  ( -20.98155299119999739, 1444.799239553469988, 222.3056163179979876 ) ) ;
#72989=CARTESIAN_POINT ( 'NONE',  ( 19.08704549389999627, 1456.215544484829934, 225.8584252592980022 ) ) ;
#72991=VERTEX_POINT ( 'NONE', #20046 ) ;
#72994=CARTESIAN_POINT ( 'NONE',  ( 1.774875596600000049, 1405.867537697030002, 267.2336946155980399 ) ) ;
#73000=CARTESIAN_POINT ( 'NONE',  ( 24.65284846709989708, 1440.998862877870124, 212.5088464049670165 ) ) ;
#73001=CARTESIAN_POINT ( 'NONE',  ( -23.91828057749999914, 1452.077818060030040, 136.8096204223980124 ) ) ;
#73003=CARTESIAN_POINT ( 'NONE',  ( -1.466050900909950050, 1450.686205460179963, 155.3356496213909850 ) ) ;
#73004=CARTESIAN_POINT ( 'NONE',  ( -1.556377437525894969, 1451.184650619072954, 183.7355129867053734 ) ) ;
#73005=CARTESIAN_POINT ( 'NONE',  ( 2.498115803822699821, 1449.212599866119945, 155.3362470018159911 ) ) ;
#73007=CARTESIAN_POINT ( 'NONE',  ( 12.78776258890000150, 1416.851343894929869, 222.4918226423980059 ) ) ;
#73008=CARTESIAN_POINT ( 'NONE',  ( -20.41675369440000054, 1438.655740950709969, 219.6133835466979747 ) ) ;
#73010=CARTESIAN_POINT ( 'NONE',  ( 2.500000000000000000, 1439.072300154540017, 157.1879318970979966 ) ) ;
#73011=CARTESIAN_POINT ( 'NONE',  ( -2.094747537599999987, 1475.526797592629919, 269.2930943650979998 ) ) ;
#73012=CARTESIAN_POINT ( 'NONE',  ( -4.232601323828700579, 1446.314705677049915, 164.3433706556850211 ) ) ;
#73016=CARTESIAN_POINT ( 'NONE',  ( 3.827327205999999649, 1432.413060387330006, 146.1721969590979882 ) ) ;
#73021=CARTESIAN_POINT ( 'NONE',  ( -2.832629554588100174, 1396.011977991119920, 219.7725838655079826 ) ) ;
#73023=CARTESIAN_POINT ( 'NONE',  ( -14.65117625699999948, 1422.174524681930279, 228.3982350620979958 ) ) ;
#73024=CARTESIAN_POINT ( 'NONE',  ( -44.92382433299999889, 1440.913060387330006, 269.6913831256979961 ) ) ;
#73030=CARTESIAN_POINT ( 'NONE',  ( 11.41401861810000007, 1426.451055098430061, 121.0026485950980089 ) ) ;
#73032=CARTESIAN_POINT ( 'NONE',  ( 9794.298952142280541, 2837.541834147234567, -1088.485031629833202 ) ) ;
#73037=CARTESIAN_POINT ( 'NONE',  ( 3.214223997639999997, 1507.157966923930189, 181.4588691503979874 ) ) ;
#73043=VERTEX_POINT ( 'NONE', #72147 ) ;
#73045=CARTESIAN_POINT ( 'NONE',  ( 11.60004869885203682, 0.000000000000000000, 137.0999999980979851 ) ) ;
#73046=CARTESIAN_POINT ( 'NONE',  ( -7.105427357599999217E-15, 1423.509254465030153, 167.6739826277979830 ) ) ;
#73047=CARTESIAN_POINT ( 'NONE',  ( 1.440662989070000011, 1507.675818290129882, 236.8848933730980093 ) ) ;
#73048=CARTESIAN_POINT ( 'NONE',  ( -13.44029829071352289, 1444.325445693611982, 169.3641228205755169 ) ) ;
#73049=CARTESIAN_POINT ( 'NONE',  ( 3.487133837120000024, 1431.113060387329824, 227.6029907049980068 ) ) ;
#73052=CARTESIAN_POINT ( 'NONE',  ( 17.58529957360000040, 1413.534267924229880, 225.6949097933979829 ) ) ;
#73053=CARTESIAN_POINT ( 'NONE',  ( 10.37662516520000011, 1410.292580643930023, 188.8195959794979899 ) ) ;
#73055=EDGE_CURVE ( 'NONE', #64407, #104566, #21125, .T. ) ;
#73056=CARTESIAN_POINT ( 'NONE',  ( -39.04566459149999957, 1447.730051266930104, 136.5320742054979917 ) ) ;
#73057=CARTESIAN_POINT ( 'NONE',  ( 11.03661645814000103, 1396.298467526650029, 208.2457624720319984 ) ) ;
#73058=CARTESIAN_POINT ( 'NONE',  ( 1.547118986179999878, 1416.568813549730066, 190.2343231038979923 ) ) ;
#73059=CARTESIAN_POINT ( 'NONE',  ( 11.73653109249999993, 1426.280329148629789, 144.1709412064980143 ) ) ;
#73062=CARTESIAN_POINT ( 'NONE',  ( 4.218115660059999605, 1425.254488096429895, 185.4299414137979909 ) ) ;
#73066=CARTESIAN_POINT ( 'NONE',  ( -19.86657363567449863, 1497.939529676289794, 228.5868823338410039 ) ) ;
#73076=CARTESIAN_POINT ( 'NONE',  ( 0.04954745150389999742, 1508.966889293630175, 179.3740839253979971 ) ) ;
#73079=CARTESIAN_POINT ( 'NONE',  ( 18.69410140469999959, 1415.934222461130048, 210.6093379841479987 ) ) ;
#73083=CARTESIAN_POINT ( 'NONE',  ( -35.05411225082677618, 1424.110335121155231, 269.5322562813408922 ) ) ;
#73084=CARTESIAN_POINT ( 'NONE',  ( -1.953612668519999707, 1408.981282045029957, 231.3328323811979885 ) ) ;
#73085=CARTESIAN_POINT ( 'NONE',  ( -2.442490654179999457E-15, 1519.913060387329779, 186.5374469562979698 ) ) ;
#73086=EDGE_LOOP ( 'NONE', ( #96785, #108034, #27933, #28951 ) ) ;
#73087=CARTESIAN_POINT ( 'NONE',  ( -0.01304300961527469875, 1452.999749643619907, 183.2385070609109903 ) ) ;
#73088=CARTESIAN_POINT ( 'NONE',  ( -31.74795755313090240, 1440.913060389009843, 243.4509895537200066 ) ) ;
#73090=CARTESIAN_POINT ( 'NONE',  ( -0.3644052467364989889, 1465.020711461070050, 237.7552395868789858 ) ) ;
#73091=AXIS2_PLACEMENT_3D ( 'NONE', #38450, #89957, #64795 ) ;
#73092=CARTESIAN_POINT ( 'NONE',  ( 25.30727743885159953, 1414.908034988650115, 270.3546021691070109 ) ) ;
#73095=CARTESIAN_POINT ( 'NONE',  ( 23.53385057170000039, 1410.392363598830116, 208.0208997170380201 ) ) ;
#73100=CARTESIAN_POINT ( 'NONE',  ( 4.180280406913070124, 1421.234997433459966, 185.2258708144169930 ) ) ;
#73101=CARTESIAN_POINT ( 'NONE',  ( -0.6154731172430000230, 1417.919335479829897, 233.4687737631979871 ) ) ;
#73102=CARTESIAN_POINT ( 'NONE',  ( 9.482715713316885342, 1424.109889425399160, 139.1406707392753219 ) ) ;
#73105=CARTESIAN_POINT ( 'NONE',  ( -15.36551281277120040, 1420.352422733189769, 229.0210882522540032 ) ) ;
#73106=CARTESIAN_POINT ( 'NONE',  ( 0.4612165794449999967, 1416.141396914929828, 233.4958257179979739 ) ) ;
#73113=CARTESIAN_POINT ( 'NONE',  ( -26.60987491003508865, 1450.724930346239034, 136.4551442334351350 ) ) ;
#73119=CARTESIAN_POINT ( 'NONE',  ( 11.60004869885204570, 1426.273943615695998, 138.2686089212693332 ) ) ;
#73120=CARTESIAN_POINT ( 'NONE',  ( 23.21630602169999946, 1448.997447280589995, 218.4239157672980127 ) ) ;
#73121=CARTESIAN_POINT ( 'NONE',  ( 7.905726602093638533, 1438.201532849469913, 153.7305789053409057 ) ) ;
#73125=CARTESIAN_POINT ( 'NONE',  ( -3.123967365489999981, 1446.720974256299996, 162.7331173440980194 ) ) ;
#73126=CARTESIAN_POINT ( 'NONE',  ( -19.61843130789999989, 1426.543110900729744, 225.3457329349979830 ) ) ;
#73129=CARTESIAN_POINT ( 'NONE',  ( 15.40324653509999919, 1508.176740489129998, 186.7739816122980017 ) ) ;
#73131=CARTESIAN_POINT ( 'NONE',  ( -17.34555439375539976, 1433.759845372730069, 216.6575063138343182 ) ) ;
#73139=CARTESIAN_POINT ( 'NONE',  ( 1.450275408081650008, 1505.525276553959884, 181.1825906324010020 ) ) ;
#73141=CARTESIAN_POINT ( 'NONE',  ( -12.82065136370706959, 1442.853462007010876, 186.3191038284279841 ) ) ;
#73142=CARTESIAN_POINT ( 'NONE',  ( 8.999538239140179030, 1407.274461440940058, 198.9439808189530083 ) ) ;
#73146=CARTESIAN_POINT ( 'NONE',  ( 17.60611259787588523, 1410.890515051577950, 223.7447835159890985 ) ) ;
#73147=AXIS2_PLACEMENT_3D ( 'NONE', #71639, #78907, #28489 ) ;
#73148=CARTESIAN_POINT ( 'NONE',  ( 23.77649893510000112, 1435.334014145809988, 137.3596790345980025 ) ) ;
#73155=ORIENTED_EDGE ( 'NONE', *, *, #50118, .T. ) ;
#73159=CARTESIAN_POINT ( 'NONE',  ( 35.00577369931135507, 1424.057531348699285, 269.5315920939452781 ) ) ;
#73160=CARTESIAN_POINT ( 'NONE',  ( -24.64758684859999960, 1455.655050827730065, 240.2509105628980137 ) ) ;
#73161=CARTESIAN_POINT ( 'NONE',  ( -20.26716426260000148, 1499.099646743829908, 190.0126279463979984 ) ) ;
#73162=CARTESIAN_POINT ( 'NONE',  ( -11.90126260809999970, 1433.308376196790050, 149.9471563285979983 ) ) ;
#73164=CARTESIAN_POINT ( 'NONE',  ( -19.34584564980000110, 1485.639564621229965, 189.8374633502980089 ) ) ;
#73166=CARTESIAN_POINT ( 'NONE',  ( 24.71878886508709883, 1425.936351871569968, 209.5854886089860258 ) ) ;
#73168=CARTESIAN_POINT ( 'NONE',  ( -24.67000132220000097, 1440.968503961899842, 210.6876455942679911 ) ) ;
#73169=CARTESIAN_POINT ( 'NONE',  ( 6.907297471969998881, 1441.639242655719954, 154.4648439803980011 ) ) ;
#73173=CARTESIAN_POINT ( 'NONE',  ( 1.314629143778269967E-08, 1407.049767188329952, 264.9246803212090526 ) ) ;
#73178=CARTESIAN_POINT ( 'NONE',  ( -15.30542548040000028, 1471.644218537830056, 270.3573229403979781 ) ) ;
#73179=CARTESIAN_POINT ( 'NONE',  ( 13.19514936480000067, 1509.316610144029937, 234.6191713803979724 ) ) ;
#73182=CARTESIAN_POINT ( 'NONE',  ( 0.2118832605204210018, 1452.815003554979967, 183.2547493383920028 ) ) ;
#73184=LINE ( 'NONE', #69204, #89583 ) ;
#73187=CARTESIAN_POINT ( 'NONE',  ( -28.78832826715930082, 1414.041031752499975, 269.2046387276820383 ) ) ;
#73188=B_SPLINE_CURVE_WITH_KNOTS ( 'NONE', 3,
 ( #26167, #60353, #94476, #17749, #77697, #36245, #103425, #95050, #18318, #52509, #44104, #13221, #55276, #22162, #12694, #81003, #45778, #56362, #97793, #98895, #28398, #46875, #4310, #96715, #89406, #21070, #79913, #107304, #63145, #105673, #30031, #105107, #80462, #106744, #88856, #38437, #37908, #63682, #98348, #64225, #3226, #72613, #64785, #13769, #47411, #70991, #20521, #73159, #88307, #28956, #36799, #62598, #90494, #37353, #21621, #81533, #55826, #46332, #89946, #4835, #38982, #30597, #29486, #3775, #47953, #2674, #19985, #97246, #54179, #54728, #72090, #12140, #106204, #11599, #71552, #15974, #22712, #101086, #91604, #14331, #92697, #16516 ),
 .UNSPECIFIED., .F., .F.,
 ( 4, 2, 2, 2, 1, 1, 1, 1, 1, 2, 2, 2, 2, 2, 1, 1, 1, 1, 1, 1, 1, 2, 2, 2, 2, 2, 2, 2, 1, 1, 1, 1, 1, 2, 2, 2, 2, 2, 1, 1, 1, 1, 1, 2, 2, 2, 2, 1, 1, 1, 1, 2, 2, 4 ),
 ( 0.000000000000000000, 0.1250000000125275623, 0.1875000000187913851, 0.2187500000219232965, 0.2343750000234892383, 0.2421875000242721954, 0.2460937500246623000, 0.2480468750248588650, 0.2490234375249570642, 0.2495117187750076626, 0.2500000000250582888, 0.3750000000379676290, 0.4375000000444223547, 0.4687500000476496620, 0.4843750000492632046, 0.4921875000500729458, 0.4960937500504778441, 0.4980468750506802933, 0.4990234375507814901, 0.4995117188008350584, 0.4997558594258618703, 0.4998779297383753595, 0.5000000000508888487, 0.5312500000477524686, 0.5625000000446159776, 0.5937500000414795975, 0.6093750000399111855, 0.6171875000391271460, 0.6210937500387376797, 0.6230468750385455001, 0.6240234375384495769, 0.6245117187884015042, 0.6247558594133776344, 0.6248779297258629795, 0.6250000000383483245, 0.6875000000317065263, 0.7187500000283806312, 0.7343750000267115219, 0.7421875000258768562, 0.7460937500254666288, 0.7480468750252686760, 0.7490234375251770826, 0.7495117187751239030, 0.7497558594000971466, 0.7500000000250703902, 0.8125000000181976656, 0.8437500000147613033, 0.8593750000130431221, 0.8671875000121839205, 0.8710937500117614807, 0.8730468750115574217, 0.8740234375114624976, 0.8750000000113676846, 1.000000000000000000 ),
 .UNSPECIFIED. ) ;
#73189=ORIENTED_EDGE ( 'NONE', *, *, #61343, .F. ) ;
#73191=ORIENTED_EDGE ( 'NONE', *, *, #49364, .F. ) ;
#73192=ORIENTED_EDGE ( 'NONE', *, *, #66450, .T. ) ;
#73197=CARTESIAN_POINT ( 'NONE',  ( -16.37744738580000003, 1440.438196244339906, 190.1083942918979801 ) ) ;
#73198=B_SPLINE_CURVE_WITH_KNOTS ( 'NONE', 3,
 ( #8388, #22, #33583, #40345, #25733, #109226 ),
 .UNSPECIFIED., .F., .F.,
 ( 4, 2, 4 ),
 ( 0.000000000000000000, 0.5000000000000000000, 1.000000000000000000 ),
 .UNSPECIFIED. ) ;
#73199=DIRECTION ( 'NONE',  ( 0.000000000000000000, 0.000000000000000000, -1.000000000000000000 ) ) ;
#73202=CARTESIAN_POINT ( 'NONE',  ( -26.03017368029999901, 1436.520442997449891, 136.8941006876979998 ) ) ;
#73205=CARTESIAN_POINT ( 'NONE',  ( 1.546867617820790075, 1416.839692126689897, 190.2222510973109877 ) ) ;
#73207=CARTESIAN_POINT ( 'NONE',  ( -27.82281737747349837, 1416.493833913160188, 270.3515857537420288 ) ) ;
#73209=CARTESIAN_POINT ( 'NONE',  ( -2.551337388519999916, 1397.989667269630218, 196.2720235379979954 ) ) ;
#73212=ORIENTED_EDGE ( 'NONE', *, *, #51936, .F. ) ;
#73213=CARTESIAN_POINT ( 'NONE',  ( 32.91700288581939304, 1464.589777195947590, 269.2964102291147697 ) ) ;
#73215=CARTESIAN_POINT ( 'NONE',  ( -14.59020679048630065, 1436.244981818430006, 149.8726110424499893 ) ) ;
#73216=CARTESIAN_POINT ( 'NONE',  ( -0.03728987521009100026, 1409.697654410689893, 185.1798867859249924 ) ) ;
#73217=VECTOR ( 'NONE', #86469, 1000.000000000000114 ) ;
#73220=CARTESIAN_POINT ( 'NONE',  ( 3.034663161748390348, 1440.440203176670138, 157.2490260270419924 ) ) ;
#73223=CARTESIAN_POINT ( 'NONE',  ( 12.22173834910000068, 1416.311719782429918, 223.5326879811980234 ) ) ;
#73224=CARTESIAN_POINT ( 'NONE',  ( 12.37688904839999893, 1445.074465566569870, 186.3522953654979801 ) ) ;
#73228=CARTESIAN_POINT ( 'NONE',  ( -23.83739627443888409, 1446.557502124605435, 213.8096630186308573 ) ) ;
#73232=CARTESIAN_POINT ( 'NONE',  ( 24.18662061371099981, 1452.052842388240151, 136.8071046221860172 ) ) ;
#73233=CARTESIAN_POINT ( 'NONE',  ( -4.122298849506555563, 1439.983387333591963, 185.4581667231335302 ) ) ;
#73234=CARTESIAN_POINT ( 'NONE',  ( 2.431412526649999961, 1428.647745098929818, 149.4227846719979880 ) ) ;
#73235=CARTESIAN_POINT ( 'NONE',  ( 22.51990846810000235, 1410.619212186030154, 206.2037071705079825 ) ) ;
#73237=CARTESIAN_POINT ( 'NONE',  ( -24.89775108082510968, 1442.835550636541257, 210.5176539979092638 ) ) ;
#73240=DIRECTION ( 'NONE',  ( 0.000000000000000000, 0.000000000000000000, 1.000000000000000000 ) ) ;
#73242=DIRECTION ( 'NONE',  ( 1.000000000000000000, 0.000000000000000000, 0.000000000000000000 ) ) ;
#73244=ORIENTED_EDGE ( 'NONE', *, *, #76661, .F. ) ;
#73246=CARTESIAN_POINT ( 'NONE',  ( -4.161605046760000093, 1448.983014852180077, 185.0801900870980035 ) ) ;
#73248=CARTESIAN_POINT ( 'NONE',  ( 0.3220030984499608340, 1452.978637988592709, 183.2674086474032720 ) ) ;
#73249=EDGE_CURVE ( 'NONE', #64698, #2577, #6007, .T. ) ;
#73251=CARTESIAN_POINT ( 'NONE',  ( 11.60004869885203682, 1426.339115466829298, 138.4394687558738042 ) ) ;
#73252=CARTESIAN_POINT ( 'NONE',  ( -16.06428795287819966, 1416.913060341709979, 209.3174441336760196 ) ) ;
#73253=CARTESIAN_POINT ( 'NONE',  ( -2.500000000000000000, 1430.722531270429954, 157.4400244878979720 ) ) ;
#73256=CARTESIAN_POINT ( 'NONE',  ( -5.461771172978369628E-06, 1406.917628766249891, 222.1218527342900018 ) ) ;
#73257=CARTESIAN_POINT ( 'NONE',  ( 34.44461235088070339, 1440.913060385129938, 249.8013572737719983 ) ) ;
#73259=DIRECTION ( 'NONE',  ( 1.000000000000000000, 0.000000000000000000, 0.000000000000000000 ) ) ;
#73271=CARTESIAN_POINT ( 'NONE',  ( -13.29290641609999923, 1434.997135647470031, 194.5463675775980334 ) ) ;
#73275=CARTESIAN_POINT ( 'NONE',  ( 1.783238944200000065, 1465.101364307329732, 235.5168545023980187 ) ) ;
#73277=VERTEX_POINT ( 'NONE', #21270 ) ;
#73278=CARTESIAN_POINT ( 'NONE',  ( -0.3197736170449999582, 1452.655606759629791, 183.2748911062979857 ) ) ;
#73282=CARTESIAN_POINT ( 'NONE',  ( -18.15372975567069957, 1416.529254608160045, 209.0703203373900010 ) ) ;
#73285=EDGE_LOOP ( 'NONE', ( #46599, #39627, #44098 ) ) ;
#73287=EDGE_CURVE ( 'NONE', #105413, #76827, #25472, .T. ) ;
#73291=CIRCLE ( 'NONE', #50039, 0.5000000000000000000 ) ;
#73296=CARTESIAN_POINT ( 'NONE',  ( 9.328875054663598121, 1409.238831882729755, 197.4315850328979707 ) ) ;
#73297=CARTESIAN_POINT ( 'NONE',  ( 18.02092397397800028, 1424.326467398671866, 225.2005593169499775 ) ) ;
#73300=CARTESIAN_POINT ( 'NONE',  ( 26.45259648960871601, 1507.993349550278708, 202.6659236194934124 ) ) ;
#73301=VECTOR ( 'NONE', #18995, 1000.000000000000114 ) ;
#73302=CARTESIAN_POINT ( 'NONE',  ( -2.642710937080679834, 1449.302916809479939, 183.9132731832050069 ) ) ;
#73306=CARTESIAN_POINT ( 'NONE',  ( 17.74781233178610051, 1458.373075302629786, 228.4006037624550061 ) ) ;
#73307=CARTESIAN_POINT ( 'NONE',  ( -11.57148588749999973, 1434.949327167670162, 151.3949104721980063 ) ) ;
#73308=CARTESIAN_POINT ( 'NONE',  ( -2.205916257146450025E-10, 1466.549663538289906, 243.4496450869259832 ) ) ;
#73309=CARTESIAN_POINT ( 'NONE',  ( -20.59250019004760190, 1507.621919103199843, 190.3962728046239761 ) ) ;
#73315=CARTESIAN_POINT ( 'NONE',  ( -20.59684415639999955, 1507.762623717429960, 190.9355247909979880 ) ) ;
#73318=AXIS2_PLACEMENT_3D ( 'NONE', #32659, #102590, #85815 ) ;
#73319=CARTESIAN_POINT ( 'NONE',  ( -13.89810820305640071, 1435.230276586210039, 149.5229838337619981 ) ) ;
#73321=B_SPLINE_SURFACE_WITH_KNOTS ( 'NONE', 5, 4, ( 
 ( #39533, #6478, #48502, #31121, #13200 ),
 ( #47390, #99970, #49600, #58001, #66413 ),
 ( #92135, #5932, #74258, #81511, #108390 ),
 ( #89925, #22142, #56342, #83733, #5374 ),
 ( #90474, #4814, #32774, #13749, #57461 ),
 ( #47935, #23263, #31671, #65852, #98324 ) ),
 .UNSPECIFIED., .F., .F., .F.,
 ( 6, 6 ),
 ( 5, 5 ),
 ( 0.000000000000000000, 111.1101480259999903 ),
 ( 25.81581217359999769, 39.03307591160000101 ),
 .UNSPECIFIED. ) ;
#73322=CARTESIAN_POINT ( 'NONE',  ( 10.87683910581177216, 1427.022019987679414, 224.8651914639115432 ) ) ;
#73325=EDGE_LOOP ( 'NONE', ( #62799, #76635, #22458, #39728, #92655 ) ) ;
#73326=CARTESIAN_POINT ( 'NONE',  ( 33.60183515729999471, 1438.777037861339977, 248.0844435631979650 ) ) ;
#73328=CARTESIAN_POINT ( 'NONE',  ( 1.491332443579999945, 1469.880992466429916, 182.7373208613979898 ) ) ;
#73330=CARTESIAN_POINT ( 'NONE',  ( -23.40570496174960269, 1412.384583249233174, 270.0161671065278028 ) ) ;
#73332=CARTESIAN_POINT ( 'NONE',  ( -25.42953928600000069, 1428.064052528830189, 238.1443913133980175 ) ) ;
#73333=DIRECTION ( 'NONE',  ( -0.6396908461234346310, -0.7404633132259050843, 0.2061788135391205146 ) ) ;
#73334=CARTESIAN_POINT ( 'NONE',  ( -1.247677516857949989E-10, 1452.913060387320002, 152.5211338456990120 ) ) ;
#73335=CARTESIAN_POINT ( 'NONE',  ( 30.24884739909999709, 1451.401555985529967, 136.0545012092980244 ) ) ;
#73336=ORIENTED_EDGE ( 'NONE', *, *, #61669, .F. ) ;
#73339=CARTESIAN_POINT ( 'NONE',  ( 8.956493609840000758, 1509.358276789029787, 238.0100333225980194 ) ) ;
#73343=CARTESIAN_POINT ( 'NONE',  ( -22.91552897997099691, 1409.723198887639910, 208.8960376927099958 ) ) ;
#73344=EDGE_CURVE ( 'NONE', #25549, #102491, #84193, .T. ) ;
#73349=CARTESIAN_POINT ( 'NONE',  ( -3.198241401019999763, 1489.061078771829898, 235.9665387607980165 ) ) ;
#73352=CARTESIAN_POINT ( 'NONE',  ( 11.73652925620000076, 1426.280330920429833, 144.1708004945979837 ) ) ;
#73353=CARTESIAN_POINT ( 'NONE',  ( -12.74111629470790064, 1416.830086716310007, 221.9830696278120001 ) ) ;
#73356=EDGE_LOOP ( 'NONE', ( #76602, #36719, #78290, #78016 ) ) ;
#73360=DIRECTION ( 'NONE',  ( 0.9750097311986455351, 0.1381407795329493426, -0.1739918075599369285 ) ) ;
#73361=ORIENTED_EDGE ( 'NONE', *, *, #51331, .T. ) ;
#73365=CARTESIAN_POINT ( 'NONE',  ( -22.64306613040000116, 1409.703773680230142, 208.6811978374589955 ) ) ;
#73366=CARTESIAN_POINT ( 'NONE',  ( -4.567580137773889604, 1425.583738731856783, 186.2099746554915782 ) ) ;
#73371=CARTESIAN_POINT ( 'NONE',  ( 19.02704169900689735, 1456.915441405320053, 225.6706379604710264 ) ) ;
#73372=CARTESIAN_POINT ( 'NONE',  ( -10.98084453577630093, 1433.016921785290151, 151.7694248368179899 ) ) ;
#73373=CARTESIAN_POINT ( 'NONE',  ( 0.005542294731646350836, 1408.915806758429653, 231.8992816016082941 ) ) ;
#73377=CARTESIAN_POINT ( 'NONE',  ( -25.58488017426969918, 1509.794763074989987, 223.0410912172320081 ) ) ;
#73379=CARTESIAN_POINT ( 'NONE',  ( 4.897375497219999652, 1432.353341358199941, 150.0655110971979980 ) ) ;
#73381=DIRECTION ( 'NONE',  ( 0.000000000000000000, 0.000000000000000000, 1.000000000000000000 ) ) ;
#73382=CIRCLE ( 'NONE', #80567, 1.000000000000000000 ) ;
#73385=EDGE_CURVE ( 'NONE', #25549, #74855, #29450, .T. ) ;
#73387=CARTESIAN_POINT ( 'NONE',  ( -3.527569048119670203, 1486.518325592330029, 181.8541486797999767 ) ) ;
#73392=CARTESIAN_POINT ( 'NONE',  ( -0.8288084222790000899, 1440.444625599219989, 150.6821045058979962 ) ) ;
#73393=CARTESIAN_POINT ( 'NONE',  ( -13.79577745739999983, 1416.837309312929847, 221.9091491129979943 ) ) ;
#73394=CARTESIAN_POINT ( 'NONE',  ( 11.92878151090000038, 1433.442688111030066, 149.9099994665980091 ) ) ;
#73395=CARTESIAN_POINT ( 'NONE',  ( 28.52406123160000107, 1451.758636106830181, 255.3819207682979595 ) ) ;
#73396=CARTESIAN_POINT ( 'NONE',  ( 12.31551432482880060, 1414.913060387399810, 198.2593941373620225 ) ) ;
#73399=CARTESIAN_POINT ( 'NONE',  ( 13.47673469449999928, 1422.102502196930118, 228.8541257092979890 ) ) ;
#73404=CARTESIAN_POINT ( 'NONE',  ( -18.39618391109999607, 1410.051843682230128, 223.6762995290979745 ) ) ;
#73405=CARTESIAN_POINT ( 'NONE',  ( 1.548232229107720181, 1416.321686226080146, 190.3132320445130006 ) ) ;
#73406=CARTESIAN_POINT ( 'NONE',  ( 20.93328349789999976, 1508.014070803829782, 190.4233152825979971 ) ) ;
#73408=B_SPLINE_CURVE_WITH_KNOTS ( 'NONE', 5,
 ( #16487, #8108, #24889, #59096, #109488, #51226 ),
 .UNSPECIFIED., .F., .F.,
 ( 6, 6 ),
 ( 0.000000000000000000, 1.000000000000000000 ),
 .UNSPECIFIED. ) ;
#73410=CARTESIAN_POINT ( 'NONE',  ( -17.60627488151730091, 1410.895757528699960, 193.4350316887010024 ) ) ;
#73414=CARTESIAN_POINT ( 'NONE',  ( -9.790177377270000036, 1414.971287085229960, 222.6285949133980182 ) ) ;
#73415=CARTESIAN_POINT ( 'NONE',  ( 0.2093852927156230059, 1457.693901257390280, 183.0520252844249853 ) ) ;
#73416=CARTESIAN_POINT ( 'NONE',  ( -11.43679079880000060, 1409.312441922530070, 199.2442402772080072 ) ) ;
#73417=CARTESIAN_POINT ( 'NONE',  ( -14.63039435740000016, 1416.519106787730152, 198.5326739117980139 ) ) ;
#73419=CARTESIAN_POINT ( 'NONE',  ( -28.18627406427190252, 1509.319237329340012, 210.8542828833879810 ) ) ;
#73420=CARTESIAN_POINT ( 'NONE',  ( 11.94148329819999965, 1433.615059856560038, 147.6243649254979857 ) ) ;
#73421=CARTESIAN_POINT ( 'NONE',  ( -33.91369120210140409, 1435.681798817159915, 134.0999999980979851 ) ) ;
#73422=CARTESIAN_POINT ( 'NONE',  ( 11.73542121899999913, 1441.459447619979983, 188.0641116183980159 ) ) ;
#73429=ADVANCED_FACE ( 'NONE', ( #59887 ), #40564, .T. ) ;
#73431=CARTESIAN_POINT ( 'NONE',  ( -15.57748978299999898, 1507.212883763329955, 192.6976421578980023 ) ) ;
#73432=CARTESIAN_POINT ( 'NONE',  ( 45.47494684930080666, 1437.303802531743713, 268.9792534891967648 ) ) ;
#73434=CARTESIAN_POINT ( 'NONE',  ( 20.50343491230000126, 1453.154616238729886, 210.0312230869269854 ) ) ;
#73439=EDGE_CURVE ( 'NONE', #77078, #62097, #28071, .T. ) ;
#73440=CARTESIAN_POINT ( 'NONE',  ( -27.52167012439999993, 1450.663735262239925, 136.4333507960980114 ) ) ;
#73441=PLANE ( 'NONE',  #76737 ) ;
#73442=CARTESIAN_POINT ( 'NONE',  ( -16.98264939016419817, 1410.452980272770219, 226.1748295909769695 ) ) ;
#73444=EDGE_LOOP ( 'NONE', ( #97986, #23241, #19779, #40279 ) ) ;
#73447=B_SPLINE_CURVE_WITH_KNOTS ( 'NONE', 3,
 ( #83646, #92054, #14788, #67433 ),
 .UNSPECIFIED., .F., .F.,
 ( 4, 4 ),
 ( 0.000000000000000000, 1.000000000000000000 ),
 .UNSPECIFIED. ) ;
#73450=CARTESIAN_POINT ( 'NONE',  ( -0.1314651167789250008, 1419.667472256169958, 184.2940143127850092 ) ) ;
#73452=CARTESIAN_POINT ( 'NONE',  ( 0.0006788796961669999862, 1465.026769819230140, 237.7732385775979935 ) ) ;
#73453=CARTESIAN_POINT ( 'NONE',  ( 21.29410851689999973, 1409.656667046429902, 215.2264874598780011 ) ) ;
#73454=B_SPLINE_SURFACE_WITH_KNOTS ( 'NONE', 5, 5, ( 
 ( #76744, #67811, #94082, #103597, #58851, #26897 ),
 ( #16257, #61086, #95201, #8419, #17352, #51547 ),
 ( #8981, #18462, #84036, #7334, #33076, #67267 ),
 ( #101359, #43153, #50460, #34187, #77309, #68927 ),
 ( #101925, #25211, #59416, #53218, #53788, #44822 ),
 ( #11746, #45915, #78975, #2819, #104150, #1715 ) ),
 .UNSPECIFIED., .F., .F., .F.,
 ( 6, 6 ),
 ( 6, 6 ),
 ( 111.4340720229999988, 112.5451345809999992 ),
 ( 0.000000000000000000, 2.000000000000000000 ),
 .UNSPECIFIED. ) ;
#73455=CARTESIAN_POINT ( 'NONE',  ( -2.670080947820280048, 1412.658061024129893, 186.4741318146120079 ) ) ;
#73457=CARTESIAN_POINT ( 'NONE',  ( -17.59443979970000171, 1423.391293522529850, 226.3973360769979877 ) ) ;
#73459=CARTESIAN_POINT ( 'NONE',  ( 17.06591927879999915, 1409.674274255629825, 223.8482220529980111 ) ) ;
#73464=CARTESIAN_POINT ( 'NONE',  ( 18.89959486413309975, 1416.839692127159879, 210.6687135792209915 ) ) ;
#73466=CARTESIAN_POINT ( 'NONE',  ( -6.384986843198960038, 1485.140801668499989, 183.7378743282880009 ) ) ;
#73468=CARTESIAN_POINT ( 'NONE',  ( -4.230746000628669456, 1441.524192597599949, 164.6884930711709956 ) ) ;
#73473=CARTESIAN_POINT ( 'NONE',  ( 28.26971619830000293, 1508.651289825929780, 209.4063489423409976 ) ) ;
#73477=CARTESIAN_POINT ( 'NONE',  ( -8.178500771994089646, 1441.152429774469965, 153.9860759686779943 ) ) ;
#73478=CARTESIAN_POINT ( 'NONE',  ( 21.39322610469999830, 1453.000988217330132, 223.2795384177979940 ) ) ;
#73480=CARTESIAN_POINT ( 'NONE',  ( -24.17245393478090065, 1452.068978953060196, 136.5158210362200180 ) ) ;
#73482=CARTESIAN_POINT ( 'NONE',  ( 2.923521116649999918, 1410.394928919730091, 231.6309306915980244 ) ) ;
#73485=CARTESIAN_POINT ( 'NONE',  ( 35.74845714555229392, 1451.452973098439998, 134.0999999985519935 ) ) ;
#73486=CIRCLE ( 'NONE', #101316, 27.00880975787848470 ) ;
#73493=CARTESIAN_POINT ( 'NONE',  ( 13.46271771603947087, 1410.756095866311398, 228.3121742440291655 ) ) ;
#73499=B_SPLINE_CURVE_WITH_KNOTS ( 'NONE', 5,
 ( #99282, #22558, #21468, #47805, #72470, #12548 ),
 .UNSPECIFIED., .F., .F.,
 ( 6, 6 ),
 ( -0.9266590516050000614, 5.517428931161120431 ),
 .UNSPECIFIED. ) ;
#73500=CARTESIAN_POINT ( 'NONE',  ( -2.500000000000000000, 1439.624617065190023, 168.6282375182209989 ) ) ;
#73505=CARTESIAN_POINT ( 'NONE',  ( 11.41806921110000062, 1414.913060387329779, 197.3911438671979965 ) ) ;
#73510=ORIENTED_EDGE ( 'NONE', *, *, #54271, .F. ) ;
#73511=CARTESIAN_POINT ( 'NONE',  ( 11.00355868729999997, 1414.913528139930122, 222.3255397388979873 ) ) ;
#73513=ADVANCED_FACE ( 'NONE', ( #105187 ), #87572, .T. ) ;
#73514=CARTESIAN_POINT ( 'NONE',  ( -0.0002319074763942019469, 1452.464470640482432, 153.6345273712305186 ) ) ;
#73516=CARTESIAN_POINT ( 'NONE',  ( -33.91369114349999592, 1451.728768196330066, 134.7155300131979914 ) ) ;
#73523=CARTESIAN_POINT ( 'NONE',  ( 4.970023385829999363, 1406.187660922729947, 266.9514890597980070 ) ) ;
#73526=CARTESIAN_POINT ( 'NONE',  ( 16.35084419920000087, 1459.109911444630143, 230.6444591943979958 ) ) ;
#73527=CARTESIAN_POINT ( 'NONE',  ( -10.63901352068986483, 1424.089911397193191, 137.5855889613041256 ) ) ;
#73528=CARTESIAN_POINT ( 'NONE',  ( -4.733473252797362640, 1422.203616401994850, 184.7151843475826922 ) ) ;
#73530=CARTESIAN_POINT ( 'NONE',  ( -0.2728668963706926687, 1486.429877400285932, 181.7829858203650986 ) ) ;
#73534=CARTESIAN_POINT ( 'NONE',  ( 18.62446811629999743, 1507.629699719829887, 188.5309061728979998 ) ) ;
#73535=CARTESIAN_POINT ( 'NONE',  ( -11.60004869885203682, 1426.459394169735333, 139.0224411922850436 ) ) ;
#73539=CARTESIAN_POINT ( 'NONE',  ( 15.63397015710000026, 1455.915410822730109, 213.2303957300479738 ) ) ;
#73541=CARTESIAN_POINT ( 'NONE',  ( -11.75482189299999902, 1431.209516603920065, 150.7135045689980188 ) ) ;
#73544=CARTESIAN_POINT ( 'NONE',  ( 4.401092417150000102, 1420.174153566729956, 185.7217845719979721 ) ) ;
#73549=CARTESIAN_POINT ( 'NONE',  ( -20.73607666650000070, 1470.086132943030179, 225.0942381079979953 ) ) ;
#73550=CARTESIAN_POINT ( 'NONE',  ( -6.736199635445266232, 1420.681931525483833, 137.0999999980981272 ) ) ;
#73551=CARTESIAN_POINT ( 'NONE',  ( 25.98102620618460179, 1446.564900598649956, 138.2990622187049894 ) ) ;
#73554=CARTESIAN_POINT ( 'NONE',  ( 7.030088544379999860, 1406.659535857730134, 269.2761678244980317 ) ) ;
#73556=CARTESIAN_POINT ( 'NONE',  ( 0.3610052795299999451, 1409.865909187230045, 185.0540742924980009 ) ) ;
#73557=CARTESIAN_POINT ( 'NONE',  ( 18.67620478639999959, 1410.876507162430016, 194.6621290597979907 ) ) ;
#73558=EDGE_CURVE ( 'NONE', #80324, #81409, #69561, .T. ) ;
#73559=CARTESIAN_POINT ( 'NONE',  ( 24.59474210122779425, 1439.616678441558406, 212.4961791304409076 ) ) ;
#73564=CARTESIAN_POINT ( 'NONE',  ( -2.500000001420000117, 1449.201558854039831, 155.6080925163979884 ) ) ;
#73565=CARTESIAN_POINT ( 'NONE',  ( -12.32298830910000120, 1445.672643151689954, 187.1727947595979913 ) ) ;
#73566=CARTESIAN_POINT ( 'NONE',  ( -19.88442509963795857, 1485.192351728225049, 190.7964254835079885 ) ) ;
#73569=CARTESIAN_POINT ( 'NONE',  ( -3.444929440920000197, 1424.916853926129988, 224.8635561966979708 ) ) ;
#73572=CARTESIAN_POINT ( 'NONE',  ( 2.500000000000000000, 1439.577074560470010, 165.1593652681980018 ) ) ;
#73573=VECTOR ( 'NONE', #26279, 1000.000000000000114 ) ;
#73574=CARTESIAN_POINT ( 'NONE',  ( -2.102271589710000388, 1475.801440029330024, 266.9594147012980443 ) ) ;
#73575=CARTESIAN_POINT ( 'NONE',  ( -4.221728487123090012, 1446.223285440960126, 169.8967716716199732 ) ) ;
#73576=CARTESIAN_POINT ( 'NONE',  ( -18.15573260460000071, 1428.693028929629918, 192.9183044383979961 ) ) ;
#73577=ADVANCED_FACE ( 'NONE', ( #96603 ), #33829, .T. ) ;
#73578=CARTESIAN_POINT ( 'NONE',  ( -10.32949511124177633, 1486.513216322853395, 183.6385995678631389 ) ) ;
#73581=CARTESIAN_POINT ( 'NONE',  ( 12.25049518300349938, 1416.576002137149999, 223.5606104245470078 ) ) ;
#73585=CARTESIAN_POINT ( 'NONE',  ( -19.99185821690000253, 1409.775774462230174, 199.2575659085879920 ) ) ;
#73588=CARTESIAN_POINT ( 'NONE',  ( -44.34342732500000039, 1432.315964142800112, 269.0104413644979786 ) ) ;
#73590=CARTESIAN_POINT ( 'NONE',  ( -5.511118846543562100, 1410.480444842805809, 231.6789814916551506 ) ) ;
#73594=CARTESIAN_POINT ( 'NONE',  ( 10.81507089449999981, 1424.921187596630034, 144.1620444886980010 ) ) ;
#73597=CARTESIAN_POINT ( 'NONE',  ( 27.28327538803539909, 1449.032212788670222, 136.7238666261060018 ) ) ;
#73604=AXIS2_PLACEMENT_3D ( 'NONE', #55119, #45066, #71390 ) ;
#73607=ORIENTED_EDGE ( 'NONE', *, *, #19926, .F. ) ;
#73609=CARTESIAN_POINT ( 'NONE',  ( -12.25627298530000076, 1396.517938870329999, 207.5036536129880176 ) ) ;
#73610=CARTESIAN_POINT ( 'NONE',  ( -20.28244347700000105, 1409.621338920729841, 216.0116594248979993 ) ) ;
#73612=CARTESIAN_POINT ( 'NONE',  ( -13.50678276547792578, 1444.060212379681616, 169.3531415429766867 ) ) ;
#73613=CARTESIAN_POINT ( 'NONE',  ( -25.84053268629999778, 1509.815431673230023, 196.9032967497980167 ) ) ;
#73617=CARTESIAN_POINT ( 'NONE',  ( -1.362051879945949784, 1414.539935085650086, 185.4257519797239979 ) ) ;
#73618=CARTESIAN_POINT ( 'NONE',  ( 13.45197010939999949, 1429.761463759329899, 189.7509718724980132 ) ) ;
#73619=CARTESIAN_POINT ( 'NONE',  ( -11.60080416610000142, 1414.971439108430104, 195.8791986486979795 ) ) ;
#73620=CARTESIAN_POINT ( 'NONE',  ( -41.63813770664379632, 1444.512218055099993, 135.5979372019099856 ) ) ;
#73621=CARTESIAN_POINT ( 'NONE',  ( 6.227580691487869302, 1396.130532339959927, 200.0029583712910153 ) ) ;
#73622=CARTESIAN_POINT ( 'NONE',  ( 0.9297777941500000587, 1416.254459046630018, 190.2947620677979899 ) ) ;
#73623=CARTESIAN_POINT ( 'NONE',  ( 11.75224816899999958, 1426.683125471030053, 145.2383014675980064 ) ) ;
#73624=CARTESIAN_POINT ( 'NONE',  ( 41.49257106529999817, 1443.690927668370023, 136.5669627357980005 ) ) ;
#73626=CARTESIAN_POINT ( 'NONE',  ( 3.964339422799999735, 1425.349073522829940, 185.3440290947980031 ) ) ;
#73627=CARTESIAN_POINT ( 'NONE',  ( 1.514738106409309948, 1507.606285602550088, 186.2052147526660235 ) ) ;
#73631=CARTESIAN_POINT ( 'NONE',  ( -15.33872957789999880, 1460.931222701129855, 228.7803497734979885 ) ) ;
#73640=CARTESIAN_POINT ( 'NONE',  ( 17.84625751240000113, 1415.088275290029969, 210.3637142236279942 ) ) ;
#73644=CARTESIAN_POINT ( 'NONE',  ( -19.94909556640000048, 1508.591193276130070, 229.3655219236979974 ) ) ;
#73645=CARTESIAN_POINT ( 'NONE',  ( -30.76343349190171139, 1420.155678438769428, 269.4791553875487011 ) ) ;
#73646=CARTESIAN_POINT ( 'NONE',  ( -2.942223483390000283, 1409.952541811230049, 232.5239949635980281 ) ) ;
#73647=CARTESIAN_POINT ( 'NONE',  ( -4.314829847434394239, 1413.913060387330006, 201.2236029046909209 ) ) ;
#73648=EDGE_LOOP ( 'NONE', ( #6105, #35466, #5773, #42117 ) ) ;
#73649=CARTESIAN_POINT ( 'NONE',  ( -0.003590212486869529679, 1450.985003860830147, 181.7900261978950027 ) ) ;
#73650=CARTESIAN_POINT ( 'NONE',  ( -28.62889416593939984, 1440.913060387320002, 233.6045261250210103 ) ) ;
#73654=B_SPLINE_CURVE_WITH_KNOTS ( 'NONE', 5,
 ( #22407, #56609, #82354, #90744, #6187, #39802 ),
 .UNSPECIFIED., .F., .F.,
 ( 6, 6 ),
 ( -1.020974158415999922, 5.536280491647819879 ),
 .UNSPECIFIED. ) ;
#73655=CARTESIAN_POINT ( 'NONE',  ( 12.98193753819199792, 1411.684960533729964, 269.6330119701129888 ) ) ;
#73658=CARTESIAN_POINT ( 'NONE',  ( 24.12183011420000156, 1410.980265346130182, 208.8601329017200214 ) ) ;
#73659=CARTESIAN_POINT ( 'NONE',  ( -20.65862871410000423, 1509.573541660129877, 188.2595635174980089 ) ) ;
#73663=CARTESIAN_POINT ( 'NONE',  ( 4.188808935644120268, 1421.671353483030089, 184.7101618531249869 ) ) ;
#73664=CARTESIAN_POINT ( 'NONE',  ( 0.1469469801610000237, 1420.465541450629871, 183.3355677249980147 ) ) ;
#73668=ORIENTED_EDGE ( 'NONE', *, *, #59118, .T. ) ;
#73672=CARTESIAN_POINT ( 'NONE',  ( 18.79707643829999952, 1416.837309283529976, 209.8349447685179996 ) ) ;
#73674=CARTESIAN_POINT ( 'NONE',  ( 0.1425930925969999818, 1416.432970197429995, 233.7167792884980031 ) ) ;
#73685=CARTESIAN_POINT ( 'NONE',  ( 21.03123203779729877, 1507.789098030329797, 226.0655639048319756 ) ) ;
#73688=CARTESIAN_POINT ( 'NONE',  ( -0.04790324752389999580, 1506.806593731130079, 231.2201824205980074 ) ) ;
#73689=ADVANCED_FACE ( 'NONE', ( #87911 ), #77837, .F. ) ;
#73690=CARTESIAN_POINT ( 'NONE',  ( 22.30619483830000149, 1451.363309493629913, 221.4011829164979872 ) ) ;
#73693=VECTOR ( 'NONE', #102600, 1000.000000000000227 ) ;
#73695=CARTESIAN_POINT ( 'NONE',  ( 17.02668221408760019, 1422.112876149069962, 226.8213126862850118 ) ) ;
#73696=CARTESIAN_POINT ( 'NONE',  ( -2.499999995540000075, 1447.977244151060177, 159.5594115894979836 ) ) ;
#73697=CARTESIAN_POINT ( 'NONE',  ( -19.25146917829999893, 1426.258557004829754, 225.2352025288980144 ) ) ;
#73698=CARTESIAN_POINT ( 'NONE',  ( -25.78987273775174671, 1469.122194850858023, 269.4331841604852116 ) ) ;
#73700=CARTESIAN_POINT ( 'NONE',  ( 18.60936348979999977, 1461.935155496729976, 190.4888835971979972 ) ) ;
#73702=CARTESIAN_POINT ( 'NONE',  ( -20.75102955870752908, 1467.505718010989767, 269.3935093439889101 ) ) ;
#73703=ORIENTED_EDGE ( 'NONE', *, *, #7769, .F. ) ;
#73709=CARTESIAN_POINT ( 'NONE',  ( -0.02598383688650000162, 1416.108377156529968, 233.5481721888980076 ) ) ;
#73710=CARTESIAN_POINT ( 'NONE',  ( -12.96403976842712069, 1442.927061488039499, 186.4958570142325698 ) ) ;
#73713=SPHERICAL_SURFACE ( 'NONE', #15015, 2.000000000000000000 ) ;
#73719=CARTESIAN_POINT ( 'NONE',  ( 17.93635821316399870, 1424.337455629530041, 225.8600358504349970 ) ) ;
#73723=ORIENTED_EDGE ( 'NONE', *, *, #52876, .T. ) ;
#73724=EDGE_LOOP ( 'NONE', ( #81066, #64819, #5928, #99139 ) ) ;
#73728=CARTESIAN_POINT ( 'NONE',  ( -4.804950789190000293, 1465.695272584430086, 240.4142139981979938 ) ) ;
#73730=CARTESIAN_POINT ( 'NONE',  ( -11.63477288290000011, 1433.176682644480024, 151.0246002562979868 ) ) ;
#73733=CARTESIAN_POINT ( 'NONE',  ( 17.59268578599999699, 1410.455475235630047, 224.1775087684979724 ) ) ;
#73734=CARTESIAN_POINT ( 'NONE',  ( -26.87493968100000075, 1439.491391334960099, 137.1013534362979840 ) ) ;
#73736=CARTESIAN_POINT ( 'NONE',  ( 16.80709188200000170, 1415.354938809929763, 226.6316513545979774 ) ) ;
#73737=CARTESIAN_POINT ( 'NONE',  ( 0.5620975284970839425, 1416.851343896850040, 190.4751211475700075 ) ) ;
#73740=CARTESIAN_POINT ( 'NONE',  ( 5.068991372531999845E-09, 1406.036819823360247, 266.8717186750929500 ) ) ;
#73741=VERTEX_POINT ( 'NONE', #36928 ) ;
#73743=CARTESIAN_POINT ( 'NONE',  ( -11.86205860565950054, 1432.053659880270061, 149.9751002826119759 ) ) ;
#73745=CARTESIAN_POINT ( 'NONE',  ( -8.194407608160000578, 1472.709661065629916, 270.4215667392979867 ) ) ;
#73746=CARTESIAN_POINT ( 'NONE',  ( 12.70677192039999959, 1507.773872374229995, 233.3565881929980037 ) ) ;
#73755=CARTESIAN_POINT ( 'NONE',  ( -42.19526865402289673, 1426.222309814289929, 267.1071618434610286 ) ) ;
#73762=CARTESIAN_POINT ( 'NONE',  ( 41.49081953422589919, 1444.098784150369738, 136.3336049811159967 ) ) ;
#73765=CARTESIAN_POINT ( 'NONE',  ( -17.62598095200000259, 1440.442471470339797, 190.9074128188979955 ) ) ;
#73767=CARTESIAN_POINT ( 'NONE',  ( -17.54299231450000107, 1415.063410489729904, 207.9622084005079898 ) ) ;
#73769=DIRECTION ( 'NONE',  ( 0.000000000000000000, -1.000000000000000000, 0.000000000000000000 ) ) ;
#73771=CARTESIAN_POINT ( 'NONE',  ( -36.40679624375492551, 1451.403536190284058, 134.6865211625845973 ) ) ;
#73773=CARTESIAN_POINT ( 'NONE',  ( -38.85064735957119808, 1426.481882780939941, 270.1670862944069995 ) ) ;
#73775=CARTESIAN_POINT ( 'NONE',  ( -5.639077242409999968, 1396.170382959830022, 198.9228296104979847 ) ) ;
#73777=ORIENTED_EDGE ( 'NONE', *, *, #42327, .T. ) ;
#73779=CARTESIAN_POINT ( 'NONE',  ( -11.86816883041749904, 1432.490446933490148, 149.9820829498439991 ) ) ;
#73786=CARTESIAN_POINT ( 'NONE',  ( -2.754695366840110182, 1484.262296928430032, 183.2948712447399657 ) ) ;
#73787=DIRECTION ( 'NONE',  ( 0.000000000000000000, 0.000000000000000000, 1.000000000000000000 ) ) ;
#73788=CARTESIAN_POINT ( 'NONE',  ( 11.30241272710000011, 1414.983773852929744, 222.3815203350980028 ) ) ;
#73789=CARTESIAN_POINT ( 'NONE',  ( 12.22832204270000034, 1445.155618030669984, 186.6170962671980078 ) ) ;
#73791=ORIENTED_EDGE ( 'NONE', *, *, #29516, .F. ) ;
#73792=CARTESIAN_POINT ( 'NONE',  ( -42.60628463550339973, 1443.705283444799761, 134.7398504477979770 ) ) ;
#73794=CARTESIAN_POINT ( 'NONE',  ( -23.79010043309475364, 1446.860041990635182, 214.1309382182860475 ) ) ;
#73796=CARTESIAN_POINT ( 'NONE',  ( 18.07871887829625379, 1459.074710307333362, 227.9662036257006434 ) ) ;
#73797=CARTESIAN_POINT ( 'NONE',  ( -29.02628104977890189, 1509.926680457060002, 211.9910930732060024 ) ) ;
#73798=CARTESIAN_POINT ( 'NONE',  ( 13.68684928399999912, 1415.245980412430072, 197.2862492497980043 ) ) ;
#73801=B_SPLINE_CURVE_WITH_KNOTS ( 'NONE', 3,
 ( #58325, #50483, #24676, #23039, #58874, #49923, #75135, #6796, #41522, #82963, #75679, #108716, #23601 ),
 .UNSPECIFIED., .F., .F.,
 ( 4, 3, 3, 3, 4 ),
 ( -14.83961564490000029, -13.59114161543520005, -10.15622042185490059, -6.776369974453789524, -3.432288051224929859 ),
 .UNSPECIFIED. ) ;
#73802=CARTESIAN_POINT ( 'NONE',  ( 17.13422049400000446, 1410.007864041130006, 225.8552460202980114 ) ) ;
#73803=CARTESIAN_POINT ( 'NONE',  ( -24.68077630836099701, 1437.736159206269804, 210.5119845322900005 ) ) ;
#73805=CARTESIAN_POINT ( 'NONE',  ( 22.89696446689377041, 1450.775607349197571, 218.3304116664471906 ) ) ;
#73806=CARTESIAN_POINT ( 'NONE',  ( 2.500000000000000000, 1439.579545565689841, 165.8618548744180146 ) ) ;
#73807=DIRECTION ( 'NONE',  ( -0.4874171250595387694, 0.8731692540388111823, 0.000000000000000000 ) ) ;
#73811=CARTESIAN_POINT ( 'NONE',  ( -7.343342699544049739E-05, 1510.912287627390015, 179.8420056942519807 ) ) ;
#73812=CARTESIAN_POINT ( 'NONE',  ( -2.696218734819999963, 1448.944770110710124, 184.2305108069980122 ) ) ;
#73814=CARTESIAN_POINT ( 'NONE',  ( -11.15268736319570131, 1425.700851422820051, 101.7515742452400076 ) ) ;
#73816=CARTESIAN_POINT ( 'NONE',  ( 11.43192506429821087, 1425.760849248890963, 138.9701389427312961 ) ) ;
#73817=CARTESIAN_POINT ( 'NONE',  ( 2.616097128857913123, 1417.751789119419755, 233.8775321444583710 ) ) ;
#73818=CARTESIAN_POINT ( 'NONE',  ( -2.383222864668309793, 1471.336174120430087, 183.7826184400119871 ) ) ;
#73822=CARTESIAN_POINT ( 'NONE',  ( 30.16636262817999992, 1440.913060385679955, 238.8788807354779919 ) ) ;
#73823=CARTESIAN_POINT ( 'NONE',  ( 3.211105652400000121, 1415.841839642130026, 233.8555032973979735 ) ) ;
#73828=CARTESIAN_POINT ( 'NONE',  ( 13.51610093808350577, 1445.063428794548372, 206.7785865123599365 ) ) ;
#73830=CARTESIAN_POINT ( 'NONE',  ( 15.75336812958949828, 1414.913060387329779, 205.2106275740719639 ) ) ;
#73833=CARTESIAN_POINT ( 'NONE',  ( -17.59428824464819741, 1418.369366143110028, 226.0269679427519804 ) ) ;
#73834=CARTESIAN_POINT ( 'NONE',  ( -5.409864544089550087, 1440.893826657579893, 154.8143284515260234 ) ) ;
#73836=CARTESIAN_POINT ( 'NONE',  ( -16.26078157602950114, 1501.999196264480133, 224.5383738374800089 ) ) ;
#73837=CARTESIAN_POINT ( 'NONE',  ( -15.59061307530000029, 1507.637957906029897, 192.6843184329979977 ) ) ;
#73839=CARTESIAN_POINT ( 'NONE',  ( 2.095292362720000412, 1464.774291476929875, 236.0651601893980001 ) ) ;
#73842=CARTESIAN_POINT ( 'NONE',  ( -0.7457676837669999781, 1451.082419665830002, 182.3677269424979954 ) ) ;
#73845=CARTESIAN_POINT ( 'NONE',  ( -18.20034151899999841, 1415.948532224930204, 208.7150056808090142 ) ) ;
#73852=CARTESIAN_POINT ( 'NONE',  ( -11.60004869885203505, 1426.637431940826900, 134.7518097448552794 ) ) ;
#73855=CARTESIAN_POINT ( 'NONE',  ( 19.76910848268742882, 1509.626936452628797, 187.0485031433751999 ) ) ;
#73856=CARTESIAN_POINT ( 'NONE',  ( 12.48631014972050046, 1409.349091945879991, 200.9084573645220075 ) ) ;
#73857=CARTESIAN_POINT ( 'NONE',  ( 18.80431613299999682, 1425.839299934830024, 225.4579059055980110 ) ) ;
#73860=CARTESIAN_POINT ( 'NONE',  ( 26.86204993032690069, 1508.007394616730153, 206.2315948942269870 ) ) ;
#73861=CARTESIAN_POINT ( 'NONE',  ( -2.289270335424059777, 1449.884603672450112, 183.2456841540659980 ) ) ;
#73865=CARTESIAN_POINT ( 'NONE',  ( -2.500000000000000000, 1439.615672362210034, 183.5288080682979910 ) ) ;
#73867=CARTESIAN_POINT ( 'NONE',  ( -20.41179666374959822, 1501.768784456520052, 190.5662750394010061 ) ) ;
#73872=CARTESIAN_POINT ( 'NONE',  ( -46.27886737059069588, 1440.913065768309934, 267.5894398601490138 ) ) ;
#73874=CARTESIAN_POINT ( 'NONE',  ( -20.42459865780000072, 1488.376572794829826, 192.7920252002980135 ) ) ;
#73877=CARTESIAN_POINT ( 'NONE',  ( 1.284229296498709871, 1407.590765714829786, 222.1854359568369830 ) ) ;
#73878=CARTESIAN_POINT ( 'NONE',  ( -13.36099673570619828, 1435.014160632789981, 149.5726766897830089 ) ) ;
#73879=SURFACE_STYLE_USAGE ( .BOTH. , #39715 ) ;
#73880=CARTESIAN_POINT ( 'NONE',  ( 5.850881932830000132, 1422.777642752129850, 112.2633461691979875 ) ) ;
#73882=ORIENTED_EDGE ( 'NONE', *, *, #92452, .T. ) ;
#73883=CARTESIAN_POINT ( 'NONE',  ( 39.71667994350000441, 1440.913060391249928, 259.0958843719980109 ) ) ;
#73885=CARTESIAN_POINT ( 'NONE',  ( -0.5171656703849999426, 1486.441294966730084, 181.7112151590980034 ) ) ;
#73887=EDGE_CURVE ( 'NONE', #56546, #50244, #76967, .T. ) ;
#73888=CARTESIAN_POINT ( 'NONE',  ( 20.59848286226652903, 1506.575640307617050, 201.1096833366487147 ) ) ;
#73889=CARTESIAN_POINT ( 'NONE',  ( -27.78131445089999829, 1437.273604214180068, 231.6915032127979828 ) ) ;
#73890=CARTESIAN_POINT ( 'NONE',  ( -29.50368436323640609, 1509.962337460696517, 206.4587159585742597 ) ) ;
#73892=CARTESIAN_POINT ( 'NONE',  ( -8.399306680986638796, 1452.619750134839933, 151.1947243576269955 ) ) ;
#73893=CARTESIAN_POINT ( 'NONE',  ( 27.44752899740000274, 1451.502705272029971, 136.1440125272980026 ) ) ;
#73898=CARTESIAN_POINT ( 'NONE',  ( 16.81223453394349932, 1414.913060391199906, 210.6693087035600058 ) ) ;
#73900=ORIENTED_EDGE ( 'NONE', *, *, #41147, .T. ) ;
#73902=CARTESIAN_POINT ( 'NONE',  ( -22.91026015634600199, 1409.742958369740109, 209.5388009460739909 ) ) ;
#73903=ORIENTED_EDGE ( 'NONE', *, *, #96141, .F. ) ;
#73906=CARTESIAN_POINT ( 'NONE',  ( -3.905916658650000262, 1507.638362680030014, 236.6212078316980012 ) ) ;
#73908=CARTESIAN_POINT ( 'NONE',  ( 43.50346336978830664, 1452.801732798669946, 268.2946146135880099 ) ) ;
#73909=CARTESIAN_POINT ( 'NONE',  ( -12.98785519611649875, 1415.943166310999914, 221.7006290623930056 ) ) ;
#73910=CARTESIAN_POINT ( 'NONE',  ( 0.07377261094400000552, 1419.750880451330204, 184.3782704745979686 ) ) ;
#73912=VERTEX_POINT ( 'NONE', #90633 ) ;
#73915=CARTESIAN_POINT ( 'NONE',  ( 13.20732832327373885, 1443.125461821982526, 187.5576213471996994 ) ) ;
#73916=ORIENTED_EDGE ( 'NONE', *, *, #91840, .T. ) ;
#73917=ORIENTED_EDGE ( 'NONE', *, *, #4420, .T. ) ;
#73920=CARTESIAN_POINT ( 'NONE',  ( -4.315706650834171931, 1423.871734710937062, 184.5076872321269263 ) ) ;
#73926=PLANE ( 'NONE',  #28507 ) ;
#73930=CARTESIAN_POINT ( 'NONE',  ( -24.10874530002790195, 1508.417687901419868, 222.3557339921229925 ) ) ;
#73931=CARTESIAN_POINT ( 'NONE',  ( 2.409586283469999923, 1426.663880916129983, 144.1938086916980239 ) ) ;
#73932=ORIENTED_EDGE ( 'NONE', *, *, #2511, .F. ) ;
#73933=CARTESIAN_POINT ( 'NONE',  ( 11.09668834239110069, 1414.913057819769847, 222.2791104406980196 ) ) ;
#73942=CARTESIAN_POINT ( 'NONE',  ( 22.91663120903140083, 1507.606285602550088, 210.6365840681099826 ) ) ;
#73944=CARTESIAN_POINT ( 'NONE',  ( 11.88150807299999911, 1433.590365853900039, 150.5399244709980167 ) ) ;
#73951=CARTESIAN_POINT ( 'NONE',  ( 15.81588731469999942, 1422.108138393630043, 227.5712429109979951 ) ) ;
#73952=CARTESIAN_POINT ( 'NONE',  ( 0.9862806562982793235, 1410.322815818307618, 232.9487999948802610 ) ) ;
#73954=SPHERICAL_SURFACE ( 'NONE', #3449, 2.000000000000000000 ) ;
#73955=CARTESIAN_POINT ( 'NONE',  ( 5.511665417999469900E-05, 1508.970066526555001, 238.8757070596369942 ) ) ;
#73963=CARTESIAN_POINT ( 'NONE',  ( -10.58917179050000001, 1416.519106787530063, 223.7522405382979684 ) ) ;
#73964=CARTESIAN_POINT ( 'NONE',  ( 0.2176556265100970111, 1453.071422968439947, 183.2503276199190339 ) ) ;
#73965=CARTESIAN_POINT ( 'NONE',  ( -10.09629858792809820, 1408.224493087130213, 200.4271526767499836 ) ) ;
#73966=CARTESIAN_POINT ( 'NONE',  ( -17.23902921200000193, 1416.518938591829965, 202.8396764550879823 ) ) ;
#73967=CARTESIAN_POINT ( 'NONE',  ( -28.85025895338739588, 1509.857219934619934, 211.4429886291059972 ) ) ;
#73968=CARTESIAN_POINT ( 'NONE',  ( 12.06109101570000064, 1433.903535342440136, 148.5015073091980184 ) ) ;
#73969=CARTESIAN_POINT ( 'NONE',  ( -27.26082647600000186, 1435.920819023299828, 136.5169790846980220 ) ) ;
#73970=CARTESIAN_POINT ( 'NONE',  ( 10.96698248110000051, 1442.551897621980061, 185.4780326627980003 ) ) ;
#73973=CARTESIAN_POINT ( 'NONE',  ( -11.60004869885203860, 1428.965959225140750, 137.0999999980979851 ) ) ;
#73976=EDGE_CURVE ( 'NONE', #87520, #96030, #86341, .T. ) ;
#73977=CARTESIAN_POINT ( 'NONE',  ( -1.297832609859999931, 1452.391379596130037, 183.7169094889979988 ) ) ;
#73978=CARTESIAN_POINT ( 'NONE',  ( 14.88455046320870068, 1507.555441264370074, 232.3243942964739972 ) ) ;
#73979=CARTESIAN_POINT ( 'NONE',  ( 39.98720484010659248, 1424.431172289532697, 269.1289939770674664 ) ) ;
#73980=CARTESIAN_POINT ( 'NONE',  ( -19.57278477748463530, 1493.745073078330051, 189.3793122366375030 ) ) ;
#73985=CARTESIAN_POINT ( 'NONE',  ( -26.79413315976150045, 1435.433175095809929, 135.2874648155150226 ) ) ;
#73986=EDGE_LOOP ( 'NONE', ( #34214, #106005, #36737, #83374 ) ) ;
#73988=CARTESIAN_POINT ( 'NONE',  ( -16.18192080235260022, 1409.728958692500100, 226.0642444559119895 ) ) ;
#73990=ORIENTED_EDGE ( 'NONE', *, *, #93355, .T. ) ;
#73991=DIRECTION ( 'NONE',  ( 3.772597702940000410E-15, 3.330669073880000444E-15, -1.000000000000000000 ) ) ;
#73993=B_SPLINE_CURVE_WITH_KNOTS ( 'NONE', 5,
 ( #41860, #35111, #34007, #76013, #77135, #102304, #110166, #49727, #16621, #42409, #25591, #17726, #59782, #93902, #17168 ),
 .UNSPECIFIED., .F., .F.,
 ( 6, 3, 3, 3, 6 ),
 ( 7.637039622810000594, 10.13387562650000007, 11.38229362830000113, 12.23404602909999994, 12.63071163020000043 ),
 .UNSPECIFIED. ) ;
#73997=CARTESIAN_POINT ( 'NONE',  ( 0.4259571265750000113, 1466.740460378930038, 235.5880773660980196 ) ) ;
#73998=CARTESIAN_POINT ( 'NONE',  ( 18.08473414950000091, 1409.544593222829917, 221.2175231340980019 ) ) ;
#74001=CARTESIAN_POINT ( 'NONE',  ( -17.17385843950000179, 1423.847787907029897, 228.5629967713979909 ) ) ;
#74003=CARTESIAN_POINT ( 'NONE',  ( 1.228114002177200126, 1450.757138880049979, 181.5372592238319953 ) ) ;
#74004=CARTESIAN_POINT ( 'NONE',  ( 26.57998359885230144, 1469.327412704790049, 209.4675454856640044 ) ) ;
#74006=CARTESIAN_POINT ( 'NONE',  ( 3.820260774390000039E-10, 1453.313060387329870, 228.7984261690980077 ) ) ;
#74011=CARTESIAN_POINT ( 'NONE',  ( -6.599338478058309754, 1485.999004717200023, 182.7565567968090079 ) ) ;
#74012=EDGE_LOOP ( 'NONE', ( #79887, #50378, #982, #83666, #24951 ) ) ;
#74016=EDGE_LOOP ( 'NONE', ( #2091, #16437, #87896, #31022, #14776 ) ) ;
#74018=ORIENTED_EDGE ( 'NONE', *, *, #49453, .T. ) ;
#74020=ADVANCED_FACE ( 'NONE', ( #64362 ), #59786, .T. ) ;
#74022=CARTESIAN_POINT ( 'NONE',  ( -10.81674490862216587, 1424.920146621146387, 144.2681340705726996 ) ) ;
#74023=CARTESIAN_POINT ( 'NONE',  ( 15.93480775089659751, 1410.857278985090034, 191.5296905502239895 ) ) ;
#74026=ADVANCED_FACE ( 'NONE', ( #109116 ), #28557, .T. ) ;
#74032=CARTESIAN_POINT ( 'NONE',  ( 38.87405678795120423, 1449.786581495179917, 134.0999999981590065 ) ) ;
#74033=FACE_OUTER_BOUND ( 'NONE', #107056, .T. ) ;
#74034=ORIENTED_EDGE ( 'NONE', *, *, #74444, .F. ) ;
#74036=CARTESIAN_POINT ( 'NONE',  ( -18.64140136670000203, 1458.043073665729935, 227.4221190980979941 ) ) ;
#74037=ORIENTED_EDGE ( 'NONE', *, *, #61122, .F. ) ;
#74038=ORIENTED_EDGE ( 'NONE', *, *, #51945, .T. ) ;
#74041=CARTESIAN_POINT ( 'NONE',  ( 7.859233469507785230, 1410.563491206050458, 230.5393502882801897 ) ) ;
#74042=CARTESIAN_POINT ( 'NONE',  ( 3.774742873677630645E-15, 1432.353321343819971, 155.3998100167600001 ) ) ;
#74043=DIRECTION ( 'NONE',  ( 0.000000000000000000, 0.000000000000000000, -1.000000000000000000 ) ) ;
#74045=CARTESIAN_POINT ( 'NONE',  ( -2.500000000000000000, 1439.624612762049992, 169.0979939332570154 ) ) ;
#74047=CARTESIAN_POINT ( 'NONE',  ( 40.71747596219820053, 1448.637563214439979, 135.0591086893190038 ) ) ;
#74049=PLANE ( 'NONE',  #40940 ) ;
#74051=ADVANCED_FACE ( 'NONE', ( #86650 ), #104003, .F. ) ;
#74057=CARTESIAN_POINT ( 'NONE',  ( 36.80170786347940037, 1440.913060387330006, 263.3930352349019586 ) ) ;
#74059=CARTESIAN_POINT ( 'NONE',  ( -0.0002133035632435401063, 1452.198735795263474, 153.8525164413085804 ) ) ;
#74060=ORIENTED_EDGE ( 'NONE', *, *, #76681, .T. ) ;
#74061=CARTESIAN_POINT ( 'NONE',  ( -33.92644755664575484, 1451.728309075015204, 135.1499336227579420 ) ) ;
#74066=CARTESIAN_POINT ( 'NONE',  ( -12.87559654649999885, 1416.820969729929857, 221.9332893899980093 ) ) ;
#74068=CARTESIAN_POINT ( 'NONE',  ( -2.864908171889999799, 1508.665746313929958, 180.3512637796979732 ) ) ;
#74069=EDGE_CURVE ( 'NONE', #52697, #15766, #88867, .T. ) ;
#74070=CARTESIAN_POINT ( 'NONE',  ( -11.87595595039999807, 1433.006363244510112, 146.4341588726979921 ) ) ;
#74072=CARTESIAN_POINT ( 'NONE',  ( 13.98523055529999937, 1460.766604684630011, 232.5051451957979793 ) ) ;
#74073=CARTESIAN_POINT ( 'NONE',  ( -11.60004869885203860, 1422.222932908415032, 137.0999999980989230 ) ) ;
#74077=VERTEX_POINT ( 'NONE', #73737 ) ;
#74078=EDGE_CURVE ( 'NONE', #106610, #66046, #39472, .T. ) ;
#74079=LINE ( 'NONE', #57831, #8624 ) ;
#74080=CARTESIAN_POINT ( 'NONE',  ( -0.08433784210662320646, 1508.474253462899924, 180.2861765906610003 ) ) ;
#74081=CARTESIAN_POINT ( 'NONE',  ( 19.24684531284998457, 1443.257586225273144, 213.2797261564643634 ) ) ;
#74083=CARTESIAN_POINT ( 'NONE',  ( 18.59400664349999843, 1508.850372361629979, 188.2535539507980218 ) ) ;
#74084=CARTESIAN_POINT ( 'NONE',  ( -11.60004869885203682, 1426.433005303874552, 138.8017569497143029 ) ) ;
#74088=CARTESIAN_POINT ( 'NONE',  ( 23.21471032630000053, 1448.940680683610026, 217.4907001339380201 ) ) ;
#74089=CARTESIAN_POINT ( 'NONE',  ( -11.84024944870000162, 1430.562290793029888, 149.6945522165979980 ) ) ;
#74094=CARTESIAN_POINT ( 'NONE',  ( 12.39622442890000009, 1445.662712069799909, 187.7408842649980159 ) ) ;
#74095=B_SPLINE_CURVE_WITH_KNOTS ( 'NONE', 3,
 ( #85072, #59361, #43095, #33018, #8364, #25708, #33559, #24052, #94577, #102971, #67204, #68318, #101864, #41989, #59909, #77256, #26269, #16201, #60459, #94030, #49847, #58246, #17852, #66660, #92368, #83978, #101303, #58790, #36888 ),
 .UNSPECIFIED., .F., .F.,
 ( 4, 2, 2, 2, 1, 1, 2, 2, 2, 2, 1, 1, 1, 2, 2, 2, 4 ),
 ( 0.000000000000000000, 0.2499999999996999067, 0.3749999999995535238, 0.4374999999994803046, 0.4687499999995227706, 0.4843749999995431432, 0.4921874999994815814, 0.4999999999994200195, 0.6249999999994992894, 0.6874999999994761968, 0.7187499999994140243, 0.7343749999993890443, 0.7421874999993431921, 0.7460937499993604005, 0.7499999999993776090, 0.8749999999996888045, 1.000000000000000000 ),
 .UNSPECIFIED. ) ;
#74096=CARTESIAN_POINT ( 'NONE',  ( -21.39643523319999829, 1470.084198994129792, 223.9144824582980107 ) ) ;
#74097=CARTESIAN_POINT ( 'NONE',  ( -6.075418287417217122, 1422.570870580908149, 139.1419350296167750 ) ) ;
#74098=CARTESIAN_POINT ( 'NONE',  ( -2.596287949829999775, 1485.851551602029986, 182.3980973359980169 ) ) ;
#74099=EDGE_LOOP ( 'NONE', ( #31633, #76938, #102616, #109693 ) ) ;
#74101=CARTESIAN_POINT ( 'NONE',  ( 12.70479734420000106, 1407.160844702129907, 267.1691044294979633 ) ) ;
#74102=CARTESIAN_POINT ( 'NONE',  ( 0.04703880850090000343, 1408.914703018729824, 186.4620821680980214 ) ) ;
#74103=CARTESIAN_POINT ( 'NONE',  ( 17.80682964389999867, 1410.881321328729882, 193.1487614658980192 ) ) ;
#74104=EDGE_CURVE ( 'NONE', #103213, #80324, #18727, .T. ) ;
#74105=CARTESIAN_POINT ( 'NONE',  ( 24.52504064068541823, 1438.798626852492362, 212.6115771953019191 ) ) ;
#74108=CARTESIAN_POINT ( 'NONE',  ( -0.4967073565345429542, 1415.438070636819930, 233.3911243540180180 ) ) ;
#74110=CARTESIAN_POINT ( 'NONE',  ( -0.5709835574781669809, 1450.893121202140037, 154.5155306351130093 ) ) ;
#74111=CARTESIAN_POINT ( 'NONE',  ( -12.33291429870000044, 1446.185421286020073, 187.5047377990980237 ) ) ;
#74112=CARTESIAN_POINT ( 'NONE',  ( -19.85687491537112948, 1485.534782846681765, 190.5734348709216022 ) ) ;
#74113=CARTESIAN_POINT ( 'NONE',  ( -14.14026437170590000, 1415.666200591660072, 221.0665809521190113 ) ) ;
#74115=CARTESIAN_POINT ( 'NONE',  ( -8.276897555935638806, 1409.202096019020019, 196.6540098276539936 ) ) ;
#74117=EDGE_CURVE ( 'NONE', #28394, #11116, #81608, .T. ) ;
#74118=CARTESIAN_POINT ( 'NONE',  ( 10.88870480703258181, 1425.078866303880886, 139.1353458172395392 ) ) ;
#74119=CARTESIAN_POINT ( 'NONE',  ( 2.500000056489999789, 1440.197744908439972, 166.9350760962979905 ) ) ;
#74120=CARTESIAN_POINT ( 'NONE',  ( -2.086529340449999825, 1475.285345059530073, 269.4971841000979680 ) ) ;
#74121=CARTESIAN_POINT ( 'NONE',  ( -4.228535446720999680, 1446.279644958110111, 165.3431147484849930 ) ) ;
#74127=LINE ( 'NONE', #30996, #18159 ) ;
#74134=EDGE_CURVE ( 'NONE', #39656, #101005, #90939, .T. ) ;
#74135=CARTESIAN_POINT ( 'NONE',  ( -41.06045305519999289, 1425.496138736429884, 269.1004795120979907 ) ) ;
#74138=CARTESIAN_POINT ( 'NONE',  ( -8.494778598486192323, 1410.581904811623190, 230.3839334887708503 ) ) ;
#74141=CARTESIAN_POINT ( 'NONE',  ( 11.54052597689999970, 1425.927346755429880, 137.4287998514980131 ) ) ;
#74142=CARTESIAN_POINT ( 'NONE',  ( -1.547462741870939906, 1414.913060391199906, 225.9340804956229931 ) ) ;
#74144=CARTESIAN_POINT ( 'NONE',  ( 12.66727660429999958, 1410.284599989729941, 190.2680586556980131 ) ) ;
#74149=CARTESIAN_POINT ( 'NONE',  ( -13.15726454016349933, 1414.996443537369942, 220.4820293315119955 ) ) ;
#74154=CARTESIAN_POINT ( 'NONE',  ( 21.22263075940009713, 1509.591229450340052, 229.2473791923050044 ) ) ;
#74155=CARTESIAN_POINT ( 'NONE',  ( 17.38482601099109814, 1410.884446382940041, 192.4603632472940262 ) ) ;
#74158=CARTESIAN_POINT ( 'NONE',  ( -5.426610168820000801, 1398.074626792930076, 221.4287301764979929 ) ) ;
#74159=CARTESIAN_POINT ( 'NONE',  ( -21.03404397679999960, 1411.006872173530155, 218.3490652940980112 ) ) ;
#74161=CARTESIAN_POINT ( 'NONE',  ( -12.78521579352120874, 1444.986520829063011, 169.4510614378021103 ) ) ;
#74163=CARTESIAN_POINT ( 'NONE',  ( -24.72367498159999855, 1509.776430142329900, 194.9388027315980025 ) ) ;
#74168=CARTESIAN_POINT ( 'NONE',  ( 0.5282840713740000194, 1449.243076562319857, 183.4277266703979876 ) ) ;
#74169=ADVANCED_FACE ( 'NONE', ( #42312 ), #70590, .F. ) ;
#74173=CARTESIAN_POINT ( 'NONE',  ( 10.86624720370559949, 1396.292518101280166, 211.2454897527340165 ) ) ;
#74174=CARTESIAN_POINT ( 'NONE',  ( 1.163296394699999903, 1415.996778985530000, 190.3611342671979969 ) ) ;
#74175=CARTESIAN_POINT ( 'NONE',  ( 11.54437222630000015, 1429.905666691229953, 150.7682469490980282 ) ) ;
#74176=ORIENTED_EDGE ( 'NONE', *, *, #106852, .T. ) ;
#74177=CARTESIAN_POINT ( 'NONE',  ( 12.96886119409670002, 1435.558602358280041, 150.5951603274380091 ) ) ;
#74178=CARTESIAN_POINT ( 'NONE',  ( 1.694697516987165420, 1450.498567134253790, 181.7745810472625578 ) ) ;
#74179=ORIENTED_EDGE ( 'NONE', *, *, #55101, .T. ) ;
#74189=ORIENTED_EDGE ( 'NONE', *, *, #79743, .F. ) ;
#74197=CARTESIAN_POINT ( 'NONE',  ( -16.29362902913419120, 1412.794248246716506, 269.3703535479344851 ) ) ;
#74199=CARTESIAN_POINT ( 'NONE',  ( 0.2193365490036129906, 1416.521607925270018, 227.1760551913189659 ) ) ;
#74200=ORIENTED_EDGE ( 'NONE', *, *, #96960, .T. ) ;
#74201=ADVANCED_FACE ( 'NONE', ( #32130 ), #66315, .F. ) ;
#74202=CARTESIAN_POINT ( 'NONE',  ( 2.500000000000000000, 1419.382882622020134, 144.1048175974189860 ) ) ;
#74203=CARTESIAN_POINT ( 'NONE',  ( -31.32171718324010357, 1440.913060388459826, 242.2919686410689906 ) ) ;
#74206=CARTESIAN_POINT ( 'NONE',  ( -0.1883026784911550067, 1465.099972048609970, 237.0083040624210184 ) ) ;
#74207=B_SPLINE_CURVE_WITH_KNOTS ( 'NONE', 5,
 ( #103845, #102709, #10898, #96557, #103263, #94320 ),
 .UNSPECIFIED., .F., .F.,
 ( 6, 6 ),
 ( -1.452619041900000019, -1.364055982389089650E-06 ),
 .UNSPECIFIED. ) ;
#74208=CARTESIAN_POINT ( 'NONE',  ( 5.402393448019999767, 1407.889686284330082, 270.1311850753980366 ) ) ;
#74209=VECTOR ( 'NONE', #55073, 999.9999999999998863 ) ;
#74210=ADVANCED_FACE ( 'NONE', ( #93663 ), #18673, .F. ) ;
#74213=CARTESIAN_POINT ( 'NONE',  ( 22.80370811929999775, 1409.709376436929915, 209.3213622003410137 ) ) ;
#74214=CARTESIAN_POINT ( 'NONE',  ( -20.24816999180000110, 1507.884035326030016, 189.2341655923979999 ) ) ;
#74219=B_SPLINE_CURVE_WITH_KNOTS ( 'NONE', 3,
 ( #37745, #62427, #95991, #70837 ),
 .UNSPECIFIED., .F., .F.,
 ( 4, 4 ),
 ( 7.974131824220000553, 16.25123407829999778 ),
 .UNSPECIFIED. ) ;
#74220=FACE_OUTER_BOUND ( 'NONE', #40109, .T. ) ;
#74221=CARTESIAN_POINT ( 'NONE',  ( 10.97048253690000053, 1432.408103991110011, 151.7701133072980042 ) ) ;
#74223=ORIENTED_EDGE ( 'NONE', *, *, #74104, .F. ) ;
#74228=CARTESIAN_POINT ( 'NONE',  ( -5.439673085259999041, 1437.306888043809977, 154.7134238268980084 ) ) ;
#74230=CARTESIAN_POINT ( 'NONE',  ( -11.90000415720300175, 1434.913060496859998, 147.6452464505769910 ) ) ;
#74241=CARTESIAN_POINT ( 'NONE',  ( 24.39988810369999683, 1444.709222782450070, 214.8827041012880272 ) ) ;
#74242=CARTESIAN_POINT ( 'NONE',  ( 7.922665854446364619, 1438.183228455332710, 153.7218973692720283 ) ) ;
#74245=CARTESIAN_POINT ( 'NONE',  ( 15.20786797544739422, 1420.724135117424112, 227.8586414243133902 ) ) ;
#74246=CARTESIAN_POINT ( 'NONE',  ( 39.87271423621129429, 1446.097205234940020, 136.7849415641429971 ) ) ;
#74247=CARTESIAN_POINT ( 'NONE',  ( -18.79768836659999565, 1425.701458444829996, 225.3470275129980109 ) ) ;
#74248=CARTESIAN_POINT ( 'NONE',  ( -23.41638159929999929, 1435.743789844690127, 140.4321931749979910 ) ) ;
#74250=CARTESIAN_POINT ( 'NONE',  ( 17.96015235289999978, 1488.325118637129890, 189.1250949044980132 ) ) ;
#74253=CARTESIAN_POINT ( 'NONE',  ( -33.82528723393350845, 1458.993493484178998, 269.5158104617022445 ) ) ;
#74258=CARTESIAN_POINT ( 'NONE',  ( -8.010413950200000244, 1453.313060387329870, 227.4940039322979999 ) ) ;
#74259=CARTESIAN_POINT ( 'NONE',  ( -1.065145167260631354, 1486.514686996405544, 181.6828421078873248 ) ) ;
#74260=CARTESIAN_POINT ( 'NONE',  ( -13.03778803710101997, 1442.976472216123284, 186.5873176571947738 ) ) ;
#74261=B_SPLINE_SURFACE_WITH_KNOTS ( 'NONE', 5, 5, ( 
 ( #57728, #74522, #40341, #56056, #90746, #48216, #14025, #56610, #41461 ),
 ( #90183, #14583, #33037, #31940, #58265, #15659, #75623, #82355, #5655 ),
 ( #75073, #48771, #99680, #81784, #91846, #5086, #15123, #83997, #82897 ),
 ( #13466, #32507, #99129, #6734, #31388, #22408, #39803, #22972, #57178 ),
 ( #39239, #65569, #73414, #91300, #107550, #100782, #109222, #73963, #30837 ),
 ( #66135, #66677, #108653, #109757, #108093, #24073, #67225, #92386, #100256 ) ),
 .UNSPECIFIED., .F., .F., .F.,
 ( 6, 6 ),
 ( 6, 3, 6 ),
 ( 39.30568950680000029, 56.26183429820000015 ),
 ( 0.000000000000000000, 1.000000000000000000, 2.000000000000000000 ),
 .UNSPECIFIED. ) ;
#74266=CARTESIAN_POINT ( 'NONE',  ( 24.53658740500000235, 1435.634184005399902, 137.4974649685979955 ) ) ;
#74267=( BOUNDED_CURVE ( )  B_SPLINE_CURVE ( 3, ( #20669, #37498, #97400, #54870 ),
 .UNSPECIFIED., .F., .F. ) 
 B_SPLINE_CURVE_WITH_KNOTS ( ( 4, 4 ),
 ( 2.890157662648249914, 3.288561242448070132 ),
 .UNSPECIFIED. ) 
 CURVE ( )  GEOMETRIC_REPRESENTATION_ITEM ( )  RATIONAL_B_SPLINE_CURVE ( ( 1.000000000000000000, 0.9868165636475595415, 0.9868165636475595415, 1.000000000000000000 ) ) 
 REPRESENTATION_ITEM ( '' )  );
#74269=CARTESIAN_POINT ( 'NONE',  ( -4.026786250540000722, 1408.413060387330006, 121.6099336315979969 ) ) ;
#74279=CARTESIAN_POINT ( 'NONE',  ( -23.04246322899999910, 1448.885557893680016, 216.4413416304380178 ) ) ;
#74280=CARTESIAN_POINT ( 'NONE',  ( -20.01144489670000226, 1507.902391332829893, 188.9701987092980175 ) ) ;
#74281=CARTESIAN_POINT ( 'NONE',  ( -11.50373587760000049, 1433.458593519129863, 151.2690138048979804 ) ) ;
#74282=CARTESIAN_POINT ( 'NONE',  ( -4.219439023932549659, 1446.230224804030058, 183.1418048969109975 ) ) ;
#74284=CARTESIAN_POINT ( 'NONE',  ( -27.11119864980000216, 1438.398422475539974, 136.9641100155979814 ) ) ;
#74285=CARTESIAN_POINT ( 'NONE',  ( -24.32490777769999823, 1438.502494616239801, 211.0439858967079942 ) ) ;
#74287=CARTESIAN_POINT ( 'NONE',  ( 1.916752472390000017, 1450.614851703330260, 182.7228952166980207 ) ) ;
#74290=CARTESIAN_POINT ( 'NONE',  ( -1.866069976159590112E-09, 1413.704851968730054, 248.6276318723759857 ) ) ;
#74292=ORIENTED_EDGE ( 'NONE', *, *, #99580, .T. ) ;
#74293=CARTESIAN_POINT ( 'NONE',  ( -11.86352235238380004, 1432.155850026679900, 149.9794201586200018 ) ) ;
#74294=AXIS2_PLACEMENT_3D ( 'NONE', #68219, #102324, #59802 ) ;
#74296=CARTESIAN_POINT ( 'NONE',  ( -4.281468237010000344, 1473.749348323329968, 270.2892484966980078 ) ) ;
#74297=CARTESIAN_POINT ( 'NONE',  ( -1.546949757679999760, 1416.828040475729949, 228.0209010782980101 ) ) ;
#74298=CARTESIAN_POINT ( 'NONE',  ( -8.881784196999999612E-15, 1434.913060387330006, 126.8032249175980155 ) ) ;
#74303=B_SPLINE_SURFACE_WITH_KNOTS ( 'NONE', 5, 5, ( 
 ( #68741, #96689, #70966, #27266, #96122, #42974 ),
 ( #9909, #19396, #87745, #52487, #105081, #36222 ),
 ( #51927, #984, #70407, #35109, #86069, #35661 ),
 ( #36774, #77133, #104526, #17725, #28370, #439 ),
 ( #34560, #45194, #43529, #94446, #102845, #53600 ),
 ( #69292, #86615, #79335, #103396, #2646, #95573 ) ),
 .UNSPECIFIED., .F., .F., .F.,
 ( 6, 6 ),
 ( 6, 6 ),
 ( 30.67014437039999919, 168.1723206030000028 ),
 ( 0.000000000000000000, 2.000000000000000000 ),
 .UNSPECIFIED. ) ;
#74307=CARTESIAN_POINT ( 'NONE',  ( -37.50711329737600153, 1420.224927873189927, 268.4873400273870061 ) ) ;
#74308=ADVANCED_FACE ( 'NONE', ( #85839 ), #8797, .T. ) ;
#74309=ORIENTED_EDGE ( 'NONE', *, *, #18488, .F. ) ;
#74315=CARTESIAN_POINT ( 'NONE',  ( -7.105427357599999217E-15, 1425.413060387329779, 188.2701767054980166 ) ) ;
#74316=CARTESIAN_POINT ( 'NONE',  ( 4.363122647530000009, 1418.913060387330006, 172.2701767054979882 ) ) ;
#74319=CARTESIAN_POINT ( 'NONE',  ( -17.46563763389999835, 1440.441821941650232, 190.8018186351980034 ) ) ;
#74321=CARTESIAN_POINT ( 'NONE',  ( 3.453399489167784608, 1420.336197137674162, 144.1207137702020873 ) ) ;
#74323=CARTESIAN_POINT ( 'NONE',  ( -26.64524886190000075, 1436.744926164489925, 136.7854674159979993 ) ) ;
#74329=CARTESIAN_POINT ( 'NONE',  ( 0.05087731831460000353, 1408.368774904629845, 195.5796676385980106 ) ) ;
#74330=DIRECTION ( 'NONE',  ( -0.4857256630471089576, -0.7475168770206177538, 0.4530884006756178972 ) ) ;
#74331=CARTESIAN_POINT ( 'NONE',  ( -5.077127106479999874, 1398.064300162629934, 197.0820720787980065 ) ) ;
#74335=CARTESIAN_POINT ( 'NONE',  ( -11.87109248081550028, 1432.710597699950085, 149.9814569640180082 ) ) ;
#74336=CARTESIAN_POINT ( 'NONE',  ( 3.777455811129835084, 1425.600239829200063, 185.2244255622378262 ) ) ;
#74339=CARTESIAN_POINT ( 'NONE',  ( -0.6863442344880000823, 1485.336931685030095, 181.8984760979980138 ) ) ;
#74343=CARTESIAN_POINT ( 'NONE',  ( 5.459750082109999347, 1438.302868353570148, 154.7313708644979897 ) ) ;
#74348=EDGE_CURVE ( 'NONE', #45663, #68424, #108187, .T. ) ;
#74351=CARTESIAN_POINT ( 'NONE',  ( -11.01123599387699947, 1428.984116122770047, 91.31161349935790383 ) ) ;
#74352=CARTESIAN_POINT ( 'NONE',  ( -19.59613263891256452, 1457.072187391607486, 225.8973385439780088 ) ) ;
#74353=VERTEX_POINT ( 'NONE', #57085 ) ;
#74355=CARTESIAN_POINT ( 'NONE',  ( 13.02629732915830019, 1434.894639379329874, 149.7937853367240280 ) ) ;
#74356=CARTESIAN_POINT ( 'NONE',  ( 13.57674101270000122, 1415.245980409429876, 197.2205466607979929 ) ) ;
#74358=CARTESIAN_POINT ( 'NONE',  ( 4.500000000000000000, 1448.210448412289907, 182.3842140122979743 ) ) ;
#74362=CARTESIAN_POINT ( 'NONE',  ( 24.33332407789799134, 1445.509459226046147, 214.1965185073686939 ) ) ;
#74363=CARTESIAN_POINT ( 'NONE',  ( 40.26322134699998401, 1439.095365326212459, 135.2291194917982295 ) ) ;
#74364=CARTESIAN_POINT ( 'NONE',  ( 16.57641951891043419, 1409.993768444886882, 226.3203854180307815 ) ) ;
#74366=ORIENTED_EDGE ( 'NONE', *, *, #41982, .F. ) ;
#74368=CARTESIAN_POINT ( 'NONE',  ( -44.93136599389160324, 1440.913052653349951, 269.6838063022050278 ) ) ;
#74369=CARTESIAN_POINT ( 'NONE',  ( 2.077546474020000034, 1420.933967010829974, 184.3471949240980052 ) ) ;
#74373=CARTESIAN_POINT ( 'NONE',  ( -0.05334543264060000178, 1509.045412427330120, 179.1219820337979911 ) ) ;
#74374=LINE ( 'NONE', #65977, #42489 ) ;
#74376=CARTESIAN_POINT ( 'NONE',  ( -2.500000000000000000, 1428.057245272730142, 156.8186834866980064 ) ) ;
#74380=CARTESIAN_POINT ( 'NONE',  ( 35.00939270688730431, 1440.913060385989866, 250.9518149144350332 ) ) ;
#74387=CARTESIAN_POINT ( 'NONE',  ( -19.47602705472021967, 1485.559858681225023, 189.9955089004985780 ) ) ;
#74396=CARTESIAN_POINT ( 'NONE',  ( -14.41709712029999935, 1471.312091222230038, 193.4155243667980244 ) ) ;
#74397=DIRECTION ( 'NONE',  ( 0.000000000000000000, 0.000000000000000000, -1.000000000000000000 ) ) ;
#74401=CARTESIAN_POINT ( 'NONE',  ( -1.287812843440000021, 1452.072817564129991, 183.7203104394979789 ) ) ;
#74407=( BOUNDED_CURVE ( )  B_SPLINE_CURVE ( 3, ( #76007, #100107, #23388, #83853 ),
 .UNSPECIFIED., .F., .T. ) 
 B_SPLINE_CURVE_WITH_KNOTS ( ( 4, 4 ),
 ( 2.890157727407254740, 3.288561306705124920 ),
 .UNSPECIFIED. ) 
 CURVE ( )  GEOMETRIC_REPRESENTATION_ITEM ( )  RATIONAL_B_SPLINE_CURVE ( ( 1.000000000000000000, 0.9868165636806693897, 0.9868165636806693897, 1.000000000000000000 ) ) 
 REPRESENTATION_ITEM ( '' )  );
#74410=CARTESIAN_POINT ( 'NONE',  ( -11.48266949309999951, 1442.832333866149838, 147.8781297902980043 ) ) ;
#74411=CARTESIAN_POINT ( 'NONE',  ( 11.88383461994949997, 1433.642778044820034, 147.6544717983980206 ) ) ;
#74416=CARTESIAN_POINT ( 'NONE',  ( -8.301987938657498844, 1512.913060387330006, 185.0111222839169898 ) ) ;
#74417=CARTESIAN_POINT ( 'NONE',  ( 18.52259402964000046, 1425.591791501662101, 225.5512587368259858 ) ) ;
#74420=CARTESIAN_POINT ( 'NONE',  ( 11.76966145709999978, 1432.350018154600093, 150.8118972717979887 ) ) ;
#74421=CARTESIAN_POINT ( 'NONE',  ( -4.161605034536901115, 1448.982995605119868, 185.0801909513209864 ) ) ;
#74424=CARTESIAN_POINT ( 'NONE',  ( 3.677837710089999800E-15, 1426.566393376330097, 144.1938086916980239 ) ) ;
#74425=CARTESIAN_POINT ( 'NONE',  ( 18.16363651209229957, 1457.500868343169941, 229.3031588784930079 ) ) ;
#74426=CARTESIAN_POINT ( 'NONE',  ( -12.17235240719999823, 1434.042297368109985, 149.7137827380979900 ) ) ;
#74427=CARTESIAN_POINT ( 'NONE',  ( 1.477069687100340089E-10, 1465.967699521269878, 241.3588474068609742 ) ) ;
#74429=CARTESIAN_POINT ( 'NONE',  ( -20.53900256050109618, 1505.889087235659872, 190.4466324654250116 ) ) ;
#74432=CARTESIAN_POINT ( 'NONE',  ( -0.9046723551649999973, 1484.832931805229919, 182.0120543415980023 ) ) ;
#74434=CARTESIAN_POINT ( 'NONE',  ( -45.63701710503070075, 1440.701692410139913, 268.9748479612790106 ) ) ;
#74435=CARTESIAN_POINT ( 'NONE',  ( -21.29751270369999716, 1429.161938467929986, 221.7940764617979994 ) ) ;
#74436=CARTESIAN_POINT ( 'NONE',  ( -20.13089310500000195, 1488.371301023830028, 192.3463370429979875 ) ) ;
#74438=CARTESIAN_POINT ( 'NONE',  ( 2.867497623927549810, 1409.013195610850062, 223.6255212523830096 ) ) ;
#74440=CARTESIAN_POINT ( 'NONE',  ( 5.973824899667066646, 1425.157018348714246, 226.5484819897127124 ) ) ;
#74444=EDGE_CURVE ( 'NONE', #105289, #22747, #42755, .T. ) ;
#74445=CARTESIAN_POINT ( 'NONE',  ( 4.804950790719999532, 1416.130848190230154, 240.4142139981979938 ) ) ;
#74446=CARTESIAN_POINT ( 'NONE',  ( -0.5624690339869999889, 1416.828040475229955, 227.7677324846980014 ) ) ;
#74447=CARTESIAN_POINT ( 'NONE',  ( -2.498001343329999901, 1464.114461778829991, 182.6719732163979870 ) ) ;
#74448=DIRECTION ( 'NONE',  ( 0.000000000000000000, -1.000000000000000000, 0.000000000000000000 ) ) ;
#74449=CARTESIAN_POINT ( 'NONE',  ( 14.45783227242900004, 1416.839692127189892, 196.8516148535319985 ) ) ;
#74450=CARTESIAN_POINT ( 'NONE',  ( -9.545816653860001111, 1416.905270227430037, 240.4008508676979829 ) ) ;
#74451=DIRECTION ( 'NONE',  ( 0.03489949670250479252, 0.9993908270190956511, 0.000000000000000000 ) ) ;
#74453=CARTESIAN_POINT ( 'NONE',  ( -21.97965021947160125, 1452.145514088490017, 140.5363500159340049 ) ) ;
#74454=CARTESIAN_POINT ( 'NONE',  ( -18.90776592919999644, 1416.839648759230158, 208.2177104760110069 ) ) ;
#74458=CARTESIAN_POINT ( 'NONE',  ( 16.39875021229349983, 1422.270930245990030, 227.2883076116929999 ) ) ;
#74463=CARTESIAN_POINT ( 'NONE',  ( -22.67876275168039868, 1409.704989955349902, 209.2849217834479987 ) ) ;
#74466=CARTESIAN_POINT ( 'NONE',  ( 6.536123391264514026, 1446.776743555406711, 154.4253092722253200 ) ) ;
#74467=CARTESIAN_POINT ( 'NONE',  ( -5.850656168700000492, 1507.636149491230071, 236.0722295150979733 ) ) ;
#74469=AXIS2_PLACEMENT_3D ( 'NONE', #99356, #72537, #47324 ) ;
#74471=CARTESIAN_POINT ( 'NONE',  ( 43.38413226852659932, 1452.743835328579962, 268.5823572257330056 ) ) ;
#74475=EDGE_CURVE ( 'NONE', #2114, #99633, #46738, .T. ) ;
#74478=CARTESIAN_POINT ( 'NONE',  ( 0.1955981723673640149, 1414.913060387329779, 225.1861338915940109 ) ) ;
#74479=CARTESIAN_POINT ( 'NONE',  ( 12.82354616867442054, 1442.855160287932449, 186.8966734488652435 ) ) ;
#74482=CARTESIAN_POINT ( 'NONE',  ( 26.83593419056240137, 1450.879312558440006, 136.4219504817619963 ) ) ;
#74484=CARTESIAN_POINT ( 'NONE',  ( 1.863634235144320028, 1452.847980845800066, 152.4700529009420222 ) ) ;
#74486=CARTESIAN_POINT ( 'NONE',  ( 17.22271612299999788, 1410.011821425830249, 192.5801709317979942 ) ) ;
#74489=CARTESIAN_POINT ( 'NONE',  ( 0.03683352690712138333, 1409.764797560680563, 233.0950034937904150 ) ) ;
#74490=CARTESIAN_POINT ( 'NONE',  ( -13.32966728119899891, 1434.904994951539948, 148.9243255523419975 ) ) ;
#74496=CARTESIAN_POINT ( 'NONE',  ( 14.35418281379999961, 1430.829918313929966, 214.3676144195279676 ) ) ;
#74497=DIRECTION ( 'NONE',  ( -0.7067692896845355621, 0.03085827994953252440, -0.7067707815956835171 ) ) ;
#74504=CARTESIAN_POINT ( 'NONE',  ( 4.714294778569999749E-15, 1435.943783413959864, 150.5249316333980119 ) ) ;
#74506=CARTESIAN_POINT ( 'NONE',  ( -12.78723757166081754, 1416.835806642020316, 195.5393902064313636 ) ) ;
#74507=CARTESIAN_POINT ( 'NONE',  ( 11.07527106835961916, 1414.913060387329779, 220.8418235494980877 ) ) ;
#74512=CARTESIAN_POINT ( 'NONE',  ( 13.40512367049999831, 1419.762041482030099, 228.7767913457980171 ) ) ;
#74513=CARTESIAN_POINT ( 'NONE',  ( -18.39408727770000240, 1486.478860455830045, 188.6611279849980178 ) ) ;
#74515=CARTESIAN_POINT ( 'NONE',  ( -16.64778341059999889, 1409.494413794329830, 224.2640771540980040 ) ) ;
#74519=CARTESIAN_POINT ( 'NONE',  ( 6.536538287287070992E-07, 1407.436810216500135, 196.0562222547989961 ) ) ;
#74522=CARTESIAN_POINT ( 'NONE',  ( -1.075903594600000179, 1414.913060387329779, 226.3952325314980101 ) ) ;
#74523=CARTESIAN_POINT ( 'NONE',  ( 0.1945320816990730173, 1466.113474688809902, 182.6906957989669991 ) ) ;
#74524=CARTESIAN_POINT ( 'NONE',  ( -0.1955981723043500320, 1414.913060387329779, 193.0575580317509718 ) ) ;
#74526=CARTESIAN_POINT ( 'NONE',  ( -27.73483395940000307, 1444.994950788470987, 161.2078980334979690 ) ) ;
#74527=CARTESIAN_POINT ( 'NONE',  ( -28.07727371017839957, 1509.147381901259905, 210.7551250638759655 ) ) ;
#74528=CARTESIAN_POINT ( 'NONE',  ( 13.50082440470000122, 1434.968962347899833, 149.4780432086979829 ) ) ;
#74529=CARTESIAN_POINT ( 'NONE',  ( -41.59656558017320549, 1442.666623283399986, 134.0999999980969903 ) ) ;
#74531=ORIENTED_EDGE ( 'NONE', *, *, #48928, .F. ) ;
#74537=CARTESIAN_POINT ( 'NONE',  ( 40.48954223343692860, 1425.136313467639638, 269.1159157282953061 ) ) ;
#74538=CARTESIAN_POINT ( 'NONE',  ( 21.84849975889999740, 1489.480617680729893, 209.7146558588220273 ) ) ;
#74540=CARTESIAN_POINT ( 'NONE',  ( 2.500000001190000098, 1425.952486855329880, 183.8951078798980063 ) ) ;
#74543=CARTESIAN_POINT ( 'NONE',  ( -24.83643123910302464, 1443.481921562399293, 210.6071950037623708 ) ) ;
#74544=ORIENTED_EDGE ( 'NONE', *, *, #15352, .F. ) ;
#74546=CARTESIAN_POINT ( 'NONE',  ( -15.99166196625810166, 1409.471479983660174, 225.2129078530250013 ) ) ;
#74551=CARTESIAN_POINT ( 'NONE',  ( 23.45884178989999924, 1509.732261194629928, 225.1742078074979929 ) ) ;
#74554=CARTESIAN_POINT ( 'NONE',  ( 0.6844602914180001330, 1466.314900821229912, 235.5924101916979794 ) ) ;
#74555=CARTESIAN_POINT ( 'NONE',  ( 16.87240681180000124, 1409.502257816329802, 222.1138738933979937 ) ) ;
#74556=CARTESIAN_POINT ( 'NONE',  ( -2.423460974664930045, 1412.654287068640087, 186.3965991398220012 ) ) ;
#74557=CARTESIAN_POINT ( 'NONE',  ( -16.87496977620000038, 1423.389150575329950, 227.5705651359979811 ) ) ;
#74561=CARTESIAN_POINT ( 'NONE',  ( -4.440892098499999806E-15, 1519.913060387329779, 231.7062449670980300 ) ) ;
#74564=CARTESIAN_POINT ( 'NONE',  ( -8.375290140818398399, 1485.147173385050110, 184.2408640538430120 ) ) ;
#74566=CARTESIAN_POINT ( 'NONE',  ( -1.572308128563102869, 1420.974599004695847, 183.2802011453454440 ) ) ;
#74571=EDGE_LOOP ( 'NONE', ( #38898, #59997, #49503, #51837, #48551 ) ) ;
#74573=CARTESIAN_POINT ( 'NONE',  ( -22.14275666580000035, 1410.906117103929773, 202.5124468041880164 ) ) ;
#74575=CARTESIAN_POINT ( 'NONE',  ( -10.82013115906650036, 1424.918091613318893, 144.4803130008261007 ) ) ;
#74576=CARTESIAN_POINT ( 'NONE',  ( 15.94649789270860119, 1409.495428613550075, 192.6881838021419924 ) ) ;
#74578=CARTESIAN_POINT ( 'NONE',  ( 39.00001286119130128, 1437.776791841900149, 135.9885178820470060 ) ) ;
#74581=CARTESIAN_POINT ( 'NONE',  ( 11.49474869997571247, 1464.050871868342483, 231.7668017734373791 ) ) ;
#74584=CARTESIAN_POINT ( 'NONE',  ( 34.34692909021160290, 1451.701922534439973, 134.0999999981429767 ) ) ;
#74588=CARTESIAN_POINT ( 'NONE',  ( -18.72407806909999906, 1458.246133455830204, 227.3156640602979905 ) ) ;
#74592=CARTESIAN_POINT ( 'NONE',  ( -2.938318217019999956, 1419.338735643829978, 183.9627234138980043 ) ) ;
#74594=CARTESIAN_POINT ( 'NONE',  ( -3.240679945760000180, 1484.702199250929880, 183.3401715852980089 ) ) ;
#74595=CARTESIAN_POINT ( 'NONE',  ( -2.500000000000079936, 1439.283173988879980, 159.9470331267719985 ) ) ;
#74599=CARTESIAN_POINT ( 'NONE',  ( 38.81202644819820335, 1450.612734570869861, 134.4205495056820041 ) ) ;
#74602=CARTESIAN_POINT ( 'NONE',  ( 33.05507863147482794, 1442.773887286371291, 154.3538505727091206 ) ) ;
#74609=CARTESIAN_POINT ( 'NONE',  ( 36.18824964826809776, 1440.913060387330006, 262.5531867102749857 ) ) ;
#74610=CARTESIAN_POINT ( 'NONE',  ( -0.0007986355180737672761, 1451.919156408470826, 154.0006015666134260 ) ) ;
#74612=CARTESIAN_POINT ( 'NONE',  ( -14.15566883900000050, 1416.254459047329874, 221.6674824254980081 ) ) ;
#74616=CARTESIAN_POINT ( 'NONE',  ( -12.51099981740000011, 1416.825784017230035, 222.1450729860980005 ) ) ;
#74619=CARTESIAN_POINT ( 'NONE',  ( -12.40443716549999920, 1434.419911639550037, 147.1503489169979844 ) ) ;
#74622=CARTESIAN_POINT ( 'NONE',  ( 12.66475911230000051, 1461.490340252930082, 232.8294749871980116 ) ) ;
#74623=CARTESIAN_POINT ( 'NONE',  ( 2.531940903048510086E-08, 1457.850589566970029, 229.0733431205499926 ) ) ;
#74627=CARTESIAN_POINT ( 'NONE',  ( -22.63977338456492916, 1409.703622513127584, 209.3606416856607382 ) ) ;
#74628=CARTESIAN_POINT ( 'NONE',  ( -0.1451720414164340001, 1507.596876506829858, 180.8216655926840133 ) ) ;
#74631=CARTESIAN_POINT ( 'NONE',  ( 18.52542017129999863, 1508.846193922329803, 188.2533944517980160 ) ) ;
#74634=ORIENTED_EDGE ( 'NONE', *, *, #97902, .T. ) ;
#74637=CARTESIAN_POINT ( 'NONE',  ( -10.96338982440000009, 1431.906653981850013, 151.7581583521979951 ) ) ;
#74642=B_SPLINE_CURVE_WITH_KNOTS ( 'NONE', 5,
 ( #87786, #53079, #69892, #1570, #19443, #96731 ),
 .UNSPECIFIED., .F., .F.,
 ( 6, 6 ),
 ( -7.104449043337727865, 0.000000000000000000 ),
 .UNSPECIFIED. ) ;
#74643=CARTESIAN_POINT ( 'NONE',  ( 12.98218568629999936, 1444.905773837279867, 186.8780337078979983 ) ) ;
#74644=CARTESIAN_POINT ( 'NONE',  ( -19.99968608059999653, 1495.374354163629960, 228.2163264703980019 ) ) ;
#74645=CARTESIAN_POINT ( 'NONE',  ( -10.73514660619479955, 1424.973046414658938, 139.1354236203746098 ) ) ;
#74650=CARTESIAN_POINT ( 'NONE',  ( 14.64031841569999948, 1407.520860949229927, 268.3932868650979913 ) ) ;
#74651=CARTESIAN_POINT ( 'NONE',  ( 0.1416802514830000082, 1408.918007970730059, 186.4630591869979810 ) ) ;
#74654=CARTESIAN_POINT ( 'NONE',  ( 24.64646478266137208, 1440.604980622881385, 212.4694330774556192 ) ) ;
#74657=CARTESIAN_POINT ( 'NONE',  ( 12.78690713350000152, 1416.828040475229955, 222.7042044314979989 ) ) ;
#74660=CARTESIAN_POINT ( 'NONE',  ( -2.314829430188050097, 1449.816261314480016, 155.0640873339540065 ) ) ;
#74661=CARTESIAN_POINT ( 'NONE',  ( -1.639149609193548240, 1450.659151795366597, 183.2023271470939960 ) ) ;
#74663=CARTESIAN_POINT ( 'NONE',  ( -19.76130828083433855, 1485.974801659758896, 190.2327744154961522 ) ) ;
#74664=EDGE_CURVE ( 'NONE', #24304, #66906, #81517, .T. ) ;
#74665=CARTESIAN_POINT ( 'NONE',  ( -14.43002663333860092, 1416.512142030599989, 221.3633489337159688 ) ) ;
#74667=CARTESIAN_POINT ( 'NONE',  ( -14.35418281399999962, 1430.829918314029783, 214.3676144200779845 ) ) ;
#74668=VECTOR ( 'NONE', #100382, 1000.000000000000114 ) ;
#74669=DIRECTION ( 'NONE',  ( -0.000000000000000000, 1.000000000000000000, -0.000000000000000000 ) ) ;
#74670=CARTESIAN_POINT ( 'NONE',  ( 2.704557286920000081, 1440.782450355879973, 168.7248561158979783 ) ) ;
#74671=CARTESIAN_POINT ( 'NONE',  ( -4.970712357689999195, 1475.638404632529955, 266.9514863814980004 ) ) ;
#74672=CARTESIAN_POINT ( 'NONE',  ( -11.28910848134292699, 1425.472454366105467, 139.1360123033548462 ) ) ;
#74673=CARTESIAN_POINT ( 'NONE',  ( -19.45107472759999823, 1470.650217123529956, 191.6852195815980053 ) ) ;
#74674=CARTESIAN_POINT ( 'NONE',  ( -11.88019884917019553, 1486.509635274632274, 184.3263142426127388 ) ) ;
#74677=AXIS2_PLACEMENT_3D ( 'NONE', #20270, #54471, #105961 ) ;
#74681=CARTESIAN_POINT ( 'NONE',  ( 24.04921872038306674, 1508.500196458096980, 195.9136755597566264 ) ) ;
#74682=CARTESIAN_POINT ( 'NONE',  ( -1.009090409386799836, 1395.948298600919998, 220.0848352038350129 ) ) ;
#74684=CARTESIAN_POINT ( 'NONE',  ( -15.81341253836600025, 1421.037553285879994, 227.0412314586560001 ) ) ;
#74687=CARTESIAN_POINT ( 'NONE',  ( -7.497914047782630931, 1410.547968552112707, 230.8512428201019020 ) ) ;
#74690=CARTESIAN_POINT ( 'NONE',  ( -2.370970874524634286, 1427.002265528474027, 134.0999999980980135 ) ) ;
#74691=DIRECTION ( 'NONE',  ( -0.7071067811865475727, 0.000000000000000000, 0.7071067811865475727 ) ) ;
#74694=EDGE_CURVE ( 'NONE', #107294, #48829, #12763, .T. ) ;
#74703=CARTESIAN_POINT ( 'NONE',  ( 20.61223612676809935, 1508.367027694390117, 227.7934906704109892 ) ) ;
#74707=CARTESIAN_POINT ( 'NONE',  ( 11.37512727334929963, 1434.390363725699899, 151.4928147334219943 ) ) ;
#74708=CARTESIAN_POINT ( 'NONE',  ( -11.59628660009999912, 1396.377029133129781, 211.2534838439580085 ) ) ;
#74709=CARTESIAN_POINT ( 'NONE',  ( -19.55811020839999870, 1410.091525468729742, 221.3856977114979827 ) ) ;
#74710=ORIENTED_EDGE ( 'NONE', *, *, #4362, .F. ) ;
#74711=CARTESIAN_POINT ( 'NONE',  ( -13.50123011842539711, 1444.098455846193701, 169.3544814583405582 ) ) ;
#74712=CARTESIAN_POINT ( 'NONE',  ( 22.41814969565213289, 1509.697587479513004, 228.1798637225821551 ) ) ;
#74714=CARTESIAN_POINT ( 'NONE',  ( 1.581901184577762853, 1426.946688134061105, 134.0999999980979851 ) ) ;
#74715=CARTESIAN_POINT ( 'NONE',  ( -13.87674170834680076, 1508.783404247360068, 183.8810751069530056 ) ) ;
#74716=CARTESIAN_POINT ( 'NONE',  ( 0.8724072853540000283, 1429.775567651030087, 184.3285425289979855 ) ) ;
#74719=CARTESIAN_POINT ( 'NONE',  ( 9.572892907575269561, 1396.247353193519984, 203.5817440233749949 ) ) ;
#74720=CARTESIAN_POINT ( 'NONE',  ( 1.396725214909999790, 1415.041103191630100, 191.5122427437979979 ) ) ;
#74721=CARTESIAN_POINT ( 'NONE',  ( 10.89169420240000008, 1427.021371490929823, 149.7235597410980006 ) ) ;
#74722=CARTESIAN_POINT ( 'NONE',  ( 7.812244556781691607, 1509.186435478737394, 180.8337954617522882 ) ) ;
#74724=CARTESIAN_POINT ( 'NONE',  ( 13.07453333027640063, 1436.035540400220043, 150.7116512640230042 ) ) ;
#74725=EDGE_LOOP ( 'NONE', ( #58811, #26887, #69490, #4487 ) ) ;
#74726=ORIENTED_EDGE ( 'NONE', *, *, #14548, .F. ) ;
#74727=LINE ( 'NONE', #107760, #21549 ) ;
#74728=CARTESIAN_POINT ( 'NONE',  ( -9.055072417550000807, 1464.016001224229967, 233.0040833371979829 ) ) ;
#74738=VERTEX_POINT ( 'NONE', #56394 ) ;
#74740=CARTESIAN_POINT ( 'NONE',  ( -21.21436197740000296, 1509.702916646330095, 230.0075723124979845 ) ) ;
#74741=CARTESIAN_POINT ( 'NONE',  ( -38.96076896855542770, 1429.469642160400554, 269.5922795220489547 ) ) ;
#74744=CARTESIAN_POINT ( 'NONE',  ( 24.60632198259999726, 1440.982726376320215, 212.6699524588079839 ) ) ;
#74745=CARTESIAN_POINT ( 'NONE',  ( -29.31706666688599938, 1440.913060386920051, 236.0794183928230154 ) ) ;
#74749=EDGE_CURVE ( 'NONE', #41855, #39980, #6643, .T. ) ;
#74751=CARTESIAN_POINT ( 'NONE',  ( 5.165173145674029520, 1410.469967527520112, 269.6177701542679870 ) ) ;
#74753=CARTESIAN_POINT ( 'NONE',  ( 23.73237516220000032, 1410.130224032329807, 209.2990132785999720 ) ) ;
#74754=CARTESIAN_POINT ( 'NONE',  ( -20.01700974779999953, 1508.374998501830078, 188.9474888133980244 ) ) ;
#74756=AXIS2_PLACEMENT_3D ( 'NONE', #20293, #72387, #106516 ) ;
#74760=CARTESIAN_POINT ( 'NONE',  ( 0.2920509773060000480, 1419.245382216430016, 184.6471073958980185 ) ) ;
#74761=CARTESIAN_POINT ( 'NONE',  ( 3.921275451871176987, 1421.968795751384505, 139.1411894380421472 ) ) ;
#74765=ADVANCED_FACE ( 'NONE', ( #85419 ), #8166, .T. ) ;
#74766=CARTESIAN_POINT ( 'NONE',  ( 45.67186675490000169, 1440.913060379579974, 266.1886920260980105 ) ) ;
#74768=CARTESIAN_POINT ( 'NONE',  ( -16.98603957050000091, 1470.451033259130099, 228.5667712960980111 ) ) ;
#74774=CARTESIAN_POINT ( 'NONE',  ( -25.87869575008628686, 1450.783544060030181, 136.8232913390557144 ) ) ;
#74775=CARTESIAN_POINT ( 'NONE',  ( 10.10004869885234058, 1422.222932908421171, 137.0999999980978430 ) ) ;
#74777=ORIENTED_EDGE ( 'NONE', *, *, #54196, .T. ) ;
#74782=CARTESIAN_POINT ( 'NONE',  ( 21.16233094960000116, 1454.406918326630148, 221.8286195809980086 ) ) ;
#74784=CARTESIAN_POINT ( 'NONE',  ( -5.441602405930001218, 1420.475810304129936, 186.6133007815980136 ) ) ;
#74786=CARTESIAN_POINT ( 'NONE',  ( 3.851527341300000185, 1440.290862272119966, 184.6363558007980146 ) ) ;
#74788=CARTESIAN_POINT ( 'NONE',  ( 40.02436149072349991, 1445.627823825280075, 136.8606774784030051 ) ) ;
#74789=CARTESIAN_POINT ( 'NONE',  ( -20.08934789279999933, 1426.987235077529931, 222.3577178168980026 ) ) ;
#74792=CARTESIAN_POINT ( 'NONE',  ( 15.36922853749999973, 1507.577586422630020, 186.8522449740979994 ) ) ;
#74794=CARTESIAN_POINT ( 'NONE',  ( -30.89477149620823937, 1461.567857698084026, 269.4805871490156619 ) ) ;
#74796=CARTESIAN_POINT ( 'NONE',  ( 0.8141018274779999730, 1430.453334911130241, 150.3332009510979788 ) ) ;
#74797=CARTESIAN_POINT ( 'NONE',  ( -42.05335041385732353, 1427.628721445028987, 269.0743441695974525 ) ) ;
#74802=CARTESIAN_POINT ( 'NONE',  ( -0.01334073050390000015, 1417.281753868929854, 234.8503427052979760 ) ) ;
#74803=CARTESIAN_POINT ( 'NONE',  ( -13.09006439999744309, 1443.016537806267934, 186.6523555623594177 ) ) ;
#74807=CARTESIAN_POINT ( 'NONE',  ( -1.160519492789278573, 1415.499451156714713, 233.2391781844445404 ) ) ;
#74810=CARTESIAN_POINT ( 'NONE',  ( -12.90463020832708452, 1442.893833669162404, 169.4357342695923592 ) ) ;
#74811=CARTESIAN_POINT ( 'NONE',  ( -15.05358279999999915, 1410.831827720429828, 226.7261506157979909 ) ) ;
#74812=VERTEX_POINT ( 'NONE', #83236 ) ;
#74813=CARTESIAN_POINT ( 'NONE',  ( 0.6611933174841589933, 1415.434635989099888, 191.1758574623620177 ) ) ;
#74814=CARTESIAN_POINT ( 'NONE',  ( 21.93662947122204443, 1509.528752753375102, 226.8343663891151323 ) ) ;
#74815=VERTEX_POINT ( 'NONE', #40679 ) ;
#74816=ORIENTED_EDGE ( 'NONE', *, *, #89132, .T. ) ;
#74817=CARTESIAN_POINT ( 'NONE',  ( 17.06443472855709942, 1415.088506334920112, 209.4325226847720103 ) ) ;
#74818=CARTESIAN_POINT ( 'NONE',  ( 13.19315069080000136, 1509.373775394329869, 234.6191799994980158 ) ) ;
#74820=CARTESIAN_POINT ( 'NONE',  ( -24.34117855639999917, 1445.812453778969939, 216.4489897547180135 ) ) ;
#74824=CARTESIAN_POINT ( 'NONE',  ( -11.64622956740000070, 1433.292780563709812, 151.0149266372979753 ) ) ;
#74826=CARTESIAN_POINT ( 'NONE',  ( 24.08426297012860218, 1411.115209414830133, 209.6325633951909708 ) ) ;
#74828=CARTESIAN_POINT ( 'NONE',  ( -25.87016399559999869, 1438.590621495679898, 137.3979509201980136 ) ) ;
#74829=CARTESIAN_POINT ( 'NONE',  ( -24.36309863860000391, 1438.807150111159899, 211.0250922072579840 ) ) ;
#74832=CARTESIAN_POINT ( 'NONE',  ( 2.380479430399999874, 1449.688732974869936, 182.4840047008979980 ) ) ;
#74834=CARTESIAN_POINT ( 'NONE',  ( -29.86499995759902859, 1510.066214768678947, 213.4342127740283388 ) ) ;
#74835=CARTESIAN_POINT ( 'NONE',  ( -2.638813393498400254E-09, 1414.425016002700204, 246.3383374633879725 ) ) ;
#74838=CARTESIAN_POINT ( 'NONE',  ( -11.77304318683200002, 1427.201803926489902, 146.6198829697760004 ) ) ;
#74841=CARTESIAN_POINT ( 'NONE',  ( -4.986174233689999902, 1473.385195802330145, 270.3887730020979916 ) ) ;
#74851=CARTESIAN_POINT ( 'NONE',  ( -43.87218737955609527, 1429.907377119439843, 267.0500106768220121 ) ) ;
#74854=B_SPLINE_CURVE_WITH_KNOTS ( 'NONE', 3,
 ( #56016, #73366, #56567, #64431, #99088, #90140, #22925, #72820, #73920, #66085 ),
 .UNSPECIFIED., .F., .F.,
 ( 4, 2, 2, 2, 4 ),
 ( 0.000000000000000000, 0.2500000000000000000, 0.5000000000000000000, 0.7500000000000000000, 1.000000000000000000 ),
 .UNSPECIFIED. ) ;
#74855=VERTEX_POINT ( 'NONE', #9833 ) ;
#74856=EDGE_LOOP ( 'NONE', ( #24849, #99632, #87060, #61930 ) ) ;
#74858=CARTESIAN_POINT ( 'NONE',  ( 4.687027516810611694, 1423.666285210286560, 183.9319128431047261 ) ) ;
#74862=CARTESIAN_POINT ( 'NONE',  ( -2.370970874524632510, 1427.002265528473799, 137.0999999980979851 ) ) ;
#74863=CARTESIAN_POINT ( 'NONE',  ( -15.12939613400000027, 1455.450849537030081, 188.6308199800980105 ) ) ;
#74866=CARTESIAN_POINT ( 'NONE',  ( -26.81148555899999764, 1435.638120290539973, 136.0770497519980040 ) ) ;
#74868=CARTESIAN_POINT ( 'NONE',  ( -41.57727730138044109, 1445.035122391737787, 135.5177457120996110 ) ) ;
#74870=CARTESIAN_POINT ( 'NONE',  ( -42.72426141366479868, 1430.577730169959978, 270.2287312818410214 ) ) ;
#74872=CARTESIAN_POINT ( 'NONE',  ( -2.228622948780000446, 1395.990885615630077, 198.2489192474980086 ) ) ;
#74873=CARTESIAN_POINT ( 'NONE',  ( -38.60856581307790236, 1443.613625294319945, 137.1750438966080026 ) ) ;
#74876=CARTESIAN_POINT ( 'NONE',  ( 0.3174014934009999900, 1451.682253938030044, 183.0610148633980145 ) ) ;
#74880=CARTESIAN_POINT ( 'NONE',  ( -25.03982234340000090, 1436.292317311149873, 137.6710093398980064 ) ) ;
#74881=CARTESIAN_POINT ( 'NONE',  ( -24.66797713489999921, 1441.969358036629956, 210.7253539414180068 ) ) ;
#74885=CARTESIAN_POINT ( 'NONE',  ( -2.355747397201679583, 1484.256314648310081, 183.1724393876219779 ) ) ;
#74887=CARTESIAN_POINT ( 'NONE',  ( 3.751161017837588041, 1440.869524849231766, 156.4631710623298204 ) ) ;
#74889=ORIENTED_EDGE ( 'NONE', *, *, #12469, .F. ) ;
#74896=CARTESIAN_POINT ( 'NONE',  ( 12.88043371926620040, 1435.836274709469990, 150.7661302149069797 ) ) ;
#74898=CARTESIAN_POINT ( 'NONE',  ( 13.36059434040000049, 1414.988017874730076, 197.8813517676980211 ) ) ;
#74899=CARTESIAN_POINT ( 'NONE',  ( 15.68481150160000048, 1430.205911231830214, 190.9194062192979970 ) ) ;
#74900=CARTESIAN_POINT ( 'NONE',  ( 23.84533589473599946, 1452.080362908450070, 136.9869410992479857 ) ) ;
#74902=CARTESIAN_POINT ( 'NONE',  ( 3.545671383367217100, 1450.748354634506541, 184.0780438961519678 ) ) ;
#74905=CARTESIAN_POINT ( 'NONE',  ( 24.55734822141088003, 1443.697998701720280, 213.2430772723361372 ) ) ;
#74907=STYLED_ITEM ( 'NONE', ( #82809 ), #45166 ) ;
#74908=CARTESIAN_POINT ( 'NONE',  ( -1.731498172528467938, 1450.471748407974928, 182.5592355860798648 ) ) ;
#74913=AXIS2_PLACEMENT_3D ( 'NONE', #36383, #70571, #27984 ) ;
#74914=CARTESIAN_POINT ( 'NONE',  ( 2.378562897450000158, 1421.262547136429930, 183.2548472359979996 ) ) ;
#74917=CARTESIAN_POINT ( 'NONE',  ( -11072.05219665070763, 50.13405481564041821, -8413.031381324366521 ) ) ;
#74920=CARTESIAN_POINT ( 'NONE',  ( 18.72518989680000345, 1416.274718422629803, 209.8658817986590179 ) ) ;
#74923=CARTESIAN_POINT ( 'NONE',  ( -9.429479337035831822E-07, 1408.510422154009802, 222.8906800396250105 ) ) ;
#74924=CARTESIAN_POINT ( 'NONE',  ( 38.81943119499100447, 1440.913060376880139, 257.5592801587829968 ) ) ;
#74929=ADVANCED_FACE ( 'NONE', ( #60824 ), #53607, .T. ) ;
#74930=ORIENTED_EDGE ( 'NONE', *, *, #81221, .F. ) ;
#74932=ADVANCED_FACE ( 'NONE', ( #42897 ), #27195, .F. ) ;
#74933=CARTESIAN_POINT ( 'NONE',  ( -19.67949054060972003, 1485.238787255277430, 190.3370324724980662 ) ) ;
#74935=CARTESIAN_POINT ( 'NONE',  ( -0.5620977654635980203, 1416.851343899799986, 227.7685710128770040 ) ) ;
#74936=CARTESIAN_POINT ( 'NONE',  ( 1.747240526076377476, 1508.468491276751138, 237.2463171574812293 ) ) ;
#74937=CARTESIAN_POINT ( 'NONE',  ( 26.95974481528090649, 1509.967011703660091, 222.3600134204636163 ) ) ;
#74944=CARTESIAN_POINT ( 'NONE',  ( 5.360248604747719803, 1422.242465614079947, 144.1680528682020110 ) ) ;
#74953=VERTEX_POINT ( 'NONE', #87096 ) ;
#74955=CARTESIAN_POINT ( 'NONE',  ( 35.78517889623469728, 1437.356590274589962, 136.5362015133650004 ) ) ;
#74957=CARTESIAN_POINT ( 'NONE',  ( 1.137831829869999867, 1408.952794351630018, 231.4765879240979984 ) ) ;
#74958=ADVANCED_FACE ( 'NONE', ( #906 ), #79522, .F. ) ;
#74963=CARTESIAN_POINT ( 'NONE',  ( 10.09968471107369936, 1409.265749149070189, 198.0954670411109930 ) ) ;
#74964=CARTESIAN_POINT ( 'NONE',  ( 18.03149116639599825, 1424.668758022952034, 225.2946740050300036 ) ) ;
#74968=CARTESIAN_POINT ( 'NONE',  ( -2.500000000000000000, 1439.447167954220049, 162.2860246256229857 ) ) ;
#74970=CARTESIAN_POINT ( 'NONE',  ( -2.497948021501850135, 1449.239010218830117, 183.3628261147359808 ) ) ;
#74971=ORIENTED_EDGE ( 'NONE', *, *, #83036, .F. ) ;
#74972=EDGE_CURVE ( 'NONE', #60117, #59101, #72516, .T. ) ;
#74973=CARTESIAN_POINT ( 'NONE',  ( 3.946018174590000300E-15, 1427.166763959530044, 147.9649995502979891 ) ) ;
#74974=CARTESIAN_POINT ( 'NONE',  ( -5.510229795562198163, 1427.334330648820014, 134.0999999980980135 ) ) ;
#74975=CARTESIAN_POINT ( 'NONE',  ( -12.84242185500000133, 1435.935690871960105, 150.8114634387980004 ) ) ;
#74981=CARTESIAN_POINT ( 'NONE',  ( -1.213587419969999859, 1484.841083681130158, 182.2078730101980000 ) ) ;
#74987=CARTESIAN_POINT ( 'NONE',  ( 4.305761763093079786, 1409.063420901319887, 223.2590317760309802 ) ) ;
#74988=CARTESIAN_POINT ( 'NONE',  ( -1.887379141860000057E-14, 1421.846726402829972, 101.6565998076979866 ) ) ;
#74991=ORIENTED_EDGE ( 'NONE', *, *, #26521, .F. ) ;
#74993=CARTESIAN_POINT ( 'NONE',  ( 25.42954073489999800, 1428.064052004430096, 238.1443969920979953 ) ) ;
#74994=CARTESIAN_POINT ( 'NONE',  ( -2.469785781769999744, 1452.697316747630111, 183.1533515108980055 ) ) ;
#74998=CARTESIAN_POINT ( 'NONE',  ( 0.5000000000000000000, 1448.894380913990062, 169.0327022760979787 ) ) ;
#74999=CARTESIAN_POINT ( 'NONE',  ( -14.69392519634950034, 1452.399937212599980, 148.0737491589720207 ) ) ;
#75000=CARTESIAN_POINT ( 'NONE',  ( -18.95862648649999826, 1416.832348283729971, 207.7798716402180048 ) ) ;
#75001=VERTEX_POINT ( 'NONE', #107204 ) ;
#75002=CARTESIAN_POINT ( 'NONE',  ( -2.500000000000000000, 1419.382839489710022, 144.1073622044459910 ) ) ;
#75004=CARTESIAN_POINT ( 'NONE',  ( 16.26552582369990319, 1422.904278802180215, 227.8875789372550003 ) ) ;
#75009=CARTESIAN_POINT ( 'NONE',  ( -22.93094644840109808, 1409.723536851819972, 208.9950183821200085 ) ) ;
#75010=CARTESIAN_POINT ( 'NONE',  ( -3.826489878020000290, 1424.302205092830036, 185.3920305880980095 ) ) ;
#75013=CARTESIAN_POINT ( 'NONE',  ( -10.00550473600000068, 1507.632999467629816, 234.5106451484979857 ) ) ;
#75016=CARTESIAN_POINT ( 'NONE',  ( 43.45502302935310723, 1452.785528273959926, 266.7626567147260062 ) ) ;
#75018=CARTESIAN_POINT ( 'NONE',  ( 0.01343953231439999965, 1420.440497145129939, 182.6621881913980019 ) ) ;
#75020=VERTEX_POINT ( 'NONE', #80909 ) ;
#75021=CARTESIAN_POINT ( 'NONE',  ( 18.94560633146422646, 1457.569462139888174, 226.8026088545746575 ) ) ;
#75024=ORIENTED_EDGE ( 'NONE', *, *, #30281, .T. ) ;
#75027=CARTESIAN_POINT ( 'NONE',  ( 26.92382706682879956, 1450.690882430039892, 136.4499193319570054 ) ) ;
#75034=CARTESIAN_POINT ( 'NONE',  ( 2.069045789006210168, 1408.985313058389920, 186.9468566560059912 ) ) ;
#75035=CARTESIAN_POINT ( 'NONE',  ( -13.70980395804599894, 1434.975228763560153, 148.6203963862629962 ) ) ;
#75036=CARTESIAN_POINT ( 'NONE',  ( -9.849896899200842881, 1512.913060387330006, 185.5490084180013923 ) ) ;
#75040=ORIENTED_EDGE ( 'NONE', *, *, #83689, .F. ) ;
#75041=CARTESIAN_POINT ( 'NONE',  ( 13.84930592310000108, 1431.437219492539953, 209.1218459616979999 ) ) ;
#75043=CARTESIAN_POINT ( 'NONE',  ( 19.42500282749999840, 1440.913060387330006, 212.4633492400480179 ) ) ;
#75049=B_SPLINE_CURVE_WITH_KNOTS ( 'NONE', 5,
 ( #24217, #15264, #33725, #58403, #101467, #92528 ),
 .UNSPECIFIED., .F., .F.,
 ( 6, 6 ),
 ( 0.000000000000000000, 1.000000000000000000 ),
 .UNSPECIFIED. ) ;
#75051=CARTESIAN_POINT ( 'NONE',  ( -38.34143788450000301, 1440.913060387330006, 265.6112250856980381 ) ) ;
#75054=CARTESIAN_POINT ( 'NONE',  ( 11.19902647940000051, 1433.912128383429945, 151.6118626633980284 ) ) ;
#75056=CARTESIAN_POINT ( 'NONE',  ( 38.34143791959999703, 1445.301772804310076, 265.6112249940979950 ) ) ;
#75058=CARTESIAN_POINT ( 'NONE',  ( 0.6029167771809720300, 1450.892006063709914, 181.3029698405979957 ) ) ;
#75061=CARTESIAN_POINT ( 'NONE',  ( -15.06280282045160135, 1422.388303761650150, 229.4662100962750060 ) ) ;
#75063=CARTESIAN_POINT ( 'NONE',  ( 0.4794255386042003408, 1405.913060387330006, 209.9994285235883922 ) ) ;
#75064=CARTESIAN_POINT ( 'NONE',  ( -16.38529143830000123, 1409.485247372730100, 224.6959630481979957 ) ) ;
#75066=CARTESIAN_POINT ( 'NONE',  ( 23.34982412120000106, 1410.912491262029789, 212.3764570079079874 ) ) ;
#75068=CARTESIAN_POINT ( 'NONE',  ( -16.57803587077799889, 1409.491951770299920, 193.0403171756620111 ) ) ;
#75073=CARTESIAN_POINT ( 'NONE',  ( -5.414686741919999768, 1414.913060387329779, 224.5644280759980234 ) ) ;
#75074=CARTESIAN_POINT ( 'NONE',  ( 0.2010103898936379807, 1462.424627048520051, 182.8490255985700230 ) ) ;
#75075=CARTESIAN_POINT ( 'NONE',  ( -3.177625270220000075, 1409.024025506930002, 224.1218459461979933 ) ) ;
#75077=CARTESIAN_POINT ( 'NONE',  ( -20.75326766870000128, 1443.913060387330006, 176.0807405191980024 ) ) ;
#75079=CARTESIAN_POINT ( 'NONE',  ( 11.94108349800000113, 1433.615462819619779, 149.6992079387979970 ) ) ;
#75080=CARTESIAN_POINT ( 'NONE',  ( -41.02967923220330704, 1440.575676735369825, 134.0999999980680002 ) ) ;
#75081=DIRECTION ( 'NONE',  ( 0.000000000000000000, 1.000000000000000000, 0.000000000000000000 ) ) ;
#75088=CARTESIAN_POINT ( 'NONE',  ( 40.31042593601753055, 1424.878999494629170, 269.1206013125691356 ) ) ;
#75098=CARTESIAN_POINT ( 'NONE',  ( -33.91369284169999787, 1450.440667306779915, 136.2454489651980225 ) ) ;
#75099=CARTESIAN_POINT ( 'NONE',  ( -15.92413569481509938, 1410.572088914639835, 226.6904944114299951 ) ) ;
#75101=ORIENTED_EDGE ( 'NONE', *, *, #99936, .F. ) ;
#75104=ADVANCED_FACE ( 'NONE', ( #98247 ), #43706, .T. ) ;
#75105=CARTESIAN_POINT ( 'NONE',  ( -20.45839004848103926, 1410.987468509325026, 219.7938153870166218 ) ) ;
#75107=CARTESIAN_POINT ( 'NONE',  ( -11.58478124459999847, 1415.063410489729904, 195.8970895505979968 ) ) ;
#75109=CARTESIAN_POINT ( 'NONE',  ( 17.99954280510000260, 1410.904693935329988, 222.9872207667980035 ) ) ;
#75111=CARTESIAN_POINT ( 'NONE',  ( -17.31663460169999880, 1423.877174748429979, 228.8047149553979978 ) ) ;
#75115=CARTESIAN_POINT ( 'NONE',  ( 22.72745892751103369, 1509.726953286472281, 190.1320399485649375 ) ) ;
#75118=CARTESIAN_POINT ( 'NONE',  ( -6.358210821802259716, 1484.708390028690019, 183.8747304888279928 ) ) ;
#75121=CARTESIAN_POINT ( 'NONE',  ( -4.244378810408340641, 1441.402155946249877, 162.0389632095809986 ) ) ;
#75124=CARTESIAN_POINT ( 'NONE',  ( -17.86814680931840016, 1424.407636215880075, 228.2372741570307255 ) ) ;
#75125=ORIENTED_EDGE ( 'NONE', *, *, #110155, .F. ) ;
#75128=CARTESIAN_POINT ( 'NONE',  ( -10.81505178339999951, 1424.921174125060134, 144.1620446054460274 ) ) ;
#75129=CARTESIAN_POINT ( 'NONE',  ( 15.81800194485040123, 1409.465360594919957, 192.8631252433119982 ) ) ;
#75131=CARTESIAN_POINT ( 'NONE',  ( 38.16825441870970081, 1438.635335183450024, 136.6032594511559921 ) ) ;
#75135=CARTESIAN_POINT ( 'NONE',  ( -1.507975160943080040, 1509.033140630240268, 179.3618957914489727 ) ) ;
#75136=CARTESIAN_POINT ( 'NONE',  ( 8.727063097277033776, 1465.247437969211205, 232.8215983573240635 ) ) ;
#75137=DIRECTION ( 'NONE',  ( 0.3081687959821757805, 0.7660444431188054848, 0.5640991972602825699 ) ) ;
#75138=CARTESIAN_POINT ( 'NONE',  ( -12.53380499174499896, 1442.773887286369927, 169.4755105688890069 ) ) ;
#75141=AXIS2_PLACEMENT_3D ( 'NONE', #81156, #89005, #61629 ) ;
#75143=VERTEX_POINT ( 'NONE', #3546 ) ;
#75145=DIRECTION ( 'NONE',  ( 0.000000000000000000, 0.000000000000000000, -1.000000000000000000 ) ) ;
#75147=CARTESIAN_POINT ( 'NONE',  ( 0.03326171229690000342, 1452.996462166429865, 183.2389499340980024 ) ) ;
#75149=CARTESIAN_POINT ( 'NONE',  ( -2.500000000000000000, 1439.384186984480039, 161.5055418259740065 ) ) ;
#75152=CARTESIAN_POINT ( 'NONE',  ( 11.76268527979999945, 1441.457099483779757, 188.0189021094980149 ) ) ;
#75153=CARTESIAN_POINT ( 'NONE',  ( -14.35695723135263080, 1409.414416381394858, 225.2789668424194929 ) ) ;
#75155=CARTESIAN_POINT ( 'NONE',  ( 25.00813785679999768, 1436.589730024439859, 137.9321018740980094 ) ) ;
#75162=CARTESIAN_POINT ( 'NONE',  ( 36.59185764445249589, 1440.913060387330006, 263.1072593421939700 ) ) ;
#75163=CARTESIAN_POINT ( 'NONE',  ( -0.0007030488943480552033, 1451.930198993764179, 153.9960485520721534 ) ) ;
#75165=CARTESIAN_POINT ( 'NONE',  ( -13.28956057169999916, 1415.163755984229965, 220.9230430223980193 ) ) ;
#75166=CARTESIAN_POINT ( 'NONE',  ( -11.50213147263169944, 1432.340329783160087, 151.2059272481280061 ) ) ;
#75173=CARTESIAN_POINT ( 'NONE',  ( 23.15595999055019760, 1424.857126420280110, 206.2044122327660034 ) ) ;
#75174=CARTESIAN_POINT ( 'NONE',  ( 15.52105024970000002, 1459.722504423429882, 231.1950374654979896 ) ) ;
#75176=CARTESIAN_POINT ( 'NONE',  ( -4.917407973280459643, 1422.446740859282954, 184.8124456577417334 ) ) ;
#75185=CARTESIAN_POINT ( 'NONE',  ( -11.12297507747387648, 1425.174378293636664, 138.4895836007016783 ) ) ;
#75189=AXIS2_PLACEMENT_3D ( 'NONE', #50787, #412, #34529 ) ;
#75191=CARTESIAN_POINT ( 'NONE',  ( -11.29090808720000005, 1431.527451484140101, 151.4782487668979911 ) ) ;
#75194=CARTESIAN_POINT ( 'NONE',  ( -1.143529715360000064E-14, 1421.542806690330053, 144.1893924737979944 ) ) ;
#75196=CARTESIAN_POINT ( 'NONE',  ( -2.500000000000000000, 1443.913060387330006, 150.6726614421979775 ) ) ;
#75197=CARTESIAN_POINT ( 'NONE',  ( -25.84761762660000173, 1508.004946167130129, 217.5423480708579689 ) ) ;
#75198=CARTESIAN_POINT ( 'NONE',  ( -11.86982405321400691, 1423.326458348926963, 137.0999999980979567 ) ) ;
#75199=CARTESIAN_POINT ( 'NONE',  ( -1.831351330479999762, 1484.703635172929808, 182.8316381303979767 ) ) ;
#75200=EDGE_LOOP ( 'NONE', ( #2347, #48986, #44635, #66751 ) ) ;
#75202=CARTESIAN_POINT ( 'NONE',  ( 4.968383026439999739, 1406.259165937729904, 269.0361203054980024 ) ) ;
#75205=CARTESIAN_POINT ( 'NONE',  ( 24.08566870183141262, 1435.968196123745429, 213.6274238454907106 ) ) ;
#75211=CARTESIAN_POINT ( 'NONE',  ( -12.96862445230000027, 1444.929287191270078, 186.6030988806980133 ) ) ;
#75213=CARTESIAN_POINT ( 'NONE',  ( -19.89217962195755263, 1485.003688521414915, 190.9128337503663317 ) ) ;
#75218=CARTESIAN_POINT ( 'NONE',  ( -3.114882401780000087, 1426.979439823029907, 214.3676144197979738 ) ) ;
#75219=CARTESIAN_POINT ( 'NONE',  ( 10.73498917976377243, 1424.972937926497934, 139.1354244534461202 ) ) ;
#75221=CARTESIAN_POINT ( 'NONE',  ( -1.764294607579999896, 1475.537171245129912, 269.2935847982979567 ) ) ;
#75222=DIRECTION ( 'NONE',  ( -0.003573437736213522058, 0.9999913661844085366, -0.002120872317155135696 ) ) ;
#75228=CARTESIAN_POINT ( 'NONE',  ( 11.48964235903519970, 1415.152886233159961, 222.8125005102990031 ) ) ;
#75233=CARTESIAN_POINT ( 'NONE',  ( -22.51025611740000087, 1410.194216029730114, 203.9745233452079844 ) ) ;
#75235=CARTESIAN_POINT ( 'NONE',  ( -15.64999484340200198, 1421.347476133591954, 227.1285184359570053 ) ) ;
#75236=CARTESIAN_POINT ( 'NONE',  ( -35.67154068219999630, 1419.369011970829888, 269.2338164377980547 ) ) ;
#75237=EDGE_LOOP ( 'NONE', ( #19239, #33870, #39496, #103773 ) ) ;
#75242=CARTESIAN_POINT ( 'NONE',  ( 10.77813231690000073, 1424.944499019330124, 141.8424095806979892 ) ) ;
#75248=CARTESIAN_POINT ( 'NONE',  ( -11.17472318950760979, 1414.941152333697573, 196.0144180821544353 ) ) ;
#75249=AXIS2_PLACEMENT_3D ( 'NONE', #105202, #97338, #20076 ) ;
#75251=LINE ( 'NONE', #86800, #26723 ) ;
#75252=CARTESIAN_POINT ( 'NONE',  ( -8.792429487396887566, 1398.173735791722265, 199.4398815334327537 ) ) ;
#75259=ORIENTED_EDGE ( 'NONE', *, *, #13323, .F. ) ;
#75260=CARTESIAN_POINT ( 'NONE',  ( 11.97071048005270022, 1433.593009549930002, 149.8699161731940137 ) ) ;
#75261=CARTESIAN_POINT ( 'NONE',  ( -10.12349441079999934, 1396.444906704929735, 216.2323542477279830 ) ) ;
#75262=CARTESIAN_POINT ( 'NONE',  ( -21.78276643210000074, 1409.837828932429829, 213.4025661265980034 ) ) ;
#75264=CARTESIAN_POINT ( 'NONE',  ( -13.50816072687143610, 1444.048915240285851, 169.3527851728482005 ) ) ;
#75265=CARTESIAN_POINT ( 'NONE',  ( 21.68893548844135921, 1509.708255528440077, 229.4365290369073875 ) ) ;
#75268=CARTESIAN_POINT ( 'NONE',  ( -14.01968694497010048, 1509.108030625119909, 183.6010202189160054 ) ) ;
#75269=( BOUNDED_CURVE ( )  B_SPLINE_CURVE ( 3, ( #27302, #1023, #10505, #12154 ),
 .UNSPECIFIED., .F., .T. ) 
 B_SPLINE_CURVE_WITH_KNOTS ( ( 4, 4 ),
 ( 2.650173097296665059, 3.567460430156555340 ),
 .UNSPECIFIED. ) 
 CURVE ( )  GEOMETRIC_REPRESENTATION_ITEM ( )  RATIONAL_B_SPLINE_CURVE ( ( 1.000000000000000000, 0.9311025432363498888, 0.9311025432363498888, 1.000000000000000000 ) ) 
 REPRESENTATION_ITEM ( '' )  );
#75271=CARTESIAN_POINT ( 'NONE',  ( 0.7226347908460000191, 1449.242467270309817, 183.4668519528979971 ) ) ;
#75273=CARTESIAN_POINT ( 'NONE',  ( -28.84709929359999947, 1507.919204203629988, 212.2396942135479776 ) ) ;
#75274=CARTESIAN_POINT ( 'NONE',  ( 10.81179928114259958, 1396.290616737959908, 211.5056212398530135 ) ) ;
#75275=CARTESIAN_POINT ( 'NONE',  ( 1.052431931509999918, 1415.163755984130148, 191.3800010946980024 ) ) ;
#75276=CARTESIAN_POINT ( 'NONE',  ( 10.95104177029999981, 1431.009226238560132, 151.6519986001979987 ) ) ;
#75277=CARTESIAN_POINT ( 'NONE',  ( 7.368183369116096060, 1509.171485936123418, 180.6959945992290670 ) ) ;
#75279=CARTESIAN_POINT ( 'NONE',  ( 13.45926565268829833, 1434.961840340200069, 149.1575143944549779 ) ) ;
#75280=VERTEX_POINT ( 'NONE', #1745 ) ;
#75281=ORIENTED_EDGE ( 'NONE', *, *, #86512, .F. ) ;
#75282=B_SPLINE_CURVE_WITH_KNOTS ( 'NONE', 5,
 ( #39665, #63781, #73833, #40211, #107960, #31257 ),
 .UNSPECIFIED., .F., .F.,
 ( 6, 6 ),
 ( -26.18269281474930210, -9.354787281509999275 ),
 .UNSPECIFIED. ) ;
#75284=CARTESIAN_POINT ( 'NONE',  ( -11.28279764400000040, 1462.173053641429988, 233.6667625336980052 ) ) ;
#75290=CARTESIAN_POINT ( 'NONE',  ( -1.802000870929999943, 1412.180318182730161, 185.9687240695979824 ) ) ;
#75292=ADVANCED_FACE ( 'NONE', ( #68954 ), #105468, .T. ) ;
#75297=CARTESIAN_POINT ( 'NONE',  ( -20.16473732820000109, 1508.103700725129784, 228.9069202426980212 ) ) ;
#75299=CARTESIAN_POINT ( 'NONE',  ( -4.377978033840000727, 1409.571113459229991, 187.0373285412979953 ) ) ;
#75302=CARTESIAN_POINT ( 'NONE',  ( -0.4156091144146349947, 1414.971513442450032, 225.9103026676290256 ) ) ;
#75303=ORIENTED_EDGE ( 'NONE', *, *, #44047, .T. ) ;
#75304=CARTESIAN_POINT ( 'NONE',  ( 19.28571478079999935, 1426.671932083830143, 223.6657923338979970 ) ) ;
#75307=CARTESIAN_POINT ( 'NONE',  ( -0.1360178087611779996, 1465.118855296690072, 238.1340914064880110 ) ) ;
#75308=CARTESIAN_POINT ( 'NONE',  ( 7.287605107886430567, 1410.487174745140010, 269.8696506321609832 ) ) ;
#75311=CARTESIAN_POINT ( 'NONE',  ( 23.58142271390000033, 1409.993431820429805, 209.1798619000200290 ) ) ;
#75312=DIRECTION ( 'NONE',  ( 0.03489949670250207941, -0.9993908270190957621, 0.000000000000000000 ) ) ;
#75313=CARTESIAN_POINT ( 'NONE',  ( -9.052499326103495392, 1423.899425168531707, 139.1406965814004764 ) ) ;
#75316=CARTESIAN_POINT ( 'NONE',  ( 6.661338147749999709E-15, 1409.413060387330006, 271.1218459616979999 ) ) ;
#75317=CARTESIAN_POINT ( 'NONE',  ( 0.1095215363050000001, 1420.452175220630124, 183.3292552232980199 ) ) ;
#75319=CARTESIAN_POINT ( 'NONE',  ( 10.97434689771020011, 1432.635640446739899, 151.7699405381439988 ) ) ;
#75321=ORIENTED_EDGE ( 'NONE', *, *, #59024, .T. ) ;
#75323=CARTESIAN_POINT ( 'NONE',  ( 21.01925983530000153, 1472.811094121630049, 267.0604550193979776 ) ) ;
#75326=CARTESIAN_POINT ( 'NONE',  ( -2.256759385399999651, 1417.436677706029968, 235.4758680199980176 ) ) ;
#75327=CARTESIAN_POINT ( 'NONE',  ( -2.502335351479658687, 1409.000443863340479, 194.1336473601319028 ) ) ;
#75328=CARTESIAN_POINT ( 'NONE',  ( -22.76291043979999884, 1450.494225485409743, 218.6578027092980108 ) ) ;
#75329=CARTESIAN_POINT ( 'NONE',  ( 1.442588533962650077, 1452.743361456999992, 183.4687140882980145 ) ) ;
#75335=ORIENTED_EDGE ( 'NONE', *, *, #77509, .T. ) ;
#75338=CARTESIAN_POINT ( 'NONE',  ( 29.22958591949999985, 1509.933780019529877, 206.4713313151879959 ) ) ;
#75339=CARTESIAN_POINT ( 'NONE',  ( 23.25962669879999822, 1449.876265820790195, 217.4989437420879881 ) ) ;
#75340=CARTESIAN_POINT ( 'NONE',  ( 8.737553414955298692, 1437.268927995063223, 153.2801379038078267 ) ) ;
#75343=CARTESIAN_POINT ( 'NONE',  ( 15.59609131893944145, 1421.004437767239551, 227.6468209294606027 ) ) ;
#75345=CARTESIAN_POINT ( 'NONE',  ( 29.70843182346579781, 1435.695031758189998, 136.0745602649149930 ) ) ;
#75347=CARTESIAN_POINT ( 'NONE',  ( -21.38922153579999730, 1429.213524300029803, 219.6571118298979854 ) ) ;
#75348=CARTESIAN_POINT ( 'NONE',  ( -40.78917446724263840, 1456.261474242062377, 269.1081404453464074 ) ) ;
#75350=CARTESIAN_POINT ( 'NONE',  ( -16.16168812540000133, 1413.305022623530022, 226.8025051581979881 ) ) ;
#75353=CARTESIAN_POINT ( 'NONE',  ( -36.74716693956014524, 1455.731669175984734, 269.5566863843520764 ) ) ;
#75354=ORIENTED_EDGE ( 'NONE', *, *, #39428, .F. ) ;
#75360=CARTESIAN_POINT ( 'NONE',  ( -12.81686556575074754, 1444.973820179284985, 186.0349837055798901 ) ) ;
#75364=DIRECTION ( 'NONE',  ( 0.000000000000000000, -1.000000000000000000, 0.000000000000000000 ) ) ;
#75365=CARTESIAN_POINT ( 'NONE',  ( -14.06542466742875241, 1451.183651944110807, 150.3012616716959542 ) ) ;
#75366=CARTESIAN_POINT ( 'NONE',  ( 25.19391193610000101, 1436.451707861340083, 137.5385279504980076 ) ) ;
#75367=CARTESIAN_POINT ( 'NONE',  ( -12.74333518134357135, 1442.824178483951528, 169.4555743853381102 ) ) ;
#75368=CARTESIAN_POINT ( 'NONE',  ( -14.29519668260000032, 1410.788278260029983, 226.8469779139979892 ) ) ;
#75370=CARTESIAN_POINT ( 'NONE',  ( 0.02268235321126050100, 1415.088136167450102, 192.1344077303680251 ) ) ;
#75371=CARTESIAN_POINT ( 'NONE',  ( 21.03123203779729877, 1507.789098030329797, 226.0655639048319756 ) ) ;
#75372=ORIENTED_EDGE ( 'NONE', *, *, #48382, .F. ) ;
#75373=ORIENTED_EDGE ( 'NONE', *, *, #100810, .F. ) ;
#75377=CARTESIAN_POINT ( 'NONE',  ( -28.01911545579999796, 1440.913060392269927, 231.7019063163980093 ) ) ;
#75379=CARTESIAN_POINT ( 'NONE',  ( -11.25532750870000065, 1433.153001996420016, 151.5352189930979989 ) ) ;
#75380=EDGE_CURVE ( 'NONE', #18861, #30773, #101870, .T. ) ;
#75385=CARTESIAN_POINT ( 'NONE',  ( -24.38798815950000076, 1440.053814498560087, 212.0105281139480269 ) ) ;
#75389=CARTESIAN_POINT ( 'NONE',  ( -28.89012903238323204, 1510.032946564538861, 217.2102799419582482 ) ) ;
#75390=CARTESIAN_POINT ( 'NONE',  ( -9.230644300605730931E-10, 1416.774826112419987, 237.8701337189920082 ) ) ;
#75393=CARTESIAN_POINT ( 'NONE',  ( -11.84606637905420001, 1430.951851344180113, 149.8078499364760034 ) ) ;
#75395=CARTESIAN_POINT ( 'NONE',  ( -7.559855553260000249, 1473.430876107429867, 270.2818740090979759 ) ) ;
#75398=AXIS2_PLACEMENT_3D ( 'NONE', #61668, #26372, #79561 ) ;
#75402=CARTESIAN_POINT ( 'NONE',  ( 18.94015090468417739, 1456.918315522688317, 229.2628234610467359 ) ) ;
#75404=CARTESIAN_POINT ( 'NONE',  ( -20.65321958619999876, 1453.313060387329870, 208.1452065820600126 ) ) ;
#75406=CARTESIAN_POINT ( 'NONE',  ( -12.08748390050469901, 1407.204040152260177, 266.9029471222330017 ) ) ;
#75409=VERTEX_POINT ( 'NONE', #71728 ) ;
#75410=VERTEX_POINT ( 'NONE', #96333 ) ;
#75413=CARTESIAN_POINT ( 'NONE',  ( 4.919706779345196956, 1422.462138335776672, 184.3625360145741467 ) ) ;
#75418=CARTESIAN_POINT ( 'NONE',  ( -16.16311898949999915, 1470.468432338930143, 188.4789380148980058 ) ) ;
#75419=CARTESIAN_POINT ( 'NONE',  ( -16.56024668282710266, 1489.054572897799972, 229.4033101248429887 ) ) ;
#75422=ADVANCED_FACE ( 'NONE', ( #80077 ), #2652, .F. ) ;
#75426=CARTESIAN_POINT ( 'NONE',  ( -0.5805478587719999917, 1457.956445075529928, 229.5817085818979990 ) ) ;
#75427=EDGE_CURVE ( 'NONE', #103585, #98527, #73291, .T. ) ;
#75429=CARTESIAN_POINT ( 'NONE',  ( -44.70567387637289869, 1440.913053093850067, 269.9105629710239782 ) ) ;
#75431=CARTESIAN_POINT ( 'NONE',  ( -4.500000000000000000, 1425.929641636930000, 184.1455913746980002 ) ) ;
#75432=ORIENTED_EDGE ( 'NONE', *, *, #16752, .F. ) ;
#75433=CARTESIAN_POINT ( 'NONE',  ( 0.5697987610180000884, 1450.893162576140185, 181.2939918234980041 ) ) ;
#75436=DIRECTION ( 'NONE',  ( 0.9995237709234254808, 0.03085824620771311644, 1.984177796020841428E-13 ) ) ;
#75437=CARTESIAN_POINT ( 'NONE',  ( -12.87169627017330065, 1435.949072046520087, 150.7991738863709941 ) ) ;
#75438=CARTESIAN_POINT ( 'NONE',  ( -24.36381069329999960, 1441.240813755360023, 211.7027932903779970 ) ) ;
#75442=CARTESIAN_POINT ( 'NONE',  ( -0.1414919709576896445, 1452.990816532969802, 183.2406312904289223 ) ) ;
#75444=CARTESIAN_POINT ( 'NONE',  ( 3.203920217234287993, 1440.606318824109167, 157.0470840658564100 ) ) ;
#75447=CARTESIAN_POINT ( 'NONE',  ( -2.244421813216840089, 1451.951705408559974, 184.5463975505989822 ) ) ;
#75450=VECTOR ( 'NONE', #89566, 1000.000000000000000 ) ;
#75451=CARTESIAN_POINT ( 'NONE',  ( -19.40858652965227904, 1457.338511877794417, 226.2137482204685455 ) ) ;
#75454=CARTESIAN_POINT ( 'NONE',  ( 13.04232454877760006, 1435.170642384910252, 150.2281921783049938 ) ) ;
#75455=CARTESIAN_POINT ( 'NONE',  ( 12.33253873727779926, 1469.000856890969999, 231.6620758685679959 ) ) ;
#75458=CARTESIAN_POINT ( 'NONE',  ( 12.37159932449999822, 1415.628674266529742, 222.5813136582980007 ) ) ;
#75460=EDGE_CURVE ( 'NONE', #97581, #45814, #1777, .T. ) ;
#75462=CARTESIAN_POINT ( 'NONE',  ( 4.221456909779160327, 1441.605107385089923, 169.1511311007560039 ) ) ;
#75464=CARTESIAN_POINT ( 'NONE',  ( -11.97827956719999776, 1441.604408666619975, 150.7817505876979851 ) ) ;
#75468=CARTESIAN_POINT ( 'NONE',  ( -10.78869841497320081, 1414.913060387399810, 196.3854094717209762 ) ) ;
#75469=CARTESIAN_POINT ( 'NONE',  ( 15.75929536665272224, 1409.463372041439243, 192.9545506605122114 ) ) ;
#75471=FACE_OUTER_BOUND ( 'NONE', #85959, .T. ) ;
#75473=DIRECTION ( 'NONE',  ( 0.000000000000000000, -0.5032391393578591332, 0.8641471915237364243 ) ) ;
#75477=CARTESIAN_POINT ( 'NONE',  ( 17.27621958092441545, 1422.524277846433961, 226.6568626525910304 ) ) ;
#75478=CARTESIAN_POINT ( 'NONE',  ( 18.31070135516566211, 1425.421135919995777, 224.8731613538174656 ) ) ;
#75479=CARTESIAN_POINT ( 'NONE',  ( -10.96966316950000042, 1432.359729192660097, 151.7701366810979948 ) ) ;
#75480=CARTESIAN_POINT ( 'NONE',  ( 44.76106499233450364, 1440.913060369829964, 265.2081040044519682 ) ) ;
#75484=ORIENTED_EDGE ( 'NONE', *, *, #2658, .F. ) ;
#75486=CARTESIAN_POINT ( 'NONE',  ( -9.082054625942792114, 1506.560171907502763, 229.2575063132023558 ) ) ;
#75491=CARTESIAN_POINT ( 'NONE',  ( -11.40384261557694856, 1425.336176176961089, 144.1584481726092122 ) ) ;
#75492=ADVANCED_FACE ( 'NONE', ( #94385 ), #96512, .T. ) ;
#75496=CARTESIAN_POINT ( 'NONE',  ( -14.97895622270000082, 1489.469559537229998, 192.8507424827979833 ) ) ;
#75500=ORIENTED_EDGE ( 'NONE', *, *, #106537, .T. ) ;
#75505=VERTEX_POINT ( 'NONE', #38896 ) ;
#75506=ORIENTED_EDGE ( 'NONE', *, *, #70766, .F. ) ;
#75510=CARTESIAN_POINT ( 'NONE',  ( 0.8265244082521410185, 1408.941923255679967, 231.1644249228330068 ) ) ;
#75518=CARTESIAN_POINT ( 'NONE',  ( 0.8297112819069999423, 1408.942034543729960, 186.6238164324980175 ) ) ;
#75519=CARTESIAN_POINT ( 'NONE',  ( 13.03373128269810088, 1424.818470566259975, 222.5271577161219909 ) ) ;
#75521=CARTESIAN_POINT ( 'NONE',  ( -3.656266903649279865, 1441.517177768429974, 170.5484099602190042 ) ) ;
#75522=AXIS2_PLACEMENT_3D ( 'NONE', #22246, #99514, #73240 ) ;
#75523=CARTESIAN_POINT ( 'NONE',  ( -1.835529294006269962, 1450.383122819009941, 182.7749848618290116 ) ) ;
#75524=EDGE_LOOP ( 'NONE', ( #71057, #8452, #82740, #98925 ) ) ;
#75525=CARTESIAN_POINT ( 'NONE',  ( -4.310970535356173805, 1398.041661513277631, 196.6635432619665380 ) ) ;
#75526=CARTESIAN_POINT ( 'NONE',  ( 19.08737576949210180, 1456.351080380050007, 226.3347076951879728 ) ) ;
#75528=ADVANCED_FACE ( 'NONE', ( #39468 ), #36601, .T. ) ;
#75530=CARTESIAN_POINT ( 'NONE',  ( 18.44118978608688764, 1436.374823392123290, 146.9772265392791439 ) ) ;
#75536=CARTESIAN_POINT ( 'NONE',  ( 13.64863627425580006, 1508.988455644710029, 233.7698699238879954 ) ) ;
#75540=CARTESIAN_POINT ( 'NONE',  ( 5.096730495175649800, 1407.739527309109917, 221.2177969142850031 ) ) ;
#75543=CARTESIAN_POINT ( 'NONE',  ( -27.01669389746110284, 1451.969651449090179, 135.0017772683769977 ) ) ;
#75544=ORIENTED_EDGE ( 'NONE', *, *, #26363, .F. ) ;
#75545=CARTESIAN_POINT ( 'NONE',  ( 30.53571888390000311, 1438.952188675479874, 240.1260121752980012 ) ) ;
#75547=CARTESIAN_POINT ( 'NONE',  ( -17.45344265050000132, 1410.019001388030119, 194.6345986913979971 ) ) ;
#75548=ADVANCED_FACE ( 'NONE', ( #96431 ), #11581, .F. ) ;
#75549=CARTESIAN_POINT ( 'NONE',  ( -2.441800263710489638, 1419.516450075849889, 186.0746046563270113 ) ) ;
#75550=DIRECTION ( 'NONE',  ( -0.8383970168982891602, -0.5450600352768949497, 0.000000000000000000 ) ) ;
#75551=CARTESIAN_POINT ( 'NONE',  ( 0.5987183461865049905, 1507.212886145319999, 186.4932301926239688 ) ) ;
#75552=EDGE_CURVE ( 'NONE', #52837, #107294, #79184, .T. ) ;
#75553=CARTESIAN_POINT ( 'NONE',  ( -20.52850840453259806, 1452.196189077299778, 142.6025761593519974 ) ) ;
#75554=LINE ( 'NONE', #67153, #72212 ) ;
#75557=CARTESIAN_POINT ( 'NONE',  ( 16.91352249406399721, 1423.656902980690120, 228.6870985840920127 ) ) ;
#75559=ORIENTED_EDGE ( 'NONE', *, *, #100152, .T. ) ;
#75560=ORIENTED_EDGE ( 'NONE', *, *, #38039, .T. ) ;
#75562=CARTESIAN_POINT ( 'NONE',  ( -22.71281444701029884, 1409.706191629969908, 209.1573898883480069 ) ) ;
#75564=ORIENTED_EDGE ( 'NONE', *, *, #16557, .F. ) ;
#75565=CARTESIAN_POINT ( 'NONE',  ( -0.4885701619419999808, 1464.413060387330006, 229.7716327975979880 ) ) ;
#75566=FACE_OUTER_BOUND ( 'NONE', #68554, .T. ) ;
#75567=B_SPLINE_CURVE_WITH_KNOTS ( 'NONE', 3,
 ( #81233, #105915, #46019, #80147, #62276, #4013, #3467, #37595, #70689, #104801, #28647, #80704, #47107, #53887, #88023, #11307, #2922 ),
 .UNSPECIFIED., .F., .F.,
 ( 4, 2, 2, 2, 2, 1, 2, 2, 4 ),
 ( 0.000000000000000000, 0.2499999999999922284, 0.3749999999999876765, 0.4999999999999831246, 0.6249999999999785727, 0.6874999999999729106, 0.7187499999999863443, 0.7499999999999997780, 1.000000000000000000 ),
 .UNSPECIFIED. ) ;
#75568=EDGE_CURVE ( 'NONE', #3563, #24877, #30644, .T. ) ;
#75569=CARTESIAN_POINT ( 'NONE',  ( -4.416454581009999991, 1498.348563960429829, 236.0667878369980031 ) ) ;
#75570=CARTESIAN_POINT ( 'NONE',  ( -21.66372438889999685, 1410.866044241829968, 216.3363889088479937 ) ) ;
#75572=CARTESIAN_POINT ( 'NONE',  ( 44.51450203682119877, 1449.929878811980188, 268.5455458174560022 ) ) ;
#75574=CARTESIAN_POINT ( 'NONE',  ( -16.94980721129255841, 1421.957272272979026, 226.8340596599985872 ) ) ;
#75577=ORIENTED_EDGE ( 'NONE', *, *, #29783, .T. ) ;
#75578=CARTESIAN_POINT ( 'NONE',  ( 18.93123594888506389, 1457.623381184288746, 226.8509991318317986 ) ) ;
#75582=CARTESIAN_POINT ( 'NONE',  ( 2.500000000000000000, 1448.210448407430022, 182.3842139046979867 ) ) ;
#75583=CARTESIAN_POINT ( 'NONE',  ( 26.65315064050000160, 1451.818441385129745, 135.6605374257979975 ) ) ;
#75590=CARTESIAN_POINT ( 'NONE',  ( 2.975652649659970006, 1409.016972467610003, 187.2097493808250306 ) ) ;
#75591=CARTESIAN_POINT ( 'NONE',  ( 1.649770437750000207, 1417.467804857230021, 234.2977195291979911 ) ) ;
#75592=CARTESIAN_POINT ( 'NONE',  ( 27.01382310970000233, 1451.969724731730139, 134.9184576876980088 ) ) ;
#75596=ADVANCED_FACE ( 'NONE', ( #107161 ), #27650, .F. ) ;
#75597=CARTESIAN_POINT ( 'NONE',  ( 2.431412526649999961, 1428.647745098929818, 149.4227846719979880 ) ) ;
#75599=CARTESIAN_POINT ( 'NONE',  ( 12.73136601901799914, 1416.225364278609959, 221.9752797600760061 ) ) ;
#75600=CARTESIAN_POINT ( 'NONE',  ( 11.79676934137780187, 1432.336587679680179, 150.5395560521619984 ) ) ;
#75603=CARTESIAN_POINT ( 'NONE',  ( 9.407086540023099630, 1428.119775475241568, 137.0999999980979567 ) ) ;
#75606=CARTESIAN_POINT ( 'NONE',  ( -31.32742178079999462, 1444.517716081189974, 255.3819207742980097 ) ) ;
#75608=CARTESIAN_POINT ( 'NONE',  ( 11.79248762149999941, 1433.694417784170128, 150.8231452198980094 ) ) ;
#75609=FACE_OUTER_BOUND ( 'NONE', #8829, .T. ) ;
#75611=DIRECTION ( 'NONE',  ( -0.8862055364699944482, 0.4630717415824551764, 0.01429367964246674658 ) ) ;
#75614=CARTESIAN_POINT ( 'NONE',  ( -19.62297883809999988, 1486.467287247530066, 189.8658461344980140 ) ) ;
#75615=CARTESIAN_POINT ( 'NONE',  ( 11.34243525793542595, 1398.249318583079003, 215.4825434740161541 ) ) ;
#75616=CARTESIAN_POINT ( 'NONE',  ( -16.75996197530000131, 1409.498331158530164, 224.9264968051979849 ) ) ;
#75617=FACE_OUTER_BOUND ( 'NONE', #83525, .T. ) ;
#75618=CARTESIAN_POINT ( 'NONE',  ( 12.59650095789967494, 1416.818673810193104, 223.3990019334950716 ) ) ;
#75619=CARTESIAN_POINT ( 'NONE',  ( -16.98925717958650239, 1409.671016636710192, 192.8613407240889899 ) ) ;
#75623=CARTESIAN_POINT ( 'NONE',  ( -3.923552080019999444, 1416.217772598529791, 227.2437918289980132 ) ) ;
#75625=CARTESIAN_POINT ( 'NONE',  ( 0.1707805864721430034, 1479.871249927690087, 182.0999213800499774 ) ) ;
#75627=ORIENTED_EDGE ( 'NONE', *, *, #52162, .T. ) ;
#75629=CARTESIAN_POINT ( 'NONE',  ( 0.4885701619419999808, 1464.413060387330006, 188.4720591257980118 ) ) ;
#75630=CARTESIAN_POINT ( 'NONE',  ( 13.19837685220000090, 1434.900414701970021, 149.9808420451980169 ) ) ;
#75631=CARTESIAN_POINT ( 'NONE',  ( -41.66177311457460064, 1443.657316188219966, 134.0999999982009854 ) ) ;
#75639=DIRECTION ( 'NONE',  ( -1.986099751379994994E-13, 1.179495926710000177E-14, 1.000000000000000000 ) ) ;
#75642=CARTESIAN_POINT ( 'NONE',  ( 3.913694301390000518, 1434.228895445299941, 184.9284356229979949 ) ) ;
#75646=ORIENTED_EDGE ( 'NONE', *, *, #66990, .F. ) ;
#75647=CARTESIAN_POINT ( 'NONE',  ( -30.94580702080000023, 1450.971962479829926, 136.2591019887980224 ) ) ;
#75648=CARTESIAN_POINT ( 'NONE',  ( -15.72592697610619972, 1409.716376149900043, 226.1430192477070023 ) ) ;
#75650=VERTEX_POINT ( 'NONE', #39959 ) ;
#75652=CARTESIAN_POINT ( 'NONE',  ( -17.74610122149952574, 1410.896492951278333, 225.1977723225998886 ) ) ;
#75655=CARTESIAN_POINT ( 'NONE',  ( 41.99750770990659277, 1442.862246457818856, 269.6474897767589027 ) ) ;
#75657=CARTESIAN_POINT ( 'NONE',  ( 18.99772002587713970, 1437.736752343170338, 213.2567656554087705 ) ) ;
#75658=CARTESIAN_POINT ( 'NONE',  ( 2.500000000000000000, 1436.879499737369997, 182.8948590198639863 ) ) ;
#75660=CARTESIAN_POINT ( 'NONE',  ( 8.099819236969999281, 1497.713060387329961, 229.6744222972979799 ) ) ;
#75663=CARTESIAN_POINT ( 'NONE',  ( 2.500000000320000026, 1447.619163115829906, 168.9991029863980145 ) ) ;
#75664=VERTEX_POINT ( 'NONE', #75774 ) ;
#75665=CARTESIAN_POINT ( 'NONE',  ( 14.90597039080000030, 1485.461822778330088, 224.8639988762980124 ) ) ;
#75666=FACE_OUTER_BOUND ( 'NONE', #20427, .T. ) ;
#75668=VERTEX_POINT ( 'NONE', #58426 ) ;
#75672=CARTESIAN_POINT ( 'NONE',  ( -24.18568768169999927, 1430.355574618330138, 205.7586331603280030 ) ) ;
#75673=CARTESIAN_POINT ( 'NONE',  ( -11.71631912920000040, 1426.708822453530047, 142.6848033031979810 ) ) ;
#75674=CARTESIAN_POINT ( 'NONE',  ( 16.11026621011109938, 1409.500970208199988, 192.7569509766140072 ) ) ;
#75676=CARTESIAN_POINT ( 'NONE',  ( 40.71506559347059806, 1443.618839491749895, 137.1015882309970095 ) ) ;
#75678=CARTESIAN_POINT ( 'NONE',  ( -6.814833847790001009, 1407.100405669529891, 264.8986903022980073 ) ) ;
#75679=CARTESIAN_POINT ( 'NONE',  ( -2.953034986745780355, 1509.089592128550066, 179.4428969035240016 ) ) ;
#75684=CARTESIAN_POINT ( 'NONE',  ( -36.32303967410180690, 1437.564594092069910, 136.5418270925559909 ) ) ;
#75690=CARTESIAN_POINT ( 'NONE',  ( -29.76000164536801762, 1509.996124611334608, 209.6549034325891796 ) ) ;
#75695=CARTESIAN_POINT ( 'NONE',  ( -40.70526293792549666, 1444.199265999389809, 137.0833899199729728 ) ) ;
#75697=FACE_OUTER_BOUND ( 'NONE', #97824, .T. ) ;
#75699=CARTESIAN_POINT ( 'NONE',  ( 38.70145357755679782, 1443.501467202841695, 136.9791754767358611 ) ) ;
#75705=CARTESIAN_POINT ( 'NONE',  ( 11.77190271057030202, 1427.168883215420010, 146.5473278980630027 ) ) ;
#75708=CARTESIAN_POINT ( 'NONE',  ( -13.56343219680000090, 1416.311719779230089, 221.8446948800979897 ) ) ;
#75709=CARTESIAN_POINT ( 'NONE',  ( -11.04095478537250052, 1432.346658662259870, 151.7150578551980118 ) ) ;
#75712=CARTESIAN_POINT ( 'NONE',  ( 24.16126765782752983, 1411.115443491750057, 209.3031085556986568 ) ) ;
#75713=CARTESIAN_POINT ( 'NONE',  ( -12.60572195280000152, 1419.902368950130040, 222.2409655462980140 ) ) ;
#75718=CARTESIAN_POINT ( 'NONE',  ( 23.38056391995960226, 1429.882408728640030, 206.2064200242359959 ) ) ;
#75724=ORIENTED_EDGE ( 'NONE', *, *, #46851, .F. ) ;
#75725=CARTESIAN_POINT ( 'NONE',  ( -1.313821539278499539, 1486.248793315761759, 181.8009333484911565 ) ) ;
#75728=CARTESIAN_POINT ( 'NONE',  ( -2.905385431959103482, 1484.613154424542927, 183.2707264708236892 ) ) ;
#75735=CARTESIAN_POINT ( 'NONE',  ( -11.73152282100000043, 1429.503122515530094, 150.1532985455980054 ) ) ;
#75736=CARTESIAN_POINT ( 'NONE',  ( 19.03555911386669663, 1456.921423106470002, 225.4803602023239932 ) ) ;
#75737=CARTESIAN_POINT ( 'NONE',  ( -5.711199616050000039, 1441.581233931670113, 184.9882973716979961 ) ) ;
#75740=CARTESIAN_POINT ( 'NONE',  ( 0.2707604742883649718, 1473.796951665749930, 188.2801592720749966 ) ) ;
#75741=CARTESIAN_POINT ( 'NONE',  ( -20.86338484379999869, 1482.728658250230183, 225.9420377470979986 ) ) ;
#75743=DIRECTION ( 'NONE',  ( -0.7067702477489239410, 0.03085653766399039377, -0.7067698995998028533 ) ) ;
#75744=VERTEX_POINT ( 'NONE', #97536 ) ;
#75746=CARTESIAN_POINT ( 'NONE',  ( 6.105441334590000046, 1407.073549914729938, 269.6382019816980460 ) ) ;
#75748=CARTESIAN_POINT ( 'NONE',  ( 19.03615913129999981, 1430.304308985630087, 193.6166698355980031 ) ) ;
#75749=CARTESIAN_POINT ( 'NONE',  ( 19.90509729610057121, 1426.429786633350204, 221.4441842125065705 ) ) ;
#75751=CARTESIAN_POINT ( 'NONE',  ( -1.497109119499999919, 1451.179563906029898, 183.7882761563980125 ) ) ;
#75754=CARTESIAN_POINT ( 'NONE',  ( -13.98755486559999817, 1445.075814781340114, 188.4942211249980062 ) ) ;
#75755=CARTESIAN_POINT ( 'NONE',  ( -17.70665509759999878, 1431.113060387329824, 216.0622255360179906 ) ) ;
#75758=CARTESIAN_POINT ( 'NONE',  ( 1.456387282373979852, 1499.454921913780026, 181.4473683478569797 ) ) ;
#75759=CARTESIAN_POINT ( 'NONE',  ( -18.41412373400000035, 1436.828957585569924, 209.1218459616979999 ) ) ;
#75760=CARTESIAN_POINT ( 'NONE',  ( 11.37049604718461460, 1425.640868497123847, 139.1352433683615288 ) ) ;
#75762=CARTESIAN_POINT ( 'NONE',  ( -7.085242296889999736, 1475.668883530029916, 267.5158693932980327 ) ) ;
#75763=CARTESIAN_POINT ( 'NONE',  ( 1.363639811660000145, 1415.765555525229956, 232.8698637559979829 ) ) ;
#75765=CARTESIAN_POINT ( 'NONE',  ( 17.99974041169339856, 1410.897141673580109, 222.9863982244630165 ) ) ;
#75768=CARTESIAN_POINT ( 'NONE',  ( 11.39648212921470005, 1415.089996090470095, 222.7196566067729862 ) ) ;
#75771=CARTESIAN_POINT ( 'NONE',  ( -2.370970874524632510, 1427.002265528473799, 137.0999999980979851 ) ) ;
#75772=CARTESIAN_POINT ( 'NONE',  ( -20.52142497200000193, 1409.629684344930183, 201.2216482221679712 ) ) ;
#75774=CARTESIAN_POINT ( 'NONE',  ( 22.86388141461030088, 1452.114636054890070, 134.1000000004160029 ) ) ;
#75775=CARTESIAN_POINT ( 'NONE',  ( 2.812944321919999856E-11, 1407.650947899530138, 270.1377426963979929 ) ) ;
#75780=CARTESIAN_POINT ( 'NONE',  ( 11.71755446250000077, 1426.708321543429975, 142.7746014835979906 ) ) ;
#75782=CARTESIAN_POINT ( 'NONE',  ( 11.69707250263080134, 1426.722100592200150, 141.3107068769770081 ) ) ;
#75783=CARTESIAN_POINT ( 'NONE',  ( -15.80104652479535865, 1409.464839237975184, 225.2834576049114617 ) ) ;
#75789=DIRECTION ( 'NONE',  ( 0.9993908270190955401, -0.03489949670250328678, 0.000000000000000000 ) ) ;
#75790=CARTESIAN_POINT ( 'NONE',  ( -7.235185706049999332, 1427.271387135730038, 145.8323558008980001 ) ) ;
#75794=CARTESIAN_POINT ( 'NONE',  ( 20.36359139708810062, 1509.286488361670081, 229.5241780718589837 ) ) ;
#75795=CIRCLE ( 'NONE', #79397, 1.999999999999998224 ) ;
#75798=VERTEX_POINT ( 'NONE', #79102 ) ;
#75799=CARTESIAN_POINT ( 'NONE',  ( 12.03364418142640169, 1433.763248732019974, 149.8196365535399934 ) ) ;
#75800=CARTESIAN_POINT ( 'NONE',  ( -5.378824549970000035, 1397.157102389529882, 221.2434471751980141 ) ) ;
#75801=EDGE_LOOP ( 'NONE', ( #94, #48061, #22903 ) ) ;
#75805=FACE_OUTER_BOUND ( 'NONE', #31341, .T. ) ;
#75806=CARTESIAN_POINT ( 'NONE',  ( 17.63676453250000264, 1421.690910225529933, 226.2934404118979899 ) ) ;
#75807=CARTESIAN_POINT ( 'NONE',  ( 4.752926588879999414, 1507.807331693730021, 235.7611666444980187 ) ) ;
#75809=CARTESIAN_POINT ( 'NONE',  ( 1.435641954649999885, 1429.773781293429920, 184.4573210536979957 ) ) ;
#75810=CARTESIAN_POINT ( 'NONE',  ( -0.3443454749849999552, 1415.932840167130053, 191.2798017309980025 ) ) ;
#75812=B_SPLINE_SURFACE_WITH_KNOTS ( 'NONE', 5, 4, ( 
 ( #8158, #110631, #101108, #8709, #49641 ),
 ( #66458, #109538, #23850, #34478, #41771 ),
 ( #67551, #83778, #7615, #110081, #41229 ),
 ( #50199, #351, #58042, #17082, #68653 ),
 ( #93273, #32812, #33358, #14903, #92179 ),
 ( #101653, #24940, #25503, #51277, #16536 ) ),
 .UNSPECIFIED., .F., .F., .F.,
 ( 6, 6 ),
 ( 5, 5 ),
 ( 0.000000000000000000, 111.1101480259999903 ),
 ( 25.81581217359999769, 39.03307591160000101 ),
 .UNSPECIFIED. ) ;
#75814=CARTESIAN_POINT ( 'NONE',  ( 1.477202341570000188, 1415.048591094029916, 191.4945646901979899 ) ) ;
#75815=CARTESIAN_POINT ( 'NONE',  ( 11.76498060490000164, 1431.988698125490146, 150.8030710463980029 ) ) ;
#75818=CARTESIAN_POINT ( 'NONE',  ( 13.21130589195640148, 1435.383535301609982, 150.2969612372090182 ) ) ;
#75820=EDGE_LOOP ( 'NONE', ( #1063, #17702, #71020, #16009 ) ) ;
#75822=CARTESIAN_POINT ( 'NONE',  ( 13.07404856258703418, 1444.822502266877109, 169.4100179250317524 ) ) ;
#75823=CARTESIAN_POINT ( 'NONE',  ( -9.455441787850000779, 1462.981412785230077, 234.6731641070979890 ) ) ;
#75827=B_SPLINE_SURFACE_WITH_KNOTS ( 'NONE', 5, 5, ( 
 ( #94477, #96716, #62029, #96149, #27291, #60922, #95598, #44105, #52510, #86639, #2675, #105108 ),
 ( #36800, #78805, #61472, #17750, #19986, #35137, #95051, #36246, #103426, #68768, #18867, #53064 ),
 ( #87201, #10493, #44664, #51952, #43551, #69318, #78242, #86094, #1555, #2120, #45779, #70434 ),
 ( #77698, #18319, #35687, #69878, #103993, #104552, #27848, #19427, #11052, #53629, #87771, #70992 ),
 ( #45223, #28399, #62599, #54180, #88308, #11600, #79914, #34583, #102871, #81004, #4311, #38438 ),
 ( #56911, #65325, #106205, #30598, #72614, #106745, #30032, #90495, #82095, #89407, #28957, #64226 ),
 ( #64786, #4836, #81534, #98349, #91044, #21622, #98896, #31140, #37354, #80463, #20522, #12695 ),
 ( #89947, #105674, #5396, #46333, #47412, #55827, #99435, #13222, #38983, #55277, #3776, #46876 ),
 ( #39554, #73728, #88857, #29487, #22713, #73160, #97794, #107305, #22163, #56363, #54729, #13770 ),
 ( #3227, #47954, #14332, #12141, #107851, #48522, #37909, #71553, #63146, #63683, #97247, #72091 ),
 ( #21071, #75909, #66976, #7595, #68089, #41750, #59673, #31690, #33893, #110061, #33336, #75377 ),
 ( #92156, #100549, #23829, #16517, #42304, #65872, #84838, #15975, #109516, #99992, #102201, #83208 ),
 ( #84304, #40649, #5952, #101087, #32792, #7049, #24385, #58569, #92698, #108408, #91605, #49073 ),
 ( #23284, #58021, #50176, #93783, #67531, #50707, #57480, #74279, #74820, #14882, #15428, #6497 ),
 ( #108966, #59130, #101631, #24920, #8138, #32253, #93252, #76457, #110611, #66433, #25481, #17060 ) ),
 .UNSPECIFIED., .F., .F., .F.,
 ( 6, 3, 3, 3, 6 ),
 ( 6, 3, 3, 6 ),
 ( 1.933760562350000045, 17.84603210599999912, 29.17820978809999843, 40.51038747020000130, 63.41552668279999949 ),
 ( 84.36360869960000741, 126.5454130579999941, 147.6363152340000227, 168.7272174100000086 ),
 .UNSPECIFIED. ) ;
#75828=ORIENTED_EDGE ( 'NONE', *, *, #10386, .T. ) ;
#75829=CARTESIAN_POINT ( 'NONE',  ( -15.46700379407589843, 1461.188231737419756, 228.6959062608830209 ) ) ;
#75830=CARTESIAN_POINT ( 'NONE',  ( 3.500000000000000000, 1422.625370988529994, 168.5578661042980286 ) ) ;
#75837=CARTESIAN_POINT ( 'NONE',  ( -18.70459389479999857, 1509.566239199129996, 231.7064163551980016 ) ) ;
#75839=CARTESIAN_POINT ( 'NONE',  ( -5.839839396159999474, 1410.494359662829993, 187.1215865486979908 ) ) ;
#75841=CARTESIAN_POINT ( 'NONE',  ( 0.3622025831177250188, 1416.825783990419950, 227.1772706819449752 ) ) ;
#75842=EDGE_LOOP ( 'NONE', ( #108153, #48802, #41548, #61801, #66936 ) ) ;
#75843=CARTESIAN_POINT ( 'NONE',  ( 20.55965903059999889, 1427.339473409130051, 220.5198651377980070 ) ) ;
#75848=CARTESIAN_POINT ( 'NONE',  ( 22.71938917269999791, 1409.706427035829847, 209.1785880919549925 ) ) ;
#75849=CARTESIAN_POINT ( 'NONE',  ( -20.70499093180000116, 1508.886810853430006, 189.6386861211979920 ) ) ;
#75854=CARTESIAN_POINT ( 'NONE',  ( 1.232505279462991599, 1409.632634667178309, 232.4911126170792386 ) ) ;
#75856=ORIENTED_EDGE ( 'NONE', *, *, #40020, .T. ) ;
#75858=CARTESIAN_POINT ( 'NONE',  ( 6.248998597759999996, 1472.348800618430005, 259.9484879023979715 ) ) ;
#75863=CARTESIAN_POINT ( 'NONE',  ( 1.082466572113199854, 1452.866867491690073, 183.3918909070579844 ) ) ;
#75871=FACE_OUTER_BOUND ( 'NONE', #93283, .T. ) ;
#75873=CARTESIAN_POINT ( 'NONE',  ( 12.64331018290000053, 1422.763132344930227, 223.6605244860979838 ) ) ;
#75879=CARTESIAN_POINT ( 'NONE',  ( 27.59657656778820112, 1436.356223077960067, 136.7068084802659769 ) ) ;
#75880=CARTESIAN_POINT ( 'NONE',  ( 39.68989170827939716, 1446.546521785269988, 136.7137753855650146 ) ) ;
#75881=CARTESIAN_POINT ( 'NONE',  ( 19.72497240319906453, 1506.501081259675175, 218.9625358929377228 ) ) ;
#75882=CARTESIAN_POINT ( 'NONE',  ( -31.92678845819044753, 1465.333974304449157, 269.3172746343190056 ) ) ;
#75884=CARTESIAN_POINT ( 'NONE',  ( 13.71041708839999984, 1507.516673751029884, 185.7221359422979958 ) ) ;
#75886=CARTESIAN_POINT ( 'NONE',  ( -38.72028640208406358, 1452.776172727556059, 269.5884039666330523 ) ) ;
#75888=CARTESIAN_POINT ( 'NONE',  ( -25.74682230153359797, 1470.140385610140129, 210.8607376181039683 ) ) ;
#75889=CARTESIAN_POINT ( 'NONE',  ( 8.899872388108134302, 1506.575640307498816, 188.8910645225604128 ) ) ;
#75892=CARTESIAN_POINT ( 'NONE',  ( 11.60004869885203327, 1427.574042486475491, 134.2792576386086694 ) ) ;
#75893=CARTESIAN_POINT ( 'NONE',  ( 19.47367602328466774, 1455.619968770807645, 226.0154353848046469 ) ) ;
#75896=CARTESIAN_POINT ( 'NONE',  ( -10.29038504730294079, 1418.125687189650080, 229.8187361617479496 ) ) ;
#75897=CARTESIAN_POINT ( 'NONE',  ( -6.735029543969123900, 1451.432364504263887, 153.2907587394053337 ) ) ;
#75899=CARTESIAN_POINT ( 'NONE',  ( 25.67235157149999836, 1436.336280272470049, 137.0204247850980153 ) ) ;
#75900=CARTESIAN_POINT ( 'NONE',  ( -12.66129559865252041, 1442.799074774669862, 169.4635015124096071 ) ) ;
#75902=CARTESIAN_POINT ( 'NONE',  ( 0.2892576526144139959, 1415.943166310999914, 191.0435026498350055 ) ) ;
#75903=CARTESIAN_POINT ( 'NONE',  ( 21.33887654814517632, 1508.922069170062969, 226.3421127776584285 ) ) ;
#75906=CARTESIAN_POINT ( 'NONE',  ( 12.53380665967529950, 1445.052233242549846, 186.0874955919830143 ) ) ;
#75909=CARTESIAN_POINT ( 'NONE',  ( -4.375233889810000498, 1463.532726167829878, 231.7907868280979926 ) ) ;
#75911=CARTESIAN_POINT ( 'NONE',  ( 4.228620053163889558, 1425.167187284519969, 185.3096231440469808 ) ) ;
#75913=CARTESIAN_POINT ( 'NONE',  ( -2.542765869541859569, 1420.835077523395967, 185.4948760842592606 ) ) ;
#75915=CARTESIAN_POINT ( 'NONE',  ( -14.66856476219100891, 1429.940063103053717, 222.0536632632462215 ) ) ;
#75917=CARTESIAN_POINT ( 'NONE',  ( 1.111971660999999889, 1450.991721771130187, 182.4208345951979879 ) ) ;
#75920=CARTESIAN_POINT ( 'NONE',  ( -2.708169622750910029E-09, 1414.562637300989763, 245.8823571257100014 ) ) ;
#75923=CARTESIAN_POINT ( 'NONE',  ( -11.80278639884820002, 1428.367824666609977, 148.3230517217830027 ) ) ;
#75925=CARTESIAN_POINT ( 'NONE',  ( -4.301461581549999913, 1474.025770959829970, 270.1336327149980434 ) ) ;
#75930=DIRECTION ( 'NONE',  ( 0.000000000000000000, -1.000000000000000000, 0.000000000000000000 ) ) ;
#75931=CARTESIAN_POINT ( 'NONE',  ( 38.63560632403650175, 1444.097728697520097, 137.1726987354860228 ) ) ;
#75934=CARTESIAN_POINT ( 'NONE',  ( -20.41013681796389889, 1410.032071447750013, 269.3516173646369793 ) ) ;
#75935=CARTESIAN_POINT ( 'NONE',  ( -13.39296744828000030, 1434.924871481009859, 148.8778569621510144 ) ) ;
#75938=B_SPLINE_SURFACE_WITH_KNOTS ( 'NONE', 4, 5, ( 
 ( #48708, #58746, #33512, #90677, #82831, #23475 ),
 ( #6123, #57668, #75010, #109160, #100723, #24006 ),
 ( #92329, #68826, #27342, #52566, #44163, #86699 ),
 ( #9993, #77214, #52009, #26228, #78300, #2181 ),
 ( #34087, #94534, #18371, #1614, #110794, #35751 ) ),
 .UNSPECIFIED., .F., .F., .F.,
 ( 5, 5 ),
 ( 6, 6 ),
 ( 7.049146647299999735, 7.791777982190000174 ),
 ( 0.000000000000000000, 2.000000000000000000 ),
 .UNSPECIFIED. ) ;
#75941=ORIENTED_EDGE ( 'NONE', *, *, #6990, .T. ) ;
#75942=CARTESIAN_POINT ( 'NONE',  ( 4.827146942024284293, 1422.311623617143596, 184.2770325824816666 ) ) ;
#75943=CARTESIAN_POINT ( 'NONE',  ( -10.32735784461773498, 1512.913060387330006, 184.1749888460368538 ) ) ;
#75946=CARTESIAN_POINT ( 'NONE',  ( -18.93280221739999902, 1485.490082012730227, 189.5191571945979945 ) ) ;
#75948=CARTESIAN_POINT ( 'NONE',  ( -17.38692480600779788, 1507.629789030409938, 229.8496573937590028 ) ) ;
#75951=CARTESIAN_POINT ( 'NONE',  ( -28.77730029287999969, 1509.917985857419808, 212.2396942430650029 ) ) ;
#75953=CARTESIAN_POINT ( 'NONE',  ( -29.71730757640000320, 1509.987350256529908, 208.1891636974079915 ) ) ;
#75954=B_SPLINE_SURFACE_WITH_KNOTS ( 'NONE', 5, 5, ( 
 ( #100539, #48512, #99983, #103146, #31131, #109507 ),
 ( #22704, #101077, #66967, #23274, #108956, #58011 ),
 ( #82651, #85810, #82084, #92147, #99426, #75368 ),
 ( #9108, #66424, #65314, #56902, #32783, #57471 ),
 ( #32243, #5387, #83199, #24376, #23819, #91035 ),
 ( #5943, #83743, #40088, #40639, #108398, #74811 ) ),
 .UNSPECIFIED., .F., .F., .F.,
 ( 6, 6 ),
 ( 6, 6 ),
 ( 8.936092213160000242, 11.91340804030000022 ),
 ( 0.000000000000000000, 1.442075847869999983 ),
 .UNSPECIFIED. ) ;
#75955=CARTESIAN_POINT ( 'NONE',  ( 2.370970874524634286, 1427.002265528474027, 134.0999999980980135 ) ) ;
#75957=CARTESIAN_POINT ( 'NONE',  ( -2.599869711270000217, 1407.016598365429900, 196.2843278663980016 ) ) ;
#75958=CARTESIAN_POINT ( 'NONE',  ( -12.14658859679999914, 1409.337228609230124, 227.1535549678980317 ) ) ;
#75961=CARTESIAN_POINT ( 'NONE',  ( -27.47792036623960144, 1488.737008339370050, 209.1940319314329884 ) ) ;
#75962=CARTESIAN_POINT ( 'NONE',  ( 26.39526639180000345, 1469.246565959629834, 210.4302785482780109 ) ) ;
#75965=CARTESIAN_POINT ( 'NONE',  ( -24.09633375880000017, 1435.413152144519927, 137.5044708534980202 ) ) ;
#75966=CARTESIAN_POINT ( 'NONE',  ( -24.32956343839999747, 1442.099522796889914, 211.7759529297080121 ) ) ;
#75969=CARTESIAN_POINT ( 'NONE',  ( -0.01304300961527469875, 1452.999749643619907, 183.2385070609109903 ) ) ;
#75970=CARTESIAN_POINT ( 'NONE',  ( -14.54088437389999910, 1410.754219534529966, 226.7644051071980016 ) ) ;
#75971=CARTESIAN_POINT ( 'NONE',  ( 3.397541313661426976, 1440.732790238158714, 156.8344482731262133 ) ) ;
#75974=DIRECTION ( 'NONE',  ( 0.8771707529346988164, 0.03063147765598519048, -0.4792005663316608599 ) ) ;
#75979=CARTESIAN_POINT ( 'NONE',  ( 12.82065956846409804, 1434.792185812719936, 149.9145850215789721 ) ) ;
#75980=CARTESIAN_POINT ( 'NONE',  ( -4.086192991946269615, 1440.407209789042327, 185.3182923436035026 ) ) ;
#75983=CARTESIAN_POINT ( 'NONE',  ( 11.80119706069999985, 1415.163755984229965, 222.4114065333980079 ) ) ;
#75985=CARTESIAN_POINT ( 'NONE',  ( -18.13594796521936559, 1507.809373629487709, 187.1116949291995013 ) ) ;
#75987=ADVANCED_FACE ( 'NONE', ( #104284 ), #19591, .F. ) ;
#75989=CARTESIAN_POINT ( 'NONE',  ( 39.14754387628220655, 1437.687579064466945, 135.1140641504456426 ) ) ;
#75990=CARTESIAN_POINT ( 'NONE',  ( 20.67559640589999859, 1509.531575910530137, 188.3714930344980019 ) ) ;
#75992=ORIENTED_EDGE ( 'NONE', *, *, #97271, .F. ) ;
#75993=CARTESIAN_POINT ( 'NONE',  ( -12.78667974309999877, 1416.822694190629818, 195.3262915446979946 ) ) ;
#76003=CARTESIAN_POINT ( 'NONE',  ( 18.14860257456183845, 1425.108924779807012, 224.7878952339535488 ) ) ;
#76004=CARTESIAN_POINT ( 'NONE',  ( -9.771922359260001301, 1440.444625599219989, 148.8200729295979841 ) ) ;
#76005=CARTESIAN_POINT ( 'NONE',  ( 37.77835552715119860, 1440.913060384539904, 255.9250353463820034 ) ) ;
#76007=CARTESIAN_POINT ( 'NONE',  ( -16.06428792994629973, 1414.913060387329779, 209.3174441339999987 ) ) ;
#76008=CARTESIAN_POINT ( 'NONE',  ( -2.253566441613126910E-10, 1426.918876941764893, 137.0999999980980135 ) ) ;
#76012=CARTESIAN_POINT ( 'NONE',  ( -4.144683537393576422, 1507.117986068643631, 231.4540176283237543 ) ) ;
#76013=CARTESIAN_POINT ( 'NONE',  ( -24.38138866919999970, 1442.062446048410038, 212.1316646185979948 ) ) ;
#76014=CARTESIAN_POINT ( 'NONE',  ( 0.5133626083067620582, 1410.311097044259895, 185.0719925509139898 ) ) ;
#76015=DIRECTION ( 'NONE',  ( 0.000000000000000000, 0.000000000000000000, -1.000000000000000000 ) ) ;
#76016=CARTESIAN_POINT ( 'NONE',  ( 27.60404634758340947, 1509.989021275989899, 220.8700857203302519 ) ) ;
#76024=CARTESIAN_POINT ( 'NONE',  ( 10.67630109080000089, 1452.395781299630244, 151.6471186536979872 ) ) ;
#76030=CARTESIAN_POINT ( 'NONE',  ( -1.438892182569999845, 1452.191226611430011, 183.8587016213980121 ) ) ;
#76031=B_SPLINE_SURFACE_WITH_KNOTS ( 'NONE', 2, 5, ( 
 ( #85511, #60913, #103984, #8807, #44654, #59796 ),
 ( #77148, #86630, #1000, #103416, #26722, #18310 ),
 ( #452, #69867, #9924, #44095, #35678, #61463 ) ),
 .UNSPECIFIED., .F., .F., .F.,
 ( 3, 3 ),
 ( 6, 6 ),
 ( 1.399803019509999968, 2.016961153540000051 ),
 ( 0.000000000000000000, 1.000000000000000000 ),
 .UNSPECIFIED. ) ;
#76033=EDGE_CURVE ( 'NONE', #50772, #65089, #16585, .T. ) ;
#76039=CARTESIAN_POINT ( 'NONE',  ( 13.88129723608619948, 1507.515551148199847, 232.8168547917639728 ) ) ;
#76041=CARTESIAN_POINT ( 'NONE',  ( 39.82865069103799982, 1441.236877534039877, 136.8517713851130111 ) ) ;
#76042=CARTESIAN_POINT ( 'NONE',  ( -11.81135191919999983, 1436.410413307749877, 147.6956600043980075 ) ) ;
#76048=LINE ( 'NONE', #82785, #56766 ) ;
#76050=CARTESIAN_POINT ( 'NONE',  ( 3.378643529439999682, 1409.031045219230009, 187.3370713307979827 ) ) ;
#76053=CARTESIAN_POINT ( 'NONE',  ( -3.137828956056770480, 1440.800072403580089, 158.1453491124979962 ) ) ;
#76054=DIRECTION ( 'NONE',  ( 0.000000000000000000, 0.000000000000000000, -1.000000000000000000 ) ) ;
#76058=CARTESIAN_POINT ( 'NONE',  ( -1.633469776390000128, 1432.353341358199941, 150.3624711946980028 ) ) ;
#76062=CARTESIAN_POINT ( 'NONE',  ( 15.16669330050000042, 1430.147119278929949, 190.8796077056979925 ) ) ;
#76063=CARTESIAN_POINT ( 'NONE',  ( -1.718598421969799969E-10, 1470.598202367599924, 255.5842205547500043 ) ) ;
#76065=CARTESIAN_POINT ( 'NONE',  ( -0.9297777941500000587, 1416.254459046630018, 227.9489298555980099 ) ) ;
#76066=CARTESIAN_POINT ( 'NONE',  ( -23.75590350410000440, 1435.760101040910058, 211.5282110633580146 ) ) ;
#76071=CARTESIAN_POINT ( 'NONE',  ( -0.4936889915673177698, 1485.614862604095151, 181.8905814463562365 ) ) ;
#76073=CARTESIAN_POINT ( 'NONE',  ( -46.14792574297130301, 1439.829534759850048, 266.9721075858579979 ) ) ;
#76074=CARTESIAN_POINT ( 'NONE',  ( 13.83038607890710203, 1509.255194850690032, 234.1910450026739738 ) ) ;
#76079=B_SPLINE_SURFACE_WITH_KNOTS ( 'NONE', 5, 5, ( 
 ( #5580, #108585, #108022, #31319, #109153, #32437, #57661, #65502, #31871 ),
 ( #23998, #58194, #67707, #34081, #101816, #52557, #50359, #43598, #78291 ),
 ( #60408, #94526, #50895, #8318, #35742, #68818, #110232, #17800, #60972 ),
 ( #69929, #43050, #77207, #33506, #35185, #34634, #104042, #76094, #68274 ),
 ( #52001, #27334, #95097, #102381, #86141, #9434, #85025, #42479, #61520 ),
 ( #25110, #77749, #18363, #102919, #95648, #509, #26219, #59314, #69370 ),
 ( #84485, #93426, #25663, #1058, #103479, #7772, #86691, #9985, #41938 ),
 ( #44155, #1605, #26784, #16695, #76636, #110788, #59856, #93980, #17246 ),
 ( #51439, #8866, #85569, #62077, #21115, #88355, #46927, #55320, #63727 ),
 ( #29540, #38488, #96203, #11644, #28448, #37956, #45271, #80511, #97837 ),
 ( #63191, #19478, #89452, #72136, #97298, #62642, #3828, #3271, #2173 ),
 ( #54228, #37401, #71035, #36288, #78867, #70480, #79409, #12745, #96763 ),
 ( #71600, #105721, #12186, #106791, #72665, #30081, #104601, #20033, #45821 ),
 ( #44715, #29005, #53680, #27894, #81045, #87822, #11110, #2721, #53113 ),
 ( #46379, #4359, #36843, #64275, #79954, #88900, #20569, #105156, #54768 ),
 ( #106254, #18915, #87250, #10541, #73207, #14925, #91651, #5994, #48006 ),
 ( #82144, #55874, #107351, #49120, #30647, #92203, #66486, #83253, #6548 ),
 ( #108457, #31739, #49670, #39028, #40699, #73773, #64833, #89995, #100047 ),
 ( #21668, #100593, #15475, #74870, #13270, #7099, #90542, #23335, #22762 ),
 ( #39603, #4887, #47461, #98940, #5443, #58070, #31190, #57527, #82705 ),
 ( #109019, #75429, #41255, #109566, #22215, #65377, #99480, #65925, #81583 ) ),
 .UNSPECIFIED., .F., .F., .F.,
 ( 6, 3, 3, 3, 3, 3, 6 ),
 ( 6, 3, 6 ),
 ( 24.25933569942640133, 29.62372026779999956, 34.98808232409999874, 45.71680643680000600, 67.17425466199999562, 83.91850212199999248, 143.5761545054720045 ),
 ( -3.635447242111609987E-05, 1.000000000000000000, 2.000013395910110070 ),
 .UNSPECIFIED. ) ;
#76082=EDGE_CURVE ( 'NONE', #64525, #68085, #109022, .T. ) ;
#76083=CARTESIAN_POINT ( 'NONE',  ( -26.38863270286480045, 1451.975261639769997, 135.2102608963000137 ) ) ;
#76085=CARTESIAN_POINT ( 'NONE',  ( 26.67762293060000189, 1439.176105477569990, 225.6805344121979999 ) ) ;
#76087=CARTESIAN_POINT ( 'NONE',  ( 14.96370694810000046, 1488.812149333129810, 194.0324691636979821 ) ) ;
#76088=CARTESIAN_POINT ( 'NONE',  ( 14.45771159804956874, 1416.835807151514246, 196.8517380151662053 ) ) ;
#76091=CARTESIAN_POINT ( 'NONE',  ( -23.21186549893350204, 1452.102484182780017, 138.3455140363329861 ) ) ;
#76094=CARTESIAN_POINT ( 'NONE',  ( -1.793964770197490122, 1410.263195636249975, 269.6152129905299830 ) ) ;
#76095=CARTESIAN_POINT ( 'NONE',  ( -0.05321753368360000042, 1509.045416894829941, 239.1217103925980041 ) ) ;
#76099=CARTESIAN_POINT ( 'NONE',  ( -22.81975492585869958, 1409.709889425679876, 209.1761138208090074 ) ) ;
#76102=CARTESIAN_POINT ( 'NONE',  ( -45.67175128301336429, 1440.701170895977839, 266.1885892358925503 ) ) ;
#76103=CARTESIAN_POINT ( 'NONE',  ( -16.98033619447083353, 1436.324910093480185, 148.2366724938339928 ) ) ;
#76105=CARTESIAN_POINT ( 'NONE',  ( 35.68833539314010039, 1463.121747042800052, 268.5374238623429619 ) ) ;
#76108=CARTESIAN_POINT ( 'NONE',  ( -17.14314410641370046, 1422.256345865689354, 226.7315907088579650 ) ) ;
#76111=CARTESIAN_POINT ( 'NONE',  ( -11.59421085610000013, 1433.816539371060117, 151.1950375012979748 ) ) ;
#76113=CARTESIAN_POINT ( 'NONE',  ( 22.64490784369999687, 1409.703832166029997, 208.7208416667509994 ) ) ;
#76122=CARTESIAN_POINT ( 'NONE',  ( 1.483224784644179950, 1408.964855738119923, 186.7893816159290168 ) ) ;
#76123=CARTESIAN_POINT ( 'NONE',  ( 1.004776255440000154, 1416.277075963729885, 233.2712822367979868 ) ) ;
#76124=FACE_OUTER_BOUND ( 'NONE', #52157, .T. ) ;
#76125=ADVANCED_FACE ( 'NONE', ( #37495 ), #51759, .F. ) ;
#76129=CARTESIAN_POINT ( 'NONE',  ( 12.44185449472429994, 1415.426561690370136, 221.4308737802959968 ) ) ;
#76130=CARTESIAN_POINT ( 'NONE',  ( 11.00562616383409953, 1432.347154498319924, 151.7431425785430292 ) ) ;
#76132=AXIS2_PLACEMENT_3D ( 'NONE', #102750, #7611, #9819 ) ;
#76137=CARTESIAN_POINT ( 'NONE',  ( -32.79207798990000100, 1453.265480485330045, 262.6648722463980334 ) ) ;
#76139=LINE ( 'NONE', #34130, #7391 ) ;
#76140=CARTESIAN_POINT ( 'NONE',  ( 11.26095182839999964, 1433.846396481040074, 151.5570170780979993 ) ) ;
#76141=CARTESIAN_POINT ( 'NONE',  ( 21.34957048960000137, 1448.971257410079943, 234.3916895488980003 ) ) ;
#76147=CARTESIAN_POINT ( 'NONE',  ( 0.8265242352189998698, 1408.941923249630008, 231.1644247498980178 ) ) ;
#76150=CARTESIAN_POINT ( 'NONE',  ( 26.44407582984479532, 1436.722936376503412, 136.8187510453977325 ) ) ;
#76157=CARTESIAN_POINT ( 'NONE',  ( 0.2052462343486599894, 1460.027118118999852, 182.9519127876829998 ) ) ;
#76159=VERTEX_POINT ( 'NONE', #73865 ) ;
#76160=CARTESIAN_POINT ( 'NONE',  ( -28.38894342380001490, 1444.994950788470987, 176.3316754166978910 ) ) ;
#76161=ADVANCED_FACE ( 'NONE', ( #107993 ), #808, .T. ) ;
#76164=CARTESIAN_POINT ( 'NONE',  ( -39.89055406580479968, 1448.739173191730060, 134.0999999981559938 ) ) ;
#76166=VERTEX_POINT ( 'NONE', #43019 ) ;
#76172=ADVANCED_FACE ( 'NONE', ( #83898 ), #41359, .F. ) ;
#76173=CARTESIAN_POINT ( 'NONE',  ( -14.54584372631119926, 1473.797026299110030, 194.1930890860980128 ) ) ;
#76174=CARTESIAN_POINT ( 'NONE',  ( 22.91749086919999812, 1507.625766668030110, 210.6365783057379701 ) ) ;
#76175=CARTESIAN_POINT ( 'NONE',  ( 7.204667672338278983, 1409.164652926410099, 222.2401956198280004 ) ) ;
#76181=CARTESIAN_POINT ( 'NONE',  ( -32.67729508290000240, 1450.483548884780021, 136.2818069901979925 ) ) ;
#76183=DIRECTION ( 'NONE',  ( 0.000000000000000000, -1.000000000000000000, 0.000000000000000000 ) ) ;
#76184=AXIS2_PLACEMENT_3D ( 'NONE', #95788, #87962, #77346 ) ;
#76186=ORIENTED_EDGE ( 'NONE', *, *, #29537, .T. ) ;
#76194=CARTESIAN_POINT ( 'NONE',  ( 16.16623905053635823, 1432.037924341066628, 218.4554949826395500 ) ) ;
#76198=CARTESIAN_POINT ( 'NONE',  ( 7.713339349770000020, 1475.513060387329915, 228.7257818846979944 ) ) ;
#76202=CARTESIAN_POINT ( 'NONE',  ( 3.148243353760000307, 1447.343022348850127, 154.4222316864979803 ) ) ;
#76204=CARTESIAN_POINT ( 'NONE',  ( 1.546867746950000067, 1416.839692131129823, 190.2222509470979901 ) ) ;
#76205=CARTESIAN_POINT ( 'NONE',  ( 19.85510561680000308, 1471.391771582229921, 270.0615508828979614 ) ) ;
#76208=AXIS2_PLACEMENT_3D ( 'NONE', #75431, #110111, #8737 ) ;
#76212=CARTESIAN_POINT ( 'NONE',  ( -25.41997721759999962, 1449.801887509380094, 207.2020760266680099 ) ) ;
#76213=CARTESIAN_POINT ( 'NONE',  ( -11.44610352279480203, 1425.985488001439990, 130.8067335706190022 ) ) ;
#76214=CARTESIAN_POINT ( 'NONE',  ( 16.42397614938620265, 1410.721834178540121, 191.6524092019909915 ) ) ;
#76217=CARTESIAN_POINT ( 'NONE',  ( 29.01787501698136396, 1510.037283517486912, 201.5082493885905421 ) ) ;
#76218=CARTESIAN_POINT ( 'NONE',  ( 1.424296475967616660, 1450.671211070973186, 181.6313727864856560 ) ) ;
#76224=CARTESIAN_POINT ( 'NONE',  ( -39.53412538496939987, 1440.582317794330038, 136.7849119739890114 ) ) ;
#76226=CARTESIAN_POINT ( 'NONE',  ( 12.64873006253779941, 1397.980667074559733, 213.9846389742999975 ) ) ;
#76229=ORIENTED_EDGE ( 'NONE', *, *, #87858, .T. ) ;
#76230=B_SPLINE_CURVE_WITH_KNOTS ( 'NONE', 3,
 ( #69947, #60991, #104619, #43619, #44737, #36862 ),
 .UNSPECIFIED., .F., .F.,
 ( 4, 2, 4 ),
 ( -0.08571269188183310017, -0.04143665797639420334, -1.438549643295594649E-08 ),
 .UNSPECIFIED. ) ;
#76231=CARTESIAN_POINT ( 'NONE',  ( -29.64937900391915093, 1509.975914221921357, 210.4712216346827915 ) ) ;
#76232=FACE_OUTER_BOUND ( 'NONE', #11936, .T. ) ;
#76237=CARTESIAN_POINT ( 'NONE',  ( 33.91369117179520032, 1435.681798755330192, 134.4205480820800176 ) ) ;
#76242=VERTEX_POINT ( 'NONE', #20544 ) ;
#76246=CARTESIAN_POINT ( 'NONE',  ( 11.08206323080000111, 1414.913528139129994, 222.2042284754980130 ) ) ;
#76249=CARTESIAN_POINT ( 'NONE',  ( -13.88473851270000026, 1415.296882296330068, 220.8066774238980088 ) ) ;
#76254=CARTESIAN_POINT ( 'NONE',  ( -7.720339733105665125, 1446.701196261682981, 154.1134164384996268 ) ) ;
#76258=CARTESIAN_POINT ( 'NONE',  ( -15.73134880039999928, 1485.117178942230112, 224.0171761809980069 ) ) ;
#76261=CARTESIAN_POINT ( 'NONE',  ( 15.13342375178309851, 1507.606285622089899, 226.3974328904010065 ) ) ;
#76264=CARTESIAN_POINT ( 'NONE',  ( -2.499956565898610261, 1419.670774135810007, 129.2260277615939970 ) ) ;
#76265=ORIENTED_EDGE ( 'NONE', *, *, #20160, .T. ) ;
#76266=CARTESIAN_POINT ( 'NONE',  ( -1.290830522935544789, 1486.252651503785501, 181.7990903393099700 ) ) ;
#76269=CARTESIAN_POINT ( 'NONE',  ( -2.991115354478053767, 1485.673002022499531, 182.6499386298461616 ) ) ;
#76272=VERTEX_POINT ( 'NONE', #9955 ) ;
#76273=CARTESIAN_POINT ( 'NONE',  ( 0.5620975284769998970, 1416.851343898729965, 190.4751211474980153 ) ) ;
#76275=B_SPLINE_CURVE_WITH_KNOTS ( 'NONE', 3,
 ( #12758, #19491, #37966, #21679, #105170, #2733, #53694, #81057, #62654, #38501, #96776, #55886, #46390, #72678, #97850 ),
 .UNSPECIFIED., .F., .F.,
 ( 4, 2, 2, 1, 1, 1, 2, 2, 4 ),
 ( 0.000000000000000000, 0.2500000000000007216, 0.3750000000000014433, 0.4375000000000032196, 0.4687500000000054401, 0.4843750000000056066, 0.4921875000000097145, 0.5000000000000137668, 1.000000000000000000 ),
 .UNSPECIFIED. ) ;
#76277=CARTESIAN_POINT ( 'NONE',  ( -10.92384068729999846, 1429.091921970129988, 151.0140743380979984 ) ) ;
#76279=CARTESIAN_POINT ( 'NONE',  ( -7.624682118549999998, 1442.078355704660225, 184.2071361224980137 ) ) ;
#76280=CARTESIAN_POINT ( 'NONE',  ( -28.15442856212169787, 1509.896234822020006, 200.8410265843269826 ) ) ;
#76281=DIRECTION ( 'NONE',  ( 1.000000000000000000, 0.000000000000000000, 0.000000000000000000 ) ) ;
#76282=CARTESIAN_POINT ( 'NONE',  ( 0.2660838379469560033, 1443.814632406239980, 189.5938922378529981 ) ) ;
#76283=CARTESIAN_POINT ( 'NONE',  ( -20.54580208550000009, 1495.372389045430054, 227.4306167334980273 ) ) ;
#76285=CARTESIAN_POINT ( 'NONE',  ( -16.96961820828100187, 1460.580780704285871, 228.2620474942170006 ) ) ;
#76288=CARTESIAN_POINT ( 'NONE',  ( 36.03851880410000064, 1418.520028046229982, 267.9355420903980303 ) ) ;
#76290=CARTESIAN_POINT ( 'NONE',  ( 18.99729322769999840, 1449.733786570959865, 191.9831398968979954 ) ) ;
#76292=CARTESIAN_POINT ( 'NONE',  ( -0.02088553982763170086, 1508.565558233520051, 237.9144398107179939 ) ) ;
#76295=CARTESIAN_POINT ( 'NONE',  ( 15.26419385149999997, 1460.025905744229931, 232.1043486749979934 ) ) ;
#76297=CARTESIAN_POINT ( 'NONE',  ( -13.65702322080000108, 1443.964959164910169, 187.8161327681980026 ) ) ;
#76298=EDGE_CURVE ( 'NONE', #28737, #26609, #59871, .T. ) ;
#76299=CARTESIAN_POINT ( 'NONE',  ( -22.44565107540000071, 1519.913060387329779, 213.3775353178480145 ) ) ;
#76301=CARTESIAN_POINT ( 'NONE',  ( 0.9912867144625557847, 1407.655978792028236, 270.1376065696978799 ) ) ;
#76302=EDGE_CURVE ( 'NONE', #101078, #75505, #25059, .T. ) ;
#76304=CARTESIAN_POINT ( 'NONE',  ( -19.62446893450000118, 1440.913060387330006, 214.3676144200779845 ) ) ;
#76307=DIRECTION ( 'NONE',  ( 1.000000000000000000, 0.000000000000000000, 0.000000000000000000 ) ) ;
#76308=CARTESIAN_POINT ( 'NONE',  ( -9.770742656079999477, 1474.306579240830160, 269.6204776596980537 ) ) ;
#76311=CARTESIAN_POINT ( 'NONE',  ( 17.93928201133349987, 1417.697889326150062, 223.6392055776269956 ) ) ;
#76313=DIRECTION ( 'NONE',  ( 0.03489949670247723124, 0.9993908270190966503, -2.775557561563011889E-14 ) ) ;
#76314=CARTESIAN_POINT ( 'NONE',  ( 11.93592535262039966, 1415.651572961180136, 223.2534673748540115 ) ) ;
#76320=CARTESIAN_POINT ( 'NONE',  ( -22.12837256650000128, 1409.685800185430026, 205.2451141150779677 ) ) ;
#76324=CARTESIAN_POINT ( 'NONE',  ( 1.639582970820000041, 1434.541746329560056, 150.4377894671980016 ) ) ;
#76328=CARTESIAN_POINT ( 'NONE',  ( -21.62710251429999886, 1409.668295441930013, 211.5114173564280122 ) ) ;
#76330=CARTESIAN_POINT ( 'NONE',  ( 11.72797607332480041, 1426.701692393189887, 143.5212822355949811 ) ) ;
#76334=CARTESIAN_POINT ( 'NONE',  ( -2.500000000000000000, 1439.615672362369878, 128.3512065685980019 ) ) ;
#76337=CARTESIAN_POINT ( 'NONE',  ( -11.74015320060000001, 1428.979986575930070, 144.1938086916980239 ) ) ;
#76340=CARTESIAN_POINT ( 'NONE',  ( 1.874390728800000128, 1508.748819628430056, 237.3943831762979926 ) ) ;
#76341=ADVANCED_FACE ( 'NONE', ( #79380 ), #26707, .F. ) ;
#76342=CARTESIAN_POINT ( 'NONE',  ( 21.26194160363760233, 1509.381988423189796, 228.0863887365900098 ) ) ;
#76346=ORIENTED_EDGE ( 'NONE', *, *, #98178, .T. ) ;
#76347=CARTESIAN_POINT ( 'NONE',  ( 11.45376624174839897, 1434.341927546149918, 151.4236503405790017 ) ) ;
#76348=CARTESIAN_POINT ( 'NONE',  ( -12.72899733799999922, 1397.389012456630098, 211.4694218863679964 ) ) ;
#76353=CARTESIAN_POINT ( 'NONE',  ( 16.06955848517850072, 1424.062620710240026, 191.1090677130400195 ) ) ;
#76354=CARTESIAN_POINT ( 'NONE',  ( -14.13384278227159818, 1509.281245845819967, 183.3826977356570183 ) ) ;
#76356=CARTESIAN_POINT ( 'NONE',  ( 17.31741470348719858, 1498.111796630450044, 230.4563530528860156 ) ) ;
#76357=CARTESIAN_POINT ( 'NONE',  ( 1.530673255310000203, 1429.773503041730009, 184.4796783900980301 ) ) ;
#76358=CARTESIAN_POINT ( 'NONE',  ( -2.676551809669999837, 1415.087818611729972, 192.3610496020979781 ) ) ;
#76359=CARTESIAN_POINT ( 'NONE',  ( 42.54900162989899570, 1440.913053717579942, 270.0692078703979746 ) ) ;
#76360=CARTESIAN_POINT ( 'NONE',  ( 0.9175745326867349450, 1395.945102796070159, 198.1514473720520186 ) ) ;
#76361=CARTESIAN_POINT ( 'NONE',  ( 0.1681681984989999989, 1420.473120458229914, 179.3023655596979893 ) ) ;
#76362=CARTESIAN_POINT ( 'NONE',  ( 11.86318670040000001, 1432.127862331690039, 150.3942814104979959 ) ) ;
#76365=CARTESIAN_POINT ( 'NONE',  ( 13.52173958309080071, 1435.750944454330011, 150.3327472168750205 ) ) ;
#76366=EDGE_LOOP ( 'NONE', ( #19342, #110754, #421, #3961 ) ) ;
#76368=CARTESIAN_POINT ( 'NONE',  ( 13.21106958178233270, 1444.696289312639465, 169.3897206396751756 ) ) ;
#76369=CARTESIAN_POINT ( 'NONE',  ( -9.313356613159999853, 1463.019685538429940, 234.3550464167980181 ) ) ;
#76370=CARTESIAN_POINT ( 'NONE',  ( -8.168076443215248617, 1407.240959200780026, 219.8347814960359869 ) ) ;
#76371=CIRCLE ( 'NONE', #37036, 9.000000000000007105 ) ;
#76375=CARTESIAN_POINT ( 'NONE',  ( 2.500000000000000000, 1448.210397838020072, 167.6163145387380098 ) ) ;
#76377=ORIENTED_EDGE ( 'NONE', *, *, #11122, .F. ) ;
#76381=CARTESIAN_POINT ( 'NONE',  ( -18.63864992400000276, 1509.044553702130088, 230.2784244607980213 ) ) ;
#76382=CARTESIAN_POINT ( 'NONE',  ( -6.931887347990000059, 1409.155127227530102, 188.8914258914980167 ) ) ;
#76386=CARTESIAN_POINT ( 'NONE',  ( 23.70375358549999945, 1434.825524415949985, 215.3081005562079895 ) ) ;
#76387=CARTESIAN_POINT ( 'NONE',  ( 11.86716023049999968, 1432.353341358199941, 147.6509521729980179 ) ) ;
#76393=CARTESIAN_POINT ( 'NONE',  ( 24.02347886858969872, 1410.714002848892278, 209.6150515799677976 ) ) ;
#76397=CARTESIAN_POINT ( 'NONE',  ( 13.86092958890000126, 1410.765486798930169, 191.1266625105979813 ) ) ;
#76398=CARTESIAN_POINT ( 'NONE',  ( 2.461132262735347798, 1421.750034555250522, 139.1420193590112717 ) ) ;
#76402=CARTESIAN_POINT ( 'NONE',  ( 1.052045010949999979E-09, 1470.400767512030143, 255.2684314988979963 ) ) ;
#76409=CARTESIAN_POINT ( 'NONE',  ( 16.96418136024609780, 1409.508820805990126, 222.1821933189740150 ) ) ;
#76413=ORIENTED_EDGE ( 'NONE', *, *, #101536, .F. ) ;
#76416=CARTESIAN_POINT ( 'NONE',  ( 14.80435908759999997, 1474.026124292930035, 223.3946435410979916 ) ) ;
#76417=CIRCLE ( 'NONE', #6637, 2.028272653252106927 ) ;
#76421=CARTESIAN_POINT ( 'NONE',  ( 25.99184421905080811, 1450.775692673193362, 136.7467824686237918 ) ) ;
#76422=CARTESIAN_POINT ( 'NONE',  ( 15.49277546151340879, 1420.928748437756440, 227.7039097393026452 ) ) ;
#76423=CARTESIAN_POINT ( 'NONE',  ( 32.02224580989319946, 1436.511321034889988, 136.5688601130949849 ) ) ;
#76424=SPHERICAL_SURFACE ( 'NONE', #18092, 2.000000000000000000 ) ;
#76428=CARTESIAN_POINT ( 'NONE',  ( 14.69816566019999904, 1509.426331642330069, 184.0211180668979978 ) ) ;
#76433=CARTESIAN_POINT ( 'NONE',  ( -35.99825504957585309, 1419.870133879962850, 269.2276119577702502 ) ) ;
#76435=CARTESIAN_POINT ( 'NONE',  ( 15.97551097353819927, 1477.212431653470048, 189.0465089897220139 ) ) ;
#76436=CARTESIAN_POINT ( 'NONE',  ( -2.710264235259999877E-09, 1476.076643212929866, 267.5371647992980115 ) ) ;
#76438=AXIS2_PLACEMENT_3D ( 'NONE', #91983, #49449, #40478 ) ;
#76439=CARTESIAN_POINT ( 'NONE',  ( -28.29412264859999837, 1508.657108475729956, 208.9834593761570147 ) ) ;
#76443=CARTESIAN_POINT ( 'NONE',  ( -6.982994490885238825, 1451.423926582423519, 153.2281128498337637 ) ) ;
#76445=CARTESIAN_POINT ( 'NONE',  ( -18.16418870590820234, 1416.835419214280137, 209.0763567938479923 ) ) ;
#76446=CARTESIAN_POINT ( 'NONE',  ( 25.87190634410000101, 1436.506016957939892, 136.9687052083980063 ) ) ;
#76447=CARTESIAN_POINT ( 'NONE',  ( -7.872426330613159884, 1396.187971572860079, 201.3681491859670132 ) ) ;
#76448=ORIENTED_EDGE ( 'NONE', *, *, #93835, .F. ) ;
#76449=CARTESIAN_POINT ( 'NONE',  ( -0.05448001189851819914, 1416.221314539589912, 191.0976842799670123 ) ) ;
#76450=CARTESIAN_POINT ( 'NONE',  ( 21.18003081007569932, 1508.593876612841086, 226.2067732376109177 ) ) ;
#76452=EDGE_LOOP ( 'NONE', ( #86279, #103633 ) ) ;
#76453=ORIENTED_EDGE ( 'NONE', *, *, #92607, .F. ) ;
#76457=CARTESIAN_POINT ( 'NONE',  ( -22.42801321349999810, 1448.695731516339947, 212.0101260109479995 ) ) ;
#76459=CARTESIAN_POINT ( 'NONE',  ( -11.87550762409999905, 1433.043840478560242, 149.9802072585979715 ) ) ;
#76462=CARTESIAN_POINT ( 'NONE',  ( -2.749484708945287181, 1420.045225311068180, 186.0761315375977176 ) ) ;
#76464=CARTESIAN_POINT ( 'NONE',  ( -24.42787553970000047, 1439.418188418060026, 210.9954768190879975 ) ) ;
#76465=B_SPLINE_CURVE_WITH_KNOTS ( 'NONE', 3,
 ( #627, #86817, #86260, #103619, #102498, #10109, #77327, #44281, #67833, #34207, #103046, #25787, #17374, #26344, #42066, #101943, #78425, #9549, #60541, #25232, #51572, #59435, #76, #1180, #52132, #34758, #43719, #35311, #85154, #85706, #94662, #9001, #43174, #76217, #69497, #42613, #110362, #68946, #26917, #61107, #93546, #17934, #95222, #16819, #18484, #51020, #76766, #68391, #76016, #67092, #59241, #49184, #109086, #74937, #101751, #15534, #31255, #57589, #65996, #92263, #7704, #91713 ),
 .UNSPECIFIED., .F., .F.,
 ( 4, 2, 2, 2, 2, 2, 1, 1, 1, 1, 1, 2, 2, 2, 2, 2, 2, 2, 1, 1, 1, 2, 2, 2, 2, 2, 2, 1, 1, 1, 1, 2, 2, 2, 2, 2, 4 ),
 ( 0.000000000000000000, 0.06250000000010860757, 0.1250000000002172151, 0.1875000000003258227, 0.2187500000003799461, 0.2343750000004068135, 0.2421875000004203027, 0.2460937500004272693, 0.2480468750004305167, 0.2490234375004321821, 0.2495117187504330147, 0.2497558593754329592, 0.2500000000004328760, 0.3125000000004529155, 0.3750000000004730105, 0.4375000000004930500, 0.4687500000005025980, 0.4843750000005078160, 0.4921875000005098144, 0.4960937500005103695, 0.4980468750005100365, 0.4990234375005098699, 0.5000000000005097034, 0.6250000000003840261, 0.6875000000003212985, 0.7187500000002903233, 0.7343750000002747802, 0.7421875000002672307, 0.7460937500002634559, 0.7480468750002610134, 0.7490234375002594591, 0.7495117187502580158, 0.7500000000002566836, 0.8125000000001925127, 0.8750000000001283418, 0.9375000000000642819, 1.000000000000000000 ),
 .UNSPECIFIED. ) ;
#76467=CARTESIAN_POINT ( 'NONE',  ( 2.146415212520000004, 1450.119370040659760, 182.3300074786979792 ) ) ;
#76469=CARTESIAN_POINT ( 'NONE',  ( -30.16373308232411787, 1510.076423030737942, 210.1342399186210628 ) ) ;
#76470=CARTESIAN_POINT ( 'NONE',  ( -2.797080001758770053E-09, 1414.990986343060058, 244.4381637399740157 ) ) ;
#76471=ORIENTED_EDGE ( 'NONE', *, *, #67080, .F. ) ;
#76472=ORIENTED_EDGE ( 'NONE', *, *, #18796, .T. ) ;
#76473=CARTESIAN_POINT ( 'NONE',  ( -11.83258938619150058, 1430.066262795869989, 149.4976403726300305 ) ) ;
#76481=CARTESIAN_POINT ( 'NONE',  ( -17.42808535260000014, 1431.113060387329824, 201.5089395310880036 ) ) ;
#76484=CARTESIAN_POINT ( 'NONE',  ( -10.63393819740299939, 1406.766374306999978, 267.1884441437949818 ) ) ;
#76485=CARTESIAN_POINT ( 'NONE',  ( -14.32024519749940161, 1436.001929727169909, 149.9627363249020107 ) ) ;
#76488=CARTESIAN_POINT ( 'NONE',  ( 13.24110963769999927, 1443.105933592210022, 187.8974491670979887 ) ) ;
#76489=ORIENTED_EDGE ( 'NONE', *, *, #36038, .F. ) ;
#76490=VECTOR ( 'NONE', #48920, 1000.000000000000000 ) ;
#76493=DIRECTION ( 'NONE',  ( -0.7071067657658171024, -0.01693754150844739917, 0.7069039124915460492 ) ) ;
#76496=CIRCLE ( 'NONE', #12152, 2.000000000000000000 ) ;
#76497=CARTESIAN_POINT ( 'NONE',  ( -17.02086975159189919, 1479.748893642479970, 228.8538236634169891 ) ) ;
#76498=ORIENTED_EDGE ( 'NONE', *, *, #48415, .F. ) ;
#76502=CARTESIAN_POINT ( 'NONE',  ( -27.26565262369999942, 1508.025370090229899, 204.2545478268079933 ) ) ;
#76503=CARTESIAN_POINT ( 'NONE',  ( -1.523967229539999746, 1477.816987455330036, 230.7230646392980020 ) ) ;
#76505=CARTESIAN_POINT ( 'NONE',  ( -2.589228330169999648, 1407.329175972530265, 196.2821412641980316 ) ) ;
#76508=CARTESIAN_POINT ( 'NONE',  ( -25.47454973720070370, 1449.924923776209880, 210.2506139651870001 ) ) ;
#76509=CARTESIAN_POINT ( 'NONE',  ( 26.53588231950000065, 1469.248395150029864, 209.7046586876050185 ) ) ;
#76512=CARTESIAN_POINT ( 'NONE',  ( -24.74905961449999836, 1435.859003228780239, 137.6504519889980145 ) ) ;
#76513=CIRCLE ( 'NONE', #28245, 4079.102317997178943 ) ;
#76516=CARTESIAN_POINT ( 'NONE',  ( -14.95253593330000008, 1415.584822001330167, 226.8728895648979744 ) ) ;
#76518=( BOUNDED_CURVE ( )  B_SPLINE_CURVE ( 3, ( #95010, #62553, #96673, #95559 ),
 .UNSPECIFIED., .F., .F. ) 
 B_SPLINE_CURVE_WITH_KNOTS ( ( 4, 4 ),
 ( 4.177898496273999562, 5.246908467225170014 ),
 .UNSPECIFIED. ) 
 CURVE ( )  GEOMETRIC_REPRESENTATION_ITEM ( )  RATIONAL_B_SPLINE_CURVE ( ( 1.000000000000000000, 0.9070139350561767788, 0.9070139350561767788, 1.000000000000000000 ) ) 
 REPRESENTATION_ITEM ( '' )  );
#76521=CARTESIAN_POINT ( 'NONE',  ( -2.587453686403140107, 1451.957470480449956, 184.6860871491240061 ) ) ;
#76522=CARTESIAN_POINT ( 'NONE',  ( -12.81728032640000059, 1415.366301205729997, 228.1481425647979790 ) ) ;
#76525=DIRECTION ( 'NONE',  ( 0.6677681214262592979, -0.7443693545591762994, 0.000000000000000000 ) ) ;
#76527=CARTESIAN_POINT ( 'NONE',  ( 12.75105367887320007, 1435.273936497249906, 150.5906040834139787 ) ) ;
#76528=CARTESIAN_POINT ( 'NONE',  ( -4.119144758445948185, 1441.439880715936170, 184.2549068806088712 ) ) ;
#76533=CARTESIAN_POINT ( 'NONE',  ( 4.221427320000399774, 1441.605329825029912, 168.6675303822389935 ) ) ;
#76539=ORIENTED_EDGE ( 'NONE', *, *, #14782, .F. ) ;
#76540=CARTESIAN_POINT ( 'NONE',  ( -12.45642918560000112, 1416.822692809430009, 194.7673859448979954 ) ) ;
#76543=CARTESIAN_POINT ( 'NONE',  ( 1.308044573769999941, 1420.880219163630045, 182.9927263326979983 ) ) ;
#76549=CARTESIAN_POINT ( 'NONE',  ( 17.21543977323896613, 1422.420158212175465, 226.7018114670726447 ) ) ;
#76550=CARTESIAN_POINT ( 'NONE',  ( 18.11449771340117820, 1507.710592339239383, 230.4427339259977998 ) ) ;
#76552=CARTESIAN_POINT ( 'NONE',  ( -2.493947715939999643, 1442.756953654919926, 150.6345094620980092 ) ) ;
#76553=CARTESIAN_POINT ( 'NONE',  ( 45.41371203904640197, 1440.913060377029979, 265.9156451615399988 ) ) ;
#76557=VERTEX_POINT ( 'NONE', #22188 ) ;
#76561=CARTESIAN_POINT ( 'NONE',  ( -10.26697147908009811, 1506.473665945047060, 228.6001773789730862 ) ) ;
#76562=CARTESIAN_POINT ( 'NONE',  ( -27.78452750869999832, 1508.000976251930069, 210.4681927209580010 ) ) ;
#76565=CARTESIAN_POINT ( 'NONE',  ( -3.897008745070269509, 1426.015660802909224, 186.0506595318446728 ) ) ;
#76569=CARTESIAN_POINT ( 'NONE',  ( 13.31050689230000117, 1414.983771850430003, 197.8499836737979933 ) ) ;
#76571=ADVANCED_FACE ( 'NONE', ( #40116 ), #103606, .F. ) ;
#76573=CARTESIAN_POINT ( 'NONE',  ( 16.43064545349999861, 1451.907610170929729, 148.9104844442979925 ) ) ;
#76574=CARTESIAN_POINT ( 'NONE',  ( -27.36889314738404977, 1509.257027982647969, 212.0753268043458775 ) ) ;
#76576=CARTESIAN_POINT ( 'NONE',  ( 23.71809045669999705, 1508.481479934130220, 195.1786701157980133 ) ) ;
#76577=ORIENTED_EDGE ( 'NONE', *, *, #93250, .F. ) ;
#76578=VECTOR ( 'NONE', #61095, 1000.000000000000000 ) ;
#76584=ORIENTED_EDGE ( 'NONE', *, *, #53184, .F. ) ;
#76587=CARTESIAN_POINT ( 'NONE',  ( 38.97238355074230043, 1439.678263993750079, 136.6980159596599833 ) ) ;
#76593=CARTESIAN_POINT ( 'NONE',  ( -11.56020812217769489, 1434.913448849900533, 151.4031740279024802 ) ) ;
#76595=CIRCLE ( 'NONE', #21169, 7.016581249619902039 ) ;
#76596=CARTESIAN_POINT ( 'NONE',  ( 4.970581720019999317, 1409.086636925830135, 187.4197542652979962 ) ) ;
#76599=CARTESIAN_POINT ( 'NONE',  ( -3.697587031422459702, 1440.988254563350210, 157.0261807637750167 ) ) ;
#76600=CARTESIAN_POINT ( 'NONE',  ( -21.40326933649999575, 1452.165641750530085, 142.6046343431980006 ) ) ;
#76601=CARTESIAN_POINT ( 'NONE',  ( 0.9755134735189999740, 1466.582224391130012, 235.3782024704980245 ) ) ;
#76602=ORIENTED_EDGE ( 'NONE', *, *, #54960, .T. ) ;
#76609=CARTESIAN_POINT ( 'NONE',  ( -2.295465748574410035E-11, 1470.383016079100116, 255.0304770405179511 ) ) ;
#76611=CARTESIAN_POINT ( 'NONE',  ( -1.552659050370000182, 1415.628674276829770, 227.5866819053980237 ) ) ;
#76612=CARTESIAN_POINT ( 'NONE',  ( -3.037920316420000155, 1417.285933716130103, 233.5158617220979806 ) ) ;
#76615=CARTESIAN_POINT ( 'NONE',  ( -0.3887204637380738403, 1485.756074821177890, 181.8627589278759729 ) ) ;
#76617=CARTESIAN_POINT ( 'NONE',  ( -45.91620460975560292, 1438.463282072589891, 268.4996293049820224 ) ) ;
#76618=CARTESIAN_POINT ( 'NONE',  ( 13.85848044686079916, 1509.281222645870002, 234.2549437311519966 ) ) ;
#76622=CARTESIAN_POINT ( 'NONE',  ( -5.429844217520000349, 1436.698278606120084, 154.7014901950980175 ) ) ;
#76625=CARTESIAN_POINT ( 'NONE',  ( -25.77240273999639797, 1452.013063856540157, 135.1833753210919724 ) ) ;
#76627=CARTESIAN_POINT ( 'NONE',  ( 18.32607164059999860, 1423.244042729530065, 231.9815855802980025 ) ) ;
#76629=CARTESIAN_POINT ( 'NONE',  ( 14.54643167989999952, 1470.812340170230073, 194.6419432318980114 ) ) ;
#76635=ORIENTED_EDGE ( 'NONE', *, *, #40496, .F. ) ;
#76636=CARTESIAN_POINT ( 'NONE',  ( -6.685506928249539627, 1409.565136544780216, 270.3700927272910235 ) ) ;
#76637=CARTESIAN_POINT ( 'NONE',  ( 8.813846681050000242, 1418.026211838229756, 230.6754341397980284 ) ) ;
#76641=CARTESIAN_POINT ( 'NONE',  ( -23.50732105891940193, 1410.149254099409973, 209.9394804832799935 ) ) ;
#76645=FACE_OUTER_BOUND ( 'NONE', #44613, .T. ) ;
#76647=CARTESIAN_POINT ( 'NONE',  ( -20.57476409830681874, 1436.447616954657860, 144.8090829293095680 ) ) ;
#76650=CARTESIAN_POINT ( 'NONE',  ( 35.58359713094720433, 1463.005569991589709, 268.8138335405850512 ) ) ;
#76655=ORIENTED_EDGE ( 'NONE', *, *, #40020, .F. ) ;
#76656=CARTESIAN_POINT ( 'NONE',  ( 18.22805055419890152, 1459.311389626190021, 227.8763770136359881 ) ) ;
#76659=EDGE_LOOP ( 'NONE', ( #93704, #71697, #13998, #62356, #89847 ) ) ;
#76660=CARTESIAN_POINT ( 'NONE',  ( 2.500000005550000015, 1448.575512279979876, 182.8814919026980021 ) ) ;
#76661=EDGE_CURVE ( 'NONE', #12048, #93687, #39221, .T. ) ;
#76662=CARTESIAN_POINT ( 'NONE',  ( 27.02609346130070023, 1451.901655341519927, 135.4159119962619968 ) ) ;
#76663=EDGE_CURVE ( 'NONE', #70222, #60117, #106076, .T. ) ;
#76668=CARTESIAN_POINT ( 'NONE',  ( 27.23063139319997816, 1443.913060387329097, 161.8596747266978753 ) ) ;
#76669=CARTESIAN_POINT ( 'NONE',  ( 4.180008225707200431, 1409.059029491030060, 187.6061561084030131 ) ) ;
#76670=CARTESIAN_POINT ( 'NONE',  ( 2.446918720040000217, 1417.581962241529936, 234.9465420055979905 ) ) ;
#76674=CARTESIAN_POINT ( 'NONE',  ( 15.29896286170615305, 1422.370102515510780, 230.0239554351165907 ) ) ;
#76677=CARTESIAN_POINT ( 'NONE',  ( 11.86607448679350085, 1432.335963006760039, 150.0622438253739972 ) ) ;
#76681=EDGE_CURVE ( 'NONE', #65089, #74815, #100710, .T. ) ;
#76684=CARTESIAN_POINT ( 'NONE',  ( -42.15865170690000241, 1450.809155637750109, 271.1218459616979999 ) ) ;
#76686=CARTESIAN_POINT ( 'NONE',  ( 11.49921796000000107, 1433.639916894349881, 151.2944310539980108 ) ) ;
#76687=CARTESIAN_POINT ( 'NONE',  ( 23.42675388089999799, 1443.575607730780121, 234.3916895488980003 ) ) ;
#76689=ADVANCED_FACE ( 'NONE', ( #108702 ), #99733, .T. ) ;
#76690=CARTESIAN_POINT ( 'NONE',  ( 0.5992832621693802153, 1467.074120444730170, 235.5491957431187586 ) ) ;
#76692=CARTESIAN_POINT ( 'NONE',  ( -14.49383181622579997, 1422.099016211560183, 229.4564907068830166 ) ) ;
#76693=CARTESIAN_POINT ( 'NONE',  ( 12.86122366611430046, 1416.830086716310007, 221.8629622564060071 ) ) ;
#76694=PLANE ( 'NONE',  #23425 ) ;
#76695=CARTESIAN_POINT ( 'NONE',  ( -25.85060555058009868, 1509.854941346010037, 193.0608776564500317 ) ) ;
#76697=FACE_OUTER_BOUND ( 'NONE', #28035, .T. ) ;
#76698=CARTESIAN_POINT ( 'NONE',  ( -41.66768200349253704, 1443.241368483788392, 135.6286826123361777 ) ) ;
#76701=CARTESIAN_POINT ( 'NONE',  ( -11.04413905111285565, 1433.699474062253785, 151.7296044286115944 ) ) ;
#76705=CARTESIAN_POINT ( 'NONE',  ( 0.1715556276115110246, 1479.416462729990144, 182.1194568275189738 ) ) ;
#76706=CARTESIAN_POINT ( 'NONE',  ( -7.491155460717596526, 1414.913060387329779, 194.4095434935337039 ) ) ;
#76709=AXIS2_PLACEMENT_3D ( 'NONE', #73046, #44688, #55712 ) ;
#76710=CARTESIAN_POINT ( 'NONE',  ( -5.389719915088219793, 1440.971386074470047, 154.8246291213590098 ) ) ;
#76711=LINE ( 'NONE', #68896, #46135 ) ;
#76712=EDGE_CURVE ( 'NONE', #75505, #46627, #53739, .T. ) ;
#76713=CARTESIAN_POINT ( 'NONE',  ( -39.34220581718710008, 1449.349331648840234, 134.0999999980729740 ) ) ;
#76719=CARTESIAN_POINT ( 'NONE',  ( -16.30669498860000033, 1415.087745006229852, 214.1831677707580184 ) ) ;
#76722=CARTESIAN_POINT ( 'NONE',  ( -14.03642065347150236, 1457.296397347949778, 194.7061520102889745 ) ) ;
#76723=CARTESIAN_POINT ( 'NONE',  ( -28.25086642335310216, 1508.135711581739997, 208.8579954535609886 ) ) ;
#76727=CARTESIAN_POINT ( 'NONE',  ( 13.15726445491959851, 1416.851343895820037, 196.3340833728059920 ) ) ;
#76730=AXIS2_PLACEMENT_3D ( 'NONE', #32481, #31914, #94023 ) ;
#76731=CARTESIAN_POINT ( 'NONE',  ( -32.69005726390000177, 1451.771678911430172, 135.1859641189979868 ) ) ;
#76732=B_SPLINE_CURVE_WITH_KNOTS ( 'NONE', 5,
 ( #92815, #58681, #94454, #34011, #77679, #86075 ),
 .UNSPECIFIED., .F., .F.,
 ( 6, 6 ),
 ( -93.45893461050000894, -23.20786975740000457 ),
 .UNSPECIFIED. ) ;
#76733=CARTESIAN_POINT ( 'NONE',  ( 16.90742463042001376, 1442.831169986190844, 162.4348201727408991 ) ) ;
#76737=AXIS2_PLACEMENT_3D ( 'NONE', #107575, #30861, #105946 ) ;
#76738=CARTESIAN_POINT ( 'NONE',  ( 26.80001153169999739, 1509.848937414829834, 219.2969692978980163 ) ) ;
#76741=CARTESIAN_POINT ( 'NONE',  ( 40.12840166341722181, 1450.023108907809046, 269.6125932357766146 ) ) ;
#76742=CARTESIAN_POINT ( 'NONE',  ( 13.04207810306199988, 1409.368499790489750, 192.3005055522939983 ) ) ;
#76743=CARTESIAN_POINT ( 'NONE',  ( 5.492330840890000232, 1396.104856806630096, 219.0480561951579830 ) ) ;
#76744=CARTESIAN_POINT ( 'NONE',  ( 1.797565579259999824, 1415.903556500329842, 232.4419632410979943 ) ) ;
#76746=CARTESIAN_POINT ( 'NONE',  ( -22.14848735670008395, 1507.850285361328133, 225.9298081188978813 ) ) ;
#76749=ADVANCED_FACE ( 'NONE', ( #75666 ), #61627, .F. ) ;
#76752=CARTESIAN_POINT ( 'NONE',  ( 3.692944191490000083, 1446.771171062450094, 157.7765864143980252 ) ) ;
#76753=ADVANCED_FACE ( 'NONE', ( #34196 ), #80444, .F. ) ;
#76754=B_SPLINE_SURFACE_WITH_KNOTS ( 'NONE', 5, 5, ( 
 ( #48857, #23621, #49392, #65649, #32586, #15201, #83520, #84077, #67855 ),
 ( #110384, #99765, #57805, #91929, #24152, #49939, #108176, #5738, #84622 ),
 ( #39880, #23055, #82982, #74047, #58342, #33119, #31468, #66761, #82440 ),
 ( #109842, #100862, #57264, #6273, #91391, #7918, #109300, #67307, #40423 ),
 ( #42088, #14669, #74599, #101403, #92467, #24695, #108735, #6814, #76237 ),
 ( #32026, #58891, #93024, #16296, #15738, #7375, #90826, #41539, #66215 ) ),
 .UNSPECIFIED., .F., .F., .F.,
 ( 6, 6 ),
 ( 6, 3, 6 ),
 ( 40.37450813634060154, 42.94666622520000487 ),
 ( 0.000000000000000000, 8.028376882759999944, 16.05675376549999811 ),
 .UNSPECIFIED. ) ;
#76755=CARTESIAN_POINT ( 'NONE',  ( -2.500000000000000000, 1432.496417326090068, 157.4993228830980172 ) ) ;
#76759=CARTESIAN_POINT ( 'NONE',  ( -18.64672481365220236, 1416.851343896850040, 208.5597484336410048 ) ) ;
#76760=VERTEX_POINT ( 'NONE', #85694 ) ;
#76761=CARTESIAN_POINT ( 'NONE',  ( 4.363122647529283249, 1409.354802298928007, 137.0999999980979851 ) ) ;
#76762=CARTESIAN_POINT ( 'NONE',  ( -23.54254250629999845, 1430.351957812429873, 203.7587613919580178 ) ) ;
#76763=CARTESIAN_POINT ( 'NONE',  ( -11.30526943965280040, 1426.459633991370083, 113.0055148446249973 ) ) ;
#76764=CARTESIAN_POINT ( 'NONE',  ( 17.06148083016629968, 1410.141651639420161, 192.3522963160290260 ) ) ;
#76766=CARTESIAN_POINT ( 'NONE',  ( 27.81444809721715927, 1509.996208870221835, 220.3660356682784141 ) ) ;
#76767=CARTESIAN_POINT ( 'NONE',  ( 1.327771434284243934, 1450.718180199849940, 181.5841407004881773 ) ) ;
#76769=CARTESIAN_POINT ( 'NONE',  ( 16.68893861061719974, 1509.501544872269960, 233.4110457454409868 ) ) ;
#76770=CARTESIAN_POINT ( 'NONE',  ( 15.08870150073219207, 1461.900455706623006, 229.9510696313039091 ) ) ;
#76774=CARTESIAN_POINT ( 'NONE',  ( 7.810568386166560018, 1396.185811445500121, 217.7799683602849825 ) ) ;
#76776=CARTESIAN_POINT ( 'NONE',  ( -18.24693087420000381, 1457.532738398730089, 228.9631694535979989 ) ) ;
#76780=DIRECTION ( 'NONE',  ( -0.6081597637245996779, 0.7938146520356244018, 0.000000000000000000 ) ) ;
#76785=VECTOR ( 'NONE', #21823, 1000.000000000000114 ) ;
#76786=CARTESIAN_POINT ( 'NONE',  ( 0.4794255386045085388, 1547.913060387330006, 209.9994285235883922 ) ) ;
#76787=CARTESIAN_POINT ( 'NONE',  ( 26.86204993032690069, 1508.007394616730153, 206.2315948942269870 ) ) ;
#76788=CARTESIAN_POINT ( 'NONE',  ( 3.783303485079999806, 1421.764240203399822, 183.6423304018649958 ) ) ;
#76789=ADVANCED_FACE ( 'NONE', ( #97411 ), #72239, .F. ) ;
#76797=CARTESIAN_POINT ( 'NONE',  ( 11.78922831828120010, 1427.761296424969942, 147.5992861727949901 ) ) ;
#76800=CARTESIAN_POINT ( 'NONE',  ( 20.51182933999999847, 1507.864840975229981, 228.4145674124980303 ) ) ;
#76802=CARTESIAN_POINT ( 'NONE',  ( -13.57674101270000122, 1415.245980409529921, 221.0231452625980069 ) ) ;
#76803=CARTESIAN_POINT ( 'NONE',  ( -17.11746647137171706, 1443.086052842848176, 162.7559337440806644 ) ) ;
#76806=CARTESIAN_POINT ( 'NONE',  ( -6.719886790419999478, 1423.239095099330143, 186.8024023444980060 ) ) ;
#76812=CARTESIAN_POINT ( 'NONE',  ( 22.73961117905130180, 1415.546519254560053, 206.2005574400780006 ) ) ;
#76813=EDGE_CURVE ( 'NONE', #59275, #101745, #66035, .T. ) ;
#76816=CARTESIAN_POINT ( 'NONE',  ( -4.654161102448804321, 1423.691786733173558, 184.4582529657765235 ) ) ;
#76817=CARTESIAN_POINT ( 'NONE',  ( -5.800581839631719916, 1423.415691768110037, 91.00909034883800075 ) ) ;
#76818=ORIENTED_EDGE ( 'NONE', *, *, #41280, .F. ) ;
#76820=ADVANCED_FACE ( 'NONE', ( #12849 ), #29109, .F. ) ;
#76821=CARTESIAN_POINT ( 'NONE',  ( 18.30039643192660037, 1424.506794127079957, 223.6085225123430007 ) ) ;
#76823=CARTESIAN_POINT ( 'NONE',  ( -2.904196725509198718, 1484.572852589933518, 183.2790564706236580 ) ) ;
#76824=CARTESIAN_POINT ( 'NONE',  ( 5.895408526091680201, 1407.650947103020144, 270.1377427648220078 ) ) ;
#76825=EDGE_CURVE ( 'NONE', #105791, #37255, #18006, .T. ) ;
#76827=VERTEX_POINT ( 'NONE', #71144 ) ;
#76828=CARTESIAN_POINT ( 'NONE',  ( 1.520093416789999985, 1489.468502498129965, 187.0056096891980246 ) ) ;
#76831=CARTESIAN_POINT ( 'NONE',  ( -10.85481319969999880, 1425.430217766629994, 147.2777488329979860 ) ) ;
#76832=DIRECTION ( 'NONE',  ( 0.000000000000000000, 1.000000000000000000, 0.000000000000000000 ) ) ;
#76838=CARTESIAN_POINT ( 'NONE',  ( 5.826988351930000753, 1410.392867642730153, 231.1209932769980071 ) ) ;
#76839=CARTESIAN_POINT ( 'NONE',  ( -19.67423585419999910, 1495.375718038329978, 228.6692629309980020 ) ) ;
#76841=CARTESIAN_POINT ( 'NONE',  ( -16.13435506578399981, 1459.076926233949962, 230.3615790949820052 ) ) ;
#76845=CARTESIAN_POINT ( 'NONE',  ( 31.74787428599999828, 1415.252022282229973, 268.0541964391980514 ) ) ;
#76846=B_SPLINE_CURVE_WITH_KNOTS ( 'NONE', 3,
 ( #85199, #41565, #16322, #32608 ),
 .UNSPECIFIED., .F., .F.,
 ( 4, 4 ),
 ( 0.000000000000000000, 0.03289823588023810252 ),
 .UNSPECIFIED. ) ;
#76849=CARTESIAN_POINT ( 'NONE',  ( 21.79136847569999702, 1469.153666633229932, 195.1686735108980031 ) ) ;
#76850=CARTESIAN_POINT ( 'NONE',  ( 0.3821805048270000005, 1506.433683729329914, 231.1012307613979999 ) ) ;
#76852=CARTESIAN_POINT ( 'NONE',  ( -1.321099038869999909, 1450.950434108429818, 183.2266072565980153 ) ) ;
#76856=CARTESIAN_POINT ( 'NONE',  ( -13.20913601900000067, 1444.817643627899997, 187.1579182788979949 ) ) ;
#76859=CARTESIAN_POINT ( 'NONE',  ( 20.94370973160000204, 1411.258104562529979, 270.0430967323979417 ) ) ;
#76862=CARTESIAN_POINT ( 'NONE',  ( -13.20657463812640131, 1409.374244136060270, 216.1033536567719864 ) ) ;
#76865=CARTESIAN_POINT ( 'NONE',  ( -23.72448802369999754, 1471.157921940630104, 268.2433403273980161 ) ) ;
#76868=CARTESIAN_POINT ( 'NONE',  ( -24.33598933562576150, 1444.630201432154536, 211.2345754049932509 ) ) ;
#76871=CARTESIAN_POINT ( 'NONE',  ( 11.94034776663059993, 1415.658863692289970, 223.2578065737770032 ) ) ;
#76873=B_SPLINE_SURFACE_WITH_KNOTS ( 'NONE', 5, 5, ( 
 ( #95181, #68903, #17888, #43677, #18437, #35268, #43128, #52087, #110317 ),
 ( #69452, #103570, #94060, #30, #77829, #70012, #86774, #50978, #10063 ),
 ( #34712, #42021, #59392, #44236, #85107, #78380, #104126, #27413, #16775 ),
 ( #61596, #95729, #18993, #76719, #25189, #51522, #8396, #33591, #101896 ),
 ( #42566, #68349, #25742, #17328, #85656, #8955, #71114, #72210, #45353 ),
 ( #36369, #105238, #96848, #62156, #87333, #2256, #62726, #4439, #29082 ) ),
 .UNSPECIFIED., .F., .F., .F.,
 ( 6, 6 ),
 ( 6, 3, 6 ),
 ( 25.26539605949999867, 42.22154059670000237 ),
 ( 0.000000000000000000, 1.000000000000000000, 2.000000000000000000 ),
 .UNSPECIFIED. ) ;
#76877=CARTESIAN_POINT ( 'NONE',  ( -22.44875270440000392, 1409.696988105930131, 206.2467493338480153 ) ) ;
#76878=EDGE_CURVE ( 'NONE', #76557, #104116, #62698, .T. ) ;
#76879=( BOUNDED_SURFACE ( )  B_SPLINE_SURFACE ( 3, 2, ( 
 ( #65265, #99375, #30533 ),
 ( #38922, #22649, #73102 ),
 ( #107241, #88797, #64724 ),
 ( #56299, #90429, #13708 ),
 ( #11541, #79853, #37296 ),
 ( #49562, #66920, #74761 ),
 ( #32190, #56854, #32740 ),
 ( #41695, #6986, #76398 ) ),
 .UNSPECIFIED., .F., .F., .T. ) 
 B_SPLINE_SURFACE_WITH_KNOTS ( ( 4, 2, 2, 4 ),
 ( 3, 3 ),
 ( 0.000000000000000000, 0.004949390070308980552, 0.007424085105463470828, 0.009898780140617961104 ),
 ( 0.000000000000000000, 1.000000000000000000 ),
 .UNSPECIFIED. ) 
 GEOMETRIC_REPRESENTATION_ITEM ( )  RATIONAL_B_SPLINE_SURFACE ( (
 ( 1.000000000000000000, 0.7008166191799920508, 1.000000000000000000),
 ( 1.000000000000000000, 0.6998717291170757360, 1.000000000000000000),
 ( 1.000000000000000000, 0.6996362392812857101, 1.000000000000000000),
 ( 1.000000000000000000, 0.6996543790199832857, 1.000000000000000000),
 ( 1.000000000000000000, 0.6997206315696691270, 1.000000000000000000),
 ( 1.000000000000000000, 0.6997875685659131761, 1.000000000000000000),
 ( 1.000000000000000000, 0.6997874683881916136, 1.000000000000000000),
 ( 1.000000000000000000, 0.6996393069086717098, 1.000000000000000000) ) ) 
 REPRESENTATION_ITEM ( '' )  SURFACE ( )  );
#76880=CARTESIAN_POINT ( 'NONE',  ( 17.84636975430000305, 1416.824060884929850, 206.2620219508280286 ) ) ;
#76882=VECTOR ( 'NONE', #86408, 1000.000000000000000 ) ;
#76884=B_SPLINE_SURFACE_WITH_KNOTS ( 'NONE', 5, 5, ( 
 ( #79076, #18023, #95306, #77948, #36499, #94743, #1254, #103699, #70695 ),
 ( #96969, #62282, #88028, #45481, #2928, #20233, #37044, #9088, #77402 ),
 ( #706, #22410, #39805, #72326, #12389, #37600, #98595, #99133, #30287 ),
 ( #73416, #54976, #107552, #11851, #72863, #73965, #3473, #106456, #22975 ),
 ( #39241, #63926, #80152, #90748, #46574, #56612, #80709, #30839, #71803 ),
 ( #4018, #65015, #81786, #105922, #38144, #14027, #82357, #99682, #29202 ),
 ( #106998, #108096, #63391, #29739, #88567, #48218, #5657, #98041, #97506 ),
 ( #21315, #31390, #55518, #65571, #20775, #46024, #89101, #90185, #89646 ),
 ( #4555, #5088, #12932, #47113, #81239, #38688, #64479, #21859, #56058 ),
 ( #13468, #47659, #23538, #8386, #58810, #50967, #32509, #66679, #14585 ),
 ( #75075, #101325, #57730, #16764, #59382, #85095, #84552, #91849, #91302 ),
 ( #16222, #92950, #24615, #100784, #100258, #67229, #15126, #24077, #68339 ) ),
 .UNSPECIFIED., .F., .F., .F.,
 ( 6, 3, 3, 6 ),
 ( 6, 3, 6 ),
 ( 15.94786254319999941, 27.90018821209999800, 46.89625937809999812, 68.39792989049999505 ),
 ( 0.000000000000000000, 1.000000000000000000, 2.000000005329749975 ),
 .UNSPECIFIED. ) ;
#76885=CARTESIAN_POINT ( 'NONE',  ( 2.471608048749999842, 1438.194204504490017, 150.4833623973980252 ) ) ;
#76888=CARTESIAN_POINT ( 'NONE',  ( -3.535390505542900019, 1507.776748193199865, 180.9473287765760006 ) ) ;
#76889=FACE_OUTER_BOUND ( 'NONE', #11239, .T. ) ;
#76891=CARTESIAN_POINT ( 'NONE',  ( 11.70201856712229826, 1426.718767056610204, 141.6641753760530094 ) ) ;
#76893=AXIS2_PLACEMENT_3D ( 'NONE', #77176, #110204, #35155 ) ;
#76899=CARTESIAN_POINT ( 'NONE',  ( -4.215652631204428680, 1398.038844839439435, 221.4193366157311118 ) ) ;
#76900=CARTESIAN_POINT ( 'NONE',  ( 0.000000000000000000, 1514.413060387330006, 209.1218459616979999 ) ) ;
#76902=CARTESIAN_POINT ( 'NONE',  ( -17.60543171180000144, 1410.868334040629861, 194.0670716385980086 ) ) ;
#76907=VERTEX_POINT ( 'NONE', #20022 ) ;
#76908=CARTESIAN_POINT ( 'NONE',  ( 12.04588369443019857, 1433.807560102029811, 150.0158760707519718 ) ) ;
#76911=CARTESIAN_POINT ( 'NONE',  ( -0.0002573390537614959981, 1396.305641767069801, 221.3136691980663784 ) ) ;
#76914=CARTESIAN_POINT ( 'NONE',  ( 16.09580795758349936, 1424.963234393459970, 191.0812631129040255 ) ) ;
#76915=CARTESIAN_POINT ( 'NONE',  ( 9.534219445089998857, 1428.030197386430018, 144.1938086916980239 ) ) ;
#76916=CARTESIAN_POINT ( 'NONE',  ( 18.87825204697160331, 1498.114858794700240, 229.4168632574339881 ) ) ;
#76917=EDGE_CURVE ( 'NONE', #59045, #6757, #66203, .T. ) ;
#76918=CARTESIAN_POINT ( 'NONE',  ( 0.2362929480300000051, 1488.177340598630053, 181.7177447157979771 ) ) ;
#76919=CARTESIAN_POINT ( 'NONE',  ( -0.3551208789749999983, 1416.218047894730262, 191.1510192753979993 ) ) ;
#76920=CARTESIAN_POINT ( 'NONE',  ( -24.52161429607329879, 1444.774474201280100, 210.9829639010650055 ) ) ;
#76921=CARTESIAN_POINT ( 'NONE',  ( 5.293700147766140063, 1396.097920486130079, 199.4374042141640189 ) ) ;
#76922=CARTESIAN_POINT ( 'NONE',  ( 35.32500643191499279, 1435.854286985769932, 134.0999999975889807 ) ) ;
#76923=CARTESIAN_POINT ( 'NONE',  ( 11.57048490630000082, 1431.876862801990001, 151.1817391485979840 ) ) ;
#76925=ORIENTED_EDGE ( 'NONE', *, *, #18286, .F. ) ;
#76926=CARTESIAN_POINT ( 'NONE',  ( 14.13185208260100012, 1435.965080345399883, 150.0649179125809951 ) ) ;
#76927=ADVANCED_FACE ( 'NONE', ( #2160 ), #52668, .F. ) ;
#76929=ORIENTED_EDGE ( 'NONE', *, *, #41147, .F. ) ;
#76930=CARTESIAN_POINT ( 'NONE',  ( 13.14582496903311259, 1444.761283730599416, 169.3990323816187527 ) ) ;
#76931=CARTESIAN_POINT ( 'NONE',  ( -4.469061828439999218, 1464.606722983030295, 237.1332388458979779 ) ) ;
#76932=AXIS2_PLACEMENT_3D ( 'NONE', #52341, #27669, #61309 ) ;
#76933=CARTESIAN_POINT ( 'NONE',  ( 25.78167222729700114, 1509.813387082529971, 195.1140727163279962 ) ) ;
#76938=ORIENTED_EDGE ( 'NONE', *, *, #95259, .T. ) ;
#76943=CARTESIAN_POINT ( 'NONE',  ( -19.06981053970000062, 1509.578992845429866, 231.5773580161979908 ) ) ;
#76946=CARTESIAN_POINT ( 'NONE',  ( -13.01091002569999944, 1409.534180062029918, 190.3248903057979931 ) ) ;
#76949=ORIENTED_EDGE ( 'NONE', *, *, #14854, .F. ) ;
#76950=CARTESIAN_POINT ( 'NONE',  ( 24.55105544570000120, 1439.606887532569999, 213.0196149167179840 ) ) ;
#76959=CARTESIAN_POINT ( 'NONE',  ( -20.61444355170000264, 1508.354544900629890, 190.2376287260979950 ) ) ;
#76962=CARTESIAN_POINT ( 'NONE',  ( 14.66466848360000164, 1409.425161895129804, 192.9600527036979827 ) ) ;
#76967=CIRCLE ( 'NONE', #7251, 1.999999999997927436 ) ;
#76968=CARTESIAN_POINT ( 'NONE',  ( 11.55308038760000144, 1469.479404942429937, 255.2309336889980216 ) ) ;
#76969=CARTESIAN_POINT ( 'NONE',  ( 1.897589185483037122, 1452.532807482775752, 183.5787857509751859 ) ) ;
#76970=CARTESIAN_POINT ( 'NONE',  ( -28.17578495147160211, 1509.896980478850082, 217.3377154775169799 ) ) ;
#76971=CARTESIAN_POINT ( 'NONE',  ( -2.549355810456779725, 1507.417392930419965, 236.9597321781060089 ) ) ;
#76974=CARTESIAN_POINT ( 'NONE',  ( -23.99136450790000197, 1445.147507561969860, 213.3355241665780113 ) ) ;
#76975=B_SPLINE_CURVE_WITH_KNOTS ( 'NONE', 3,
 ( #19711, #53914, #88049, #11334 ),
 .UNSPECIFIED., .F., .F.,
 ( 4, 4 ),
 ( 0.000000000000000000, 1.000000000000000000 ),
 .UNSPECIFIED. ) ;
#76976=CARTESIAN_POINT ( 'NONE',  ( -11.60004869885203682, 1411.254281879943164, 137.0999999980979851 ) ) ;
#76977=CARTESIAN_POINT ( 'NONE',  ( 17.76902723066159950, 1410.077149175569957, 222.7945870334489769 ) ) ;
#76981=CARTESIAN_POINT ( 'NONE',  ( 0.2163172094670000045, 1405.717036350329863, 267.8540247887980286 ) ) ;
#76984=CARTESIAN_POINT ( 'NONE',  ( 28.63451943380000131, 1509.912999839629947, 206.7172238586179844 ) ) ;
#76985=CARTESIAN_POINT ( 'NONE',  ( 24.57126113369999842, 1440.930743420699855, 213.1726824911179961 ) ) ;
#76989=CARTESIAN_POINT ( 'NONE',  ( -20.99310762600000047, 1509.712614273529880, 187.9175820947980071 ) ) ;
#76990=CARTESIAN_POINT ( 'NONE',  ( 29.16087826349600221, 1436.844756045629993, 136.7088000707439903 ) ) ;
#76991=CARTESIAN_POINT ( 'NONE',  ( 34.97887668886630053, 1450.312591923280024, 136.2298315295870168 ) ) ;
#76992=CARTESIAN_POINT ( 'NONE',  ( 3.207026754074329869E-15, 1467.715966850440054, 261.8343058931689598 ) ) ;
#76994=CARTESIAN_POINT ( 'NONE',  ( 8.878917281270000572, 1509.223119011030121, 181.5151191445980032 ) ) ;
#76997=CARTESIAN_POINT ( 'NONE',  ( -38.88868005081535273, 1452.484090863069014, 269.5912342720579318 ) ) ;
#76999=CARTESIAN_POINT ( 'NONE',  ( -18.93537658700000037, 1413.766156166430164, 268.3665355202980436 ) ) ;
#77003=CARTESIAN_POINT ( 'NONE',  ( 26.79414481833639883, 1435.433178084320161, 135.2874577367330176 ) ) ;
#77005=CARTESIAN_POINT ( 'NONE',  ( -0.3883820753600000231, 1416.446510123330199, 233.6943695348979873 ) ) ;
#77008=CARTESIAN_POINT ( 'NONE',  ( -13.07100154019126315, 1444.825073959231759, 186.3867726210717137 ) ) ;
#77015=CARTESIAN_POINT ( 'NONE',  ( 25.63655495179999733, 1436.189972215739999, 136.9580440781980144 ) ) ;
#77016=CARTESIAN_POINT ( 'NONE',  ( -10.88335057715240062, 1396.293115364239839, 207.0876604851810043 ) ) ;
#77019=CARTESIAN_POINT ( 'NONE',  ( -17.21692188389469891, 1410.879836749619926, 226.0201596333920122 ) ) ;
#77020=CARTESIAN_POINT ( 'NONE',  ( 12.00000000000000000, 1443.913060387330006, 147.5878346084980137 ) ) ;
#77021=VERTEX_POINT ( 'NONE', #56266 ) ;
#77022=ORIENTED_EDGE ( 'NONE', *, *, #13091, .F. ) ;
#77027=CARTESIAN_POINT ( 'NONE',  ( 22.68528333430000288, 1409.869697741029995, 212.6986685081479891 ) ) ;
#77035=CARTESIAN_POINT ( 'NONE',  ( -2.528665822673169918E-09, 1414.285713195190056, 246.7922399721219904 ) ) ;
#77038=CARTESIAN_POINT ( 'NONE',  ( -11.82137633359979922, 1429.378842759500003, 149.1280831305220147 ) ) ;
#77040=CARTESIAN_POINT ( 'NONE',  ( -2.303611226680000179, 1473.224731274329770, 270.4285322737979982 ) ) ;
#77044=B_SPLINE_CURVE_WITH_KNOTS ( 'NONE', 3,
 ( #55984, #5009, #39156, #72787, #106914, #106373, #64941, #90663, #54888, #64393, #73888, #63303, #80627, #21228, #82274 ),
 .UNSPECIFIED., .F., .F.,
 ( 4, 2, 2, 1, 1, 1, 2, 2, 4 ),
 ( 0.000000000000000000, 0.2499999999999962252, 0.3749999999999940048, 0.4374999999999953926, 0.4687499999999934497, 0.4843749999999965583, 0.4921874999999956146, 0.4999999999999946709, 1.000000000000000000 ),
 .UNSPECIFIED. ) ;
#77046=CARTESIAN_POINT ( 'NONE',  ( 14.43914856551324100, 1435.431933939060400, 149.5787995519261528 ) ) ;
#77049=CARTESIAN_POINT ( 'NONE',  ( -22.72903601768109993, 1507.336004462989877, 208.4180099543350195 ) ) ;
#77051=CARTESIAN_POINT ( 'NONE',  ( 9.888001510779538705, 1409.198532364260018, 197.8619322872570194 ) ) ;
#77052=CARTESIAN_POINT ( 'NONE',  ( -15.53680187063869944, 1407.737570638100124, 268.3823695302049828 ) ) ;
#77053=CARTESIAN_POINT ( 'NONE',  ( -14.33596079271969970, 1436.258147809659931, 150.0352455327449945 ) ) ;
#77055=DIRECTION ( 'NONE',  ( 1.000000000000000000, 0.000000000000000000, 0.000000000000000000 ) ) ;
#77056=CARTESIAN_POINT ( 'NONE',  ( 13.42771486050000007, 1443.428666381239964, 188.1474344706980162 ) ) ;
#77059=CARTESIAN_POINT ( 'NONE',  ( -22.06116865633574164, 1506.527232288060532, 209.1639464567564346 ) ) ;
#77062=CARTESIAN_POINT ( 'NONE',  ( -16.06248428700000375, 1485.484064211630084, 187.6661218516980227 ) ) ;
#77063=CARTESIAN_POINT ( 'NONE',  ( 8.742163716520650412E-12, 1408.913060387359792, 224.1216835645979870 ) ) ;
#77067=CARTESIAN_POINT ( 'NONE',  ( -2.500000000000000000, 1419.365678191629968, 145.1702635125890311 ) ) ;
#77070=CARTESIAN_POINT ( 'NONE',  ( -27.58156214539999951, 1508.605065867730218, 205.3521991578080019 ) ) ;
#77074=CARTESIAN_POINT ( 'NONE',  ( -5.683186617470000535, 1409.111521637029909, 195.5271251408980220 ) ) ;
#77077=CARTESIAN_POINT ( 'NONE',  ( -38.39760561535049987, 1443.174109818610077, 137.1306153789020073 ) ) ;
#77078=VERTEX_POINT ( 'NONE', #8601 ) ;
#77079=CARTESIAN_POINT ( 'NONE',  ( -28.25140912874190136, 1508.152706103189757, 208.8568142479740004 ) ) ;
#77080=CARTESIAN_POINT ( 'NONE',  ( 27.14725374240000022, 1488.689090776530065, 210.8864821603579855 ) ) ;
#77082=CARTESIAN_POINT ( 'NONE',  ( 19.75967613925110200, 1467.111012934069777, 224.7767255004650053 ) ) ;
#77083=CARTESIAN_POINT ( 'NONE',  ( -13.17868479539550108, 1436.069128864759932, 150.6624180133409823 ) ) ;
#77088=CARTESIAN_POINT ( 'NONE',  ( -15.28683124289999995, 1417.995325491429867, 226.9473089156979881 ) ) ;
#77092=DIRECTION ( 'NONE',  ( -1.000000000000000000, 0.000000000000000000, -0.000000000000000000 ) ) ;
#77093=CARTESIAN_POINT ( 'NONE',  ( 3.023156474270449756, 1440.625623375490250, 157.2242885116500020 ) ) ;
#77099=ORIENTED_EDGE ( 'NONE', *, *, #76712, .T. ) ;
#77100=CARTESIAN_POINT ( 'NONE',  ( 12.48554310994400041, 1434.717551771250101, 150.3686571217509993 ) ) ;
#77101=CARTESIAN_POINT ( 'NONE',  ( 7.681229707928440398, 1459.296350014880090, 232.9086509542260046 ) ) ;
#77102=CARTESIAN_POINT ( 'NONE',  ( -24.44688238734340047, 1509.532643014110135, 223.1734339750240110 ) ) ;
#77107=CARTESIAN_POINT ( 'NONE',  ( 14.31611368511230076, 1440.103953689049831, 195.6162067410979830 ) ) ;
#77108=CARTESIAN_POINT ( 'NONE',  ( 19.86721287640000000, 1507.838653413830116, 189.0155849983980261 ) ) ;
#77109=CARTESIAN_POINT ( 'NONE',  ( 18.80339027203730140, 1425.953307585449693, 225.0197318394450008 ) ) ;
#77110=VERTEX_POINT ( 'NONE', #79702 ) ;
#77111=CARTESIAN_POINT ( 'NONE',  ( -12.73048917230000043, 1416.839648759230158, 195.1127161226980036 ) ) ;
#77114=ORIENTED_EDGE ( 'NONE', *, *, #40376, .F. ) ;
#77120=CARTESIAN_POINT ( 'NONE',  ( -9816.840209716168829, 50.13405481564039690, 1424.308828391800034 ) ) ;
#77123=CARTESIAN_POINT ( 'NONE',  ( 17.79796669920695962, 1423.568134027953874, 226.0479527846472934 ) ) ;
#77126=CARTESIAN_POINT ( 'NONE',  ( 17.27558691658489920, 1507.606285602530079, 193.9884222186300065 ) ) ;
#77127=CARTESIAN_POINT ( 'NONE',  ( 26.51885050974659919, 1446.534126665770145, 137.5835070401340090 ) ) ;
#77132=CARTESIAN_POINT ( 'NONE',  ( 1.546943247107299912, 1416.828039266790029, 190.2227890105679933 ) ) ;
#77133=CARTESIAN_POINT ( 'NONE',  ( 25.16773666439999957, 1469.174723959130233, 206.4821696811979734 ) ) ;
#77135=CARTESIAN_POINT ( 'NONE',  ( -24.39471867520000004, 1441.818671411180048, 212.1017248715180017 ) ) ;
#77136=CARTESIAN_POINT ( 'NONE',  ( 9.754839755262800338, 1410.624863008607917, 188.5069135823247848 ) ) ;
#77137=CARTESIAN_POINT ( 'NONE',  ( -3.841995486307249852, 1426.014736440487241, 186.0323716116992614 ) ) ;
#77143=CARTESIAN_POINT ( 'NONE',  ( -27.73009598743778170, 1509.592383908645388, 212.1188701747986158 ) ) ;
#77147=EDGE_LOOP ( 'NONE', ( #43890, #20072, #26003, #17340 ) ) ;
#77148=CARTESIAN_POINT ( 'NONE',  ( -1.555730441549999954, 1414.913528139930122, 226.2389583330979974 ) ) ;
#77150=CARTESIAN_POINT ( 'NONE',  ( -16.88043746970000214, 1409.502538253129842, 223.8714129622979954 ) ) ;
#77152=ORIENTED_EDGE ( 'NONE', *, *, #38617, .T. ) ;
#77153=CARTESIAN_POINT ( 'NONE',  ( 20.02269696830319745, 1509.646906251600058, 231.0594384784430133 ) ) ;
#77155=CARTESIAN_POINT ( 'NONE',  ( 39.52630824909760321, 1440.563701659530125, 136.7829907804839991 ) ) ;
#77156=CARTESIAN_POINT ( 'NONE',  ( 18.34422345790000008, 1416.813004075630033, 209.3831160866600101 ) ) ;
#77157=CARTESIAN_POINT ( 'NONE',  ( 1.804213551060599885, 1410.351307734219972, 232.1928989352460064 ) ) ;
#77158=B_SPLINE_CURVE_WITH_KNOTS ( 'NONE', 3,
 ( #19131, #71256, #97521, #19703, #96984, #70707 ),
 .UNSPECIFIED., .F., .F.,
 ( 4, 2, 4 ),
 ( -0.08456724678697399855, -0.04349631223698429555, -3.514124158332521120E-09 ),
 .UNSPECIFIED. ) ;
#77159=CARTESIAN_POINT ( 'NONE',  ( -18.53418666356940037, 1507.620785846770104, 229.7143111648900060 ) ) ;
#77162=CARTESIAN_POINT ( 'NONE',  ( -12.74251030676457219, 1435.892414221138324, 150.8545518745174263 ) ) ;
#77163=CARTESIAN_POINT ( 'NONE',  ( -19.87223104929999806, 1484.291808912129909, 191.2808552885979907 ) ) ;
#77164=CARTESIAN_POINT ( 'NONE',  ( 2.296480925049999566, 1409.498280224829841, 185.7306842272979850 ) ) ;
#77166=CARTESIAN_POINT ( 'NONE',  ( -6.218421316459999737, 1442.637438626040193, 154.8383831912979929 ) ) ;
#77167=CARTESIAN_POINT ( 'NONE',  ( 9.273216669420000002, 1438.130896514020151, 153.0611339723980109 ) ) ;
#77168=CARTESIAN_POINT ( 'NONE',  ( -2.500000000000000000, 1438.975676423110144, 156.0980984760799970 ) ) ;
#77170=CARTESIAN_POINT ( 'NONE',  ( 1.793053373890000080, 1464.825772794629984, 236.8167814476979913 ) ) ;
#77173=CARTESIAN_POINT ( 'NONE',  ( -39.85331664670000151, 1454.050829305929938, 270.3388278179979807 ) ) ;
#77174=CARTESIAN_POINT ( 'NONE',  ( -23.71336536504703574, 1436.266214628221860, 212.4341823126743520 ) ) ;
#77176=CARTESIAN_POINT ( 'NONE',  ( 0.000000000000000000, 1511.163060387329779, 209.1218459616979999 ) ) ;
#77177=AXIS2_PLACEMENT_3D ( 'NONE', #16635, #50302, #57048 ) ;
#77178=CARTESIAN_POINT ( 'NONE',  ( -5.234639134658570038E-09, 1472.084393564380207, 259.1903821046649909 ) ) ;
#77179=CARTESIAN_POINT ( 'NONE',  ( -19.94885833576309864, 1486.773834316860075, 191.0002569412860112 ) ) ;
#77180=CARTESIAN_POINT ( 'NONE',  ( -1.309033247469999717, 1415.245980412430072, 227.1689405978980290 ) ) ;
#77181=CARTESIAN_POINT ( 'NONE',  ( -9.915983682350001160, 1418.249051007830076, 230.0631123014979664 ) ) ;
#77186=CARTESIAN_POINT ( 'NONE',  ( -46.08525396504009564, 1437.664701401070261, 267.5961899802729818 ) ) ;
#77189=ORIENTED_EDGE ( 'NONE', *, *, #38464, .F. ) ;
#77191=CARTESIAN_POINT ( 'NONE',  ( -5.423613671689999194, 1436.253592826889872, 154.6924146223979903 ) ) ;
#77192=CARTESIAN_POINT ( 'NONE',  ( 19.26235814462797080, 1456.284170134162196, 224.9177539954318945 ) ) ;
#77194=AXIS2_PLACEMENT_3D ( 'NONE', #97191, #31088, #54675 ) ;
#77195=CARTESIAN_POINT ( 'NONE',  ( -25.57130305119999747, 1451.861998525429954, 136.0021594398979801 ) ) ;
#77197=CARTESIAN_POINT ( 'NONE',  ( 22.58669161350000110, 1429.440852403829922, 225.6931608660979975 ) ) ;
#77202=CARTESIAN_POINT ( 'NONE',  ( -19.27620331059999970, 1429.330891638030153, 211.8895311099979892 ) ) ;
#77206=EDGE_LOOP ( 'NONE', ( #27725, #36425, #5275, #23754 ) ) ;
#77207=CARTESIAN_POINT ( 'NONE',  ( -1.857564137763940026, 1408.260413705610063, 270.3921255040010010 ) ) ;
#77208=CARTESIAN_POINT ( 'NONE',  ( 6.289830419486070134, 1417.554321210839817, 231.5395384113830062 ) ) ;
#77211=ORIENTED_EDGE ( 'NONE', *, *, #1647, .T. ) ;
#77212=VERTEX_POINT ( 'NONE', #83373 ) ;
#77213=CARTESIAN_POINT ( 'NONE',  ( -23.79955979311329983, 1410.855393305810139, 210.1471472738759871 ) ) ;
#77214=CARTESIAN_POINT ( 'NONE',  ( -4.117509958049999419, 1423.942521120929996, 184.8346656465980118 ) ) ;
#77215=CARTESIAN_POINT ( 'NONE',  ( -12.84239665067440050, 1435.935719077439899, 150.8114796122480072 ) ) ;
#77216=CARTESIAN_POINT ( 'NONE',  ( -9.393138309199999370, 1428.175987565129844, 133.6118001900980232 ) ) ;
#77218=CARTESIAN_POINT ( 'NONE',  ( -20.72930395482273980, 1436.452857176349426, 144.6331020082059524 ) ) ;
#77219=CARTESIAN_POINT ( 'NONE',  ( -22.76855102469999892, 1420.825742769929775, 213.4933674877779879 ) ) ;
#77221=CARTESIAN_POINT ( 'NONE',  ( 39.21901426951580305, 1459.467597158179842, 268.4332945158389521 ) ) ;
#77226=CARTESIAN_POINT ( 'NONE',  ( 18.37403822010337606, 1459.029453797243377, 227.7512596423872537 ) ) ;
#77231=CARTESIAN_POINT ( 'NONE',  ( 25.64531625424840300, 1451.299216082280054, 136.7230207455749849 ) ) ;
#77236=CARTESIAN_POINT ( 'NONE',  ( 18.19540490880000050, 1409.548457928130119, 195.8472809290980194 ) ) ;
#77237=CARTESIAN_POINT ( 'NONE',  ( 13.51610093809999924, 1443.913060387330006, 169.3501091259980171 ) ) ;
#77239=CARTESIAN_POINT ( 'NONE',  ( 1.161811177069999923, 1415.656198137530055, 233.0499152497979765 ) ) ;
#77240=CARTESIAN_POINT ( 'NONE',  ( -18.87276086228866134, 1424.762499899002478, 224.4369045893865859 ) ) ;
#77241=CARTESIAN_POINT ( 'NONE',  ( 1.245434630070580084, 1451.852414238919891, 183.2837320638540177 ) ) ;
#77242=CIRCLE ( 'NONE', #86176, 1.999999999999967359 ) ;
#77243=CARTESIAN_POINT ( 'NONE',  ( -0.2698014165509999840, 1467.673031231229743, 229.6951974530979896 ) ) ;
#77245=CARTESIAN_POINT ( 'NONE',  ( 16.62685400382315137, 1423.339598140291173, 229.2113107412401121 ) ) ;
#77247=CARTESIAN_POINT ( 'NONE',  ( 10.86245182430920053, 1414.913060387399810, 221.4373602865120176 ) ) ;
#77248=CYLINDRICAL_SURFACE ( 'NONE', #101729, 8.000000000000000000 ) ;
#77249=CARTESIAN_POINT ( 'NONE',  ( 19.65496168979899849, 1477.254282174050104, 226.3273697325350042 ) ) ;
#77252=CARTESIAN_POINT ( 'NONE',  ( -35.49482433925479796, 1450.187122272009901, 136.2332348560269679 ) ) ;
#77254=VECTOR ( 'NONE', #41013, 1000.000000000000114 ) ;
#77255=CARTESIAN_POINT ( 'NONE',  ( -6.832964021560000489, 1472.413060387330006, 271.1218459616979999 ) ) ;
#77256=CARTESIAN_POINT ( 'NONE',  ( -21.72816396132508387, 1509.385241977931855, 191.5789249730982817 ) ) ;
#77257=CARTESIAN_POINT ( 'NONE',  ( 11.07785633880000020, 1433.780515129440118, 151.7038518673980150 ) ) ;
#77258=CARTESIAN_POINT ( 'NONE',  ( 20.74408968300000211, 1445.748654444839985, 224.8635562271979893 ) ) ;
#77263=CARTESIAN_POINT ( 'NONE',  ( 22.65292971370000075, 1409.704085498430004, 208.9051947466459751 ) ) ;
#77264=CARTESIAN_POINT ( 'NONE',  ( 11.57393272574848098, 1398.256210180372136, 215.0439578202975497 ) ) ;
#77265=CARTESIAN_POINT ( 'NONE',  ( -21.51266965019000210, 1509.664297269830058, 231.4111640300060060 ) ) ;
#77267=CARTESIAN_POINT ( 'NONE',  ( 23.22702228879999709, 1430.350733257130059, 215.3285367829879817 ) ) ;
#77269=CARTESIAN_POINT ( 'NONE',  ( 25.55657149410041029, 1436.634586687895762, 137.2252252342358076 ) ) ;
#77271=CARTESIAN_POINT ( 'NONE',  ( 18.88069888589999934, 1519.913060387329779, 221.9840912428979891 ) ) ;
#77280=CARTESIAN_POINT ( 'NONE',  ( -17.22592475669603473, 1444.324653571829685, 162.9227486557985003 ) ) ;
#77281=CARTESIAN_POINT ( 'NONE',  ( 13.19839718189999900, 1434.900414472690045, 149.8854151423980170 ) ) ;
#77282=CARTESIAN_POINT ( 'NONE',  ( -37.48372878019959842, 1450.753171827299866, 134.0999999986339901 ) ) ;
#77283=CARTESIAN_POINT ( 'NONE',  ( 0.000000000000000000, 1512.413060387330006, 209.1218459616979999 ) ) ;
#77284=ORIENTED_EDGE ( 'NONE', *, *, #38349, .F. ) ;
#77285=CARTESIAN_POINT ( 'NONE',  ( -38.64250925225250199, 1443.812098351759914, 137.1879208927209959 ) ) ;
#77292=CARTESIAN_POINT ( 'NONE',  ( -17.99954540876850118, 1410.904693920620048, 195.2564682659330231 ) ) ;
#77295=CARTESIAN_POINT ( 'NONE',  ( -17.34479452230000263, 1421.466062287029899, 191.6560375100980025 ) ) ;
#77297=ORIENTED_EDGE ( 'NONE', *, *, #84652, .F. ) ;
#77306=CARTESIAN_POINT ( 'NONE',  ( -4.468129194875738897, 1440.960114343879923, 155.7399638150290002 ) ) ;
#77307=CARTESIAN_POINT ( 'NONE',  ( -22.52609270459879909, 1509.699688878229836, 190.3921826462719764 ) ) ;
#77308=CARTESIAN_POINT ( 'NONE',  ( 16.50752364097115432, 1432.498724059854794, 217.9353314166346536 ) ) ;
#77309=CARTESIAN_POINT ( 'NONE',  ( 2.324664979250000041, 1417.769420424829832, 234.1229704360980008 ) ) ;
#77311=CARTESIAN_POINT ( 'NONE',  ( -0.4794255386042055589, 1405.913060387330006, 208.2442633998076076 ) ) ;
#77315=CARTESIAN_POINT ( 'NONE',  ( 3.143430471549999883, 1447.188766879889954, 156.1110924090980063 ) ) ;
#77316=LINE ( 'NONE', #60527, #78047 ) ;
#77323=CARTESIAN_POINT ( 'NONE',  ( -24.81840806659999998, 1430.361839728229825, 208.2500735500409803 ) ) ;
#77324=CARTESIAN_POINT ( 'NONE',  ( -11.32017911025210033, 1426.032081424100170, 121.9038151518229967 ) ) ;
#77325=CARTESIAN_POINT ( 'NONE',  ( 16.90311995223630248, 1409.749624152390197, 192.7847012683340040 ) ) ;
#77327=CARTESIAN_POINT ( 'NONE',  ( 13.83427921383815296, 1509.519097606679679, 182.4629909201055113 ) ) ;
#77329=CARTESIAN_POINT ( 'NONE',  ( -41.56051825480000161, 1440.913060433189912, 261.5689736827979459 ) ) ;
#77330=CARTESIAN_POINT ( 'NONE',  ( 14.12038737319999804, 1509.406339941330089, 234.8413163218980060 ) ) ;
#77331=CARTESIAN_POINT ( 'NONE',  ( 17.83610898133235523, 1459.676779477080800, 228.1619011578495702 ) ) ;
#77334=CARTESIAN_POINT ( 'NONE',  ( -34.23216826509359834, 1437.030530471749898, 136.5523443324769914 ) ) ;
#77336=CARTESIAN_POINT ( 'NONE',  ( 7.347645689298669680, 1396.698419829339855, 197.9933311278070107 ) ) ;
#77338=CARTESIAN_POINT ( 'NONE',  ( -16.17568645049999887, 1459.146939831430018, 230.7169136887979732 ) ) ;
#77342=CARTESIAN_POINT ( 'NONE',  ( 5.662127998274639649E-15, 1428.868816406519954, 155.3340242552920074 ) ) ;
#77346=DIRECTION ( 'NONE',  ( -0.2020450484956257953, -0.9583089390315990830, 0.2020439945916019109 ) ) ;
#77347=CARTESIAN_POINT ( 'NONE',  ( -2.074664006059999899, 1461.195951710430109, 235.0034078370979955 ) ) ;
#77352=VERTEX_POINT ( 'NONE', #57663 ) ;
#77356=CARTESIAN_POINT ( 'NONE',  ( 10.79382126600000014, 1414.913060387329779, 222.1041115775979904 ) ) ;
#77358=ORIENTED_EDGE ( 'NONE', *, *, #62048, .F. ) ;
#77359=CARTESIAN_POINT ( 'NONE',  ( -1.464954376784709966, 1483.297409201249820, 182.5266383246559769 ) ) ;
#77360=EDGE_CURVE ( 'NONE', #13046, #76760, #11296, .T. ) ;
#77361=CARTESIAN_POINT ( 'NONE',  ( -11.79676896300389899, 1432.336587515399970, 150.5395565867330276 ) ) ;
#77362=CARTESIAN_POINT ( 'NONE',  ( 3.014560028699999616, 1509.018331143230171, 237.6263297230979958 ) ) ;
#77364=CARTESIAN_POINT ( 'NONE',  ( -5.092207154709999628, 1422.992073831329890, 184.8686965921980061 ) ) ;
#77365=CARTESIAN_POINT ( 'NONE',  ( 6.470863363499999465, 1408.267973739730223, 270.2848116647979850 ) ) ;
#77370=CARTESIAN_POINT ( 'NONE',  ( -16.32008265250000179, 1485.103448096529974, 223.8634069782979736 ) ) ;
#77372=DIRECTION ( 'NONE',  ( 0.03489949670244951035, -0.9993908270190976495, 0.000000000000000000 ) ) ;
#77373=CARTESIAN_POINT ( 'NONE',  ( -4.996827698378051075, 1423.157233635628472, 184.7741671071053986 ) ) ;
#77375=CARTESIAN_POINT ( 'NONE',  ( -5.360123413344440202, 1422.242518929100015, 144.1648998030460120 ) ) ;
#77379=CARTESIAN_POINT ( 'NONE',  ( -2.953143827464752125, 1485.357549468870047, 182.9368206477720662 ) ) ;
#77382=ORIENTED_EDGE ( 'NONE', *, *, #24147, .F. ) ;
#77383=CARTESIAN_POINT ( 'NONE',  ( 0.7397222398529998966, 1507.631725798030175, 186.3339393659980203 ) ) ;
#77385=CARTESIAN_POINT ( 'NONE',  ( -10.92055574760000169, 1428.871682173630006, 150.9007266609980320 ) ) ;
#77386=CARTESIAN_POINT ( 'NONE',  ( 19.30758915063299952, 1456.939942660950010, 224.6494214983680138 ) ) ;
#77392=EDGE_CURVE ( 'NONE', #34085, #88970, #51325, .T. ) ;
#77395=CARTESIAN_POINT ( 'NONE',  ( -16.78521628583800052, 1460.263955658562054, 228.3353027301660063 ) ) ;
#77397=CARTESIAN_POINT ( 'NONE',  ( 31.69002272450000035, 1415.319682416229853, 267.1138992859980021 ) ) ;
#77398=CARTESIAN_POINT ( 'NONE',  ( 6.763640255447179445E-10, 1465.118916387369836, 238.1343321182859825 ) ) ;
#77399=CARTESIAN_POINT ( 'NONE',  ( 22.21890555590000105, 1469.152603482329823, 196.0583803768979863 ) ) ;
#77400=CARTESIAN_POINT ( 'NONE',  ( -0.2273306708084070205, 1508.146722782000097, 237.5484237907730005 ) ) ;
#77401=CARTESIAN_POINT ( 'NONE',  ( -1.676216088789999947, 1450.511947750759873, 182.4451611760979972 ) ) ;
#77402=CARTESIAN_POINT ( 'NONE',  ( -7.605711504302860249, 1407.218299713070110, 198.4634440487380118 ) ) ;
#77404=CARTESIAN_POINT ( 'NONE',  ( -14.52606424000000018, 1443.052989431600054, 188.9151166515979980 ) ) ;
#77408=ORIENTED_EDGE ( 'NONE', *, *, #59298, .F. ) ;
#77410=CARTESIAN_POINT ( 'NONE',  ( -14.83265502289820148, 1409.431028114330047, 210.8625800445090022 ) ) ;
#77411=B_SPLINE_CURVE_WITH_KNOTS ( 'NONE', 3,
 ( #101762, #68215, #59798, #102320, #50304, #24502, #58692, #25606, #83325, #92825, #23948, #6620, #58145, #86632, #45771, #62021, #71546, #1002, #70426, #61465, #105667, #44657, #87194, #95591, #78798, #36239, #10486, #86087, #45215, #9927, #52503, #43544, #78235, #104545, #60347, #2113, #19979 ),
 .UNSPECIFIED., .F., .F.,
 ( 4, 3, 3, 3, 3, 3, 3, 3, 3, 3, 3, 3, 4 ),
 ( -1.999999730069600190, -1.888170853378660086, -1.719898845985929903, -1.549431836185619860, -1.377736129787159980, -1.204387122194009896, -1.030404623667469988, -0.8562074511777200136, -0.6822290056525619484, -0.5094606239557140093, -0.3379870002562179732, -0.1681008084855228901, -7.314383555279135862E-06 ),
 .UNSPECIFIED. ) ;
#77414=CARTESIAN_POINT ( 'NONE',  ( -27.01637664349999923, 1469.366081882129947, 266.9349976846980326 ) ) ;
#77416=CARTESIAN_POINT ( 'NONE',  ( 0.1634414413833199797, 1420.301959611109851, 183.5344649337699821 ) ) ;
#77417=CARTESIAN_POINT ( 'NONE',  ( -25.23662982120000109, 1509.794342920329882, 222.8844980439979793 ) ) ;
#77422=CARTESIAN_POINT ( 'NONE',  ( 11.86597105769770089, 1415.542389211310137, 223.1847760632660140 ) ) ;
#77425=CARTESIAN_POINT ( 'NONE',  ( -2.253566441613126910E-10, 1426.918876941764893, 137.0999999980980135 ) ) ;
#77427=CARTESIAN_POINT ( 'NONE',  ( -23.37532479789999940, 1410.224545597529868, 206.6383130864379893 ) ) ;
#77429=EDGE_CURVE ( 'NONE', #94174, #15766, #17778, .T. ) ;
#77430=CARTESIAN_POINT ( 'NONE',  ( 17.83292642509999837, 1416.519106787730152, 206.2642702630979841 ) ) ;
#77433=EDGE_CURVE ( 'NONE', #9799, #75668, #33869, .T. ) ;
#77434=CARTESIAN_POINT ( 'NONE',  ( 0.8348477807080000312, 1443.913060387330006, 150.8032249175980155 ) ) ;
#77439=CARTESIAN_POINT ( 'NONE',  ( -21.33808675349999717, 1409.658202796229943, 210.9642962936580091 ) ) ;
#77441=CARTESIAN_POINT ( 'NONE',  ( 11.69356494263769974, 1426.724475661050292, 141.0600989001800087 ) ) ;
#77446=CARTESIAN_POINT ( 'NONE',  ( 11.60004869885203682, 1428.983126981193436, 134.0999999980966777 ) ) ;
#77448=B_SPLINE_CURVE_WITH_KNOTS ( 'NONE', 5,
 ( #68614, #16501, #58553, #51240, #15956, #26579 ),
 .UNSPECIFIED., .F., .F.,
 ( 6, 6 ),
 ( 0.000000000000000000, 1.000000000000000000 ),
 .UNSPECIFIED. ) ;
#77451=CARTESIAN_POINT ( 'NONE',  ( -18.84520706720000049, 1449.647908397599849, 193.3285045537979840 ) ) ;
#77455=ORIENTED_EDGE ( 'NONE', *, *, #26199, .F. ) ;
#77457=CARTESIAN_POINT ( 'NONE',  ( 11.94671513487030090, 1433.512659209229923, 149.9919407150609914 ) ) ;
#77463=CARTESIAN_POINT ( 'NONE',  ( 16.05359747075639731, 1423.514842284070028, 191.1259792483479885 ) ) ;
#77464=CARTESIAN_POINT ( 'NONE',  ( 4.496878417739999634, 1428.155750001629940, 101.8807690336980016 ) ) ;
#77465=CARTESIAN_POINT ( 'NONE',  ( 10.89898159000000000, 1507.806799034729920, 234.1500837693980088 ) ) ;
#77467=CARTESIAN_POINT ( 'NONE',  ( 1.347910446750000268, 1507.642032470829918, 181.0718040488980023 ) ) ;
#77468=CARTESIAN_POINT ( 'NONE',  ( -2.824000289829999844, 1415.931784856029935, 191.4879063651980289 ) ) ;
#77473=CARTESIAN_POINT ( 'NONE',  ( 13.94822761382920184, 1415.393085341020196, 197.3723107886449952 ) ) ;
#77474=CARTESIAN_POINT ( 'NONE',  ( 11.75433822149999941, 1431.172422370689901, 150.7091801069980193 ) ) ;
#77477=CARTESIAN_POINT ( 'NONE',  ( 13.97106068711859983, 1435.306965887609977, 149.5915603287180033 ) ) ;
#77482=CARTESIAN_POINT ( 'NONE',  ( 12.89600770202496882, 1444.937073510895061, 169.4370095252451733 ) ) ;
#77483=CARTESIAN_POINT ( 'NONE',  ( -0.3222264186639999806, 1466.023156234830140, 235.8295837109980084 ) ) ;
#77488=CARTESIAN_POINT ( 'NONE',  ( -18.66998849382813219, 1445.113969046085003, 213.7790260993002107 ) ) ;
#77493=ORIENTED_EDGE ( 'NONE', *, *, #35497, .F. ) ;
#77497=CARTESIAN_POINT ( 'NONE',  ( -7.050955535139999952, 1409.159285179630160, 188.4661246024980130 ) ) ;
#77499=CARTESIAN_POINT ( 'NONE',  ( -7.052967567875161770, 1427.664849047028611, 137.0999999980979851 ) ) ;
#77501=CARTESIAN_POINT ( 'NONE',  ( 24.45814044340000137, 1438.107944938759829, 212.7365612476880017 ) ) ;
#77504=CARTESIAN_POINT ( 'NONE',  ( 9.959920982146540425, 1432.347050772769990, 152.5236881046529902 ) ) ;
#77509=EDGE_CURVE ( 'NONE', #5014, #39452, #88902, .T. ) ;
#77510=CARTESIAN_POINT ( 'NONE',  ( -20.55810159319999997, 1507.794327612029974, 189.9655093376980233 ) ) ;
#77514=CARTESIAN_POINT ( 'NONE',  ( 14.06841109650000021, 1410.335884455629866, 191.3015486027980216 ) ) ;
#77515=CARTESIAN_POINT ( 'NONE',  ( -17.05332910918329148, 1486.127261448098807, 187.7340081784555537 ) ) ;
#77517=ORIENTED_EDGE ( 'NONE', *, *, #30133, .F. ) ;
#77519=CARTESIAN_POINT ( 'NONE',  ( 31.44037043649999674, 1456.450353286529889, 254.7811851438980284 ) ) ;
#77522=CARTESIAN_POINT ( 'NONE',  ( -3.915418352780020150, 1508.947664731669875, 237.8621089956459969 ) ) ;
#77523=CARTESIAN_POINT ( 'NONE',  ( -23.35577775049999971, 1449.058501480780251, 216.5496097239480093 ) ) ;
#77525=CARTESIAN_POINT ( 'NONE',  ( 11.76895983000000001, 1432.299379893459900, 150.8120316597980093 ) ) ;
#77526=CARTESIAN_POINT ( 'NONE',  ( 17.10104755112020314, 1409.537284391650019, 222.2845644592789824 ) ) ;
#77533=CARTESIAN_POINT ( 'NONE',  ( 12.82226628359999943, 1419.802649937829983, 223.2233948557979772 ) ) ;
#77534=CARTESIAN_POINT ( 'NONE',  ( 5.398680167209999325, 1433.945743868580166, 154.6429197126979886 ) ) ;
#77536=CARTESIAN_POINT ( 'NONE',  ( -28.11203376899999995, 1444.250560465929993, 137.5208087134980133 ) ) ;
#77538=CARTESIAN_POINT ( 'NONE',  ( 27.34169902030170363, 1435.611507683570153, 136.1486617027460113 ) ) ;
#77547=CARTESIAN_POINT ( 'NONE',  ( -6.438546668759999925, 1410.951844103529993, 268.3665355202980436 ) ) ;
#77548=ADVANCED_FACE ( 'NONE', ( #37404 ), #9850, .T. ) ;
#77553=CARTESIAN_POINT ( 'NONE',  ( -2.805498944269999911E-09, 1475.983410498229887, 267.2349610869979983 ) ) ;
#77555=CARTESIAN_POINT ( 'NONE',  ( -17.22592475670000312, 1444.324653571829913, 162.9227486557980171 ) ) ;
#77556=CARTESIAN_POINT ( 'NONE',  ( 19.19535387687943029, 1456.080104641030175, 225.8939609127118047 ) ) ;
#77560=CARTESIAN_POINT ( 'NONE',  ( -14.98234439516031813, 1451.152531978053503, 149.7337978842586779 ) ) ;
#77562=CARTESIAN_POINT ( 'NONE',  ( 25.40170928279999885, 1435.672096233849970, 136.5747932110980116 ) ) ;
#77563=ADVANCED_FACE ( 'NONE', ( #56969 ), #55476, .F. ) ;
#77564=CARTESIAN_POINT ( 'NONE',  ( -7.287693820798589961, 1396.167552263480047, 200.8210620288550103 ) ) ;
#77565=ORIENTED_EDGE ( 'NONE', *, *, #86306, .T. ) ;
#77566=CARTESIAN_POINT ( 'NONE',  ( -16.24136799685820165, 1409.480169776980119, 225.1139067059710044 ) ) ;
#77567=EDGE_CURVE ( 'NONE', #94550, #35126, #55876, .T. ) ;
#77572=CARTESIAN_POINT ( 'NONE',  ( 10.33654884809999963, 1425.426884123429772, 91.92460148769789896 ) ) ;
#77574=CARTESIAN_POINT ( 'NONE',  ( -11.07712053549999887, 1433.090719799819908, 151.6979285180979957 ) ) ;
#77575=CARTESIAN_POINT ( 'NONE',  ( -2.497425431713394151, 1421.160177316890895, 184.9476756208646293 ) ) ;
#77578=CARTESIAN_POINT ( 'NONE',  ( 8.326542548460000859, 1507.918730797030094, 183.0016923208980018 ) ) ;
#77579=CARTESIAN_POINT ( 'NONE',  ( 3.492106839979999933, 1450.387407648259796, 184.0776196846979929 ) ) ;
#77583=CARTESIAN_POINT ( 'NONE',  ( -9.617209101676776228, 1463.011625816246806, 234.9738961404823954 ) ) ;
#77585=ORIENTED_EDGE ( 'NONE', *, *, #19298, .T. ) ;
#77586=CARTESIAN_POINT ( 'NONE',  ( -41.49257713859999797, 1443.691015385260016, 136.5669737734980345 ) ) ;
#77588=CARTESIAN_POINT ( 'NONE',  ( -0.9653266517330000296, 1472.614618005129842, 270.3713489653979991 ) ) ;
#77590=CARTESIAN_POINT ( 'NONE',  ( -3.527564898500000101, 1486.518325717629978, 181.8541436997979872 ) ) ;
#77593=CARTESIAN_POINT ( 'NONE',  ( 21.33808983710000007, 1409.658202903930032, 207.2794041873680158 ) ) ;
#77594=CARTESIAN_POINT ( 'NONE',  ( -22.92687821287150030, 1507.614846683489986, 207.6532172876729874 ) ) ;
#77596=CARTESIAN_POINT ( 'NONE',  ( 6.262051076867260591, 1407.785014201449940, 196.9935646766689956 ) ) ;
#77597=CARTESIAN_POINT ( 'NONE',  ( -20.62979332817520017, 1409.412394061799887, 267.3561677121959974 ) ) ;
#77598=CARTESIAN_POINT ( 'NONE',  ( -10.79382269979189957, 1414.913060387349788, 196.1395788316550011 ) ) ;
#77600=DIRECTION ( 'NONE',  ( 0.000000000000000000, 1.000000000000000000, 0.000000000000000000 ) ) ;
#77601=CARTESIAN_POINT ( 'NONE',  ( 13.50895069809999960, 1444.844319576610133, 188.7199091778979891 ) ) ;
#77602=EDGE_LOOP ( 'NONE', ( #13859, #27056, #82576, #7927 ) ) ;
#77608=CARTESIAN_POINT ( 'NONE',  ( -15.62157406900000112, 1485.483397133530161, 187.4151579208979967 ) ) ;
#77609=VERTEX_POINT ( 'NONE', #76387 ) ;
#77613=CARTESIAN_POINT ( 'NONE',  ( -26.37683023809999838, 1508.582706905729992, 201.5299876253779985 ) ) ;
#77617=CARTESIAN_POINT ( 'NONE',  ( -3.862688431370000064, 1407.379791273530145, 196.6061506809980131 ) ) ;
#77618=CARTESIAN_POINT ( 'NONE',  ( -13.75903318429999977, 1409.893112517929922, 226.9379566688979821 ) ) ;
#77619=CARTESIAN_POINT ( 'NONE',  ( -10.51245417620000033, 1447.347034548050033, 186.8435989827979711 ) ) ;
#77621=CARTESIAN_POINT ( 'NONE',  ( -28.27963355899620268, 1508.150913702349953, 209.6131352202170035 ) ) ;
#77622=CARTESIAN_POINT ( 'NONE',  ( 27.39969415949999743, 1508.129222249830036, 213.4901677084380083 ) ) ;
#77624=CARTESIAN_POINT ( 'NONE',  ( 20.71370920478009836, 1497.619563572799962, 225.7436213016659963 ) ) ;
#77625=CARTESIAN_POINT ( 'NONE',  ( -25.39307201429999949, 1435.891440879340053, 136.8929830188979793 ) ) ;
#77629=CARTESIAN_POINT ( 'NONE',  ( -4.363122647530000009, 1432.413060387330006, 146.1721969590979882 ) ) ;
#77634=CARTESIAN_POINT ( 'NONE',  ( -1.013019939329999897, 1412.845282977929855, 233.1607918147980172 ) ) ;
#77636=ORIENTED_EDGE ( 'NONE', *, *, #39255, .F. ) ;
#77639=CARTESIAN_POINT ( 'NONE',  ( 12.12303243055349888, 1434.792252859569999, 150.9027648073679870 ) ) ;
#77640=B_SPLINE_SURFACE_WITH_KNOTS ( 'NONE', 5, 5, ( 
 ( #104838, #26030, #34459, #20811, #51258, #105393 ),
 ( #89136, #72357, #88057, #68635, #71837, #102736 ),
 ( #55009, #10786, #19145, #95884, #11885, #105955 ),
 ( #37631, #28125, #45514, #53352, #46610, #87497 ),
 ( #79105, #12422, #79655, #8687, #2960, #44957 ),
 ( #4051, #11342, #62317, #46057, #2412, #37077 ),
 ( #80742, #20264, #29233, #71280, #63422, #97539 ),
 ( #88602, #80190, #36529, #3507, #19720, #97001 ),
 ( #38177, #70725, #53922, #106488, #96442, #29774 ),
 ( #28686, #62891, #63962, #98077, #85391, #333 ),
 ( #42868, #61758, #77027, #65605, #99717, #109256 ),
 ( #22444, #100290, #12962, #40931, #56645, #90779 ),
 ( #107035, #72895, #56092, #47145, #81270, #107585 ),
 ( #30322, #15156, #81820, #5691, #99163, #5123 ),
 ( #4586, #66713, #23571, #64510, #14062, #108688 ),
 ( #23010, #73453, #21348, #48251, #98626, #57214 ),
 ( #14622, #108129, #38720, #21893, #65049, #82393 ),
 ( #57764, #91883, #90219, #32540, #13503, #39835 ),
 ( #6767, #47692, #31422, #39279, #82932, #91339 ),
 ( #30871, #73998, #48809, #6224, #40377, #89680 ),
 ( #74555, #31980, #49347, #66170, #83474, #75109 ) ),
 .UNSPECIFIED., .F., .F., .F.,
 ( 6, 3, 3, 3, 3, 3, 6 ),
 ( 6, 6 ),
 ( 41.21984250090000046, 43.22195389150000011, 43.93735686660000539, 45.64078810350000026, 47.34421934030000045, 50.75108181390000084, 60.28232112689999411 ),
 ( 0.000000000000000000, 1.469175964770000009 ),
 .UNSPECIFIED. ) ;
#77641=CARTESIAN_POINT ( 'NONE',  ( 14.47037193060810090, 1459.302085855910036, 230.1578363246120205 ) ) ;
#77643=CARTESIAN_POINT ( 'NONE',  ( -2.113408855709999923, 1409.489867483530134, 186.5712290354979928 ) ) ;
#77645=CARTESIAN_POINT ( 'NONE',  ( 4.230878294131939832, 1441.526452546219843, 164.7455269374289912 ) ) ;
#77648=CARTESIAN_POINT ( 'NONE',  ( 19.89462793710000099, 1508.347918119229917, 188.9544000135980184 ) ) ;
#77650=VERTEX_POINT ( 'NONE', #50099 ) ;
#77651=CARTESIAN_POINT ( 'NONE',  ( -11.29419939623580049, 1414.913057855109855, 197.0838916197120056 ) ) ;
#77652=B_SPLINE_SURFACE_WITH_KNOTS ( 'NONE', 5, 5, ( 
 ( #30895, #11909, #4611, #46084, #105981, #72923, #98652, #21918, #56114, #47716, #45541, #81846 ),
 ( #37106, #71305, #62916, #97027, #23035, #33097, #24670, #14647, #57237, #84601, #40952, #14087 ),
 ( #16275, #108157, #24129, #50477, #108712, #67286, #23596, #66191, #101941, #57785, #83495, #48833 ),
 ( #48276, #75129, #56670, #65630, #15718, #82956, #82421, #99744, #39860, #5715, #32003, #74023 ),
 ( #58869, #15180, #100311, #74576, #66737, #92999, #91903, #31447, #49367, #84053, #6791, #6249 ),
 ( #109278, #32561, #100840, #101378, #7892, #91368, #42064, #58320, #92442, #40399, #76214, #49919 ),
 ( #7352, #41515, #90806, #75674, #109818, #110359, #33636, #67830, #52129, #51018, #10106, #51570 ),
 ( #8438, #43171, #69495, #36407, #77869, #95769, #42611, #26342, #1178, #73, #624, #34204 ),
 ( #68388, #1734, #35308, #43717, #27454, #25785, #103617, #86815, #60538, #85152, #78993, #87378 ),
 ( #52678, #94660, #103044, #17931, #35873, #104168, #34755, #76764, #86257, #102495, #44279, #26915 ),
 ( #9547, #2296, #61103, #78423, #53236, #59432, #59984, #94101, #68944, #95220, #18481, #16817 ),
 ( #70057, #61638, #10672, #19035, #44838, #77325, #17372, #70599, #25229, #93544, #85703, #8999 ) ),
 .UNSPECIFIED., .F., .F., .F.,
 ( 6, 3, 3, 6 ),
 ( 6, 3, 3, 6 ),
 ( 6.297091802710249375, 6.724583630079999708, 7.579194017749999901, 8.375326175313119847 ),
 ( -3.459696186616099858E-05, 0.3241439638239999588, 0.9724318914720000429, 1.438929940459749979 ),
 .UNSPECIFIED. ) ;
#77653=DIRECTION ( 'NONE',  ( 0.000000000000000000, 0.7071067811865198172, -0.7071067811865753283 ) ) ;
#77655=CARTESIAN_POINT ( 'NONE',  ( 2.648695236860000080, 1421.139663013429754, 184.4912115941980062 ) ) ;
#77657=CARTESIAN_POINT ( 'NONE',  ( 0.000000000000000000, 1414.913060387329779, 209.1218459616979999 ) ) ;
#77662=CARTESIAN_POINT ( 'NONE',  ( 18.41105348850000212, 1415.553739807329976, 210.1831042486080037 ) ) ;
#77663=CARTESIAN_POINT ( 'NONE',  ( 13.88131303110161596, 1507.515608694632874, 232.8168500089977044 ) ) ;
#77664=DIRECTION ( 'NONE',  ( 0.000000000000000000, 1.000000000000000000, 0.000000000000000000 ) ) ;
#77666=CARTESIAN_POINT ( 'NONE',  ( 15.68557539840000103, 1410.853897593630109, 191.5168599455980143 ) ) ;
#77670=ORIENTED_EDGE ( 'NONE', *, *, #29773, .F. ) ;
#77671=CARTESIAN_POINT ( 'NONE',  ( 0.7038424768878800419, 1507.336011380059972, 186.3928043249479742 ) ) ;
#77673=CARTESIAN_POINT ( 'NONE',  ( -27.77037812200000033, 1508.603156321929873, 210.5143981962980035 ) ) ;
#77674=CARTESIAN_POINT ( 'NONE',  ( 3.744175762052851297, 1410.420533046074297, 185.9466301700599047 ) ) ;
#77675=CARTESIAN_POINT ( 'NONE',  ( -3.569562092499118489, 1426.009408117103476, 185.9142566006702850 ) ) ;
#77676=B_SPLINE_SURFACE_WITH_KNOTS ( 'NONE', 5, 5, ( 
 ( #41085, #30476, #5279, #39434, #108840, #22592 ),
 ( #107739, #22044, #75262, #31024, #83092, #23169 ),
 ( #91496, #31576, #65753, #107187, #65205, #99318 ),
 ( #73610, #109411, #39983, #64664, #99870, #98781 ),
 ( #6928, #32687, #56241, #56795, #90932, #74159 ),
 ( #57369, #108290, #81971, #32137, #14219, #66322 ),
 ( #48405, #5843, #14775, #15314, #82549, #23723 ),
 ( #48961, #6385, #40533, #74709, #90370, #100440 ),
 ( #13648, #57908, #92042, #49507, #47838, #83632 ),
 ( #2918, #30277, #4545, #54426, #37035, #47646 ),
 ( #106989, #38135, #5078, #80144, #38679, #39228 ),
 ( #11842, #81775, #64470, #63382, #94878, #89637 ),
 ( #88020, #98585, #88559, #21851, #71230, #46013 ),
 ( #98032, #56048, #90175, #72316, #11304, #55509 ),
 ( #72855, #3463, #29191, #73404, #106448, #13457 ),
 ( #107541, #63917, #30829, #71793, #29731, #19678 ),
 ( #53883, #105352, #105912, #12924, #37591, #21304 ),
 ( #45472, #47104, #12379, #79614, #89092, #80700 ),
 ( #28642, #97498, #62846, #96959, #20766, #20225 ),
 ( #54965, #46566, #81230, #4010, #108084, #57170 ),
 ( #92940, #83431, #49856, #91293, #39795, #92378 ),
 ( #40334, #31379, #14574, #108645, #31931, #16212 ),
 ( #74515, #67218, #15650, #24064, #91838, #50415 ),
 ( #66125, #82346, #109749, #83989, #22962, #5645 ),
 ( #75064, #75616, #6728, #84540, #48763, #7289 ),
 ( #41451, #49306, #7829, #90734, #82890, #40884 ),
 ( #22400, #101314, #100249, #109214, #57720, #42000 ) ),
 .UNSPECIFIED., .F., .F., .F.,
 ( 6, 3, 3, 3, 3, 3, 3, 3, 6 ),
 ( 6, 6 ),
 ( 50.96205257140000100, 60.48206970939999394, 63.97289610280000005, 65.71830929959999423, 66.59101589789999309, 67.46372249629999374, 67.82259044730000141, 68.73290467190000186, 70.00208684739999399 ),
 ( 0.000000000000000000, 1.468559632160000072 ),
 .UNSPECIFIED. ) ;
#77679=CARTESIAN_POINT ( 'NONE',  ( -1.527346172629999943, 1467.905318097929921, 230.2847532987979946 ) ) ;
#77682=CARTESIAN_POINT ( 'NONE',  ( -0.05914945545369999780, 1451.662743606630102, 154.0810024862979901 ) ) ;
#77690=DIRECTION ( 'NONE',  ( -0.03206683765522939239, -0.9990097422274648586, 0.03084238734935479398 ) ) ;
#77693=CARTESIAN_POINT ( 'NONE',  ( 18.17240998359999793, 1509.561555716230032, 232.4487212659979889 ) ) ;
#77696=CARTESIAN_POINT ( 'NONE',  ( 37.77063578043529901, 1438.437603869379700, 136.5939142087520111 ) ) ;
#77697=CARTESIAN_POINT ( 'NONE',  ( 10.92533434161652828, 1411.430006105364782, 269.3500472981405096 ) ) ;
#77698=CARTESIAN_POINT ( 'NONE',  ( 3.374205057650000136E-09, 1472.348783246430003, 259.9484461764980097 ) ) ;
#77704=CARTESIAN_POINT ( 'NONE',  ( -12.79212758865954846, 1435.914429446145050, 150.8331423002523763 ) ) ;
#77706=CARTESIAN_POINT ( 'NONE',  ( 2.985074718659999959, 1409.521906423129849, 185.9264304420979954 ) ) ;
#77707=CARTESIAN_POINT ( 'NONE',  ( 13.15671565689999944, 1428.802034784529951, 222.6511392629980151 ) ) ;
#77708=CARTESIAN_POINT ( 'NONE',  ( -6.472929290989999807, 1440.851741214640015, 154.4738949224980047 ) ) ;
#77709=CARTESIAN_POINT ( 'NONE',  ( 11.70596015200000117, 1435.783535252809997, 151.4055867023980113 ) ) ;
#77711=AXIS2_PLACEMENT_3D ( 'NONE', #12824, #106339, #72217 ) ;
#77712=EDGE_CURVE ( 'NONE', #104308, #74738, #28085, .T. ) ;
#77713=CARTESIAN_POINT ( 'NONE',  ( -3.415166128929299827, 1451.477990676830132, 184.8447288809229860 ) ) ;
#77714=CARTESIAN_POINT ( 'NONE',  ( 0.1613156720539999922, 1465.436708526229950, 236.3249312579980028 ) ) ;
#77717=CARTESIAN_POINT ( 'NONE',  ( -41.93729219490000304, 1443.867285198199852, 269.6463924139980008 ) ) ;
#77718=CARTESIAN_POINT ( 'NONE',  ( 11.88064286090000010, 1433.444786854229960, 151.0525681022980109 ) ) ;
#77723=CARTESIAN_POINT ( 'NONE',  ( -5.100895039060000080, 1418.043138886930137, 233.8666107664980132 ) ) ;
#77727=CARTESIAN_POINT ( 'NONE',  ( -45.77324011850739538, 1438.474511334749877, 266.4156763373180183 ) ) ;
#77728=CARTESIAN_POINT ( 'NONE',  ( -2.694116389579999993, 1425.979849364829988, 185.2590652528979831 ) ) ;
#77731=ORIENTED_EDGE ( 'NONE', *, *, #93987, .T. ) ;
#77733=CARTESIAN_POINT ( 'NONE',  ( -2.478673243200000265, 1436.180421119320044, 157.6364458798979911 ) ) ;
#77736=CARTESIAN_POINT ( 'NONE',  ( -26.33488014430039925, 1451.993447629259890, 134.9643013293120077 ) ) ;
#77737=VERTEX_POINT ( 'NONE', #3028 ) ;
#77738=CARTESIAN_POINT ( 'NONE',  ( -14.45358395259999895, 1470.808655613429892, 194.4307210385980227 ) ) ;
#77740=CARTESIAN_POINT ( 'NONE',  ( 13.71645562369999993, 1434.810047171300084, 195.7796452459980117 ) ) ;
#77741=B_SPLINE_CURVE_WITH_KNOTS ( 'NONE', 5,
 ( #100679, #83887, #104974, #89818, #71420, #55149 ),
 .UNSPECIFIED., .F., .F.,
 ( 6, 6 ),
 ( -74.30665799839999863, -17.67736075759999892 ),
 .UNSPECIFIED. ) ;
#77742=EDGE_CURVE ( 'NONE', #76242, #74812, #1775, .T. ) ;
#77744=CARTESIAN_POINT ( 'NONE',  ( 11.60004869885203860, 1424.140503711560086, 136.0100193273773357 ) ) ;
#77746=CARTESIAN_POINT ( 'NONE',  ( -14.45750500688560081, 1416.828039245989885, 221.3916439204320170 ) ) ;
#77747=FACE_OUTER_BOUND ( 'NONE', #74012, .T. ) ;
#77749=CARTESIAN_POINT ( 'NONE',  ( -4.355561652949340612, 1408.080063563500062, 270.2891561468720170 ) ) ;
#77751=CARTESIAN_POINT ( 'NONE',  ( 8.767012977189999390, 1418.317283281629898, 230.8509917594979868 ) ) ;
#77754=EDGE_LOOP ( 'NONE', ( #19200, #17402, #64897, #69800 ) ) ;
#77757=CARTESIAN_POINT ( 'NONE',  ( -0.004805506605713849924, 1408.913228200830190, 186.0222358698079859 ) ) ;
#77759=CARTESIAN_POINT ( 'NONE',  ( -18.72591792251515486, 1409.005171047454724, 266.8216848252018281 ) ) ;
#77760=CARTESIAN_POINT ( 'NONE',  ( -18.83966063982870054, 1437.724940806150016, 194.4009572081200190 ) ) ;
#77761=CARTESIAN_POINT ( 'NONE',  ( -19.04810011320000029, 1425.814708983130231, 224.2238500513979886 ) ) ;
#77762=CARTESIAN_POINT ( 'NONE',  ( 28.38017910033849844, 1468.283441186749997, 268.9888031847070238 ) ) ;
#77763=CARTESIAN_POINT ( 'NONE',  ( -3.301631116843481983, 1466.760662549056860, 234.9475888533459056 ) ) ;
#77764=CARTESIAN_POINT ( 'NONE',  ( -16.97240415505549294, 1421.991001403454675, 226.8235528602522777 ) ) ;
#77766=ORIENTED_EDGE ( 'NONE', *, *, #76681, .F. ) ;
#77767=CARTESIAN_POINT ( 'NONE',  ( 19.02527238669184584, 1457.194456449220070, 226.3937467632252378 ) ) ;
#77768=CARTESIAN_POINT ( 'NONE',  ( 1.477399147100459942, 1480.042335471780007, 182.2939015677119983 ) ) ;
#77769=CARTESIAN_POINT ( 'NONE',  ( 23.55027989260000254, 1410.975381342730088, 207.7696266105379834 ) ) ;
#77772=CARTESIAN_POINT ( 'NONE',  ( 25.74980778770000001, 1451.774094166629993, 136.0745756758980178 ) ) ;
#77776=CARTESIAN_POINT ( 'NONE',  ( 17.05796332999999976, 1409.508737592730085, 194.6785584388979942 ) ) ;
#77778=CARTESIAN_POINT ( 'NONE',  ( 17.22592482065188335, 1444.324653571828321, 162.9227486220069352 ) ) ;
#77780=CARTESIAN_POINT ( 'NONE',  ( 3.771179646140724540, 1439.700054869645101, 184.6351339312261643 ) ) ;
#77781=CARTESIAN_POINT ( 'NONE',  ( 1.319771658879999920, 1416.088550827329982, 232.9278251303979914 ) ) ;
#77782=CARTESIAN_POINT ( 'NONE',  ( -19.25680457745775698, 1425.292773199313388, 223.7995632996566826 ) ) ;
#77783=CARTESIAN_POINT ( 'NONE',  ( 1.304065981556200127, 1452.805067748419788, 183.4358032751680128 ) ) ;
#77788=ORIENTED_EDGE ( 'NONE', *, *, #48546, .F. ) ;
#77790=CARTESIAN_POINT ( 'NONE',  ( 11.77504716261359974, 1432.336839668820176, 150.6178349985629836 ) ) ;
#77791=CARTESIAN_POINT ( 'NONE',  ( -0.3329445438763140031, 1408.995598260099996, 232.2005901765320175 ) ) ;
#77794=CARTESIAN_POINT ( 'NONE',  ( -8.301987938657498844, 1512.913060387330006, 185.0111222839169898 ) ) ;
#77796=CARTESIAN_POINT ( 'NONE',  ( -2.984513020910000147, 1453.913060387330006, 209.1218459616979999 ) ) ;
#77797=CARTESIAN_POINT ( 'NONE',  ( 43.12279225419995043, 1452.630096070929540, 266.2619628294978043 ) ) ;
#77798=CARTESIAN_POINT ( 'NONE',  ( 11.91185892230000043, 1433.366769854990025, 149.9329001653979674 ) ) ;
#77799=CARTESIAN_POINT ( 'NONE',  ( 8.518323191219998591, 1460.717990419130047, 243.9198229383979992 ) ) ;
#77805=CARTESIAN_POINT ( 'NONE',  ( -13.67685946489999971, 1486.238555760329973, 185.2440325359980022 ) ) ;
#77806=CARTESIAN_POINT ( 'NONE',  ( 9.119196661296259165, 1398.183650043934222, 199.8491675525386313 ) ) ;
#77807=CARTESIAN_POINT ( 'NONE',  ( -21.91919261220000337, 1509.808421474629995, 231.8378097518979928 ) ) ;
#77808=CARTESIAN_POINT ( 'NONE',  ( 20.81017606039999990, 1469.236365764530092, 223.5860970572980193 ) ) ;
#77809=CARTESIAN_POINT ( 'NONE',  ( 4.054153981253102224, 1446.253642626345709, 170.5365981473220813 ) ) ;
#77812=AXIS2_PLACEMENT_3D ( 'NONE', #30385, #90283, #81330 ) ;
#77816=CARTESIAN_POINT ( 'NONE',  ( 0.1616823930634609940, 1485.255944980259983, 181.8685822356719939 ) ) ;
#77818=ORIENTED_EDGE ( 'NONE', *, *, #22334, .F. ) ;
#77819=CARTESIAN_POINT ( 'NONE',  ( -1.341950169539999793, 1416.837177091229705, 228.0806925298979877 ) ) ;
#77821=EDGE_CURVE ( 'NONE', #16145, #59173, #20948, .T. ) ;
#77823=CARTESIAN_POINT ( 'NONE',  ( -33.91369120143989591, 1451.728768194249824, 134.0999999980979851 ) ) ;
#77829=CARTESIAN_POINT ( 'NONE',  ( -15.13954165719999878, 1415.426091369430196, 218.9613120750979931 ) ) ;
#77832=DIRECTION ( 'NONE',  ( -0.07222731439955003274, -0.9674608870543032202, 0.2424925711743135259 ) ) ;
#77836=CARTESIAN_POINT ( 'NONE',  ( -17.67020261369999901, 1412.966317095329941, 192.9698263009980224 ) ) ;
#77837=CYLINDRICAL_SURFACE ( 'NONE', #78796, 2.000000000000001776 ) ;
#77838=ORIENTED_EDGE ( 'NONE', *, *, #110454, .T. ) ;
#77840=EDGE_CURVE ( 'NONE', #6139, #32742, #56492, .T. ) ;
#77843=DIRECTION ( 'NONE',  ( 0.000000000000000000, 1.000000000000000000, 0.000000000000000000 ) ) ;
#77850=CARTESIAN_POINT ( 'NONE',  ( 35.92105933033366938, 1456.729054770310313, 269.5445013229119127 ) ) ;
#77851=CARTESIAN_POINT ( 'NONE',  ( 21.13431379670319998, 1409.651086887829933, 206.4149708788170301 ) ) ;
#77852=CARTESIAN_POINT ( 'NONE',  ( 6.240887162079999939, 1397.787773554729938, 220.5258548213979850 ) ) ;
#77853=DIRECTION ( 'NONE',  ( -1.000000000000000000, 0.000000000000000000, 0.000000000000000000 ) ) ;
#77859=DIRECTION ( 'NONE',  ( 0.000000000000000000, -1.000000000000000000, 0.000000000000000000 ) ) ;
#77860=CARTESIAN_POINT ( 'NONE',  ( 31.97288361449999883, 1465.739487317430076, 269.9246165631980148 ) ) ;
#77862=ORIENTED_EDGE ( 'NONE', *, *, #82871, .T. ) ;
#77865=CARTESIAN_POINT ( 'NONE',  ( 26.19682441240000159, 1416.543454811029733, 259.6167016350979679 ) ) ;
#77866=CARTESIAN_POINT ( 'NONE',  ( -23.83044711870000043, 1430.353408626829832, 204.6119512178680111 ) ) ;
#77867=CARTESIAN_POINT ( 'NONE',  ( -11.61158519821730017, 1426.364169946740049, 135.2602023053949836 ) ) ;
#77869=CARTESIAN_POINT ( 'NONE',  ( 16.39238061357189835, 1409.586354316659936, 192.5911623901700125 ) ) ;
#77873=CARTESIAN_POINT ( 'NONE',  ( -22.64731540989999914, 1507.637957906029897, 208.5229870085950097 ) ) ;
#77874=CARTESIAN_POINT ( 'NONE',  ( -40.44435334479999966, 1427.769454619329963, 264.0385764254980359 ) ) ;
#77875=CARTESIAN_POINT ( 'NONE',  ( 18.36180303385479817, 1509.570204029540037, 232.3072875949450236 ) ) ;
#77876=CARTESIAN_POINT ( 'NONE',  ( 29.40921901591849874, 1509.877385647309893, 209.6267707321559897 ) ) ;
#77878=CARTESIAN_POINT ( 'NONE',  ( -34.71462694457399323, 1437.089205478310078, 136.5423016297559968 ) ) ;
#77880=CARTESIAN_POINT ( 'NONE',  ( 12.47743726298899958, 1397.381078991009872, 213.9104067551370179 ) ) ;
#77882=CARTESIAN_POINT ( 'NONE',  ( -16.78297372800000176, 1460.265260285829982, 228.3353414857980113 ) ) ;
#77884=ORIENTED_EDGE ( 'NONE', *, *, #100590, .T. ) ;
#77885=CARTESIAN_POINT ( 'NONE',  ( -29.24222810794026728, 1509.934246511754054, 211.7448759012906976 ) ) ;
#77890=CARTESIAN_POINT ( 'NONE',  ( 22.28696231330000188, 1506.798305107829947, 209.3970118511340104 ) ) ;
#77891=CARTESIAN_POINT ( 'NONE',  ( -12.89099770320000005, 1461.186125398530066, 230.5721238860979838 ) ) ;
#77901=CARTESIAN_POINT ( 'NONE',  ( 11.74890926396520108, 1426.742300306969810, 145.0013950776020124 ) ) ;
#77902=CARTESIAN_POINT ( 'NONE',  ( 12.83373743668885503, 1444.966504083088466, 186.6095280254539830 ) ) ;
#77904=CARTESIAN_POINT ( 'NONE',  ( 9.048691962705447622, 1423.897446184702403, 139.1407012399385223 ) ) ;
#77906=CARTESIAN_POINT ( 'NONE',  ( 7.315253172540000293, 1509.168514657129890, 237.2865368194979965 ) ) ;
#77907=AXIS2_PLACEMENT_3D ( 'NONE', #103642, #19057, #96902 ) ;
#77909=CARTESIAN_POINT ( 'NONE',  ( -4.954458045509999131, 1424.150364743330101, 185.8728153432979866 ) ) ;
#77910=CARTESIAN_POINT ( 'NONE',  ( 3.530738010049999875, 1408.338100458330018, 270.3906828179979698 ) ) ;
#77911=CARTESIAN_POINT ( 'NONE',  ( -3.500000000000000000, 1407.163060387330006, 146.1721969590979882 ) ) ;
#77916=CARTESIAN_POINT ( 'NONE',  ( 14.45783194710000075, 1416.839692140529905, 196.8516150077980171 ) ) ;
#77917=CARTESIAN_POINT ( 'NONE',  ( -4.573812764092838101, 1423.750333358086891, 184.3978805773018905 ) ) ;
#77918=CARTESIAN_POINT ( 'NONE',  ( 17.81052644217599834, 1417.511519687270038, 225.0007343307930228 ) ) ;
#77919=CARTESIAN_POINT ( 'NONE',  ( -9.052208719341413357, 1506.643733544970701, 188.8170897969911266 ) ) ;
#77920=ORIENTED_EDGE ( 'NONE', *, *, #85881, .T. ) ;
#77923=CARTESIAN_POINT ( 'NONE',  ( -2.941051375418705760, 1485.222273148426211, 183.0255250225658870 ) ) ;
#77927=CARTESIAN_POINT ( 'NONE',  ( 17.10420012035890025, 1414.913526845469960, 210.6212183496899968 ) ) ;
#77929=CARTESIAN_POINT ( 'NONE',  ( -11.49189579029999919, 1426.655527037130241, 148.3077481762979914 ) ) ;
#77933=CARTESIAN_POINT ( 'NONE',  ( 13.18752275098719906, 1428.876431498459851, 222.4037147343619836 ) ) ;
#77935=CARTESIAN_POINT ( 'NONE',  ( 9.265269351469999748, 1412.734572620129939, 230.2246370649980065 ) ) ;
#77937=CARTESIAN_POINT ( 'NONE',  ( -15.83861837100000081, 1459.345690884129908, 229.6260692152980027 ) ) ;
#77939=CARTESIAN_POINT ( 'NONE',  ( 31.52953872790000034, 1415.569331350129914, 268.9168057298979306 ) ) ;
#77940=CARTESIAN_POINT ( 'NONE',  ( 1.963370004590500262, 1464.924280329780913, 237.5709148626887952 ) ) ;
#77941=CARTESIAN_POINT ( 'NONE',  ( 20.81072686770000146, 1430.297633082429911, 197.0877802440980133 ) ) ;
#77942=CARTESIAN_POINT ( 'NONE',  ( -23.34239156850000185, 1434.464133788829940, 214.4674836295579894 ) ) ;
#77944=CARTESIAN_POINT ( 'NONE',  ( -10.10004869885203682, 1425.894669202444675, 137.5118601406020673 ) ) ;
#77946=CARTESIAN_POINT ( 'NONE',  ( 8.759919950853198856, 1423.587268813439778, 144.1551655176990039 ) ) ;
#77948=CARTESIAN_POINT ( 'NONE',  ( -6.688849035430000534, 1408.965348140629885, 196.7627783224980078 ) ) ;
#77949=CARTESIAN_POINT ( 'NONE',  ( -16.25813024210000179, 1415.087797054229895, 203.3133064409179838 ) ) ;
#77950=CARTESIAN_POINT ( 'NONE',  ( -12.71183112859999831, 1441.878635263719843, 187.9184463588980236 ) ) ;
#77952=B_SPLINE_SURFACE_WITH_KNOTS ( 'NONE', 5, 5, ( 
 ( #4211, #27886, #68808, #52549, #70472, #104591 ),
 ( #78282, #9426, #27326, #43590, #86681, #21523 ),
 ( #81433, #77738, #62069, #35732, #102910, #80915 ),
 ( #38342, #29941, #64133, #9976, #98254, #60398 ),
 ( #55735, #26776, #100460, #31046, #90955, #47860 ),
 ( #107762, #40556, #32708, #66344, #83116, #15336 ) ),
 .UNSPECIFIED., .F., .F., .F.,
 ( 6, 6 ),
 ( 6, 6 ),
 ( 30.40177460629999828, 157.7844419379999863 ),
 ( -6.245004513519998715E-17, 1.000000000000000000 ),
 .UNSPECIFIED. ) ;
#77953=CARTESIAN_POINT ( 'NONE',  ( -33.92723112960000265, 1435.682240498669898, 135.5030908497980136 ) ) ;
#77957=CARTESIAN_POINT ( 'NONE',  ( -11.52135570437129886, 1409.315394994109965, 199.5950662629080057 ) ) ;
#77959=CARTESIAN_POINT ( 'NONE',  ( -12.67256029850000054, 1474.517343106330145, 266.8981073570980129 ) ) ;
#77965=CARTESIAN_POINT ( 'NONE',  ( 18.04679706737850253, 1424.839701421730069, 226.5258000463729786 ) ) ;
#77966=CARTESIAN_POINT ( 'NONE',  ( 21.92068900019999944, 1509.678547715230025, 227.8376466598980130 ) ) ;
#77967=CARTESIAN_POINT ( 'NONE',  ( 14.37537801800000103, 1463.298671107329938, 223.1724039782979787 ) ) ;
#77969=CARTESIAN_POINT ( 'NONE',  ( -26.86198109714170101, 1508.007473140129832, 212.0127264923079906 ) ) ;
#77971=CARTESIAN_POINT ( 'NONE',  ( -5.688831827459999602, 1508.347319533530253, 181.0331735192980034 ) ) ;
#77973=CARTESIAN_POINT ( 'NONE',  ( -22.29341197009999931, 1409.691563488129987, 205.7443763409079907 ) ) ;
#77974=CARTESIAN_POINT ( 'NONE',  ( 16.36865316639999790, 1414.913060387329779, 208.9007811298039883 ) ) ;
#77977=CARTESIAN_POINT ( 'NONE',  ( -1.127597643542621819, 1410.331959298673837, 233.0285034547154055 ) ) ;
#77981=( BOUNDED_SURFACE ( )  B_SPLINE_SURFACE ( 1, 2, ( 
 ( #65650, #39330, #14110 ),
 ( #64560, #80792, #98679 ) ),
 .UNSPECIFIED., .F., .F., .F. ) 
 B_SPLINE_SURFACE_WITH_KNOTS ( ( 2, 2 ),
 ( 3, 3 ),
 ( -10000.00000000000000, 10000.00000000000000 ),
 ( 5.300753508068379638, 6.146881668033620016 ),
 .UNSPECIFIED. ) 
 GEOMETRIC_REPRESENTATION_ITEM ( )  RATIONAL_B_SPLINE_SURFACE ( (
 ( 0.8627701935022120683, 0.8231901671891870276, 0.9535799773170169358),
 ( 0.8627701935022120683, 0.8231901671891870276, 0.9535799773170169358) ) ) 
 REPRESENTATION_ITEM ( '' )  SURFACE ( )  );
#77983=CARTESIAN_POINT ( 'NONE',  ( 11.07188855578698039, 1414.941240495246575, 222.3943915280714521 ) ) ;
#77988=CARTESIAN_POINT ( 'NONE',  ( -1.203807798849710009, 1419.233902311370002, 185.0625641774459780 ) ) ;
#77990=CARTESIAN_POINT ( 'NONE',  ( -5.116792858579263026, 1398.065454244455623, 221.0739902772355663 ) ) ;
#77993=CARTESIAN_POINT ( 'NONE',  ( -19.81810597710000010, 1468.980723873930174, 193.4065930840980059 ) ) ;
#77997=ORIENTED_EDGE ( 'NONE', *, *, #107812, .T. ) ;
#77999=CARTESIAN_POINT ( 'NONE',  ( 11.33466614171230091, 1434.021404067120102, 151.4990630526469886 ) ) ;
#78003=CARTESIAN_POINT ( 'NONE',  ( -24.21946005650000089, 1509.534793663830214, 195.2515658952980004 ) ) ;
#78005=CARTESIAN_POINT ( 'NONE',  ( 16.34335051667209981, 1433.455134956249822, 190.8190931015600142 ) ) ;
#78007=CARTESIAN_POINT ( 'NONE',  ( 13.70362658034589920, 1498.107102624340087, 232.4496494982320201 ) ) ;
#78008=CARTESIAN_POINT ( 'NONE',  ( 0.4496490820779999731, 1488.176790722930036, 181.7536822793979638 ) ) ;
#78011=CARTESIAN_POINT ( 'NONE',  ( 37.65468647792339851, 1436.753545005050000, 134.0999999968539953 ) ) ;
#78014=VERTEX_POINT ( 'NONE', #20332 ) ;
#78015=CARTESIAN_POINT ( 'NONE',  ( 13.76342018928679956, 1434.978124368779845, 148.5737756231810351 ) ) ;
#78016=ORIENTED_EDGE ( 'NONE', *, *, #82382, .F. ) ;
#78020=CARTESIAN_POINT ( 'NONE',  ( -1.103937759919999984, 1466.689616642629971, 235.4490393618980022 ) ) ;
#78022=B_SPLINE_CURVE_WITH_KNOTS ( 'NONE', 5,
 ( #110685, #32867, #110137, #8212, #101164, #33410 ),
 .UNSPECIFIED., .F., .F.,
 ( 6, 6 ),
 ( 0.000000000000000000, 1.000000000000000000 ),
 .UNSPECIFIED. ) ;
#78025=CARTESIAN_POINT ( 'NONE',  ( -18.99986283518648023, 1443.243851081979983, 211.4893642521566051 ) ) ;
#78027=CARTESIAN_POINT ( 'NONE',  ( 4.240875174286579785, 1446.389522495240044, 162.6875343836649961 ) ) ;
#78029=EDGE_LOOP ( 'NONE', ( #86250, #77284, #14615, #76925, #79765, #16461, #86456 ) ) ;
#78031=ORIENTED_EDGE ( 'NONE', *, *, #98649, .F. ) ;
#78033=CARTESIAN_POINT ( 'NONE',  ( -18.93308225230000019, 1509.362410706630044, 230.7219330744979686 ) ) ;
#78035=CARTESIAN_POINT ( 'NONE',  ( 27.12879168973760002, 1450.023363157879885, 136.5580283348670037 ) ) ;
#78036=CARTESIAN_POINT ( 'NONE',  ( -14.86692150049999839, 1409.934051351630160, 190.9079559787980145 ) ) ;
#78037=CARTESIAN_POINT ( 'NONE',  ( -24.38138454299999935, 1442.062445815139881, 212.1316645750080170 ) ) ;
#78040=CARTESIAN_POINT ( 'NONE',  ( -13.34384734591514565, 1434.923148256851618, 146.7534062989944914 ) ) ;
#78043=CARTESIAN_POINT ( 'NONE',  ( -26.13601501283269712, 1491.681802943529874, 212.0165345522650000 ) ) ;
#78047=VECTOR ( 'NONE', #25776, 1000.000000000000000 ) ;
#78048=DIRECTION ( 'NONE',  ( 0.4794255386041986200, 0.000000000000000000, 0.8775825618903752012 ) ) ;
#78049=CARTESIAN_POINT ( 'NONE',  ( 29.39269299460000084, 1509.939475844130129, 206.8231667076280189 ) ) ;
#78052=EDGE_CURVE ( 'NONE', #6924, #5604, #23151, .T. ) ;
#78053=CARTESIAN_POINT ( 'NONE',  ( 14.77051248179999909, 1409.598147030530072, 192.0760700751979755 ) ) ;
#78058=CARTESIAN_POINT ( 'NONE',  ( 39.71670573500000501, 1440.913060382410094, 259.0959246117979546 ) ) ;
#78059=ADVANCED_FACE ( 'NONE', ( #64028 ), #31187, .T. ) ;
#78060=CARTESIAN_POINT ( 'NONE',  ( 3.052254580091493530, 1451.555641073906145, 183.9065986230910426 ) ) ;
#78063=CARTESIAN_POINT ( 'NONE',  ( -2.556789166010999814, 1507.689321980810064, 237.0181741517399985 ) ) ;
#78065=CARTESIAN_POINT ( 'NONE',  ( -19.87162007319999901, 1456.113380717730024, 225.4101704608979730 ) ) ;
#78066=CARTESIAN_POINT ( 'NONE',  ( 10.97356389379999975, 1432.589699276930105, 151.7700026489980019 ) ) ;
#78068=CARTESIAN_POINT ( 'NONE',  ( -0.3822501820940000239, 1506.811133726930166, 187.1259390350979857 ) ) ;
#78072=CARTESIAN_POINT ( 'NONE',  ( 0.5565654927739999147, 1405.991402147929875, 266.9610393333979914 ) ) ;
#78073=CARTESIAN_POINT ( 'NONE',  ( 28.26671296840000025, 1509.671138067530137, 207.1993025267279904 ) ) ;
#78074=CARTESIAN_POINT ( 'NONE',  ( -4.754578092089379674E-06, 1472.619500892389851, 270.3713690308879904 ) ) ;
#78075=CARTESIAN_POINT ( 'NONE',  ( 5.418632516149999745, 1435.861377308850024, 154.6842388019980206 ) ) ;
#78078=CARTESIAN_POINT ( 'NONE',  ( -20.65862765212969876, 1509.573540226620253, 188.2595568902629850 ) ) ;
#78080=CARTESIAN_POINT ( 'NONE',  ( -26.05451239549999798, 1447.172171551439988, 137.7976690009980132 ) ) ;
#78081=CARTESIAN_POINT ( 'NONE',  ( -0.8724913965011420469, 1450.882592297439942, 154.2430449224139863 ) ) ;
#78088=CARTESIAN_POINT ( 'NONE',  ( 1.608351468689999786, 1426.598937817530214, 144.1938086916980239 ) ) ;
#78089=CARTESIAN_POINT ( 'NONE',  ( 12.40447486740000116, 1434.419892962859876, 146.9204490281980213 ) ) ;
#78091=CARTESIAN_POINT ( 'NONE',  ( -1.260684556148445212, 1450.744076110377364, 181.7878351591420767 ) ) ;
#78092=CARTESIAN_POINT ( 'NONE',  ( 15.36367305140250039, 1457.934436068309878, 189.6495915026669934 ) ) ;
#78093=CARTESIAN_POINT ( 'NONE',  ( -1.282992545539999837E-09, 1475.759805456229969, 269.0456997843980389 ) ) ;
#78098=CARTESIAN_POINT ( 'NONE',  ( -18.47106347599999765, 1415.579607678529783, 207.7286614539779634 ) ) ;
#78099=B_SPLINE_CURVE_WITH_KNOTS ( 'NONE', 5,
 ( #5762, #108202, #12501, #39904, #47758, #55632 ),
 .UNSPECIFIED., .F., .F.,
 ( 6, 6 ),
 ( -65.26196056268710777, -30.37524181780000276 ),
 .UNSPECIFIED. ) ;
#78100=CARTESIAN_POINT ( 'NONE',  ( -18.09157779502649888, 1416.524489948229984, 209.2020736640780001 ) ) ;
#78101=CARTESIAN_POINT ( 'NONE',  ( 18.64672481363430379, 1416.851343896850040, 209.6839434896919840 ) ) ;
#78102=CARTESIAN_POINT ( 'NONE',  ( -13.45503186213775138, 1443.537314858658419, 169.3628516250983012 ) ) ;
#78103=ORIENTED_EDGE ( 'NONE', *, *, #49528, .F. ) ;
#78104=CARTESIAN_POINT ( 'NONE',  ( -16.25887119586559848, 1409.480822287279807, 225.0886774072699836 ) ) ;
#78105=CARTESIAN_POINT ( 'NONE',  ( 9.821550493440000196, 1443.913060387330006, 148.8455630174979945 ) ) ;
#78112=CARTESIAN_POINT ( 'NONE',  ( -11.87010322290000097, 1433.046492610579890, 150.1772076958980051 ) ) ;
#78113=CARTESIAN_POINT ( 'NONE',  ( -2.822636040217339826, 1419.812953946676771, 186.1531589886093911 ) ) ;
#78117=CARTESIAN_POINT ( 'NONE',  ( 3.732008881810000123, 1450.492772364150142, 184.1420057466980040 ) ) ;
#78120=ORIENTED_EDGE ( 'NONE', *, *, #91352, .F. ) ;
#78121=ORIENTED_EDGE ( 'NONE', *, *, #45505, .T. ) ;
#78122=CARTESIAN_POINT ( 'NONE',  ( -12.33746580920000113, 1440.929426004120160, 187.9427475994980057 ) ) ;
#78124=CARTESIAN_POINT ( 'NONE',  ( -0.9866794285430001699, 1473.892698774330029, 270.2925939122980594 ) ) ;
#78126=CARTESIAN_POINT ( 'NONE',  ( -1.314910794049999776, 1486.515044105329935, 181.6997297598980197 ) ) ;
#78129=CARTESIAN_POINT ( 'NONE',  ( 21.99779757700000005, 1409.845346003030045, 206.2854406303680150 ) ) ;
#78131=CARTESIAN_POINT ( 'NONE',  ( -2.500000000000000000, 1448.561607529700041, 159.6824365648180049 ) ) ;
#78133=CARTESIAN_POINT ( 'NONE',  ( 13.38380976650000065, 1409.321262751630002, 216.4729699453379794 ) ) ;
#78134=CARTESIAN_POINT ( 'NONE',  ( -2.267841090553740280, 1406.812775593299875, 269.6487269905239827 ) ) ;
#78136=ORIENTED_EDGE ( 'NONE', *, *, #53056, .F. ) ;
#78137=CARTESIAN_POINT ( 'NONE',  ( -10.96941897680000011, 1432.344069211809938, 151.7701285249980003 ) ) ;
#78138=CARTESIAN_POINT ( 'NONE',  ( 13.54145629459999967, 1443.508061120249977, 188.5908682209980327 ) ) ;
#78139=ORIENTED_EDGE ( 'NONE', *, *, #53572, .F. ) ;
#78140=EDGE_LOOP ( 'NONE', ( #13216, #88972, #30229, #80031, #79867, #25779, #29250, #72380, #10121, #82415, #6134, #102153, #16223, #77731 ) ) ;
#78142=B_SPLINE_CURVE_WITH_KNOTS ( 'NONE', 3,
 ( #31536, #56756, #5804, #39945, #74115, #48921, #65711, #99833, #23124, #57329, #6342, #40490, #32094, #94754, #59517, #79084, #102034, #77957, #85800, #86908, #60076, #26436, #1263, #93629, #70152, #18574, #52769, #43263, #94192, #27009, #19127, #61197, #34294, #10198, #69590, #18032, #25320, #42706, #52224, #68477, #44373, #51662, #35964, #60631, #87476, #9635, #17461, #86351, #78518, #44937, #16907, #27554, #9098, #77410, #1829, #95314, #43807, #103708, #35402, #36507, #104264, #34844, #61736, #95860, #716, #51113, #8531, #53328, #10766, #2391, #85237, #76862, #102578, #25874, #69035, #103136, #173, #98605, #88036, #13479, #53901, #70703, #81797, #54443, #79632, #12398, #5099, #28662, #11320, #54985, #55529, #38698, #63937, #3482, #30297, #72874, #81249, #96420, #89110, #37610, #19698, #4564, #62867, #45491, #71812, #2936, #64490, #4027, #63400, #21869, #97516, #28102, #47669, #104814, #46584, #88577, #89655, #96979, #56068, #37053, #11860 ),
 .UNSPECIFIED., .F., .F.,
 ( 4, 3, 3, 3, 3, 3, 3, 3, 3, 3, 3, 3, 3, 3, 3, 3, 3, 3, 3, 3, 3, 3, 3, 3, 3, 3, 3, 3, 3, 3, 3, 3, 3, 3, 3, 3, 3, 3, 3, 3, 4 ),
 ( 15.94786254319999941, 17.28652221311410031, 18.62887769919689873, 19.97220876837939940, 21.31551003014599743, 22.65777570309839817, 23.99648260799839861, 25.33228087000049911, 26.66197833009550067, 27.90025324481390356, 29.21922251675360016, 30.54537470099209884, 31.87781318686680265, 33.21548123473309744, 34.55717461623120101, 35.90156568275600080, 37.27590617873740086, 38.62028396294829946, 39.96291520885479542, 41.30221225282429032, 42.70073160226989728, 44.02712524576659803, 45.34784220011430023, 46.65983834663869345, 46.89628965060690291, 48.21084064340449515, 49.53265281890470817, 50.86114174345969730, 52.24619684876979875, 53.58794959607750741, 54.99465588038880526, 56.40136216470000363, 57.75144886590140914, 59.10083358886660676, 60.44821813932610155, 61.79246594079870647, 63.13251995115560078, 64.46420547887859698, 65.79044557759550571, 67.10676169860950324, 68.30549982530000364 ),
 .UNSPECIFIED. ) ;
#78154=CARTESIAN_POINT ( 'NONE',  ( -27.56049296109999958, 1508.045672656129909, 205.3679835307079884 ) ) ;
#78158=CARTESIAN_POINT ( 'NONE',  ( -4.305815836009999842, 1409.063422789429978, 194.9846847171979789 ) ) ;
#78160=CARTESIAN_POINT ( 'NONE',  ( -10.82839717969999960, 1445.293858117500122, 185.2652248665980039 ) ) ;
#78163=CARTESIAN_POINT ( 'NONE',  ( 22.56155900549999771, 1488.679832657330053, 222.5656005121980172 ) ) ;
#78164=CARTESIAN_POINT ( 'NONE',  ( 19.47156422787159968, 1467.105613706720078, 225.2196683951030138 ) ) ;
#78165=CARTESIAN_POINT ( 'NONE',  ( -25.15095490240000231, 1436.448645567330004, 137.6015634021979679 ) ) ;
#78171=CARTESIAN_POINT ( 'NONE',  ( -11.60004869885203860, 1423.633889433519244, 135.8155558205586999 ) ) ;
#78176=CARTESIAN_POINT ( 'NONE',  ( -6.472888217819999568, 1410.296278320529836, 231.2922198908979965 ) ) ;
#78183=CARTESIAN_POINT ( 'NONE',  ( 12.10947664135730051, 1433.934507095030085, 149.7604101384789885 ) ) ;
#78184=CARTESIAN_POINT ( 'NONE',  ( 16.39369216350290159, 1478.707785154150088, 230.0407356733170161 ) ) ;
#78185=CARTESIAN_POINT ( 'NONE',  ( -21.84620687390529881, 1509.359330091720039, 227.5754383244390056 ) ) ;
#78186=CARTESIAN_POINT ( 'NONE',  ( -2.559321582819999996, 1409.169965997630015, 187.1278009686979829 ) ) ;
#78187=CARTESIAN_POINT ( 'NONE',  ( -20.64978683589999875, 1464.413060387330006, 208.6332757997560066 ) ) ;
#78188=CARTESIAN_POINT ( 'NONE',  ( -0.1622974587355989762, 1420.471025021490050, 182.7601356185510042 ) ) ;
#78191=CARTESIAN_POINT ( 'NONE',  ( 13.94974641142899863, 1428.477645029930045, 195.9751451731039822 ) ) ;
#78195=ORIENTED_EDGE ( 'NONE', *, *, #90435, .F. ) ;
#78196=CARTESIAN_POINT ( 'NONE',  ( -11.49746945758320038, 1414.913060387399810, 197.9010059328040256 ) ) ;
#78197=CARTESIAN_POINT ( 'NONE',  ( -0.7401336709869998920, 1504.313428565929826, 180.8842383983980255 ) ) ;
#78198=ORIENTED_EDGE ( 'NONE', *, *, #21299, .T. ) ;
#78199=CARTESIAN_POINT ( 'NONE',  ( 3.865613834079999922, 1421.793636752730208, 184.2641810182979896 ) ) ;
#78206=CARTESIAN_POINT ( 'NONE',  ( 18.01569507700000017, 1415.245980409429876, 210.3065621575879902 ) ) ;
#78209=CARTESIAN_POINT ( 'NONE',  ( -11.98890328080000067, 1442.756953654919926, 147.5994355510979688 ) ) ;
#78210=CARTESIAN_POINT ( 'NONE',  ( 17.28367426750000035, 1438.551524929770039, 190.7595339831979970 ) ) ;
#78213=CARTESIAN_POINT ( 'NONE',  ( 11.89956352200635514, 1433.602129414034835, 150.4843578385222429 ) ) ;
#78215=CARTESIAN_POINT ( 'NONE',  ( 1.555056480579879885, 1415.348334734329910, 191.0095454046629868 ) ) ;
#78219=CARTESIAN_POINT ( 'NONE',  ( -23.76810219530000268, 1436.580689387229995, 212.1216956802879849 ) ) ;
#78221=CARTESIAN_POINT ( 'NONE',  ( -3.767230627251568542, 1426.013493162819032, 186.0052132243664857 ) ) ;
#78222=EDGE_CURVE ( 'NONE', #27899, #94269, #97916, .T. ) ;
#78223=CARTESIAN_POINT ( 'NONE',  ( -10.82822666317459870, 1452.534930380020796, 150.8032249176135906 ) ) ;
#78226=CARTESIAN_POINT ( 'NONE',  ( 12.98226561589999939, 1414.913060387329779, 198.3280246956980193 ) ) ;
#78228=CARTESIAN_POINT ( 'NONE',  ( 20.30910795649999656, 1452.203850710330016, 143.8526422108979830 ) ) ;
#78233=CARTESIAN_POINT ( 'NONE',  ( -18.54348539920661310, 1458.676082630350265, 227.5712260952941506 ) ) ;
#78235=CARTESIAN_POINT ( 'NONE',  ( 20.44002321923020205, 1509.591610260329844, 230.3558478251790120 ) ) ;
#78236=ORIENTED_EDGE ( 'NONE', *, *, #76813, .T. ) ;
#78238=CARTESIAN_POINT ( 'NONE',  ( 18.87514223596030050, 1508.290019403229735, 229.9499626354140105 ) ) ;
#78240=CARTESIAN_POINT ( 'NONE',  ( 36.46881799559510284, 1437.630696346240029, 136.5444991984829812 ) ) ;
#78241=CARTESIAN_POINT ( 'NONE',  ( 19.73776679929999744, 1452.815214894130122, 209.1683919043709921 ) ) ;
#78242=CARTESIAN_POINT ( 'NONE',  ( -35.51625744890000647, 1458.123784601630177, 261.8360505382980250 ) ) ;
#78244=VECTOR ( 'NONE', #5643, 1000.000000000000000 ) ;
#78247=CARTESIAN_POINT ( 'NONE',  ( -19.21347146162490205, 1475.323696206919976, 227.8639392199079907 ) ) ;
#78248=CARTESIAN_POINT ( 'NONE',  ( 2.331552110770000130, 1409.931811533030213, 185.5473801112979686 ) ) ;
#78249=CARTESIAN_POINT ( 'NONE',  ( 6.032762746330000425, 1424.401310572229931, 186.1143022581979949 ) ) ;
#78250=CARTESIAN_POINT ( 'NONE',  ( -11.10313724959999959, 1434.937811603489990, 151.7082816907980032 ) ) ;
#78254=CARTESIAN_POINT ( 'NONE',  ( 0.04349594477419999744, 1452.084370642229942, 153.9873474275979959 ) ) ;
#78255=CARTESIAN_POINT ( 'NONE',  ( 2.439425361020000071, 1464.676489221029897, 236.7027247366980021 ) ) ;
#78256=VERTEX_POINT ( 'NONE', #48731 ) ;
#78259=CARTESIAN_POINT ( 'NONE',  ( -43.48864174949999750, 1442.487458641120156, 270.3367078953979785 ) ) ;
#78261=CARTESIAN_POINT ( 'NONE',  ( 9.522333297019999421, 1438.200918636809774, 153.1793569429979982 ) ) ;
#78262=CARTESIAN_POINT ( 'NONE',  ( -14.65012730729999824, 1474.165513649029890, 223.7053439215980006 ) ) ;
#78263=CARTESIAN_POINT ( 'NONE',  ( 12.86224528119999988, 1519.913060387329779, 190.2411470757980112 ) ) ;
#78264=CARTESIAN_POINT ( 'NONE',  ( 2.785137360674800000, 1409.020299217710090, 230.3656739585919979 ) ) ;
#78266=CARTESIAN_POINT ( 'NONE',  ( -4.149035421649998945, 1416.659952005129981, 232.5357826803979719 ) ) ;
#78267=FACE_OUTER_BOUND ( 'NONE', #3659, .T. ) ;
#78269=CARTESIAN_POINT ( 'NONE',  ( -45.83452011949149352, 1439.843055403779999, 268.7569621144950247 ) ) ;
#78270=CARTESIAN_POINT ( 'NONE',  ( -2.500000000000000000, 1428.691959813929998, 184.5792689180979949 ) ) ;
#78273=ORIENTED_EDGE ( 'NONE', *, *, #102850, .T. ) ;
#78278=CARTESIAN_POINT ( 'NONE',  ( -25.91590772737680126, 1441.261220175949802, 138.4451201564890255 ) ) ;
#78279=CARTESIAN_POINT ( 'NONE',  ( -16.18321133039999893, 1425.423028787829935, 190.7319080598980179 ) ) ;
#78281=EDGE_LOOP ( 'NONE', ( #43451, #5746, #95022, #79045 ) ) ;
#78282=CARTESIAN_POINT ( 'NONE',  ( -15.00906777690000027, 1488.801231226830168, 193.7268783320979821 ) ) ;
#78284=CARTESIAN_POINT ( 'NONE',  ( 14.28229724340000040, 1470.816572150529964, 194.5131132564980021 ) ) ;
#78286=CARTESIAN_POINT ( 'NONE',  ( -11.54861850680875435, 1426.051521667020324, 138.9191312498616071 ) ) ;
#78287=EDGE_CURVE ( 'NONE', #57816, #7082, #76371, .T. ) ;
#78290=ORIENTED_EDGE ( 'NONE', *, *, #72108, .F. ) ;
#78291=CARTESIAN_POINT ( 'NONE',  ( -0.5908173565667990124, 1410.389843549470015, 269.3346523052649673 ) ) ;
#78293=CARTESIAN_POINT ( 'NONE',  ( 4.949847236731660161, 1418.068533308110091, 233.9905393452280009 ) ) ;
#78298=ORIENTED_EDGE ( 'NONE', *, *, #92734, .F. ) ;
#78300=CARTESIAN_POINT ( 'NONE',  ( -4.320810598459999596, 1425.290410123230004, 186.1758918437979844 ) ) ;
#78301=CARTESIAN_POINT ( 'NONE',  ( -10.78266347204017883, 1438.594363250573679, 152.4465531432095418 ) ) ;
#78304=CARTESIAN_POINT ( 'NONE',  ( -18.43142101346469985, 1424.689440642639966, 194.8163951100160034 ) ) ;
#78305=CARTESIAN_POINT ( 'NONE',  ( -18.25008163810000283, 1425.818581969829893, 225.5639177453979869 ) ) ;
#78306=CARTESIAN_POINT ( 'NONE',  ( 33.11929144969669636, 1465.571379411549970, 267.3866912509090525 ) ) ;
#78309=CARTESIAN_POINT ( 'NONE',  ( 9.095534004770000180, 1445.600425117210079, 184.8596504565979899 ) ) ;
#78313=CARTESIAN_POINT ( 'NONE',  ( 1.479947764255840070, 1478.089622790649855, 182.3790958322389884 ) ) ;
#78314=CARTESIAN_POINT ( 'NONE',  ( 23.61060712979999821, 1411.111110838729928, 207.8239932459379986 ) ) ;
#78317=EDGE_CURVE ( 'NONE', #34791, #21200, #72561, .T. ) ;
#78318=CARTESIAN_POINT ( 'NONE',  ( 25.51240218741290278, 1451.577767330780034, 136.5542256109710024 ) ) ;
#78324=CARTESIAN_POINT ( 'NONE',  ( 17.69895706029999971, 1410.894947626029989, 192.9683006637980043 ) ) ;
#78326=CARTESIAN_POINT ( 'NONE',  ( 3.206067321177020979, 1439.684559099622675, 184.2987211024194778 ) ) ;
#78327=CARTESIAN_POINT ( 'NONE',  ( 2.046266125239999845, 1417.477797419130184, 235.2693601201980016 ) ) ;
#78328=CARTESIAN_POINT ( 'NONE',  ( -19.86494872359075003, 1426.191873834269927, 222.7246227809951336 ) ) ;
#78330=CARTESIAN_POINT ( 'NONE',  ( 1.111973768122940021, 1450.991701817079957, 182.4208154947999958 ) ) ;
#78331=EDGE_CURVE ( 'NONE', #944, #30887, #69256, .T. ) ;
#78332=CARTESIAN_POINT ( 'NONE',  ( 18.50343566175140353, 1467.878388117720078, 228.1213590980190133 ) ) ;
#78339=CARTESIAN_POINT ( 'NONE',  ( -24.34268787264259970, 1442.549328851149994, 212.2035684885649687 ) ) ;
#78340=CARTESIAN_POINT ( 'NONE',  ( -0.4546767127886620075, 1409.373319351459941, 232.7794293636910083 ) ) ;
#78341=B_SPLINE_CURVE_WITH_KNOTS ( 'NONE', 5,
 ( #54429, #38138, #64474, #13461, #79619, #72320, #71797, #63385, #72858, #12927, #55512, #90179 ),
 .UNSPECIFIED., .F., .F.,
 ( 6, 3, 3, 6 ),
 ( 0.000000000000000000, 0.3850691707344797710, 0.6691521531983583015, 1.000000000000000000 ),
 .UNSPECIFIED. ) ;
#78345=CARTESIAN_POINT ( 'NONE',  ( -33.91369269983620427, 1450.440666099120108, 136.2454419983430114 ) ) ;
#78347=CARTESIAN_POINT ( 'NONE',  ( -18.41412373400000035, 1444.997163189090088, 209.1218459616979999 ) ) ;
#78348=CARTESIAN_POINT ( 'NONE',  ( -2.649360860297129694, 1451.956705521739877, 184.7216075439289966 ) ) ;
#78349=CARTESIAN_POINT ( 'NONE',  ( 11.30061245240000112, 1433.709615238220067, 151.5117488965980215 ) ) ;
#78350=CARTESIAN_POINT ( 'NONE',  ( 1.110223024629999949E-15, 1454.846680951630105, 214.3676144195279676 ) ) ;
#78351=CARTESIAN_POINT ( 'NONE',  ( 26.56266887126210108, 1440.913060393550040, 224.7525115906159954 ) ) ;
#78357=CARTESIAN_POINT ( 'NONE',  ( -29.00753178363559570, 1509.926023647250076, 200.7080847602200038 ) ) ;
#78360=CARTESIAN_POINT ( 'NONE',  ( 19.06924801490000121, 1449.793579036090023, 224.4195381262979936 ) ) ;
#78362=CARTESIAN_POINT ( 'NONE',  ( 5.807361285020000314E-16, 1430.453334911130241, 150.3332009510979788 ) ) ;
#78368=CARTESIAN_POINT ( 'NONE',  ( 0.1610941246609420008, 1485.608819109279921, 181.8534184629149877 ) ) ;
#78371=DIRECTION ( 'NONE',  ( 0.000000000000000000, 0.000000000000000000, 1.000000000000000000 ) ) ;
#78372=B_SPLINE_CURVE_WITH_KNOTS ( 'NONE', 3,
 ( #81333, #3026, #4114, #71345, #4647, #88120, #80257, #64578, #29840, #38785, #107098, #81887, #11409, #37149, #30387, #88668, #98697, #21957, #11946, #47752, #3574, #37698, #71901, #58360, #15220, #110401, #24713, #108751, #91946, #92485, #58911, #100351, #57821, #42106, #49412, #49956, #23074, #50516, #6830, #90842 ),
 .UNSPECIFIED., .F., .F.,
 ( 4, 3, 3, 3, 3, 3, 3, 3, 3, 3, 3, 3, 3, 4 ),
 ( -1.459712257500000110, -1.414311702603749943, -1.300049757133459938, -1.184105919937280094, -1.067104322070629996, -0.9485798734533590348, -0.8293278323600270507, -0.7096591974163730665, -0.5899191834374760690, -0.4656630299999721112, -0.3474018752853509362, -0.2302575540096110096, -0.1144180656139759389, 2.220446049250313081E-16 ),
 .UNSPECIFIED. ) ;
#78380=CARTESIAN_POINT ( 'NONE',  ( -16.44108894340000049, 1415.931669658129977, 216.8029115086079628 ) ) ;
#78381=CARTESIAN_POINT ( 'NONE',  ( -0.4986843622567649348, 1508.982343520079894, 238.8510830230749775 ) ) ;
#78383=AXIS2_PLACEMENT_3D ( 'NONE', #86524, #51838, #94932 ) ;
#78386=CARTESIAN_POINT ( 'NONE',  ( 14.70986748862159921, 1409.426740279159958, 206.5596626142009882 ) ) ;
#78389=CARTESIAN_POINT ( 'NONE',  ( -16.66093153799999982, 1410.867388830529990, 191.7374817029979681 ) ) ;
#78391=EDGE_LOOP ( 'NONE', ( #22435, #106505, #53833, #8114 ) ) ;
#78393=CARTESIAN_POINT ( 'NONE',  ( 12.78776258891489981, 1416.851343896290018, 222.2791104166909975 ) ) ;
#78395=CARTESIAN_POINT ( 'NONE',  ( 33.91369278643569629, 1437.010534640189690, 136.5611839302279691 ) ) ;
#78396=ORIENTED_EDGE ( 'NONE', *, *, #92452, .F. ) ;
#78399=CARTESIAN_POINT ( 'NONE',  ( -11.71170459750000070, 1433.766298954200238, 151.0909624611979893 ) ) ;
#78400=CARTESIAN_POINT ( 'NONE',  ( 29.84411685202790565, 1462.363335203606994, 269.4691510201575966 ) ) ;
#78407=FACE_OUTER_BOUND ( 'NONE', #91742, .T. ) ;
#78413=CARTESIAN_POINT ( 'NONE',  ( 6.817746255100000319, 1475.057956560229968, 269.6447263236980234 ) ) ;
#78417=CARTESIAN_POINT ( 'NONE',  ( 11.36018337630000019, 1414.996442546230128, 222.2791104318980047 ) ) ;
#78421=CARTESIAN_POINT ( 'NONE',  ( -26.47779523690000048, 1469.247571742229866, 208.2308877974680001 ) ) ;
#78422=CARTESIAN_POINT ( 'NONE',  ( -10.97659976954949990, 1425.661045819329956, 113.0066238976479980 ) ) ;
#78423=CARTESIAN_POINT ( 'NONE',  ( 16.40767016540999634, 1409.511151603330063, 193.0217009399570145 ) ) ;
#78425=CARTESIAN_POINT ( 'NONE',  ( 18.37396616818673678, 1509.673958510744797, 185.4069322651564846 ) ) ;
#78426=CARTESIAN_POINT ( 'NONE',  ( -21.84849975889999740, 1489.480617680329942, 208.5290360645649912 ) ) ;
#78427=CARTESIAN_POINT ( 'NONE',  ( -28.66942461389999863, 1426.582479899429927, 248.2467662554980166 ) ) ;
#78428=CARTESIAN_POINT ( 'NONE',  ( 18.52468149035910017, 1509.577301616600153, 232.1917227349059942 ) ) ;
#78429=CARTESIAN_POINT ( 'NONE',  ( 17.24781598545795802, 1460.195507983534526, 228.5738697325721773 ) ) ;
#78431=CARTESIAN_POINT ( 'NONE',  ( 2.994688454485729956, 1464.609795419120246, 236.6065850994260131 ) ) ;
#78433=CARTESIAN_POINT ( 'NONE',  ( 12.59185353107299932, 1397.673301978809832, 213.9584579308699972 ) ) ;
#78435=CARTESIAN_POINT ( 'NONE',  ( -18.32069918539999875, 1457.567609363029987, 229.9399091793980006 ) ) ;
#78436=ORIENTED_EDGE ( 'NONE', *, *, #80813, .T. ) ;
#78438=CARTESIAN_POINT ( 'NONE',  ( -29.24670345068486910, 1509.934423202144217, 211.7350478754418930 ) ) ;
#78439=CARTESIAN_POINT ( 'NONE',  ( -6.356853423171860307, 1423.329120530439923, 150.6733129965809894 ) ) ;
#78441=CARTESIAN_POINT ( 'NONE',  ( 0.5075932631809999540, 1412.056819125330094, 184.9972924272980208 ) ) ;
#78445=CARTESIAN_POINT ( 'NONE',  ( -2.412918666629999986, 1461.195343464629786, 234.9240695220980228 ) ) ;
#78450=EDGE_LOOP ( 'NONE', ( #81322, #95255, #51376, #100685 ) ) ;
#78454=CARTESIAN_POINT ( 'NONE',  ( 11.85272800890160028, 1431.406550633420011, 149.9031061979179924 ) ) ;
#78458=DIRECTION ( 'NONE',  ( 0.08014523039090584722, -0.9891236767552784581, -0.1233332644816800827 ) ) ;
#78463=CARTESIAN_POINT ( 'NONE',  ( -4.785570096949999908, 1423.623530998630031, 184.5509701510979710 ) ) ;
#78464=CARTESIAN_POINT ( 'NONE',  ( 3.400294879866609943, 1410.489090383209941, 269.3360835134739659 ) ) ;
#78474=CARTESIAN_POINT ( 'NONE',  ( -13.86092847646930082, 1410.765486861110048, 227.1170286572800023 ) ) ;
#78476=CARTESIAN_POINT ( 'NONE',  ( 17.26713005559999914, 1428.027535763729929, 234.3916895853979838 ) ) ;
#78477=DIRECTION ( 'NONE',  ( 0.000000000000000000, -0.000000000000000000, 1.000000000000000000 ) ) ;
#78478=B_SPLINE_SURFACE_WITH_KNOTS ( 'NONE', 5, 5, ( 
 ( #108327, #31060, #100473, #56831, #83126, #14254, #83668, #75297, #23756 ),
 ( #74740, #40569, #4756, #13137, #5874, #91530, #65788, #65241, #32721 ),
 ( #66902, #99908, #48994, #108878, #66355, #24308, #58488, #47321, #81448 ),
 ( #56276, #13685, #47872, #82009, #5315, #73644, #99352, #22627, #27095 ),
 ( #86433, #69111, #1341, #16439, #18114, #43347, #85313, #35480, #52309 ),
 ( #68009, #42233, #26518, #110530, #69673, #33814, #8608, #102119, #25398 ),
 ( #33264, #59048, #59591, #92616, #9724, #43889, #103212, #51183, #42784 ),
 ( #76943, #51747, #60716, #78033, #25953, #50093, #93169, #15893, #60148 ),
 ( #75837, #24845, #94838, #253, #76381, #103796, #84220, #109987, #34380 ) ),
 .UNSPECIFIED., .F., .F., .F.,
 ( 6, 3, 6 ),
 ( 6, 3, 6 ),
 ( 1.119735183810000034, 3.314582533139999843, 6.273244355579999265 ),
 ( 0.000000000000000000, 1.000000000000000000, 2.000000000000000000 ),
 .UNSPECIFIED. ) ;
#78490=FACE_OUTER_BOUND ( 'NONE', #94632, .T. ) ;
#78491=CARTESIAN_POINT ( 'NONE',  ( 13.40566205669149902, 1429.098591087019940, 222.0107402452829888 ) ) ;
#78493=CARTESIAN_POINT ( 'NONE',  ( 11.23079704630000109, 1415.077546157430106, 229.5486842020980021 ) ) ;
#78495=CARTESIAN_POINT ( 'NONE',  ( -16.21296007320000143, 1459.516395508230062, 228.9531164853979988 ) ) ;
#78498=CARTESIAN_POINT ( 'NONE',  ( 21.81698820680000495, 1410.329754421929920, 269.1143266171980031 ) ) ;
#78500=EDGE_CURVE ( 'NONE', #91965, #9014, #36191, .T. ) ;
#78503=CARTESIAN_POINT ( 'NONE',  ( 19.34978595810000002, 1469.161539876029792, 191.0314867524980116 ) ) ;
#78504=CARTESIAN_POINT ( 'NONE',  ( -21.78276816909999880, 1430.096355600930110, 220.5348153272979914 ) ) ;
#78506=LINE ( 'NONE', #69580, #49501 ) ;
#78507=( BOUNDED_CURVE ( )  B_SPLINE_CURVE ( 3, ( #95862, #79086, #69593, #53331 ),
 .UNSPECIFIED., .F., .F. ) 
 B_SPLINE_CURVE_WITH_KNOTS ( ( 4, 4 ),
 ( 5.085528608296080222, 5.733722764883870227 ),
 .UNSPECIFIED. ) 
 CURVE ( )  GEOMETRIC_REPRESENTATION_ITEM ( )  RATIONAL_B_SPLINE_CURVE ( ( 1.000000000000000000, 0.9652924339432646939, 0.9652924339432646939, 1.000000000000000000 ) ) 
 REPRESENTATION_ITEM ( '' )  );
#78510=CARTESIAN_POINT ( 'NONE',  ( -19.72497237273909931, 1506.501081260519868, 199.2811559755782014 ) ) ;
#78511=CARTESIAN_POINT ( 'NONE',  ( -17.84625751240000113, 1415.088275290029969, 207.8799776997580011 ) ) ;
#78512=CARTESIAN_POINT ( 'NONE',  ( -12.47743317399999974, 1441.795364512870037, 187.8062295142980247 ) ) ;
#78514=CARTESIAN_POINT ( 'NONE',  ( -31.76432995890000299, 1436.935670857599916, 136.6280379864980148 ) ) ;
#78515=CARTESIAN_POINT ( 'NONE',  ( -0.8190328885345301568, 1418.969064690915957, 184.8287215811062651 ) ) ;
#78518=CARTESIAN_POINT ( 'NONE',  ( -14.93003779297889899, 1409.434428795590065, 209.1736875269810128 ) ) ;
#78521=CARTESIAN_POINT ( 'NONE',  ( -44.77906958589999675, 1451.150212632430112, 268.5354239598979689 ) ) ;
#78523=CIRCLE ( 'NONE', #107128, 1.999999954377635225 ) ;
#78524=CARTESIAN_POINT ( 'NONE',  ( 0.4837104977199940259, 1418.710257852230143, 184.7118620339130075 ) ) ;
#78528=CARTESIAN_POINT ( 'NONE',  ( 17.04506599712540194, 1423.842078673229935, 228.2841224977100296 ) ) ;
#78529=CARTESIAN_POINT ( 'NONE',  ( 14.85820445110000065, 1414.971262582530017, 216.9249339935579997 ) ) ;
#78530=CARTESIAN_POINT ( 'NONE',  ( -3.229222591820000154, 1433.444289491620111, 155.4497426196979859 ) ) ;
#78531=CARTESIAN_POINT ( 'NONE',  ( -25.84539468360279812, 1482.717571151330048, 211.4979452547460141 ) ) ;
#78533=CARTESIAN_POINT ( 'NONE',  ( -10.12762402319999921, 1509.205805730729935, 181.4374674442979938 ) ) ;
#78534=CARTESIAN_POINT ( 'NONE',  ( -23.76303430200000122, 1410.238322737530098, 208.1246107068909907 ) ) ;
#78535=CARTESIAN_POINT ( 'NONE',  ( 16.56387297150000393, 1416.216596894529857, 201.3979519333380210 ) ) ;
#78542=CARTESIAN_POINT ( 'NONE',  ( -22.47141948400000189, 1410.193803399830131, 211.4552637418080110 ) ) ;
#78549=CARTESIAN_POINT ( 'NONE',  ( -14.37359814958930038, 1486.056774777669943, 185.9402136656559890 ) ) ;
#78550=CARTESIAN_POINT ( 'NONE',  ( 1.455000239979999943, 1507.073729426630052, 236.7651042955980074 ) ) ;
#78553=CARTESIAN_POINT ( 'NONE',  ( 40.05116234797749541, 1447.068974477369920, 136.6106942782779754 ) ) ;
#78556=B_SPLINE_CURVE_WITH_KNOTS ( 'NONE', 3,
 ( #107154, #90341, #39404, #108811, #73581, #107712, #65173, #32105, #25330, #51674, #58968, #109917, #9109, #24236, #51122, #85246, #726, #66833, #84697, #84151, #103147, #18043, #7451, #76871, #76314, #67937, #77422, #94201, #60085, #94765, #52236, #93102, #85811, #33196, #67387, #75228, #93638, #75768, #24772, #185, #43276, #102044, #86365 ),
 .UNSPECIFIED., .F., .F.,
 ( 4, 3, 3, 3, 3, 3, 3, 3, 3, 3, 3, 3, 3, 3, 4 ),
 ( 0.7655572723410000169, 0.9910019231850759613, 1.224379699286819889, 1.462078616762300109, 1.704827355037529912, 1.793853281190000093, 2.038466588173669880, 2.281256469890939886, 2.316155491860000026, 2.583989317150000353, 2.855920918845609613, 3.139267314119390306, 3.387490793019999558, 3.680707214893210732, 3.835724788439999422 ),
 .UNSPECIFIED. ) ;
#78557=ORIENTED_EDGE ( 'NONE', *, *, #25126, .F. ) ;
#78558=CARTESIAN_POINT ( 'NONE',  ( 11.96574013264010006, 1433.577777978849781, 149.9770704080709720 ) ) ;
#78560=ORIENTED_EDGE ( 'NONE', *, *, #83296, .F. ) ;
#78564=CARTESIAN_POINT ( 'NONE',  ( 4.743041381730000339, 1427.184332118029943, 133.6118001900980232 ) ) ;
#78567=FACE_OUTER_BOUND ( 'NONE', #5965, .T. ) ;
#78568=CARTESIAN_POINT ( 'NONE',  ( 10.35429883085484981, 1439.070324005060911, 152.7368639322063189 ) ) ;
#78569=CARTESIAN_POINT ( 'NONE',  ( -24.21915031236209970, 1444.789092827589911, 211.4477932164650156 ) ) ;
#78570=B_SPLINE_SURFACE_WITH_KNOTS ( 'NONE', 5, 4, ( 
 ( #83045, #40487, #81372, #32643, #24220 ),
 ( #16359, #86346, #75755, #9092, #69029 ),
 ( #25868, #59512, #84684, #35397, #69585 ),
 ( #50003, #15799, #25314, #85232, #67371 ),
 ( #93624, #24757, #101470, #58955, #50558 ),
 ( #16902, #76299, #84137, #17456, #7982 ) ),
 .UNSPECIFIED., .F., .F., .F.,
 ( 6, 6 ),
 ( 5, 5 ),
 ( 0.000000000000000000, 111.1101480259999903 ),
 ( 25.81581217359999769, 39.03307591160000101 ),
 .UNSPECIFIED. ) ;
#78572=CARTESIAN_POINT ( 'NONE',  ( 14.22819488943649979, 1415.834070663119974, 197.0873419266759754 ) ) ;
#78575=ORIENTED_EDGE ( 'NONE', *, *, #101841, .T. ) ;
#78576=CARTESIAN_POINT ( 'NONE',  ( 13.91219551702819857, 1436.092364807330114, 150.2494214597319910 ) ) ;
#78580=CARTESIAN_POINT ( 'NONE',  ( 12.57924958998592402, 1445.046140314299691, 169.4707391365555793 ) ) ;
#78581=CARTESIAN_POINT ( 'NONE',  ( -1.463875870539999902, 1465.932623932230172, 235.6053488212979801 ) ) ;
#78588=CARTESIAN_POINT ( 'NONE',  ( 4.221461520009319734, 1446.221124511070002, 168.5615742123870291 ) ) ;
#78594=CARTESIAN_POINT ( 'NONE',  ( 32.68061409889739366, 1440.913060387330006, 257.1432865577979783 ) ) ;
#78598=CARTESIAN_POINT ( 'NONE',  ( -14.07231417549999897, 1409.404476426829888, 191.3682123889980176 ) ) ;
#78600=CARTESIAN_POINT ( 'NONE',  ( -11.01884469515209908, 1414.913527275050001, 195.9427818023129930 ) ) ;
#78608=B_SPLINE_SURFACE_WITH_KNOTS ( 'NONE', 5, 5, ( 
 ( #17956, #59456, #77891, #36429, #35332, #19056, #16841, #61128, #649, #68413, #1199, #104741, #93566, #25807, #94126, #78445, #77347, #27474, #43195, #102516, #60005, #18505, #1759, #52703 ),
 ( #51043, #17397, #34780, #86837, #10130, #35897, #53260, #10694, #53825, #21801, #72806, #87964, #2855, #20172, #11253, #106395, #81179, #45413, #80645, #19623, #20709, #12876, #38086, #71172 ),
 ( #56001, #46511, #47055, #54369, #29135, #90125, #28585, #105294, #4495, #38628, #64410, #63862, #97978, #28030, #72262, #80088, #62786, #96901, #3408, #47595, #3959, #81722, #98533, #63324 ),
 ( #88499, #79557, #13408, #29678, #106933, #21244, #5029, #30222, #11783, #39173, #62219, #12322, #73349, #36978, #45950, #96346, #37538, #89585, #71740, #105857, #97444, #54908, #89032, #55457 ),
 ( #41402, #90681, #100726, #92890, #99622, #108032, #13969, #32976, #57116, #75569, #91242, #50368, #109163, #109702, #15604, #92332, #49260, #41950, #15061, #101263, #84494, #6684, #82834, #83941 ),
 ( #14521, #40839, #31328, #67166, #75013, #48712, #6126, #74467, #91785, #23479, #73906, #64958, #32449, #7784, #24010, #58751, #24562, #39740, #30779, #16165, #22908, #66625, #58204, #49810 ) ),
 .UNSPECIFIED., .F., .F., .F.,
 ( 6, 6 ),
 ( 6, 3, 3, 3, 3, 3, 3, 6 ),
 ( 52.54788734150000096, 99.04053960890000496 ),
 ( 27.66747964320000008, 34.02592213510000363, 36.52949902339999966, 37.78128746749999323, 38.40718168960000156, 39.03307591160000101, 39.70872026930000231, 40.38436462709999830 ),
 .UNSPECIFIED. ) ;
#78610=CARTESIAN_POINT ( 'NONE',  ( 22.90250716390000107, 1409.721554320030009, 209.3445813094469941 ) ) ;
#78612=ADVANCED_FACE ( 'NONE', ( #70934 ), #67025, .F. ) ;
#78615=CARTESIAN_POINT ( 'NONE',  ( 15.06903345039999920, 1410.389868239730049, 191.5311856341979819 ) ) ;
#78621=CARTESIAN_POINT ( 'NONE',  ( 29.66529950099999624, 1450.991311272329767, 244.2516413617979936 ) ) ;
#78624=CARTESIAN_POINT ( 'NONE',  ( -3.665607323393529793, 1507.166784210740161, 236.6858246876950034 ) ) ;
#78625=CARTESIAN_POINT ( 'NONE',  ( -20.99439929950000305, 1454.025623455230061, 225.3869460595979888 ) ) ;
#78626=CARTESIAN_POINT ( 'NONE',  ( 11.30788561520000002, 1432.726986962210049, 151.5212569857980327 ) ) ;
#78627=CARTESIAN_POINT ( 'NONE',  ( 17.82217580153020009, 1410.175561989269909, 222.8366056556930062 ) ) ;
#78628=CARTESIAN_POINT ( 'NONE',  ( 0.2728724028810000091, 1488.801231226530035, 187.6229463501980206 ) ) ;
#78632=CARTESIAN_POINT ( 'NONE',  ( 1.810797400909999994E-09, 1405.989059426729909, 266.9611530680980422 ) ) ;
#78633=DIRECTION ( 'NONE',  ( 1.000000000000000000, 0.000000000000000000, 0.000000000000000000 ) ) ;
#78634=CARTESIAN_POINT ( 'NONE',  ( 18.82307291165939844, 1468.777348105939836, 269.3734094525160572 ) ) ;
#78635=CARTESIAN_POINT ( 'NONE',  ( 5.386772287290000349, 1432.443201990170110, 154.6097844173980036 ) ) ;
#78636=CARTESIAN_POINT ( 'NONE',  ( -27.13948102820610231, 1449.857017199720076, 136.5863992428030258 ) ) ;
#78638=CARTESIAN_POINT ( 'NONE',  ( -44.14497367832510122, 1440.913060404099951, 264.5199370315700094 ) ) ;
#78639=AXIS2_PLACEMENT_3D ( 'NONE', #55415, #82799, #30742 ) ;
#78640=CARTESIAN_POINT ( 'NONE',  ( 36.08172904959410232, 1449.985944480599983, 136.2472095414419755 ) ) ;
#78641=DIRECTION ( 'NONE',  ( 0.000000000000000000, -0.9990482215818579093, 0.04361938736533144123 ) ) ;
#78643=CARTESIAN_POINT ( 'NONE',  ( 2.491511751652589979, 1449.258137923909999, 154.2481093066819824 ) ) ;
#78649=CARTESIAN_POINT ( 'NONE',  ( -39.48812356999999906, 1431.587789824249967, 268.3665355199980240 ) ) ;
#78652=CARTESIAN_POINT ( 'NONE',  ( -0.6528690470989999550, 1417.364746825729981, 235.5198400807980192 ) ) ;
#78653=CARTESIAN_POINT ( 'NONE',  ( -4.249354323605699868, 1446.471035334290036, 161.2178408973400110 ) ) ;
#78658=CARTESIAN_POINT ( 'NONE',  ( -18.72518989680000345, 1416.274718422629803, 208.3778101247369818 ) ) ;
#78659=CARTESIAN_POINT ( 'NONE',  ( 11.87399071922619953, 1432.929227292529959, 149.9807480848299974 ) ) ;
#78660=CARTESIAN_POINT ( 'NONE',  ( 26.61739034963180117, 1435.433209610839867, 135.4670460917660080 ) ) ;
#78661=CARTESIAN_POINT ( 'NONE',  ( -12.53380499169999851, 1445.052233488290085, 169.4755105685979970 ) ) ;
#78663=CARTESIAN_POINT ( 'NONE',  ( -17.27769651085920088, 1410.881435910499931, 225.9445911753860230 ) ) ;
#78669=DIRECTION ( 'NONE',  ( 1.000000000000000000, 0.000000000000000000, 0.000000000000000000 ) ) ;
#78673=CIRCLE ( 'NONE', #101900, 3678.960170865509554 ) ;
#78679=CARTESIAN_POINT ( 'NONE',  ( 2.863305601979999615, 1449.090055474780002, 183.5657516826979929 ) ) ;
#78683=ORIENTED_EDGE ( 'NONE', *, *, #6527, .F. ) ;
#78684=CARTESIAN_POINT ( 'NONE',  ( -40.71170020219999941, 1443.968826064090081, 137.1159894999980224 ) ) ;
#78685=EDGE_CURVE ( 'NONE', #76272, #16145, #4817, .T. ) ;
#78686=CARTESIAN_POINT ( 'NONE',  ( 1.146809930359999896, 1466.701590537929860, 235.3106089818980138 ) ) ;
#78687=CARTESIAN_POINT ( 'NONE',  ( 0.2538829723067779764, 1420.503732877419907, 182.7635795570130028 ) ) ;
#78689=CARTESIAN_POINT ( 'NONE',  ( -3.526834439349999961, 1486.375772999530000, 181.8601271665980050 ) ) ;
#78690=AXIS2_PLACEMENT_3D ( 'NONE', #30334, #47704, #23023 ) ;
#78694=CARTESIAN_POINT ( 'NONE',  ( -34.99243995798710216, 1450.827641384700200, 136.1403221839539981 ) ) ;
#78695=EDGE_CURVE ( 'NONE', #6800, #44714, #6656, .T. ) ;
#78697=CARTESIAN_POINT ( 'NONE',  ( 33.93525352000410322, 1435.841465267310014, 135.9408836255369977 ) ) ;
#78698=CARTESIAN_POINT ( 'NONE',  ( 32.64368752077381686, 1435.637503394754049, 135.1055172344166522 ) ) ;
#78699=CARTESIAN_POINT ( 'NONE',  ( -0.01096400588092319960, 1407.225809178260079, 196.1218459624460024 ) ) ;
#78700=DIRECTION ( 'NONE',  ( -0.2342910579933019377, -0.2476038117450569398, -0.9401064049104748133 ) ) ;
#78701=CARTESIAN_POINT ( 'NONE',  ( -11.20854089327220038, 1414.996442620800053, 195.7122650692939771 ) ) ;
#78703=CARTESIAN_POINT ( 'NONE',  ( -10.96917002040000000, 1432.328099320269985, 151.7701195717980056 ) ) ;
#78704=CARTESIAN_POINT ( 'NONE',  ( 13.49481936589999975, 1445.992738435850015, 188.9449086255979751 ) ) ;
#78705=B_SPLINE_SURFACE_WITH_KNOTS ( 'NONE', 5, 5, ( 
 ( #31484, #99782, #65665, #101422, #83000, #6293, #40440, #68429, #16858 ),
 ( #86854, #95261, #8478, #17413, #104209, #1215, #35350, #69537, #85744 ),
 ( #34246, #103657, #26956, #60580, #18522, #9042, #2334, #27496, #61146 ),
 ( #86302, #60024, #102531, #17975, #43215, #1776, #52719, #94700, #79033 ),
 ( #77364, #52171, #10146, #61683, #68984, #26385, #10711, #9586, #76806 ),
 ( #103085, #94142, #95806, #25823, #34796, #44319, #43757, #51610, #70096 ),
 ( #78463, #36446, #51062, #53277, #77909, #665, #35913, #19073, #87416 ),
 ( #44883, #101985, #25271, #59472, #93582, #85192, #42652, #122, #53844 ),
 ( #71190, #96921, #72280, #28604, #28046, #105312, #38645, #90141, #54386 ) ),
 .UNSPECIFIED., .F., .F., .F.,
 ( 6, 3, 6 ),
 ( 6, 3, 6 ),
 ( 5.472486514890000819, 9.497846738619999840, 12.82121481780000138 ),
 ( 0.000000000000000000, 1.000000000000000000, 2.000000000000000000 ),
 .UNSPECIFIED. ) ;
#78707=ORIENTED_EDGE ( 'NONE', *, *, #97972, .T. ) ;
#78714=CARTESIAN_POINT ( 'NONE',  ( 7.747670780530000023, 1416.518938592030054, 225.7538447804980137 ) ) ;
#78716=CARTESIAN_POINT ( 'NONE',  ( 5.343479918049999888, 1396.099658817830004, 218.7752541424879951 ) ) ;
#78721=CARTESIAN_POINT ( 'NONE',  ( -5.667817220899999953, 1409.110984927429854, 230.5553178883980081 ) ) ;
#78723=CARTESIAN_POINT ( 'NONE',  ( -9.116846773499998946, 1445.598699692060109, 184.9636421048979855 ) ) ;
#78724=ORIENTED_EDGE ( 'NONE', *, *, #5669, .T. ) ;
#78725=CARTESIAN_POINT ( 'NONE',  ( 29.24087330780000116, 1451.891771913630237, 134.8528131887979953 ) ) ;
#78726=CARTESIAN_POINT ( 'NONE',  ( 11.02433906870393265, 1425.200908241132538, 139.1360266714638101 ) ) ;
#78727=CARTESIAN_POINT ( 'NONE',  ( 21.03150544155480262, 1507.789100631340261, 226.0652199028830012 ) ) ;
#78728=CARTESIAN_POINT ( 'NONE',  ( 17.02668221408760019, 1422.112876149069962, 226.8213126862850118 ) ) ;
#78729=CARTESIAN_POINT ( 'NONE',  ( -24.32488869200000181, 1435.346926706200065, 136.3493805836980073 ) ) ;
#78737=EDGE_LOOP ( 'NONE', ( #105436, #51075, #47998, #76498 ) ) ;
#78738=CARTESIAN_POINT ( 'NONE',  ( 2.500000000000000000, 1432.302110539269961, 157.4936333739979943 ) ) ;
#78739=CARTESIAN_POINT ( 'NONE',  ( -0.6620138580789999283, 1412.846677813530050, 233.2438720524980056 ) ) ;
#78741=EDGE_LOOP ( 'NONE', ( #23297, #45964, #89977 ) ) ;
#78742=DIRECTION ( 'NONE',  ( 0.4990868182759217730, -0.2476038119106064028, -0.8304244096548186738 ) ) ;
#78744=CARTESIAN_POINT ( 'NONE',  ( 12.12754418595840100, 1433.981883138469811, 149.9562185505259890 ) ) ;
#78745=EDGE_CURVE ( 'NONE', #21185, #86873, #72364, .T. ) ;
#78746=CARTESIAN_POINT ( 'NONE',  ( 15.49878809011119962, 1469.005027229599818, 230.0777613073749706 ) ) ;
#78747=CARTESIAN_POINT ( 'NONE',  ( -25.23663147221330050, 1509.794343225200009, 222.8844807554229988 ) ) ;
#78748=CARTESIAN_POINT ( 'NONE',  ( -2.644001908849999971, 1409.509886481130025, 186.7831889129979857 ) ) ;
#78749=PLANE ( 'NONE',  #34075 ) ;
#78750=CARTESIAN_POINT ( 'NONE',  ( -0.01543823104247980284, 1420.444145791279880, 182.6744822797599852 ) ) ;
#78751=CIRCLE ( 'NONE', #57289, 3678.960196675449879 ) ;
#78753=DIRECTION ( 'NONE',  ( 0.7059212408186743559, 0.02465132495770355758, 0.7078612250567569708 ) ) ;
#78754=CARTESIAN_POINT ( 'NONE',  ( 19.65556712749999946, 1509.582207825729938, 187.2736428280979908 ) ) ;
#78755=CARTESIAN_POINT ( 'NONE',  ( -5.360152366205530150, 1422.242722016050038, 144.1549655170190078 ) ) ;
#78757=CARTESIAN_POINT ( 'NONE',  ( -11.74757148147149977, 1414.971390223329990, 197.2503777628510022 ) ) ;
#78762=CARTESIAN_POINT ( 'NONE',  ( 10.15354923512214036, 1435.473398722268257, 152.3868440969227152 ) ) ;
#78767=AXIS2_PLACEMENT_3D ( 'NONE', #958, #41286, #17139 ) ;
#78768=CARTESIAN_POINT ( 'NONE',  ( -2.500000001370000113, 1448.248591364029835, 156.2049463022979978 ) ) ;
#78769=CARTESIAN_POINT ( 'NONE',  ( -18.59208672289999953, 1425.224709566930187, 227.1497469740980080 ) ) ;
#78770=CARTESIAN_POINT ( 'NONE',  ( -19.43950658530000197, 1435.604459603690202, 145.6038571952979908 ) ) ;
#78774=CARTESIAN_POINT ( 'NONE',  ( 1.600048698852036821, 1401.254281879943164, 137.0999999980979851 ) ) ;
#78777=CARTESIAN_POINT ( 'NONE',  ( 0.5987183461865049905, 1507.212886145319999, 186.4932301926239688 ) ) ;
#78779=ADVANCED_FACE ( 'NONE', ( #65816 ), #83981, .T. ) ;
#78780=CARTESIAN_POINT ( 'NONE',  ( -11.91180745165941879, 1433.366507474078617, 149.9330222961037009 ) ) ;
#78783=CARTESIAN_POINT ( 'NONE',  ( -18.62830157129999620, 1508.852446407129946, 229.9890140626980042 ) ) ;
#78784=CARTESIAN_POINT ( 'NONE',  ( -3.511054680705768316, 1426.007948959481382, 185.8822184451843498 ) ) ;
#78785=CARTESIAN_POINT ( 'NONE',  ( -16.19492410612830113, 1409.478599598990058, 194.0661808939520085 ) ) ;
#78786=CARTESIAN_POINT ( 'NONE',  ( -25.00976051679999657, 1436.598010167069788, 137.9330532114979917 ) ) ;
#78793=CARTESIAN_POINT ( 'NONE',  ( 23.24537980070000032, 1509.679808356930153, 191.7928441131979866 ) ) ;
#78794=ORIENTED_EDGE ( 'NONE', *, *, #14745, .F. ) ;
#78795=CARTESIAN_POINT ( 'NONE',  ( -18.20051592215423142, 1459.364021588609603, 227.8976272857560730 ) ) ;
#78796=AXIS2_PLACEMENT_3D ( 'NONE', #45906, #35278, #1698 ) ;
#78798=CARTESIAN_POINT ( 'NONE',  ( 20.15304608505310213, 1509.294231923400048, 229.9324461821670127 ) ) ;
#78801=CARTESIAN_POINT ( 'NONE',  ( 19.77970829033609945, 1507.818029077260007, 229.2755469930129948 ) ) ;
#78803=CARTESIAN_POINT ( 'NONE',  ( 13.14149025202757670, 1443.060851088390791, 169.3996772419945103 ) ) ;
#78805=CARTESIAN_POINT ( 'NONE',  ( -6.814834796379999560, 1474.725719091730070, 264.8986983612979884 ) ) ;
#78810=CARTESIAN_POINT ( 'NONE',  ( 26.47490684719999976, 1509.166822683030205, 201.9133613274379968 ) ) ;
#78812=CARTESIAN_POINT ( 'NONE',  ( 5.526936513739999945, 1409.106065263330038, 188.1071742970979983 ) ) ;
#78813=CARTESIAN_POINT ( 'NONE',  ( 5.580754349969999417, 1425.065972486529972, 185.9108535249980036 ) ) ;
#78814=CARTESIAN_POINT ( 'NONE',  ( -12.38112447369999991, 1436.607677290789979, 151.2275677899980053 ) ) ;
#78818=CARTESIAN_POINT ( 'NONE',  ( -19.08699729579999982, 1452.246527754430190, 144.6803158024980007 ) ) ;
#78826=CARTESIAN_POINT ( 'NONE',  ( -44.43454715010000200, 1442.549948691149893, 270.0922452043980115 ) ) ;
#78828=CARTESIAN_POINT ( 'NONE',  ( 17.22039721829999692, 1409.679124255730130, 223.1987974457980215 ) ) ;
#78830=CARTESIAN_POINT ( 'NONE',  ( -14.61250254350000155, 1485.050473465629921, 224.2691043937979885 ) ) ;
#78833=PLANE ( 'NONE',  #76709 ) ;
#78834=CARTESIAN_POINT ( 'NONE',  ( 1.399926847669999974, 1507.072115598929940, 236.8180522793980174 ) ) ;
#78835=CARTESIAN_POINT ( 'NONE',  ( -6.229487579010000609, 1417.187363815429990, 231.8072993723980062 ) ) ;
#78836=EDGE_CURVE ( 'NONE', #48650, #55354, #63503, .T. ) ;
#78840=CARTESIAN_POINT ( 'NONE',  ( -45.37234497165430014, 1435.615442251129934, 266.4280287536979586 ) ) ;
#78843=CARTESIAN_POINT ( 'NONE',  ( 23.99508155959999911, 1435.335429155559950, 136.6133439143980013 ) ) ;
#78851=CARTESIAN_POINT ( 'NONE',  ( -15.63847246700000149, 1410.407006983229849, 191.1385721762979699 ) ) ;
#78853=ORIENTED_EDGE ( 'NONE', *, *, #16619, .T. ) ;
#78854=CARTESIAN_POINT ( 'NONE',  ( -16.44161674339963142, 1409.512373515832905, 225.1669987584983232 ) ) ;
#78855=AXIS2_PLACEMENT_3D ( 'NONE', #61351, #10352, #36669 ) ;
#78856=CARTESIAN_POINT ( 'NONE',  ( 0.4061596876509999676, 1451.157747844730238, 182.5691048874980140 ) ) ;
#78864=EDGE_CURVE ( 'NONE', #52333, #85422, #100500, .T. ) ;
#78867=CARTESIAN_POINT ( 'NONE',  ( -16.68259885503249862, 1411.554578397300020, 270.3635884854259643 ) ) ;
#78869=CARTESIAN_POINT ( 'NONE',  ( 8.049312594969689982, 1418.917536817879864, 232.8636318953529667 ) ) ;
#78872=VERTEX_POINT ( 'NONE', #105898 ) ;
#78873=ORIENTED_EDGE ( 'NONE', *, *, #109978, .T. ) ;
#78876=CARTESIAN_POINT ( 'NONE',  ( -0.5818514064668890429, 1408.933379414289902, 186.2126681199449934 ) ) ;
#78877=CARTESIAN_POINT ( 'NONE',  ( 3.688094639622395920, 1424.199184244893104, 183.9771557187304438 ) ) ;
#78878=CARTESIAN_POINT ( 'NONE',  ( -6.096353515327549211, 1406.294149656895570, 266.9463287792909227 ) ) ;
#78880=CARTESIAN_POINT ( 'NONE',  ( -17.67363391227470260, 1415.089996090750219, 207.5652716405009812 ) ) ;
#78881=CARTESIAN_POINT ( 'NONE',  ( -23.42424912799999959, 1430.786185988730040, 212.0133531227079970 ) ) ;
#78882=CARTESIAN_POINT ( 'NONE',  ( 5.300423936813779768, 1475.561024740650055, 269.2948677518700151 ) ) ;
#78884=CARTESIAN_POINT ( 'NONE',  ( 10.82658308979999973, 1445.294115142620058, 185.4165881730980061 ) ) ;
#78887=CARTESIAN_POINT ( 'NONE',  ( 22.76145762336689771, 1411.068184256920404, 214.2186865606036861 ) ) ;
#78888=CARTESIAN_POINT ( 'NONE',  ( 1.473900770646640046, 1482.958075957350047, 182.1667372775690126 ) ) ;
#78889=VERTEX_POINT ( 'NONE', #69560 ) ;
#78891=CARTESIAN_POINT ( 'NONE',  ( 26.19227466039749785, 1451.106985942830079, 136.5081610195809958 ) ) ;
#78892=CARTESIAN_POINT ( 'NONE',  ( 14.00875078090000159, 1416.819756528429934, 196.3921943334979971 ) ) ;
#78895=CARTESIAN_POINT ( 'NONE',  ( 19.04580826369999969, 1410.500985970229976, 195.3929509149980106 ) ) ;
#78896=CARTESIAN_POINT ( 'NONE',  ( 16.90742463041998178, 1444.994950788469168, 162.4348201727410981 ) ) ;
#78897=CARTESIAN_POINT ( 'NONE',  ( 3.050517026533811293, 1439.677820960868303, 184.1494276813981799 ) ) ;
#78898=CARTESIAN_POINT ( 'NONE',  ( -0.02597213800960000013, 1416.108377370330118, 233.5481719747979810 ) ) ;
#78900=CARTESIAN_POINT ( 'NONE',  ( 0.8424627026991029499, 1452.935544315429979, 183.3439428731419980 ) ) ;
#78901=CARTESIAN_POINT ( 'NONE',  ( 2.500000000000000000, 1448.210448412289907, 170.5244215879980061 ) ) ;
#78903=CARTESIAN_POINT ( 'NONE',  ( -3.835404308830568265, 1412.913060387329779, 202.1011854665805743 ) ) ;
#78907=DIRECTION ( 'NONE',  ( 1.137551646196209927E-09, 1.000000000000000000, -9.990831686207409361E-10 ) ) ;
#78910=CARTESIAN_POINT ( 'NONE',  ( -8602.628222780835131, 50.13405481578727318, -10923.45535519210353 ) ) ;
#78911=ADVANCED_FACE ( 'NONE', ( #10735 ), #68872, .F. ) ;
#78913=AXIS2_PLACEMENT_3D ( 'NONE', #99488, #75436, #109572 ) ;
#78914=CARTESIAN_POINT ( 'NONE',  ( 0.3821805048270000005, 1506.433683729329914, 231.1012307613979999 ) ) ;
#78915=CARTESIAN_POINT ( 'NONE',  ( -17.24149055319999846, 1446.934121893590145, 209.1218459616979999 ) ) ;
#78916=CARTESIAN_POINT ( 'NONE',  ( 38.96329220849997910, 1459.274185255430666, 266.3801432638982760 ) ) ;
#78918=CARTESIAN_POINT ( 'NONE',  ( -26.61274952006059991, 1468.149000416469789, 269.9851188083980560 ) ) ;
#78922=DIRECTION ( 'NONE',  ( 0.000000000000000000, -1.000000000000000000, 0.000000000000000000 ) ) ;
#78927=CARTESIAN_POINT ( 'NONE',  ( -15.15175306172240077, 1509.481969237379872, 236.4739884436810087 ) ) ;
#78928=CARTESIAN_POINT ( 'NONE',  ( 25.66628087189999974, 1469.241412578029895, 213.4071819949780036 ) ) ;
#78930=CARTESIAN_POINT ( 'NONE',  ( -15.40310530260000021, 1508.176735222329853, 231.4698242431979907 ) ) ;
#78933=CARTESIAN_POINT ( 'NONE',  ( 10.24761658979999979, 1409.091680548530121, 219.5424323772980131 ) ) ;
#78935=CARTESIAN_POINT ( 'NONE',  ( 0.1648540493162710119, 1483.364881617609853, 181.9498374863690060 ) ) ;
#78938=CARTESIAN_POINT ( 'NONE',  ( -0.5200257807070000071, 1450.894900823180024, 181.6063032255979977 ) ) ;
#78944=VERTEX_POINT ( 'NONE', #73942 ) ;
#78950=CARTESIAN_POINT ( 'NONE',  ( -4.453834213590135427, 1509.079627139014747, 238.2871813933543876 ) ) ;
#78955=CARTESIAN_POINT ( 'NONE',  ( 12.43454791605049969, 1409.347284361509992, 217.4061878439790121 ) ) ;
#78956=LINE ( 'NONE', #46461, #36545 ) ;
#78958=CARTESIAN_POINT ( 'NONE',  ( -17.43112864230000270, 1424.169315834030158, 191.5803361794979764 ) ) ;
#78960=EDGE_LOOP ( 'NONE', ( #29123, #82568, #57838, #52101 ) ) ;
#78964=ORIENTED_EDGE ( 'NONE', *, *, #46651, .T. ) ;
#78968=CARTESIAN_POINT ( 'NONE',  ( 23.59424604019999805, 1507.884706830530149, 222.5751569823979992 ) ) ;
#78970=CARTESIAN_POINT ( 'NONE',  ( -11.97668390569999985, 1433.616603791269881, 149.8660147765980071 ) ) ;
#78971=EDGE_CURVE ( 'NONE', #105450, #109428, #13611, .T. ) ;
#78972=CARTESIAN_POINT ( 'NONE',  ( 29.50369192380506433, 1509.962379296385507, 211.7848930765254920 ) ) ;
#78974=CARTESIAN_POINT ( 'NONE',  ( 4.911909971580000089, 1396.617946523930186, 220.6495969109980138 ) ) ;
#78975=CARTESIAN_POINT ( 'NONE',  ( 1.381906298289999890, 1417.049103970330179, 233.2953579960980051 ) ) ;
#78977=CARTESIAN_POINT ( 'NONE',  ( -0.5378485204050000856, 1471.144553927230163, 182.4732557751979982 ) ) ;
#78982=CARTESIAN_POINT ( 'NONE',  ( -13.04882216325809985, 1434.812040110809903, 149.3440682124420107 ) ) ;
#78984=CARTESIAN_POINT ( 'NONE',  ( 11.58690141939999840, 1425.690684998030292, 133.5558073867980227 ) ) ;
#78987=ADVANCED_FACE ( 'NONE', ( #107528 ), #43830, .T. ) ;
#78988=CARTESIAN_POINT ( 'NONE',  ( 40.54813384580009483, 1444.189903829430023, 137.0615966367320198 ) ) ;
#78991=CARTESIAN_POINT ( 'NONE',  ( -27.49404549240000151, 1488.693617964029954, 209.3049790079790000 ) ) ;
#78992=CARTESIAN_POINT ( 'NONE',  ( -10.38662965184200004, 1425.402516998919964, 95.13675362039579397 ) ) ;
#78993=CARTESIAN_POINT ( 'NONE',  ( 17.09872249335660044, 1410.735067943620152, 192.0960184572400067 ) ) ;
#78995=CARTESIAN_POINT ( 'NONE',  ( 0.6591021011063420421, 1395.936076739869804, 198.1345608290150153 ) ) ;
#78996=CARTESIAN_POINT ( 'NONE',  ( -19.59664182070000038, 1435.002040243690089, 208.4023078862850014 ) ) ;
#78997=CARTESIAN_POINT ( 'NONE',  ( -34.21122779019999882, 1429.487523400830014, 254.6787106624979629 ) ) ;
#78999=CARTESIAN_POINT ( 'NONE',  ( 28.49886664283559767, 1509.035040371930108, 209.4553795045120239 ) ) ;
#79001=CYLINDRICAL_SURFACE ( 'NONE', #6076, 0.9999999999999465983 ) ;
#79002=ORIENTED_EDGE ( 'NONE', *, *, #88133, .T. ) ;
#79006=CARTESIAN_POINT ( 'NONE',  ( -16.69641803230000221, 1458.740222332030044, 230.3336308253980178 ) ) ;
#79007=ORIENTED_EDGE ( 'NONE', *, *, #39126, .T. ) ;
#79013=CARTESIAN_POINT ( 'NONE',  ( -5.273680927263949769, 1398.098440474080235, 199.4684377759750191 ) ) ;
#79014=CARTESIAN_POINT ( 'NONE',  ( 8.076329059878878169, 1446.679444598521059, 154.0159284771656871 ) ) ;
#79017=CARTESIAN_POINT ( 'NONE',  ( 27.40792072111510080, 1509.298959737374616, 206.1637269058524282 ) ) ;
#79018=CARTESIAN_POINT ( 'NONE',  ( 2.025872226998560510, 1421.136586182680048, 183.1659243740039926 ) ) ;
#79021=CARTESIAN_POINT ( 'NONE',  ( 0.1681676109750000203, 1420.473121951529947, 182.7464980200980165 ) ) ;
#79024=ORIENTED_EDGE ( 'NONE', *, *, #52467, .T. ) ;
#79025=CARTESIAN_POINT ( 'NONE',  ( 11.86554121557050046, 1432.296927349550060, 149.9822551877360013 ) ) ;
#79026=CIRCLE ( 'NONE', #57603, 1.000000000000000000 ) ;
#79027=CARTESIAN_POINT ( 'NONE',  ( 13.21297046888754068, 1444.693905304529835, 187.3376099162051673 ) ) ;
#79029=DIRECTION ( 'NONE',  ( 0.000000000000000000, 0.000000000000000000, -1.000000000000000000 ) ) ;
#79031=CARTESIAN_POINT ( 'NONE',  ( 2.881519388670000126, 1507.413003788429933, 235.9584917197979905 ) ) ;
#79033=CARTESIAN_POINT ( 'NONE',  ( -6.451353027019999686, 1421.812455514629846, 186.8014209383979960 ) ) ;
#79034=CARTESIAN_POINT ( 'NONE',  ( 1.417322805690939935, 1410.048863607139992, 269.8655646141270381 ) ) ;
#79040=CARTESIAN_POINT ( 'NONE',  ( -17.26759053627300133, 1429.542278724649805, 191.2131399352340111 ) ) ;
#79045=ORIENTED_EDGE ( 'NONE', *, *, #85411, .F. ) ;
#79046=CARTESIAN_POINT ( 'NONE',  ( 1.199040866600000048E-14, 1419.211677883429957, 248.0989693021979861 ) ) ;
#79051=CARTESIAN_POINT ( 'NONE',  ( 17.47708894566800097, 1409.791774897460300, 270.0791891301039982 ) ) ;
#79053=VERTEX_POINT ( 'NONE', #33016 ) ;
#79059=CARTESIAN_POINT ( 'NONE',  ( -9.117626234630000326, 1442.289878148370008, 185.2642562222980018 ) ) ;
#79060=CARTESIAN_POINT ( 'NONE',  ( 19.47548006807109999, 1509.632698354770127, 231.9332913439310175 ) ) ;
#79062=CARTESIAN_POINT ( 'NONE',  ( -4.424139982966695861, 1432.332219231797808, 155.5697322143722943 ) ) ;
#79063=CARTESIAN_POINT ( 'NONE',  ( 2.917282800289999756, 1415.076022899730106, 231.8410176321980032 ) ) ;
#79065=CARTESIAN_POINT ( 'NONE',  ( -16.02253603680000182, 1459.141923948030126, 230.3636548079979889 ) ) ;
#79067=CARTESIAN_POINT ( 'NONE',  ( 44.05617169130000121, 1429.881624369530073, 266.7430392887980020 ) ) ;
#79069=CARTESIAN_POINT ( 'NONE',  ( 20.26752588049999915, 1435.348985798829972, 144.1465333546979934 ) ) ;
#79070=CARTESIAN_POINT ( 'NONE',  ( 19.68293457889999942, 1488.589411887629922, 190.0755286157979924 ) ) ;
#79071=CARTESIAN_POINT ( 'NONE',  ( -23.10492689500000196, 1433.621912620239982, 215.5179811059879853 ) ) ;
#79073=CARTESIAN_POINT ( 'NONE',  ( -9.885589491230001968, 1475.057254907329934, 266.9235355597979833 ) ) ;
#79075=CARTESIAN_POINT ( 'NONE',  ( -41.10478585342460178, 1442.607632416070146, 136.7995045943229968 ) ) ;
#79076=CARTESIAN_POINT ( 'NONE',  ( -7.121584071090000023, 1409.161751583130126, 195.9581075130980139 ) ) ;
#79077=CARTESIAN_POINT ( 'NONE',  ( -17.56697300799999795, 1414.971439108430104, 207.9608875356680073 ) ) ;
#79078=CARTESIAN_POINT ( 'NONE',  ( -11.97846764590000035, 1441.462071183699891, 187.7017596415979881 ) ) ;
#79081=CARTESIAN_POINT ( 'NONE',  ( -1.203801419936314954, 1419.233897949102811, 185.0625596308904051 ) ) ;
#79084=CARTESIAN_POINT ( 'NONE',  ( -11.07873686478040121, 1409.299938403639999, 199.0863655858090056 ) ) ;
#79086=CARTESIAN_POINT ( 'NONE',  ( -21.58938578137761866, 1409.666978351642001, 210.4204379443588664 ) ) ;
#79087=CARTESIAN_POINT ( 'NONE',  ( -45.63714053399999671, 1445.950958213619970, 268.9747508869979811 ) ) ;
#79089=CARTESIAN_POINT ( 'NONE',  ( 0.1761179889197699855, 1419.971149309630164, 184.0347958421160115 ) ) ;
#79090=CARTESIAN_POINT ( 'NONE',  ( -25.89799839909999690, 1509.146170697830030, 218.4252831721279904 ) ) ;
#79093=CARTESIAN_POINT ( 'NONE',  ( 16.85987604637189818, 1423.620959927220156, 227.7720207472910090 ) ) ;
#79094=CARTESIAN_POINT ( 'NONE',  ( 13.01304944610000192, 1416.520646107730045, 221.6242398431980121 ) ) ;
#79095=CARTESIAN_POINT ( 'NONE',  ( 14.80905694640000192, 1474.177104242629866, 223.3992951678980035 ) ) ;
#79100=CARTESIAN_POINT ( 'NONE',  ( 18.04214300190000131, 1416.520646107730045, 208.7607579491829881 ) ) ;
#79101=AXIS2_PLACEMENT_3D ( 'NONE', #96829, #11707, #56475 ) ;
#79102=CARTESIAN_POINT ( 'NONE',  ( -2.829801042252522159, 1451.871858332230204, 184.7457192350124160 ) ) ;
#79104=ADVANCED_FACE ( 'NONE', ( #32487 ), #50950, .F. ) ;
#79105=CARTESIAN_POINT ( 'NONE',  ( 22.40106396050000015, 1409.695322778229865, 210.5405262121579995 ) ) ;
#79108=CARTESIAN_POINT ( 'NONE',  ( -5.360171697043470296, 1422.243961768539748, 144.5806141462400092 ) ) ;
#79109=CARTESIAN_POINT ( 'NONE',  ( -10.97356441630000212, 1432.589727400840047, 151.7700027225980079 ) ) ;
#79112=CARTESIAN_POINT ( 'NONE',  ( 0.3821805048270000005, 1506.433683729329914, 231.1012307613979999 ) ) ;
#79118=CARTESIAN_POINT ( 'NONE',  ( -16.74544130042350076, 1485.914225547749993, 187.7220481146609927 ) ) ;
#79121=CARTESIAN_POINT ( 'NONE',  ( -4.276331814141159704, 1441.049878954770065, 157.0171284178840097 ) ) ;
#79123=ORIENTED_EDGE ( 'NONE', *, *, #110361, .F. ) ;
#79125=VERTEX_POINT ( 'NONE', #107946 ) ;
#79126=CARTESIAN_POINT ( 'NONE',  ( 11.82610189953429902, 1433.713742287859759, 150.7576001896150046 ) ) ;
#79127=FACE_OUTER_BOUND ( 'NONE', #103357, .T. ) ;
#79130=FACE_OUTER_BOUND ( 'NONE', #46452, .T. ) ;
#79131=CARTESIAN_POINT ( 'NONE',  ( 15.97992989932220098, 1420.985315616920161, 191.2040731956429909 ) ) ;
#79132=CARTESIAN_POINT ( 'NONE',  ( 13.89869200000000049, 1452.835253893030085, 223.8385666725980059 ) ) ;
#79133=CARTESIAN_POINT ( 'NONE',  ( 11.98951922200000020, 1442.759074889710064, 150.6922381223979812 ) ) ;
#79134=CARTESIAN_POINT ( 'NONE',  ( 1.430900451930000150, 1488.174586716330168, 181.9313141933980091 ) ) ;
#79138=CARTESIAN_POINT ( 'NONE',  ( 38.70428745349820332, 1437.478004125059897, 134.0999999972650016 ) ) ;
#79141=CARTESIAN_POINT ( 'NONE',  ( 13.81563158420089898, 1434.988513889579963, 148.7679932446569921 ) ) ;
#79143=ORIENTED_EDGE ( 'NONE', *, *, #36043, .F. ) ;
#79146=CARTESIAN_POINT ( 'NONE',  ( 12.79376191942176355, 1444.983190770407418, 169.4500884308193918 ) ) ;
#79147=CARTESIAN_POINT ( 'NONE',  ( -3.168849912869999841, 1464.840305621330117, 237.5147281217979867 ) ) ;
#79153=CARTESIAN_POINT ( 'NONE',  ( -17.47732762797510375, 1448.300284982579797, 218.1790054843986866 ) ) ;
#79155=CARTESIAN_POINT ( 'NONE',  ( 4.240346634148639993, 1446.384605460860030, 162.7848567526920078 ) ) ;
#79156=EDGE_CURVE ( 'NONE', #79540, #35766, #64008, .T. ) ;
#79160=B_SPLINE_CURVE_WITH_KNOTS ( 'NONE', 5,
 ( #77157, #40781, #67661, #41341, #74957, #75510 ),
 .UNSPECIFIED., .F., .F.,
 ( 6, 6 ),
 ( 0.000000000000000000, 1.000000000000000000 ),
 .UNSPECIFIED. ) ;
#79161=VERTEX_POINT ( 'NONE', #12232 ) ;
#79162=CARTESIAN_POINT ( 'NONE',  ( 24.52819686174909819, 1440.913060387330006, 237.5178590015389943 ) ) ;
#79163=CARTESIAN_POINT ( 'NONE',  ( -18.54934599400000295, 1509.628428428030020, 185.6625796504979746 ) ) ;
#79164=ORIENTED_EDGE ( 'NONE', *, *, #36424, .T. ) ;
#79166=CARTESIAN_POINT ( 'NONE',  ( -15.00074258620000123, 1410.809359295230024, 190.7496526661980170 ) ) ;
#79168=CARTESIAN_POINT ( 'NONE',  ( -24.89939544960000006, 1440.978110081060095, 210.4300214544979895 ) ) ;
#79170=CARTESIAN_POINT ( 'NONE',  ( -11.20854072740000085, 1414.996442553730049, 195.7122652358980304 ) ) ;
#79171=B_SPLINE_CURVE_WITH_KNOTS ( 'NONE', 5,
 ( #10086, #96866, #10652, #36392, #54329, #45914, #44260, #19014, #80050 ),
 .UNSPECIFIED., .F., .F.,
 ( 6, 3, 6 ),
 ( 0.000000000000000000, 0.4153946668491772520, 1.000000000000000000 ),
 .UNSPECIFIED. ) ;
#79173=CARTESIAN_POINT ( 'NONE',  ( -12.34777630145106464, 1434.274821752217804, 147.3832369842282333 ) ) ;
#79174=CARTESIAN_POINT ( 'NONE',  ( -12.40409029009999919, 1434.420083644240094, 149.2722339323979952 ) ) ;
#79175=CARTESIAN_POINT ( 'NONE',  ( 20.10060672000000181, 1435.200054686760041, 143.0090892206980016 ) ) ;
#79176=CARTESIAN_POINT ( 'NONE',  ( 4.645519865709999863, 1464.326374023630024, 236.0120472652980084 ) ) ;
#79181=CARTESIAN_POINT ( 'NONE',  ( 28.30178298809999760, 1508.659383665829864, 208.9628371413840000 ) ) ;
#79183=CARTESIAN_POINT ( 'NONE',  ( -18.10327300539999840, 1416.823634022829992, 209.2064603946170109 ) ) ;
#79184=( BOUNDED_CURVE ( )  B_SPLINE_CURVE ( 3, ( #22996, #4574, #74543, #22430 ),
 .UNSPECIFIED., .F., .F. ) 
 B_SPLINE_CURVE_WITH_KNOTS ( ( 4, 4 ),
 ( 2.995780018818399615, 3.061202631949359709 ),
 .UNSPECIFIED. ) 
 CURVE ( )  GEOMETRIC_REPRESENTATION_ITEM ( )  RATIONAL_B_SPLINE_CURVE ( ( 1.000000000000000000, 0.9996433552776613496, 0.9996433552776613496, 1.000000000000000000 ) ) 
 REPRESENTATION_ITEM ( '' )  );
#79189=CARTESIAN_POINT ( 'NONE',  ( 22.11712025849999819, 1461.968260155829967, 248.4077083995979933 ) ) ;
#79190=CARTESIAN_POINT ( 'NONE',  ( -17.73420755029999896, 1458.087872027529784, 230.3493948207980395 ) ) ;
#79192=CARTESIAN_POINT ( 'NONE',  ( -5.668048117390779517, 1509.094485824230105, 237.7474958631910056 ) ) ;
#79193=CARTESIAN_POINT ( 'NONE',  ( -22.47453833620000196, 1450.822336665940156, 220.0988823947979824 ) ) ;
#79194=CARTESIAN_POINT ( 'NONE',  ( -21.72999032162606525, 1411.032272965445372, 201.5736073022784467 ) ) ;
#79195=CARTESIAN_POINT ( 'NONE',  ( 19.01627661470000064, 1456.566751503029991, 225.7645316237980069 ) ) ;
#79196=CARTESIAN_POINT ( 'NONE',  ( 0.2703785145419999592, 1470.804162800830227, 188.4112092155980065 ) ) ;
#79200=CARTESIAN_POINT ( 'NONE',  ( 0.5499324067410000794, 1406.779957305129756, 269.6499793198979660 ) ) ;
#79202=CARTESIAN_POINT ( 'NONE',  ( 12.79131911510310005, 1470.700977594940014, 269.6259408100920041 ) ) ;
#79203=CARTESIAN_POINT ( 'NONE',  ( 2.478710532469999617, 1435.788277702919913, 157.6232518516980008 ) ) ;
#79204=CARTESIAN_POINT ( 'NONE',  ( -27.87287880750000113, 1445.634712502449929, 137.2901167009979986 ) ) ;
#79205=B_SPLINE_CURVE_WITH_KNOTS ( 'NONE', 3,
 ( #101921, #16794, #75655, #109795, #24646, #84033, #7332, #110339, #33073, #101357, #17911, #50457, #85129, #42588, #84581, #76741, #58847, #35288, #52107, #92980, #53, #85681, #7873, #86237, #51544, #102476, #42041, #25765, #33611, #43696, #59964, #34734, #77850, #1158, #8978, #58298, #43149, #62746, #10084, #44819, #35851, #29098, #63284, #88456, #10650, #44258, #52656, #37496, #69474, #11209, #18459, #105820, #88991, #104696, #86793, #11743, #78400, #12279, #71702, #27433, #61616, #27991, #28547, #1711, #97398, #20667, #45912, #103594, #62176, #70035, #71132, #3370, #46473, #53215, #80048, #96864, #45372, #105253, #20133, #70579, #96303, #26894 ),
 .UNSPECIFIED., .F., .F.,
 ( 4, 2, 2, 1, 1, 1, 1, 2, 2, 2, 2, 1, 1, 1, 1, 1, 1, 2, 2, 2, 2, 2, 1, 1, 1, 1, 1, 1, 2, 2, 2, 2, 2, 2, 2, 1, 1, 1, 1, 1, 2, 2, 2, 2, 2, 1, 1, 1, 1, 1, 2, 2, 2, 4 ),
 ( 0.000000000000000000, 0.06249999999717108234, 0.09374999999575661658, 0.1093749999950493351, 0.1171874999947023904, 0.1210937499945289597, 0.1230468749944356316, 0.1240234374943823825, 0.1249999999943291334, 0.1874999999906900305, 0.2187499999888705138, 0.2343749999879550239, 0.2421874999875027745, 0.2460937499872765666, 0.2480468749871633793, 0.2490234374871120038, 0.2495117187370914924, 0.2497558593620759493, 0.2499999999870604062, 0.3124999999819546015, 0.3437499999793964811, 0.3593749999781175597, 0.3671874999774781267, 0.3710937499771584935, 0.3730468749769986769, 0.3740234374769187964, 0.3745117187268751091, 0.3747558593518534042, 0.3748779296643461323, 0.3749999999768389158, 0.4062499999757702707, 0.4374999999747016255, 0.4687499999736333134, 0.4843749999730991296, 0.4921874999728319544, 0.4960937499727078315, 0.4980468749726460476, 0.4990234374726151279, 0.4995117187226121858, 0.4997558593476237876, 0.4998779296601298938, 0.4999999999726359445, 0.6249999999793900418, 0.6874999999827670072, 0.7187499999844575438, 0.7343749999853008692, 0.7421874999857207555, 0.7460937499859289224, 0.7480468749860331723, 0.7490234374860871291, 0.7495117187361139965, 0.7499999999861407529, 0.8749999999930704320, 1.000000000000000000 ),
 .UNSPECIFIED. ) ;
#79206=CARTESIAN_POINT ( 'NONE',  ( -45.22500823550609539, 1440.913060396110041, 265.7132613544649757 ) ) ;
#79207=CARTESIAN_POINT ( 'NONE',  ( -26.18941195200000394, 1448.070469784879833, 137.2980963937980050 ) ) ;
#79209=LINE ( 'NONE', #62423, #28832 ) ;
#79210=CARTESIAN_POINT ( 'NONE',  ( 2.501005634817679901, 1448.957421962729995, 154.2481697353020138 ) ) ;
#79214=CARTESIAN_POINT ( 'NONE',  ( 0.8115383875230000044, 1428.579607037230062, 149.5143047311979672 ) ) ;
#79217=CARTESIAN_POINT ( 'NONE',  ( -0.7768863733780000391, 1475.978544761829880, 267.2347138124980006 ) ) ;
#79221=CARTESIAN_POINT ( 'NONE',  ( 3.156166260290000025, 1466.544008048530031, 236.1241471695980181 ) ) ;
#79223=CARTESIAN_POINT ( 'NONE',  ( -18.76071169450000298, 1415.996778985530000, 207.9585495669979878 ) ) ;
#79224=CARTESIAN_POINT ( 'NONE',  ( 11.86919408122879993, 1432.567571621249954, 149.9818808296639929 ) ) ;
#79225=CARTESIAN_POINT ( 'NONE',  ( 26.55522734722419997, 1435.968459176769784, 136.4840774741649909 ) ) ;
#79226=CARTESIAN_POINT ( 'NONE',  ( -7.275039510604740300, 1396.167110366489851, 217.4379085327780103 ) ) ;
#79227=CARTESIAN_POINT ( 'NONE',  ( -14.89068146630000022, 1422.385042061529930, 229.1196406006980055 ) ) ;
#79228=CARTESIAN_POINT ( 'NONE',  ( -16.90423294166100021, 1409.877128282629883, 225.7261434717579789 ) ) ;
#79229=CARTESIAN_POINT ( 'NONE',  ( 9.788350359310001636, 1441.600846913620217, 148.8293326998980035 ) ) ;
#79232=CARTESIAN_POINT ( 'NONE',  ( 2.425147433399999830, 1410.373299717429973, 231.7452901618979979 ) ) ;
#79234=CARTESIAN_POINT ( 'NONE',  ( 10.49341911620000189, 1425.372128361229898, 101.9093738396979916 ) ) ;
#79237=CARTESIAN_POINT ( 'NONE',  ( -12.53380498098199602, 1442.773887284840612, 151.6125157144320212 ) ) ;
#79238=B_SPLINE_CURVE_WITH_KNOTS ( 'NONE', 5,
 ( #81642, #4947, #39089, #99548, #22273, #90606 ),
 .UNSPECIFIED., .F., .F.,
 ( 6, 6 ),
 ( 0.000000000000000000, 1.000000000000000000 ),
 .UNSPECIFIED. ) ;
#79244=CARTESIAN_POINT ( 'NONE',  ( 2.831794687379999953, 1449.370045669049887, 183.5403809041980026 ) ) ;
#79246=CARTESIAN_POINT ( 'NONE',  ( -3.168849847270283959, 1464.840305569651491, 237.5147278964450948 ) ) ;
#79249=ADVANCED_FACE ( 'NONE', ( #13867 ), #90590, .F. ) ;
#79250=CARTESIAN_POINT ( 'NONE',  ( -41.48883687280000032, 1443.959535018250108, 136.5760642042980066 ) ) ;
#79251=CARTESIAN_POINT ( 'NONE',  ( 0.1053863349198899957, 1507.126692871930118, 237.3870350735109866 ) ) ;
#79252=CARTESIAN_POINT ( 'NONE',  ( 15.96958168569999970, 1519.913060387329779, 226.4768549569980109 ) ) ;
#79255=CARTESIAN_POINT ( 'NONE',  ( 11.60004869885203682, 1426.786827912535728, 134.3786173235958472 ) ) ;
#79259=CARTESIAN_POINT ( 'NONE',  ( -2.500000000000000000, 1448.763984273669848, 157.0970650823900314 ) ) ;
#79260=CARTESIAN_POINT ( 'NONE',  ( 6.662077426295040183, 1396.145705257569944, 217.9277218839869761 ) ) ;
#79261=CARTESIAN_POINT ( 'NONE',  ( 3.460935634467220190, 1409.033918922830026, 194.4343271261309951 ) ) ;
#79262=CARTESIAN_POINT ( 'NONE',  ( -3.834150157287569805, 1405.859129154519906, 267.5313358287059486 ) ) ;
#79263=CARTESIAN_POINT ( 'NONE',  ( 40.26396426040000165, 1444.186530281040177, 137.1012295722979957 ) ) ;
#79265=CARTESIAN_POINT ( 'NONE',  ( -11.57624701299999970, 1432.320296571700055, 151.1967064316980043 ) ) ;
#79266=CARTESIAN_POINT ( 'NONE',  ( 11.79480876540000089, 1441.728078750129953, 187.9005510439980071 ) ) ;
#79267=ORIENTED_EDGE ( 'NONE', *, *, #75380, .F. ) ;
#79276=EDGE_CURVE ( 'NONE', #103585, #87841, #106801, .T. ) ;
#79279=CARTESIAN_POINT ( 'NONE',  ( -16.02094686025720094, 1507.732436784892116, 185.5304883000871428 ) ) ;
#79280=CARTESIAN_POINT ( 'NONE',  ( -41.26944936248266771, 1435.051291618910000, 269.6336527597242707 ) ) ;
#79281=CARTESIAN_POINT ( 'NONE',  ( 0.000000000000000000, 1450.913060387330006, 198.0847581327979867 ) ) ;
#79282=CARTESIAN_POINT ( 'NONE',  ( -3.706743637329999785, 1410.419263482230235, 232.3104563135979959 ) ) ;
#79284=ORIENTED_EDGE ( 'NONE', *, *, #105656, .T. ) ;
#79285=CARTESIAN_POINT ( 'NONE',  ( 30.80316622530000004, 1451.837341253830118, 134.8070091183980139 ) ) ;
#79289=CARTESIAN_POINT ( 'NONE',  ( -25.47400523009999773, 1435.387084339240118, 135.4904355849980107 ) ) ;
#79290=CARTESIAN_POINT ( 'NONE',  ( 24.79113421610179913, 1415.879394787770252, 269.6862526298410216 ) ) ;
#79293=CARTESIAN_POINT ( 'NONE',  ( 0.01703802077549729579, 1507.628843765722650, 237.4425282897537386 ) ) ;
#79298=CARTESIAN_POINT ( 'NONE',  ( 15.33708232923881987, 1509.448643104055918, 184.3329835401579260 ) ) ;
#79299=CARTESIAN_POINT ( 'NONE',  ( -14.16989803769999945, 1420.440733405429910, 227.4201729013980184 ) ) ;
#79301=ORIENTED_EDGE ( 'NONE', *, *, #105036, .F. ) ;
#79304=CARTESIAN_POINT ( 'NONE',  ( 16.65976538191360135, 1469.007159623620055, 229.3912229546239985 ) ) ;
#79306=CARTESIAN_POINT ( 'NONE',  ( -22.73782236065209972, 1507.861788290109871, 224.9164081595820051 ) ) ;
#79307=CARTESIAN_POINT ( 'NONE',  ( -1.802301037019999885, 1409.910657972530089, 186.0681197405980072 ) ) ;
#79308=CARTESIAN_POINT ( 'NONE',  ( -0.2331143098109999812, 1408.921200918430031, 231.7611568695980111 ) ) ;
#79309=CARTESIAN_POINT ( 'NONE',  ( -14.27756185697911029, 1416.835288273484821, 221.7190706085977467 ) ) ;
#79312=CARTESIAN_POINT ( 'NONE',  ( 15.50537652237009922, 1477.920142942969960, 194.4487094663240043 ) ) ;
#79313=CARTESIAN_POINT ( 'NONE',  ( 18.87980474539999776, 1507.654596655130035, 188.5454329983980131 ) ) ;
#79316=CARTESIAN_POINT ( 'NONE',  ( -12.81185530964340025, 1416.835419214280137, 196.2456592538570135 ) ) ;
#79317=CARTESIAN_POINT ( 'NONE',  ( -11.87933480400000086, 1508.913060324029857, 182.4413436122979988 ) ) ;
#79319=CARTESIAN_POINT ( 'NONE',  ( 2.446918720040000217, 1417.581962241529936, 234.9465420055979905 ) ) ;
#79324=CARTESIAN_POINT ( 'NONE',  ( -16.57358609848514064, 1410.166789121471311, 191.9182324867213936 ) ) ;
#79325=CARTESIAN_POINT ( 'NONE',  ( 4.363122647530000009, 1423.854802298929826, 172.2701767054979882 ) ) ;
#79326=CARTESIAN_POINT ( 'NONE',  ( -18.16339525799999777, 1424.367498598930069, 225.5894832976980240 ) ) ;
#79327=CARTESIAN_POINT ( 'NONE',  ( -18.07916955490000177, 1435.128322693429936, 145.8330392763979830 ) ) ;
#79330=CARTESIAN_POINT ( 'NONE',  ( 0.5943821362729999613, 1416.311719779230089, 190.5346383329979858 ) ) ;
#79331=CARTESIAN_POINT ( 'NONE',  ( 0.5620975284970839425, 1416.851343896850040, 190.4751211475700075 ) ) ;
#79333=ORIENTED_EDGE ( 'NONE', *, *, #71060, .F. ) ;
#79334=CARTESIAN_POINT ( 'NONE',  ( 1.325823199544269748, 1507.620489763490014, 186.1815209864240046 ) ) ;
#79335=CARTESIAN_POINT ( 'NONE',  ( 26.96771577539999853, 1508.002232633729818, 206.7596878312280069 ) ) ;
#79336=CARTESIAN_POINT ( 'NONE',  ( -24.09224057910000028, 1438.023770130810135, 211.8323676549379968 ) ) ;
#79347=DIRECTION ( 'NONE',  ( 0.000000000000000000, -1.000000000000000000, 0.000000000000000000 ) ) ;
#79349=CARTESIAN_POINT ( 'NONE',  ( 21.50111106039999953, 1509.340465056330004, 190.1785649164980043 ) ) ;
#79350=ORIENTED_EDGE ( 'NONE', *, *, #26356, .F. ) ;
#79352=B_SPLINE_CURVE_WITH_KNOTS ( 'NONE', 3,
 ( #17229, #1590, #51426, #9422, #93414, #9972, #77192, #50345, #17787, #52543, #33493, #60393, #86675, #34067, #103464, #59841, #102367, #27322 ),
 .UNSPECIFIED., .F., .F.,
 ( 4, 2, 1, 1, 2, 2, 2, 1, 1, 2, 4 ),
 ( 0.5596618113830474917, 0.5734223797774827824, 0.5871829481719181842, 0.6147040849608105262, 0.6697463585384014761, 0.7798309056937928752, 0.7935914740879851381, 0.8073520424821772901, 0.8348731792705625931, 0.8899154528471214798, 1.000000000000000000 ),
 .UNSPECIFIED. ) ;
#79355=ORIENTED_EDGE ( 'NONE', *, *, #84249, .F. ) ;
#79356=ORIENTED_EDGE ( 'NONE', *, *, #87713, .F. ) ;
#79359=CARTESIAN_POINT ( 'NONE',  ( 13.14376209273458329, 1443.062932975139347, 169.3993363818228488 ) ) ;
#79360=CARTESIAN_POINT ( 'NONE',  ( 22.00315959510000141, 1506.810797420329891, 208.8865261091119976 ) ) ;
#79364=CARTESIAN_POINT ( 'NONE',  ( -11.12212972500000063, 1433.940546708779948, 151.6712922175980225 ) ) ;
#79366=CARTESIAN_POINT ( 'NONE',  ( -19.68929325700000277, 1486.263866003429939, 189.9954379505980171 ) ) ;
#79367=CARTESIAN_POINT ( 'NONE',  ( 5.966377939340000047, 1409.624321257429983, 186.9574265255979810 ) ) ;
#79369=CARTESIAN_POINT ( 'NONE',  ( -12.84239781829999849, 1435.935717376499952, 150.8114785589980045 ) ) ;
#79370=FACE_OUTER_BOUND ( 'NONE', #3366, .T. ) ;
#79372=CARTESIAN_POINT ( 'NONE',  ( -9.452332281189999463, 1451.760532249029893, 152.6698088060980183 ) ) ;
#79377=CARTESIAN_POINT ( 'NONE',  ( -44.43455565579999700, 1440.913065169949959, 270.0922445381979742 ) ) ;
#79379=CARTESIAN_POINT ( 'NONE',  ( 17.84751137929999842, 1410.898165765230260, 223.1918699671979880 ) ) ;
#79380=FACE_OUTER_BOUND ( 'NONE', #21444, .T. ) ;
#79381=B_SPLINE_CURVE_WITH_KNOTS ( 'NONE', 3,
 ( #27507, #53855, #3435, #52182, #18534, #37566, #26397, #71767, #1225, #79585, #86313, #17987, #1785, #53288, #45984, #60591, #2345, #52729, #104219, #44331, #11814, #95816, #9597, #77918, #70107, #87991, #10722, #2890, #35361, #54397, #103668, #69547, #96372, #19651, #88530, #80116, #26968, #61156, #95272, #105322 ),
 .UNSPECIFIED., .F., .F.,
 ( 4, 3, 3, 3, 3, 3, 3, 3, 3, 3, 3, 3, 3, 4 ),
 ( -25.42450308940000170, -24.37555945047400030, -23.28024511109189731, -22.14444905835580002, -20.97885384835930012, -19.74476178579540075, -18.44871831345919944, -17.06465298523080065, -15.53335940394270054, -12.73670746646559948, -11.09712870486940162, -9.657147941009078806, -8.324531407576071018, -7.064711944746168371 ),
 .UNSPECIFIED. ) ;
#79382=CARTESIAN_POINT ( 'NONE',  ( 12.29727565780000020, 1497.713060387329961, 191.0778421084980039 ) ) ;
#79384=CARTESIAN_POINT ( 'NONE',  ( -14.33548068480000026, 1422.080119723229927, 229.2153237933979710 ) ) ;
#79385=CARTESIAN_POINT ( 'NONE',  ( -1.342620828053903592, 1484.506070987844851, 182.3616606809996483 ) ) ;
#79387=CARTESIAN_POINT ( 'NONE',  ( -44.01834660311930492, 1430.717886937790126, 268.5615389372139816 ) ) ;
#79389=ORIENTED_EDGE ( 'NONE', *, *, #90472, .F. ) ;
#79392=EDGE_LOOP ( 'NONE', ( #15346, #64255, #110074, #7501 ) ) ;
#79395=CARTESIAN_POINT ( 'NONE',  ( -20.59684415610000130, 1507.762623716230109, 190.3921826404979925 ) ) ;
#79396=CARTESIAN_POINT ( 'NONE',  ( -9.380213083140001018, 1425.410769174930010, 187.4587521971979811 ) ) ;
#79397=AXIS2_PLACEMENT_3D ( 'NONE', #100603, #18663, #60720 ) ;
#79400=EDGE_LOOP ( 'NONE', ( #23296, #96620, #14345, #93774 ) ) ;
#79404=B_SPLINE_CURVE_WITH_KNOTS ( 'NONE', 4,
 ( #94567, #7809, #103522, #17839, #9471 ),
 .UNSPECIFIED., .F., .F.,
 ( 5, 5 ),
 ( 3.613988937050000239, 5.260361675040000407 ),
 .UNSPECIFIED. ) ;
#79409=CARTESIAN_POINT ( 'NONE',  ( -16.42979742323149850, 1412.363408827170133, 269.8873871863210070 ) ) ;
#79411=CARTESIAN_POINT ( 'NONE',  ( -2.409586283469999923, 1426.663880916129983, 144.1938086916980239 ) ) ;
#79414=EDGE_LOOP ( 'NONE', ( #107736, #90834, #16905, #20604, #59402, #108704 ) ) ;
#79416=CARTESIAN_POINT ( 'NONE',  ( 42.06154873321850118, 1454.182881615767201, 269.0741535282402879 ) ) ;
#79417=EDGE_CURVE ( 'NONE', #27144, #98691, #61648, .T. ) ;
#79419=CARTESIAN_POINT ( 'NONE',  ( 3.639664930319541636, 1424.874334646760644, 184.8560718889175121 ) ) ;
#79423=CARTESIAN_POINT ( 'NONE',  ( -18.22757619631530090, 1415.441076447700198, 207.5675272910649767 ) ) ;
#79424=CARTESIAN_POINT ( 'NONE',  ( -22.50079280529999792, 1430.784053779030046, 216.6565829457279904 ) ) ;
#79425=CARTESIAN_POINT ( 'NONE',  ( 10.67568936471529994, 1475.522394824059802, 267.8226452972320430 ) ) ;
#79426=CARTESIAN_POINT ( 'NONE',  ( -9.791756963356650800, 1464.727237775841331, 232.4252867197243120 ) ) ;
#79427=CARTESIAN_POINT ( 'NONE',  ( 5.558723128650000511, 1446.585823782530042, 184.2862713098979839 ) ) ;
#79430=CARTESIAN_POINT ( 'NONE',  ( 18.75028616197712950, 1410.930186477558209, 221.9761678810336036 ) ) ;
#79431=CARTESIAN_POINT ( 'NONE',  ( 1.473031652072160025, 1483.720148366529884, 182.1335069566439984 ) ) ;
#79432=VERTEX_POINT ( 'NONE', #101735 ) ;
#79433=CARTESIAN_POINT ( 'NONE',  ( -0.6472592568835300320, 1457.969941384779986, 229.6490092412300044 ) ) ;
#79434=CARTESIAN_POINT ( 'NONE',  ( 26.11955021798470256, 1451.995689794530108, 135.1738199034059846 ) ) ;
#79435=CARTESIAN_POINT ( 'NONE',  ( -13.02322703936409987, 1416.825784014559986, 196.6108461303639672 ) ) ;
#79438=CARTESIAN_POINT ( 'NONE',  ( 17.85589594940000424, 1410.900194280930009, 193.2270198764980194 ) ) ;
#79439=CARTESIAN_POINT ( 'NONE',  ( 12.91247410300000276, 1445.052233488288948, 177.4417055768979026 ) ) ;
#79440=CARTESIAN_POINT ( 'NONE',  ( 17.60627508980000044, 1410.895669370830092, 224.8086596393980017 ) ) ;
#79441=CARTESIAN_POINT ( 'NONE',  ( -0.02516806119179999801, 1415.404723302029879, 233.4400559027980080 ) ) ;
#79443=CARTESIAN_POINT ( 'NONE',  ( 1.074521542462559820, 1452.881655443580257, 183.3871671006969848 ) ) ;
#79447=VERTEX_POINT ( 'NONE', #7689 ) ;
#79454=CARTESIAN_POINT ( 'NONE',  ( -38.01811172100560299, 1448.806981927099969, 136.3823620645019901 ) ) ;
#79457=CARTESIAN_POINT ( 'NONE',  ( 1.376676550539999851E-14, 1458.952956304630106, 234.3916895801979763 ) ) ;
#79458=CARTESIAN_POINT ( 'NONE',  ( 45.67177343720949523, 1440.913060382069943, 266.1885934449759930 ) ) ;
#79459=CARTESIAN_POINT ( 'NONE',  ( 11.41977517999999847, 1433.011620482069929, 151.3551162631979992 ) ) ;
#79460=CARTESIAN_POINT ( 'NONE',  ( -44.70486280913989674, 1448.425642251100044, 269.0002212091439446 ) ) ;
#79462=CARTESIAN_POINT ( 'NONE',  ( -21.92914334769999840, 1508.011510023030041, 226.2921371285980001 ) ) ;
#79464=VERTEX_POINT ( 'NONE', #61437 ) ;
#79467=CARTESIAN_POINT ( 'NONE',  ( 15.56469051819999905, 1506.798305132829910, 225.0756798403980099 ) ) ;
#79468=CARTESIAN_POINT ( 'NONE',  ( -4.703685162790000263, 1486.384485551830039, 182.0120322998980100 ) ) ;
#79471=CARTESIAN_POINT ( 'NONE',  ( 24.42679094799999717, 1430.357408108330219, 211.6184629891579903 ) ) ;
#79474=CARTESIAN_POINT ( 'NONE',  ( -12.57479191030000010, 1509.295195185829925, 234.7571869286980188 ) ) ;
#79479=ADVANCED_FACE ( 'NONE', ( #34546 ), #27811, .F. ) ;
#79484=CARTESIAN_POINT ( 'NONE',  ( -16.68463233076019492, 1445.052233488289630, 162.0935120523188857 ) ) ;
#79487=CARTESIAN_POINT ( 'NONE',  ( -38.02701353892550173, 1450.427746997079794, 134.0999999984749991 ) ) ;
#79491=EDGE_CURVE ( 'NONE', #99599, #18619, #35053, .T. ) ;
#79495=EDGE_CURVE ( 'NONE', #22249, #14981, #33492, .T. ) ;
#79499=CARTESIAN_POINT ( 'NONE',  ( 9.257676694381489213, 1409.236345580020043, 220.8738777432600102 ) ) ;
#79500=DIRECTION ( 'NONE',  ( -9.551066682124683589E-08, 1.946171191268429024E-07, -0.9999999999999764633 ) ) ;
#79502=CARTESIAN_POINT ( 'NONE',  ( -18.11586804879999946, 1430.614621825330005, 192.0644440209979962 ) ) ;
#79506=DIRECTION ( 'NONE',  ( 0.03489949694567519994, 0.9993908270106039993, -7.428258325848019394E-09 ) ) ;
#79509=CARTESIAN_POINT ( 'NONE',  ( 18.37311908421290241, 1459.092070059970183, 227.7653000740450011 ) ) ;
#79511=CARTESIAN_POINT ( 'NONE',  ( -11.21624399399999916, 1434.255326149100028, 151.6033521221980038 ) ) ;
#79512=CARTESIAN_POINT ( 'NONE',  ( 29.52276419461297152, 1509.964122545872442, 211.6544716486868367 ) ) ;
#79514=CARTESIAN_POINT ( 'NONE',  ( 5.086366865409999605, 1397.753027540630001, 221.1576708939979881 ) ) ;
#79517=CARTESIAN_POINT ( 'NONE',  ( -1.192273007929999906, 1462.370957484029987, 183.1676254752979958 ) ) ;
#79521=CARTESIAN_POINT ( 'NONE',  ( -12.92355159029609979, 1434.740261887239967, 149.3124598003599885 ) ) ;
#79522=B_SPLINE_SURFACE_WITH_KNOTS ( 'NONE', 4, 5, ( 
 ( #2016, #103320, #18218, #10381, #36152, #70336 ),
 ( #5295, #99333, #97702, #39453, #37253, #79819 ),
 ( #3125, #13120, #65222, #38881, #73626, #56257 ),
 ( #106644, #38336, #89303, #81427, #47303, #89848 ),
 ( #54629, #88762, #71993, #12599, #73062, #64681 ) ),
 .UNSPECIFIED., .F., .F., .F.,
 ( 5, 5 ),
 ( 6, 6 ),
 ( 9.410946460789999080, 10.17443977840000002 ),
 ( 0.000000000000000000, 2.000000000000000000 ),
 .UNSPECIFIED. ) ;
#79524=CARTESIAN_POINT ( 'NONE',  ( 19.61399504222830004, 1475.927339034750048, 226.7148328204089864 ) ) ;
#79526=B_SPLINE_CURVE_WITH_KNOTS ( 'NONE', 5,
 ( #107710, #31544, #57875, #33195, #65721, #58419 ),
 .UNSPECIFIED., .F., .F.,
 ( 6, 6 ),
 ( 0.000000000000000000, 1.000000000000000000 ),
 .UNSPECIFIED. ) ;
#79527=CARTESIAN_POINT ( 'NONE',  ( 41.32873071537510157, 1444.134764045589918, 136.5772078548479840 ) ) ;
#79528=ORIENTED_EDGE ( 'NONE', *, *, #59039, .T. ) ;
#79529=CARTESIAN_POINT ( 'NONE',  ( 6.526375164530000106, 1408.296884814930081, 262.4989465380980391 ) ) ;
#79530=CARTESIAN_POINT ( 'NONE',  ( -26.53391208829999925, 1488.685287628730066, 204.7973103800780166 ) ) ;
#79531=CARTESIAN_POINT ( 'NONE',  ( -10.42417239279969898, 1425.389265345479998, 97.52672419341850230 ) ) ;
#79532=CARTESIAN_POINT ( 'NONE',  ( -0.8911603994707960608, 1507.483750189549937, 231.9683985349379896 ) ) ;
#79535=CARTESIAN_POINT ( 'NONE',  ( -35.93744546429999787, 1433.966419625349999, 254.6052901707979572 ) ) ;
#79537=CARTESIAN_POINT ( 'NONE',  ( 29.47598808511030199, 1509.906165459849944, 209.6382085403890017 ) ) ;
#79539=CARTESIAN_POINT ( 'NONE',  ( 31.78277078219999296, 1450.942628683829980, 136.2347627311980034 ) ) ;
#79540=VERTEX_POINT ( 'NONE', #10452 ) ;
#79541=CARTESIAN_POINT ( 'NONE',  ( -2.500000000000000000, 1432.254430813080035, 157.4928808715980040 ) ) ;
#79548=CARTESIAN_POINT ( 'NONE',  ( -22.71348251198360302, 1409.706229765729859, 208.9920888512519923 ) ) ;
#79557=CARTESIAN_POINT ( 'NONE',  ( -15.00193899359999961, 1489.054902418029997, 230.6310622563979962 ) ) ;
#79559=ORIENTED_EDGE ( 'NONE', *, *, #98768, .T. ) ;
#79560=CARTESIAN_POINT ( 'NONE',  ( 11.73702549210000079, 1426.695992139529835, 144.1699184469979969 ) ) ;
#79561=DIRECTION ( 'NONE',  ( -0.9417419115949053898, 0.3363363969979660806, 0.000000000000000000 ) ) ;
#79565=VERTEX_POINT ( 'NONE', #66813 ) ;
#79566=CARTESIAN_POINT ( 'NONE',  ( 11.86374746855640083, 1432.171576367579974, 149.9798746170999948 ) ) ;
#79568=CARTESIAN_POINT ( 'NONE',  ( 13.37674189238196831, 1444.464913678520134, 187.6830941488352948 ) ) ;
#79571=CARTESIAN_POINT ( 'NONE',  ( -15.76866869242515889, 1506.436298853504013, 193.8022778273726203 ) ) ;
#79573=CARTESIAN_POINT ( 'NONE',  ( 8.908297959360000462, 1507.934933949130027, 234.8994657747980170 ) ) ;
#79575=CARTESIAN_POINT ( 'NONE',  ( 21.12668385848170161, 1452.175300330200116, 141.8024459500680052 ) ) ;
#79576=CARTESIAN_POINT ( 'NONE',  ( 3.148011791780000124, 1408.641849370629870, 270.4279803160980009 ) ) ;
#79583=CARTESIAN_POINT ( 'NONE',  ( 14.36570857389999922, 1435.002040243630063, 195.7737178941980005 ) ) ;
#79585=CARTESIAN_POINT ( 'NONE',  ( 17.94842024908709632, 1421.978012596150165, 225.1306823722440242 ) ) ;
#79588=CARTESIAN_POINT ( 'NONE',  ( 18.93537658700000037, 1413.766156166430164, 268.3665355202980436 ) ) ;
#79589=PLANE ( 'NONE',  #40842 ) ;
#79592=AXIS2_PLACEMENT_3D ( 'NONE', #34221, #43190, #76780 ) ;
#79599=CARTESIAN_POINT ( 'NONE',  ( -24.29684349240000074, 1443.814603648100046, 211.2876295167179705 ) ) ;
#79602=CARTESIAN_POINT ( 'NONE',  ( 18.42577555256999844, 1424.509265906519886, 223.4215472205989954 ) ) ;
#79603=CARTESIAN_POINT ( 'NONE',  ( 0.1955981720603170160, 1416.913060341699975, 225.1861339145730199 ) ) ;
#79605=CARTESIAN_POINT ( 'NONE',  ( 21.81700915577159705, 1509.753451845790096, 229.9156308900480212 ) ) ;
#79606=CARTESIAN_POINT ( 'NONE',  ( 13.28372496219609822, 1428.987819674619914, 222.1683325723000166 ) ) ;
#79607=CARTESIAN_POINT ( 'NONE',  ( 11.97075771579980596, 1433.593156705993579, 149.8706697297947699 ) ) ;
#79608=CARTESIAN_POINT ( 'NONE',  ( 16.42992099730000177, 1412.750267290230113, 226.7405470936979839 ) ) ;
#79611=CARTESIAN_POINT ( 'NONE',  ( -15.80102657300000146, 1459.267675803429938, 229.9937850598980162 ) ) ;
#79613=CARTESIAN_POINT ( 'NONE',  ( 45.85460769310000018, 1438.922387676499966, 268.7562792744979561 ) ) ;
#79614=CARTESIAN_POINT ( 'NONE',  ( -18.14294508140000062, 1410.043204499329931, 224.1267514446980158 ) ) ;
#79615=CARTESIAN_POINT ( 'NONE',  ( 22.42231863760000010, 1436.510268101429801, 142.5443955390980193 ) ) ;
#79617=CARTESIAN_POINT ( 'NONE',  ( 22.18897252830000255, 1508.010880766430091, 192.3772255266979982 ) ) ;
#79619=CARTESIAN_POINT ( 'NONE',  ( 23.78270988279999898, 1434.944176083839920, 215.5045224494480181 ) ) ;
#79621=CARTESIAN_POINT ( 'NONE',  ( 12.78776258870000149, 1416.851343894929869, 222.7045348337980215 ) ) ;
#79623=CARTESIAN_POINT ( 'NONE',  ( -35.70148625528900510, 1436.782343446300047, 136.4713999753330143 ) ) ;
#79624=CARTESIAN_POINT ( 'NONE',  ( -19.47833338605401821, 1506.473666148849816, 198.8548778393590624 ) ) ;
#79626=CARTESIAN_POINT ( 'NONE',  ( -13.34543549089999992, 1442.214279694210063, 188.2228390031980041 ) ) ;
#79627=CARTESIAN_POINT ( 'NONE',  ( -27.85054259011099731, 1508.556494693910054, 210.5418393889420088 ) ) ;
#79628=CARTESIAN_POINT ( 'NONE',  ( -31.78594533009999878, 1436.083197293939975, 136.3653833256979908 ) ) ;
#79629=CARTESIAN_POINT ( 'NONE',  ( -13.62133678120479985, 1452.879579795280051, 223.2680741433150047 ) ) ;
#79632=CARTESIAN_POINT ( 'NONE',  ( -10.82804715662830120, 1409.291184126150029, 219.4290004596960273 ) ) ;
#79636=CARTESIAN_POINT ( 'NONE',  ( -5.098844004812243647, 1422.101748936080412, 138.2836814087048651 ) ) ;
#79637=CARTESIAN_POINT ( 'NONE',  ( -42.40186856140000771, 1456.064825133729755, 268.3356964774980042 ) ) ;
#79639=CARTESIAN_POINT ( 'NONE',  ( 5.370527602886283169, 1422.356908813907012, 139.1416118586824666 ) ) ;
#79640=EDGE_CURVE ( 'NONE', #4089, #75020, #11564, .T. ) ;
#79641=CARTESIAN_POINT ( 'NONE',  ( -4.438186827019999854E-16, 1395.913060387330006, 217.1218459616979999 ) ) ;
#79644=CARTESIAN_POINT ( 'NONE',  ( 18.16724748010459933, 1425.011512764430108, 226.2496254856820030 ) ) ;
#79645=CARTESIAN_POINT ( 'NONE',  ( 22.52353380589999787, 1509.699599519530011, 227.8169178641979897 ) ) ;
#79646=CARTESIAN_POINT ( 'NONE',  ( 15.56469051819999905, 1506.798305132929954, 225.0756798403980099 ) ) ;
#79647=CARTESIAN_POINT ( 'NONE',  ( -26.52533711670449890, 1495.354429453090006, 211.2459270037799968 ) ) ;
#79649=DIRECTION ( 'NONE',  ( 0.2495203186574841137, -0.1962602071994360708, -0.9482729257165904979 ) ) ;
#79652=CARTESIAN_POINT ( 'NONE',  ( 27.43355929049999986, 1507.980920699130138, 207.4175378521480013 ) ) ;
#79653=CARTESIAN_POINT ( 'NONE',  ( -11.80119706069999985, 1415.163755984130148, 195.8322853899979918 ) ) ;
#79655=CARTESIAN_POINT ( 'NONE',  ( 23.24640105429999792, 1409.889347847929912, 210.7611772360680220 ) ) ;
#79657=DIRECTION ( 'NONE',  ( -1.000000000000000000, 0.000000000000000000, 0.000000000000000000 ) ) ;
#79659=CARTESIAN_POINT ( 'NONE',  ( -15.03158816200000025, 1422.458662492329950, 229.1221043826980122 ) ) ;
#79660=CARTESIAN_POINT ( 'NONE',  ( -11.57592119009999898, 1432.301067315389901, 151.1967988364980044 ) ) ;
#79665=CARTESIAN_POINT ( 'NONE',  ( -23.20186844609999710, 1425.882783674430129, 212.0388266151180119 ) ) ;
#79666=CARTESIAN_POINT ( 'NONE',  ( -1.328211266513899869, 1420.347263902439863, 184.8989585457709950 ) ) ;
#79669=CARTESIAN_POINT ( 'NONE',  ( -18.11634809011280112, 1485.171219500319921, 188.9687042995529964 ) ) ;
#79675=CARTESIAN_POINT ( 'NONE',  ( 27.14773470689999968, 1508.594019929430033, 214.4840992054080004 ) ) ;
#79679=CARTESIAN_POINT ( 'NONE',  ( 1.414439329599999962, 1414.913528139129994, 192.0350025121979911 ) ) ;
#79680=CARTESIAN_POINT ( 'NONE',  ( -2.913665321129999787E-15, 1426.935925255829943, 133.6118001900980232 ) ) ;
#79681=CARTESIAN_POINT ( 'NONE',  ( 0.5892548269570000441, 1508.868282030629871, 179.9181551937980146 ) ) ;
#79682=CARTESIAN_POINT ( 'NONE',  ( 11.94046459599999999, 1438.194204504490017, 147.6340003373980210 ) ) ;
#79683=CARTESIAN_POINT ( 'NONE',  ( -25.17222414333650349, 1451.970523125299906, 135.9900793875290219 ) ) ;
#79685=CARTESIAN_POINT ( 'NONE',  ( 5.558638042260000134, 1409.107172305129779, 229.7071683781979914 ) ) ;
#79687=CARTESIAN_POINT ( 'NONE',  ( 39.48425676673629425, 1438.208629468120080, 134.0999999978120059 ) ) ;
#79690=CARTESIAN_POINT ( 'NONE',  ( -0.5642542037087260320, 1421.257282776259899, 227.9630948969180224 ) ) ;
#79691=ORIENTED_EDGE ( 'NONE', *, *, #31923, .T. ) ;
#79694=EDGE_LOOP ( 'NONE', ( #84833, #81712, #1890, #94426 ) ) ;
#79697=CARTESIAN_POINT ( 'NONE',  ( 12.53380499174499896, 1445.052233488290085, 169.4755105688890069 ) ) ;
#79698=CARTESIAN_POINT ( 'NONE',  ( -0.3690468201050000063, 1465.421769112429956, 236.2943548505980118 ) ) ;
#79699=EDGE_CURVE ( 'NONE', #50703, #94116, #97924, .T. ) ;
#79700=CARTESIAN_POINT ( 'NONE',  ( 21.44083111125928909, 1450.933478988742081, 143.9289517833655623 ) ) ;
#79702=CARTESIAN_POINT ( 'NONE',  ( -2.253566441613126910E-10, 1426.918876941764893, 137.0999999980980135 ) ) ;
#79705=CARTESIAN_POINT ( 'NONE',  ( 4.229824676192839306, 1446.290629315919887, 165.0048999265850114 ) ) ;
#79707=ORIENTED_EDGE ( 'NONE', *, *, #9305, .F. ) ;
#79709=ORIENTED_EDGE ( 'NONE', *, *, #70277, .T. ) ;
#79710=CARTESIAN_POINT ( 'NONE',  ( 29.78885521565789674, 1440.913060387330006, 251.6509508777969870 ) ) ;
#79711=ADVANCED_FACE ( 'NONE', ( #64612 ), #51869, .F. ) ;
#79715=CARTESIAN_POINT ( 'NONE',  ( -13.63985639130000038, 1409.389374668229948, 191.6355463836979709 ) ) ;
#79717=CARTESIAN_POINT ( 'NONE',  ( -24.30106948394094957, 1439.034099877470453, 212.0667701832317675 ) ) ;
#79721=CARTESIAN_POINT ( 'NONE',  ( 27.22939932153649778, 1441.374094540659826, 137.3495838342670083 ) ) ;
#79724=CARTESIAN_POINT ( 'NONE',  ( 2.858162928570000094, 1466.265918564530011, 234.1316300927979910 ) ) ;
#79729=CARTESIAN_POINT ( 'NONE',  ( 29.22958591730000322, 1509.933780019529877, 206.4713312915380072 ) ) ;
#79731=DIRECTION ( 'NONE',  ( -0.001027118858030306352, 0.9999913661844073154, -0.004026485253177600199 ) ) ;
#79736=CARTESIAN_POINT ( 'NONE',  ( 28.66942461040000012, 1455.243640875029996, 248.2467662549979934 ) ) ;
#79739=CARTESIAN_POINT ( 'NONE',  ( -26.49480178416090226, 1509.838279253159953, 221.7449016213969912 ) ) ;
#79740=CARTESIAN_POINT ( 'NONE',  ( 1.799212021300000020, 1414.514225440530026, 232.3796572949979975 ) ) ;
#79741=ADVANCED_FACE ( 'NONE', ( #31932 ), #84888, .T. ) ;
#79742=CARTESIAN_POINT ( 'NONE',  ( -20.46956895259999953, 1454.794904290429940, 224.5075067967979976 ) ) ;
#79743=EDGE_CURVE ( 'NONE', #39621, #25855, #103053, .T. ) ;
#79744=CARTESIAN_POINT ( 'NONE',  ( -20.67788066618572529, 1410.996043025710378, 199.4490997680371152 ) ) ;
#79745=CARTESIAN_POINT ( 'NONE',  ( 2.500000000000000000, 1432.253675377960008, 157.4927705404979861 ) ) ;
#79750=CARTESIAN_POINT ( 'NONE',  ( 3.426893344479999826, 1406.086097517129929, 266.9564242903979903 ) ) ;
#79754=CARTESIAN_POINT ( 'NONE',  ( 42.85031254769640441, 1445.998884488219801, 270.2009481598719844 ) ) ;
#79756=CARTESIAN_POINT ( 'NONE',  ( 10.81433178877583501, 1424.654531174282056, 138.0162591780839136 ) ) ;
#79757=CARTESIAN_POINT ( 'NONE',  ( -36.52292854368610620, 1440.913060387330006, 253.7928692754429676 ) ) ;
#79759=CARTESIAN_POINT ( 'NONE',  ( 2.356271506361870216, 1449.642660013894783, 154.4296805934006898 ) ) ;
#79761=CARTESIAN_POINT ( 'NONE',  ( 1.174890886735320050, 1450.814461567769968, 154.7898993816909865 ) ) ;
#79763=CARTESIAN_POINT ( 'NONE',  ( -1.546869376352204339, 1416.835807507126901, 228.0212684238467489 ) ) ;
#79765=ORIENTED_EDGE ( 'NONE', *, *, #17252, .F. ) ;
#79766=CARTESIAN_POINT ( 'NONE',  ( -7.553102830249999400, 1423.481562104430168, 234.3916895697979612 ) ) ;
#79769=CARTESIAN_POINT ( 'NONE',  ( -1.312418798399999753, 1475.035471520030114, 269.6495476954979722 ) ) ;
#79771=CARTESIAN_POINT ( 'NONE',  ( -27.92763793890000201, 1508.597377666530065, 210.3373496168879910 ) ) ;
#79773=CARTESIAN_POINT ( 'NONE',  ( -2.499999999999999556, 1448.225424448829699, 183.4745085405895679 ) ) ;
#79777=CARTESIAN_POINT ( 'NONE',  ( 26.64494604805370059, 1435.509179537890077, 135.8250902819609962 ) ) ;
#79778=CARTESIAN_POINT ( 'NONE',  ( -3.852081035159350186, 1396.047578021569961, 219.4511520228920176 ) ) ;
#79779=ADVANCED_FACE ( 'NONE', ( #75617 ), #34866, .F. ) ;
#79780=B_SPLINE_CURVE_WITH_KNOTS ( 'NONE', 5,
 ( #47517, #30138, #12797, #11702, #46432, #55924 ),
 .UNSPECIFIED., .F., .F.,
 ( 6, 6 ),
 ( 0.000000000000000000, 1.000000000000000000 ),
 .UNSPECIFIED. ) ;
#79781=CARTESIAN_POINT ( 'NONE',  ( -15.97381121195400056, 1420.723668288270119, 227.0315409032249931 ) ) ;
#79782=CARTESIAN_POINT ( 'NONE',  ( -16.78937331912329967, 1410.728390654980103, 226.4051236745929998 ) ) ;
#79783=FACE_OUTER_BOUND ( 'NONE', #17674, .T. ) ;
#79787=CARTESIAN_POINT ( 'NONE',  ( -11.84030381978469926, 1430.235986086469893, 151.0624496547240199 ) ) ;
#79788=CARTESIAN_POINT ( 'NONE',  ( 11.23805577879999973, 1426.459959828230012, 108.0450254846979874 ) ) ;
#79790=CARTESIAN_POINT ( 'NONE',  ( 11.68426330212614239, 1428.980873612041023, 140.1562216286907869 ) ) ;
#79791=CARTESIAN_POINT ( 'NONE',  ( -11.23388613411650638, 1445.063428794548372, 151.7784653951601399 ) ) ;
#79794=CARTESIAN_POINT ( 'NONE',  ( -9.660544699540000835, 1432.353341358199941, 148.7316627034979888 ) ) ;
#79795=CARTESIAN_POINT ( 'NONE',  ( 5.709868603420000355, 1508.901606182030037, 181.0882369999980028 ) ) ;
#79796=DIRECTION ( 'NONE',  ( 0.3363363969981477131, 0.6659120918162938496, -0.6659120918162938496 ) ) ;
#79803=CARTESIAN_POINT ( 'NONE',  ( -14.52606424000000018, 1443.052989431600054, 188.9151166515979980 ) ) ;
#79804=CARTESIAN_POINT ( 'NONE',  ( -5.555854370870000558, 1409.107075097130291, 188.5359587977980027 ) ) ;
#79808=LINE ( 'NONE', #70325, #68337 ) ;
#79811=CARTESIAN_POINT ( 'NONE',  ( -41.57727771173860276, 1445.035119975709904, 135.5177309179229894 ) ) ;
#79813=CARTESIAN_POINT ( 'NONE',  ( -2.500000000000000000, 1448.283978340080012, 164.7255006787519847 ) ) ;
#79814=CARTESIAN_POINT ( 'NONE',  ( 9.773096794904308382, 1396.254344449989958, 214.3031617136149976 ) ) ;
#79815=CARTESIAN_POINT ( 'NONE',  ( -39.26371633287709528, 1437.713075516209983, 136.4559412716930353 ) ) ;
#79816=CARTESIAN_POINT ( 'NONE',  ( -2.304693369170319972, 1405.812077718989940, 268.4818566354389873 ) ) ;
#79817=CARTESIAN_POINT ( 'NONE',  ( 0.000000000000000000, 1413.913060387330006, 209.1218459616979999 ) ) ;
#79819=CARTESIAN_POINT ( 'NONE',  ( 4.029435563379999863, 1425.967794969329816, 185.3373052141980111 ) ) ;
#79822=EDGE_LOOP ( 'NONE', ( #34364, #107415, #32829, #13555 ) ) ;
#79834=CARTESIAN_POINT ( 'NONE',  ( -41.56672249360055815, 1436.264666313427597, 269.6392715097015298 ) ) ;
#79836=CARTESIAN_POINT ( 'NONE',  ( -4.049849602479999255, 1409.054484251730173, 230.6815826274979884 ) ) ;
#79837=CARTESIAN_POINT ( 'NONE',  ( -1.549455982270276921, 1452.110832695822410, 183.9727752664628042 ) ) ;
#79838=ORIENTED_EDGE ( 'NONE', *, *, #81705, .F. ) ;
#79840=CARTESIAN_POINT ( 'NONE',  ( -26.20202373978780130, 1440.913060467019932, 222.9344598648480087 ) ) ;
#79843=CARTESIAN_POINT ( 'NONE',  ( 36.48439800688450418, 1420.562376931399967, 269.8440692582560700 ) ) ;
#79848=CARTESIAN_POINT ( 'NONE',  ( -0.3788383082595139784, 1408.926289712549988, 186.6322538385570056 ) ) ;
#79850=ORIENTED_EDGE ( 'NONE', *, *, #91819, .F. ) ;
#79851=CARTESIAN_POINT ( 'NONE',  ( 2.500000000000000000, 1438.733025222760034, 157.7103763496980093 ) ) ;
#79852=CARTESIAN_POINT ( 'NONE',  ( -0.9510881122189999148, 1420.454310056129998, 233.4992290069980072 ) ) ;
#79853=CARTESIAN_POINT ( 'NONE',  ( 5.347888905970906492, 1422.377615597161594, 137.0999999981554254 ) ) ;
#79857=EDGE_CURVE ( 'NONE', #91877, #84761, #101657, .T. ) ;
#79858=CARTESIAN_POINT ( 'NONE',  ( 15.79979472558019893, 1478.706781717480226, 230.3901329066689811 ) ) ;
#79859=CARTESIAN_POINT ( 'NONE',  ( 19.97269026569999895, 1507.847566758330004, 189.1149477268980093 ) ) ;
#79861=CARTESIAN_POINT ( 'NONE',  ( -0.009250756501870001022, 1410.298659367929758, 233.2341916293980262 ) ) ;
#79862=CARTESIAN_POINT ( 'NONE',  ( -0.02494278528423909957, 1420.444533703900106, 182.6761653814459976 ) ) ;
#79865=CARTESIAN_POINT ( 'NONE',  ( 18.68654020960000040, 1509.565608750529918, 186.8439702849979938 ) ) ;
#79867=ORIENTED_EDGE ( 'NONE', *, *, #106736, .T. ) ;
#79869=CARTESIAN_POINT ( 'NONE',  ( -16.78942537780000066, 1508.913060324029857, 185.4904754144979790 ) ) ;
#79871=DIRECTION ( 'NONE',  ( 0.2342910577437130604, -0.2476038162833715528, 0.9401064037773823046 ) ) ;
#79873=CARTESIAN_POINT ( 'NONE',  ( 4.500000000000000000, 1425.929641636930000, 172.2701767017979932 ) ) ;
#79876=CARTESIAN_POINT ( 'NONE',  ( -27.18296536300610100, 1509.563679778480036, 201.2124616717040055 ) ) ;
#79879=CARTESIAN_POINT ( 'NONE',  ( -18.27807275150000166, 1423.991801469829852, 225.3729312157979905 ) ) ;
#79880=CARTESIAN_POINT ( 'NONE',  ( -22.74371025250000145, 1435.291990449120249, 140.0265565429980086 ) ) ;
#79881=EDGE_CURVE ( 'NONE', #63032, #34701, #80490, .T. ) ;
#79882=CARTESIAN_POINT ( 'NONE',  ( -0.5883740847710429156, 1477.659013864529925, 230.4497675389389997 ) ) ;
#79884=CARTESIAN_POINT ( 'NONE',  ( 0.8805854391707040874, 1409.878736129950084, 233.0125103023929967 ) ) ;
#79885=CARTESIAN_POINT ( 'NONE',  ( -15.83997831783995736, 1431.256282991279932, 220.2014388792205182 ) ) ;
#79887=ORIENTED_EDGE ( 'NONE', *, *, #32172, .T. ) ;
#79888=CARTESIAN_POINT ( 'NONE',  ( 1.550352066763079906, 1415.948038442049892, 190.4790932164650030 ) ) ;
#79890=CARTESIAN_POINT ( 'NONE',  ( -11.90008666459999986, 1434.920851464509951, 147.6452002888979962 ) ) ;
#79892=CARTESIAN_POINT ( 'NONE',  ( 0.000000000000000000, 1519.913060387329779, 209.1218459616979999 ) ) ;
#79894=CARTESIAN_POINT ( 'NONE',  ( -10.98084453577630093, 1433.016921785290151, 151.7694248368179899 ) ) ;
#79895=CARTESIAN_POINT ( 'NONE',  ( -24.84524933634759947, 1439.550688600570084, 210.4208596888960017 ) ) ;
#79904=DIRECTION ( 'NONE',  ( 0.7074300732568278294, -0.02470400251969398844, 0.7063514732138287400 ) ) ;
#79912=CARTESIAN_POINT ( 'NONE',  ( 12.95705078732472515, 1442.923589581116175, 169.4279645666727561 ) ) ;
#79913=CARTESIAN_POINT ( 'NONE',  ( 29.71190172082722114, 1419.366236750363669, 269.4677692610073905 ) ) ;
#79914=CARTESIAN_POINT ( 'NONE',  ( -31.44036148889999538, 1456.450349409130013, 254.7811646097979974 ) ) ;
#79916=CARTESIAN_POINT ( 'NONE',  ( -11.32027785699999889, 1433.946929803360035, 151.5080542412979980 ) ) ;
#79918=CARTESIAN_POINT ( 'NONE',  ( -19.67553321019999757, 1485.964808132929875, 190.1451763510979731 ) ) ;
#79919=CARTESIAN_POINT ( 'NONE',  ( 9.907168344889999645, 1409.425378975729927, 189.1781829689979872 ) ) ;
#79920=CARTESIAN_POINT ( 'NONE',  ( 4.936249769079999794, 1423.379993255829959, 184.2513112279979737 ) ) ;
#79922=CARTESIAN_POINT ( 'NONE',  ( 5.445836176130000261, 1441.097906882780080, 154.8052917028979607 ) ) ;
#79924=CARTESIAN_POINT ( 'NONE',  ( -6.040726587390000013, 1452.702113566630032, 152.1320015699980104 ) ) ;
#79926=ORIENTED_EDGE ( 'NONE', *, *, #99685, .F. ) ;
#79929=CARTESIAN_POINT ( 'NONE',  ( -10.86918694159999887, 1472.641908963629930, 270.3751304083979790 ) ) ;
#79931=CARTESIAN_POINT ( 'NONE',  ( 3.255911231930000316, 1435.946191916090129, 155.5160642224979881 ) ) ;
#79932=CARTESIAN_POINT ( 'NONE',  ( -14.51158588560000062, 1474.168193539429922, 223.7580015587980142 ) ) ;
#79933=CARTESIAN_POINT ( 'NONE',  ( 10.60236678890000128, 1431.113060387329824, 193.5879272064979943 ) ) ;
#79934=CARTESIAN_POINT ( 'NONE',  ( -12.52061335139999976, 1420.940692459130105, 230.1659492372980083 ) ) ;
#79938=CARTESIAN_POINT ( 'NONE',  ( -44.91570373049209763, 1434.529260160309832, 266.2100032643309646 ) ) ;
#79941=EDGE_LOOP ( 'NONE', ( #57928, #20001, #59820, #39673, #65133 ) ) ;
#79943=CARTESIAN_POINT ( 'NONE',  ( 2.895377824650565923, 1447.016636168100604, 182.3842140122979743 ) ) ;
#79944=CARTESIAN_POINT ( 'NONE',  ( 13.03169765326649987, 1424.752599651019864, 222.9539081381209940 ) ) ;
#79945=DIRECTION ( 'NONE',  ( 0.8304244102910536274, -0.2476038100681244025, 0.4990868181313787844 ) ) ;
#79953=EDGE_LOOP ( 'NONE', ( #26311, #23824, #30864, #62373 ) ) ;
#79954=CARTESIAN_POINT ( 'NONE',  ( -26.32366284865300088, 1415.625410839150163, 270.3533368716700238 ) ) ;
#79956=CARTESIAN_POINT ( 'NONE',  ( -2.205156445730000137, 1428.435894572430016, 91.31218443469779800 ) ) ;
#79960=ORIENTED_EDGE ( 'NONE', *, *, #20315, .F. ) ;
#79961=CARTESIAN_POINT ( 'NONE',  ( 45.62277040061831457, 1441.770530636094918, 268.9751422883944656 ) ) ;
#79964=CARTESIAN_POINT ( 'NONE',  ( -0.01749107806689290112, 1408.977739893769922, 186.0382551112710132 ) ) ;
#79967=CARTESIAN_POINT ( 'NONE',  ( 5.386185205460879644, 1432.347042709529887, 154.6076275981190236 ) ) ;
#79968=CARTESIAN_POINT ( 'NONE',  ( -13.68772360880000072, 1420.178243169430061, 222.0123197414980041 ) ) ;
#79969=CARTESIAN_POINT ( 'NONE',  ( -1.653188813474884666, 1467.000319734719596, 235.3477346490027742 ) ) ;
#79970=CARTESIAN_POINT ( 'NONE',  ( 10.69046686070000085, 1445.373974055579993, 185.6902835676980033 ) ) ;
#79974=CARTESIAN_POINT ( 'NONE',  ( 1.474754854666479931, 1482.224443677059980, 182.1987295621239866 ) ) ;
#79975=ORIENTED_EDGE ( 'NONE', *, *, #96028, .T. ) ;
#79976=CARTESIAN_POINT ( 'NONE',  ( 3.915817772150960607, 1457.457976147669569, 228.5041087852198132 ) ) ;
#79977=CARTESIAN_POINT ( 'NONE',  ( 24.33536485855309905, 1452.047573491060120, 136.5413356103030083 ) ) ;
#79978=CARTESIAN_POINT ( 'NONE',  ( -13.84855700446339988, 1443.315687757889918, 195.7951355894199992 ) ) ;
#79981=CARTESIAN_POINT ( 'NONE',  ( 19.41452480519999924, 1410.952374995430091, 196.0910004049979989 ) ) ;
#79982=CARTESIAN_POINT ( 'NONE',  ( 12.93811130839999812, 1444.994950788469851, 169.4238961894979809 ) ) ;
#79983=CARTESIAN_POINT ( 'NONE',  ( 16.16109259539999954, 1409.477418176630181, 225.0245223578980074 ) ) ;
#79985=CARTESIAN_POINT ( 'NONE',  ( 4.500000000000000000, 1448.210448412289907, 182.3842140122979743 ) ) ;
#79986=AXIS2_PLACEMENT_3D ( 'NONE', #47771, #21432, #56726 ) ;
#79987=CARTESIAN_POINT ( 'NONE',  ( 2.500000000000000000, 1439.114301455650093, 157.7261946041980138 ) ) ;
#79990=ORIENTED_EDGE ( 'NONE', *, *, #93991, .F. ) ;
#79992=DIRECTION ( 'NONE',  ( 0.2562858833364869415, 0.008949701426205170993, -0.9665595940483019399 ) ) ;
#79996=CARTESIAN_POINT ( 'NONE',  ( -38.15885483313930138, 1448.679264857810040, 136.3994482979960026 ) ) ;
#79997=DIRECTION ( 'NONE',  ( 0.002120872317174225027, 0.9999913661844083146, -0.003573437736249155880 ) ) ;
#79998=CARTESIAN_POINT ( 'NONE',  ( -22.74199305119999792, 1446.314437877210139, 234.3916895697979612 ) ) ;
#80000=CARTESIAN_POINT ( 'NONE',  ( 11.59597807620000154, 1433.182955382529826, 151.0968555446979735 ) ) ;
#80001=ADVANCED_FACE ( 'NONE', ( #10972 ), #55200, .T. ) ;
#80002=CARTESIAN_POINT ( 'NONE',  ( -2.086158904326180341, 1474.140508472220063, 270.1368012846049851 ) ) ;
#80003=CARTESIAN_POINT ( 'NONE',  ( 24.69096861020820199, 1440.913060394919967, 214.0095001576269738 ) ) ;
#80006=EDGE_LOOP ( 'NONE', ( #108150, #2978, #61300, #106331 ) ) ;
#80008=CARTESIAN_POINT ( 'NONE',  ( 18.89959486413309975, 1416.839692127159879, 210.6687135792209915 ) ) ;
#80009=CIRCLE ( 'NONE', #8454, 65.59183216034817576 ) ;
#80010=CARTESIAN_POINT ( 'NONE',  ( -19.31939586139944254, 1485.616822396989619, 189.8190535202998603 ) ) ;
#80011=CARTESIAN_POINT ( 'NONE',  ( 8.104840167896952607, 1398.153761633497197, 198.9574189372607123 ) ) ;
#80012=CARTESIAN_POINT ( 'NONE',  ( 2.637616553089999982, 1474.725858340030072, 234.5358300088979888 ) ) ;
#80013=B_SPLINE_CURVE_WITH_KNOTS ( 'NONE', 3,
 ( #25619, #96156, #61476, #27852, #78247, #68228, #103430 ),
 .UNSPECIFIED., .F., .F.,
 ( 4, 3, 4 ),
 ( -108.0170515669999958, -74.06595527500620335, -37.80268138969999825 ),
 .UNSPECIFIED. ) ;
#80014=CARTESIAN_POINT ( 'NONE',  ( 24.93139309710000262, 1449.798359900550167, 212.9211815600280033 ) ) ;
#80017=CARTESIAN_POINT ( 'NONE',  ( -14.38163500639999981, 1509.358420488030106, 233.7087952759979999 ) ) ;
#80020=CARTESIAN_POINT ( 'NONE',  ( 6.294750265859999416, 1408.079328832830015, 220.7028845648979711 ) ) ;
#80022=DIRECTION ( 'NONE',  ( 0.4794254784390402646, 5.727640580602533849E-10, 0.8775825947587483356 ) ) ;
#80023=CARTESIAN_POINT ( 'NONE',  ( -41.65810620650000828, 1443.954352776429914, 135.6863023723980177 ) ) ;
#80024=ORIENTED_EDGE ( 'NONE', *, *, #54205, .F. ) ;
#80025=CARTESIAN_POINT ( 'NONE',  ( -1.297832609859999931, 1452.391379596130037, 183.7169094889979988 ) ) ;
#80031=ORIENTED_EDGE ( 'NONE', *, *, #62287, .T. ) ;
#80034=CARTESIAN_POINT ( 'NONE',  ( 28.34436068694596500, 1509.902867273254287, 202.2339729425384007 ) ) ;
#80036=CARTESIAN_POINT ( 'NONE',  ( 20.40004974522683767, 1509.667807812142883, 187.4863181757289681 ) ) ;
#80038=CARTESIAN_POINT ( 'NONE',  ( 13.82144533499180028, 1409.395715893920169, 203.4549396693699919 ) ) ;
#80043=CARTESIAN_POINT ( 'NONE',  ( 13.51610093809999924, 1443.913060387330006, 169.3501091259980171 ) ) ;
#80045=ORIENTED_EDGE ( 'NONE', *, *, #107537, .T. ) ;
#80046=CARTESIAN_POINT ( 'NONE',  ( -11.57234447566209923, 1415.219159636060112, 195.3490233354060308 ) ) ;
#80048=CARTESIAN_POINT ( 'NONE',  ( 16.20698216735619468, 1469.058401758687296, 269.3699621073229196 ) ) ;
#80049=FACE_OUTER_BOUND ( 'NONE', #26768, .T. ) ;
#80050=CARTESIAN_POINT ( 'NONE',  ( -27.78452750130110260, 1508.000976266860107, 210.4681927182890036 ) ) ;
#80052=CARTESIAN_POINT ( 'NONE',  ( -0.1575406214799999760, 1462.356505213130049, 182.8094439125979989 ) ) ;
#80054=CARTESIAN_POINT ( 'NONE',  ( -25.77751368618157102, 1436.654609691480573, 137.0719439152050256 ) ) ;
#80056=CIRCLE ( 'NONE', #83567, 40.01690241380000401 ) ;
#80060=CARTESIAN_POINT ( 'NONE',  ( 20.36637623643389716, 1500.297579758999973, 227.4379270215500242 ) ) ;
#80063=ORIENTED_EDGE ( 'NONE', *, *, #100660, .F. ) ;
#80065=CARTESIAN_POINT ( 'NONE',  ( -26.30775428199999766, 1469.245646017629952, 207.3898640084980229 ) ) ;
#80066=CARTESIAN_POINT ( 'NONE',  ( -11.01735835230000049, 1426.937595289829915, 91.95967800869790665 ) ) ;
#80067=CARTESIAN_POINT ( 'NONE',  ( 13.45946769660000086, 1415.628674266529742, 196.7502466371980177 ) ) ;
#80070=CARTESIAN_POINT ( 'NONE',  ( -36.81312563220000555, 1438.597774659029938, 254.5659314777980455 ) ) ;
#80072=EDGE_CURVE ( 'NONE', #60488, #41404, #22926, .T. ) ;
#80075=CARTESIAN_POINT ( 'NONE',  ( -22.91555022173351475, 1409.723203468988913, 208.8960394818137161 ) ) ;
#80076=EDGE_LOOP ( 'NONE', ( #32209, #38456, #61264, #76448 ) ) ;
#80077=FACE_OUTER_BOUND ( 'NONE', #75237, .T. ) ;
#80079=CARTESIAN_POINT ( 'NONE',  ( 5.857737085409999267, 1509.117617073830161, 238.0531267651979874 ) ) ;
#80080=VERTEX_POINT ( 'NONE', #37739 ) ;
#80082=AXIS2_PLACEMENT_3D ( 'NONE', #84006, #8392, #66686 ) ;
#80086=CARTESIAN_POINT ( 'NONE',  ( -1.074930184170000080, 1413.843955136130035, 185.1690177555979915 ) ) ;
#80088=CARTESIAN_POINT ( 'NONE',  ( -2.361437468280000118, 1479.773351731729917, 235.7524046215980036 ) ) ;
#80090=ORIENTED_EDGE ( 'NONE', *, *, #72671, .T. ) ;
#80092=FACE_OUTER_BOUND ( 'NONE', #45938, .T. ) ;
#80093=CARTESIAN_POINT ( 'NONE',  ( -12.77961858748070156, 1414.913057834409983, 220.2176620357280115 ) ) ;
#80094=CARTESIAN_POINT ( 'NONE',  ( 13.89869200000000049, 1452.835253893030085, 223.8385666725980059 ) ) ;
#80098=CARTESIAN_POINT ( 'NONE',  ( 11.85300018840249869, 1431.425274647949891, 149.9062840562949930 ) ) ;
#80099=CARTESIAN_POINT ( 'NONE',  ( 12.69590191108945376, 1445.017070807032269, 186.3645745659958095 ) ) ;
#80100=VERTEX_POINT ( 'NONE', #26564 ) ;
#80107=CARTESIAN_POINT ( 'NONE',  ( 23.43477590392700094, 1452.094699979900042, 137.9018702996609989 ) ) ;
#80108=CARTESIAN_POINT ( 'NONE',  ( 0.4870561706949109726, 1408.236684636520067, 270.3925729436620031 ) ) ;
#80111=CARTESIAN_POINT ( 'NONE',  ( -19.59037083185129546, 1509.615009600280473, 231.2999628551918363 ) ) ;
#80116=CARTESIAN_POINT ( 'NONE',  ( 17.64461694360119992, 1412.137575667770079, 224.8446746702369978 ) ) ;
#80118=VERTEX_POINT ( 'NONE', #47242 ) ;
#80119=CARTESIAN_POINT ( 'NONE',  ( 36.99165393039999827, 1427.133824787730191, 268.3665355202980436 ) ) ;
#80129=CARTESIAN_POINT ( 'NONE',  ( -24.89775517959999718, 1442.835547152150184, 210.5176497469579999 ) ) ;
#80130=CARTESIAN_POINT ( 'NONE',  ( -11.63669227459999966, 1425.864836378729933, 144.1684971660979784 ) ) ;
#80135=CARTESIAN_POINT ( 'NONE',  ( 13.11760263369310131, 1509.411057675469692, 181.1735613693849984 ) ) ;
#80137=CARTESIAN_POINT ( 'NONE',  ( -13.15726448721240160, 1416.851343896870048, 221.9096085506390068 ) ) ;
#80138=CARTESIAN_POINT ( 'NONE',  ( 13.51135493409999988, 1415.081657033430020, 228.4979249935979908 ) ) ;
#80141=CARTESIAN_POINT ( 'NONE',  ( -16.61355167848200054, 1459.966389597419948, 228.4924131504890283 ) ) ;
#80143=CARTESIAN_POINT ( 'NONE',  ( 46.27884742629999693, 1440.913084543189825, 267.5894369069980030 ) ) ;
#80144=CARTESIAN_POINT ( 'NONE',  ( -18.90483148029999683, 1410.069205653730023, 222.7218158439980016 ) ) ;
#80145=CARTESIAN_POINT ( 'NONE',  ( 19.01901943839999731, 1435.591100437959767, 145.9747268152980268 ) ) ;
#80146=CARTESIAN_POINT ( 'NONE',  ( 24.99925640249999859, 1488.577142715929995, 200.8921111725379944 ) ) ;
#80147=CARTESIAN_POINT ( 'NONE',  ( 29.76859869597256036, 1509.997910412159627, 208.7253019497961475 ) ) ;
#80149=CARTESIAN_POINT ( 'NONE',  ( -0.1075775631909999946, 1475.837061347730014, 266.9611530679979978 ) ) ;
#80151=CARTESIAN_POINT ( 'NONE',  ( -33.93525073091490185, 1436.160847652960001, 136.3001632569819890 ) ) ;
#80152=CARTESIAN_POINT ( 'NONE',  ( -13.59572565769999919, 1409.328701682329893, 203.3447866184380075 ) ) ;
#80154=CARTESIAN_POINT ( 'NONE',  ( -16.19493240869999795, 1409.478599888930148, 193.4350318414979881 ) ) ;
#80156=CARTESIAN_POINT ( 'NONE',  ( 11.87591311449999942, 1433.006404943239886, 146.5967610804979984 ) ) ;
#80157=CARTESIAN_POINT ( 'NONE',  ( -26.79413260980000189, 1435.433175380389912, 135.2874982680980054 ) ) ;
#80161=CARTESIAN_POINT ( 'NONE',  ( 27.93599228869999607, 1442.648988978960006, 137.4365311675980195 ) ) ;
#80166=CARTESIAN_POINT ( 'NONE',  ( -38.70127719692458612, 1443.913060387331370, 136.9798462687442679 ) ) ;
#80167=CARTESIAN_POINT ( 'NONE',  ( -26.91513671580000278, 1469.147785373630086, 269.0204381106979667 ) ) ;
#80170=FACE_OUTER_BOUND ( 'NONE', #81658, .T. ) ;
#80174=B_SPLINE_SURFACE_WITH_KNOTS ( 'NONE', 5, 5, ( 
 ( #105071, #37319, #71515, #43519, #103386, #10453 ),
 ( #60889, #78768, #9899, #974, #19385, #69281 ),
 ( #2083, #70397, #61438, #18283, #86605, #27813 ),
 ( #82056, #73696, #63647, #106171, #22681, #89911 ),
 ( #30562, #65290, #46298, #73125, #99403, #46841 ),
 ( #72580, #90459, #80969, #56326, #107822, #13736 ),
 ( #28920, #38404, #105634, #3740, #64752, #21034 ),
 ( #13184, #47920, #98311, #4274, #63111, #48490 ),
 ( #64189, #106708, #12662, #4800, #31110, #29998 ) ),
 .UNSPECIFIED., .F., .F., .F.,
 ( 6, 3, 6 ),
 ( 6, 6 ),
 ( 8.763103464980000368, 19.90566978349999872, 30.47641535120000000 ),
 ( -2.775557561569999727E-17, 2.000000000000000000 ),
 .UNSPECIFIED. ) ;
#80177=CARTESIAN_POINT ( 'NONE',  ( 22.52097504219999990, 1509.699510165530000, 227.8690926855979910 ) ) ;
#80179=CARTESIAN_POINT ( 'NONE',  ( -6.446325585610000353, 1432.345375419369930, 154.6647257196979979 ) ) ;
#80182=VERTEX_POINT ( 'NONE', #39385 ) ;
#80185=DIRECTION ( 'NONE',  ( -2.275957200478543654E-15, -0.7071067811865475727, -0.7071067811865475727 ) ) ;
#80188=CARTESIAN_POINT ( 'NONE',  ( -12.33246611440000073, 1415.579607672129896, 195.5076102655979753 ) ) ;
#80190=CARTESIAN_POINT ( 'NONE',  ( 22.60280089679999804, 1409.702367587229901, 211.4725249609479931 ) ) ;
#80193=CARTESIAN_POINT ( 'NONE',  ( -15.97230909389999987, 1420.722884146229717, 227.0315162960980047 ) ) ;
#80194=CARTESIAN_POINT ( 'NONE',  ( -11.87312849439999951, 1432.864063127479994, 149.9809861782979965 ) ) ;
#80196=CARTESIAN_POINT ( 'NONE',  ( 1.363639804150000190, 1415.765549334430034, 232.8698634931980109 ) ) ;
#80203=CARTESIAN_POINT ( 'NONE',  ( -20.58707213139999936, 1427.974737749530050, 223.4007331328979831 ) ) ;
#80205=CARTESIAN_POINT ( 'NONE',  ( -16.28303581252109922, 1485.105577738389911, 187.8116298709459784 ) ) ;
#80209=VERTEX_POINT ( 'NONE', #99269 ) ;
#80210=CARTESIAN_POINT ( 'NONE',  ( 29.42769729879999829, 1509.955660133030051, 212.2907639111579954 ) ) ;
#80215=CARTESIAN_POINT ( 'NONE',  ( 1.525139958810000085, 1427.692446166030095, 112.4493539157979995 ) ) ;
#80216=DIRECTION ( 'NONE',  ( -2.028721370088317945E-13, -0.03085824620774639884, 0.9995237709234243706 ) ) ;
#80219=CARTESIAN_POINT ( 'NONE',  ( -24.93976076479000170, 1451.594252318390090, 137.3267138200340014 ) ) ;
#80221=CARTESIAN_POINT ( 'NONE',  ( 10.56558922819999857, 1409.282018893330132, 228.0601045111980056 ) ) ;
#80225=CARTESIAN_POINT ( 'NONE',  ( 41.66188030070010484, 1443.907795131820194, 134.0999999982419979 ) ) ;
#80231=ORIENTED_EDGE ( 'NONE', *, *, #85761, .F. ) ;
#80235=CARTESIAN_POINT ( 'NONE',  ( 15.34791040292138220, 1451.140134807847289, 149.4943114245902223 ) ) ;
#80237=B_SPLINE_CURVE_WITH_KNOTS ( 'NONE', 5,
 ( #103271, #42288, #75893, #26011, #69166, #77556 ),
 .UNSPECIFIED., .F., .F.,
 ( 6, 6 ),
 ( 0.000000000000000000, 0.5082988451364722771 ),
 .UNSPECIFIED. ) ;
#80243=CARTESIAN_POINT ( 'NONE',  ( 0.9304290756690000164, 1507.643508851029765, 237.2595324437979798 ) ) ;
#80248=CARTESIAN_POINT ( 'NONE',  ( 29.36784481322840179, 1440.913060387330006, 250.7515280202720191 ) ) ;
#80249=CARTESIAN_POINT ( 'NONE',  ( -15.09049181950000040, 1508.196604722230177, 184.9938367632979919 ) ) ;
#80251=CARTESIAN_POINT ( 'NONE',  ( 27.43704247741250057, 1448.208574544649991, 136.8607721885420005 ) ) ;
#80252=CARTESIAN_POINT ( 'NONE',  ( -14.90953803460000060, 1409.433712928330124, 191.8387206668980127 ) ) ;
#80257=CARTESIAN_POINT ( 'NONE',  ( 22.50914366684990142, 1410.820172114669958, 206.2042648971080041 ) ) ;
#80258=CARTESIAN_POINT ( 'NONE',  ( 18.80339018749999980, 1425.953307693130000, 225.0197311690980086 ) ) ;
#80261=FACE_OUTER_BOUND ( 'NONE', #100613, .T. ) ;
#80262=CARTESIAN_POINT ( 'NONE',  ( -15.13342374508840038, 1507.606285602760181, 191.8462590464540085 ) ) ;
#80263=CARTESIAN_POINT ( 'NONE',  ( 15.72511249053680160, 1409.739245071985579, 192.0850589048065729 ) ) ;
#80267=AXIS2_PLACEMENT_3D ( 'NONE', #47008, #21754, #23432 ) ;
#80272=CARTESIAN_POINT ( 'NONE',  ( 17.82490373129249406, 1447.533498047817830, 216.9633381424519030 ) ) ;
#80277=ORIENTED_EDGE ( 'NONE', *, *, #74664, .T. ) ;
#80279=CARTESIAN_POINT ( 'NONE',  ( 25.42954105229999939, 1453.762068885830104, 238.1443982248979978 ) ) ;
#80281=CARTESIAN_POINT ( 'NONE',  ( -25.78156655170059608, 1509.813372604039841, 223.1298223243570078 ) ) ;
#80282=CARTESIAN_POINT ( 'NONE',  ( 1.983025529729999681, 1411.743863471630220, 232.0748871707980072 ) ) ;
#80284=CARTESIAN_POINT ( 'NONE',  ( -18.89405915729999919, 1457.450104263030198, 227.0059657532979998 ) ) ;
#80285=CARTESIAN_POINT ( 'NONE',  ( 2.500000000000000000, 1421.075716575930073, 150.9130928818979953 ) ) ;
#80286=CARTESIAN_POINT ( 'NONE',  ( -0.08886200314649998766, 1488.812149332629815, 187.8711066492980137 ) ) ;
#80288=AXIS2_PLACEMENT_3D ( 'NONE', #88897, #70477, #37953 ) ;
#80291=CARTESIAN_POINT ( 'NONE',  ( 1.757128879749999983, 1406.530468631129906, 269.4976381029979962 ) ) ;
#80293=ADVANCED_FACE ( 'NONE', ( #25864 ), #25310, .T. ) ;
#80294=CARTESIAN_POINT ( 'NONE',  ( 6.382104022434670121, 1471.436293962050058, 269.3346712093340329 ) ) ;
#80295=EDGE_CURVE ( 'NONE', #62931, #91917, #40484, .T. ) ;
#80303=CARTESIAN_POINT ( 'NONE',  ( 18.16298593701623076, 1438.550562606129006, 191.5625238809707298 ) ) ;
#80305=CARTESIAN_POINT ( 'NONE',  ( -34.97756117570000356, 1432.582706845480061, 262.6648722511980054 ) ) ;
#80306=EDGE_CURVE ( 'NONE', #59255, #19757, #45598, .T. ) ;
#80308=CARTESIAN_POINT ( 'NONE',  ( -0.5589788533730000175, 1476.074308366130026, 267.5370429008980295 ) ) ;
#80309=CARTESIAN_POINT ( 'NONE',  ( -4.256948536952839923, 1446.548991557320051, 160.0047540042930052 ) ) ;
#80311=CARTESIAN_POINT ( 'NONE',  ( -3.622779532894428556, 1448.291314561123500, 184.9376262326799463 ) ) ;
#80314=B_SPLINE_SURFACE_WITH_KNOTS ( 'NONE', 5, 5, ( 
 ( #20484, #11566, #105635, #104516, #11014, #44628 ),
 ( #37320, #3193, #105072, #46299, #88820, #87736 ),
 ( #95564, #54694, #45185, #80427, #12106, #97212 ),
 ( #28921, #1519, #35652, #86606, #54144, #78769 ),
 ( #79879, #79326, #37872, #61995, #106172, #69842 ),
 ( #96679, #27814, #71516, #2637, #103960, #62559 ),
 ( #29452, #52478, #63648, #18284, #27257, #18834 ),
 ( #19951, #10454, #36213, #96113, #45742, #80970 ),
 ( #31111, #57451, #49042, #99404, #13185, #89371 ),
 ( #97763, #21591, #55796, #74247, #46842, #47374 ),
 ( #31660, #81499, #40068, #108378, #22682, #55238 ),
 ( #39522, #89912, #4801, #56881, #73697, #65840 ),
 ( #12663, #65291, #91011, #38946, #83178, #73126 ),
 ( #107268, #30563, #5362, #40618, #48491, #56327 ),
 ( #64753, #91578, #107823, #98864, #14301, #82630 ),
 ( #22129, #6468, #5922, #4275, #38405, #90460 ),
 ( #13737, #47921, #82057, #72581, #99958, #23252 ),
 ( #14851, #74789, #108931, #29999, #64190, #98312 ),
 ( #106709, #32220, #21035, #1815, #86890, #86338 ),
 ( #18019, #49589, #58540, #43792, #53316, #100520 ),
 ( #10753, #75347, #83721, #57990, #52212, #78504 ),
 ( #92124, #7566, #15400, #87460, #26995, #27541 ),
 ( #84271, #69577, #95845, #44924, #109487, #103695 ),
 ( #94739, #104251, #10185, #44359, #79071, #2376 ),
 ( #24354, #95302, #9623, #32764, #77942, #101056 ),
 ( #61185, #1249, #35952, #70138, #7016, #35389 ),
 ( #92666, #66401, #15943, #18562, #103123, #50144 ) ),
 .UNSPECIFIED., .F., .F., .F.,
 ( 6, 3, 3, 3, 3, 3, 3, 3, 6 ),
 ( 6, 6 ),
 ( 103.3477632230000012, 105.7451336970000000, 107.5792266200000000, 108.1425041709999988, 110.4591985809999954, 112.7758929910000063, 117.4092818109999996, 129.0014047420000054, 142.9189258060000043 ),
 ( 0.000000000000000000, 2.000000000000000000 ),
 .UNSPECIFIED. ) ;
#80316=CARTESIAN_POINT ( 'NONE',  ( 11.87502392341400004, 1433.007271648830056, 149.9804723818110119 ) ) ;
#80317=CARTESIAN_POINT ( 'NONE',  ( 26.46020439838580174, 1436.724525556780009, 136.8114229838039932 ) ) ;
#80318=CARTESIAN_POINT ( 'NONE',  ( -5.519596238180829673, 1396.105808937369829, 218.6807260319289696 ) ) ;
#80319=CARTESIAN_POINT ( 'NONE',  ( -14.89476520160000028, 1422.388268083329876, 228.7586242300979791 ) ) ;
#80321=EDGE_CURVE ( 'NONE', #44371, #8321, #75049, .T. ) ;
#80322=CARTESIAN_POINT ( 'NONE',  ( 19.32723965911517183, 1455.838101669217849, 225.3662149856213830 ) ) ;
#80324=VERTEX_POINT ( 'NONE', #51104 ) ;
#80326=CARTESIAN_POINT ( 'NONE',  ( 0.8265245808140000427, 1408.941923261729926, 231.1644250952979860 ) ) ;
#80328=CARTESIAN_POINT ( 'NONE',  ( 11.00743345139999896, 1426.053315483930191, 99.60275282069790137 ) ) ;
#80331=EDGE_CURVE ( 'NONE', #94948, #95283, #56407, .T. ) ;
#80332=CARTESIAN_POINT ( 'NONE',  ( -12.45478753333599720, 1442.762691980110048, 205.2115877711401026 ) ) ;
#80336=CARTESIAN_POINT ( 'NONE',  ( 3.395856411370000050, 1508.797082644030070, 180.5462404550980011 ) ) ;
#80344=DIRECTION ( 'NONE',  ( 0.000000000000000000, 0.000000000000000000, -1.000000000000000000 ) ) ;
#80346=CARTESIAN_POINT ( 'NONE',  ( -21.65324558190001980, 1435.253471290908919, 140.9571069649979904 ) ) ;
#80349=CARTESIAN_POINT ( 'NONE',  ( -1.367322260308200255, 1418.654931759450164, 185.2513577252690311 ) ) ;
#80350=CARTESIAN_POINT ( 'NONE',  ( 1.657366258489999966, 1410.306738087430176, 185.3518365496979925 ) ) ;
#80353=CARTESIAN_POINT ( 'NONE',  ( -40.23885053629599895, 1448.346527775979894, 135.0415120907709934 ) ) ;
#80355=CARTESIAN_POINT ( 'NONE',  ( -2.500000000000000000, 1448.216394621219933, 167.2095406785390139 ) ) ;
#80358=CARTESIAN_POINT ( 'NONE',  ( -5.320809690189729935, 1406.488740053329821, 269.2842400656589916 ) ) ;
#80359=CARTESIAN_POINT ( 'NONE',  ( -19.00254521766261107, 1416.818673809775419, 207.9334427874379116 ) ) ;
#80360=ORIENTED_EDGE ( 'NONE', *, *, #52198, .T. ) ;
#80364=VERTEX_POINT ( 'NONE', #24754 ) ;
#80371=EDGE_CURVE ( 'NONE', #23739, #85422, #69432, .T. ) ;
#80372=ORIENTED_EDGE ( 'NONE', *, *, #57648, .T. ) ;
#80373=CARTESIAN_POINT ( 'NONE',  ( 0.5624690339869999889, 1416.828040475229955, 190.4759594386979984 ) ) ;
#80375=CARTESIAN_POINT ( 'NONE',  ( 0.3443454750360000483, 1415.932840167130053, 226.9638901923979972 ) ) ;
#80377=AXIS2_PLACEMENT_3D ( 'NONE', #85528, #17199, #49760 ) ;
#80380=CARTESIAN_POINT ( 'NONE',  ( -3.314356077729999406, 1409.028800251930079, 230.9273595247980211 ) ) ;
#80382=EDGE_CURVE ( 'NONE', #8790, #24414, #72939, .T. ) ;
#80384=CARTESIAN_POINT ( 'NONE',  ( -24.67970723617740347, 1440.913060461539771, 213.9247834336929941 ) ) ;
#80385=CARTESIAN_POINT ( 'NONE',  ( 20.32791520299490173, 1497.608840033019987, 226.4479123882990166 ) ) ;
#80386=CARTESIAN_POINT ( 'NONE',  ( 15.68254779764047235, 1506.474306118306004, 224.5749311187954902 ) ) ;
#80387=CARTESIAN_POINT ( 'NONE',  ( 20.94370973160000204, 1411.258104562529979, 270.0430967323979417 ) ) ;
#80388=ADVANCED_FACE ( 'NONE', ( #1820 ), #9627, .F. ) ;
#80392=CARTESIAN_POINT ( 'NONE',  ( 23.96253434680000183, 1410.844299666830011, 208.4004183790169975 ) ) ;
#80393=CARTESIAN_POINT ( 'NONE',  ( 0.01990864597794416921, 1507.260534525954881, 237.3641690013145649 ) ) ;
#80395=CARTESIAN_POINT ( 'NONE',  ( 19.20874097899815780, 1410.945473914794547, 195.6776540737980383 ) ) ;
#80397=ORIENTED_EDGE ( 'NONE', *, *, #57560, .F. ) ;
#80398=CARTESIAN_POINT ( 'NONE',  ( 22.53878404599999641, 1411.058442739730026, 206.1986151668880041 ) ) ;
#80399=CARTESIAN_POINT ( 'NONE',  ( -8.447610866089998893, 1417.903240752429838, 230.8139735681979801 ) ) ;
#80408=CARTESIAN_POINT ( 'NONE',  ( -0.3331897858350000297, 1408.924695719030069, 232.1910296785979995 ) ) ;
#80409=CARTESIAN_POINT ( 'NONE',  ( -0.1423985958509380034, 1420.464637908429950, 182.7409013480950080 ) ) ;
#80421=CARTESIAN_POINT ( 'NONE',  ( -1.729960644012338955, 1451.871857846600051, 184.1618444272322108 ) ) ;
#80425=CARTESIAN_POINT ( 'NONE',  ( -26.53762114791049598, 1508.774119630419818, 201.4667103074619945 ) ) ;
#80427=CARTESIAN_POINT ( 'NONE',  ( -17.95690667590000089, 1424.708104102629932, 226.6788193228979935 ) ) ;
#80428=CARTESIAN_POINT ( 'NONE',  ( -14.28308187130000029, 1434.994876553209906, 148.2389740282980028 ) ) ;
#80430=CARTESIAN_POINT ( 'NONE',  ( 19.30519085950000147, 1478.522678847230054, 190.2770777040979908 ) ) ;
#80432=CARTESIAN_POINT ( 'NONE',  ( 28.45309226149999660, 1509.159855970130138, 209.4524995968540111 ) ) ;
#80434=EDGE_LOOP ( 'NONE', ( #26298, #93429, #62205, #22158 ) ) ;
#80437=CARTESIAN_POINT ( 'NONE',  ( -45.51398236499812811, 1438.090180991398029, 268.9782812080896974 ) ) ;
#80438=CARTESIAN_POINT ( 'NONE',  ( -24.02573159490000165, 1437.659110011540179, 211.8884722500880002 ) ) ;
#80441=CARTESIAN_POINT ( 'NONE',  ( -18.46438761779999993, 1509.557851011129969, 231.7133587053980079 ) ) ;
#80443=CARTESIAN_POINT ( 'NONE',  ( 20.26030320659999617, 1497.713060387329961, 217.9272749506380080 ) ) ;
#80444=B_SPLINE_SURFACE_WITH_KNOTS ( 'NONE', 5, 1, ( 
 ( #26333, #68379 ),
 ( #35864, #60528 ),
 ( #68935, #1726 ),
 ( #94091, #104160 ),
 ( #77860, #50469 ),
 ( #76205, #17362 ),
 ( #7884, #8991 ),
 ( #27446, #78413 ),
 ( #92991, #103608 ) ),
 .UNSPECIFIED., .F., .F., .F.,
 ( 6, 3, 6 ),
 ( 2, 2 ),
 ( -5.179891626739999739E-09, 44.04929316810000017, 84.36259054890000186 ),
 ( 2.018291184700000240, 3.029415486610000041 ),
 .UNSPECIFIED. ) ;
#80445=CARTESIAN_POINT ( 'NONE',  ( -16.81223226430000039, 1414.913060387329779, 207.5743821216680089 ) ) ;
#80446=CARTESIAN_POINT ( 'NONE',  ( -1.419022340012153993, 1507.123642348895146, 237.1495897167226587 ) ) ;
#80458=ORIENTED_EDGE ( 'NONE', *, *, #110361, .T. ) ;
#80461=CARTESIAN_POINT ( 'NONE',  ( 12.55167427646019718, 1442.776442884412745, 169.4734868725398371 ) ) ;
#80462=CARTESIAN_POINT ( 'NONE',  ( 29.83023163778732467, 1419.452610179523845, 269.4690072239820324 ) ) ;
#80463=CARTESIAN_POINT ( 'NONE',  ( -33.33289073529999769, 1445.199364517940012, 248.0947902359980048 ) ) ;
#80464=CARTESIAN_POINT ( 'NONE',  ( -19.29261533819999741, 1484.706083574029890, 189.6393559541980096 ) ) ;
#80465=CARTESIAN_POINT ( 'NONE',  ( -11.58371378220000025, 1433.785063954710040, 151.2033516465980085 ) ) ;
#80466=CARTESIAN_POINT ( 'NONE',  ( 26.23319076840000008, 1508.580492117430140, 201.9768647809279969 ) ) ;
#80467=CARTESIAN_POINT ( 'NONE',  ( -19.46358587980000365, 1485.590242327929900, 189.9720724388979818 ) ) ;
#80468=CARTESIAN_POINT ( 'NONE',  ( 8.359567452010001176, 1410.137012574430173, 187.7727004011979659 ) ) ;
#80469=CARTESIAN_POINT ( 'NONE',  ( 4.976421422960000562, 1422.135394151030141, 185.3303333604980025 ) ) ;
#80472=CARTESIAN_POINT ( 'NONE',  ( 13.08769715623770047, 1428.580231863860035, 223.4460403848140118 ) ) ;
#80474=CARTESIAN_POINT ( 'NONE',  ( 1.099242448648459977E-08, 1409.143622018159931, 260.5448422644799962 ) ) ;
#80476=ORIENTED_EDGE ( 'NONE', *, *, #40810, .F. ) ;
#80477=CARTESIAN_POINT ( 'NONE',  ( -11.86456335612260027, 1432.228581043409804, 149.9813182647349947 ) ) ;
#80479=CARTESIAN_POINT ( 'NONE',  ( -10.57863510019999964, 1471.118849071129944, 270.0764144472979638 ) ) ;
#80481=( BOUNDED_CURVE ( )  B_SPLINE_CURVE ( 3, ( #3123, #98245, #80359, #12597 ),
 .UNSPECIFIED., .F., .F. ) 
 B_SPLINE_CURVE_WITH_KNOTS ( ( 4, 4 ),
 ( 1.036305842674305921, 2.105309002732549839 ),
 .UNSPECIFIED. ) 
 CURVE ( )  GEOMETRIC_REPRESENTATION_ITEM ( )  RATIONAL_B_SPLINE_CURVE ( ( 1.000000000000000000, 0.9070150915768222522, 0.9070150915768222522, 1.000000000000000000 ) ) 
 REPRESENTATION_ITEM ( '' )  );
#80484=EDGE_CURVE ( 'NONE', #19775, #67049, #49666, .T. ) ;
#80485=CARTESIAN_POINT ( 'NONE',  ( 0.3570880529365150213, 1450.920097230550027, 181.5564549562909917 ) ) ;
#80486=EDGE_CURVE ( 'NONE', #109427, #20723, #11312, .T. ) ;
#80487=CARTESIAN_POINT ( 'NONE',  ( 11.20854089337319870, 1414.996442620860080, 222.5314268542019818 ) ) ;
#80490=B_SPLINE_CURVE_WITH_KNOTS ( 'NONE', 5,
 ( #12064, #54106, #20995, #54654, #2041, #88784 ),
 .UNSPECIFIED., .F., .F.,
 ( 6, 6 ),
 ( -87.06999293180000166, -29.77037674149489987 ),
 .UNSPECIFIED. ) ;
#80492=CARTESIAN_POINT ( 'NONE',  ( -45.36837539640040262, 1437.179215847679870, 268.9823049396750321 ) ) ;
#80494=VERTEX_POINT ( 'NONE', #28652 ) ;
#80495=CARTESIAN_POINT ( 'NONE',  ( -3.536362979286669983, 1494.571137096670100, 181.5117196762699905 ) ) ;
#80500=CARTESIAN_POINT ( 'NONE',  ( 17.31001952156929491, 1410.038354363751978, 224.8086568639813834 ) ) ;
#80501=CARTESIAN_POINT ( 'NONE',  ( -4.111558752199999667, 1410.393682478630126, 186.7772447052980169 ) ) ;
#80504=EDGE_CURVE ( 'NONE', #102730, #7200, #41718, .T. ) ;
#80508=CARTESIAN_POINT ( 'NONE',  ( 3.118627138969999990, 1507.020746158230168, 237.9289388427980043 ) ) ;
#80510=VERTEX_POINT ( 'NONE', #86343 ) ;
#80511=CARTESIAN_POINT ( 'NONE',  ( -9.504797446096199920, 1411.012292308769702, 269.6245613120399867 ) ) ;
#80512=CARTESIAN_POINT ( 'NONE',  ( 3.043140677541010142, 1417.779445265420009, 234.3218410894589852 ) ) ;
#80517=CARTESIAN_POINT ( 'NONE',  ( 45.33376732508579465, 1444.887998074412053, 268.9831579371490307 ) ) ;
#80519=CARTESIAN_POINT ( 'NONE',  ( -14.02058551345489867, 1436.245318346960175, 150.2233960230930165 ) ) ;
#80520=AXIS2_PLACEMENT_3D ( 'NONE', #73823, #23927, #73259 ) ;
#80521=CARTESIAN_POINT ( 'NONE',  ( -0.03713005249742180186, 1409.802211749629805, 185.1324229550240261 ) ) ;
#80523=CARTESIAN_POINT ( 'NONE',  ( -18.53331733233340017, 1415.778512717889953, 207.5702610487440154 ) ) ;
#80524=CARTESIAN_POINT ( 'NONE',  ( 5.388168580889999504, 1432.635621093390000, 154.6140392605979912 ) ) ;
#80525=CARTESIAN_POINT ( 'NONE',  ( -0.0001223106876275270073, 1475.759747512889817, 269.0458114371340343 ) ) ;
#80526=CARTESIAN_POINT ( 'NONE',  ( 11.58478124470000026, 1415.063410489829948, 222.3466023727980030 ) ) ;
#80527=CARTESIAN_POINT ( 'NONE',  ( 5.538520585190000567, 1447.740028701229903, 184.7993824163979752 ) ) ;
#80529=ADVANCED_FACE ( 'NONE', ( #54434 ), #76884, .F. ) ;
#80530=VERTEX_POINT ( 'NONE', #102445 ) ;
#80531=FACE_OUTER_BOUND ( 'NONE', #16102, .T. ) ;
#80532=CARTESIAN_POINT ( 'NONE',  ( -21.56756540081639173, 1453.725795844561617, 221.9610449306620126 ) ) ;
#80534=CARTESIAN_POINT ( 'NONE',  ( 13.42479616400980014, 1453.338203267170002, 224.7140346886050111 ) ) ;
#80536=CARTESIAN_POINT ( 'NONE',  ( 24.72977296794550028, 1451.893578074279958, 136.8099502904200051 ) ) ;
#80537=CARTESIAN_POINT ( 'NONE',  ( 10.85845406881951192, 1424.793774302243946, 138.1921923613813590 ) ) ;
#80539=CARTESIAN_POINT ( 'NONE',  ( 20.08164004260000013, 1410.974782856229922, 197.5376054386979945 ) ) ;
#80540=CARTESIAN_POINT ( 'NONE',  ( 22.50660266490000083, 1409.865199449729971, 207.4947920653180233 ) ) ;
#80541=CARTESIAN_POINT ( 'NONE',  ( -24.25923418980000079, 1435.344651399380155, 136.2870029874980276 ) ) ;
#80543=CARTESIAN_POINT ( 'NONE',  ( 0.8365135405962150772, 1450.872666035589873, 181.3727942470009680 ) ) ;
#80544=CARTESIAN_POINT ( 'NONE',  ( 2.500000000000000000, 1439.611175471030037, 167.3041001658060054 ) ) ;
#80547=ORIENTED_EDGE ( 'NONE', *, *, #38495, .T. ) ;
#80549=CARTESIAN_POINT ( 'NONE',  ( 4.363122647530000009, 1409.354802298930053, 121.6099336315979969 ) ) ;
#80550=CARTESIAN_POINT ( 'NONE',  ( 11072.05219664940523, 50.13405481578727318, -8413.031381323531605 ) ) ;
#80551=CARTESIAN_POINT ( 'NONE',  ( -39.28604983332469658, 1447.310147778509872, 136.5961217192789832 ) ) ;
#80554=VECTOR ( 'NONE', #63203, 1000.000000000000000 ) ;
#80555=CARTESIAN_POINT ( 'NONE',  ( -2.375604933953470166, 1484.258301715329935, 183.2084465395040240 ) ) ;
#80556=CARTESIAN_POINT ( 'NONE',  ( 11.58906603029999971, 1433.009685293250186, 151.1019960182979958 ) ) ;
#80563=CARTESIAN_POINT ( 'NONE',  ( 11.23388613411650638, 1442.762691980111640, 150.9272215568491049 ) ) ;
#80564=CARTESIAN_POINT ( 'NONE',  ( -19.22829456215601240, 1485.595672753383042, 189.7356968105359840 ) ) ;
#80567=AXIS2_PLACEMENT_3D ( 'NONE', #2158, #70465, #62062 ) ;
#80569=CARTESIAN_POINT ( 'NONE',  ( -10.16988517760000121, 1507.385799736029867, 234.4102472725979851 ) ) ;
#80572=CARTESIAN_POINT ( 'NONE',  ( 6.244762013140000789, 1407.784308382130121, 220.5925233730980040 ) ) ;
#80574=CARTESIAN_POINT ( 'NONE',  ( 1.679567668810000081, 1466.272168333229956, 234.7591022376979879 ) ) ;
#80577=CARTESIAN_POINT ( 'NONE',  ( -0.8431545162750000433, 1451.883321300629859, 183.2674326525980177 ) ) ;
#80578=B_SPLINE_CURVE_WITH_KNOTS ( 'NONE', 3,
 ( #91443, #57854, #65150, #14719, #66269, #100386 ),
 .UNSPECIFIED., .F., .F.,
 ( 4, 2, 4 ),
 ( -0.03032162748288879869, -0.01516384315529340117, -1.347308482557360576E-05 ),
 .UNSPECIFIED. ) ;
#80581=FACE_OUTER_BOUND ( 'NONE', #16093, .T. ) ;
#80584=VERTEX_POINT ( 'NONE', #48774 ) ;
#80593=CARTESIAN_POINT ( 'NONE',  ( 14.43827355286400049, 1409.417256009360017, 212.9437002319959902 ) ) ;
#80594=CARTESIAN_POINT ( 'NONE',  ( -7.000000000000000000, 1418.913060387330006, 172.2701767054979882 ) ) ;
#80600=ORIENTED_EDGE ( 'NONE', *, *, #91995, .F. ) ;
#80602=CARTESIAN_POINT ( 'NONE',  ( -12.21876415543579952, 1416.384967875050052, 194.7139283324180212 ) ) ;
#80604=CIRCLE ( 'NONE', #5468, 10.00000000000000000 ) ;
#80605=CARTESIAN_POINT ( 'NONE',  ( 28.93380231721798523, 1509.926839725682157, 214.7155417130382205 ) ) ;
#80606=CARTESIAN_POINT ( 'NONE',  ( -20.19390448100880064, 1494.711078886199857, 190.7708293110239879 ) ) ;
#80607=CARTESIAN_POINT ( 'NONE',  ( 1.233310677790000032, 1396.496404931630195, 221.5848227596979996 ) ) ;
#80609=CARTESIAN_POINT ( 'NONE',  ( -0.1493273780539999818, 1457.270727498030055, 183.0267056797979990 ) ) ;
#80611=CARTESIAN_POINT ( 'NONE',  ( -21.56441729487620051, 1490.297465683720020, 208.8487828826750103 ) ) ;
#80613=B_SPLINE_CURVE_WITH_KNOTS ( 'NONE', 3,
 ( #53414, #70243, #36056, #104906, #97065, #104350, #1347, #87565, #43896, #10280, #3575, #96506, #106018, #35486, #28194, #95951, #29294, #88121, #62380 ),
 .UNSPECIFIED., .F., .F.,
 ( 4, 2, 2, 2, 1, 1, 1, 2, 2, 2, 4 ),
 ( 0.000000000000000000, 0.2500000000062882477, 0.3750000000094199648, 0.4375000000109754983, 0.4687500000117625354, 0.4843750000120938259, 0.4921875000122678534, 0.4960937500122905575, 0.5000000000123132615, 0.7500000000061566308, 1.000000000000000000 ),
 .UNSPECIFIED. ) ;
#80615=CARTESIAN_POINT ( 'NONE',  ( -13.25366502360200016, 1435.447908314299866, 150.3196125349689964 ) ) ;
#80617=CARTESIAN_POINT ( 'NONE',  ( 1.546869375790000056, 1416.835808384130132, 190.2224234606979962 ) ) ;
#80622=EDGE_CURVE ( 'NONE', #2110, #101455, #9178, .T. ) ;
#80623=CARTESIAN_POINT ( 'NONE',  ( 33.93598468090000608, 1424.339495328229987, 259.3467913669979907 ) ) ;
#80624=CARTESIAN_POINT ( 'NONE',  ( -26.79586899859999960, 1488.686659795530204, 205.7928254789879929 ) ) ;
#80625=CARTESIAN_POINT ( 'NONE',  ( -1.548023937630000013, 1507.264922098230045, 180.7964191004979853 ) ) ;
#80626=CARTESIAN_POINT ( 'NONE',  ( 13.28956057169999916, 1415.163755984130148, 197.3206489009980089 ) ) ;
#80627=CARTESIAN_POINT ( 'NONE',  ( 19.81028111248627610, 1506.776553286653552, 198.6443937896351031 ) ) ;
#80628=CARTESIAN_POINT ( 'NONE',  ( -33.60183516099999679, 1440.913060382750018, 248.0844435644980024 ) ) ;
#80632=CARTESIAN_POINT ( 'NONE',  ( -11.86982405321553813, 1423.326458348927872, 139.0999999980981556 ) ) ;
#80633=VERTEX_POINT ( 'NONE', #42009 ) ;
#80634=CARTESIAN_POINT ( 'NONE',  ( 3.344986830760000363, 1396.029869901429947, 197.7886967553979787 ) ) ;
#80636=CARTESIAN_POINT ( 'NONE',  ( 38.57017548136569474, 1443.484401788910191, 137.1611502647569978 ) ) ;
#80637=ORIENTED_EDGE ( 'NONE', *, *, #105614, .T. ) ;
#80642=CARTESIAN_POINT ( 'NONE',  ( 0.4843940562340000033, 1419.324133249529950, 184.6861775234980030 ) ) ;
#80645=CARTESIAN_POINT ( 'NONE',  ( -1.522526128800000045, 1470.485953140730089, 235.5269617602980077 ) ) ;
#80646=CARTESIAN_POINT ( 'NONE',  ( -8.301987938657498844, 1519.913060387329779, 186.6498241004079262 ) ) ;
#80648=CARTESIAN_POINT ( 'NONE',  ( 11.43740528939999912, 1425.481182534629852, 144.1672625331979987 ) ) ;
#80649=CARTESIAN_POINT ( 'NONE',  ( -12.85343379847840062, 1416.225364278609959, 221.8532119807159972 ) ) ;
#80650=CARTESIAN_POINT ( 'NONE',  ( 0.1144963318970000088, 1419.768049673130008, 184.3728032279979914 ) ) ;
#80651=ORIENTED_EDGE ( 'NONE', *, *, #97413, .F. ) ;
#80655=CARTESIAN_POINT ( 'NONE',  ( 11.86306020403040051, 1432.123576808339976, 149.9782128633559921 ) ) ;
#80656=CARTESIAN_POINT ( 'NONE',  ( 3.211105652400000121, 1415.841839642130026, 233.8555032973979735 ) ) ;
#80658=ORIENTED_EDGE ( 'NONE', *, *, #39236, .T. ) ;
#80664=CARTESIAN_POINT ( 'NONE',  ( 15.39361870879080030, 1452.375503376769984, 147.5811169514580001 ) ) ;
#80667=CARTESIAN_POINT ( 'NONE',  ( 19.19535387687943029, 1456.080104641030175, 225.8939609127118047 ) ) ;
#80668=CARTESIAN_POINT ( 'NONE',  ( -19.76905052135469987, 1509.627051507924534, 231.1952065043512619 ) ) ;
#80669=CARTESIAN_POINT ( 'NONE',  ( 0.002606494515621919725, 1408.913151437613124, 231.8315478586514189 ) ) ;
#80673=VECTOR ( 'NONE', #66961, 1000.000000000000000 ) ;
#80677=CARTESIAN_POINT ( 'NONE',  ( 1.088018564129999997E-14, 1422.873164470030133, 234.3916895801979763 ) ) ;
#80690=CARTESIAN_POINT ( 'NONE',  ( -8.954747414950000817, 1440.423832500330036, 186.6003702932979991 ) ) ;
#80692=CARTESIAN_POINT ( 'NONE',  ( 18.94483675106589970, 1509.587814354350257, 184.9180970421039945 ) ) ;
#80693=CARTESIAN_POINT ( 'NONE',  ( 2.923521462801879967, 1410.394928839790055, 231.6309329194170061 ) ) ;
#80695=CARTESIAN_POINT ( 'NONE',  ( 16.91151655639999518, 1417.432431737429852, 226.6666944154980001 ) ) ;
#80699=CARTESIAN_POINT ( 'NONE',  ( 46.02997383769999828, 1440.913083148580199, 268.4959101745980092 ) ) ;
#80700=CARTESIAN_POINT ( 'NONE',  ( -18.31053858800000000, 1410.915397185529855, 224.2400752736980110 ) ) ;
#80701=CARTESIAN_POINT ( 'NONE',  ( 15.36997192539999979, 1435.038989691999859, 147.5081777520979927 ) ) ;
#80703=CARTESIAN_POINT ( 'NONE',  ( 21.43187510470000134, 1508.012749821929901, 191.1662891575980154 ) ) ;
#80704=CARTESIAN_POINT ( 'NONE',  ( 29.55474026598078652, 1509.961787258783716, 207.3740816649607552 ) ) ;
#80705=CARTESIAN_POINT ( 'NONE',  ( -14.57206770570000032, 1474.063984277629970, 266.8771244472980015 ) ) ;
#80707=CARTESIAN_POINT ( 'NONE',  ( -35.91420678757950213, 1436.070278595480204, 135.9004835983330111 ) ) ;
#80708=CARTESIAN_POINT ( 'NONE',  ( 0.2144289812932060058, 1454.866627002209952, 183.1733190174600168 ) ) ;
#80709=CARTESIAN_POINT ( 'NONE',  ( -12.40156580232079975, 1408.024392905250124, 203.8687696987620086 ) ) ;
#80710=CARTESIAN_POINT ( 'NONE',  ( 1.590050350630178855, 1426.843352158476364, 137.0999999982234385 ) ) ;
#80714=CARTESIAN_POINT ( 'NONE',  ( -37.46849106905889926, 1436.652236075829933, 134.0999999968449856 ) ) ;
#80716=ORIENTED_EDGE ( 'NONE', *, *, #16624, .F. ) ;
#80722=CARTESIAN_POINT ( 'NONE',  ( 15.86904733465020101, 1508.170982057090214, 231.8327019708549983 ) ) ;
#80723=CARTESIAN_POINT ( 'NONE',  ( -37.32007217949999500, 1461.346032246330196, 269.2040743517979990 ) ) ;
#80726=DIRECTION ( 'NONE',  ( 0.03489949194094554841, 0.9993908271853728653, 4.612811327639278900E-09 ) ) ;
#80731=CARTESIAN_POINT ( 'NONE',  ( -28.75826058165200294, 1509.399771098719839, 208.7351958221130133 ) ) ;
#80733=CARTESIAN_POINT ( 'NONE',  ( 0.4970513752842960487, 1415.323890719899964, 184.8574490102490131 ) ) ;
#80736=CARTESIAN_POINT ( 'NONE',  ( -23.55538518210000021, 1409.900238766430220, 208.7448397572840122 ) ) ;
#80737=B_SPLINE_CURVE_WITH_KNOTS ( 'NONE', 3,
 ( #26886, #70027, #104690, #1702 ),
 .UNSPECIFIED., .F., .F.,
 ( 4, 4 ),
 ( 0.000000000000000000, 1.000000000000000000 ),
 .UNSPECIFIED. ) ;
#80740=CARTESIAN_POINT ( 'NONE',  ( -12.26151716610000086, 1416.568813549730066, 194.6723721426980092 ) ) ;
#80742=CARTESIAN_POINT ( 'NONE',  ( 22.27637251949999708, 1409.690968457230156, 211.0033668272880050 ) ) ;
#80745=CARTESIAN_POINT ( 'NONE',  ( -15.03569858740000065, 1422.461940334329938, 228.7610666488980087 ) ) ;
#80748=CARTESIAN_POINT ( 'NONE',  ( 25.19844959086550062, 1449.936406620129901, 207.7167063678460011 ) ) ;
#80751=B_SPLINE_CURVE_WITH_KNOTS ( 'NONE', 3,
 ( #6479, #49601, #56894, #39535, #92136, #58002, #40630, #83734, #7029, #101068, #100531, #23811 ),
 .UNSPECIFIED., .F., .F.,
 ( 4, 2, 2, 2, 2, 4 ),
 ( 0.000000000000000000, 0.1249999999998835931, 0.2499999999997671862, 0.4999999999998447908, 0.7499999999999223954, 1.000000000000000000 ),
 .UNSPECIFIED. ) ;
#80752=CARTESIAN_POINT ( 'NONE',  ( -22.75992841280000079, 1415.999885432929887, 212.0429175107379933 ) ) ;
#80757=VERTEX_POINT ( 'NONE', #34153 ) ;
#80762=VERTEX_POINT ( 'NONE', #57180 ) ;
#80763=CARTESIAN_POINT ( 'NONE',  ( 27.44017514259999757, 1508.035989681029832, 213.3629512357580325 ) ) ;
#80764=ORIENTED_EDGE ( 'NONE', *, *, #41271, .F. ) ;
#80767=CARTESIAN_POINT ( 'NONE',  ( -15.73553964349176226, 1409.462560401643486, 225.4753464985124367 ) ) ;
#80768=CARTESIAN_POINT ( 'NONE',  ( -11.99512490559999911, 1410.769353062130222, 225.2869993423979906 ) ) ;
#80770=CARTESIAN_POINT ( 'NONE',  ( -25.25207292682919658, 1450.803465017199869, 137.6137618836170020 ) ) ;
#80773=CARTESIAN_POINT ( 'NONE',  ( 9.206517179299998688, 1410.169093132829857, 230.1231226820979998 ) ) ;
#80777=CARTESIAN_POINT ( 'NONE',  ( 40.60962964061170055, 1447.683802590399864, 134.0999999984219926 ) ) ;
#80780=CARTESIAN_POINT ( 'NONE',  ( 14.30278547136329870, 1435.293658520200097, 149.3523124186869779 ) ) ;
#80784=ORIENTED_EDGE ( 'NONE', *, *, #6976, .T. ) ;
#80785=CARTESIAN_POINT ( 'NONE',  ( 8.710226003111458226, 1410.592674012450061, 230.2685501115730915 ) ) ;
#80788=CARTESIAN_POINT ( 'NONE',  ( -3.054816054689999838, 1485.996906145230014, 182.1538611197979947 ) ) ;
#80790=CARTESIAN_POINT ( 'NONE',  ( -17.78690504666375816, 1447.654120957741043, 217.2684850421684359 ) ) ;
#80792=CARTESIAN_POINT ( 'NONE',  ( 9221.844915941721410, 50.28429875041810249, -5636.577220268512065 ) ) ;
#80795=CARTESIAN_POINT ( 'NONE',  ( 1.543258704960000172, 1416.522662136229883, 190.2352491560979786 ) ) ;
#80797=EDGE_LOOP ( 'NONE', ( #88096, #38938, #20852, #110713, #37327 ) ) ;
#80800=CARTESIAN_POINT ( 'NONE',  ( 25.39713358094629569, 1440.913060387330006, 240.3806062677190027 ) ) ;
#80804=CARTESIAN_POINT ( 'NONE',  ( -15.88334012139999984, 1409.634352649830134, 191.9077379488980171 ) ) ;
#80805=CARTESIAN_POINT ( 'NONE',  ( -23.20186796309999977, 1425.882772870329973, 212.0388266195080007 ) ) ;
#80806=CARTESIAN_POINT ( 'NONE',  ( -24.39260148680000029, 1440.996668616129909, 211.3370849838079835 ) ) ;
#80810=CARTESIAN_POINT ( 'NONE',  ( 35.72701205430000471, 1418.844138006729963, 266.4694652101980523 ) ) ;
#80811=CARTESIAN_POINT ( 'NONE',  ( -27.66673063000770227, 1441.266444767720259, 137.2829077538830234 ) ) ;
#80812=CARTESIAN_POINT ( 'NONE',  ( 14.60161135774977126, 1435.005028810949170, 148.0399020830880659 ) ) ;
#80813=EDGE_CURVE ( 'NONE', #42031, #94989, #108730, .T. ) ;
#80816=CARTESIAN_POINT ( 'NONE',  ( 11.63669227459999966, 1425.864836378729933, 144.1684971660979784 ) ) ;
#80817=CARTESIAN_POINT ( 'NONE',  ( -0.1604665283746669890, 1507.146139023270052, 180.9012722249049716 ) ) ;
#80818=CARTESIAN_POINT ( 'NONE',  ( 19.43120254477782893, 1441.383652375895053, 212.5091604960843767 ) ) ;
#80820=CARTESIAN_POINT ( 'NONE',  ( -20.52471789389999657, 1470.812340169729850, 209.0748028894099946 ) ) ;
#80824=CARTESIAN_POINT ( 'NONE',  ( 15.47923624849999946, 1465.564491349630089, 248.5133305153979961 ) ) ;
#80825=CARTESIAN_POINT ( 'NONE',  ( -11.86593889309999916, 1432.333689122770011, 150.3973551558979977 ) ) ;
#80828=CARTESIAN_POINT ( 'NONE',  ( -0.3973340087122340103, 1418.672806152889962, 184.7148007238050127 ) ) ;
#80830=CARTESIAN_POINT ( 'NONE',  ( -18.70316662140000119, 1457.451126846130137, 227.2880144703979965 ) ) ;
#80831=CARTESIAN_POINT ( 'NONE',  ( 2.500000000000000000, 1430.041878304429929, 157.3252622477980083 ) ) ;
#80836=CARTESIAN_POINT ( 'NONE',  ( 1.770390159249999984, 1406.013915744430051, 266.9599398126979963 ) ) ;
#80839=CARTESIAN_POINT ( 'NONE',  ( 38.28767213281710724, 1455.716104437349941, 270.0147264652339913 ) ) ;
#80842=DIRECTION ( 'NONE',  ( 0.000000000000000000, 0.000000000000000000, -1.000000000000000000 ) ) ;
#80843=ADVANCED_FACE ( 'NONE', ( #27402 ), #35817, .F. ) ;
#80849=CARTESIAN_POINT ( 'NONE',  ( 2.310870013312309901, 1449.824111145019970, 154.7919404106129946 ) ) ;
#80850=EDGE_CURVE ( 'NONE', #56812, #52184, #3260, .T. ) ;
#80851=CARTESIAN_POINT ( 'NONE',  ( -14.37881581502230155, 1416.259629948920065, 221.3107050206100155 ) ) ;
#80855=CARTESIAN_POINT ( 'NONE',  ( -24.08292308869999943, 1431.749769072390109, 243.9198229650980068 ) ) ;
#80858=CARTESIAN_POINT ( 'NONE',  ( -0.5580518338940000378, 1475.981069911630129, 267.2348423975979586 ) ) ;
#80859=DIRECTION ( 'NONE',  ( -8.703204010890035850E-06, -3.665990706876905690E-05, 0.9999999992901525969 ) ) ;
#80861=CARTESIAN_POINT ( 'NONE',  ( -2.991382624059956807, 1448.269496906028508, 184.4535707602067021 ) ) ;
#80867=CARTESIAN_POINT ( 'NONE',  ( -10.79328541798980012, 1396.289970219479983, 211.5874294395580080 ) ) ;
#80868=EDGE_CURVE ( 'NONE', #104691, #45986, #25731, .T. ) ;
#80869=CARTESIAN_POINT ( 'NONE',  ( -15.65995984010000086, 1420.957345113829888, 227.0387551958980055 ) ) ;
#80873=CARTESIAN_POINT ( 'NONE',  ( 2.445258106880000337, 1408.998450681829809, 230.6876405877980005 ) ) ;
#80875=CARTESIAN_POINT ( 'NONE',  ( -18.75204458307589661, 1485.356665832905264, 189.3982496731914580 ) ) ;
#80876=CARTESIAN_POINT ( 'NONE',  ( 10.14778948840000083, 1425.169760000230099, 103.4485609486980024 ) ) ;
#80879=EDGE_CURVE ( 'NONE', #46444, #90450, #5517, .T. ) ;
#80880=CARTESIAN_POINT ( 'NONE',  ( -11.23388613411650638, 1442.762691980111640, 205.3674499604519212 ) ) ;
#80884=CARTESIAN_POINT ( 'NONE',  ( 3.240124005049999756, 1507.974159727629967, 181.2795196955979975 ) ) ;
#80890=ORIENTED_EDGE ( 'NONE', *, *, #71422, .T. ) ;
#80891=CARTESIAN_POINT ( 'NONE',  ( -10.60278645200000192, 1398.227574263030192, 200.8859367841879759 ) ) ;
#80892=CARTESIAN_POINT ( 'NONE',  ( 1.151838181399999828, 1507.064426625830038, 237.0475204680980141 ) ) ;
#80893=CARTESIAN_POINT ( 'NONE',  ( 0.8073615121260000471, 1466.693077628429819, 235.5175635199979922 ) ) ;
#80894=CARTESIAN_POINT ( 'NONE',  ( 12.45610846519999981, 1519.913060387329779, 228.8821925242980058 ) ) ;
#80897=CARTESIAN_POINT ( 'NONE',  ( -1.359208896535600175, 1412.363887663969990, 185.5179172785579738 ) ) ;
#80898=CARTESIAN_POINT ( 'NONE',  ( 4.222593189340000386, 1429.767617791429984, 185.2245064671979833 ) ) ;
#80900=CARTESIAN_POINT ( 'NONE',  ( -40.68043012285709636, 1444.654440062869980, 137.0056235015979951 ) ) ;
#80902=CARTESIAN_POINT ( 'NONE',  ( 39.39001429889999883, 1440.250354032689984, 136.7508189299979904 ) ) ;
#80904=CARTESIAN_POINT ( 'NONE',  ( 33.92729710940290744, 1435.682235881620045, 135.5031028085159903 ) ) ;
#80905=CARTESIAN_POINT ( 'NONE',  ( 11.84773374989999972, 1431.064121367410053, 149.8383244911979943 ) ) ;
#80909=CARTESIAN_POINT ( 'NONE',  ( -3.827327206003696247, 1409.546157813740592, 137.0999999980979851 ) ) ;
#80911=ORIENTED_EDGE ( 'NONE', *, *, #98162, .T. ) ;
#80913=CARTESIAN_POINT ( 'NONE',  ( -19.06375576466449928, 1488.013913749329959, 228.8372936450909947 ) ) ;
#80914=CARTESIAN_POINT ( 'NONE',  ( -14.33877495950000025, 1460.594445894529827, 230.1573440692980341 ) ) ;
#80915=CARTESIAN_POINT ( 'NONE',  ( -14.70465418319999884, 1470.816980702929868, 194.9479760845979968 ) ) ;
#80919=CARTESIAN_POINT ( 'NONE',  ( -11.71614241347159968, 1509.388950667939980, 181.5344912488080240 ) ) ;
#80922=CARTESIAN_POINT ( 'NONE',  ( 16.61533299009999709, 1414.913060387329779, 212.4682773652579897 ) ) ;
#80924=ORIENTED_EDGE ( 'NONE', *, *, #95034, .T. ) ;
#80927=CARTESIAN_POINT ( 'NONE',  ( -2.697248550460000338, 1409.007250382230040, 231.5774121206980283 ) ) ;
#80928=CARTESIAN_POINT ( 'NONE',  ( -6.553899686920000356, 1408.913060387329779, 192.3638312768979972 ) ) ;
#80931=CARTESIAN_POINT ( 'NONE',  ( -30.39409183528769987, 1440.913060387249971, 239.5824303925190009 ) ) ;
#80935=CARTESIAN_POINT ( 'NONE',  ( 43.35688237767370623, 1431.798309265539956, 270.1056626526180366 ) ) ;
#80938=CARTESIAN_POINT ( 'NONE',  ( 23.66578124539999806, 1410.976491880930098, 207.8922445630679761 ) ) ;
#80939=CARTESIAN_POINT ( 'NONE',  ( -12.08786860576782729, 1428.067598096224174, 223.1528678408886037 ) ) ;
#80943=CARTESIAN_POINT ( 'NONE',  ( 4.172805552454540212, 1421.497310399080106, 184.9553930896919951 ) ) ;
#80944=LINE ( 'NONE', #54668, #64554 ) ;
#80949=EDGE_CURVE ( 'NONE', #84894, #107129, #91092, .T. ) ;
#80950=CARTESIAN_POINT ( 'NONE',  ( 18.90776592919999644, 1416.839648759230158, 210.0259814473739937 ) ) ;
#80951=CARTESIAN_POINT ( 'NONE',  ( -21.06135014068000189, 1509.319523268100056, 228.6460338313929981 ) ) ;
#80952=EDGE_CURVE ( 'NONE', #104178, #34578, #24242, .T. ) ;
#80955=CARTESIAN_POINT ( 'NONE',  ( -14.94707557629999961, 1464.413060387330006, 223.3779789887979916 ) ) ;
#80963=CARTESIAN_POINT ( 'NONE',  ( 11.60004869884835621, 1426.501518730301996, 135.6460183129449604 ) ) ;
#80965=CARTESIAN_POINT ( 'NONE',  ( 9.928347934575134204, 1435.779368277902222, 152.5402617987141696 ) ) ;
#80968=CARTESIAN_POINT ( 'NONE',  ( -26.90301038610129680, 1509.321327670540086, 201.3214349759640243 ) ) ;
#80969=CARTESIAN_POINT ( 'NONE',  ( -2.705316718739999793, 1447.083576453610021, 165.9366052023979989 ) ) ;
#80970=CARTESIAN_POINT ( 'NONE',  ( -19.14726318969999852, 1425.916566196629901, 226.2004032037980039 ) ) ;
#80972=CARTESIAN_POINT ( 'NONE',  ( -20.53413670659999823, 1435.214474261499845, 143.2474216777980018 ) ) ;
#80973=CARTESIAN_POINT ( 'NONE',  ( -0.5954300179934969295, 1497.361593313569983, 231.3170566686650034 ) ) ;
#80974=CARTESIAN_POINT ( 'NONE',  ( 16.10738486569999850, 1509.418797648129839, 185.7100371376980092 ) ) ;
#80976=CARTESIAN_POINT ( 'NONE',  ( -17.88309616991011453, 1434.908678899640790, 215.0727088695880127 ) ) ;
#80986=CARTESIAN_POINT ( 'NONE',  ( -2.968899200039013753, 1425.987603892220477, 185.4310391008963563 ) ) ;
#80987=CARTESIAN_POINT ( 'NONE',  ( -12.58579218318286053, 1442.781936543507527, 186.0352767261755105 ) ) ;
#80988=CARTESIAN_POINT ( 'NONE',  ( 13.56949689579999863, 1407.458599673630033, 211.9076660747180085 ) ) ;
#80999=ORIENTED_EDGE ( 'NONE', *, *, #98162, .F. ) ;
#81000=CARTESIAN_POINT ( 'NONE',  ( 24.96344457455600008, 1444.384464582640021, 207.7241043758569674 ) ) ;
#81003=CARTESIAN_POINT ( 'NONE',  ( 16.16460400119147778, 1412.754790776669097, 269.3697747609250541 ) ) ;
#81004=CARTESIAN_POINT ( 'NONE',  ( -36.52133863790000134, 1445.557345868840230, 254.5789810496980010 ) ) ;
#81005=CARTESIAN_POINT ( 'NONE',  ( -20.47178266730000118, 1503.711780051630058, 190.1944351405979887 ) ) ;
#81008=CARTESIAN_POINT ( 'NONE',  ( 11.62784611939870061, 1426.769117065760156, 136.3672025267389927 ) ) ;
#81010=CARTESIAN_POINT ( 'NONE',  ( -25.18648013920000039, 1436.583765715590062, 137.5280688333979811 ) ) ;
#81016=CARTESIAN_POINT ( 'NONE',  ( 5.086570735490939355E-09, 1409.986055680089976, 258.6209524227260204 ) ) ;
#81021=CARTESIAN_POINT ( 'NONE',  ( -13.37958332629999880, 1471.793002122430153, 270.4094488012979696 ) ) ;
#81025=CARTESIAN_POINT ( 'NONE',  ( 0.2383086145270630063, 1451.487641661899943, 182.6700190730029760 ) ) ;
#81026=CARTESIAN_POINT ( 'NONE',  ( -14.06463665569999932, 1420.693613352630109, 227.5127406239979848 ) ) ;
#81030=CARTESIAN_POINT ( 'NONE',  ( -45.04224761993110349, 1433.697822895979925, 268.5281460005010103 ) ) ;
#81032=CARTESIAN_POINT ( 'NONE',  ( -3.542414024086459889, 1500.294088126669976, 181.2680764341660051 ) ) ;
#81036=CARTESIAN_POINT ( 'NONE',  ( 4.494990604111427146, 1423.798284629885757, 183.7099184631668720 ) ) ;
#81038=CARTESIAN_POINT ( 'NONE',  ( -6.310775319510000259, 1470.460832479730243, 184.4692652257980114 ) ) ;
#81039=CARTESIAN_POINT ( 'NONE',  ( 5.360207926212690488, 1422.242713656610022, 144.1549664376839814 ) ) ;
#81045=CARTESIAN_POINT ( 'NONE',  ( -22.76371513368420452, 1413.786089238920113, 270.3574169790829842 ) ) ;
#81046=CARTESIAN_POINT ( 'NONE',  ( -30.19569412050000068, 1435.551785849099815, 135.1818641824980034 ) ) ;
#81050=EDGE_LOOP ( 'NONE', ( #25453, #38197, #58652, #49266 ) ) ;
#81051=CARTESIAN_POINT ( 'NONE',  ( 40.87089738971353370, 1456.294579038563143, 269.1063834202503813 ) ) ;
#81054=CARTESIAN_POINT ( 'NONE',  ( -13.95044291110659884, 1436.238062604179959, 150.2632303846619948 ) ) ;
#81055=CARTESIAN_POINT ( 'NONE',  ( -0.03462643923284049879, 1410.128970406620056, 185.0390004595289781 ) ) ;
#81057=CARTESIAN_POINT ( 'NONE',  ( -20.74431189456849722, 1506.539416732394102, 216.6629043160080812 ) ) ;
#81059=CARTESIAN_POINT ( 'NONE',  ( -0.0001244928238367220131, 1476.109334953009920, 267.8539258397410094 ) ) ;
#81060=CARTESIAN_POINT ( 'NONE',  ( 11.76272948489999948, 1415.263254653229978, 222.9123187206980106 ) ) ;
#81064=CARTESIAN_POINT ( 'NONE',  ( -36.37832872588079169, 1451.642701155429904, 134.7398512091019995 ) ) ;
#81065=CARTESIAN_POINT ( 'NONE',  ( -23.84299525371533690, 1446.521247574655490, 213.7712371745673465 ) ) ;
#81066=ORIENTED_EDGE ( 'NONE', *, *, #100084, .T. ) ;
#81067=CARTESIAN_POINT ( 'NONE',  ( 3.955232551284513232, 1457.450780121971093, 228.4962720231502828 ) ) ;
#81069=CARTESIAN_POINT ( 'NONE',  ( 24.07258447067579965, 1452.056610454110114, 137.0856313116819933 ) ) ;
#81070=CARTESIAN_POINT ( 'NONE',  ( 13.91566348329999947, 1415.553739809529816, 196.9408153421979932 ) ) ;
#81072=CARTESIAN_POINT ( 'NONE',  ( 22.02260509859999971, 1411.040493132430129, 203.2687847944879991 ) ) ;
#81073=CARTESIAN_POINT ( 'NONE',  ( -2.572473174660243611, 1447.610664178797833, 170.5280181871044078 ) ) ;
#81074=CARTESIAN_POINT ( 'NONE',  ( -26.02813552489999793, 1435.406381042510020, 135.3446223067979872 ) ) ;
#81077=CARTESIAN_POINT ( 'NONE',  ( 0.8897843876074499336, 1451.970290787959811, 183.2052206821309994 ) ) ;
#81078=CARTESIAN_POINT ( 'NONE',  ( 2.500000000000199840, 1439.253548877449930, 159.5301951678090120 ) ) ;
#81082=B_SPLINE_SURFACE_WITH_KNOTS ( 'NONE', 5, 4, ( 
 ( #11468, #17615, #87059, #78105, #77020 ),
 ( #10346, #53482, #1982, #9798, #70301 ),
 ( #326, #45089, #34452, #79229, #61893 ),
 ( #43963, #873, #34997, #69177, #103283 ),
 ( #102729, #26590, #95466, #44518, #26023 ),
 ( #18730, #104413, #2538, #60787, #27706 ),
 ( #1406, #60219, #94337, #62449, #36662 ),
 ( #94913, #35547, #69742, #70856, #104967 ),
 ( #103861, #27162, #54591, #88726, #37767 ) ),
 .UNSPECIFIED., .F., .F., .F.,
 ( 6, 3, 6 ),
 ( 5, 5 ),
 ( 0.000000000000000000, 5.782490304330000441, 11.25975508159999983 ),
 ( 40.20365518519999881, 50.26548245740000453 ),
 .UNSPECIFIED. ) ;
#81084=CARTESIAN_POINT ( 'NONE',  ( -0.2587093370397540171, 1408.925427049060090, 231.8715964213000120 ) ) ;
#81085=CARTESIAN_POINT ( 'NONE',  ( -5.684698874817770253, 1422.983442514339913, 101.6537644099010009 ) ) ;
#81086=CARTESIAN_POINT ( 'NONE',  ( -39.77744193145330343, 1446.343101763050072, 136.7458254679739866 ) ) ;
#81087=CARTESIAN_POINT ( 'NONE',  ( 11.60004869885203682, 1425.678573708903514, 138.3920037478602012 ) ) ;
#81088=DIRECTION ( 'NONE',  ( -0.9955685427539349153, -0.04363816682463748930, 0.08330058268098361474 ) ) ;
#81089=CARTESIAN_POINT ( 'NONE',  ( -2.637143185960590053, 1477.800872778979965, 183.5714675770420001 ) ) ;
#81091=ADVANCED_FACE ( 'NONE', ( #68211 ), #43540, .T. ) ;
#81092=CARTESIAN_POINT ( 'NONE',  ( -3.276827735968430133, 1474.091273656589919, 270.1354579856779878 ) ) ;
#81093=CARTESIAN_POINT ( 'NONE',  ( 34.06181652996020404, 1440.913060384559913, 248.9867622432190046 ) ) ;
#81099=ADVANCED_FACE ( 'NONE', ( #34571 ), #57161, .F. ) ;
#81101=CARTESIAN_POINT ( 'NONE',  ( -28.59841874049999788, 1509.911739175030107, 211.5620548042080031 ) ) ;
#81105=CARTESIAN_POINT ( 'NONE',  ( -13.73919968929999946, 1508.116376860629998, 232.6024638145979964 ) ) ;
#81109=( BOUNDED_CURVE ( )  B_SPLINE_CURVE ( 3, ( #100552, #49076, #72617, #74282 ),
 .UNSPECIFIED., .F., .F. ) 
 B_SPLINE_CURVE_WITH_KNOTS ( ( 4, 4 ),
 ( 4.624801027031749889, 4.863190234949479773 ),
 .UNSPECIFIED. ) 
 CURVE ( )  GEOMETRIC_REPRESENTATION_ITEM ( )  RATIONAL_B_SPLINE_CURVE ( ( 1.000000000000000000, 0.9952698197215197329, 0.9952698197215197329, 1.000000000000000000 ) ) 
 REPRESENTATION_ITEM ( '' )  );
#81110=CARTESIAN_POINT ( 'NONE',  ( 1.846023538469999892, 1465.081219559430110, 235.4517473921979729 ) ) ;
#81113=CARTESIAN_POINT ( 'NONE',  ( -0.4298670265450000305, 1452.022084704629833, 183.1235002304979957 ) ) ;
#81116=CARTESIAN_POINT ( 'NONE',  ( -16.66147553287439820, 1414.913057846380070, 208.2448045594530015 ) ) ;
#81122=DIRECTION ( 'NONE',  ( 0.5450600352768949497, -0.8383970168982891602, 0.000000000000000000 ) ) ;
#81126=CARTESIAN_POINT ( 'NONE',  ( 5.844095810701279703, 1409.117140709990053, 195.3369297680639818 ) ) ;
#81127=CARTESIAN_POINT ( 'NONE',  ( 5.992819232552546005, 1413.913060387330006, 220.0916279853276762 ) ) ;
#81128=CARTESIAN_POINT ( 'NONE',  ( 2.523331955360000212, 1419.463757169429982, 185.1820755668979643 ) ) ;
#81130=CARTESIAN_POINT ( 'NONE',  ( -18.83305916869999663, 1478.165930216330025, 189.8264731359980146 ) ) ;
#81133=CARTESIAN_POINT ( 'NONE',  ( -3.503066957091310218, 1450.087732454140223, 184.8680753463810049 ) ) ;
#81138=CARTESIAN_POINT ( 'NONE',  ( -12.13275115633589962, 1416.073666499230058, 194.7976983533769726 ) ) ;
#81139=CARTESIAN_POINT ( 'NONE',  ( -12.30998824179999929, 1434.241983831289872, 150.0643212511979812 ) ) ;
#81140=B_SPLINE_CURVE_WITH_KNOTS ( 'NONE', 5,
 ( #25717, #82888, #91835, #101312, #102433, #42541 ),
 .UNSPECIFIED., .F., .F.,
 ( 6, 6 ),
 ( 0.000000000000000000, 1.000000000000000000 ),
 .UNSPECIFIED. ) ;
#81141=CARTESIAN_POINT ( 'NONE',  ( -7.502908036863889723E-10, 1468.442909337529954, 249.6120660866809828 ) ) ;
#81142=CARTESIAN_POINT ( 'NONE',  ( -20.56963670059100124, 1506.881352026369996, 190.4177983208670071 ) ) ;
#81143=CARTESIAN_POINT ( 'NONE',  ( -24.39386434493582811, 1435.492275954125716, 137.6392133633064816 ) ) ;
#81145=CARTESIAN_POINT ( 'NONE',  ( -19.15967863205523969, 1486.263174534858535, 189.4699138206827911 ) ) ;
#81150=B_SPLINE_CURVE_WITH_KNOTS ( 'NONE', 5,
 ( #3120, #72511, #52957, #96042, #53514, #37800, #36692, #29379, #10946, #78698, #106639, #45118 ),
 .UNSPECIFIED., .F., .F.,
 ( 6, 3, 3, 6 ),
 ( 0.000000000000000000, 0.1846806524304075159, 0.5540478659889513935, 1.000000000000000000 ),
 .UNSPECIFIED. ) ;
#81152=CARTESIAN_POINT ( 'NONE',  ( 11.95006413401319989, 1433.524393973229735, 149.8867095871329980 ) ) ;
#81153=CARTESIAN_POINT ( 'NONE',  ( -13.62029002549420120, 1434.976853200989808, 148.9443457557660224 ) ) ;
#81155=CARTESIAN_POINT ( 'NONE',  ( 1.546949757049999929, 1416.828042640230024, 190.2227907535979909 ) ) ;
#81156=CARTESIAN_POINT ( 'NONE',  ( -8.881784196999999612E-15, 1443.913060387330006, 126.8032249175980155 ) ) ;
#81158=ORIENTED_EDGE ( 'NONE', *, *, #11242, .T. ) ;
#81159=CARTESIAN_POINT ( 'NONE',  ( 11.55307713589999885, 1412.346723009130073, 255.2309128184979556 ) ) ;
#81160=CARTESIAN_POINT ( 'NONE',  ( -27.78146449870000012, 1508.131230135330043, 206.3146870670979922 ) ) ;
#81161=CARTESIAN_POINT ( 'NONE',  ( -10.91009346278590009, 1426.088824854960194, 92.74416427518930561 ) ) ;
#81162=CARTESIAN_POINT ( 'NONE',  ( 2.743693168446419660E-14, 1421.936573599349913, 238.0271386588229916 ) ) ;
#81163=CARTESIAN_POINT ( 'NONE',  ( -5.000068473801503544, 1407.851922743381010, 270.1322175188799974 ) ) ;
#81164=CARTESIAN_POINT ( 'NONE',  ( -24.33135486439999795, 1436.015388124420042, 216.3889742816580224 ) ) ;
#81166=CARTESIAN_POINT ( 'NONE',  ( -13.27254556637139338, 1414.941240495243619, 220.1937345174850975 ) ) ;
#81167=CARTESIAN_POINT ( 'NONE',  ( 27.01382259529999885, 1450.681608749369843, 136.4483196305980073 ) ) ;
#81169=CARTESIAN_POINT ( 'NONE',  ( 3.254127503250000331, 1396.026697023729866, 198.1014182944979893 ) ) ;
#81173=ORIENTED_EDGE ( 'NONE', *, *, #8063, .F. ) ;
#81175=CARTESIAN_POINT ( 'NONE',  ( -22.82027165193229834, 1409.709881720489875, 208.9770212787329910 ) ) ;
#81179=CARTESIAN_POINT ( 'NONE',  ( -2.040341087039999834, 1470.484922564130102, 235.4172632116979855 ) ) ;
#81181=ORIENTED_EDGE ( 'NONE', *, *, #43961, .F. ) ;
#81182=CARTESIAN_POINT ( 'NONE',  ( 11.73645620740000162, 1426.280382981230105, 144.1655706652979632 ) ) ;
#81183=CARTESIAN_POINT ( 'NONE',  ( -13.15726446870029953, 1414.972329067380088, 220.5265291070639933 ) ) ;
#81184=CARTESIAN_POINT ( 'NONE',  ( 14.27330718989999880, 1474.742293895330022, 225.2716373713979863 ) ) ;
#81187=FACE_OUTER_BOUND ( 'NONE', #46208, .T. ) ;
#81188=CARTESIAN_POINT ( 'NONE',  ( -4.500000000000000000, 1448.210448412289907, 183.1418046154980175 ) ) ;
#81193=CARTESIAN_POINT ( 'NONE',  ( 12.70677192039999959, 1507.773872374229995, 233.3565881929980037 ) ) ;
#81197=DIRECTION ( 'NONE',  ( -0.4875821524125462103, 0.8726613282937071281, 0.02694161742381519925 ) ) ;
#81200=TOROIDAL_SURFACE ( 'NONE', #49025, 8.500000000000000000, 1.500000000000000000 ) ;
#81201=CARTESIAN_POINT ( 'NONE',  ( 0.02695769203707745407, 1409.103991128304187, 232.4957075236154083 ) ) ;
#81207=EDGE_LOOP ( 'NONE', ( #46359, #69588, #10724, #75828, #18228 ) ) ;
#81208=CARTESIAN_POINT ( 'NONE',  ( 5.969073325650000150, 1428.313923095629889, 209.1218459616979999 ) ) ;
#81210=CARTESIAN_POINT ( 'NONE',  ( -11.43740528939994405, 1425.481182534629852, 144.1672625331937923 ) ) ;
#81217=CARTESIAN_POINT ( 'NONE',  ( 5.508554876272072853, 1427.333971811663332, 137.0999999980980135 ) ) ;
#81218=CARTESIAN_POINT ( 'NONE',  ( -0.8327748425420000711, 1442.756953654829886, 150.7628527808980152 ) ) ;
#81221=EDGE_CURVE ( 'NONE', #70446, #28737, #96705, .T. ) ;
#81223=CARTESIAN_POINT ( 'NONE',  ( 0.9855760050558128871, 1450.835604561619903, 181.4318144648370037 ) ) ;
#81224=CARTESIAN_POINT ( 'NONE',  ( -41.15111457195003908, 1443.645559386717878, 136.9181535104192164 ) ) ;
#81225=CARTESIAN_POINT ( 'NONE',  ( -10.03739716579999808, 1408.913060387329779, 223.8190696839980092 ) ) ;
#81226=CARTESIAN_POINT ( 'NONE',  ( 15.24121254350000143, 1417.426114801229915, 227.6809794210979874 ) ) ;
#81229=CARTESIAN_POINT ( 'NONE',  ( 45.48736378840000327, 1434.898499431709979, 266.6954231658979779 ) ) ;
#81230=CARTESIAN_POINT ( 'NONE',  ( -17.72998244229999898, 1409.697166527829950, 224.1509371522980132 ) ) ;
#81231=CARTESIAN_POINT ( 'NONE',  ( 20.10060672000000181, 1435.200054686760041, 143.0090892206980016 ) ) ;
#81232=CARTESIAN_POINT ( 'NONE',  ( -1.120901768300000212, 1420.508728649429941, 228.2469200848979938 ) ) ;
#81233=CARTESIAN_POINT ( 'NONE',  ( 29.75012120190000076, 1509.993914123429931, 209.6841247587719863 ) ) ;
#81235=CARTESIAN_POINT ( 'NONE',  ( 12.27010798620000109, 1416.835808399930102, 223.5795575983979973 ) ) ;
#81237=CARTESIAN_POINT ( 'NONE',  ( -39.66821287261589646, 1439.813157609439941, 136.6894622735260043 ) ) ;
#81238=CARTESIAN_POINT ( 'NONE',  ( 0.2164654389101900167, 1453.731855533950011, 183.2219979431039860 ) ) ;
#81239=CARTESIAN_POINT ( 'NONE',  ( -8.468073032660511146, 1408.680955921970053, 220.2966634368420102 ) ) ;
#81240=CARTESIAN_POINT ( 'NONE',  ( -0.2357814831160000291, 1418.572813431130044, 184.6863074503980044 ) ) ;
#81242=ADVANCED_FACE ( 'NONE', ( #30587 ), #43275, .T. ) ;
#81244=CARTESIAN_POINT ( 'NONE',  ( 11.94131420200000093, 1433.615230264759930, 148.5014726782980006 ) ) ;
#81245=CARTESIAN_POINT ( 'NONE',  ( -35.32500643234939730, 1435.854286985860199, 134.0999999975889807 ) ) ;
#81247=ORIENTED_EDGE ( 'NONE', *, *, #103593, .F. ) ;
#81249=CARTESIAN_POINT ( 'NONE',  ( -7.590886950367840669, 1409.178140000780104, 222.0180217246389986 ) ) ;
#81251=CARTESIAN_POINT ( 'NONE',  ( 18.05542497264820057, 1416.825784014559986, 208.7596466293869923 ) ) ;
#81252=CARTESIAN_POINT ( 'NONE',  ( -14.26885700313499861, 1464.825200350059959, 194.0278458552699874 ) ) ;
#81253=CARTESIAN_POINT ( 'NONE',  ( 26.17821860987093530, 1412.906292311588231, 269.4265852173028861 ) ) ;
#81254=CARTESIAN_POINT ( 'NONE',  ( 19.76254418480000297, 1434.994542537490133, 210.2414884005780209 ) ) ;
#81255=CARTESIAN_POINT ( 'NONE',  ( 20.99191417935101711, 1509.583341918330689, 188.7493953713247663 ) ) ;
#81260=CARTESIAN_POINT ( 'NONE',  ( -29.09134681210840156, 1509.695701326110111, 208.6729072386179951 ) ) ;
#81265=CARTESIAN_POINT ( 'NONE',  ( 2.745142294599053567, 1419.769955103634175, 137.0999999980979567 ) ) ;
#81266=ADVANCED_FACE ( 'NONE', ( #13761 ), #75954, .F. ) ;
#81268=CARTESIAN_POINT ( 'NONE',  ( -12.37159932449999822, 1415.628674266529742, 195.6623782650979990 ) ) ;
#81270=CARTESIAN_POINT ( 'NONE',  ( 22.93207306500000087, 1410.635252800330136, 213.6236024351379967 ) ) ;
#81273=CARTESIAN_POINT ( 'NONE',  ( -5.383700104412980636, 1431.668365950359885, 154.5770934270130113 ) ) ;
#81274=CARTESIAN_POINT ( 'NONE',  ( -11.30340071049999828, 1432.444836995149899, 151.5218617844980145 ) ) ;
#81276=CARTESIAN_POINT ( 'NONE',  ( 27.69051024323239929, 1508.175440098090121, 207.6659959044340269 ) ) ;
#81278=CARTESIAN_POINT ( 'NONE',  ( 25.78167222729700114, 1509.813387082529971, 195.1140727163279962 ) ) ;
#81279=CARTESIAN_POINT ( 'NONE',  ( -1.846469602520000253, 1415.927399473230025, 233.0908749537980214 ) ) ;
#81283=CARTESIAN_POINT ( 'NONE',  ( -11.28228388660000014, 1484.392611670030192, 185.3973464570979957 ) ) ;
#81287=CARTESIAN_POINT ( 'NONE',  ( -4.283151062209100246, 1440.965633392529980, 156.0301116215779871 ) ) ;
#81292=CARTESIAN_POINT ( 'NONE',  ( 28.45308972519999813, 1509.159845678430202, 209.4525048039269848 ) ) ;
#81296=CARTESIAN_POINT ( 'NONE',  ( 15.85018817003589930, 1416.524830770489871, 191.3417815159440067 ) ) ;
#81297=FACE_OUTER_BOUND ( 'NONE', #68683, .T. ) ;
#81299=CARTESIAN_POINT ( 'NONE',  ( -24.69498610859029952, 1451.810891097460171, 137.2013499168999999 ) ) ;
#81301=CARTESIAN_POINT ( 'NONE',  ( 11.95779796459999922, 1409.330635893630188, 227.4564908493979942 ) ) ;
#81304=CARTESIAN_POINT ( 'NONE',  ( 40.49955491180480038, 1447.865363690810000, 134.0999999983799853 ) ) ;
#81305=CARTESIAN_POINT ( 'NONE',  ( -40.17672711025409882, 1442.495956272649892, 136.9880589186049917 ) ) ;
#81307=CARTESIAN_POINT ( 'NONE',  ( 13.80540804498470031, 1434.979597930440150, 148.5369051581390067 ) ) ;
#81310=ORIENTED_EDGE ( 'NONE', *, *, #19177, .T. ) ;
#81313=CARTESIAN_POINT ( 'NONE',  ( 0.3919105056819999766, 1450.899374570899909, 181.2708612515980064 ) ) ;
#81315=CARTESIAN_POINT ( 'NONE',  ( -15.52964687406499955, 1451.324136384999974, 222.4830579234560162 ) ) ;
#81319=CARTESIAN_POINT ( 'NONE',  ( 28.27930517080000072, 1508.150008669530052, 208.9705538469389978 ) ) ;
#81320=CARTESIAN_POINT ( 'NONE',  ( 1.487492019119999842, 1415.934222461130048, 190.4277445559980038 ) ) ;
#81322=ORIENTED_EDGE ( 'NONE', *, *, #30133, .T. ) ;
#81325=CARTESIAN_POINT ( 'NONE',  ( 11.36018337630000019, 1414.996442546230128, 222.2791104318980047 ) ) ;
#81326=CARTESIAN_POINT ( 'NONE',  ( 19.34465229990000168, 1467.203108048530112, 226.8433508900980087 ) ) ;
#81329=CARTESIAN_POINT ( 'NONE',  ( -15.60376662210000198, 1409.457955924729958, 192.7658650750980200 ) ) ;
#81330=DIRECTION ( 'NONE',  ( 0.000000000000000000, 0.000000000000000000, -1.000000000000000000 ) ) ;
#81331=CIRCLE ( 'NONE', #84915, 27.00880975787848470 ) ;
#81333=CARTESIAN_POINT ( 'NONE',  ( 22.53878404599999641, 1411.058442739730026, 206.1986151668880041 ) ) ;
#81335=CARTESIAN_POINT ( 'NONE',  ( 3.426893344479999826, 1406.086097517129929, 266.9564242903979903 ) ) ;
#81336=CARTESIAN_POINT ( 'NONE',  ( -11.87576731660000107, 1433.006546870060220, 147.1501944259979950 ) ) ;
#81337=CARTESIAN_POINT ( 'NONE',  ( 26.73888307210470217, 1505.237121714349769, 206.2308591485389968 ) ) ;
#81338=CARTESIAN_POINT ( 'NONE',  ( 15.72885894491134806, 1409.636817080781157, 192.2423624785494951 ) ) ;
#81339=CARTESIAN_POINT ( 'NONE',  ( -11.60004869885203682, 1423.633889434096545, 135.8155558197614141 ) ) ;
#81343=CARTESIAN_POINT ( 'NONE',  ( -0.1321621631135420083, 1507.857770132879978, 180.7250568012690053 ) ) ;
#81344=CARTESIAN_POINT ( 'NONE',  ( 19.12881724366919300, 1443.878319859672729, 213.6723730806366461 ) ) ;
#81346=CARTESIAN_POINT ( 'NONE',  ( -19.13335938739999875, 1434.810047171619999, 208.8572077783250052 ) ) ;
#81350=CARTESIAN_POINT ( 'NONE',  ( -19.97269067359999895, 1507.847566760029849, 229.1287437625980203 ) ) ;
#81351=CARTESIAN_POINT ( 'NONE',  ( 3.965904004230000002, 1461.348673275530018, 221.5631610770980160 ) ) ;
#81352=CARTESIAN_POINT ( 'NONE',  ( -11.75013601680000086, 1430.854277466529766, 150.6431448726979738 ) ) ;
#81354=CARTESIAN_POINT ( 'NONE',  ( 2.668065388650000092, 1415.928191210829937, 231.9156402769980048 ) ) ;
#81358=FACE_OUTER_BOUND ( 'NONE', #78391, .T. ) ;
#81359=CARTESIAN_POINT ( 'NONE',  ( -21.38271991759999935, 1444.798061961909980, 221.4370072385979995 ) ) ;
#81360=CARTESIAN_POINT ( 'NONE',  ( 5.376760986923570407, 1429.759527328420063, 154.2914800372689967 ) ) ;
#81362=ORIENTED_EDGE ( 'NONE', *, *, #13060, .T. ) ;
#81364=CARTESIAN_POINT ( 'NONE',  ( 0.7690095136829999678, 1406.511333993930066, 269.4984834021980191 ) ) ;
#81367=CARTESIAN_POINT ( 'NONE',  ( 22.31666139102123481, 1430.631687695787832, 217.4689210016930474 ) ) ;
#81368=CARTESIAN_POINT ( 'NONE',  ( -26.33484430150000222, 1451.993449299329768, 134.9650937070979921 ) ) ;
#81369=CARTESIAN_POINT ( 'NONE',  ( 11.60004869885203682, 1425.163358000256721, 137.9635521539829313 ) ) ;
#81370=CARTESIAN_POINT ( 'NONE',  ( -2.501005686574460096, 1448.957422176130194, 154.2481697560310181 ) ) ;
#81371=CARTESIAN_POINT ( 'NONE',  ( -12.42723113640000143, 1446.757544803429937, 187.7007663958980004 ) ) ;
#81372=CARTESIAN_POINT ( 'NONE',  ( -16.75801468479999912, 1408.913060387329779, 215.6757456486180047 ) ) ;
#81375=CARTESIAN_POINT ( 'NONE',  ( -27.19819525569999996, 1434.390360740969982, 248.0989693098979956 ) ) ;
#81377=CARTESIAN_POINT ( 'NONE',  ( 2.500000000000000000, 1439.447172965609980, 162.2861354707980013 ) ) ;
#81378=CARTESIAN_POINT ( 'NONE',  ( -6.194945185159999923, 1475.672627291929984, 267.2191845881980043 ) ) ;
#81383=CARTESIAN_POINT ( 'NONE',  ( -4.095224926770001161, 1416.176064121729951, 162.4091932246979866 ) ) ;
#81388=CARTESIAN_POINT ( 'NONE',  ( -9.624269588760540728, 1396.249147287179994, 214.5727258578990018 ) ) ;
#81389=CARTESIAN_POINT ( 'NONE',  ( -15.20173261459999914, 1421.117185528429900, 227.1213815240980125 ) ) ;
#81390=CARTESIAN_POINT ( 'NONE',  ( 19.71200401973678140, 1455.391961128802677, 226.0432321991784477 ) ) ;
#81392=DIRECTION ( 'NONE',  ( 0.000000000000000000, -1.000000000000000000, 0.000000000000000000 ) ) ;
#81396=CARTESIAN_POINT ( 'NONE',  ( 10.59099531070000033, 1425.359974359930220, 108.0493016666979855 ) ) ;
#81398=DIRECTION ( 'NONE',  ( 0.000000000000000000, 1.000000000000000000, 0.000000000000000000 ) ) ;
#81403=CARTESIAN_POINT ( 'NONE',  ( 3.220346732419999913, 1507.711646624130026, 181.3860254081980088 ) ) ;
#81409=VERTEX_POINT ( 'NONE', #47945 ) ;
#81410=CARTESIAN_POINT ( 'NONE',  ( -11.60590866750000139, 1396.839197833930029, 203.5249495555179919 ) ) ;
#81413=CARTESIAN_POINT ( 'NONE',  ( -12.54683716722921893, 1445.050387070945590, 169.4738468618211016 ) ) ;
#81414=CARTESIAN_POINT ( 'NONE',  ( -15.20522052231627441, 1435.028466183189721, 147.6080187111736279 ) ) ;
#81418=CARTESIAN_POINT ( 'NONE',  ( -1.360143013212020024, 1413.075073688769862, 185.4878003428050022 ) ) ;
#81420=CARTESIAN_POINT ( 'NONE',  ( 13.15671565689999944, 1428.802034784529951, 222.6511392629980151 ) ) ;
#81421=CARTESIAN_POINT ( 'NONE',  ( -40.61865684678500088, 1445.110985547599967, 136.9289262089600072 ) ) ;
#81422=CARTESIAN_POINT ( 'NONE',  ( 9.293729047804200505, 1396.237604587079886, 203.1225184155669865 ) ) ;
#81424=CARTESIAN_POINT ( 'NONE',  ( 11.85151536849999943, 1431.322505881100142, 149.8924761066980125 ) ) ;
#81427=CARTESIAN_POINT ( 'NONE',  ( 3.970410702060000130, 1424.721377522129842, 185.1344166264979947 ) ) ;
#81428=CARTESIAN_POINT ( 'NONE',  ( 12.88731009049999976, 1442.860943865789977, 187.0020155325980227 ) ) ;
#81429=VERTEX_POINT ( 'NONE', #15419 ) ;
#81430=EDGE_LOOP ( 'NONE', ( #11115, #95229, #17616, #7122 ) ) ;
#81431=CARTESIAN_POINT ( 'NONE',  ( -18.78802005810790021, 1468.166114262229939, 227.9520744910329881 ) ) ;
#81433=CARTESIAN_POINT ( 'NONE',  ( -14.45344520480000128, 1470.804162801829989, 194.2860277952979970 ) ) ;
#81437=B_SPLINE_CURVE_WITH_KNOTS ( 'NONE', 5,
 ( #21646, #70044, #55854, #60522, #13247, #19021 ),
 .UNSPECIFIED., .F., .F.,
 ( 6, 6 ),
 ( 0.000000000000000000, 1.000000000000000000 ),
 .UNSPECIFIED. ) ;
#81440=CARTESIAN_POINT ( 'NONE',  ( -11.75444382587980030, 1509.419601378840071, 181.4412948336569968 ) ) ;
#81442=ADVANCED_FACE ( 'NONE', ( #92689 ), #24055, .F. ) ;
#81445=CARTESIAN_POINT ( 'NONE',  ( 18.34777493720000408, 1415.426952350729835, 210.5090058238380095 ) ) ;
#81448=CARTESIAN_POINT ( 'NONE',  ( -19.97269067359999895, 1507.847566760029849, 229.1287437625980203 ) ) ;
#81450=B_SPLINE_SURFACE_WITH_KNOTS ( 'NONE', 5, 5, ( 
 ( #110610, #52388, #69747, #44523, #27166, #1987 ),
 ( #51256, #17620, #18192, #9263, #77572, #61898 ),
 ( #85389, #84837, #34457, #26595, #86508, #18736 ),
 ( #43969, #33892, #879, #68633, #52931, #68088 ),
 ( #87065, #1411, #35003, #51824, #35552, #36122 ),
 ( #26028, #60792, #42866, #85963, #60224, #69182 ),
 ( #103866, #61350, #102200, #70306, #25480, #93782 ),
 ( #8685, #88731, #80328, #45094, #106074, #37221 ),
 ( #29354, #13088, #4174, #104972, #79234, #36668 ),
 ( #63019, #45648, #2543, #11473, #70861, #80876 ),
 ( #20394, #79788, #107168, #30460, #81396, #10919 ),
 ( #3644, #28261, #62455, #4708, #54054, #64645 ),
 ( #72485, #55695, #55147, #89268, #19286, #63555 ),
 ( #96578, #73030, #97670, #54598, #97125, #47273 ),
 ( #19850, #46745, #88181, #3093, #53487, #38851 ),
 ( #28822, #20942, #71418, #87631, #105533, #89816 ),
 ( #12014, #46194, #29900, #12564, #38304, #37773 ),
 ( #71964, #106614, #64092, #98214, #21482, #15296 ),
 ( #65735, #92025, #74141, #32119, #23149, #48943 ),
 ( #91477, #56224, #14756, #99300, #99854, #90916 ),
 ( #90355, #13633, #57352, #83074, #107723, #75242 ),
 ( #75780, #6909, #41065, #24253, #23705, #57889 ),
 ( #66304, #39965, #65188, #41626, #100422, #6367 ),
 ( #15831, #56778, #5263, #49488, #14201, #73594 ) ),
 .UNSPECIFIED., .F., .F., .F.,
 ( 6, 3, 3, 3, 3, 3, 3, 6 ),
 ( 6, 6 ),
 ( 14.55918620569999966, 19.99492494029999889, 25.43066367479999812, 36.30214114399999659, 58.04509608220000416, 73.63322306669999762, 84.29463333639999689, 89.22135005120000528 ),
 ( 0.000000000000000000, 2.069352078150000107 ),
 .UNSPECIFIED. ) ;
#81451=CARTESIAN_POINT ( 'NONE',  ( -39.02150397496387768, 1429.577995707119726, 269.5933091914920396 ) ) ;
#81452=EDGE_CURVE ( 'NONE', #36309, #76907, #44384, .T. ) ;
#81453=CARTESIAN_POINT ( 'NONE',  ( -0.5238648979389999294, 1409.870336987230075, 233.1507188881979857 ) ) ;
#81454=CARTESIAN_POINT ( 'NONE',  ( -10.22570915140000025, 1431.113060387329824, 192.7293421165980192 ) ) ;
#81456=CARTESIAN_POINT ( 'NONE',  ( 2.500000000000000000, 1432.279053890430077, 157.4932346246980046 ) ) ;
#81457=CARTESIAN_POINT ( 'NONE',  ( -32.01195192850000382, 1440.913060389299972, 244.1429064932979998 ) ) ;
#81459=CARTESIAN_POINT ( 'NONE',  ( -0.2199937827443219918, 1465.432054623820250, 236.3155471839449717 ) ) ;
#81460=CARTESIAN_POINT ( 'NONE',  ( 25.76377174109999757, 1414.047232564129899, 270.2932678871979988 ) ) ;
#81463=CARTESIAN_POINT ( 'NONE',  ( 23.41495040159999874, 1410.123695770630093, 208.2164741116880009 ) ) ;
#81464=CARTESIAN_POINT ( 'NONE',  ( 16.14386229810000017, 1410.940818424630152, 209.1133554891810036 ) ) ;
#81466=CONICAL_SURFACE ( 'NONE', #35044, 26.99999999999999645, 0.2186689458740001812 ) ;
#81469=CARTESIAN_POINT ( 'NONE',  ( 4.384104894483219717, 1420.229028528550089, 185.7135937214090120 ) ) ;
#81470=CARTESIAN_POINT ( 'NONE',  ( -0.6386371946080000583, 1415.383004098129959, 233.3563721401980047 ) ) ;
#81475=CARTESIAN_POINT ( 'NONE',  ( 18.64618908219999938, 1416.835809767629826, 209.6841500801740210 ) ) ;
#81476=CARTESIAN_POINT ( 'NONE',  ( 0.4646427325219999460, 1417.292090517329825, 234.8189226518980206 ) ) ;
#81485=CARTESIAN_POINT ( 'NONE',  ( 18.10358820054819873, 1416.830086716310007, 209.0369172249700114 ) ) ;
#81487=CARTESIAN_POINT ( 'NONE',  ( -11.28506483534210147, 1425.468559411955994, 139.1360102533408565 ) ) ;
#81491=ORIENTED_EDGE ( 'NONE', *, *, #105655, .F. ) ;
#81493=CARTESIAN_POINT ( 'NONE',  ( 23.11298832950000204, 1449.418514959970025, 217.9321843291079972 ) ) ;
#81497=CARTESIAN_POINT ( 'NONE',  ( -28.08690426975079646, 1509.893876697129826, 200.8665688467620214 ) ) ;
#81498=CARTESIAN_POINT ( 'NONE',  ( 5.580754349969999417, 1425.065972486529972, 185.9108535249980036 ) ) ;
#81499=CARTESIAN_POINT ( 'NONE',  ( -18.82636944589999928, 1425.197040939629915, 224.5568828730980329 ) ) ;
#81500=CARTESIAN_POINT ( 'NONE',  ( -31.48330081542915337, 1465.654837984586266, 269.3264367229945151 ) ) ;
#81502=CARTESIAN_POINT ( 'NONE',  ( 18.91741685370000070, 1507.874522288630033, 188.5215471660979745 ) ) ;
#81503=CARTESIAN_POINT ( 'NONE',  ( -0.004423692707904589884, 1409.421459607170164, 233.0174416772929931 ) ) ;
#81504=CARTESIAN_POINT ( 'NONE',  ( 29.28982057039999987, 1509.872724133429983, 209.1311963767199700 ) ) ;
#81507=( NAMED_UNIT ( * ) PLANE_ANGLE_UNIT ( ) SI_UNIT ( $, .RADIAN. ) );
#81511=CARTESIAN_POINT ( 'NONE',  ( -4.561655832029999580, 1453.313060387329870, 228.9334036006980000 ) ) ;
#81512=CARTESIAN_POINT ( 'NONE',  ( 1.466938223877110037, 1489.323189782810005, 181.8892042488770073 ) ) ;
#81513=CARTESIAN_POINT ( 'NONE',  ( 0.1439970023041980962, 1408.918088873463375, 231.7716143890593230 ) ) ;
#81514=CARTESIAN_POINT ( 'NONE',  ( -13.21516149639446525, 1444.692096246350502, 186.6006968847816836 ) ) ;
#81517=B_SPLINE_CURVE_WITH_KNOTS ( 'NONE', 5,
 ( #35722, #87803, #69910, #78843, #2154, #36829, #104583, #45807, #26200, #62059, #19459, #53659 ),
 .UNSPECIFIED., .F., .F.,
 ( 6, 3, 3, 6 ),
 ( 0.000000000000000000, 0.3019449542239004969, 0.7424883509937331150, 1.000000000000000000 ),
 .UNSPECIFIED. ) ;
#81520=CARTESIAN_POINT ( 'NONE',  ( 17.60627569411529691, 1410.895669416499913, 224.1775087544040161 ) ) ;
#81521=CIRCLE ( 'NONE', #83294, 1.999999999999998890 ) ;
#81522=CARTESIAN_POINT ( 'NONE',  ( 17.85863899644585473, 1424.390786367949886, 228.2669348674518517 ) ) ;
#81524=CARTESIAN_POINT ( 'NONE',  ( 22.78821502090000095, 1509.414782074829873, 192.0681064721979965 ) ) ;
#81530=CARTESIAN_POINT ( 'NONE',  ( 17.78809123684730054, 1415.431750870129918, 209.6300319562920151 ) ) ;
#81533=CARTESIAN_POINT ( 'NONE',  ( 37.96159890643052393, 1427.824381202910672, 269.5756791377570494 ) ) ;
#81534=CARTESIAN_POINT ( 'NONE',  ( -10.53938673230000056, 1467.231892117930101, 248.5638781414980087 ) ) ;
#81536=CARTESIAN_POINT ( 'NONE',  ( -11.79562278360000072, 1433.595085838450132, 150.7745987806980281 ) ) ;
#81539=CARTESIAN_POINT ( 'NONE',  ( 11.68880576114610115, 1426.727712291149828, 140.7201426135219720 ) ) ;
#81540=CARTESIAN_POINT ( 'NONE',  ( 26.04969316654200284, 1456.961035536420013, 209.5000640554989957 ) ) ;
#81542=CARTESIAN_POINT ( 'NONE',  ( -25.77702438540000074, 1439.619448183560053, 137.8626266291980187 ) ) ;
#81544=CARTESIAN_POINT ( 'NONE',  ( 6.267127390599999792, 1440.453901950489808, 154.5142010626979925 ) ) ;
#81549=CARTESIAN_POINT ( 'NONE',  ( 1.559404887145759819E-08, 1408.124151547700194, 262.7415101742070078 ) ) ;
#81554=CARTESIAN_POINT ( 'NONE',  ( -33.26587534239999400, 1460.596492508030224, 269.9719372418979901 ) ) ;
#81555=CARTESIAN_POINT ( 'NONE',  ( -1.552659050370000182, 1415.628674276829770, 227.5866819053980237 ) ) ;
#81556=FACE_OUTER_BOUND ( 'NONE', #23996, .T. ) ;
#81559=CARTESIAN_POINT ( 'NONE',  ( 0.2936830235118059740, 1451.092918877540114, 182.1143685304440112 ) ) ;
#81560=CARTESIAN_POINT ( 'NONE',  ( -13.99060315449999869, 1420.944189322230159, 227.6471180683980151 ) ) ;
#81561=CARTESIAN_POINT ( 'NONE',  ( 22.52609270013210008, 1509.699688878029974, 227.6602567939980020 ) ) ;
#81564=CARTESIAN_POINT ( 'NONE',  ( -27.08062899747210039, 1413.352696219579911, 269.4117077479539830 ) ) ;
#81566=CARTESIAN_POINT ( 'NONE',  ( -24.34268787264259970, 1442.549328851149994, 212.2035684885649687 ) ) ;
#81567=ORIENTED_EDGE ( 'NONE', *, *, #29645, .F. ) ;
#81568=ORIENTED_EDGE ( 'NONE', *, *, #45962, .T. ) ;
#81570=CARTESIAN_POINT ( 'NONE',  ( 4.794874430321680592, 1423.553857172505786, 184.0667277509072903 ) ) ;
#81571=EDGE_CURVE ( 'NONE', #94948, #59250, #70902, .T. ) ;
#81574=CARTESIAN_POINT ( 'NONE',  ( -17.21788923599999777, 1425.427158435330057, 191.3819988649980246 ) ) ;
#81575=CARTESIAN_POINT ( 'NONE',  ( -2.131094719222661027, 1450.051764141119293, 182.8883510409370956 ) ) ;
#81576=ORIENTED_EDGE ( 'NONE', *, *, #102818, .T. ) ;
#81577=CARTESIAN_POINT ( 'NONE',  ( -26.81198143800000011, 1435.984767782220160, 136.4831820118980090 ) ) ;
#81583=CARTESIAN_POINT ( 'NONE',  ( -42.06230555778069657, 1440.913045005490176, 269.6487386043370407 ) ) ;
#81585=CARTESIAN_POINT ( 'NONE',  ( 0.08248930346060000252, 1397.911842041330146, 196.1221076645980190 ) ) ;
#81589=CARTESIAN_POINT ( 'NONE',  ( 45.63742906433166269, 1440.984662832818231, 268.9747442027135094 ) ) ;
#81590=EDGE_CURVE ( 'NONE', #64454, #59255, #20078, .T. ) ;
#81592=CARTESIAN_POINT ( 'NONE',  ( -2.499989269620250809, 1419.524750234567819, 137.1000002976804808 ) ) ;
#81593=CARTESIAN_POINT ( 'NONE',  ( -2.446860876200000146, 1485.861696305629948, 182.3251189419979994 ) ) ;
#81595=ADVANCED_FACE ( 'NONE', ( #27980 ), #109016, .F. ) ;
#81597=CARTESIAN_POINT ( 'NONE',  ( -18.17797837000000172, 1430.799045000430169, 226.0673535798979970 ) ) ;
#81599=CARTESIAN_POINT ( 'NONE',  ( 11.95789827870000011, 1415.263254644630024, 222.5852371437979969 ) ) ;
#81604=CARTESIAN_POINT ( 'NONE',  ( -36.37832870497099691, 1435.767865672210064, 135.0584844266200264 ) ) ;
#81605=CARTESIAN_POINT ( 'NONE',  ( -22.86910817896174208, 1450.559972649895826, 218.2799029533455553 ) ) ;
#81607=CARTESIAN_POINT ( 'NONE',  ( 7.944299862241802401, 1456.350524190856049, 227.3938853663973987 ) ) ;
#81608=B_SPLINE_CURVE_WITH_KNOTS ( 'NONE', 5,
 ( #24394, #15984, #14340, #101095, #33345, #22722 ),
 .UNSPECIFIED., .F., .F.,
 ( 6, 6 ),
 ( -1.455169987240000129, -1.489991576120175409E-06 ),
 .UNSPECIFIED. ) ;
#81610=CARTESIAN_POINT ( 'NONE',  ( -4.094010558034039349, 1440.293265212250844, 185.3665320917685904 ) ) ;
#81611=CARTESIAN_POINT ( 'NONE',  ( 2.424063131930000115, 1427.257651041929876, 147.9020499575979954 ) ) ;
#81612=CARTESIAN_POINT ( 'NONE',  ( 22.31986392519999995, 1411.050752918829858, 204.7278403729679894 ) ) ;
#81613=CARTESIAN_POINT ( 'NONE',  ( 16.57641946659999732, 1409.993768443630188, 226.3203854516980300 ) ) ;
#81617=CARTESIAN_POINT ( 'NONE',  ( 24.56874431706803819, 1443.565273634055075, 213.1861617392668791 ) ) ;
#81620=EDGE_CURVE ( 'NONE', #47514, #93315, #76513, .T. ) ;
#81621=ORIENTED_EDGE ( 'NONE', *, *, #86568, .T. ) ;
#81626=CARTESIAN_POINT ( 'NONE',  ( -11.58690340151069798, 1425.690683090560015, 133.5559456973340104 ) ) ;
#81627=CARTESIAN_POINT ( 'NONE',  ( -39.43671781166209911, 1447.053669326719955, 136.6351060954069965 ) ) ;
#81628=CARTESIAN_POINT ( 'NONE',  ( 11.60004869885203682, 1426.038537708185913, 137.7598684020179007 ) ) ;
#81629=CARTESIAN_POINT ( 'NONE',  ( 2.647161304830442319, 1417.760379040673342, 233.9115002235340626 ) ) ;
#81630=CARTESIAN_POINT ( 'NONE',  ( -2.500000000000000000, 1420.232870451130111, 149.2693594355980053 ) ) ;
#81633=CARTESIAN_POINT ( 'NONE',  ( 36.81295551165820257, 1440.913060387279984, 254.3033511140860412 ) ) ;
#81635=CARTESIAN_POINT ( 'NONE',  ( -1.600048698852036821, 1411.254281879943164, 137.0999999980979851 ) ) ;
#81639=CARTESIAN_POINT ( 'NONE',  ( -19.08349653902698506, 1485.503699954400417, 189.6259701294393949 ) ) ;
#81641=CARTESIAN_POINT ( 'NONE',  ( 18.46871732690730283, 1509.558002197609767, 190.5444645169020248 ) ) ;
#81642=CARTESIAN_POINT ( 'NONE',  ( 15.05358515032119904, 1410.831827804430077, 191.5175411757069810 ) ) ;
#81646=CARTESIAN_POINT ( 'NONE',  ( -14.69331829855070026, 1452.091493848030041, 222.9975758587799817 ) ) ;
#81647=CARTESIAN_POINT ( 'NONE',  ( -12.84591856360000151, 1434.996842492640098, 194.0990980877979837 ) ) ;
#81649=CARTESIAN_POINT ( 'NONE',  ( 1.713204752390000252, 1465.618698357430276, 235.0090078382979755 ) ) ;
#81650=CARTESIAN_POINT ( 'NONE',  ( -41.66135440509999910, 1443.796918820770088, 135.6885369501979994 ) ) ;
#81651=VERTEX_POINT ( 'NONE', #21751 ) ;
#81652=CARTESIAN_POINT ( 'NONE',  ( -0.5934080169919999648, 1450.964169822730128, 181.9620993427980125 ) ) ;
#81658=EDGE_LOOP ( 'NONE', ( #50744, #63052, #49215, #106110 ) ) ;
#81666=CARTESIAN_POINT ( 'NONE',  ( 11.49168982355860003, 1409.314359038739894, 199.5648683907749898 ) ) ;
#81667=CARTESIAN_POINT ( 'NONE',  ( 18.52259598965499876, 1425.592173059454126, 225.5497999757189973 ) ) ;
#81671=CIRCLE ( 'NONE', #106783, 1.999999961249164571 ) ;
#81672=CARTESIAN_POINT ( 'NONE',  ( -3.766451722194359863, 1450.184391830480081, 184.9593740939260158 ) ) ;
#81674=ORIENTED_EDGE ( 'NONE', *, *, #31669, .F. ) ;
#81676=CARTESIAN_POINT ( 'NONE',  ( -12.20493293955300196, 1416.321686235030029, 194.7273820060790115 ) ) ;
#81677=CARTESIAN_POINT ( 'NONE',  ( -12.58535514000000077, 1434.516889947230084, 149.4256401672980132 ) ) ;
#81680=CARTESIAN_POINT ( 'NONE',  ( -20.03609527204229934, 1489.599509856700024, 190.9186466828699906 ) ) ;
#81685=CARTESIAN_POINT ( 'NONE',  ( -46.05257396074449616, 1440.913065467579827, 266.6769880795539507 ) ) ;
#81691=CARTESIAN_POINT ( 'NONE',  ( 2.658320287279529737, 1408.468079325770077, 222.5002190481939977 ) ) ;
#81692=CARTESIAN_POINT ( 'NONE',  ( -14.08843079593609993, 1436.001885614380171, 150.1056882708590194 ) ) ;
#81695=CARTESIAN_POINT ( 'NONE',  ( 6.772449311907529967, 1425.395680090955921, 226.3226949956692522 ) ) ;
#81697=VERTEX_POINT ( 'NONE', #102337 ) ;
#81698=CARTESIAN_POINT ( 'NONE',  ( 15.89627787559999916, 1415.668893200830098, 250.4785789370980069 ) ) ;
#81699=CARTESIAN_POINT ( 'NONE',  ( -0.8266050234419367593, 1416.818673806272272, 228.0313514088118723 ) ) ;
#81701=CARTESIAN_POINT ( 'NONE',  ( -16.26032719119999825, 1409.480883525030094, 194.9505595544979997 ) ) ;
#81702=CARTESIAN_POINT ( 'NONE',  ( -13.59642666202369199, 1409.123926534358816, 270.0979380971739943 ) ) ;
#81703=CARTESIAN_POINT ( 'NONE',  ( -3.933791733460000106, 1420.650940111930140, 220.7242732661979971 ) ) ;
#81705=EDGE_CURVE ( 'NONE', #102491, #52007, #55640, .T. ) ;
#81706=CARTESIAN_POINT ( 'NONE',  ( -2.467066344142949674, 1452.826908532200150, 152.4293883740839988 ) ) ;
#81707=CARTESIAN_POINT ( 'NONE',  ( 27.42695472179999783, 1451.955572177629847, 134.9063961680979844 ) ) ;
#81709=CARTESIAN_POINT ( 'NONE',  ( -2.500000000000000000, 1419.649642134729902, 147.2763244958979953 ) ) ;
#81711=FACE_OUTER_BOUND ( 'NONE', #3276, .T. ) ;
#81712=ORIENTED_EDGE ( 'NONE', *, *, #58207, .T. ) ;
#81715=CARTESIAN_POINT ( 'NONE',  ( -24.09604921521779985, 1410.858796070480139, 208.7909344980870117 ) ) ;
#81717=ORIENTED_EDGE ( 'NONE', *, *, #11089, .T. ) ;
#81722=CARTESIAN_POINT ( 'NONE',  ( -0.5993188596290000003, 1479.776975780129987, 236.1040631272980193 ) ) ;
#81725=CARTESIAN_POINT ( 'NONE',  ( 46.02990395988660310, 1441.850884208020034, 268.4960837853089970 ) ) ;
#81727=CARTESIAN_POINT ( 'NONE',  ( 0.05691672067130000567, 1419.745815343030017, 184.3817560464979977 ) ) ;
#81729=ORIENTED_EDGE ( 'NONE', *, *, #17484, .F. ) ;
#81731=CARTESIAN_POINT ( 'NONE',  ( 13.10446631662097694, 1443.028365240957783, 187.3795884430450371 ) ) ;
#81738=CARTESIAN_POINT ( 'NONE',  ( 22.23919608084329980, 1452.136450547310005, 140.1164325590560225 ) ) ;
#81739=CARTESIAN_POINT ( 'NONE',  ( -1.700037425840850145E-05, 1408.561147966129965, 270.4290818598980195 ) ) ;
#81743=CARTESIAN_POINT ( 'NONE',  ( -10.97066968179730040, 1432.419134699010101, 151.7701069147389887 ) ) ;
#81744=CARTESIAN_POINT ( 'NONE',  ( 0.02210936670623420836, 1409.026086586376778, 232.3383378967181727 ) ) ;
#81745=CARTESIAN_POINT ( 'NONE',  ( -16.81906092389080243, 1415.724267959580175, 191.6016362877150243 ) ) ;
#81746=CARTESIAN_POINT ( 'NONE',  ( -3.527569048119670203, 1486.518325592330029, 181.8541486797999767 ) ) ;
#81749=CARTESIAN_POINT ( 'NONE',  ( -25.19698811078400169, 1509.685706755500178, 222.8649656611040086 ) ) ;
#81750=EDGE_CURVE ( 'NONE', #69697, #7138, #469, .T. ) ;
#81751=FACE_OUTER_BOUND ( 'NONE', #4381, .T. ) ;
#81752=ORIENTED_EDGE ( 'NONE', *, *, #86662, .T. ) ;
#81754=CARTESIAN_POINT ( 'NONE',  ( -11.73709356416840066, 1426.695943276110029, 144.1748013770919954 ) ) ;
#81758=ADVANCED_FACE ( 'NONE', ( #79370 ), #59912, .F. ) ;
#81764=CARTESIAN_POINT ( 'NONE',  ( -0.8197920095480000224, 1434.541746329560056, 150.4759714514979976 ) ) ;
#81765=CARTESIAN_POINT ( 'NONE',  ( -14.45760372979999886, 1416.831925145830155, 221.3918073827979924 ) ) ;
#81766=CARTESIAN_POINT ( 'NONE',  ( -12.51099982459209947, 1416.825784013739849, 222.1450729932890056 ) ) ;
#81768=CARTESIAN_POINT ( 'NONE',  ( 13.15726444150010011, 1415.434635989099888, 196.8996500771419846 ) ) ;
#81771=CARTESIAN_POINT ( 'NONE',  ( 11.93521150820000010, 1422.099766630330123, 229.5825812192979924 ) ) ;
#81772=B_SPLINE_CURVE_WITH_KNOTS ( 'NONE', 5,
 ( #33407, #41828, #109593, #65956, #24455, #93324, #82732, #42375, #109050 ),
 .UNSPECIFIED., .F., .F.,
 ( 6, 3, 6 ),
 ( -5.629877540799999913, -0.1526127635309997288, 5.629877540799999913 ),
 .UNSPECIFIED. ) ;
#81775=CARTESIAN_POINT ( 'NONE',  ( -18.03030449919999612, 1409.542692494829907, 222.7095495660980191 ) ) ;
#81776=AXIS2_PLACEMENT_3D ( 'NONE', #61993, #45183, #44626 ) ;
#81777=CARTESIAN_POINT ( 'NONE',  ( -0.1664554869000815507, 1508.975239299347777, 238.8734868107800366 ) ) ;
#81778=CARTESIAN_POINT ( 'NONE',  ( 5.389719913101400195, 1440.971386073809981, 154.8246291173960003 ) ) ;
#81779=CARTESIAN_POINT ( 'NONE',  ( -26.53449174420000034, 1450.861614052709911, 136.4341869045979934 ) ) ;
#81780=CARTESIAN_POINT ( 'NONE',  ( 5.360207926212690488, 1422.242713656610022, 144.1549664376839814 ) ) ;
#81783=CARTESIAN_POINT ( 'NONE',  ( -34.74032776987759519, 1437.042396455660082, 136.5358758002960258 ) ) ;
#81784=CARTESIAN_POINT ( 'NONE',  ( -5.808538649209999960, 1415.087797054229895, 225.3799766708980030 ) ) ;
#81786=CARTESIAN_POINT ( 'NONE',  ( -14.66707320740000142, 1409.366313021530004, 207.8310585063279916 ) ) ;
#81790=CARTESIAN_POINT ( 'NONE',  ( 11.94121320300000022, 1433.615332063370033, 149.0256580470980055 ) ) ;
#81791=CARTESIAN_POINT ( 'NONE',  ( -27.70450820019999938, 1435.944202404889893, 136.4829434803980064 ) ) ;
#81792=CARTESIAN_POINT ( 'NONE',  ( 12.53380499169999851, 1442.773887286369927, 186.4115750671979868 ) ) ;
#81797=CARTESIAN_POINT ( 'NONE',  ( -11.29853220753019905, 1409.307613826159923, 218.9138666963339972 ) ) ;
#81799=CARTESIAN_POINT ( 'NONE',  ( -0.6637618131060000204, 1452.913539784329942, 183.3365650660979895 ) ) ;
#81800=CARTESIAN_POINT ( 'NONE',  ( 14.37827720497629969, 1508.124459880479890, 232.6080666346479973 ) ) ;
#81802=CARTESIAN_POINT ( 'NONE',  ( 43.01611365321106462, 1429.412580181660815, 269.0481421394022732 ) ) ;
#81803=CARTESIAN_POINT ( 'NONE',  ( 20.56075711880000156, 1453.152003547730146, 210.2400806596079974 ) ) ;
#81811=CARTESIAN_POINT ( 'NONE',  ( -16.19826984269869996, 1409.504006194269778, 225.4340666559009776 ) ) ;
#81812=CARTESIAN_POINT ( 'NONE',  ( 0.4868008580694940246, 1418.555763684930071, 184.7190794935820293 ) ) ;
#81813=ORIENTED_EDGE ( 'NONE', *, *, #27503, .T. ) ;
#81814=CARTESIAN_POINT ( 'NONE',  ( -13.70773370810000102, 1507.648153709230201, 184.2587369236979953 ) ) ;
#81820=CARTESIAN_POINT ( 'NONE',  ( 22.17406007969999848, 1409.851833609830010, 214.1807298746780077 ) ) ;
#81821=CARTESIAN_POINT ( 'NONE',  ( -2.671470825897180212, 1410.370364388000098, 186.5763473022349785 ) ) ;
#81823=CARTESIAN_POINT ( 'NONE',  ( -18.26676158009999895, 1424.840347090229898, 227.6848214930980134 ) ) ;
#81826=CARTESIAN_POINT ( 'NONE',  ( 23.83757722819380120, 1411.098961242099904, 208.0515134900099952 ) ) ;
#81830=VECTOR ( 'NONE', #87473, 1000.000000000000000 ) ;
#81833=CARTESIAN_POINT ( 'NONE',  ( -6.438481900084330078, 1485.523881333330110, 183.4856451987570267 ) ) ;
#81835=CARTESIAN_POINT ( 'NONE',  ( -4.221673790220910050, 1441.603346299159966, 168.4332526023039804 ) ) ;
#81840=CARTESIAN_POINT ( 'NONE',  ( 29.68011212880000116, 1509.981399006330093, 210.4260893018980312 ) ) ;
#81841=EDGE_LOOP ( 'NONE', ( #90691, #33652, #80600, #1424 ) ) ;
#81845=CARTESIAN_POINT ( 'NONE',  ( -11.69488816318309965, 1426.307070945479836, 141.1954652412310054 ) ) ;
#81846=CARTESIAN_POINT ( 'NONE',  ( 15.68538546202029949, 1410.854151051389863, 191.5168454177849924 ) ) ;
#81849=CARTESIAN_POINT ( 'NONE',  ( -24.80300324625899933, 1451.983833449960002, 136.3302103276260198 ) ) ;
#81850=CARTESIAN_POINT ( 'NONE',  ( -11.73704819359999973, 1426.695975325029849, 144.1715469091980140 ) ) ;
#81851=CARTESIAN_POINT ( 'NONE',  ( 9.159401628690000408, 1409.736190099430132, 229.9419424971980277 ) ) ;
#81853=EDGE_CURVE ( 'NONE', #98070, #18384, #13781, .T. ) ;
#81855=CARTESIAN_POINT ( 'NONE',  ( 41.31139259158630495, 1441.358669516819873, 134.0999999980719792 ) ) ;
#81857=CARTESIAN_POINT ( 'NONE',  ( -26.45259676378333324, 1507.993351259675364, 215.5777749561062819 ) ) ;
#81865=CARTESIAN_POINT ( 'NONE',  ( 0.3125228751849999931, 1450.902146847709901, 181.9094755473980172 ) ) ;
#81866=CARTESIAN_POINT ( 'NONE',  ( -3.324976118279999948, 1484.702107398830094, 183.3515308503979782 ) ) ;
#81867=CARTESIAN_POINT ( 'NONE',  ( -2.500000000000000000, 1439.604493174010031, 166.9187913690360006 ) ) ;
#81869=CARTESIAN_POINT ( 'NONE',  ( -41.65407148426780282, 1444.067059942649848, 136.1145735031259960 ) ) ;
#81870=ADVANCED_FACE ( 'NONE', ( #89415 ), #55285, .F. ) ;
#81874=CARTESIAN_POINT ( 'NONE',  ( 1.387159858850000038, 1415.426952350729835, 190.7740710235979975 ) ) ;
#81880=FACE_OUTER_BOUND ( 'NONE', #55305, .T. ) ;
#81881=CARTESIAN_POINT ( 'NONE',  ( -0.0002459590164598172003, 1452.612215934647338, 153.4544582660230674 ) ) ;
#81883=CARTESIAN_POINT ( 'NONE',  ( 0.06979897883669991532, 1450.915497821400095, 181.2403767522520184 ) ) ;
#81884=CARTESIAN_POINT ( 'NONE',  ( -16.17524367689999920, 1409.477912330530216, 192.6004206005979711 ) ) ;
#81885=FACE_OUTER_BOUND ( 'NONE', #89246, .T. ) ;
#81887=CARTESIAN_POINT ( 'NONE',  ( 22.42329670567509936, 1410.541750806409937, 206.2184894776289923 ) ) ;
#81889=CARTESIAN_POINT ( 'NONE',  ( -2.875659706749999600, 1507.251074149530041, 180.8868938410979865 ) ) ;
#81891=CARTESIAN_POINT ( 'NONE',  ( 26.58595117206280278, 1501.797944955920002, 206.2299323259489938 ) ) ;
#81892=CARTESIAN_POINT ( 'NONE',  ( 15.40417916130000009, 1460.637496422029926, 229.9378244178980140 ) ) ;
#81893=CARTESIAN_POINT ( 'NONE',  ( -11.60004869885203682, 1423.119248846121991, 136.9990639856974894 ) ) ;
#81896=CARTESIAN_POINT ( 'NONE',  ( 0.1595995995380000143, 1486.508831850330125, 181.8147405652979671 ) ) ;
#81898=CARTESIAN_POINT ( 'NONE',  ( 19.03234955206701073, 1444.324475315276004, 213.9789776947724249 ) ) ;
#81900=B_SPLINE_CURVE_WITH_KNOTS ( 'NONE', 3,
 ( #26848, #102980, #85631, #101313, #34142, #69430, #75615, #77264, #61036, #94039, #50414, #8931, #51498, #95157, #34689, #33027, #24605, #52064, #16211, #93480, #16750, #85083, #68879, #60468, #9488, #8372, #68326, #102434, #25718, #59919, #94585, #17865, #43654, #77806, #104103, #3334, #18973, #80011, #54829, #12244, #10604, #36347, #44775, #71093, #97355, #11170, #11703, #96261, #19537, #21167, #2779, #53744 ),
 .UNSPECIFIED., .F., .F.,
 ( 4, 2, 2, 2, 1, 1, 1, 1, 2, 2, 2, 2, 2, 1, 1, 1, 2, 2, 2, 2, 2, 1, 1, 1, 1, 1, 2, 2, 2, 2, 2, 4 ),
 ( 0.000000000000000000, 0.1250000000000079381, 0.1875000000000119071, 0.2187500000000126843, 0.2343750000000130451, 0.2421875000000132672, 0.2460937500000133782, 0.2480468750000134892, 0.2490234375000133782, 0.2500000000000132672, 0.3750000000002221001, 0.4375000000003265721, 0.4687500000003787526, 0.4843750000004061196, 0.4921875000004198863, 0.4960937500004268808, 0.4980468750004303224, 0.5000000000004337641, 0.6250000000005224710, 0.6875000000005676570, 0.7187500000005903056, 0.7343750000006006307, 0.7421875000006051826, 0.7460937500006078471, 0.7480468750006094014, 0.7490234375006091794, 0.7495117187506087353, 0.7500000000006081802, 0.8125000000004561906, 0.8750000000003042011, 0.9375000000001521006, 1.000000000000000000 ),
 .UNSPECIFIED. ) ;
#81901=CARTESIAN_POINT ( 'NONE',  ( 18.61766193520000101, 1509.563203467730091, 187.1480463371979965 ) ) ;
#81905=ORIENTED_EDGE ( 'NONE', *, *, #62608, .T. ) ;
#81908=CARTESIAN_POINT ( 'NONE',  ( -11.30117475489999990, 1432.296176012079741, 151.5220922668979995 ) ) ;
#81911=CARTESIAN_POINT ( 'NONE',  ( 27.02053748618845574, 1451.952524399011281, 135.1690508283753900 ) ) ;
#81912=CARTESIAN_POINT ( 'NONE',  ( -19.21579922906590099, 1443.315308456250023, 209.4908471617739849 ) ) ;
#81914=CARTESIAN_POINT ( 'NONE',  ( 12.50982346350000007, 1445.295918751409999, 187.3223261910979716 ) ) ;
#81915=CARTESIAN_POINT ( 'NONE',  ( -24.42891514760000149, 1457.437613031330102, 213.4851266144380020 ) ) ;
#81916=CARTESIAN_POINT ( 'NONE',  ( -5.347953505379625661, 1422.377634548564401, 137.0999999978673998 ) ) ;
#81917=CARTESIAN_POINT ( 'NONE',  ( 0.1620123089799999916, 1416.817366564930126, 190.8766898493980193 ) ) ;
#81921=CARTESIAN_POINT ( 'NONE',  ( 7.052473882389999282, 1406.463605886129926, 269.0260246300979361 ) ) ;
#81924=CARTESIAN_POINT ( 'NONE',  ( 18.53883420589999886, 1410.877181416130043, 194.4121139098979825 ) ) ;
#81926=CARTESIAN_POINT ( 'NONE',  ( 23.64215237190858332, 1434.207970953952781, 214.6801654245506370 ) ) ;
#81930=CARTESIAN_POINT ( 'NONE',  ( -0.5703798177140180226, 1450.893142285190152, 154.7888451936129854 ) ) ;
#81931=CARTESIAN_POINT ( 'NONE',  ( -1.729960644012338955, 1451.871857846600051, 184.1618444272322108 ) ) ;
#81932=CARTESIAN_POINT ( 'NONE',  ( 2.441038204699999881, 1449.508741055270093, 155.6080914322980107 ) ) ;
#81935=CARTESIAN_POINT ( 'NONE',  ( -36.06124927489999976, 1440.913060387330006, 262.6648722463980334 ) ) ;
#81936=CARTESIAN_POINT ( 'NONE',  ( -27.11938936275100076, 1507.995193792530017, 211.2322906163280152 ) ) ;
#81937=CARTESIAN_POINT ( 'NONE',  ( 2.712833823950000056, 1440.235308908170055, 157.0900337514979981 ) ) ;
#81938=CARTESIAN_POINT ( 'NONE',  ( -4.995145369879999464, 1475.912100276329966, 267.8435508500979836 ) ) ;
#81940=AXIS2_PLACEMENT_3D ( 'NONE', #76900, #103169, #94791 ) ;
#81949=CARTESIAN_POINT ( 'NONE',  ( -21.78142531070000132, 1409.673684521329960, 204.2523482604379694 ) ) ;
#81950=CARTESIAN_POINT ( 'NONE',  ( -15.06420487680200004, 1422.389038249511941, 229.4662359065569888 ) ) ;
#81951=CARTESIAN_POINT ( 'NONE',  ( -43.65584475269999842, 1432.560345650309955, 269.7151603323979998 ) ) ;
#81952=VERTEX_POINT ( 'NONE', #46887 ) ;
#81953=CARTESIAN_POINT ( 'NONE',  ( -11.90018169985392760, 1410.698182860651514, 228.4914053468817201 ) ) ;
#81958=CARTESIAN_POINT ( 'NONE',  ( -0.5000000000076130213, 1448.894380913990062, 155.6080925171820013 ) ) ;
#81970=CARTESIAN_POINT ( 'NONE',  ( -9.292968016810000620, 1396.237577981529967, 201.9577587458279879 ) ) ;
#81971=CARTESIAN_POINT ( 'NONE',  ( -19.78018474210000122, 1409.768243630330062, 220.0095457091979938 ) ) ;
#81972=CARTESIAN_POINT ( 'NONE',  ( -1.499137190340000148, 1414.988017874730076, 226.5174424890980163 ) ) ;
#81973=CARTESIAN_POINT ( 'NONE',  ( -13.26789768477497233, 1444.630613151548005, 169.3822729539114107 ) ) ;
#81977=CARTESIAN_POINT ( 'NONE',  ( 17.68836376279999811, 1413.554570832630134, 224.8857514005979965 ) ) ;
#81978=CARTESIAN_POINT ( 'NONE',  ( 3.793927053430000473, 1429.768419767629894, 185.0899286004980127 ) ) ;
#81980=CARTESIAN_POINT ( 'NONE',  ( -38.43251260839529948, 1449.162497472070072, 136.3062348396100276 ) ) ;
#81982=CARTESIAN_POINT ( 'NONE',  ( 6.667638404474650393, 1396.145899509130004, 200.3161284921849870 ) ) ;
#81983=CARTESIAN_POINT ( 'NONE',  ( 1.547930050009999947, 1416.311719782429918, 190.2897677825980054 ) ) ;
#81984=CARTESIAN_POINT ( 'NONE',  ( 11.75041584140000062, 1430.875550170730094, 150.6471352439980080 ) ) ;
#81991=FACE_OUTER_BOUND ( 'NONE', #69488, .T. ) ;
#82001=CARTESIAN_POINT ( 'NONE',  ( -5.994742217816120267, 1509.255429174939991, 179.4820970290749926 ) ) ;
#82003=EDGE_CURVE ( 'NONE', #69834, #21185, #82959, .T. ) ;
#82005=CARTESIAN_POINT ( 'NONE',  ( 4.912414298609999896, 1414.913060387329779, 224.8486248791979847 ) ) ;
#82009=CARTESIAN_POINT ( 'NONE',  ( -20.35503715340000142, 1509.384884516829743, 229.8737127907980096 ) ) ;
#82010=EDGE_CURVE ( 'NONE', #14771, #50836, #44408, .T. ) ;
#82011=CARTESIAN_POINT ( 'NONE',  ( -35.04504030444321216, 1424.100410869143616, 269.5321305596128809 ) ) ;
#82013=CARTESIAN_POINT ( 'NONE',  ( -1.910180902340000111E-10, 1431.113060387329824, 190.4145386866979948 ) ) ;
#82016=CARTESIAN_POINT ( 'NONE',  ( -30.01782267245550173, 1440.913060386890038, 238.4060211167299883 ) ) ;
#82018=CARTESIAN_POINT ( 'NONE',  ( -0.1948764052599220031, 1466.762775982959965, 235.6169484919890067 ) ) ;
#82020=CARTESIAN_POINT ( 'NONE',  ( 5.207738542198760534, 1410.011340619670136, 270.0726153996189964 ) ) ;
#82023=CARTESIAN_POINT ( 'NONE',  ( 23.26324602400000074, 1409.830269578829984, 208.8206324519090060 ) ) ;
#82032=ORIENTED_EDGE ( 'NONE', *, *, #72558, .F. ) ;
#82034=CARTESIAN_POINT ( 'NONE',  ( -10.10004869885203682, 1422.222932908413441, 135.5999999980979851 ) ) ;
#82035=CARTESIAN_POINT ( 'NONE',  ( 0.8788404816429999933, 1417.051259547929931, 234.0243021844979978 ) ) ;
#82036=DIRECTION ( 'NONE',  ( 0.000000000000000000, -0.7071067811865467956, 0.7071067811865481278 ) ) ;
#82042=CARTESIAN_POINT ( 'NONE',  ( 26.35471571933159751, 1507.985750330240080, 216.6976075425179999 ) ) ;
#82043=CARTESIAN_POINT ( 'NONE',  ( -21.56891552722479943, 1409.666264158969852, 211.8934869078800034 ) ) ;
#82047=CARTESIAN_POINT ( 'NONE',  ( -18.89959486414000267, 1416.839692127460012, 207.5749783441650038 ) ) ;
#82054=CARTESIAN_POINT ( 'NONE',  ( 16.30864140254039896, 1421.541993608423809, 227.2433116674564815 ) ) ;
#82056=CARTESIAN_POINT ( 'NONE',  ( -2.500000000000000000, 1448.555988483530200, 159.6014995286979854 ) ) ;
#82057=CARTESIAN_POINT ( 'NONE',  ( -19.81820729400000403, 1426.896038699130031, 223.1116520403979848 ) ) ;
#82058=CARTESIAN_POINT ( 'NONE',  ( -27.08407403294973292, 1468.437741058713527, 269.4108308351487722 ) ) ;
#82060=CARTESIAN_POINT ( 'NONE',  ( 19.93327782750000310, 1507.860201549930025, 189.0376985353979933 ) ) ;
#82062=CARTESIAN_POINT ( 'NONE',  ( -18.44338626690686667, 1436.494772525281178, 212.9881102422318975 ) ) ;
#82063=CARTESIAN_POINT ( 'NONE',  ( -16.10306942921122797, 1469.090033419330666, 269.3694949584788674 ) ) ;
#82064=ORIENTED_EDGE ( 'NONE', *, *, #22282, .F. ) ;
#82066=CARTESIAN_POINT ( 'NONE',  ( 28.77730036989999718, 1509.917985860129875, 206.0039977793879871 ) ) ;
#82068=CARTESIAN_POINT ( 'NONE',  ( -24.20882931179999886, 1435.739118266630157, 210.8967388383280195 ) ) ;
#82071=CARTESIAN_POINT ( 'NONE',  ( 1.455449434017229926, 1500.378593733119942, 181.4070823815799827 ) ) ;
#82072=CARTESIAN_POINT ( 'NONE',  ( 11.60004869885203682, 1428.983126981193436, 134.0999999980966777 ) ) ;
#82073=CARTESIAN_POINT ( 'NONE',  ( -13.33896809004436790, 1444.529557431482772, 186.7949707955224312 ) ) ;
#82077=CARTESIAN_POINT ( 'NONE',  ( -4.161595075237580765, 1448.982995846620042, 185.0801961897900298 ) ) ;
#82082=( BOUNDED_CURVE ( )  B_SPLINE_CURVE ( 3, ( #54709, #81513, #97228, #53605 ),
 .UNSPECIFIED., .F., .T. ) 
 B_SPLINE_CURVE_WITH_KNOTS ( ( 4, 4 ),
 ( 3.325826778622074986, 4.046911212262204849 ),
 .UNSPECIFIED. ) 
 CURVE ( )  GEOMETRIC_REPRESENTATION_ITEM ( )  RATIONAL_B_SPLINE_CURVE ( ( 1.000000000000000000, 0.9571371180642251897, 0.9571371180642251897, 1.000000000000000000 ) ) 
 REPRESENTATION_ITEM ( '' )  );
#82084=CARTESIAN_POINT ( 'NONE',  ( -14.12346018160000050, 1409.573557975030099, 226.3109121399980097 ) ) ;
#82091=ADVANCED_FACE ( 'NONE', ( #42311 ), #41214, .F. ) ;
#82092=CARTESIAN_POINT ( 'NONE',  ( 17.98384814369790163, 1416.218865267220053, 208.9184880541960183 ) ) ;
#82095=CARTESIAN_POINT ( 'NONE',  ( -33.66409354910000218, 1447.474031025510158, 250.0355534335980110 ) ) ;
#82096=CARTESIAN_POINT ( 'NONE',  ( -20.00014847029999743, 1494.489802793330000, 189.8466569891980100 ) ) ;
#82097=CARTESIAN_POINT ( 'NONE',  ( -11.16957869839999873, 1433.751945839420159, 151.6334640592980065 ) ) ;
#82098=B_SPLINE_CURVE_WITH_KNOTS ( 'NONE', 3,
 ( #19984, #45221, #80461, #63144, #3225, #71551, #36798, #105106, #46331, #70990, #55275, #3774, #61470, #97245, #95596, #28397, #89405, #37907, #18865, #20520, #53062, #87199, #79912, #10491, #2673, #45777, #62597, #54178, #103991, #78803, #54727, #53627, #79359, #12139, #96147, #96714, #37352, #105672, #88855, #12693, #44662, #2118, #72089, #4309, #87769, #36244, #88306, #104550, #106203, #11050 ),
 .UNSPECIFIED., .F., .F.,
 ( 4, 2, 2, 2, 2, 1, 2, 2, 2, 1, 1, 1, 2, 2, 2, 2, 1, 1, 2, 2, 2, 2, 2, 1, 1, 2, 2, 2, 4 ),
 ( 0.000000000000000000, 0.06250000000146122003, 0.09375000000219183005, 0.1250000000029224401, 0.1875000000044818871, 0.2187500000051815496, 0.2343750000056289418, 0.2500000000060763061, 0.3125000000082249763, 0.3437500000092993391, 0.3593750000099265596, 0.3671875000101492703, 0.3710937500102622910, 0.3750000000103753672, 0.4375000000113411502, 0.4687500000119324550, 0.4843750000122225008, 0.4921875000121107568, 0.4960937500120483068, 0.5000000000119858568, 0.5625000000117040821, 0.6250000000114224186, 0.6875000000111406440, 0.7187500000109988685, 0.7343750000110760290, 0.7421875000109645626, 0.7500000000108530962, 0.8750000000054265481, 1.000000000000000000 ),
 .UNSPECIFIED. ) ;
#82100=CARTESIAN_POINT ( 'NONE',  ( 11.73700276280139931, 1426.696010850159837, 144.1682878426319974 ) ) ;
#82103=CARTESIAN_POINT ( 'NONE',  ( -26.91513731259999886, 1437.386455222429959, 136.8516220636979881 ) ) ;
#82106=CARTESIAN_POINT ( 'NONE',  ( 13.15094574255949844, 1428.684587356050088, 223.1532025252389815 ) ) ;
#82108=CARTESIAN_POINT ( 'NONE',  ( -11.21381126459350419, 1509.429652529044688, 236.9473696240944776 ) ) ;
#82109=CARTESIAN_POINT ( 'NONE',  ( 1.547888423906569751E-08, 1407.594100959480102, 263.8350914467960138 ) ) ;
#82112=CARTESIAN_POINT ( 'NONE',  ( -11.86023832827350155, 1431.926758601109896, 149.9669891830439781 ) ) ;
#82114=CARTESIAN_POINT ( 'NONE',  ( -13.22859606919999997, 1471.163352849629973, 270.3663863922980681 ) ) ;
#82117=CARTESIAN_POINT ( 'NONE',  ( 35.94911020107750232, 1451.437441929419947, 135.1301813102820120 ) ) ;
#82118=CARTESIAN_POINT ( 'NONE',  ( 0.2184868517783540021, 1451.777963835670107, 182.9107317036869915 ) ) ;
#82123=CARTESIAN_POINT ( 'NONE',  ( -41.97207030135130168, 1426.354619028159959, 266.5340502157400238 ) ) ;
#82124=ORIENTED_EDGE ( 'NONE', *, *, #105655, .T. ) ;
#82125=CARTESIAN_POINT ( 'NONE',  ( -24.44537314746287393, 1442.730589020610978, 210.9654079490763650 ) ) ;
#82130=CARTESIAN_POINT ( 'NONE',  ( 4.906730394725735245, 1423.390749761640336, 184.2167557326281440 ) ) ;
#82133=CARTESIAN_POINT ( 'NONE',  ( -15.67917309240000279, 1455.451896433330148, 188.9440702688980025 ) ) ;
#82135=CARTESIAN_POINT ( 'NONE',  ( -18.26532265589999682, 1415.628674266529742, 208.3526068587169959 ) ) ;
#82136=B_SPLINE_SURFACE_WITH_KNOTS ( 'NONE', 5, 1, ( 
 ( #85206, #42668 ),
 ( #76824, #139 ),
 ( #44903, #10731 ),
 ( #79051, #97479 ),
 ( #20208, #63364 ),
 ( #37574, #2353 ),
 ( #38118, #71211 ),
 ( #29715, #2898 ),
 ( #54945, #89072 ) ),
 .UNSPECIFIED., .F., .F., .F.,
 ( 6, 3, 6 ),
 ( 2, 2 ),
 ( -1.085177091614590055E-05, 35.35713585580000284, 84.36278594678920228 ),
 ( 2.018291180219999870, 3.029423978413739782 ),
 .UNSPECIFIED. ) ;
#82138=CARTESIAN_POINT ( 'NONE',  ( -26.80348844950000142, 1436.439654078439844, 136.7215874007980005 ) ) ;
#82144=CARTESIAN_POINT ( 'NONE',  ( -35.38898509910070089, 1419.603228493539973, 269.8627298453310459 ) ) ;
#82146=CARTESIAN_POINT ( 'NONE',  ( -3.841870597909999852, 1398.027800385929822, 196.5971685358980210 ) ) ;
#82150=CARTESIAN_POINT ( 'NONE',  ( 0.3919059719699999889, 1450.899374729219971, 181.2708615468980042 ) ) ;
#82153=CARTESIAN_POINT ( 'NONE',  ( -13.28075528932130212, 1436.102060238340073, 150.6141327710369922 ) ) ;
#82154=CARTESIAN_POINT ( 'NONE',  ( -0.03626856688976699827, 1409.963246368600039, 185.0759526402830204 ) ) ;
#82155=AXIS2_PLACEMENT_3D ( 'NONE', #31101, #79871, #98306 ) ;
#82158=CARTESIAN_POINT ( 'NONE',  ( -18.20274223739999897, 1435.778903725820101, 226.4112149876980027 ) ) ;
#82163=EDGE_LOOP ( 'NONE', ( #40592, #102197, #26557, #71174 ) ) ;
#82165=CARTESIAN_POINT ( 'NONE',  ( -11.59417537721629898, 1428.981093291590014, 133.6116858579929954 ) ) ;
#82166=CARTESIAN_POINT ( 'NONE',  ( -23.74203090515832315, 1447.138914774234763, 214.4317863515268527 ) ) ;
#82167=ORIENTED_EDGE ( 'NONE', *, *, #9021, .F. ) ;
#82168=CARTESIAN_POINT ( 'NONE',  ( 9.932046507237075161, 1455.482931264669332, 226.5863170123957957 ) ) ;
#82170=CARTESIAN_POINT ( 'NONE',  ( -4.127455358014529452, 1439.932934338472933, 185.4683297619992288 ) ) ;
#82171=CARTESIAN_POINT ( 'NONE',  ( -2.920887357330470113, 1416.480278474030001, 186.3404578197399815 ) ) ;
#82172=CARTESIAN_POINT ( 'NONE',  ( 21.06805239210000380, 1409.648772995130003, 203.5068327927779990 ) ) ;
#82176=CARTESIAN_POINT ( 'NONE',  ( 4.248370253470151070, 1441.364699327820063, 161.3861545211829878 ) ) ;
#82179=DIRECTION ( 'NONE',  ( 0.000000000000000000, 1.000000000000000000, 0.000000000000000000 ) ) ;
#82180=CARTESIAN_POINT ( 'NONE',  ( -3.955028505459999653E-16, 1420.349145488430167, 170.8340916043979973 ) ) ;
#82186=CARTESIAN_POINT ( 'NONE',  ( 1.931781262533000117E-14, 1421.852997280460158, 133.5964121027310227 ) ) ;
#82188=CARTESIAN_POINT ( 'NONE',  ( 11.60004869885203682, 1426.444849425687153, 138.8727431505155323 ) ) ;
#82189=AXIS2_PLACEMENT_3D ( 'NONE', #64631, #105095, #10480 ) ;
#82190=CARTESIAN_POINT ( 'NONE',  ( -2.146337792930170352, 1464.869601414239924, 183.9517861855029821 ) ) ;
#82192=CARTESIAN_POINT ( 'NONE',  ( 31.68651911954009748, 1440.913060383499896, 243.2846231541469990 ) ) ;
#82199=B_SPLINE_CURVE_WITH_KNOTS ( 'NONE', 3,
 ( #91595, #66966, #82650, #5941, #14871, #66423, #49062, #75900, #6486, #108397, #75367, #8129, #40087, #40638, #7038, #107841, #83742, #74810, #24910, #41196, #109506, #67521, #92688, #59119, #31680, #93242, #101076, #15965, #31130, #32242, #65862, #16508, #100538, #65312, #23818, #99425, #26587, #61342, #96007, #68078, #43413, #87055, #18725, #86498, #42857, #78102, #70298, #102191, #69174, #27704 ),
 .UNSPECIFIED., .F., .F.,
 ( 4, 2, 2, 2, 2, 1, 2, 2, 2, 1, 1, 1, 2, 2, 2, 2, 1, 1, 2, 2, 2, 2, 2, 1, 1, 2, 2, 2, 4 ),
 ( 0.000000000000000000, 0.06249999999685171281, 0.09374999999528567385, 0.1249999999937196349, 0.1874999999906944714, 0.2187499999891768243, 0.2343749999883256441, 0.2499999999874744638, 0.3124999999842543175, 0.3437499999827312580, 0.3593749999820591845, 0.3671874999817218432, 0.3710937499815532004, 0.3749999999813845020, 0.4374999999794075278, 0.4687499999785326721, 0.4843749999780995186, 0.4921874999781875037, 0.4960937499782315796, 0.4999999999782755999, 0.5624999999801301165, 0.6249999999819845220, 0.6874999999838390385, 0.7187499999849091825, 0.7343749999852986488, 0.7421874999854947141, 0.7499999999856906685, 0.8749999999928452787, 1.000000000000000000 ),
 .UNSPECIFIED. ) ;
#82209=CARTESIAN_POINT ( 'NONE',  ( -14.56367227959999866, 1489.468502498129965, 192.4084369560980008 ) ) ;
#82211=CARTESIAN_POINT ( 'NONE',  ( 1.412514030800000153, 1466.019513801129960, 235.1197556243980102 ) ) ;
#82214=ORIENTED_EDGE ( 'NONE', *, *, #82993, .T. ) ;
#82215=CARTESIAN_POINT ( 'NONE',  ( -0.6413666067069999643, 1451.453725705629950, 182.8474195845979864 ) ) ;
#82220=CARTESIAN_POINT ( 'NONE',  ( -16.93235272047269646, 1414.913060387399810, 207.4470167978099937 ) ) ;
#82221=ORIENTED_EDGE ( 'NONE', *, *, #66087, .F. ) ;
#82224=EDGE_CURVE ( 'NONE', #110603, #70446, #5416, .T. ) ;
#82230=VECTOR ( 'NONE', #28854, 1000.000000000000000 ) ;
#82232=ADVANCED_FACE ( 'NONE', ( #52395 ), #60839, .F. ) ;
#82235=CARTESIAN_POINT ( 'NONE',  ( 20.61516490012983027, 1509.679647908174275, 187.6627224229067394 ) ) ;
#82236=CARTESIAN_POINT ( 'NONE',  ( 8.791545081663338479, 1409.220067906589748, 197.0144757566580154 ) ) ;
#82237=CARTESIAN_POINT ( 'NONE',  ( 18.12291530770000136, 1425.086651382430091, 225.0935702407979875 ) ) ;
#82238=CARTESIAN_POINT ( 'NONE',  ( 0.8259447189419999447, 1418.827400219930041, 184.7842358559980198 ) ) ;
#82239=CARTESIAN_POINT ( 'NONE',  ( -19.59136418880000008, 1478.168253370030016, 190.6957923982980105 ) ) ;
#82242=CARTESIAN_POINT ( 'NONE',  ( -2.468912052060390216, 1449.613523094110178, 183.5976281201020015 ) ) ;
#82247=CARTESIAN_POINT ( 'NONE',  ( 19.76289411957749564, 1455.644449270149835, 227.1109336957369749 ) ) ;
#82248=CARTESIAN_POINT ( 'NONE',  ( -12.68266539220000055, 1434.593723365520191, 149.3604887061979696 ) ) ;
#82250=CARTESIAN_POINT ( 'NONE',  ( -20.30854934916089860, 1498.424519700439987, 190.6632691037499967 ) ) ;
#82251=LINE ( 'NONE', #6647, #26836 ) ;
#82253=EDGE_CURVE ( 'NONE', #54360, #2110, #25501, .T. ) ;
#82256=CARTESIAN_POINT ( 'NONE',  ( -46.15241011806139682, 1440.697464424330065, 268.2044778594760146 ) ) ;
#82257=CARTESIAN_POINT ( 'NONE',  ( -18.96495392289999771, 1425.684290752429888, 226.5179610041979856 ) ) ;
#82262=CARTESIAN_POINT ( 'NONE',  ( 1.286193012929579993, 1407.887988129029736, 222.3093619251160362 ) ) ;
#82263=CARTESIAN_POINT ( 'NONE',  ( -13.42438607818310103, 1436.022353700810072, 150.5143652916869996 ) ) ;
#82265=B_SPLINE_SURFACE_WITH_KNOTS ( 'NONE', 4, 5, ( 
 ( #47471, #81593, #108467, #106264, #55883, #6005 ),
 ( #31200, #56979, #4897, #97848, #98950, #55329 ),
 ( #64284, #31750, #22224, #89462, #14387, #74339 ),
 ( #57537, #98406, #91661, #46388, #37965, #110118 ),
 ( #40709, #109574, #33390, #26523, #7653, #36054 ) ),
 .UNSPECIFIED., .F., .F., .F.,
 ( 5, 5 ),
 ( 6, 6 ),
 ( 1.756953143920000127, 12.62047352739999972 ),
 ( 0.000000000000000000, 2.000000106069999894 ),
 .UNSPECIFIED. ) ;
#82266=CARTESIAN_POINT ( 'NONE',  ( 2.755131347899999916, 1422.216165794629887, 90.98709265669789659 ) ) ;
#82270=CARTESIAN_POINT ( 'NONE',  ( 15.47923624419999911, 1416.261629425730007, 248.5133305092979867 ) ) ;
#82271=CARTESIAN_POINT ( 'NONE',  ( -24.29269244670000205, 1508.123907548630086, 196.8922397913979978 ) ) ;
#82272=CARTESIAN_POINT ( 'NONE',  ( -0.4682527189540000023, 1458.406866031629988, 182.9037998423980014 ) ) ;
#82273=DIRECTION ( 'NONE',  ( 1.000000000000000000, 0.000000000000000000, 0.000000000000000000 ) ) ;
#82274=CARTESIAN_POINT ( 'NONE',  ( 17.27558691658489920, 1507.606285602530079, 193.9884222186300065 ) ) ;
#82276=CARTESIAN_POINT ( 'NONE',  ( -24.57380889490000087, 1432.446761552710086, 225.2495674893980038 ) ) ;
#82277=CARTESIAN_POINT ( 'NONE',  ( -29.51415835736623450, 1509.963286984361730, 206.5299505428056932 ) ) ;
#82278=CARTESIAN_POINT ( 'NONE',  ( -0.02516806119179999801, 1415.404723302029879, 233.4400559027980080 ) ) ;
#82279=CARTESIAN_POINT ( 'NONE',  ( 27.84003805790000285, 1450.652436793030120, 136.4235866663979948 ) ) ;
#82280=ORIENTED_EDGE ( 'NONE', *, *, #57744, .F. ) ;
#82283=CARTESIAN_POINT ( 'NONE',  ( 13.18359814959999987, 1420.070066474529995, 228.9875191970980097 ) ) ;
#82288=CARTESIAN_POINT ( 'NONE',  ( -23.60926278007800150, 1410.014349673999959, 209.1215866734690110 ) ) ;
#82289=ORIENTED_EDGE ( 'NONE', *, *, #12720, .F. ) ;
#82292=CARTESIAN_POINT ( 'NONE',  ( -22.29678302319670280, 1436.505994161930857, 142.6647499578515976 ) ) ;
#82293=ADVANCED_FACE ( 'NONE', ( #102073 ), #16396, .T. ) ;
#82295=ORIENTED_EDGE ( 'NONE', *, *, #35229, .F. ) ;
#82296=CARTESIAN_POINT ( 'NONE',  ( 44.76515501619800119, 1450.021284846529852, 267.6430847853379760 ) ) ;
#82297=CARTESIAN_POINT ( 'NONE',  ( -12.48769551256209986, 1414.971717244350202, 220.5819595087910159 ) ) ;
#82298=ADVANCED_FACE ( 'NONE', ( #8020 ), #18068, .F. ) ;
#82299=CARTESIAN_POINT ( 'NONE',  ( -0.06475640353809999916, 1420.445361017130153, 182.6808671977979941 ) ) ;
#82304=CARTESIAN_POINT ( 'NONE',  ( 13.44976921669219649, 1443.526213651251965, 187.9650672106725722 ) ) ;
#82305=ORIENTED_EDGE ( 'NONE', *, *, #102675, .F. ) ;
#82310=CARTESIAN_POINT ( 'NONE',  ( 7.678176981006109791, 1452.644932538870080, 151.4245570955009725 ) ) ;
#82317=CARTESIAN_POINT ( 'NONE',  ( 15.86840223659999616, 1489.480617680030036, 194.0918035215979955 ) ) ;
#82321=CARTESIAN_POINT ( 'NONE',  ( 7.235185706049999332, 1427.271387135730038, 145.8323558008980001 ) ) ;
#82325=DIRECTION ( 'NONE',  ( 0.000000000000000000, 0.000000000000000000, -1.000000000000000000 ) ) ;
#82330=ORIENTED_EDGE ( 'NONE', *, *, #83792, .F. ) ;
#82333=EDGE_CURVE ( 'NONE', #109428, #70222, #34759, .T. ) ;
#82335=CARTESIAN_POINT ( 'NONE',  ( 11.93269758809999992, 1433.544831721110086, 150.2289606549979908 ) ) ;
#82336=CARTESIAN_POINT ( 'NONE',  ( 13.66603629819999810, 1471.441739209529942, 271.1218459616979999 ) ) ;
#82337=CARTESIAN_POINT ( 'NONE',  ( 0.7971436909562600315, 1450.873242978859935, 181.3626938088150098 ) ) ;
#82341=CARTESIAN_POINT ( 'NONE',  ( -15.96958168569999970, 1519.913060387329779, 225.0914276473980067 ) ) ;
#82342=CARTESIAN_POINT ( 'NONE',  ( 16.53726887470000051, 1419.770721813829823, 227.0156051753980080 ) ) ;
#82346=CARTESIAN_POINT ( 'NONE',  ( -16.85751496860000032, 1409.501737783529961, 224.7669409504980251 ) ) ;
#82348=CARTESIAN_POINT ( 'NONE',  ( -0.5656601615979999220, 1424.194575837329921, 228.0927458394980079 ) ) ;
#82351=CARTESIAN_POINT ( 'NONE',  ( 12.72965180529999962, 1416.819760301830001, 223.1305968146979808 ) ) ;
#82354=CARTESIAN_POINT ( 'NONE',  ( -7.758455216056949766, 1432.346375745089972, 153.7650376895189765 ) ) ;
#82355=CARTESIAN_POINT ( 'NONE',  ( -3.949231543599999394, 1416.520322351229879, 227.3109020079980098 ) ) ;
#82356=CARTESIAN_POINT ( 'NONE',  ( 0.2159072697397970142, 1454.042348015329935, 183.2086788371790078 ) ) ;
#82357=CARTESIAN_POINT ( 'NONE',  ( -13.37628687016149875, 1408.062381179059912, 207.9480605954729810 ) ) ;
#82358=CARTESIAN_POINT ( 'NONE',  ( -15.98493104980000190, 1416.216252248729916, 200.6524258963880243 ) ) ;
#82362=CARTESIAN_POINT ( 'NONE',  ( 13.50126846350000065, 1434.968978322849807, 147.6247934473980195 ) ) ;
#82363=CARTESIAN_POINT ( 'NONE',  ( -35.92423077455959657, 1436.007692230529983, 134.0999999972619889 ) ) ;
#82371=EDGE_CURVE ( 'NONE', #45409, #21233, #60170, .T. ) ;
#82372=CARTESIAN_POINT ( 'NONE',  ( 13.87457611739909957, 1508.109622702359957, 232.8490349609430154 ) ) ;
#82373=CARTESIAN_POINT ( 'NONE',  ( 40.50178695588397204, 1425.153962140106159, 269.1155952481692566 ) ) ;
#82376=CARTESIAN_POINT ( 'NONE',  ( 3.418717339140000089, 1426.008825657230091, 185.1440916679979978 ) ) ;
#82380=CARTESIAN_POINT ( 'NONE',  ( -27.77560428830000205, 1450.655010635179906, 136.4259719682980005 ) ) ;
#82382=EDGE_CURVE ( 'NONE', #28184, #28853, #1459, .T. ) ;
#82383=CARTESIAN_POINT ( 'NONE',  ( -16.02269354968879966, 1410.117710933159969, 226.4951371525800141 ) ) ;
#82384=CARTESIAN_POINT ( 'NONE',  ( 0.4957976563827369842, 1415.716230218539977, 184.8406531014170184 ) ) ;
#82385=ORIENTED_EDGE ( 'NONE', *, *, #110402, .F. ) ;
#82390=CARTESIAN_POINT ( 'NONE',  ( -0.2309819874101929904, 1419.229592309189911, 184.5617884385680156 ) ) ;
#82392=CARTESIAN_POINT ( 'NONE',  ( 0.2895612746910000146, 1465.119060462830021, 238.1348910625980011 ) ) ;
#82393=CARTESIAN_POINT ( 'NONE',  ( 21.39553055000000015, 1411.020667844629997, 217.4763728266080136 ) ) ;
#82394=B_SPLINE_SURFACE_WITH_KNOTS ( 'NONE', 5, 5, ( 
 ( #20792, #12405, #55536, #46590, #4033, #38161 ),
 ( #89661, #12947, #81254, #4569, #72879, #30304 ),
 ( #64495, #47674, #81803, #73434, #107567, #65029 ),
 ( #22425, #100802, #68353, #109778, #36, #40357 ),
 ( #58827, #24092, #58280, #92965, #14602, #74538 ),
 ( #76174, #42572, #16237, #82914, #7315, #25746 ) ),
 .UNSPECIFIED., .F., .F., .F.,
 ( 6, 6 ),
 ( 6, 6 ),
 ( 29.52656374800000094, 158.0439293190000001 ),
 ( -2.775557561569999727E-17, 1.000000000000000000 ),
 .UNSPECIFIED. ) ;
#82395=CARTESIAN_POINT ( 'NONE',  ( 0.5105443137851592983, 1450.895231787036892, 181.2859576932934829 ) ) ;
#82397=CARTESIAN_POINT ( 'NONE',  ( -16.17440652799999867, 1423.017051802529977, 229.3744292183979780 ) ) ;
#82399=CARTESIAN_POINT ( 'NONE',  ( 3.835404308830561160, 1412.913060387329779, 216.1425064568153687 ) ) ;
#82400=CARTESIAN_POINT ( 'NONE',  ( 24.91361133721389720, 1430.502641194839725, 209.5701750418959932 ) ) ;
#82402=CARTESIAN_POINT ( 'NONE',  ( 14.45750538832999865, 1416.828039266780024, 196.8520486936070029 ) ) ;
#82408=ORIENTED_EDGE ( 'NONE', *, *, #65942, .T. ) ;
#82412=CARTESIAN_POINT ( 'NONE',  ( -4.222081761889490359, 1441.600097058339998, 170.2277829678710077 ) ) ;
#82414=ORIENTED_EDGE ( 'NONE', *, *, #19428, .F. ) ;
#82415=ORIENTED_EDGE ( 'NONE', *, *, #95243, .T. ) ;
#82420=CARTESIAN_POINT ( 'NONE',  ( -11.74440294555880193, 1426.691427119352511, 144.6990483903438758 ) ) ;
#82421=CARTESIAN_POINT ( 'NONE',  ( 15.91660703430019730, 1409.850593835830068, 191.9602275961530040 ) ) ;
#82424=CARTESIAN_POINT ( 'NONE',  ( 2.935740384309999840, 1409.954265578529885, 231.6094181485979959 ) ) ;
#82427=CARTESIAN_POINT ( 'NONE',  ( 39.19204896952249584, 1449.501219045310108, 134.0999999980739688 ) ) ;
#82429=CARTESIAN_POINT ( 'NONE',  ( -39.59829837890580251, 1440.706476837099899, 136.7973020598680023 ) ) ;
#82431=CARTESIAN_POINT ( 'NONE',  ( -18.12714478550000052, 1457.846702312930120, 228.5127547687980041 ) ) ;
#82432=ORIENTED_EDGE ( 'NONE', *, *, #40680, .F. ) ;
#82437=CARTESIAN_POINT ( 'NONE',  ( -3.174083179560000190, 1485.815246478130121, 182.5712446315979776 ) ) ;
#82438=CARTESIAN_POINT ( 'NONE',  ( -2.500000000000000000, 1439.559074768590108, 165.1937480901340223 ) ) ;
#82439=CARTESIAN_POINT ( 'NONE',  ( -27.56049296109999958, 1508.045672656129909, 205.3679835307079884 ) ) ;
#82440=CARTESIAN_POINT ( 'NONE',  ( 33.91369111058539687, 1435.681798630800131, 135.0591074393149711 ) ) ;
#82443=CARTESIAN_POINT ( 'NONE',  ( 1.075905130380000019, 1414.913060387329779, 191.8484598369979892 ) ) ;
#82450=CARTESIAN_POINT ( 'NONE',  ( 34.63479025869150263, 1440.913060387330006, 260.2959212809009841 ) ) ;
#82452=CARTESIAN_POINT ( 'NONE',  ( -0.001699438796131666181, 1451.847275359585637, 154.0281730256439232 ) ) ;
#82454=CARTESIAN_POINT ( 'NONE',  ( 0.009324443903248720578, 1452.355234467360106, 183.2662222589769954 ) ) ;
#82458=CARTESIAN_POINT ( 'NONE',  ( -13.02607830360000030, 1426.053423478829927, 222.2684508982979992 ) ) ;
#82459=CARTESIAN_POINT ( 'NONE',  ( -20.15452302159999931, 1507.845791376729949, 228.9024215066979764 ) ) ;
#82460=CARTESIAN_POINT ( 'NONE',  ( -1.493215638020000124, 1507.691765935529929, 180.8029183418980210 ) ) ;
#82461=CARTESIAN_POINT ( 'NONE',  ( -11.87968386989999914, 1433.311128018820000, 147.1501983835979956 ) ) ;
#82463=CARTESIAN_POINT ( 'NONE',  ( 12.53348523240000034, 1462.451547715029847, 231.4893851574979919 ) ) ;
#82464=CARTESIAN_POINT ( 'NONE',  ( -10.47364140659463949, 1423.539562070946204, 137.3343660864095170 ) ) ;
#82465=CARTESIAN_POINT ( 'NONE',  ( 6.690593169671610774, 1474.175173204296698, 270.1377431963427966 ) ) ;
#82467=ORIENTED_EDGE ( 'NONE', *, *, #52467, .F. ) ;
#82468=CARTESIAN_POINT ( 'NONE',  ( -0.5206041912694210350, 1486.385752493620203, 181.7753473960027577 ) ) ;
#82469=CARTESIAN_POINT ( 'NONE',  ( -0.1467532245951940206, 1507.559297430280139, 180.8320577633109849 ) ) ;
#82470=CARTESIAN_POINT ( 'NONE',  ( 19.12310882341182250, 1443.904899534319838, 213.6905610154896635 ) ) ;
#82472=CARTESIAN_POINT ( 'NONE',  ( 18.58455362259999788, 1509.562047300529912, 186.5314039206980112 ) ) ;
#82478=CARTESIAN_POINT ( 'NONE',  ( -11.28505919290000037, 1431.090797829909889, 151.4130702670979929 ) ) ;
#82481=CARTESIAN_POINT ( 'NONE',  ( -7.105422403163559973E-15, 1425.409940805969882, 153.8890955463500063 ) ) ;
#82483=CARTESIAN_POINT ( 'NONE',  ( 12.77839545800000032, 1445.090219591050072, 187.3316831286979891 ) ) ;
#82484=CARTESIAN_POINT ( 'NONE',  ( -19.02423469520000054, 1444.806343971380102, 225.8304661078979905 ) ) ;
#82486=CARTESIAN_POINT ( 'NONE',  ( 0.04536310491940000189, 1416.820969729830040, 190.9583658068980014 ) ) ;
#82489=CARTESIAN_POINT ( 'NONE',  ( 9.928099361890000196, 1406.542887612530194, 268.4433879007979726 ) ) ;
#82491=CARTESIAN_POINT ( 'NONE',  ( 0.4960545405569999899, 1409.436441302029834, 185.2773262721979961 ) ) ;
#82492=CARTESIAN_POINT ( 'NONE',  ( 17.94874957400000071, 1410.880404130830129, 193.3864771145979944 ) ) ;
#82493=CARTESIAN_POINT ( 'NONE',  ( 22.42926025653192923, 1430.882581194299291, 217.2517530083725603 ) ) ;
#82494=CARTESIAN_POINT ( 'NONE',  ( -24.00529210049999662, 1452.074773682930072, 136.6368758670979844 ) ) ;
#82495=CARTESIAN_POINT ( 'NONE',  ( 28.07231212390000152, 1508.101920094730076, 210.4687657402579930 ) ) ;
#82497=CARTESIAN_POINT ( 'NONE',  ( -2.496316867461920275, 1449.223786180559955, 155.0643152763460080 ) ) ;
#82498=CARTESIAN_POINT ( 'NONE',  ( -12.50186341110000043, 1445.154755434839899, 186.4456158379979911 ) ) ;
#82499=ADVANCED_FACE ( 'NONE', ( #101235 ), #17856, .T. ) ;
#82500=CARTESIAN_POINT ( 'NONE',  ( -19.79527383844874677, 1485.865817549667554, 190.3272490650382451 ) ) ;
#82501=CARTESIAN_POINT ( 'NONE',  ( -14.39446395563320102, 1416.321686235100060, 221.3267789012660103 ) ) ;
#82504=B_SPLINE_CURVE_WITH_KNOTS ( 'NONE', 3,
 ( #63426, #104843, #10791, #35991 ),
 .UNSPECIFIED., .F., .F.,
 ( 4, 4 ),
 ( 0.000000000000000000, 1.000000000000000000 ),
 .UNSPECIFIED. ) ;
#82506=CARTESIAN_POINT ( 'NONE',  ( 20.53373630228941593, 1507.794800605937780, 228.2241611779419088 ) ) ;
#82507=EDGE_CURVE ( 'NONE', #94989, #97932, #76595, .T. ) ;
#82508=CARTESIAN_POINT ( 'NONE',  ( 3.659274215279999964, 1441.479476129459954, 165.0935548642979995 ) ) ;
#82509=AXIS2_PLACEMENT_3D ( 'NONE', #18435, #60489, #50435 ) ;
#82510=CARTESIAN_POINT ( 'NONE',  ( -1.775122301699999960, 1475.958576172530002, 267.2336942637979860 ) ) ;
#82511=CARTESIAN_POINT ( 'NONE',  ( -10.73010380666730690, 1424.980364244693419, 138.6337414485319641 ) ) ;
#82521=CARTESIAN_POINT ( 'NONE',  ( 0.1968062131348075061, 1420.483348320591176, 182.7518766831598214 ) ) ;
#82522=CARTESIAN_POINT ( 'NONE',  ( -1.530945675004649953, 1395.966522188359932, 220.0244024312320050 ) ) ;
#82523=CARTESIAN_POINT ( 'NONE',  ( -15.06561728630400054, 1422.389775765796230, 229.4662607246160064 ) ) ;
#82526=CARTESIAN_POINT ( 'NONE',  ( -2.413323989047310381, 1410.375482399494103, 232.6928827166564133 ) ) ;
#82533=CARTESIAN_POINT ( 'NONE',  ( 10.71141203040000001, 1409.287111137730108, 190.6699416860979852 ) ) ;
#82535=B_SPLINE_CURVE_WITH_KNOTS ( 'NONE', 3,
 ( #50277, #24479, #17160, #94440, #51353, #77127, #433, #84406, #50809, #109074 ),
 .UNSPECIFIED., .F., .F.,
 ( 4, 2, 2, 2, 4 ),
 ( 0.000000000000000000, 0.07144792451131930233, 0.1124765170753259935, 0.1725353800366839774, 0.2229999168759839723 ),
 .UNSPECIFIED. ) ;
#82538=CARTESIAN_POINT ( 'NONE',  ( -12.66923305982695958, 1398.288632557894289, 212.0380595282034619 ) ) ;
#82544=CARTESIAN_POINT ( 'NONE',  ( 19.85685705864179695, 1508.846415979930043, 229.4817442290339784 ) ) ;
#82548=CARTESIAN_POINT ( 'NONE',  ( -5.247863634239999797, 1396.629037141330173, 220.9040508069979865 ) ) ;
#82549=CARTESIAN_POINT ( 'NONE',  ( -20.05397710889999630, 1410.534994038629975, 220.7224924335979779 ) ) ;
#82551=CARTESIAN_POINT ( 'NONE',  ( -12.96259728057930793, 1444.899188585709453, 169.4271164727056771 ) ) ;
#82552=CARTESIAN_POINT ( 'NONE',  ( 0.3621993315900440269, 1416.825784014750070, 227.1772709241249970 ) ) ;
#82558=CARTESIAN_POINT ( 'NONE',  ( 5.279034537639999414, 1410.298216193129974, 186.4795294922980133 ) ) ;
#82559=CARTESIAN_POINT ( 'NONE',  ( -4.836107688109999359, 1414.913060387329779, 193.6922375078979996 ) ) ;
#82561=CARTESIAN_POINT ( 'NONE',  ( 6.002018859382760141, 1396.122655539619927, 199.8546179732479970 ) ) ;
#82562=CARTESIAN_POINT ( 'NONE',  ( 1.556370157619999972, 1414.996444526030018, 191.7142053706980107 ) ) ;
#82563=CARTESIAN_POINT ( 'NONE',  ( 11.15490121449999883, 1425.160561550830153, 144.1688093938980160 ) ) ;
#82566=CARTESIAN_POINT ( 'NONE',  ( 13.19362647665400168, 1435.060500567780082, 149.8921243419820257 ) ) ;
#82568=ORIENTED_EDGE ( 'NONE', *, *, #62285, .T. ) ;
#82571=CARTESIAN_POINT ( 'NONE',  ( -14.50827198289999842, 1461.594363702429746, 229.4507344440980035 ) ) ;
#82576=ORIENTED_EDGE ( 'NONE', *, *, #65887, .F. ) ;
#82578=CARTESIAN_POINT ( 'NONE',  ( -14.42137577593229913, 1509.529401687109839, 182.8435569880860214 ) ) ;
#82584=CARTESIAN_POINT ( 'NONE',  ( -29.85762690982718937, 1419.472691627382119, 269.4692931743723534 ) ) ;
#82585=CARTESIAN_POINT ( 'NONE',  ( -1.439448805189999847, 1408.963327047329813, 231.9239705684979924 ) ) ;
#82586=CARTESIAN_POINT ( 'NONE',  ( -4.255689356150000435, 1519.913060387329779, 186.6761948862979921 ) ) ;
#82589=CARTESIAN_POINT ( 'NONE',  ( -29.20316173986769925, 1440.913060386999859, 235.6859508697740182 ) ) ;
#82591=CARTESIAN_POINT ( 'NONE',  ( -12.53380499169999851, 1445.052233488290085, 169.4755105685979970 ) ) ;
#82593=CARTESIAN_POINT ( 'NONE',  ( 5.012278525919999339, 1408.134067213729850, 270.2879168813980186 ) ) ;
#82595=CARTESIAN_POINT ( 'NONE',  ( 24.02131707860000276, 1410.844657319930093, 208.5571756898100091 ) ) ;
#82600=CARTESIAN_POINT ( 'NONE',  ( -4.046419768304757802, 1446.994263467394603, 154.8289802513601785 ) ) ;
#82602=CARTESIAN_POINT ( 'NONE',  ( -15.00246656865998496, 1486.068585992124554, 186.3294758681441863 ) ) ;
#82607=CARTESIAN_POINT ( 'NONE',  ( 16.95307557376462171, 1410.872489480477498, 226.3250901887366240 ) ) ;
#82610=CARTESIAN_POINT ( 'NONE',  ( -5.386185223340929973, 1432.347042777500064, 154.6076275972019971 ) ) ;
#82615=CARTESIAN_POINT ( 'NONE',  ( -22.33897147115630233, 1410.187224944829950, 212.0108098745100165 ) ) ;
#82623=CARTESIAN_POINT ( 'NONE',  ( 24.34559517319999955, 1444.819512104510068, 214.6978151758279978 ) ) ;
#82624=CARTESIAN_POINT ( 'NONE',  ( 7.886710164585208460, 1438.222028729959902, 153.7402925291054316 ) ) ;
#82630=CARTESIAN_POINT ( 'NONE',  ( -19.98479248519999985, 1427.060832424730052, 224.6412401930980138 ) ) ;
#82633=ADVANCED_FACE ( 'NONE', ( #2702 ), #16928, .T. ) ;
#82634=CARTESIAN_POINT ( 'NONE',  ( 17.56771607889999842, 1461.948909412230023, 189.9394063172979941 ) ) ;
#82636=CARTESIAN_POINT ( 'NONE',  ( -12.91577053000571240, 1469.952397743109032, 269.3566365841412562 ) ) ;
#82639=CARTESIAN_POINT ( 'NONE',  ( 9.840689968320072367, 1506.501081259705870, 189.3968735791325742 ) ) ;
#82641=CARTESIAN_POINT ( 'NONE',  ( 1.956220388341530114, 1452.619890567819994, 181.5372545095350176 ) ) ;
#82642=FACE_OUTER_BOUND ( 'NONE', #83448, .T. ) ;
#82643=CARTESIAN_POINT ( 'NONE',  ( -13.48104552572402781, 1444.198070212794846, 187.0427700716132620 ) ) ;
#82648=ADVANCED_FACE ( 'NONE', ( #3121 ), #58067, .T. ) ;
#82649=CARTESIAN_POINT ( 'NONE',  ( 25.00975353569999626, 1436.598045313000057, 137.9330155572980061 ) ) ;
#82650=CARTESIAN_POINT ( 'NONE',  ( -12.55177817982819555, 1442.776457442548690, 169.4734774201230323 ) ) ;
#82651=CARTESIAN_POINT ( 'NONE',  ( -13.79685521319999886, 1409.394857187929802, 225.4822212544980289 ) ) ;
#82652=ORIENTED_EDGE ( 'NONE', *, *, #45505, .F. ) ;
#82655=ADVANCED_FACE ( 'NONE', ( #47299 ), #71447, .F. ) ;
#82656=ORIENTED_EDGE ( 'NONE', *, *, #37091, .T. ) ;
#82657=ORIENTED_EDGE ( 'NONE', *, *, #15837, .F. ) ;
#82663=CARTESIAN_POINT ( 'NONE',  ( -11.87145374459999836, 1433.215786360830180, 150.2634173165980087 ) ) ;
#82666=DIRECTION ( 'NONE',  ( -1.000000000000000000, 0.000000000000000000, -1.989567262110869994E-13 ) ) ;
#82667=CARTESIAN_POINT ( 'NONE',  ( -11.36018337610000195, 1414.996442546130083, 195.9645814914979951 ) ) ;
#82668=CARTESIAN_POINT ( 'NONE',  ( -4.500000000000000000, 1448.210448412289907, 183.1418046154980175 ) ) ;
#82669=CARTESIAN_POINT ( 'NONE',  ( -0.2350516018847411404, 1467.133467089303167, 235.6301535849441962 ) ) ;
#82671=CARTESIAN_POINT ( 'NONE',  ( -11.07653839470680346, 1509.424964076853257, 237.0021322192719424 ) ) ;
#82675=CARTESIAN_POINT ( 'NONE',  ( -11.86538321653400097, 1432.285882802679907, 149.9821595126069838 ) ) ;
#82677=CARTESIAN_POINT ( 'NONE',  ( -7.984658461500000470, 1471.246104330929938, 269.8705384494979853 ) ) ;
#82678=FACE_OUTER_BOUND ( 'NONE', #57909, .T. ) ;
#82681=CARTESIAN_POINT ( 'NONE',  ( 35.55994568960879576, 1450.202733143109981, 136.2282289233990014 ) ) ;
#82682=CARTESIAN_POINT ( 'NONE',  ( 0.2730310470048849525, 1451.200684518790013, 182.3105317300910144 ) ) ;
#82687=CARTESIAN_POINT ( 'NONE',  ( -42.01580735148260004, 1426.337994121050087, 268.6260313102509940 ) ) ;
#82688=ORIENTED_EDGE ( 'NONE', *, *, #69676, .F. ) ;
#82689=CARTESIAN_POINT ( 'NONE',  ( -3.549608351769999892, 1507.276797637930031, 180.9704965309979912 ) ) ;
#82690=ORIENTED_EDGE ( 'NONE', *, *, #71407, .T. ) ;
#82693=CARTESIAN_POINT ( 'NONE',  ( 4.563532145992947875, 1423.757224567328194, 183.7871458247886380 ) ) ;
#82694=CARTESIAN_POINT ( 'NONE',  ( -2.500000000000000000, 1431.404049859629822, 183.8987783686980038 ) ) ;
#82697=CARTESIAN_POINT ( 'NONE',  ( -17.07773618619999922, 1455.454993475929996, 189.7981302288980032 ) ) ;
#82699=CARTESIAN_POINT ( 'NONE',  ( -2.342714119161724451, 1449.671868188517237, 182.9885556723570517 ) ) ;
#82701=CARTESIAN_POINT ( 'NONE',  ( -26.24539357829999631, 1435.712694766920094, 136.2621512218979944 ) ) ;
#82705=CARTESIAN_POINT ( 'NONE',  ( -42.06230369252700285, 1436.187529677659768, 269.6487418071969842 ) ) ;
#82707=CARTESIAN_POINT ( 'NONE',  ( -1.249934943059999970, 1397.324122628329860, 196.1772859776979772 ) ) ;
#82710=ORIENTED_EDGE ( 'NONE', *, *, #18889, .F. ) ;
#82711=DIRECTION ( 'NONE',  ( 0.000000000000000000, 1.000000000000000000, 0.000000000000000000 ) ) ;
#82720=CARTESIAN_POINT ( 'NONE',  ( -13.40958072599999973, 1414.996442553830093, 220.3303866892979954 ) ) ;
#82723=ORIENTED_EDGE ( 'NONE', *, *, #54309, .F. ) ;
#82724=CARTESIAN_POINT ( 'NONE',  ( -38.81202642568450045, 1436.797832264140197, 135.0584845260209761 ) ) ;
#82726=CARTESIAN_POINT ( 'NONE',  ( -23.87523795545963168, 1446.306127926221507, 213.5443193811669857 ) ) ;
#82729=CARTESIAN_POINT ( 'NONE',  ( 12.63077516952419899, 1434.551872175529979, 149.3944923939809826 ) ) ;
#82730=CARTESIAN_POINT ( 'NONE',  ( 13.56558276610000036, 1415.128105759529944, 197.4687002248980150 ) ) ;
#82731=CARTESIAN_POINT ( 'NONE',  ( -2.875659595060000129, 1507.251074144529866, 180.8868938330980143 ) ) ;
#82732=CARTESIAN_POINT ( 'NONE',  ( 2.488082932330000219, 1441.600846913620217, 150.5962877614979902 ) ) ;
#82733=CARTESIAN_POINT ( 'NONE',  ( 16.17523438889999809, 1409.477912219330165, 225.6432943882979885 ) ) ;
#82736=CARTESIAN_POINT ( 'NONE',  ( 4.280208222382819727, 1441.004501108590148, 156.4771712661509753 ) ) ;
#82738=CARTESIAN_POINT ( 'NONE',  ( 16.66094735743510213, 1410.867388111209948, 226.5061907891179942 ) ) ;
#82740=ORIENTED_EDGE ( 'NONE', *, *, #58388, .T. ) ;
#82743=CARTESIAN_POINT ( 'NONE',  ( 2.113759566260000167, 1420.502650363029943, 184.8096912009980031 ) ) ;
#82747=CARTESIAN_POINT ( 'NONE',  ( -0.04640499230476000103, 1508.911437368330098, 179.6947746304720113 ) ) ;
#82748=CARTESIAN_POINT ( 'NONE',  ( 11.60004869885214518, 1425.158469683133717, 137.9573055125791541 ) ) ;
#82751=CARTESIAN_POINT ( 'NONE',  ( 18.01599769506526272, 1424.260621041340301, 225.3203408571521038 ) ) ;
#82753=CARTESIAN_POINT ( 'NONE',  ( -4.041733614507550032E-07, 1407.244919736519932, 222.1486585491760195 ) ) ;
#82754=CARTESIAN_POINT ( 'NONE',  ( 32.83529528479970594, 1440.913060383310039, 246.2013942643669964 ) ) ;
#82758=ORIENTED_EDGE ( 'NONE', *, *, #21376, .T. ) ;
#82759=ORIENTED_EDGE ( 'NONE', *, *, #20066, .F. ) ;
#82761=CARTESIAN_POINT ( 'NONE',  ( 17.13513247068420497, 1410.030456530622814, 192.6342742787495865 ) ) ;
#82764=CARTESIAN_POINT ( 'NONE',  ( -2.500000000000000000, 1411.429641636929773, 137.0999999980979851 ) ) ;
#82766=DIRECTION ( 'NONE',  ( 0.000000000000000000, 1.000000000000000000, 0.000000000000000000 ) ) ;
#82769=DIRECTION ( 'NONE',  ( -1.000000000000000000, 0.000000000000000000, 0.000000000000000000 ) ) ;
#82770=PLANE ( 'NONE',  #30788 ) ;
#82781=CARTESIAN_POINT ( 'NONE',  ( -11.52810963750000006, 1441.751267666019885, 147.8533156590980013 ) ) ;
#82785=CARTESIAN_POINT ( 'NONE',  ( 3.500000000000000000, 1421.663060387330006, 172.2701767054979882 ) ) ;
#82786=CARTESIAN_POINT ( 'NONE',  ( 9.850348957860671106, 1409.257042152700024, 197.8655441185040047 ) ) ;
#82788=CARTESIAN_POINT ( 'NONE',  ( 18.02214392489999994, 1424.365982604130068, 225.0542928084979906 ) ) ;
#82792=CARTESIAN_POINT ( 'NONE',  ( -10.79382269979189957, 1414.913060387349788, 196.1395788316550011 ) ) ;
#82793=VERTEX_POINT ( 'NONE', #54082 ) ;
#82795=CARTESIAN_POINT ( 'NONE',  ( -11.60004869885203682, 1428.983126981193436, 134.0999999980979851 ) ) ;
#82796=CARTESIAN_POINT ( 'NONE',  ( -12.24435440740000125, 1434.149509971349971, 149.6614242918979869 ) ) ;
#82797=CARTESIAN_POINT ( 'NONE',  ( -4.184817693673509801E-10, 1466.841376965610152, 244.4596446984610054 ) ) ;
#82799=DIRECTION ( 'NONE',  ( -0.03489949670252247976, -0.9993908270190688947, -2.284588939963739914E-07 ) ) ;
#82801=CARTESIAN_POINT ( 'NONE',  ( 0.1623851794880000199, 1484.828409465129880, 181.8869582818979893 ) ) ;
#82804=CARTESIAN_POINT ( 'NONE',  ( -19.14726318969999852, 1425.916566196629901, 226.2004032037980039 ) ) ;
#82808=CARTESIAN_POINT ( 'NONE',  ( 7.121584085660000341, 1409.161751583630121, 222.2855843900980233 ) ) ;
#82809=PRESENTATION_STYLE_ASSIGNMENT (( #73879 ) ) ;
#82810=CARTESIAN_POINT ( 'NONE',  ( 8.492686941340000573, 1424.222007991629880, 101.6998295726980075 ) ) ;
#82813=CARTESIAN_POINT ( 'NONE',  ( 29.81189561119999709, 1423.440805375829996, 254.8364577152979962 ) ) ;
#82815=CARTESIAN_POINT ( 'NONE',  ( 0.5325504066310000617, 1458.410320103429967, 183.0292182426980219 ) ) ;
#82816=CARTESIAN_POINT ( 'NONE',  ( -17.60618190530000149, 1410.892634225830079, 194.3214822148979977 ) ) ;
#82818=CARTESIAN_POINT ( 'NONE',  ( -29.63060408680000180, 1437.055400001079988, 238.0637331587980157 ) ) ;
#82820=CARTESIAN_POINT ( 'NONE',  ( 0.7313901380009910635, 1415.506039114428177, 233.2853349926991200 ) ) ;
#82821=CARTESIAN_POINT ( 'NONE',  ( 30.24883931639999801, 1451.704266439629919, 135.6947013027980233 ) ) ;
#82825=CARTESIAN_POINT ( 'NONE',  ( 14.42573317639249986, 1420.832147603980047, 228.3843187111120017 ) ) ;
#82830=CARTESIAN_POINT ( 'NONE',  ( -22.70354091851470102, 1409.705854860960017, 209.2041153040200072 ) ) ;
#82831=CARTESIAN_POINT ( 'NONE',  ( -3.939734656090000176, 1425.432672367729992, 186.1013744347979753 ) ) ;
#82834=CARTESIAN_POINT ( 'NONE',  ( -0.2986054180299999583, 1498.355349864329810, 236.9494477147979978 ) ) ;
#82838=CARTESIAN_POINT ( 'NONE',  ( 42.05291394628070378, 1455.559135556939964, 267.1115876222309566 ) ) ;
#82839=ADVANCED_FACE ( 'NONE', ( #46773 ), #17232, .F. ) ;
#82840=CARTESIAN_POINT ( 'NONE',  ( -1.543833121739990100, 1424.175334750540060, 228.3471663839470125 ) ) ;
#82841=CARTESIAN_POINT ( 'NONE',  ( -0.07944575511320001171, 1419.763150379130138, 184.3780574224979887 ) ) ;
#82845=EDGE_CURVE ( 'NONE', #85844, #11858, #73447, .T. ) ;
#82847=CARTESIAN_POINT ( 'NONE',  ( 12.74884836167065671, 1442.825961663651242, 186.7702961919069082 ) ) ;
#82848=ORIENTED_EDGE ( 'NONE', *, *, #34397, .T. ) ;
#82851=EDGE_CURVE ( 'NONE', #56464, #75143, #91508, .T. ) ;
#82856=CARTESIAN_POINT ( 'NONE',  ( 16.56432441049999937, 1409.491499342829911, 193.0008963472980099 ) ) ;
#82859=CARTESIAN_POINT ( 'NONE',  ( 0.03196084884758292749, 1409.231241321286234, 232.6875248013703867 ) ) ;
#82860=CARTESIAN_POINT ( 'NONE',  ( -16.76374941339440028, 1414.024291605689996, 191.6492321041440050 ) ) ;
#82863=CARTESIAN_POINT ( 'NONE',  ( -25.78156655170059608, 1509.813372604039841, 223.1298223243570078 ) ) ;
#82864=CARTESIAN_POINT ( 'NONE',  ( 4.823778297959999684, 1426.859560269130043, 144.1938086916980239 ) ) ;
#82866=CARTESIAN_POINT ( 'NONE',  ( 4.218847493579999853E-15, 1426.979439823029907, 214.3676144195279676 ) ) ;
#82871=EDGE_CURVE ( 'NONE', #98399, #63715, #61368, .T. ) ;
#82873=ORIENTED_EDGE ( 'NONE', *, *, #80486, .T. ) ;
#82875=CARTESIAN_POINT ( 'NONE',  ( -2.482344662330000062, 1440.444625599219989, 150.5580151863979950 ) ) ;
#82877=CARTESIAN_POINT ( 'NONE',  ( 11.27096283070000027, 1433.884051265439894, 151.5488804711980038 ) ) ;
#82878=CARTESIAN_POINT ( 'NONE',  ( 39.48812356970000081, 1450.238330950499858, 268.3665355199980240 ) ) ;
#82879=CARTESIAN_POINT ( 'NONE',  ( 0.7331802501534880889, 1450.881784651950056, 181.3416385694490032 ) ) ;
#82880=EDGE_CURVE ( 'NONE', #65905, #23724, #29395, .T. ) ;
#82885=ADVANCED_FACE ( 'NONE', ( #86961 ), #1561, .T. ) ;
#82888=CARTESIAN_POINT ( 'NONE',  ( 23.10251669230000360, 1410.654477903330189, 207.3358591529579940 ) ) ;
#82890=CARTESIAN_POINT ( 'NONE',  ( -17.47308017059999941, 1410.448094988030107, 225.6071494025980257 ) ) ;
#82897=CARTESIAN_POINT ( 'NONE',  ( -6.288099047490000260, 1416.823872462329973, 226.3732097004979948 ) ) ;
#82900=VERTEX_POINT ( 'NONE', #42762 ) ;
#82901=CARTESIAN_POINT ( 'NONE',  ( -13.74428069829999899, 1415.087818611729972, 199.1627811320679768 ) ) ;
#82903=CARTESIAN_POINT ( 'NONE',  ( 13.80559114949999966, 1434.979605424110105, 147.9458860626980083 ) ) ;
#82904=CARTESIAN_POINT ( 'NONE',  ( -41.62352936867430486, 1444.515901151979961, 134.0999999983539794 ) ) ;
#82905=CARTESIAN_POINT ( 'NONE',  ( 7.452717793499999743, 1442.053991537899947, 184.4597269369980097 ) ) ;
#82906=EDGE_LOOP ( 'NONE', ( #44515, #94339, #7738, #12620 ) ) ;
#82907=B_SPLINE_SURFACE_WITH_KNOTS ( 'NONE', 5, 5, ( 
 ( #66775, #24708, #15216, #42648, #42101, #51057 ),
 ( #93578, #16853, #117, #110397, #7932, #51606 ),
 ( #100874, #17409, #74612, #41552, #85188, #75708 ),
 ( #58356, #101980, #83532, #33132, #92480, #33677 ),
 ( #59468, #23635, #67320, #40986, #49407, #84634 ),
 ( #76249, #85740, #8474, #76802, #109855, #34240 ),
 ( #94138, #101418, #58906, #93037, #6826, #75165 ),
 ( #100347, #57817, #49952, #91942, #109313, #68425 ),
 ( #32598, #102527, #25266, #16310, #24166, #9038 ) ),
 .UNSPECIFIED., .F., .F., .F.,
 ( 6, 3, 6 ),
 ( 6, 6 ),
 ( 0.7655572723410000169, 2.316155491860000026, 3.835724788389999862 ),
 ( 0.000000000000000000, 1.000000000000000000 ),
 .UNSPECIFIED. ) ;
#82909=FACE_OUTER_BOUND ( 'NONE', #54247, .T. ) ;
#82913=CARTESIAN_POINT ( 'NONE',  ( 40.41497139838102726, 1425.029171221357274, 269.1178663084699565 ) ) ;
#82914=CARTESIAN_POINT ( 'NONE',  ( 22.89347097630000150, 1507.627022993330229, 210.0374582935500030 ) ) ;
#82921=CARTESIAN_POINT ( 'NONE',  ( -28.37476903577010034, 1508.765197044639990, 208.8169969777860047 ) ) ;
#82923=CARTESIAN_POINT ( 'NONE',  ( -15.97953102573920070, 1409.479266170219944, 225.4412730300549867 ) ) ;
#82924=CARTESIAN_POINT ( 'NONE',  ( 0.5054431922854470960, 1412.724905019189919, 184.9686944227329946 ) ) ;
#82927=CARTESIAN_POINT ( 'NONE',  ( 40.27303016874642339, 1443.635579762076532, 137.1189739665458092 ) ) ;
#82930=CARTESIAN_POINT ( 'NONE',  ( -0.2673276340219670200, 1419.096787968140006, 184.6139809674839967 ) ) ;
#82931=CARTESIAN_POINT ( 'NONE',  ( 1.260378580130000037, 1465.786016857930008, 235.4507837586979804 ) ) ;
#82932=CARTESIAN_POINT ( 'NONE',  ( 19.69577440509999988, 1410.523406920930029, 220.5361315035979999 ) ) ;
#82933=DIRECTION ( 'NONE',  ( 0.01255267363915089744, 0.04169729272521120744, -0.9990514331924543745 ) ) ;
#82934=CARTESIAN_POINT ( 'NONE',  ( -16.40174870470000101, 1423.220782154630115, 228.3136831567979925 ) ) ;
#82936=CARTESIAN_POINT ( 'NONE',  ( 23.55086976260000142, 1411.110717726029861, 207.7642927257880103 ) ) ;
#82938=CARTESIAN_POINT ( 'NONE',  ( 6.940379574320000522, 1431.113060387329824, 226.8285010592979916 ) ) ;
#82939=CARTESIAN_POINT ( 'NONE',  ( -1.555904870050000000, 1417.383305120430123, 234.5694431353979894 ) ) ;
#82941=EDGE_CURVE ( 'NONE', #55821, #67655, #7977, .T. ) ;
#82943=B_SPLINE_CURVE_WITH_KNOTS ( 'NONE', 3,
 ( #14724, #92527, #50553, #84131, #100917, #33176 ),
 .UNSPECIFIED., .F., .F.,
 ( 4, 2, 4 ),
 ( -0.2552102774606619939, -0.1273445234295760009, -2.595975838515229839E-06 ),
 .UNSPECIFIED. ) ;
#82944=CARTESIAN_POINT ( 'NONE',  ( -10.30745342060079928, 1484.762341913489990, 185.0171830968129996 ) ) ;
#82947=CARTESIAN_POINT ( 'NONE',  ( -4.221576979972950561, 1441.604095695570095, 168.5833479033780122 ) ) ;
#82953=CARTESIAN_POINT ( 'NONE',  ( 3.043251597425320032, 1417.779699503100119, 234.3208248802520188 ) ) ;
#82954=FACE_OUTER_BOUND ( 'NONE', #94253, .T. ) ;
#82955=CARTESIAN_POINT ( 'NONE',  ( -11.74144633689528128, 1426.693258465743384, 144.4869926498055293 ) ) ;
#82956=CARTESIAN_POINT ( 'NONE',  ( 15.90190012156959831, 1409.720761371890148, 192.1156709633790172 ) ) ;
#82958=CARTESIAN_POINT ( 'NONE',  ( 37.55019156315650264, 1436.545190313800049, 135.0428358297800173 ) ) ;
#82959=B_SPLINE_CURVE_WITH_KNOTS ( 'NONE', 5,
 ( #21630, #3787, #54737, #73736, #55836, #4319 ),
 .UNSPECIFIED., .F., .F.,
 ( 6, 6 ),
 ( -22.35973423652749759, -7.053367062128510057 ),
 .UNSPECIFIED. ) ;
#82961=B_SPLINE_CURVE_WITH_KNOTS ( 'NONE', 3,
 ( #92418, #54108, #45704, #80386, #46803, #52990, #96073, #36176, #105033, #3150, #105596 ),
 .UNSPECIFIED., .F., .F.,
 ( 4, 2, 1, 2, 2, 4 ),
 ( 0.000000000000000000, 0.2499999999997608024, 0.3749999999994814703, 0.4374999999994910183, 0.4999999999995006217, 1.000000000000000000 ),
 .UNSPECIFIED. ) ;
#82962=CARTESIAN_POINT ( 'NONE',  ( 33.93526097501167982, 1435.841486971047743, 135.9408947062673860 ) ) ;
#82963=CARTESIAN_POINT ( 'NONE',  ( -2.595027496015959834, 1509.076031574679973, 179.4162640487629972 ) ) ;
#82964=CARTESIAN_POINT ( 'NONE',  ( 11.44122415478343946, 1464.077397819507269, 231.7897981619890118 ) ) ;
#82966=CARTESIAN_POINT ( 'NONE',  ( 38.71265708145079287, 1449.925712784929829, 134.0999999982089719 ) ) ;
#82967=CARTESIAN_POINT ( 'NONE',  ( 3.696509732892085065, 1396.042145351627596, 219.6749981702555488 ) ) ;
#82971=ORIENTED_EDGE ( 'NONE', *, *, #86405, .F. ) ;
#82972=AXIS2_PLACEMENT_3D ( 'NONE', #18786, #44576, #30376 ) ;
#82975=DIRECTION ( 'NONE',  ( 0.3363363969984562996, 0.9417419115947303077, -4.718447854657144508E-13 ) ) ;
#82978=CARTESIAN_POINT ( 'NONE',  ( -2.500000000000000000, 1439.419208558560058, 162.1010788394430051 ) ) ;
#82981=CARTESIAN_POINT ( 'NONE',  ( -27.26565262369999942, 1508.025370090229899, 204.2545478268079933 ) ) ;
#82982=CARTESIAN_POINT ( 'NONE',  ( 38.81202642569470385, 1450.612734564189850, 135.0591088798190071 ) ) ;
#82985=CARTESIAN_POINT ( 'NONE',  ( 7.105427357599999217E-15, 1419.973720559130015, 171.2095165336979790 ) ) ;
#82986=CARTESIAN_POINT ( 'NONE',  ( 1.523413191080000173, 1416.219761279530076, 190.3037518844979843 ) ) ;
#82991=ORIENTED_EDGE ( 'NONE', *, *, #21920, .T. ) ;
#82992=CARTESIAN_POINT ( 'NONE',  ( 38.48560341180350264, 1440.913060387330006, 265.5651213211320396 ) ) ;
#82993=EDGE_CURVE ( 'NONE', #107006, #88595, #99752, .T. ) ;
#82994=CARTESIAN_POINT ( 'NONE',  ( 18.47666778710000202, 1457.021925454829898, 227.5921493168980021 ) ) ;
#82996=CARTESIAN_POINT ( 'NONE',  ( -0.07726448487090450956, 1452.995338504329993, 183.2382765356399830 ) ) ;
#82997=CARTESIAN_POINT ( 'NONE',  ( -8.313145311751080513, 1507.316772571419961, 235.1568484389069909 ) ) ;
#83000=CARTESIAN_POINT ( 'NONE',  ( -4.305050228820000768, 1421.448985974330071, 185.8634108395979752 ) ) ;
#83002=CARTESIAN_POINT ( 'NONE',  ( -0.8378200133160000895, 1507.147729961930054, 180.8463070720979999 ) ) ;
#83005=EDGE_CURVE ( 'NONE', #93599, #79565, #104991, .T. ) ;
#83006=CARTESIAN_POINT ( 'NONE',  ( 11.96123311770000086, 1461.918702350729745, 232.8139469471979908 ) ) ;
#83007=CARTESIAN_POINT ( 'NONE',  ( -10.43907017127172132, 1423.422407654868266, 137.2932306828950288 ) ) ;
#83013=CARTESIAN_POINT ( 'NONE',  ( -0.6994492260031126563, 1486.354407208097427, 181.7735033864214813 ) ) ;
#83018=CARTESIAN_POINT ( 'NONE',  ( -11.60004869885203682, 1426.458005531418394, 139.1709612739483930 ) ) ;
#83021=CARTESIAN_POINT ( 'NONE',  ( -19.86721352349999847, 1507.838653463430092, 229.2281063170979678 ) ) ;
#83022=CARTESIAN_POINT ( 'NONE',  ( 8.208155165579999135, 1461.578545524030005, 225.7601664794979968 ) ) ;
#83023=CARTESIAN_POINT ( 'NONE',  ( -10.96804868159999913, 1432.244841162460034, 151.7696487253979853 ) ) ;
#83024=CARTESIAN_POINT ( 'NONE',  ( 19.17509738295899879, 1456.935641295649930, 224.9175647810569956 ) ) ;
#83026=DIRECTION ( 'NONE',  ( -0.7799412787973096783, 0.3217084223181928548, 0.5368382369369347762 ) ) ;
#83030=CARTESIAN_POINT ( 'NONE',  ( -19.45296971400000174, 1482.733639547430130, 228.0655676717979929 ) ) ;
#83031=CARTESIAN_POINT ( 'NONE',  ( -10.71468703753418872, 1425.002736333741268, 137.0999999980979567 ) ) ;
#83032=CARTESIAN_POINT ( 'NONE',  ( -2.343308038029999985, 1485.565572279829894, 182.6780017771980056 ) ) ;
#83033=ORIENTED_EDGE ( 'NONE', *, *, #74749, .T. ) ;
#83035=CARTESIAN_POINT ( 'NONE',  ( 12.58326012370000058, 1407.771031778829865, 269.4439677704979772 ) ) ;
#83036=EDGE_CURVE ( 'NONE', #33795, #99633, #58761, .T. ) ;
#83037=CARTESIAN_POINT ( 'NONE',  ( -0.1068857359190000106, 1409.419549845830261, 185.2272142515979851 ) ) ;
#83039=CARTESIAN_POINT ( 'NONE',  ( 23.02916308347723273, 1432.351854092651138, 216.0372900143995878 ) ) ;
#83041=LINE ( 'NONE', #6334, #30731 ) ;
#83044=CARTESIAN_POINT ( 'NONE',  ( -1.602465797461561925, 1451.492110311741271, 183.9566778351376399 ) ) ;
#83045=CARTESIAN_POINT ( 'NONE',  ( -17.73803434250000066, 1408.913060387329779, 209.1218459616979999 ) ) ;
#83046=CARTESIAN_POINT ( 'NONE',  ( -14.06293010156700163, 1415.542389211330146, 220.9878170194020015 ) ) ;
#83049=B_SPLINE_SURFACE_WITH_KNOTS ( 'NONE', 5, 1, ( 
 ( #15505, #108491 ),
 ( #50261, #92234 ),
 ( #31776, #75464 ),
 ( #23907, #100088 ),
 ( #23370, #91683 ),
 ( #14958, #49153 ),
 ( #100624, #49704 ),
 ( #24460, #83833 ),
 ( #109598, #7135 ) ),
 .UNSPECIFIED., .F., .F., .F.,
 ( 6, 3, 6 ),
 ( 2, 2 ),
 ( 0.000000000000000000, 5.782490304330000441, 11.25975508159999983 ),
 ( -1.500000000000000000, 1.500000000000000000 ),
 .UNSPECIFIED. ) ;
#83051=CARTESIAN_POINT ( 'NONE',  ( 20.57820469800335061, 1507.771259987313442, 228.0150961245546455 ) ) ;
#83052=CARTESIAN_POINT ( 'NONE',  ( 4.227606371040000255, 1441.557582927179965, 165.0907967835979662 ) ) ;
#83053=CARTESIAN_POINT ( 'NONE',  ( -3.758278191160000059, 1475.720032253530007, 266.9554522522980164 ) ) ;
#83054=CARTESIAN_POINT ( 'NONE',  ( -4.240346501305279681, 1446.384605478229787, 162.7848567535889970 ) ) ;
#83059=CONICAL_SURFACE ( 'NONE', #99103, 4.000000000000003553, 0.3430239404209998177 ) ;
#83061=B_SPLINE_SURFACE_WITH_KNOTS ( 'NONE', 5, 5, ( 
 ( #1253, #85790, #61728, #86342, #10757, #705 ),
 ( #69024, #44928, #53320, #9087, #103126, #19117 ),
 ( #95851, #26427, #87466, #79075, #102024, #25863 ),
 ( #51103, #60065, #8519, #56055, #4016, #28651 ),
 ( #55516, #53891, #88027, #2927, #11311, #37599 ),
 ( #13465, #4552, #47111, #11850, #81237, #29737 ),
 ( #96411, #97504, #90182, #72323, #38142, #106454 ),
 ( #98039, #63924, #62281, #19687, #72861, #21313 ),
 ( #71801, #12387, #89099, #38686, #106996, #30285 ),
 ( #45480, #29199, #80707, #64477, #79623, #96967 ),
 ( #47655, #12930, #20773, #63389, #98592, #81783 ),
 ( #37043, #70694, #71238, #80151, #54974, #105361 ) ),
 .UNSPECIFIED., .F., .F., .F.,
 ( 6, 3, 3, 6 ),
 ( 6, 6 ),
 ( 14.42283113610000100, 18.25245354770000006, 23.76042384160000154, 29.04794202684080062 ),
 ( -1.219754076356229971E-05, 1.479898742370000075 ),
 .UNSPECIFIED. ) ;
#83062=CARTESIAN_POINT ( 'NONE',  ( 1.353901205137101993, 1408.960339659235160, 230.6360952523062338 ) ) ;
#83066=CARTESIAN_POINT ( 'NONE',  ( -21.38312428220000072, 1410.581396537829960, 200.7860588073580175 ) ) ;
#83067=CARTESIAN_POINT ( 'NONE',  ( -15.81490237038799940, 1421.038332005997972, 227.0412555000420127 ) ) ;
#83068=CARTESIAN_POINT ( 'NONE',  ( -3.345579560160000021, 1406.768167790330153, 269.6447283206980501 ) ) ;
#83074=CARTESIAN_POINT ( 'NONE',  ( 11.40309688480000005, 1425.502102498530121, 141.8402116268979967 ) ) ;
#83082=CARTESIAN_POINT ( 'NONE',  ( -11.90431320224219469, 1398.266029680347174, 203.8981089574260466 ) ) ;
#83086=CARTESIAN_POINT ( 'NONE',  ( 19.76862476762880050, 1508.335801748439962, 229.3107566332930105 ) ) ;
#83089=ORIENTED_EDGE ( 'NONE', *, *, #68063, .F. ) ;
#83090=CARTESIAN_POINT ( 'NONE',  ( 11.48004703006369986, 1434.398966934330019, 151.4080194248590203 ) ) ;
#83091=CARTESIAN_POINT ( 'NONE',  ( -10.93767073350000096, 1397.622345362329952, 216.8369142482779921 ) ) ;
#83092=CARTESIAN_POINT ( 'NONE',  ( -22.30142397239999852, 1410.611543101329971, 213.5076809071279911 ) ) ;
#83094=CARTESIAN_POINT ( 'NONE',  ( -12.76036967837525182, 1444.996034417363035, 169.4538253455069707 ) ) ;
#83095=CARTESIAN_POINT ( 'NONE',  ( 21.01461835239121001, 1509.697381924852380, 230.2161845864164320 ) ) ;
#83096=CARTESIAN_POINT ( 'NONE',  ( -0.1681681984989999989, 1405.973120458229914, 121.6099336315979969 ) ) ;
#83097=CARTESIAN_POINT ( 'NONE',  ( -2.253566441613126910E-10, 1426.918876941764893, 137.0999999980980135 ) ) ;
#83098=CARTESIAN_POINT ( 'NONE',  ( -13.70765206225300048, 1507.670578231209902, 184.2574963778999688 ) ) ;
#83102=CARTESIAN_POINT ( 'NONE',  ( 1.733308840189999867, 1468.706793215829975, 182.8378066306980259 ) ) ;
#83103=CARTESIAN_POINT ( 'NONE',  ( -7.292852437050000525, 1414.971279908829956, 193.7940289552979891 ) ) ;
#83104=CARTESIAN_POINT ( 'NONE',  ( 44.13013120502959907, 1440.913053252359987, 270.2165820558270184 ) ) ;
#83105=CARTESIAN_POINT ( 'NONE',  ( 11.07286074960780198, 1396.299733205200027, 209.1571633317650196 ) ) ;
#83106=CARTESIAN_POINT ( 'NONE',  ( 2.500000000000000000, 1419.514443097085177, 137.6548205731159555 ) ) ;
#83107=CARTESIAN_POINT ( 'NONE',  ( 11.80289981959999857, 1428.296111302430063, 148.4248248087979789 ) ) ;
#83110=CARTESIAN_POINT ( 'NONE',  ( 13.14904837430809970, 1435.770654509489987, 150.5852354599839771 ) ) ;
#83111=B_SPLINE_CURVE_WITH_KNOTS ( 'NONE', 5,
 ( #42729, #76888, #60097, #88606, #63965, #47148 ),
 .UNSPECIFIED., .F., .F.,
 ( 6, 6 ),
 ( -2.000000000000000000, -4.763377830174775340E-06 ),
 .UNSPECIFIED. ) ;
#83114=CARTESIAN_POINT ( 'NONE',  ( -18.77710419973470124, 1478.090298906489807, 228.5270538965380069 ) ) ;
#83115=CARTESIAN_POINT ( 'NONE',  ( -10.92412005059999913, 1463.498050678130085, 231.8959999115979826 ) ) ;
#83116=CARTESIAN_POINT ( 'NONE',  ( -12.93261679799999975, 1416.825245919230156, 196.5037248033980006 ) ) ;
#83124=EDGE_LOOP ( 'NONE', ( #2583, #18432, #70299, #49252 ) ) ;
#83126=CARTESIAN_POINT ( 'NONE',  ( -20.50069311049999854, 1509.057110915630119, 229.1414337057980219 ) ) ;
#83128=CARTESIAN_POINT ( 'NONE',  ( -38.49454587240603587, 1428.649003040305843, 269.5844014560237270 ) ) ;
#83131=CARTESIAN_POINT ( 'NONE',  ( 0.3142797417281940064, 1415.426207913209964, 226.6044974060719994 ) ) ;
#83132=ORIENTED_EDGE ( 'NONE', *, *, #19041, .F. ) ;
#83133=CARTESIAN_POINT ( 'NONE',  ( -0.01294480814637470091, 1452.645328572880089, 183.2233851132330074 ) ) ;
#83134=CARTESIAN_POINT ( 'NONE',  ( -28.14800220618010229, 1440.913060388109898, 231.7476473256940039 ) ) ;
#83138=CARTESIAN_POINT ( 'NONE',  ( 7.595213675750000171, 1408.121098801730113, 270.1248737335980081 ) ) ;
#83139=CIRCLE ( 'NONE', #84876, 26.99999999999999645 ) ;
#83142=CARTESIAN_POINT ( 'NONE',  ( 22.92272308539999770, 1409.722145098229930, 209.1789479422659781 ) ) ;
#83143=CARTESIAN_POINT ( 'NONE',  ( 11.44665326297827335, 1425.798162341591706, 139.1345266541928538 ) ) ;
#83148=CARTESIAN_POINT ( 'NONE',  ( 0.2805947326950000154, 1419.238439929829838, 184.6459534269980054 ) ) ;
#83149=CARTESIAN_POINT ( 'NONE',  ( 0.8732702506809227883, 1409.114780694623732, 232.1132175656460674 ) ) ;
#83157=CARTESIAN_POINT ( 'NONE',  ( -1.547462741870939906, 1414.913060391199906, 225.9340804956229931 ) ) ;
#83164=DIRECTION ( 'NONE',  ( 0.000000000000000000, -1.000000000000000000, 0.000000000000000000 ) ) ;
#83167=EDGE_CURVE ( 'NONE', #28587, #106196, #15888, .T. ) ;
#83169=CARTESIAN_POINT ( 'NONE',  ( -0.1665868851619999869, 1457.817907875729816, 229.1616989435979974 ) ) ;
#83171=CARTESIAN_POINT ( 'NONE',  ( 23.88591464079999582, 1447.475895483519935, 215.7787009847079958 ) ) ;
#83173=EDGE_CURVE ( 'NONE', #2271, #14981, #4046, .T. ) ;
#83176=CARTESIAN_POINT ( 'NONE',  ( 11.16660779294305428, 1418.351232793595273, 229.7242082764032602 ) ) ;
#83177=CARTESIAN_POINT ( 'NONE',  ( 38.35993494222029909, 1448.483858230149735, 136.4260950382250144 ) ) ;
#83178=CARTESIAN_POINT ( 'NONE',  ( -19.34868852410000173, 1426.386304191129966, 225.0623401300979936 ) ) ;
#83179=CARTESIAN_POINT ( 'NONE',  ( -23.61600082529999867, 1436.133981643489960, 140.5568767735979918 ) ) ;
#83181=CARTESIAN_POINT ( 'NONE',  ( 8.664645897209998893, 1509.043692491530010, 182.0634199293980089 ) ) ;
#83184=CARTESIAN_POINT ( 'NONE',  ( -35.98267349529331227, 1456.700699973690234, 269.5452113222285675 ) ) ;
#83185=ORIENTED_EDGE ( 'NONE', *, *, #41926, .T. ) ;
#83186=CARTESIAN_POINT ( 'NONE',  ( 0.8167354255590000278, 1432.353341358199941, 150.3995506339979897 ) ) ;
#83187=CARTESIAN_POINT ( 'NONE',  ( -36.90170175143411768, 1420.766042611142893, 269.2061551430031159 ) ) ;
#83190=CARTESIAN_POINT ( 'NONE',  ( 11.60004869885204037, 1427.049244394422431, 134.3455896538280570 ) ) ;
#83191=CARTESIAN_POINT ( 'NONE',  ( -13.21072205002341171, 1443.129466954967029, 186.8022644757624562 ) ) ;
#83195=LINE ( 'NONE', #39539, #25282 ) ;
#83197=CARTESIAN_POINT ( 'NONE',  ( 24.09734436609999975, 1435.413501786879806, 137.5049309707980001 ) ) ;
#83199=CARTESIAN_POINT ( 'NONE',  ( -14.77051726120000019, 1409.598147220230203, 226.1676228370980084 ) ) ;
#83200=ORIENTED_EDGE ( 'NONE', *, *, #105523, .T. ) ;
#83201=CARTESIAN_POINT ( 'NONE',  ( -0.007886336557676770082, 1415.935475482089942, 191.2199948426670062 ) ) ;
#83205=CARTESIAN_POINT ( 'NONE',  ( 17.97699752310530030, 1415.938742849230039, 209.2714468986380041 ) ) ;
#83208=CARTESIAN_POINT ( 'NONE',  ( -26.58541136219999856, 1440.913060377119791, 225.2688052979979716 ) ) ;
#83210=CARTESIAN_POINT ( 'NONE',  ( -11.72951527989999754, 1433.271247870570051, 150.8356771812979957 ) ) ;
#83212=CARTESIAN_POINT ( 'NONE',  ( 17.60627569411529691, 1410.895669416499913, 224.1775087544040161 ) ) ;
#83214=CARTESIAN_POINT ( 'NONE',  ( -12.72284891840000043, 1416.311719779230089, 195.5584137648980061 ) ) ;
#83216=CARTESIAN_POINT ( 'NONE',  ( 1.939356653819999998, 1451.897712681530038, 183.5537167668979919 ) ) ;
#83218=CARTESIAN_POINT ( 'NONE',  ( -21.40871077047420812, 1509.777521100951390, 188.0411421299259302 ) ) ;
#83219=CARTESIAN_POINT ( 'NONE',  ( -2.679525294690940073E-09, 1415.359588412369931, 243.1548238962059827 ) ) ;
#83220=ORIENTED_EDGE ( 'NONE', *, *, #22765, .F. ) ;
#83221=ORIENTED_EDGE ( 'NONE', *, *, #19408, .F. ) ;
#83222=CARTESIAN_POINT ( 'NONE',  ( -11.85095945016420060, 1431.285170179160104, 149.8809506189519993 ) ) ;
#83225=CARTESIAN_POINT ( 'NONE',  ( -3.182038422270000222, 1473.815937567429955, 270.2907995558980474 ) ) ;
#83228=CARTESIAN_POINT ( 'NONE',  ( 36.89893150947609968, 1450.594831177580090, 135.9584847841670125 ) ) ;
#83229=DIRECTION ( 'NONE',  ( 0.4794255386042038380, 0.000000000000000000, 0.8775825618903722036 ) ) ;
#83234=CARTESIAN_POINT ( 'NONE',  ( -43.95932380871909828, 1429.872527714419903, 267.6715504426759935 ) ) ;
#83236=CARTESIAN_POINT ( 'NONE',  ( -13.80599379854099951, 1434.979619881170038, 146.4346930281899972 ) ) ;
#83237=ORIENTED_EDGE ( 'NONE', *, *, #109837, .F. ) ;
#83240=CARTESIAN_POINT ( 'NONE',  ( 4.640548489927184050, 1423.702551843624406, 183.8769998837497610 ) ) ;
#83243=CARTESIAN_POINT ( 'NONE',  ( -4.051722416713680275, 1441.572133640756192, 170.5366858311234353 ) ) ;
#83244=CARTESIAN_POINT ( 'NONE',  ( -18.18247686910000027, 1455.458619197430153, 190.5294738202979943 ) ) ;
#83246=ORIENTED_EDGE ( 'NONE', *, *, #96527, .F. ) ;
#83247=CARTESIAN_POINT ( 'NONE',  ( -26.05003822329999963, 1435.407090719000053, 135.4328170717980129 ) ) ;
#83253=CARTESIAN_POINT ( 'NONE',  ( -33.57555963875730498, 1421.581647479509911, 269.7571208528079865 ) ) ;
#83255=CARTESIAN_POINT ( 'NONE',  ( -5.492330765480000210, 1396.104856804229939, 199.1956356928480147 ) ) ;
#83256=CARTESIAN_POINT ( 'NONE',  ( 15.27152964737910068, 1506.433683733550197, 193.3098315259690025 ) ) ;
#83257=EDGE_LOOP ( 'NONE', ( #81568, #64365, #22709, #26783 ) ) ;
#83258=VERTEX_POINT ( 'NONE', #101250 ) ;
#83259=CARTESIAN_POINT ( 'NONE',  ( -11.87044479798669983, 1432.661806071300134, 149.9816004235700007 ) ) ;
#83262=CARTESIAN_POINT ( 'NONE',  ( -24.97832055750000180, 1436.146980076459840, 137.6305210645979855 ) ) ;
#83263=CARTESIAN_POINT ( 'NONE',  ( -24.31747465770000005, 1442.264844603690108, 211.7949302672280112 ) ) ;
#83266=CARTESIAN_POINT ( 'NONE',  ( 5.418632516149999745, 1435.861377308850024, 154.6842388019980206 ) ) ;
#83267=EDGE_CURVE ( 'NONE', #68340, #80530, #104170, .T. ) ;
#83269=CARTESIAN_POINT ( 'NONE',  ( -13.25967441350000087, 1414.983771848930019, 220.4242586862980033 ) ) ;
#83272=CARTESIAN_POINT ( 'NONE',  ( -40.71747597329999735, 1448.637563247749995, 134.0999997049979982 ) ) ;
#83275=ORIENTED_EDGE ( 'NONE', *, *, #69548, .T. ) ;
#83277=CARTESIAN_POINT ( 'NONE',  ( 12.95032542627530070, 1434.763327472709989, 149.4134100183379985 ) ) ;
#83278=CARTESIAN_POINT ( 'NONE',  ( 14.41084201949999866, 1416.311719782429918, 196.9001076125980205 ) ) ;
#83279=CARTESIAN_POINT ( 'NONE',  ( 18.18137294690000161, 1507.608465325429734, 188.5297611294979845 ) ) ;
#83281=CARTESIAN_POINT ( 'NONE',  ( 3.494924776181328241, 1450.853411195030276, 184.0590517355477971 ) ) ;
#83284=CARTESIAN_POINT ( 'NONE',  ( 23.33747645580530872, 1449.558087810723009, 217.2477752679129139 ) ) ;
#83286=CARTESIAN_POINT ( 'NONE',  ( 37.14919262310827008, 1450.989556404924770, 134.7273727559652059 ) ) ;
#83290=CARTESIAN_POINT ( 'NONE',  ( 2.370970874524634286, 1427.002265528474027, 134.0999999980980135 ) ) ;
#83294=AXIS2_PLACEMENT_3D ( 'NONE', #104862, #55580, #38199 ) ;
#83296=EDGE_CURVE ( 'NONE', #73043, #75650, #102378, .T. ) ;
#83297=CARTESIAN_POINT ( 'NONE',  ( -8561.628222781668228, 50.13405481564041821, 11261.64903810799478 ) ) ;
#83300=CARTESIAN_POINT ( 'NONE',  ( 18.79647799810000208, 1416.822690122329959, 209.8352284151899880 ) ) ;
#83302=CARTESIAN_POINT ( 'NONE',  ( 34.64222682503879724, 1440.913060385429844, 250.2068170142590020 ) ) ;
#83309=CARTESIAN_POINT ( 'NONE',  ( -19.59660595549623352, 1485.403676447882845, 190.1777878984926247 ) ) ;
#83313=CARTESIAN_POINT ( 'NONE',  ( -11.73605607501253800, 1425.975716723378582, 144.1609217550800395 ) ) ;
#83318=CARTESIAN_POINT ( 'NONE',  ( 23.84529322929999751, 1452.080364399029804, 136.9869226563980078 ) ) ;
#83322=EDGE_LOOP ( 'NONE', ( #110250, #78273, #73668, #106011 ) ) ;
#83323=CARTESIAN_POINT ( 'NONE',  ( -1.371718781699999834, 1452.291798068730031, 183.7871359344979965 ) ) ;
#83325=CARTESIAN_POINT ( 'NONE',  ( 19.80644525996869731, 1508.319852367809972, 229.3611815521799997 ) ) ;
#83326=ORIENTED_EDGE ( 'NONE', *, *, #29028, .T. ) ;
#83329=CARTESIAN_POINT ( 'NONE',  ( 34.39071349362669849, 1437.045099478719976, 136.5484881409109903 ) ) ;
#83330=CARTESIAN_POINT ( 'NONE',  ( -11.72470770320000000, 1437.821967610810134, 147.7443706334980220 ) ) ;
#83336=CARTESIAN_POINT ( 'NONE',  ( 8.512645889544598887, 1409.210328532190033, 196.8199130449370102 ) ) ;
#83337=CARTESIAN_POINT ( 'NONE',  ( 0.4960531002210000207, 1409.436441156229876, 185.2773253857980080 ) ) ;
#83340=CARTESIAN_POINT ( 'NONE',  ( 11.57667674939999891, 1432.352206966599852, 151.1966745221979807 ) ) ;
#83341=DIRECTION ( 'NONE',  ( -0.01305701037215670386, -0.0004560323763018947962, 0.9999146496149624586 ) ) ;
#83343=CARTESIAN_POINT ( 'NONE',  ( -0.8115383875230000044, 1428.579607037230062, 149.5143047311979672 ) ) ;
#83344=CARTESIAN_POINT ( 'NONE',  ( -7.439099705655682016, 1427.747574558798760, 134.0999999980980419 ) ) ;
#83345=CARTESIAN_POINT ( 'NONE',  ( -12.38857139729999979, 1434.838224429319780, 150.7171454246980034 ) ) ;
#83346=CARTESIAN_POINT ( 'NONE',  ( -1.384842749328709995E-10, 1466.428514968140007, 243.0202938729159996 ) ) ;
#83348=DIRECTION ( 'NONE',  ( -0.000000000000000000, 1.000000000000000000, 0.000000000000000000 ) ) ;
#83353=CARTESIAN_POINT ( 'NONE',  ( 13.67340988617599962, 1509.035597116779854, 233.8281335272939714 ) ) ;
#83357=B_SPLINE_CURVE_WITH_KNOTS ( 'NONE', 5,
 ( #43081, #18395, #25695, #86175, #10019, #94016, #52039, #51472, #85058, #34114, #35779, #101289, #7806, #110822, #17280 ),
 .UNSPECIFIED., .F., .F.,
 ( 6, 3, 3, 3, 6 ),
 ( -40.68480120859999971, -31.17413108959999946, -27.78806269829999920, -24.40199430689999716, -21.66346122957535059 ),
 .UNSPECIFIED. ) ;
#83361=CARTESIAN_POINT ( 'NONE',  ( 27.70845915349999800, 1431.442877780980098, 238.1060703150980089 ) ) ;
#83362=CARTESIAN_POINT ( 'NONE',  ( -0.5201890262859999448, 1489.031164216529987, 181.6009856616979903 ) ) ;
#83364=CARTESIAN_POINT ( 'NONE',  ( -2.576756359376459748, 1419.518892921469842, 186.1246943225270059 ) ) ;
#83365=CARTESIAN_POINT ( 'NONE',  ( -11.53417333799999867, 1422.407019910830059, 220.7517733711979986 ) ) ;
#83366=CARTESIAN_POINT ( 'NONE',  ( -29.52277910021149410, 1509.964081442534962, 206.5892769569061045 ) ) ;
#83368=CARTESIAN_POINT ( 'NONE',  ( -18.95884658670000178, 1416.837177087930058, 207.7798958566280021 ) ) ;
#83372=CARTESIAN_POINT ( 'NONE',  ( 15.93137308367099969, 1422.193468637389742, 227.6991775834419798 ) ) ;
#83373=CARTESIAN_POINT ( 'NONE',  ( 29.02628104525710029, 1509.926680456929944, 206.2525988547419900 ) ) ;
#83374=ORIENTED_EDGE ( 'NONE', *, *, #17846, .F. ) ;
#83377=CARTESIAN_POINT ( 'NONE',  ( -24.12229142288359895, 1410.858807618380069, 209.1426138600969864 ) ) ;
#83378=B_SPLINE_CURVE_WITH_KNOTS ( 'NONE', 3,
 ( #40194, #13311, #82751, #47506, #4932, #107393, #6042, #108502, #64876, #31788, #48054, #97883, #12790, #65979, #88941, #98983, #3871, #56456, #106300, #29583, #90591, #77123, #102835, #25576, #23921, #41847, #15520, #58116, #84403, #41304, #68188, #93342, #51349, #6594, #16071, #67621, #67075, #57573, #8228, #68730, #92249, #8782, #7690, #75477, #32884, #58663, #76549, #109071, #101180, #91697, #14972, #59226 ),
 .UNSPECIFIED., .F., .F.,
 ( 4, 2, 1, 1, 2, 2, 1, 1, 1, 2, 2, 2, 2, 2, 2, 1, 1, 2, 2, 2, 2, 1, 1, 1, 2, 2, 2, 1, 1, 2, 2, 4 ),
 ( 0.000000000000000000, 0.06249999999962202457, 0.09374999999942285056, 0.1093749999993230693, 0.1171874999993217648, 0.1249999999993204602, 0.1874999999986683430, 0.2187499999984028887, 0.2343749999982787102, 0.2421874999982251975, 0.2499999999981717125, 0.3124999999986546872, 0.3437499999989667154, 0.3749999999992787991, 0.4374999999999192313, 0.4687500000002467471, 0.4843750000005004885, 0.4921875000006212253, 0.5000000000007419620, 0.6250000000024934499, 0.6875000000033619774, 0.7187500000038832271, 0.7343750000041439074, 0.7421875000042691406, 0.7460937500042493786, 0.7500000000042296167, 0.8125000000035560443, 0.8437500000031180614, 0.8593750000028943514, 0.8671875000027038372, 0.8750000000025132119, 1.000000000000000000 ),
 .UNSPECIFIED. ) ;
#83380=DIRECTION ( 'NONE',  ( 0.000000000000000000, 1.000000000000000000, 0.000000000000000000 ) ) ;
#83382=CARTESIAN_POINT ( 'NONE',  ( -0.1019605806445679913, 1450.916620931209991, 185.2438843135239779 ) ) ;
#83387=EDGE_CURVE ( 'NONE', #30233, #61499, #59311, .T. ) ;
#83388=CARTESIAN_POINT ( 'NONE',  ( 46.12601432200399643, 1442.805762345989933, 266.9727633061970096 ) ) ;
#83390=CARTESIAN_POINT ( 'NONE',  ( 0.01016139356220000130, 1420.445651128929967, 183.2785305846980179 ) ) ;
#83391=( BOUNDED_SURFACE ( )  B_SPLINE_SURFACE ( 4, 2, ( 
 ( #54446, #10200, #62870 ),
 ( #97519, #37058, #61739 ),
 ( #46036, #62295, #43811 ),
 ( #96982, #105376, #70156 ),
 ( #88582, #10768, #80166 ) ),
 .UNSPECIFIED., .F., .F., .T. ) 
 B_SPLINE_SURFACE_WITH_KNOTS ( ( 5, 5 ),
 ( 3, 3 ),
 ( 1.967616199060000071, 3.613988937050000239 ),
 ( 5.300753508050029872, 6.148918325191019996 ),
 .UNSPECIFIED. ) 
 GEOMETRIC_REPRESENTATION_ITEM ( )  RATIONAL_B_SPLINE_SURFACE ( (
 ( 0.8627701935039280290, 0.8230948968151540202, 0.9542086668560899598),
 ( 0.8627701935039280290, 0.8230948968151540202, 0.9542086668560899598),
 ( 0.8627701935039280290, 0.8230948968151540202, 0.9542086668560899598),
 ( 0.8627701935039280290, 0.8230948968151540202, 0.9542086668560899598),
 ( 0.8627701935039280290, 0.8230948968151540202, 0.9542086668560899598) ) ) 
 REPRESENTATION_ITEM ( '' )  SURFACE ( )  );
#83393=ORIENTED_EDGE ( 'NONE', *, *, #107543, .T. ) ;
#83394=CARTESIAN_POINT ( 'NONE',  ( 18.40544744198233218, 1458.966239857264327, 227.7214915631488452 ) ) ;
#83397=ORIENTED_EDGE ( 'NONE', *, *, #75460, .F. ) ;
#83398=CARTESIAN_POINT ( 'NONE',  ( 2.664611940229999920, 1448.598609929289978, 183.3941765823980177 ) ) ;
#83399=CARTESIAN_POINT ( 'NONE',  ( 27.01855575919810093, 1451.963933047730052, 135.0858731167039934 ) ) ;
#83400=EDGE_CURVE ( 'NONE', #69273, #96354, #5572, .T. ) ;
#83402=CIRCLE ( 'NONE', #103058, 2.027965567643763567 ) ;
#83408=CARTESIAN_POINT ( 'NONE',  ( 1.890470286680180134, 1408.979077064439934, 186.8977652987280180 ) ) ;
#83409=CARTESIAN_POINT ( 'NONE',  ( -16.70783830106690004, 1412.306682225960003, 191.6972782329859797 ) ) ;
#83413=CARTESIAN_POINT ( 'NONE',  ( 2.439001525050000119, 1430.488531030629929, 150.2249694046979869 ) ) ;
#83415=CARTESIAN_POINT ( 'NONE',  ( 6.215408291180000155, 1427.423536210829980, 214.3676144191779827 ) ) ;
#83416=FACE_OUTER_BOUND ( 'NONE', #1204, .T. ) ;
#83423=FACE_OUTER_BOUND ( 'NONE', #65623, .T. ) ;
#83424=CARTESIAN_POINT ( 'NONE',  ( 11.93338584299999994, 1433.461450241920147, 149.9037928783980078 ) ) ;
#83425=CARTESIAN_POINT ( 'NONE',  ( 18.93537658700000037, 1468.059964608529981, 268.3665355201979992 ) ) ;
#83428=CARTESIAN_POINT ( 'NONE',  ( -14.92155151558594106, 1422.314549108387382, 229.4637292657217813 ) ) ;
#83429=CARTESIAN_POINT ( 'NONE',  ( -17.74532079129999929, 1486.483557334729994, 188.0959163475980063 ) ) ;
#83430=CARTESIAN_POINT ( 'NONE',  ( 10.37251527352099956, 1441.250888917769998, 153.2543604269490061 ) ) ;
#83431=CARTESIAN_POINT ( 'NONE',  ( -17.25956576649999974, 1409.515777705929850, 224.0944197546979808 ) ) ;
#83432=CARTESIAN_POINT ( 'NONE',  ( 4.283856666023710069, 1440.956247486469920, 155.9231014612180104 ) ) ;
#83436=CARTESIAN_POINT ( 'NONE',  ( 12.78667967550000029, 1416.822694282129987, 222.9174006480979813 ) ) ;
#83439=DIRECTION ( 'NONE',  ( 0.8771707526546712597, 0.03063147977167200720, -0.4792005667090091237 ) ) ;
#83440=CARTESIAN_POINT ( 'NONE',  ( 0.2063577645740160005, 1459.399669238419847, 182.9788367490870087 ) ) ;
#83442=ORIENTED_EDGE ( 'NONE', *, *, #93355, .F. ) ;
#83443=CARTESIAN_POINT ( 'NONE',  ( -27.40283359139997543, 1444.740067931808653, 161.6370709818978639 ) ) ;
#83444=CARTESIAN_POINT ( 'NONE',  ( -28.01253743957580156, 1509.025311965089941, 210.6956320615649929 ) ) ;
#83445=CARTESIAN_POINT ( 'NONE',  ( 11.87564264789999946, 1433.006668304930145, 147.6243415688980178 ) ) ;
#83446=CARTESIAN_POINT ( 'NONE',  ( -41.10614458632299772, 1440.770232259229942, 134.0999999980669770 ) ) ;
#83448=EDGE_LOOP ( 'NONE', ( #87898, #68824, #80716, #25794 ) ) ;
#83455=CARTESIAN_POINT ( 'NONE',  ( 38.84918024652115065, 1422.961239324861481, 269.1580888396505316 ) ) ;
#83458=CARTESIAN_POINT ( 'NONE',  ( 3.426760023489999973, 1434.222170298339961, 184.7792794946979882 ) ) ;
#83460=CARTESIAN_POINT ( 'NONE',  ( 12.51099983133400073, 1416.825784014559986, 196.0986189223339977 ) ) ;
#83462=VERTEX_POINT ( 'NONE', #16153 ) ;
#83463=CARTESIAN_POINT ( 'NONE',  ( -33.93392822810000098, 1451.575813952230192, 135.5854759724980170 ) ) ;
#83464=CARTESIAN_POINT ( 'NONE',  ( -15.88978672354079968, 1409.721424571740044, 226.1318342661600127 ) ) ;
#83472=CARTESIAN_POINT ( 'NONE',  ( -0.08002646896166820678, 1420.301969961120221, 183.4692128524420127 ) ) ;
#83474=CARTESIAN_POINT ( 'NONE',  ( 17.98939361210000243, 1410.465183417029948, 222.9682872111980032 ) ) ;
#83475=CARTESIAN_POINT ( 'NONE',  ( 0.3919100467378520136, 1450.899374586919976, 181.2708617675390030 ) ) ;
#83476=CARTESIAN_POINT ( 'NONE',  ( -17.48680721799999915, 1424.154378231430201, 227.6286878164980010 ) ) ;
#83484=CARTESIAN_POINT ( 'NONE',  ( -5.567394890084230497, 1485.997473811110240, 182.5242378165860089 ) ) ;
#83485=ORIENTED_EDGE ( 'NONE', *, *, #82851, .T. ) ;
#83487=CARTESIAN_POINT ( 'NONE',  ( -4.236735269543610016, 1441.469422925089930, 163.3606698496620027 ) ) ;
#83494=CARTESIAN_POINT ( 'NONE',  ( -11.74088322070292634, 1426.277669831848698, 144.4824319529912202 ) ) ;
#83495=CARTESIAN_POINT ( 'NONE',  ( 15.85651032225270107, 1410.713550775690010, 191.5263126459360024 ) ) ;
#83498=CARTESIAN_POINT ( 'NONE',  ( 41.66793448034960079, 1443.219079709529979, 135.6262679568360170 ) ) ;
#83499=CARTESIAN_POINT ( 'NONE',  ( -11.15486294749999985, 1425.160588235329897, 144.1660541355979888 ) ) ;
#83501=CARTESIAN_POINT ( 'NONE',  ( 4.383261023904437614, 1466.449861621304308, 233.9444969100850642 ) ) ;
#83503=EDGE_CURVE ( 'NONE', #15766, #92171, #36958, .T. ) ;
#83505=CARTESIAN_POINT ( 'NONE',  ( -2.500000000000000000, 1443.913060387330006, 150.6726614421979775 ) ) ;
#83506=ORIENTED_EDGE ( 'NONE', *, *, #91939, .T. ) ;
#83509=ORIENTED_EDGE ( 'NONE', *, *, #62050, .T. ) ;
#83511=LINE ( 'NONE', #40965, #7342 ) ;
#83514=FACE_OUTER_BOUND ( 'NONE', #54121, .T. ) ;
#83516=CARTESIAN_POINT ( 'NONE',  ( -2.500000000000000000, 1439.402073989899918, 161.8071971399309916 ) ) ;
#83519=CARTESIAN_POINT ( 'NONE',  ( -26.74681214179999955, 1508.000506563529825, 202.6166866765980217 ) ) ;
#83520=CARTESIAN_POINT ( 'NONE',  ( 38.81202640299100182, 1436.797832147280133, 135.6938345645050106 ) ) ;
#83521=CARTESIAN_POINT ( 'NONE',  ( 2.502076662800340134, 1421.306659195480051, 183.2871562736519877 ) ) ;
#83525=EDGE_LOOP ( 'NONE', ( #68177, #48516, #15786, #51337, #65592, #39853, #28593, #61259 ) ) ;
#83528=VERTEX_POINT ( 'NONE', #43047 ) ;
#83530=CARTESIAN_POINT ( 'NONE',  ( -0.002089120988227474544, 1451.815318029500077, 154.0389770418792921 ) ) ;
#83532=CARTESIAN_POINT ( 'NONE',  ( -14.08840122829999864, 1415.996778985530000, 221.5650976514979789 ) ) ;
#83534=CARTESIAN_POINT ( 'NONE',  ( -11.84451602989710040, 1432.336085667850057, 150.3016814433159993 ) ) ;
#83538=CARTESIAN_POINT ( 'NONE',  ( 14.13657958834579986, 1436.257374515989795, 150.1576261981630012 ) ) ;
#83541=CARTESIAN_POINT ( 'NONE',  ( 24.17850564169770067, 1447.751960943020094, 206.2131088459789794 ) ) ;
#83542=CARTESIAN_POINT ( 'NONE',  ( 13.72863203839999890, 1461.767185418329973, 230.8959970784979987 ) ) ;
#83543=CARTESIAN_POINT ( 'NONE',  ( -12.25009443214260152, 1507.051235695380001, 190.1744699773550167 ) ) ;
#83544=CARTESIAN_POINT ( 'NONE',  ( -4.644457551160845910, 1422.126592464929672, 184.6658150771102953 ) ) ;
#83552=CARTESIAN_POINT ( 'NONE',  ( 18.51267882970000045, 1508.236097878829924, 188.5103842655979918 ) ) ;
#83556=CARTESIAN_POINT ( 'NONE',  ( 0.9136860870960000769, 1489.469559537029909, 187.0247168341979886 ) ) ;
#83558=CARTESIAN_POINT ( 'NONE',  ( -11.56091194390000076, 1431.144279896319858, 151.0927142626980242 ) ) ;
#83561=CARTESIAN_POINT ( 'NONE',  ( 9.236167301360001858, 1423.625854809029988, 144.1549878472980026 ) ) ;
#83563=CARTESIAN_POINT ( 'NONE',  ( 12.29928450579999932, 1445.315142612919999, 187.0920815097979926 ) ) ;
#83565=CARTESIAN_POINT ( 'NONE',  ( -26.64855247050000386, 1508.005992643229774, 213.8736264213379741 ) ) ;
#83567=AXIS2_PLACEMENT_3D ( 'NONE', #7563, #92121, #15397 ) ;
#83571=CARTESIAN_POINT ( 'NONE',  ( 12.67137506719999962, 1407.308516313030168, 266.8981195266979967 ) ) ;
#83573=CARTESIAN_POINT ( 'NONE',  ( 0.1796731001380000026, 1410.302589273230069, 185.0125001767980280 ) ) ;
#83575=CARTESIAN_POINT ( 'NONE',  ( 24.46704740869997963, 1438.251643707298626, 212.7269232099579881 ) ) ;
#83578=CARTESIAN_POINT ( 'NONE',  ( 17.96267386539620503, 1457.880262292270345, 230.1796244582303927 ) ) ;
#83580=CARTESIAN_POINT ( 'NONE',  ( -13.47721440219999955, 1444.366909545699855, 187.4582783821979888 ) ) ;
#83581=CARTESIAN_POINT ( 'NONE',  ( -19.84205502019262823, 1485.634645662600633, 190.5026249870552704 ) ) ;
#83586=CARTESIAN_POINT ( 'NONE',  ( -26.93833921311239976, 1508.003628666910117, 211.6437312287430075 ) ) ;
#83587=CARTESIAN_POINT ( 'NONE',  ( -3.756925840770000136, 1475.646169757629877, 269.0400499448979872 ) ) ;
#83588=CARTESIAN_POINT ( 'NONE',  ( -4.221461939218559500, 1446.221127877819981, 168.5609095037160046 ) ) ;
#83591=CARTESIAN_POINT ( 'NONE',  ( 17.64653741881929960, 1410.885868213330014, 223.6671089294119952 ) ) ;
#83594=AXIS2_PLACEMENT_3D ( 'NONE', #86402, #16955, #34894 ) ;
#83595=CARTESIAN_POINT ( 'NONE',  ( 16.49511133113979966, 1507.275789587220061, 193.5424140907059893 ) ) ;
#83596=CARTESIAN_POINT ( 'NONE',  ( -25.28355254197510149, 1470.075220752909900, 211.5054833620599766 ) ) ;
#83598=CARTESIAN_POINT ( 'NONE',  ( -45.67177343128329881, 1440.913044206929953, 266.1885934837860077 ) ) ;
#83599=EDGE_CURVE ( 'NONE', #43475, #13362, #22623, .T. ) ;
#83600=CARTESIAN_POINT ( 'NONE',  ( -21.22058966110000000, 1410.149336617530025, 200.8725164463980093 ) ) ;
#83601=EDGE_CURVE ( 'NONE', #63032, #71548, #49907, .T. ) ;
#83603=CARTESIAN_POINT ( 'NONE',  ( -15.23376569592200092, 1422.124418483453837, 227.7537583617639996 ) ) ;
#83606=CARTESIAN_POINT ( 'NONE',  ( -4.163396682581677943, 1410.434738167183923, 232.1586877586055095 ) ) ;
#83607=EDGE_CURVE ( 'NONE', #16982, #48606, #17659, .T. ) ;
#83615=CARTESIAN_POINT ( 'NONE',  ( 40.16554548739999575, 1445.100731327120002, 136.9467556218980064 ) ) ;
#83617=CARTESIAN_POINT ( 'NONE',  ( -0.03232799881073839671, 1407.837594165210248, 222.3069522186050051 ) ) ;
#83619=CARTESIAN_POINT ( 'NONE',  ( 0.000000000000000000, 1440.913060387330006, 134.0999999980979851 ) ) ;
#83625=CARTESIAN_POINT ( 'NONE',  ( 20.50777286777820052, 1509.292534432200227, 229.3763492124210188 ) ) ;
#83628=ORIENTED_EDGE ( 'NONE', *, *, #86576, .T. ) ;
#83630=CARTESIAN_POINT ( 'NONE',  ( 11.21685831077579820, 1434.247512195129957, 151.6038547891890005 ) ) ;
#83631=CARTESIAN_POINT ( 'NONE',  ( -12.90441353309999961, 1397.988352241829944, 211.5057569300479940 ) ) ;
#83632=CARTESIAN_POINT ( 'NONE',  ( -19.38290977210000321, 1410.951314247329947, 222.2178025500979857 ) ) ;
#83633=ORIENTED_EDGE ( 'NONE', *, *, #83601, .F. ) ;
#83634=CARTESIAN_POINT ( 'NONE',  ( -13.21180937474541572, 1444.695490197944309, 169.3896175514511242 ) ) ;
#83635=CARTESIAN_POINT ( 'NONE',  ( 21.52065832966763637, 1509.707847311939531, 229.6525536875780631 ) ) ;
#83638=CARTESIAN_POINT ( 'NONE',  ( -14.16428767310739900, 1509.316879318749898, 183.3251262769900052 ) ) ;
#83640=CARTESIAN_POINT ( 'NONE',  ( 1.016818722979999867, 1449.241593506360005, 183.5274279965980213 ) ) ;
#83644=CARTESIAN_POINT ( 'NONE',  ( 10.52768771694820060, 1396.280695343850084, 212.5326781301700123 ) ) ;
#83645=EDGE_CURVE ( 'NONE', #95978, #102807, #35592, .T. ) ;
#83646=CARTESIAN_POINT ( 'NONE',  ( -1.270728281904929924, 1414.996443537369942, 226.4582996361970118 ) ) ;
#83647=CARTESIAN_POINT ( 'NONE',  ( 11.57651590190000057, 1432.340302014539930, 151.1968537399980050 ) ) ;
#83650=CARTESIAN_POINT ( 'NONE',  ( 13.20770753281709986, 1435.164461038139962, 150.0426743444330384 ) ) ;
#83651=VERTEX_POINT ( 'NONE', #64831 ) ;
#83654=CARTESIAN_POINT ( 'NONE',  ( -19.35158686409289786, 1497.937538563279986, 229.1472795281780179 ) ) ;
#83655=CARTESIAN_POINT ( 'NONE',  ( -4.919574813549999703, 1465.704333999829942, 234.5361420446980105 ) ) ;
#83662=CARTESIAN_POINT ( 'NONE',  ( 2.500000000000000000, 1448.375488404329872, 162.6818385019500113 ) ) ;
#83666=ORIENTED_EDGE ( 'NONE', *, *, #23447, .T. ) ;
#83668=CARTESIAN_POINT ( 'NONE',  ( -20.20853920450000274, 1508.359852705729736, 228.9359805712980176 ) ) ;
#83669=CARTESIAN_POINT ( 'NONE',  ( -9.200229741499999392, 1410.168877032430146, 188.1184974272979957 ) ) ;
#83670=CARTESIAN_POINT ( 'NONE',  ( -0.2331131841380000014, 1408.921200879130083, 231.7611516523979844 ) ) ;
#83671=CARTESIAN_POINT ( 'NONE',  ( -0.1620860067307069718, 1416.842625005220043, 227.3681785903409889 ) ) ;
#83673=CARTESIAN_POINT ( 'NONE',  ( 20.22892916700000043, 1427.700964219130128, 222.9554382744980217 ) ) ;
#83676=FACE_OUTER_BOUND ( 'NONE', #73086, .T. ) ;
#83677=AXIS2_PLACEMENT_3D ( 'NONE', #27024, #52783, #62309 ) ;
#83678=CARTESIAN_POINT ( 'NONE',  ( 8.240145091180000492, 1408.795471539129949, 270.3822351589980144 ) ) ;
#83681=CARTESIAN_POINT ( 'NONE',  ( 24.04558608239999984, 1411.114406507129843, 208.5460494714599804 ) ) ;
#83682=EDGE_CURVE ( 'NONE', #109412, #96903, #89230, .T. ) ;
#83683=CARTESIAN_POINT ( 'NONE',  ( 0.02057132068849890430, 1507.157206512230232, 237.3547131625103646 ) ) ;
#83689=EDGE_CURVE ( 'NONE', #8151, #36202, #16979, .T. ) ;
#83691=CARTESIAN_POINT ( 'NONE',  ( 0.5085445767741282319, 1408.930819155293875, 231.7415010692618296 ) ) ;
#83693=ORIENTED_EDGE ( 'NONE', *, *, #72708, .F. ) ;
#83699=CARTESIAN_POINT ( 'NONE',  ( -24.02706688199999974, 1444.687161772040099, 212.1394894004279763 ) ) ;
#83711=CARTESIAN_POINT ( 'NONE',  ( -0.2712367748239999932, 1477.407383352130182, 230.1216438035979763 ) ) ;
#83712=CARTESIAN_POINT ( 'NONE',  ( 21.99352617080000272, 1452.352678890530115, 220.2843750103979801 ) ) ;
#83714=CARTESIAN_POINT ( 'NONE',  ( 7.556399103406818085, 1438.573724557855030, 153.9060459267900853 ) ) ;
#83717=CARTESIAN_POINT ( 'NONE',  ( 15.57452430335069415, 1420.988626805493368, 227.6587458589921482 ) ) ;
#83718=CARTESIAN_POINT ( 'NONE',  ( 29.18247107518470074, 1435.677098379100016, 136.0908610070169971 ) ) ;
#83719=EDGE_CURVE ( 'NONE', #10158, #98691, #64231, .T. ) ;
#83721=CARTESIAN_POINT ( 'NONE',  ( -21.39355008749999953, 1429.473757846430090, 219.8698122737980043 ) ) ;
#83724=CARTESIAN_POINT ( 'NONE',  ( -17.30756165510000244, 1415.800549802929936, 226.2855322628980161 ) ) ;
#83726=CARTESIAN_POINT ( 'NONE',  ( -35.03237507324672606, 1457.739610860745643, 269.5320035884349750 ) ) ;
#83730=CARTESIAN_POINT ( 'NONE',  ( 8.972793222467396745, 1506.569407720433446, 188.9290252029455246 ) ) ;
#83733=CARTESIAN_POINT ( 'NONE',  ( -4.762729318109999888, 1475.513060387329915, 229.9230423263979901 ) ) ;
#83734=CARTESIAN_POINT ( 'NONE',  ( -15.10152500592460711, 1451.764323980957215, 222.8996944938442937 ) ) ;
#83735=CARTESIAN_POINT ( 'NONE',  ( -28.82461960859999905, 1509.587741801030006, 208.9199936958729893 ) ) ;
#83738=CARTESIAN_POINT ( 'NONE',  ( -5.563644771257700405, 1416.329487563220937, 231.9365388964823467 ) ) ;
#83739=CARTESIAN_POINT ( 'NONE',  ( -22.83007936460490583, 1450.886360539059751, 142.2906941818467317 ) ) ;
#83740=CARTESIAN_POINT ( 'NONE',  ( 23.69434222019999936, 1435.324930578030035, 137.3226534152980207 ) ) ;
#83741=EDGE_CURVE ( 'NONE', #5014, #104178, #97421, .T. ) ;
#83742=CARTESIAN_POINT ( 'NONE',  ( -12.88149101045983969, 1442.882090648938174, 169.4389559976919202 ) ) ;
#83743=CARTESIAN_POINT ( 'NONE',  ( -15.10324083849999965, 1409.440477179229902, 225.7327363557979822 ) ) ;
#83744=EDGE_LOOP ( 'NONE', ( #52006, #59993, #86434, #63678 ) ) ;
#83745=CARTESIAN_POINT ( 'NONE',  ( -0.1744917581095109804, 1415.933499560010205, 191.2651992481820002 ) ) ;
#83748=ORIENTED_EDGE ( 'NONE', *, *, #97588, .F. ) ;
#83750=CARTESIAN_POINT ( 'NONE',  ( 18.05420922962109742, 1416.521607925270018, 208.9025094127229920 ) ) ;
#83755=CARTESIAN_POINT ( 'NONE',  ( -11.63091869309999993, 1433.120749602059959, 151.0277071862979881 ) ) ;
#83761=CARTESIAN_POINT ( 'NONE',  ( -24.46878230119999742, 1438.129412883440182, 210.7492543162080096 ) ) ;
#83763=CARTESIAN_POINT ( 'NONE',  ( 1.420881903539999991, 1452.418224524330071, 183.4780528254979970 ) ) ;
#83766=EDGE_CURVE ( 'NONE', #66886, #18900, #28466, .T. ) ;
#83767=CARTESIAN_POINT ( 'NONE',  ( -29.01830120112816758, 1510.037320134664242, 216.7338135098987095 ) ) ;
#83771=CARTESIAN_POINT ( 'NONE',  ( -11.83486635870610115, 1430.212806064799906, 149.5583259460390195 ) ) ;
#83774=CARTESIAN_POINT ( 'NONE',  ( -4.128050607539999639, 1471.647764304730117, 269.8667864051980132 ) ) ;
#83775=CARTESIAN_POINT ( 'NONE',  ( 12.71038982811789886, 1507.471771741610155, 233.3404631503599944 ) ) ;
#83777=CARTESIAN_POINT ( 'NONE',  ( 41.42720720492820163, 1445.199782766380167, 136.3775557862170160 ) ) ;
#83778=CARTESIAN_POINT ( 'NONE',  ( 19.47227132649999959, 1453.313060387329870, 205.4425732447180053 ) ) ;
#83783=CARTESIAN_POINT ( 'NONE',  ( -33.69037434309119305, 1416.536361657399766, 267.3739642188930361 ) ) ;
#83787=ORIENTED_EDGE ( 'NONE', *, *, #13053, .F. ) ;
#83788=EDGE_LOOP ( 'NONE', ( #74991, #9401, #50076 ) ) ;
#83792=EDGE_CURVE ( 'NONE', #84504, #27375, #108887, .T. ) ;
#83795=CARTESIAN_POINT ( 'NONE',  ( -17.83707058670000123, 1485.487226716729992, 188.7688766075980027 ) ) ;
#83796=CARTESIAN_POINT ( 'NONE',  ( -16.79675064196879930, 1489.050962929880143, 229.2737794733750150 ) ) ;
#83806=ORIENTED_EDGE ( 'NONE', *, *, #100669, .T. ) ;
#83807=FACE_OUTER_BOUND ( 'NONE', #67154, .T. ) ;
#83808=CARTESIAN_POINT ( 'NONE',  ( 19.85917061082260560, 1471.740793072367751, 269.5234486458308538 ) ) ;
#83810=CARTESIAN_POINT ( 'NONE',  ( -12.90095066418269987, 1435.961952425909885, 150.7867089012090105 ) ) ;
#83811=CARTESIAN_POINT ( 'NONE',  ( -24.41126177309999790, 1441.219864611299954, 212.0468573069780120 ) ) ;
#83814=DIRECTION ( 'NONE',  ( 0.000000000000000000, 2.109423746789999926E-15, -1.000000000000000000 ) ) ;
#83816=DIRECTION ( 'NONE',  ( 0.000000000000000000, 0.000000000000000000, -1.000000000000000000 ) ) ;
#83819=CARTESIAN_POINT ( 'NONE',  ( -2.291311050504480029, 1451.952740248410009, 184.5693412410579697 ) ) ;
#83820=CARTESIAN_POINT ( 'NONE',  ( -11.29523006607699998, 1425.738182144259781, 112.3423121099719850 ) ) ;
#83821=CARTESIAN_POINT ( 'NONE',  ( -19.93790229973292583, 1456.566460236430203, 225.3001283633010985 ) ) ;
#83822=ORIENTED_EDGE ( 'NONE', *, *, #94264, .F. ) ;
#83824=CARTESIAN_POINT ( 'NONE',  ( -21.39772323737049931, 1509.704958956720020, 229.7894127843639751 ) ) ;
#83826=CARTESIAN_POINT ( 'NONE',  ( 2.742624438480730120, 1469.000773353729983, 234.2676976455010163 ) ) ;
#83831=CARTESIAN_POINT ( 'NONE',  ( 4.283856666023710069, 1440.956247486469920, 155.9231014612180104 ) ) ;
#83833=CARTESIAN_POINT ( 'NONE',  ( -11.88064286090000010, 1433.444786854229960, 151.0525681022980109 ) ) ;
#83838=CARTESIAN_POINT ( 'NONE',  ( -12.78730321389999958, 1416.837309283630020, 195.3260687431979932 ) ) ;
#83839=CARTESIAN_POINT ( 'NONE',  ( 16.05363106209999557, 1409.473654529731448, 193.0726681433975784 ) ) ;
#83849=CARTESIAN_POINT ( 'NONE',  ( 18.40645885720379837, 1425.561895475727397, 224.9115623075386452 ) ) ;
#83851=CARTESIAN_POINT ( 'NONE',  ( 39.36215256232259918, 1440.913060371679876, 258.3690201510549969 ) ) ;
#83853=CARTESIAN_POINT ( 'NONE',  ( -12.98226713004480004, 1414.913060387349788, 219.9156686614909972 ) ) ;
#83854=CARTESIAN_POINT ( 'NONE',  ( 12.81144342830000049, 1416.820969729830040, 221.9974425081979916 ) ) ;
#83857=CARTESIAN_POINT ( 'NONE',  ( 16.50080780802032976, 1409.524096883290667, 193.0397102418697273 ) ) ;
#83858=CARTESIAN_POINT ( 'NONE',  ( 4.363122647530000009, 1407.471318475729959, 146.1721969590979882 ) ) ;
#83859=CARTESIAN_POINT ( 'NONE',  ( -0.8262471098266214176, 1416.839570617953314, 228.0322529358493853 ) ) ;
#83862=CARTESIAN_POINT ( 'NONE',  ( 12.94448954231351223, 1519.913060387329779, 232.8165751327380519 ) ) ;
#83865=CARTESIAN_POINT ( 'NONE',  ( -13.34812806750000114, 1435.002040243610054, 194.7561373876979758 ) ) ;
#83869=ORIENTED_EDGE ( 'NONE', *, *, #79857, .T. ) ;
#83870=CARTESIAN_POINT ( 'NONE',  ( -1.453934354320000066, 1450.715845829520049, 182.8043077764980069 ) ) ;
#83871=EDGE_CURVE ( 'NONE', #100575, #49285, #66707, .T. ) ;
#83879=CARTESIAN_POINT ( 'NONE',  ( 11.68639022145140061, 1416.948096802429973, 206.9947965055779946 ) ) ;
#83880=FACE_OUTER_BOUND ( 'NONE', #40239, .T. ) ;
#83881=B_SPLINE_CURVE_WITH_KNOTS ( 'NONE', 5,
 ( #57479, #15427, #6496, #32252, #66975, #109515 ),
 .UNSPECIFIED., .F., .F.,
 ( 6, 6 ),
 ( -10.10903599265445862, 0.000000000000000000 ),
 .UNSPECIFIED. ) ;
#83887=CARTESIAN_POINT ( 'NONE',  ( -0.3338142544270000234, 1475.117443318730011, 235.9516215253979965 ) ) ;
#83888=CARTESIAN_POINT ( 'NONE',  ( 18.12084340177599984, 1425.008237496925858, 225.3902487627179880 ) ) ;
#83889=CARTESIAN_POINT ( 'NONE',  ( 4.218089546350000774, 1425.254492614629953, 185.4299342609980101 ) ) ;
#83891=CARTESIAN_POINT ( 'NONE',  ( 11.30175581209999969, 1432.339690545260055, 151.5220148439979937 ) ) ;
#83894=CARTESIAN_POINT ( 'NONE',  ( -3.053802859332280129, 1450.477919606039904, 184.6720589006399678 ) ) ;
#83896=CARTESIAN_POINT ( 'NONE',  ( -0.8041763403130000043, 1426.566393376330097, 144.1938086916980239 ) ) ;
#83897=CARTESIAN_POINT ( 'NONE',  ( 19.03816721145270208, 1457.216680265689774, 226.4213465897580022 ) ) ;
#83898=FACE_OUTER_BOUND ( 'NONE', #45682, .T. ) ;
#83900=CARTESIAN_POINT ( 'NONE',  ( -2.503156170453839640E-09, 1471.497077799589988, 257.8074999948410095 ) ) ;
#83906=CARTESIAN_POINT ( 'NONE',  ( -45.88366687282530165, 1440.699494908059933, 266.4123290765789989 ) ) ;
#83910=B_SPLINE_CURVE_WITH_KNOTS ( 'NONE', 3,
 ( #7440, #41604, #32646, #73139, #64766, #51112, #110452, #42705, #8530, #59516, #90475, #82071, #66823, #75758, #34293, #68476, #98877, #102577, #30576, #109904, #58958, #24223, #56343, #101473, #60075, #5376, #13750, #33185, #33731, #16906, #67924, #58410, #92534, #15802, #7985, #85236, #93091, #47936, #93628, #81512, #25873, #39534, #38961, #107282, #54249, #2742, #37424, #96223, #36308, #45290, #79431, #53133, #78888, #104620, #79974, #18382, #20055, #2194, #52578, #77768, #1079, #86713, #78313, #88375, #44738, #27916, #10005, #36863, #95118, #70503, #3292, #87270, #11131, #45841, #17821, #28470, #60992, #44176, #71056, #19500, #10564, #62099, #52022, #18938, #11665, #53702, #87843, #105179, #61539, #62662, #96784, #94548, #86162, #102939, #26241, #35764, #104062 ),
 .UNSPECIFIED., .F., .F.,
 ( 4, 3, 3, 3, 3, 3, 3, 3, 3, 3, 3, 3, 3, 3, 3, 3, 3, 3, 3, 3, 3, 3, 3, 3, 3, 3, 3, 3, 3, 3, 3, 3, 4 ),
 ( 31.89279723145740064, 34.15041588771699566, 37.70401514765850237, 40.03546223828480066, 42.06456480448240143, 43.93975577359619678, 45.67355729532359732, 47.34970776216830046, 48.95441885073729793, 50.14584306709999595, 51.69408452324559988, 53.32263554308429576, 55.06445428949349719, 57.02053842314010268, 59.91870409476419468, 62.02803367172320748, 63.82160321651739565, 65.49947758280899279, 67.05801106692298674, 68.35602240260000428, 71.04588944904199366, 73.84938310448460186, 76.80220749988789919, 79.96770714888299381, 83.54395628944999430, 88.79562199458749205, 92.73437127344060116, 95.91053324874698660, 98.89661206464120369, 101.7236155873209782, 104.5506191099999853, 107.1327756825400002, 108.8243481894799913 ),
 .UNSPECIFIED. ) ;
#83911=CARTESIAN_POINT ( 'NONE',  ( 2.605323841626010495, 1407.938395893999996, 222.1469575270010068 ) ) ;
#83912=EDGE_CURVE ( 'NONE', #92743, #17250, #41300, .T. ) ;
#83913=CARTESIAN_POINT ( 'NONE',  ( 2.885914701209999933, 1421.960919705029937, 112.2554183042980185 ) ) ;
#83916=CARTESIAN_POINT ( 'NONE',  ( -26.48819218400589648, 1451.824455620959952, 135.6820404289399846 ) ) ;
#83919=CARTESIAN_POINT ( 'NONE',  ( 20.65399528909999916, 1428.491072936029923, 221.4883061032980152 ) ) ;
#83920=CARTESIAN_POINT ( 'NONE',  ( 0.4810529050879999713, 1489.033618959729893, 181.7121226793979929 ) ) ;
#83923=CARTESIAN_POINT ( 'NONE',  ( -2.178334822207929733, 1419.510208088270019, 185.9423002976799921 ) ) ;
#83924=CARTESIAN_POINT ( 'NONE',  ( -20.42128912490000303, 1430.525542552929892, 211.9067694171880021 ) ) ;
#83926=CARTESIAN_POINT ( 'NONE',  ( -14.28944682607799876, 1452.414061908529902, 148.3378489825130089 ) ) ;
#83927=CARTESIAN_POINT ( 'NONE',  ( -25.00976051679999657, 1436.598010167069788, 137.9330532114979917 ) ) ;
#83928=ORIENTED_EDGE ( 'NONE', *, *, #94463, .F. ) ;
#83930=CARTESIAN_POINT ( 'NONE',  ( 13.27836209250000010, 1419.795885124230153, 228.8595217210979911 ) ) ;
#83934=B_SPLINE_CURVE_WITH_KNOTS ( 'NONE', 3,
 ( #75371, #42298, #58014, #76450, #7589, #59667, #75903, #59124, #49614, #93245, #40643, #92150, #109510, #33887, #42861, #68083, #8679, #31684, #93777, #65866, #74814, #91599, #108960, #32247, #66427, #87626, #36117, #19845, #96572 ),
 .UNSPECIFIED., .F., .F.,
 ( 4, 2, 2, 2, 1, 1, 2, 2, 2, 2, 1, 1, 1, 2, 2, 2, 4 ),
 ( 0.000000000000000000, 0.2499999999998866462, 0.3749999999998336331, 0.4374999999997182809, 0.4687499999996613265, 0.4843749999996329048, 0.4921874999996959654, 0.4999999999997590261, 0.6250000000015900614, 0.6875000000025056623, 0.7187500000029128921, 0.7343750000031081804, 0.7421875000031570302, 0.7460937500031412650, 0.7500000000031254999, 0.8750000000015626389, 1.000000000000000000 ),
 .UNSPECIFIED. ) ;
#83936=CARTESIAN_POINT ( 'NONE',  ( -23.01639577485230248, 1409.746539370839855, 209.2889146252420005 ) ) ;
#83937=ORIENTED_EDGE ( 'NONE', *, *, #88292, .F. ) ;
#83938=DIRECTION ( 'NONE',  ( -0.7067700363771036720, 0.03085824620770448792, -0.7067700363771036720 ) ) ;
#83941=CARTESIAN_POINT ( 'NONE',  ( -0.1201301491520000014, 1498.355800884429982, 236.9777592396980310 ) ) ;
#83944=CARTESIAN_POINT ( 'NONE',  ( 44.80943101484369606, 1448.445176812669843, 268.7884264490030546 ) ) ;
#83948=VERTEX_POINT ( 'NONE', #67575 ) ;
#83949=CARTESIAN_POINT ( 'NONE',  ( 18.50997094255976450, 1458.745266264683323, 227.6095332770021287 ) ) ;
#83951=CARTESIAN_POINT ( 'NONE',  ( 22.78697251350000030, 1409.735498424730167, 208.5774519181389905 ) ) ;
#83955=CARTESIAN_POINT ( 'NONE',  ( 26.86955400987890030, 1451.969623626720022, 135.0836937022390032 ) ) ;
#83961=CARTESIAN_POINT ( 'NONE',  ( 9.679025545887689930, 1409.251059407319872, 190.1046045489409835 ) ) ;
#83962=CARTESIAN_POINT ( 'NONE',  ( 2.632612402369999938, 1417.642861214730146, 234.7516877880979962 ) ) ;
#83964=CARTESIAN_POINT ( 'NONE',  ( 2.500000000000000000, 1439.615672362369878, 170.5246407131980106 ) ) ;
#83968=CARTESIAN_POINT ( 'NONE',  ( 12.85972207402829959, 1415.932840154009909, 221.4945844118829825 ) ) ;
#83969=CARTESIAN_POINT ( 'NONE',  ( 11.07540512644239961, 1432.346177023590144, 151.6859256421019779 ) ) ;
#83973=CARTESIAN_POINT ( 'NONE',  ( 11.60004869885203860, 1428.965959225140750, 137.0999999980979851 ) ) ;
#83976=CARTESIAN_POINT ( 'NONE',  ( -5.052203703969999182, 1465.000168611230038, 255.3819207742980097 ) ) ;
#83978=CARTESIAN_POINT ( 'NONE',  ( -22.09303006097569977, 1509.609508347655265, 191.2819047646252386 ) ) ;
#83981=B_SPLINE_SURFACE_WITH_KNOTS ( 'NONE', 5, 5, ( 
 ( #74766, #92100, #91554, #14830, #55776, #23229, #49018, #108904, #75323, #15377, #6991, #32744 ),
 ( #66924, #102142, #1363, #35505, #85905, #58514, #9748, #84246, #110556, #34403, #15918, #17006 ),
 ( #101034, #86457, #16464, #43914, #819, #25976, #277, #103235, #33842, #26547, #68033, #85335 ),
 ( #78058, #50120, #68576, #7545, #41699, #50657, #43371, #94292, #60741, #34947, #75858, #110009 ),
 ( #84788, #24332, #102679, #69132, #9211, #77519, #42807, #94863, #60174, #76968, #33285, #76402 ),
 ( #67476, #92644, #101581, #24868, #17570, #59073, #42255, #8087, #93195, #25422, #8632, #51206 ),
 ( #51770, #18137, #52334, #59615, #93728, #79736, #104365, #79189, #80824, #11964, #44475, #28768 ),
 ( #70813, #2495, #105480, #20348, #78621, #36612, #61849, #19802, #10299, #97082, #62400, #36073 ),
 ( #88686, #46149, #106034, #62970, #54552, #69699, #3045, #10872, #70258, #12516, #37171, #104926 ),
 ( #89221, #29310, #28211, #4132, #103818, #80279, #27117, #46694, #52881, #96526, #71367, #95420 ),
 ( #3594, #61301, #55093, #95968, #18683, #37718, #71919, #63509, #97627, #54006, #20895, #88138 ),
 ( #87009, #1936, #27662, #19229, #53437, #87584, #45044, #11426, #45595, #83022, #55645, #89766 ),
 ( #21976, #91967, #39919, #6314, #57304, #23097, #90863, #91430, #48338, #14152, #81351, #13586 ),
 ( #64044, #106572, #4666, #29858, #74088, #15243, #90305, #56168, #65685, #72980, #72440, #47225 ),
 ( #99803, #98161, #38805, #107118, #14705, #30960, #21434, #73539, #13037, #57840, #64597, #47772 ) ),
 .UNSPECIFIED., .F., .F., .F.,
 ( 6, 3, 3, 3, 6 ),
 ( 6, 3, 3, 6 ),
 ( 1.933639075400000129, 17.84603210599999912, 29.17820978809999843, 40.51038747020000130, 62.05803630019999417 ),
 ( -1.387778780779999841E-17, 21.09090217629999842, 42.18180435250000215, 84.36360870510000609 ),
 .UNSPECIFIED. ) ;
#83983=CARTESIAN_POINT ( 'NONE',  ( 0.1285806494137262390, 1467.142390093758650, 235.6418487887863193 ) ) ;
#83987=CARTESIAN_POINT ( 'NONE',  ( -5.623474965688048840E-07, 1451.660737107639989, 154.0815186765750013 ) ) ;
#83989=CARTESIAN_POINT ( 'NONE',  ( -17.51945758520000140, 1410.021940554830053, 225.1819460669979946 ) ) ;
#83991=CARTESIAN_POINT ( 'NONE',  ( 24.03538182579999827, 1410.920334398729892, 209.8065141638319915 ) ) ;
#83997=CARTESIAN_POINT ( 'NONE',  ( -6.282168602139999614, 1416.518938592030054, 226.3608756584980028 ) ) ;
#83999=CARTESIAN_POINT ( 'NONE',  ( 0.1711675699698229913, 1479.644119743519923, 182.1096778402390157 ) ) ;
#84002=CARTESIAN_POINT ( 'NONE',  ( -27.48389906189999721, 1444.324653571829913, 168.8435737885979790 ) ) ;
#84004=CARTESIAN_POINT ( 'NONE',  ( 11.87911642610000129, 1433.311711444109960, 149.6991885728979810 ) ) ;
#84005=CARTESIAN_POINT ( 'NONE',  ( -40.60962964096870564, 1447.683802589750030, 134.0999999984229873 ) ) ;
#84006=CARTESIAN_POINT ( 'NONE',  ( -16.93236825730539863, 1416.913057013589878, 207.4470323342559936 ) ) ;
#84007=ORIENTED_EDGE ( 'NONE', *, *, #109177, .F. ) ;
#84013=CARTESIAN_POINT ( 'NONE',  ( -4.283857371189049523, 1440.956241081810049, 155.9231041381889895 ) ) ;
#84014=AXIS2_PLACEMENT_3D ( 'NONE', #9523, #77843, #29493 ) ;
#84016=CARTESIAN_POINT ( 'NONE',  ( 7.287323794812330391, 1409.167539341809970, 222.1940209109550040 ) ) ;
#84017=FACE_OUTER_BOUND ( 'NONE', #99377, .T. ) ;
#84022=CARTESIAN_POINT ( 'NONE',  ( -32.07935534639999986, 1451.639962313729939, 135.6410485310980221 ) ) ;
#84023=CARTESIAN_POINT ( 'NONE',  ( 12.93929867839850445, 1442.831169986190389, 169.4513495753705570 ) ) ;
#84028=CARTESIAN_POINT ( 'NONE',  ( -19.42542553481155210, 1410.952741031847154, 222.1281440059015040 ) ) ;
#84032=ADVANCED_FACE ( 'NONE', ( #8181 ), #23145, .T. ) ;
#84033=CARTESIAN_POINT ( 'NONE',  ( 41.56671398617861968, 1445.561493043028804, 269.6392712540816774 ) ) ;
#84035=CARTESIAN_POINT ( 'NONE',  ( -17.33360664199999945, 1423.504494455729855, 226.8663630496979806 ) ) ;
#84036=CARTESIAN_POINT ( 'NONE',  ( 1.637935685380000006, 1417.125777826330022, 233.0400666244979959 ) ) ;
#84039=CARTESIAN_POINT ( 'NONE',  ( 1.910127611640000132E-10, 1497.713060387329961, 230.7369720342980202 ) ) ;
#84042=CARTESIAN_POINT ( 'NONE',  ( 3.655438681079999697, 1446.309375399810051, 170.5481836884979714 ) ) ;
#84044=CARTESIAN_POINT ( 'NONE',  ( 15.24173004819999910, 1496.337352016130126, 225.2051578755979904 ) ) ;
#84045=CARTESIAN_POINT ( 'NONE',  ( 14.45783246989999959, 1416.839692131129823, 196.8516148386979694 ) ) ;
#84049=ORIENTED_EDGE ( 'NONE', *, *, #109332, .F. ) ;
#84052=CARTESIAN_POINT ( 'NONE',  ( -4.017110540329999856E-16, 1428.413060387330006, 91.31218443469779800 ) ) ;
#84053=CARTESIAN_POINT ( 'NONE',  ( 16.18466855446819963, 1410.575406595820141, 191.5979442498370133 ) ) ;
#84055=( BOUNDED_CURVE ( )  B_SPLINE_CURVE ( 3, ( #22391, #24053, #74506, #5635 ),
 .UNSPECIFIED., .F., .F. ) 
 B_SPLINE_CURVE_WITH_KNOTS ( ( 4, 4 ),
 ( 3.077567002946369978, 3.089415543895895233 ),
 .UNSPECIFIED. ) 
 CURVE ( )  GEOMETRIC_REPRESENTATION_ITEM ( )  RATIONAL_B_SPLINE_CURVE ( ( 1.000000000000000000, 0.9999883010406638295, 0.9999883010406638295, 1.000000000000000000 ) ) 
 REPRESENTATION_ITEM ( '' )  );
#84056=CARTESIAN_POINT ( 'NONE',  ( 40.61087357212399951, 1439.649675151470092, 135.7177083055400146 ) ) ;
#84058=B_SPLINE_SURFACE_WITH_KNOTS ( 'NONE', 5, 5, ( 
 ( #104807, #27548, #79077, #78511, #86344, #96970, #26429, #94744, #18024 ),
 ( #70696, #70143, #52217, #62283, #96413, #61730, #28653, #19689, #37045 ),
 ( #88568, #71241, #43798, #77949, #107553, #72864, #64480, #73966, #90749 ),
 ( #98042, #14028, #48219, #13469, #46575, #47114, #82358, #56613, #30840 ),
 ( #72327, #5658, #98596, #82901, #57182, #108097, #65016, #73417, #31392 ),
 ( #63927, #106457, #29740, #39806, #37601, #99134, #21316, #30288, #106999 ) ),
 .UNSPECIFIED., .F., .F., .F.,
 ( 6, 6 ),
 ( 6, 3, 6 ),
 ( 39.30566995039999512, 56.26181244329999487 ),
 ( 0.000000000000000000, 1.000000000000000000, 2.000000000000000000 ),
 .UNSPECIFIED. ) ;
#84059=CARTESIAN_POINT ( 'NONE',  ( -6.526374435250000161, 1408.296887866830048, 262.4989398474979794 ) ) ;
#84060=CARTESIAN_POINT ( 'NONE',  ( 2.923263220760000447, 1409.521015951630034, 231.4220154199980186 ) ) ;
#84061=CARTESIAN_POINT ( 'NONE',  ( 12.13888692642257183, 1463.730258954271221, 231.4890017161033597 ) ) ;
#84062=CARTESIAN_POINT ( 'NONE',  ( 14.27756146466140130, 1416.835288280145733, 196.5246214017432180 ) ) ;
#84063=CARTESIAN_POINT ( 'NONE',  ( -38.11951386541859677, 1438.734027036600082, 136.6166153979129945 ) ) ;
#84067=DIRECTION ( 'NONE',  ( -0.006061051702997927691, 0.03006260551789778981, -0.9995296410821086219 ) ) ;
#84068=ORIENTED_EDGE ( 'NONE', *, *, #26729, .T. ) ;
#84070=CARTESIAN_POINT ( 'NONE',  ( -29.58887310228988454, 1509.966559353374123, 210.7380451519620976 ) ) ;
#84072=CYLINDRICAL_SURFACE ( 'NONE', #34903, 2.000000000000000000 ) ;
#84076=CARTESIAN_POINT ( 'NONE',  ( -28.13477487810000000, 1508.112005706330137, 208.1343964124890249 ) ) ;
#84077=CARTESIAN_POINT ( 'NONE',  ( 36.37832866288330536, 1435.767865547150222, 135.6938344640039986 ) ) ;
#84086=CARTESIAN_POINT ( 'NONE',  ( 11.77965714447340062, 1427.405098614149892, 147.0346648747149914 ) ) ;
#84089=CARTESIAN_POINT ( 'NONE',  ( -15.39071949251769844, 1488.664425019170039, 224.1266901275320151 ) ) ;
#84092=CARTESIAN_POINT ( 'NONE',  ( -13.12106589760000119, 1429.130020020729944, 222.3637170071979767 ) ) ;
#84095=CARTESIAN_POINT ( 'NONE',  ( -16.66101146819999812, 1410.867390116229899, 191.7375337716979971 ) ) ;
#84097=CARTESIAN_POINT ( 'NONE',  ( 25.05069432898669746, 1467.310853283639972, 206.2197278823790043 ) ) ;
#84098=CARTESIAN_POINT ( 'NONE',  ( 14.14095063499999938, 1460.769213631630237, 232.7918287509980075 ) ) ;
#84100=CARTESIAN_POINT ( 'NONE',  ( 0.03226293719758020068, 1410.297897419189894, 233.2219341505459909 ) ) ;
#84108=CARTESIAN_POINT ( 'NONE',  ( -2.900360919557655404, 1484.442349350321592, 183.3005521221487299 ) ) ;
#84109=CARTESIAN_POINT ( 'NONE',  ( -11.36592991815751930, 1425.607193177090494, 138.8060541407250525 ) ) ;
#84111=EDGE_LOOP ( 'NONE', ( #73192, #61586, #24683, #21221, #94892, #87373 ) ) ;
#84112=CARTESIAN_POINT ( 'NONE',  ( 1.114940886579999901, 1507.624369720630057, 186.1695746267980098 ) ) ;
#84115=CARTESIAN_POINT ( 'NONE',  ( -11.81020015660000055, 1428.491553152430015, 149.0224012402979668 ) ) ;
#84121=CARTESIAN_POINT ( 'NONE',  ( -19.55717248739999903, 1482.733170048929878, 227.9176884791980058 ) ) ;
#84122=CARTESIAN_POINT ( 'NONE',  ( -9.046333464132644053, 1421.595937556994159, 137.0999999980981272 ) ) ;
#84126=CARTESIAN_POINT ( 'NONE',  ( 14.57089808959999999, 1407.761835850630177, 266.8771382033980331 ) ) ;
#84127=CARTESIAN_POINT ( 'NONE',  ( 0.3489445596310000175, 1409.432092389130048, 185.2414967315980050 ) ) ;
#84128=CARTESIAN_POINT ( 'NONE',  ( 19.40597849089999727, 1430.302767083830076, 194.2683597324979985 ) ) ;
#84129=CARTESIAN_POINT ( 'NONE',  ( 7.849644149121719927, 1506.562754132946338, 229.7714992871970878 ) ) ;
#84131=CARTESIAN_POINT ( 'NONE',  ( 11.88915038004449976, 1434.057645928349984, 147.6474571075449944 ) ) ;
#84132=CARTESIAN_POINT ( 'NONE',  ( 13.15726445491959851, 1416.851343895820037, 196.3340833728059920 ) ) ;
#84135=B_SPLINE_CURVE_WITH_KNOTS ( 'NONE', 5,
 ( #85489, #31794, #40749, #33431, #8788, #25583 ),
 .UNSPECIFIED., .F., .F.,
 ( 6, 6 ),
 ( -158.0163518690000046, -29.52656374779999737 ),
 .UNSPECIFIED. ) ;
#84136=CARTESIAN_POINT ( 'NONE',  ( -13.23918200329999983, 1446.369626751160013, 188.0966930123980205 ) ) ;
#84137=CARTESIAN_POINT ( 'NONE',  ( -21.50121674829999918, 1519.913060387329779, 217.6081450858680171 ) ) ;
#84142=B_SPLINE_CURVE_WITH_KNOTS ( 'NONE', 3,
 ( #62592, #37347, #96709, #11593, #94470, #17743, #9381, #55269, #106198, #55820 ),
 .UNSPECIFIED., .F., .F.,
 ( 4, 2, 2, 2, 4 ),
 ( 0.000000000000000000, 0.2500000000000000000, 0.5000000000000000000, 0.7500000000000000000, 1.000000000000000000 ),
 .UNSPECIFIED. ) ;
#84143=CARTESIAN_POINT ( 'NONE',  ( 11.56050893731089069, 1425.527752771575024, 138.1868504500434085 ) ) ;
#84145=CARTESIAN_POINT ( 'NONE',  ( -21.88607058480000234, 1471.666806670330061, 268.8545562589980022 ) ) ;
#84146=CARTESIAN_POINT ( 'NONE',  ( -22.45507226509999654, 1509.697208789830029, 190.1127326308979946 ) ) ;
#84147=CARTESIAN_POINT ( 'NONE',  ( -11.93960757607870526, 1486.509476884231617, 184.3548908711684362 ) ) ;
#84151=CARTESIAN_POINT ( 'NONE',  ( 12.00789815276349870, 1415.778512723340100, 223.3240165415109857 ) ) ;
#84154=CARTESIAN_POINT ( 'NONE',  ( -15.27152961130000008, 1506.433683729329914, 224.9338604266980326 ) ) ;
#84155=CARTESIAN_POINT ( 'NONE',  ( -21.39776896220000069, 1411.020744638729866, 200.7714563019480067 ) ) ;
#84157=CARTESIAN_POINT ( 'NONE',  ( -15.97682509406200069, 1420.725243137946109, 227.0315895234790275 ) ) ;
#84159=CARTESIAN_POINT ( 'NONE',  ( 1.636503137890000126, 1433.447543843880112, 150.4001344053979778 ) ) ;
#84166=CARTESIAN_POINT ( 'NONE',  ( 11.71263799655990034, 1426.711684079400129, 142.4234639450059774 ) ) ;
#84170=CARTESIAN_POINT ( 'NONE',  ( -10.79382269979189957, 1414.913060387349788, 196.1395788316550011 ) ) ;
#84173=DIRECTION ( 'NONE',  ( -0.9965178241622074662, 5.841351974388313542E-13, 0.08338001035631943669 ) ) ;
#84179=CARTESIAN_POINT ( 'NONE',  ( 21.65564397057390167, 1509.711599606019945, 229.5146149028980176 ) ) ;
#84183=CARTESIAN_POINT ( 'NONE',  ( 11.85619637978460084, 1434.445867023679966, 151.0459428651619760 ) ) ;
#84184=CARTESIAN_POINT ( 'NONE',  ( -7.640780140759999561, 1396.708123330030048, 219.5175282754979946 ) ) ;
#84185=ORIENTED_EDGE ( 'NONE', *, *, #33639, .F. ) ;
#84187=CARTESIAN_POINT ( 'NONE',  ( -25.83536284099999847, 1509.142434271929915, 199.3925956580679895 ) ) ;
#84190=CARTESIAN_POINT ( 'NONE',  ( -13.72400085267329928, 1508.042562144249814, 184.2047245799730035 ) ) ;
#84193=B_SPLINE_CURVE_WITH_KNOTS ( 'NONE', 3,
 ( #13428, #90702, #99093, #29159, #22372, #47618, #38650, #12898, #81743, #12343 ),
 .UNSPECIFIED., .F., .F.,
 ( 4, 3, 3, 4 ),
 ( 12.29943377043420050, 12.57237910427029881, 12.96917103366740065, 13.22068347260000110 ),
 .UNSPECIFIED. ) ;
#84194=CARTESIAN_POINT ( 'NONE',  ( 0.3227009101319999740, 1429.777580095530084, 184.2093850951980016 ) ) ;
#84199=CARTESIAN_POINT ( 'NONE',  ( 14.43876446305509909, 1416.576002138870081, 196.8713507784850094 ) ) ;
#84200=CARTESIAN_POINT ( 'NONE',  ( 11.76895885309999912, 1432.295726632820106, 150.8120184455979995 ) ) ;
#84201=CARTESIAN_POINT ( 'NONE',  ( 11.74015320060000001, 1428.979986575930070, 144.1938086916980239 ) ) ;
#84203=CARTESIAN_POINT ( 'NONE',  ( 13.19223160394649952, 1436.077184055619909, 150.6575128507280112 ) ) ;
#84208=CARTESIAN_POINT ( 'NONE',  ( -12.61245242799999922, 1462.538255556929926, 230.8538998375979929 ) ) ;
#84216=ORIENTED_EDGE ( 'NONE', *, *, #73344, .F. ) ;
#84220=CARTESIAN_POINT ( 'NONE',  ( -18.63787277240000151, 1508.244465050730014, 229.7911781032980230 ) ) ;
#84221=CARTESIAN_POINT ( 'NONE',  ( -2.883409893379999644, 1409.181735910630096, 187.1726428837980052 ) ) ;
#84223=CARTESIAN_POINT ( 'NONE',  ( 0.2210724871696759797, 1414.913057862230062, 225.4904853195299950 ) ) ;
#84224=ORIENTED_EDGE ( 'NONE', *, *, #33043, .F. ) ;
#84225=CARTESIAN_POINT ( 'NONE',  ( 18.52345746059999954, 1425.819856484229831, 224.6762942411980077 ) ) ;
#84229=CARTESIAN_POINT ( 'NONE',  ( 13.45498908490000112, 1409.718027471030155, 270.3655313000979845 ) ) ;
#84231=CARTESIAN_POINT ( 'NONE',  ( 23.30293074599999770, 1409.831462182929954, 209.3510310548809912 ) ) ;
#84242=ADVANCED_FACE ( 'NONE', ( #90270 ), #58559, .F. ) ;
#84246=CARTESIAN_POINT ( 'NONE',  ( 28.68965969039999919, 1467.163325376930061, 264.4914803740979892 ) ) ;
#84249=EDGE_CURVE ( 'NONE', #37815, #46291, #99982, .T. ) ;
#84251=CARTESIAN_POINT ( 'NONE',  ( -5.494428884519999556, 1439.687232618090093, 154.7535770051980251 ) ) ;
#84253=CARTESIAN_POINT ( 'NONE',  ( 1.265885663164209918, 1452.808453964450109, 183.4299257876890010 ) ) ;
#84258=CARTESIAN_POINT ( 'NONE',  ( -1.467768375174040179E-06, 1443.913060387330006, 126.8032257208279958 ) ) ;
#84262=CARTESIAN_POINT ( 'NONE',  ( -5.015142591918240125E-06, 1473.897713703340060, 270.2927021991790184 ) ) ;
#84263=CARTESIAN_POINT ( 'NONE',  ( 38.60438541171740212, 1444.259423793630049, 137.1474472167479917 ) ) ;
#84264=CARTESIAN_POINT ( 'NONE',  ( 13.15726445491959851, 1416.851343895820037, 196.3340833728059920 ) ) ;
#84267=CARTESIAN_POINT ( 'NONE',  ( 10.80652762920177068, 1418.183843313859370, 229.8617425724453653 ) ) ;
#84268=CIRCLE ( 'NONE', #59281, 1.999999905350034135 ) ;
#84269=CARTESIAN_POINT ( 'NONE',  ( 26.79407473893059688, 1436.762045311259953, 136.7822278276699990 ) ) ;
#84270=CARTESIAN_POINT ( 'NONE',  ( 40.26005730150239970, 1444.258505248250231, 137.0889318870590046 ) ) ;
#84271=CARTESIAN_POINT ( 'NONE',  ( -22.47419750299999919, 1431.292034285129830, 216.7620959875980020 ) ) ;
#84272=CARTESIAN_POINT ( 'NONE',  ( -39.37087574719232208, 1458.242454951586524, 269.1450746934871745 ) ) ;
#84274=CARTESIAN_POINT ( 'NONE',  ( -16.70916575280000060, 1418.348764620830252, 226.8567342135980027 ) ) ;
#84276=ADVANCED_FACE ( 'NONE', ( #32028 ), #93836, .F. ) ;
#84278=CARTESIAN_POINT ( 'NONE',  ( -29.59278033692705989, 1462.546246255090409, 269.4665297251061133 ) ) ;
#84281=CARTESIAN_POINT ( 'NONE',  ( -22.27581235781267210, 1411.016249941691967, 269.4899098767419900 ) ) ;
#84282=ADVANCED_FACE ( 'NONE', ( #90828 ), #74049, .F. ) ;
#84284=CARTESIAN_POINT ( 'NONE',  ( 15.81656968443809852, 1472.200743377989966, 189.2032588538999960 ) ) ;
#84285=CARTESIAN_POINT ( 'NONE',  ( -2.305574648787668934, 1486.517880883643556, 181.6960553283176978 ) ) ;
#84286=CARTESIAN_POINT ( 'NONE',  ( -12.80112241844660304, 1444.980343738463034, 186.0141167343691109 ) ) ;
#84287=LINE ( 'NONE', #14315, #96823 ) ;
#84291=CARTESIAN_POINT ( 'NONE',  ( 44.70560407356640553, 1436.310412499470203, 269.9106010176490145 ) ) ;
#84292=CARTESIAN_POINT ( 'NONE',  ( -13.79754060518530068, 1451.192747375349654, 150.4573299455038864 ) ) ;
#84293=CARTESIAN_POINT ( 'NONE',  ( -17.48265144437409901, 1415.426207913209964, 209.4361257033870061 ) ) ;
#84294=CARTESIAN_POINT ( 'NONE',  ( 24.21135359159999823, 1435.361628672109873, 136.7755279798980155 ) ) ;
#84297=CARTESIAN_POINT ( 'NONE',  ( 0.1687944357386129968, 1416.535698381769862, 190.8841062147539844 ) ) ;
#84299=ORIENTED_EDGE ( 'NONE', *, *, #67834, .T. ) ;
#84300=VERTEX_POINT ( 'NONE', #93026 ) ;
#84301=CARTESIAN_POINT ( 'NONE',  ( 18.04214276402350237, 1416.520646088689773, 208.7607546544149955 ) ) ;
#84304=CARTESIAN_POINT ( 'NONE',  ( 1.320171144199999900E-07, 1461.184553862830171, 220.7697451771979900 ) ) ;
#84306=CARTESIAN_POINT ( 'NONE',  ( -0.2155932246156589960, 1507.120203089579945, 237.3367940327759982 ) ) ;
#84308=CARTESIAN_POINT ( 'NONE',  ( -2.874266342428972720, 1419.656144692103226, 186.1867820991938913 ) ) ;
#84310=CARTESIAN_POINT ( 'NONE',  ( -24.20181402199999710, 1438.345721746319896, 212.1538216921279911 ) ) ;
#84312=CARTESIAN_POINT ( 'NONE',  ( 1.894296828289999901, 1450.413579275490065, 182.1789249826979926 ) ) ;
#84315=CARTESIAN_POINT ( 'NONE',  ( -26.18770677744814890, 1509.940770221357525, 223.8536542907335161 ) ) ;
#84316=CARTESIAN_POINT ( 'NONE',  ( -3.716008649246309893E-10, 1417.166781705879885, 236.3045603347029839 ) ) ;
#84318=ORIENTED_EDGE ( 'NONE', *, *, #35229, .T. ) ;
#84319=CARTESIAN_POINT ( 'NONE',  ( -11.74676045389069934, 1426.724606243880089, 144.8518338750650116 ) ) ;
#84321=CARTESIAN_POINT ( 'NONE',  ( -6.501109238009999736, 1473.833204323429982, 270.1283629013980203 ) ) ;
#84328=CARTESIAN_POINT ( 'NONE',  ( -16.37061378800000000, 1453.313060387329870, 197.9545095496979741 ) ) ;
#84331=CARTESIAN_POINT ( 'NONE',  ( -6.111941472593700020, 1406.147481121090095, 267.2193986730749771 ) ) ;
#84332=CARTESIAN_POINT ( 'NONE',  ( -13.44357912138760014, 1435.903515400679908, 150.4587087247620047 ) ) ;
#84333=ORIENTED_EDGE ( 'NONE', *, *, #4420, .F. ) ;
#84344=CARTESIAN_POINT ( 'NONE',  ( -16.50115809955429569, 1479.761560564670162, 228.9857987416320100 ) ) ;
#84345=ORIENTED_EDGE ( 'NONE', *, *, #91691, .T. ) ;
#84350=CARTESIAN_POINT ( 'NONE',  ( -0.9098585486950000467, 1457.945133860129999, 229.8353278698979807 ) ) ;
#84352=CARTESIAN_POINT ( 'NONE',  ( -6.232532119210000054, 1407.162969929730025, 197.7132727109980124 ) ) ;
#84358=CARTESIAN_POINT ( 'NONE',  ( 20.38375078520000017, 1488.682100828129933, 225.5247866212980057 ) ) ;
#84360=B_SPLINE_CURVE_WITH_KNOTS ( 'NONE', 5,
 ( #96524, #89220, #1935, #55092, #11425, #36611, #53435, #46693, #45043 ),
 .UNSPECIFIED., .F., .F.,
 ( 6, 3, 6 ),
 ( 0.000000000000000000, 0.5050532947773366255, 1.000000000000000000 ),
 .UNSPECIFIED. ) ;
#84362=CARTESIAN_POINT ( 'NONE',  ( -25.00975368239999952, 1436.598045630599927, 137.9330133891980097 ) ) ;
#84363=CARTESIAN_POINT ( 'NONE',  ( -24.43616090849999978, 1442.711509888459886, 211.0968183358479848 ) ) ;
#84367=CARTESIAN_POINT ( 'NONE',  ( 5.465008655120000114, 1438.535486872679940, 154.7353332079979964 ) ) ;
#84368=CARTESIAN_POINT ( 'NONE',  ( -14.01548211210000083, 1415.603106624230122, 227.2686154209980032 ) ) ;
#84369=CARTESIAN_POINT ( 'NONE',  ( 3.634203233935680899, 1440.827878596160645, 156.5853169787592094 ) ) ;
#84370=EDGE_CURVE ( 'NONE', #65085, #86613, #78523, .T. ) ;
#84371=( BOUNDED_CURVE ( )  B_SPLINE_CURVE ( 3, ( #32231, #92677, #34435, #49599 ),
 .UNSPECIFIED., .F., .F. ) 
 B_SPLINE_CURVE_WITH_KNOTS ( ( 4, 4 ),
 ( 4.712388980386121418, 5.974262833424425878 ),
 .UNSPECIFIED. ) 
 CURVE ( )  GEOMETRIC_REPRESENTATION_ITEM ( )  RATIONAL_B_SPLINE_CURVE ( ( 1.000000000000000000, 0.8716501122597870577, 0.8716501122597870577, 1.000000000000000000 ) ) 
 REPRESENTATION_ITEM ( '' )  );
#84374=CARTESIAN_POINT ( 'NONE',  ( -2.028054181814160195, 1451.945093940709967, 184.4146074275660112 ) ) ;
#84375=CARTESIAN_POINT ( 'NONE',  ( -11.43480509645590004, 1425.837052296090178, 122.9426100432909834 ) ) ;
#84376=CONICAL_SURFACE ( 'NONE', #107643, 26.99999999999999645, 0.2186689458740001812 ) ;
#84377=CARTESIAN_POINT ( 'NONE',  ( -19.59816656100214161, 1457.069254779966741, 225.8938671853012181 ) ) ;
#84380=ADVANCED_FACE ( 'NONE', ( #11787 ), #42915, .T. ) ;
#84381=CARTESIAN_POINT ( 'NONE',  ( -24.15338685722906931, 1509.761910428660258, 226.0312979713074242 ) ) ;
#84382=CARTESIAN_POINT ( 'NONE',  ( 16.05356316396359873, 1459.304920975610003, 229.2720038708899892 ) ) ;
#84384=CARTESIAN_POINT ( 'NONE',  ( -11.44665353847253186, 1425.798163151176823, 139.1345268192609126 ) ) ;
#84387=CARTESIAN_POINT ( 'NONE',  ( 4.228339101480629303, 1441.548126968499901, 165.4114336615949981 ) ) ;
#84390=CARTESIAN_POINT ( 'NONE',  ( 41.62259071379843078, 1442.636017130879281, 135.5651479417171004 ) ) ;
#84391=CARTESIAN_POINT ( 'NONE',  ( 20.07643654349999807, 1508.105275064629950, 189.2153773721979917 ) ) ;
#84393=EDGE_LOOP ( 'NONE', ( #91706, #36828, #28169, #89282 ) ) ;
#84396=CARTESIAN_POINT ( 'NONE',  ( 0.8420133151470000632, 1420.713779431030162, 183.4825641757979895 ) ) ;
#84397=ADVANCED_FACE ( 'NONE', ( #80092 ), #103732, .T. ) ;
#84403=CARTESIAN_POINT ( 'NONE',  ( 17.66474287497711515, 1423.264464242703070, 226.2584317618739078 ) ) ;
#84404=CARTESIAN_POINT ( 'NONE',  ( 18.19849895938333262, 1425.217889718911692, 224.8178544575432340 ) ) ;
#84405=CARTESIAN_POINT ( 'NONE',  ( -11.96519809220000141, 1440.444625599219989, 147.6189886498980002 ) ) ;
#84406=CARTESIAN_POINT ( 'NONE',  ( 26.13694933561869860, 1446.561492598689938, 138.0017900573960219 ) ) ;
#84409=LINE ( 'NONE', #76008, #4528 ) ;
#84413=ADVANCED_FACE ( 'NONE', ( #46940 ), #7096, .T. ) ;
#84414=CARTESIAN_POINT ( 'NONE',  ( -19.57305745864531232, 1485.442696534264769, 190.1378261536969774 ) ) ;
#84416=CARTESIAN_POINT ( 'NONE',  ( -27.76495496469999935, 1507.998797203929826, 210.4908169915179883 ) ) ;
#84417=CARTESIAN_POINT ( 'NONE',  ( 2.333436892953952402, 1410.372785154803296, 185.5288099421988477 ) ) ;
#84418=CARTESIAN_POINT ( 'NONE',  ( -12.51099982459209947, 1416.825784013739849, 222.1450729932890056 ) ) ;
#84424=CARTESIAN_POINT ( 'NONE',  ( 5.164757510559999653E-11, 1452.913060387330006, 152.5211280458980241 ) ) ;
#84429=CARTESIAN_POINT ( 'NONE',  ( -1.555023069489999799, 1450.600071333589995, 182.6247344782979951 ) ) ;
#84432=CARTESIAN_POINT ( 'NONE',  ( -17.06951414919999621, 1409.509140956229885, 223.5446133271979932 ) ) ;
#84433=ORIENTED_EDGE ( 'NONE', *, *, #57074, .F. ) ;
#84435=CARTESIAN_POINT ( 'NONE',  ( 16.15901746733320010, 1509.190936235299887, 232.4330185199439995 ) ) ;
#84438=CARTESIAN_POINT ( 'NONE',  ( 38.50077277891229954, 1439.111704508520006, 136.6477633019350151 ) ) ;
#84440=CYLINDRICAL_SURFACE ( 'NONE', #30556, 1.999999999999915179 ) ;
#84443=CARTESIAN_POINT ( 'NONE',  ( -4.161170142461470434, 1448.299083512420111, 185.1109003841999936 ) ) ;
#84444=CARTESIAN_POINT ( 'NONE',  ( -11.14671771210699980, 1434.019356486030119, 151.6529807626459956 ) ) ;
#84446=CARTESIAN_POINT ( 'NONE',  ( 2.678395535690000440, 1409.943584582829999, 185.6434079368980008 ) ) ;
#84450=VECTOR ( 'NONE', #53302, 1000.000000000000114 ) ;
#84451=CARTESIAN_POINT ( 'NONE',  ( -23.84529289740000380, 1452.080364410629954, 136.9869225417980090 ) ) ;
#84454=CARTESIAN_POINT ( 'NONE',  ( 9.865354089699437168, 1509.383614495533493, 237.5628902309379669 ) ) ;
#84455=CARTESIAN_POINT ( 'NONE',  ( 18.94792778995129723, 1457.631852883570218, 226.8423414700259855 ) ) ;
#84456=CARTESIAN_POINT ( 'NONE',  ( 12.53380499169999851, 1445.052233488290085, 169.4755105685979970 ) ) ;
#84457=CARTESIAN_POINT ( 'NONE',  ( 17.64503773310000057, 1507.624276183330039, 188.4842591371979950 ) ) ;
#84458=CARTESIAN_POINT ( 'NONE',  ( -2.104209200065090229E-11, 1469.985873362830034, 253.9841755105239827 ) ) ;
#84459=CARTESIAN_POINT ( 'NONE',  ( 18.90014522646387363, 1436.390526415187651, 146.5512626475670857 ) ) ;
#84460=CARTESIAN_POINT ( 'NONE',  ( -1.138464810440000141, 1416.254459047329874, 228.0025200077980116 ) ) ;
#84463=CARTESIAN_POINT ( 'NONE',  ( -0.04336102728451687871, 1486.225514230211502, 181.8152960724703178 ) ) ;
#84465=CARTESIAN_POINT ( 'NONE',  ( -46.03287938273930280, 1439.834097020150239, 266.6776158563489503 ) ) ;
#84466=CARTESIAN_POINT ( 'NONE',  ( -3.604910588070000088, 1439.699991058859950, 185.4007874081979992 ) ) ;
#84470=CARTESIAN_POINT ( 'NONE',  ( -4.500000000000000000, 1448.210448412289907, 183.1418046154980175 ) ) ;
#84473=CARTESIAN_POINT ( 'NONE',  ( -25.89716630254590157, 1451.282408691979981, 136.5524683703120274 ) ) ;
#84474=ORIENTED_EDGE ( 'NONE', *, *, #39882, .T. ) ;
#84475=CARTESIAN_POINT ( 'NONE',  ( 12.06072352979999884, 1421.519012089930129, 225.6702541985979735 ) ) ;
#84477=CARTESIAN_POINT ( 'NONE',  ( -16.63505975150000182, 1409.493969474430060, 194.0661809352979787 ) ) ;
#84481=EDGE_CURVE ( 'NONE', #104691, #44473, #7054, .T. ) ;
#84483=CARTESIAN_POINT ( 'NONE',  ( -25.91590772737680126, 1441.261220175949802, 138.4451201564890255 ) ) ;
#84484=ORIENTED_EDGE ( 'NONE', *, *, #2389, .F. ) ;
#84485=CARTESIAN_POINT ( 'NONE',  ( -5.000072644374990105, 1407.851873216519834, 270.1321895591700013 ) ) ;
#84486=CARTESIAN_POINT ( 'NONE',  ( 16.67138977455960003, 1423.371517972810125, 229.1847574738629874 ) ) ;
#84489=ORIENTED_EDGE ( 'NONE', *, *, #30425, .F. ) ;
#84490=CARTESIAN_POINT ( 'NONE',  ( -23.30548261472260307, 1409.842060052059878, 209.3678414107039885 ) ) ;
#84492=CARTESIAN_POINT ( 'NONE',  ( 16.87240902346729854, 1409.502257893559772, 222.1138755377239988 ) ) ;
#84493=CARTESIAN_POINT ( 'NONE',  ( -11.74015320060000001, 1428.979986575930070, 144.1938086916980239 ) ) ;
#84494=CARTESIAN_POINT ( 'NONE',  ( -0.6593404618510000370, 1498.354494260629963, 236.8901980696979876 ) ) ;
#84495=CARTESIAN_POINT ( 'NONE',  ( -18.73484119289999938, 1410.876217116529915, 223.4750562042979993 ) ) ;
#84496=CARTESIAN_POINT ( 'NONE',  ( 44.86486795881990020, 1448.468081076540102, 266.4437032002720116 ) ) ;
#84498=CARTESIAN_POINT ( 'NONE',  ( -16.47101786845277616, 1421.300047538932859, 226.9904063017911540 ) ) ;
#84501=CARTESIAN_POINT ( 'NONE',  ( 18.90551579537861926, 1457.715061770846432, 226.9289634256394663 ) ) ;
#84503=FACE_OUTER_BOUND ( 'NONE', #5894, .T. ) ;
#84504=VERTEX_POINT ( 'NONE', #39618 ) ;
#84505=CARTESIAN_POINT ( 'NONE',  ( 2.500000000000000000, 1448.894380914000067, 182.3534011237979939 ) ) ;
#84512=CARTESIAN_POINT ( 'NONE',  ( -4.115857443736018695, 1425.929640604822680, 186.1083528362279651 ) ) ;
#84514=CARTESIAN_POINT ( 'NONE',  ( 11.77382529147789825, 1409.324211426370084, 191.4068515141649982 ) ) ;
#84518=EDGE_CURVE ( 'NONE', #31602, #50150, #32075, .T. ) ;
#84520=CARTESIAN_POINT ( 'NONE',  ( 15.75226268009177133, 1422.687348061682542, 229.7547754696312268 ) ) ;
#84523=CARTESIAN_POINT ( 'NONE',  ( 11.30564476295229959, 1432.342987147049826, 151.4629857478109898 ) ) ;
#84530=CARTESIAN_POINT ( 'NONE',  ( -2.446787376320000096, 1432.353341358199941, 150.2884730787980061 ) ) ;
#84532=CARTESIAN_POINT ( 'NONE',  ( 11.90340384559999976, 1433.321539026439950, 150.0592069925980070 ) ) ;
#84534=CARTESIAN_POINT ( 'NONE',  ( 12.70648376455249995, 1416.221314539589912, 196.3383158254220007 ) ) ;
#84535=DIRECTION ( 'NONE',  ( 0.000000000000000000, 1.000000000000000000, 0.000000000000000000 ) ) ;
#84538=CARTESIAN_POINT ( 'NONE',  ( -18.30666397350000096, 1486.096651966729951, 188.7550239447980118 ) ) ;
#84540=CARTESIAN_POINT ( 'NONE',  ( -17.42058327870000056, 1410.018568801629954, 225.3436448546980273 ) ) ;
#84541=ADVANCED_FACE ( 'NONE', ( #41814 ), #100044, .T. ) ;
#84542=CARTESIAN_POINT ( 'NONE',  ( 23.81975463350000055, 1410.917033270829961, 210.6872995559480159 ) ) ;
#84543=CARTESIAN_POINT ( 'NONE',  ( 3.873467265494015432, 1446.300338666319021, 170.5362326314338191 ) ) ;
#84544=CARTESIAN_POINT ( 'NONE',  ( -35.96079425170172783, 1435.914111285932677, 135.0260409222823057 ) ) ;
#84551=CARTESIAN_POINT ( 'NONE',  ( 0.1713633400619609948, 1479.529269706499917, 182.1146112136229931 ) ) ;
#84552=CARTESIAN_POINT ( 'NONE',  ( -2.805963291598290166, 1407.650164048290208, 222.1876714739069882 ) ) ;
#84554=CARTESIAN_POINT ( 'NONE',  ( -12.73318793669440829, 1444.994950788470533, 164.6858276811441328 ) ) ;
#84555=PLANE ( 'NONE',  #22907 ) ;
#84556=CARTESIAN_POINT ( 'NONE',  ( 12.91281063729999978, 1434.774390924990257, 149.8853380536980069 ) ) ;
#84557=CARTESIAN_POINT ( 'NONE',  ( -40.02226351667210480, 1448.570981148800229, 134.0999999981999906 ) ) ;
#84558=CARTESIAN_POINT ( 'NONE',  ( -27.74152896854549866, 1446.393007474169963, 137.1637341980870133 ) ) ;
#84559=ORIENTED_EDGE ( 'NONE', *, *, #66484, .T. ) ;
#84560=DIRECTION ( 'NONE',  ( -0.7071067811870476172, -8.350994019970553111E-15, 0.7071067811860475283 ) ) ;
#84565=CARTESIAN_POINT ( 'NONE',  ( -16.14386229810000017, 1410.940818424630152, 209.1303365420530156 ) ) ;
#84566=LINE ( 'NONE', #108670, #20860 ) ;
#84568=CARTESIAN_POINT ( 'NONE',  ( 2.990245160869999808, 1439.681522767690012, 184.2324485070979847 ) ) ;
#84573=CARTESIAN_POINT ( 'NONE',  ( -30.93305835920000035, 1451.832845973630128, 134.8030507067980182 ) ) ;
#84574=CARTESIAN_POINT ( 'NONE',  ( 17.22654844235838567, 1443.501467202828508, 162.9224179604370590 ) ) ;
#84581=CARTESIAN_POINT ( 'NONE',  ( 40.71297843928967808, 1448.600067007655298, 269.6231773872929125 ) ) ;
#84583=CARTESIAN_POINT ( 'NONE',  ( 19.00106994256368864, 1437.749780598343705, 213.2493778570810434 ) ) ;
#84586=CARTESIAN_POINT ( 'NONE',  ( -6.863927053981574211, 1440.110827762987810, 185.9524514171546912 ) ) ;
#84587=CARTESIAN_POINT ( 'NONE',  ( -5.551115123129999164E-16, 1408.913060387329779, 226.8598803041980148 ) ) ;
#84590=CARTESIAN_POINT ( 'NONE',  ( 3.653657264300000040, 1446.290935082700116, 168.9981087564979987 ) ) ;
#84595=ORIENTED_EDGE ( 'NONE', *, *, #5811, .F. ) ;
#84597=EDGE_LOOP ( 'NONE', ( #109569, #51622, #51316 ) ) ;
#84599=CARTESIAN_POINT ( 'NONE',  ( -24.93712286909999776, 1430.363841025129886, 208.7990758118230019 ) ) ;
#84600=CARTESIAN_POINT ( 'NONE',  ( -10.81095005467450143, 1425.339529372819925, 121.9063493438599863 ) ) ;
#84601=CARTESIAN_POINT ( 'NONE',  ( 15.77750609497879886, 1410.568644415290009, 191.5438104861989927 ) ) ;
#84603=CARTESIAN_POINT ( 'NONE',  ( 38.46909107666640182, 1438.310882937109909, 136.5544058681170156 ) ) ;
#84605=CARTESIAN_POINT ( 'NONE',  ( -39.40331698669999838, 1435.955742992169917, 259.1105223372980504 ) ) ;
#84607=CARTESIAN_POINT ( 'NONE',  ( 13.65456221587469265, 1462.853443838520207, 230.7442824398011112 ) ) ;
#84609=CARTESIAN_POINT ( 'NONE',  ( 37.48372878014170340, 1450.753171827339884, 134.0999999986339901 ) ) ;
#84613=CARTESIAN_POINT ( 'NONE',  ( 18.54647816425740103, 1507.559819934359894, 190.5563924540620064 ) ) ;
#84614=VERTEX_POINT ( 'NONE', #54661 ) ;
#84616=CARTESIAN_POINT ( 'NONE',  ( -29.77441358006530692, 1509.998745987574921, 208.8337216755480483 ) ) ;
#84617=CARTESIAN_POINT ( 'NONE',  ( 27.74152896581870209, 1446.393007474679962, 137.1637341980689939 ) ) ;
#84622=CARTESIAN_POINT ( 'NONE',  ( 33.91369107978050579, 1435.681798568110025, 135.3769914806310055 ) ) ;
#84624=CARTESIAN_POINT ( 'NONE',  ( 26.17054978140000188, 1441.643302558009964, 138.0857572941980038 ) ) ;
#84627=VERTEX_POINT ( 'NONE', #88241 ) ;
#84631=CARTESIAN_POINT ( 'NONE',  ( 10.79382126600000014, 1414.913060387329779, 222.1041115775979904 ) ) ;
#84632=CARTESIAN_POINT ( 'NONE',  ( 20.19677127349999779, 1497.697269792330189, 228.1166628511979866 ) ) ;
#84634=CARTESIAN_POINT ( 'NONE',  ( -13.45946769660000086, 1415.628674266529742, 221.4934452861980105 ) ) ;
#84636=CARTESIAN_POINT ( 'NONE',  ( -16.90809753623369360, 1442.831169986191526, 162.4344573440251338 ) ) ;
#84640=CARTESIAN_POINT ( 'NONE',  ( -13.39783700169999925, 1429.123728478029989, 222.2884932514979823 ) ) ;
#84641=CARTESIAN_POINT ( 'NONE',  ( -8.974062746725300244, 1446.631196276342735, 153.7453213382308661 ) ) ;
#84645=CARTESIAN_POINT ( 'NONE',  ( -15.87931877369999967, 1462.584440484630022, 222.8385820429980129 ) ) ;
#84646=CARTESIAN_POINT ( 'NONE',  ( 18.07871887829999835, 1459.074710307329951, 227.9662036256980002 ) ) ;
#84648=CARTESIAN_POINT ( 'NONE',  ( -5.022887173791962923, 1423.013679199760418, 184.8136794012343103 ) ) ;
#84649=CARTESIAN_POINT ( 'NONE',  ( -2.499951737868360002, 1420.086717788219858, 94.80349057415200775 ) ) ;
#84650=ORIENTED_EDGE ( 'NONE', *, *, #26714, .F. ) ;
#84652=EDGE_CURVE ( 'NONE', #95096, #46920, #110700, .T. ) ;
#84655=CARTESIAN_POINT ( 'NONE',  ( -2.897552558531884870, 1484.306681456201659, 183.3139059294359754 ) ) ;
#84657=ORIENTED_EDGE ( 'NONE', *, *, #23472, .F. ) ;
#84658=CARTESIAN_POINT ( 'NONE',  ( 1.118234699620000105, 1453.152003547129880, 188.5610888405979892 ) ) ;
#84661=CARTESIAN_POINT ( 'NONE',  ( -11.74858685269999903, 1426.686222183830068, 144.9813623866980095 ) ) ;
#84665=SPHERICAL_SURFACE ( 'NONE', #35935, 2.000000000000000000 ) ;
#84667=CARTESIAN_POINT ( 'NONE',  ( -20.96279981269999837, 1495.371218722530102, 226.8017206206980063 ) ) ;
#84669=CARTESIAN_POINT ( 'NONE',  ( 3.156194964112319479, 1466.544005466739918, 236.1242056213270075 ) ) ;
#84672=CARTESIAN_POINT ( 'NONE',  ( 30.12538801500000218, 1414.390931448930132, 266.8625852646979979 ) ) ;
#84673=CARTESIAN_POINT ( 'NONE',  ( 4.500000000000000000, 1425.929641636930000, 183.3886486283980162 ) ) ;
#84674=CARTESIAN_POINT ( 'NONE',  ( 24.08617896360000188, 1449.722506852089964, 204.7855894934380103 ) ) ;
#84675=CARTESIAN_POINT ( 'NONE',  ( 18.91079974722019941, 1425.084603971189836, 222.8166007544258491 ) ) ;
#84678=CARTESIAN_POINT ( 'NONE',  ( -1.804408714559999849, 1450.411044013399987, 182.7103574280979785 ) ) ;
#84679=EDGE_CURVE ( 'NONE', #36772, #102747, #97206, .T. ) ;
#84680=B_SPLINE_CURVE_WITH_KNOTS ( 'NONE', 3,
 ( #26357, #36419, #10685, #85166, #97966, #54358, #19614, #80636, #12313, #20700 ),
 .UNSPECIFIED., .F., .F.,
 ( 4, 2, 2, 2, 4 ),
 ( -0.1358568304961229878, -0.09953452613532230708, -0.06373121003967659182, -0.02032877986101701284, 0.000000000000000000 ),
 .UNSPECIFIED. ) ;
#84683=CARTESIAN_POINT ( 'NONE',  ( -14.46612070239999959, 1444.027671829609972, 188.8340718453980003 ) ) ;
#84684=CARTESIAN_POINT ( 'NONE',  ( -18.65529551030000022, 1453.313060387329870, 216.4487054234179766 ) ) ;
#84688=CARTESIAN_POINT ( 'NONE',  ( -13.84930592310000108, 1431.437219492539953, 209.1218459616979999 ) ) ;
#84691=CARTESIAN_POINT ( 'NONE',  ( -14.53064231559999975, 1473.849484241330174, 269.2157382448979774 ) ) ;
#84693=CARTESIAN_POINT ( 'NONE',  ( -22.27620219389999789, 1509.702625318030186, 189.6894442619980055 ) ) ;
#84694=CARTESIAN_POINT ( 'NONE',  ( -24.44412394876377093, 1444.690170677753258, 211.0767915248584075 ) ) ;
#84697=CARTESIAN_POINT ( 'NONE',  ( 12.03450403489540044, 1415.834070662830072, 223.3500408510359989 ) ) ;
#84701=CARTESIAN_POINT ( 'NONE',  ( -23.03428792449999918, 1410.212555181330117, 205.5016647962879972 ) ) ;
#84705=B_SPLINE_CURVE_WITH_KNOTS ( 'NONE', 3,
 ( #4522, #5618, #106965, #97470, #40310, #39770, #64983, #3986, #98559, #73930, #12902, #106421, #13433, #31356, #99099, #29706, #38111, #65540, #54935, #98006, #47623, #12349, #21827, #91270, #99648, #20740, #22939, #39201, #56026, #105883, #63891, #21276, #90151, #81749, #55485, #29164, #5056, #48737, #46539, #73377, #57142, #14550, #82863 ),
 .UNSPECIFIED., .F., .F.,
 ( 4, 3, 3, 3, 3, 3, 3, 3, 3, 3, 3, 3, 3, 3, 4 ),
 ( -1.999999998304380133, -1.940506176228419921, -1.795837195207230064, -1.649175357432780098, -1.501247921597500090, -1.351435166382589870, -1.200651412290280051, -1.049213174562420026, -0.8974822393858350456, -0.7399797023974719057, -0.5893366077835271444, -0.4397854573115069776, -0.2915963409840560683, -0.1449609066947019631, 0.000000000000000000 ),
 .UNSPECIFIED. ) ;
#84711=CARTESIAN_POINT ( 'NONE',  ( -22.53878309250000100, 1411.058442772730132, 212.0450770775579770 ) ) ;
#84713=CARTESIAN_POINT ( 'NONE',  ( 11.71865588026039973, 1426.707724708179967, 142.8540073575470046 ) ) ;
#84718=CARTESIAN_POINT ( 'NONE',  ( -0.06979898235752290958, 1408.910622953190114, 224.1218459617979875 ) ) ;
#84725=CARTESIAN_POINT ( 'NONE',  ( 21.81488504828589825, 1509.642650274630114, 228.1804615763130073 ) ) ;
#84728=VERTEX_POINT ( 'NONE', #6980 ) ;
#84729=EDGE_LOOP ( 'NONE', ( #59979, #99563, #67797, #75372, #24329, #21911 ) ) ;
#84730=CARTESIAN_POINT ( 'NONE',  ( 11.37082106925189962, 1434.131391724269861, 151.4751752372850149 ) ) ;
#84731=CARTESIAN_POINT ( 'NONE',  ( -2.663926418229999982, 1397.071489263530111, 221.9487469225979908 ) ) ;
#84737=CARTESIAN_POINT ( 'NONE',  ( -13.73190975862210017, 1508.113242452410077, 184.1859641058979946 ) ) ;
#84738=CARTESIAN_POINT ( 'NONE',  ( 17.31952399019999689, 1507.813089787830222, 230.9486221998979829 ) ) ;
#84739=CARTESIAN_POINT ( 'NONE',  ( 1.921582663709999972, 1449.239314806859966, 183.7267869822979947 ) ) ;
#84740=CARTESIAN_POINT ( 'NONE',  ( -5.314268782590000129, 1416.216252248729916, 191.8300084588979928 ) ) ;
#84743=CARTESIAN_POINT ( 'NONE',  ( 4.566198684544860775, 1396.072515563980005, 199.0791066682190262 ) ) ;
#84744=DIRECTION ( 'NONE',  ( 0.000000000000000000, 0.000000000000000000, -1.000000000000000000 ) ) ;
#84745=CARTESIAN_POINT ( 'NONE',  ( 11.86664183439999931, 1432.373872705260283, 149.9823177143980217 ) ) ;
#84748=CARTESIAN_POINT ( 'NONE',  ( 13.07083448467220066, 1435.604313765049938, 150.5504815018899762 ) ) ;
#84752=CARTESIAN_POINT ( 'NONE',  ( 13.48176841661342706, 1444.196030681880757, 169.3584259374786143 ) ) ;
#84753=CARTESIAN_POINT ( 'NONE',  ( -4.034591554379999501, 1464.976194902429825, 235.4333245580980076 ) ) ;
#84757=B_SPLINE_SURFACE_WITH_KNOTS ( 'NONE', 5, 4, ( 
 ( #9152, #36555, #103763, #76915, #44422 ),
 ( #17515, #78564, #2440, #60682, #19172 ),
 ( #18083, #53947, #9691, #69640, #766 ),
 ( #34348, #27064, #8583, #51713, #1880 ),
 ( #43316, #77464, #34895, #69083, #52278 ),
 ( #1312, #103184, #18626, #86403, #43859 ) ),
 .UNSPECIFIED., .F., .F., .F.,
 ( 6, 6 ),
 ( 5, 5 ),
 ( 0.000000000000000000, 52.98902693510000006 ),
 ( 40.20365518519999881, 50.26548245740000453 ),
 .UNSPECIFIED. ) ;
#84759=CARTESIAN_POINT ( 'NONE',  ( 2.500000000000000000, 1448.201357973759968, 168.5759913970699984 ) ) ;
#84761=VERTEX_POINT ( 'NONE', #83143 ) ;
#84763=ORIENTED_EDGE ( 'NONE', *, *, #84962, .F. ) ;
#84764=CARTESIAN_POINT ( 'NONE',  ( 21.85224605700239664, 1440.913060387330006, 226.6615408831969773 ) ) ;
#84766=CARTESIAN_POINT ( 'NONE',  ( -2.760778262710000153, 1409.009468888630181, 188.0459436639980026 ) ) ;
#84770=CARTESIAN_POINT ( 'NONE',  ( 19.19790826559999886, 1425.425173530230040, 222.4585045609979943 ) ) ;
#84783=CARTESIAN_POINT ( 'NONE',  ( 13.96308414129999953, 1409.400662026229838, 192.3471292444979781 ) ) ;
#84784=CARTESIAN_POINT ( 'NONE',  ( 10.96966286673369950, 1432.359740019160199, 151.7701370213850112 ) ) ;
#84786=EDGE_LOOP ( 'NONE', ( #100896, #82657, #72082, #12602, #55908, #37788, #37266, #61119, #46306, #70701, #100972, #40560, #1003, #65640, #96279 ) ) ;
#84788=CARTESIAN_POINT ( 'NONE',  ( 36.81313713790000008, 1440.913060390829969, 254.5659540704979804 ) ) ;
#84789=DIRECTION ( 'NONE',  ( -0.9993779836618710277, -0.0009462243742934110021, -0.03525266559235790131 ) ) ;
#84790=CARTESIAN_POINT ( 'NONE',  ( -17.88319654240000034, 1498.319094940030027, 229.4271405375980066 ) ) ;
#84792=CARTESIAN_POINT ( 'NONE',  ( 44.93136576140000926, 1440.913060387330006, 269.6838065358980430 ) ) ;
#84796=DIRECTION ( 'NONE',  ( -1.986952269380850554E-13, 0.03085824620771311644, 0.9995237709234254808 ) ) ;
#84798=EDGE_LOOP ( 'NONE', ( #83089, #5023, #8337, #44856, #102615 ) ) ;
#84800=CARTESIAN_POINT ( 'NONE',  ( 0.3744771583600000064, 1467.623228442029813, 229.4021283991980056 ) ) ;
#84801=AXIS2_PLACEMENT_3D ( 'NONE', #2100, #86621, #9914 ) ;
#84802=CARTESIAN_POINT ( 'NONE',  ( 24.54353315340000208, 1443.825479976730094, 213.3278313276680080 ) ) ;
#84803=CARTESIAN_POINT ( 'NONE',  ( 38.58235177202990940, 1444.329162690310113, 137.1361782392559689 ) ) ;
#84806=CARTESIAN_POINT ( 'NONE',  ( 8.041051540796583907, 1417.091402351465149, 230.7851105917766290 ) ) ;
#84807=CARTESIAN_POINT ( 'NONE',  ( 30.86935880328820048, 1436.051794213489757, 136.3934173885100165 ) ) ;
#84808=CARTESIAN_POINT ( 'NONE',  ( 38.68457868389829457, 1448.131034673710019, 136.4755686143420235 ) ) ;
#84811=CARTESIAN_POINT ( 'NONE',  ( 14.38189351659999993, 1509.358429554029954, 184.5350612304979734 ) ) ;
#84819=CARTESIAN_POINT ( 'NONE',  ( 11.44901156743445902, 1425.804225261266083, 139.1025670327599926 ) ) ;
#84821=CARTESIAN_POINT ( 'NONE',  ( -29.28654146900000299, 1509.872632246929925, 209.3496755897299977 ) ) ;
#84824=CARTESIAN_POINT ( 'NONE',  ( -20.96933869981734588, 1450.949473037474036, 144.4962461051783578 ) ) ;
#84825=B_SPLINE_CURVE_WITH_KNOTS ( 'NONE', 5,
 ( #65513, #105858, #64411, #55458, #99623, #47596 ),
 .UNSPECIFIED., .F., .F.,
 ( 6, 6 ),
 ( 0.000000000000000000, 1.000000000000000000 ),
 .UNSPECIFIED. ) ;
#84826=CARTESIAN_POINT ( 'NONE',  ( -18.05420922962109742, 1416.521607925270018, 209.3411825106769868 ) ) ;
#84827=CARTESIAN_POINT ( 'NONE',  ( 23.99508155959999911, 1435.335429155559950, 136.6133439143980013 ) ) ;
#84830=VECTOR ( 'NONE', #51470, 1000.000000000000114 ) ;
#84831=CARTESIAN_POINT ( 'NONE',  ( 1.239262138261830071, 1414.972329067380088, 191.7539262446190094 ) ) ;
#84833=ORIENTED_EDGE ( 'NONE', *, *, #99266, .T. ) ;
#84837=CARTESIAN_POINT ( 'NONE',  ( 11.02695407560000085, 1426.510375595630194, 92.69043260369780057 ) ) ;
#84838=CARTESIAN_POINT ( 'NONE',  ( -22.50357283319999979, 1452.344118194430166, 225.2792279245980183 ) ) ;
#84840=CARTESIAN_POINT ( 'NONE',  ( 4.178231331191369691, 1424.123642773229903, 184.3799813994870078 ) ) ;
#84842=CARTESIAN_POINT ( 'NONE',  ( -2.727235894615162692, 1420.119452836188657, 186.0440366003105908 ) ) ;
#84844=CARTESIAN_POINT ( 'NONE',  ( -24.21720135390000195, 1438.555912338969847, 211.3959883349679956 ) ) ;
#84845=CARTESIAN_POINT ( 'NONE',  ( 2.246798639239999673, 1452.411382190229915, 183.6586391263979863 ) ) ;
#84848=CARTESIAN_POINT ( 'NONE',  ( -2.386211797780819926E-09, 1414.144573887250090, 247.2442443194049986 ) ) ;
#84849=ORIENTED_EDGE ( 'NONE', *, *, #22964, .F. ) ;
#84850=ORIENTED_EDGE ( 'NONE', *, *, #69999, .T. ) ;
#84851=CARTESIAN_POINT ( 'NONE',  ( -11.84830064420589935, 1431.103738429200121, 149.8426049743330282 ) ) ;
#84852=ADVANCED_FACE ( 'NONE', ( #108342 ), #90979, .T. ) ;
#84854=CARTESIAN_POINT ( 'NONE',  ( -19.87603051640006058, 1484.414881828269699, 191.2154138880676726 ) ) ;
#84855=CARTESIAN_POINT ( 'NONE',  ( -3.422119479379999607, 1471.692614597330021, 269.8663692098979823 ) ) ;
#84856=CARTESIAN_POINT ( 'NONE',  ( 13.15423960803081371, 1434.846439206664854, 146.8772667774931904 ) ) ;
#84861=ADVANCED_FACE ( 'NONE', ( #98834 ), #16022, .F. ) ;
#84862=CARTESIAN_POINT ( 'NONE',  ( -22.92822468967000304, 1507.593738162509908, 207.9867144894979845 ) ) ;
#84865=CARTESIAN_POINT ( 'NONE',  ( -8.265472002072838720, 1407.311149223810162, 269.6288060363389718 ) ) ;
#84866=CARTESIAN_POINT ( 'NONE',  ( -13.96141929067220033, 1435.007875777050003, 148.7887252966330038 ) ) ;
#84867=ORIENTED_EDGE ( 'NONE', *, *, #12567, .T. ) ;
#84869=CARTESIAN_POINT ( 'NONE',  ( 14.00316683389999994, 1442.877080914420048, 189.4713982969979895 ) ) ;
#84871=AXIS2_PLACEMENT_3D ( 'NONE', #101701, #401, #67594 ) ;
#84872=ORIENTED_EDGE ( 'NONE', *, *, #48120, .F. ) ;
#84874=CARTESIAN_POINT ( 'NONE',  ( 5.027021143375445256, 1422.868624059190324, 184.4318487489844642 ) ) ;
#84876=AXIS2_PLACEMENT_3D ( 'NONE', #35368, #102546, #60040 ) ;
#84879=CARTESIAN_POINT ( 'NONE',  ( -17.31871724090759912, 1489.038281045860003, 229.1406144452789988 ) ) ;
#84880=B_SPLINE_SURFACE_WITH_KNOTS ( 'NONE', 5, 1, ( 
 ( #95984, #77536 ),
 ( #45061, #19249 ),
 ( #60757, #2510 ),
 ( #52355, #79204 ),
 ( #95438, #62418 ),
 ( #104384, #96544 ),
 ( #86472, #87600 ),
 ( #18157, #78636 ),
 ( #52898, #103834 ) ),
 .UNSPECIFIED., .F., .F., .F.,
 ( 6, 3, 6 ),
 ( 2, 2 ),
 ( 0.7097524320850000512, 4.064565650359999616, 10.06422694349720004 ),
 ( -13.51875974050000018, -1.265881781690000096 ),
 .UNSPECIFIED. ) ;
#84887=CARTESIAN_POINT ( 'NONE',  ( -27.96811930129999979, 1509.876319213429952, 202.1748059118680203 ) ) ;
#84888=B_SPLINE_SURFACE_WITH_KNOTS ( 'NONE', 4, 5, ( 
 ( #49307, #21853, #13459, #47106, #38681, #40885 ),
 ( #56602, #12926, #100250, #106450, #4548, #106991 ),
 ( #65007, #48210, #81232, #72857, #66128, #99123 ),
 ( #5648, #22402, #30280, #47649, #14576, #14019 ),
 ( #64473, #31381, #98588, #108086, #63919, #82348 ) ),
 .UNSPECIFIED., .F., .F., .F.,
 ( 5, 5 ),
 ( 6, 6 ),
 ( 6.621488669309999686, 17.01656664660000118 ),
 ( -5.551115123129999410E-17, 1.000000000000000000 ),
 .UNSPECIFIED. ) ;
#84889=CARTESIAN_POINT ( 'NONE',  ( 10.11781796957937551, 1428.435797280887527, 134.0999999980966777 ) ) ;
#84892=CARTESIAN_POINT ( 'NONE',  ( -1.303360707740000013, 1408.418417413329962, 195.5769302267979981 ) ) ;
#84893=CARTESIAN_POINT ( 'NONE',  ( 15.71383115701936006, 1506.606278687632539, 193.5425396900113810 ) ) ;
#84894=VERTEX_POINT ( 'NONE', #25966 ) ;
#84897=CARTESIAN_POINT ( 'NONE',  ( 27.27473106160000071, 1488.690404413930082, 210.2221370544380079 ) ) ;
#84900=CARTESIAN_POINT ( 'NONE',  ( -24.16964372749999868, 1435.415582199720120, 137.3389635753979974 ) ) ;
#84903=CARTESIAN_POINT ( 'NONE',  ( -14.14317614989999861, 1413.182323360430019, 227.0405350710979633 ) ) ;
#84905=VECTOR ( 'NONE', #69658, 1000.000000000000114 ) ;
#84908=CARTESIAN_POINT ( 'NONE',  ( -11.55783143579999894, 1415.365618343329970, 228.9844200364979940 ) ) ;
#84909=CARTESIAN_POINT ( 'NONE',  ( -19.86712494847475341, 1456.673296078442945, 225.4261212115576427 ) ) ;
#84910=EDGE_LOOP ( 'NONE', ( #44055, #43164, #62926, #100342 ) ) ;
#84912=CARTESIAN_POINT ( 'NONE',  ( 12.76251288935960027, 1435.676538582969897, 150.7804224899010137 ) ) ;
#84914=CARTESIAN_POINT ( 'NONE',  ( -4.219438644781110526, 1441.595895916910195, 183.5288106640859951 ) ) ;
#84915=AXIS2_PLACEMENT_3D ( 'NONE', #47593, #83380, #99619 ) ;
#84916=CARTESIAN_POINT ( 'NONE',  ( -0.1613635714646410035, 1507.107001889669846, 180.9028745560509890 ) ) ;
#84917=CARTESIAN_POINT ( 'NONE',  ( 21.39771952614790251, 1509.704955107219803, 188.4542851670070149 ) ) ;
#84923=CARTESIAN_POINT ( 'NONE',  ( 20.65148255260000099, 1509.627424728229926, 188.0185848083980034 ) ) ;
#84927=DIRECTION ( 'NONE',  ( 0.000000000000000000, 0.000000000000000000, -1.000000000000000000 ) ) ;
#84935=B_SPLINE_CURVE_WITH_KNOTS ( 'NONE', 5,
 ( #73627, #34208, #31593, #85155, #42615, #68392 ),
 .UNSPECIFIED., .F., .F.,
 ( 6, 6 ),
 ( -157.9969979290000026, -29.50720980459999510 ),
 .UNSPECIFIED. ) ;
#84937=CARTESIAN_POINT ( 'NONE',  ( 11.74015320060000001, 1428.979986575930070, 144.1938086916980239 ) ) ;
#84939=CARTESIAN_POINT ( 'NONE',  ( 44.53839032258289876, 1440.913060367359776, 264.9617148667340416 ) ) ;
#84941=CARTESIAN_POINT ( 'NONE',  ( 16.93884299705920071, 1507.634939766059915, 188.0954313100240256 ) ) ;
#84946=EDGE_CURVE ( 'NONE', #87917, #33774, #27807, .T. ) ;
#84947=CARTESIAN_POINT ( 'NONE',  ( 16.91620036578183672, 1409.772676212749047, 192.7760182944116707 ) ) ;
#84948=CARTESIAN_POINT ( 'NONE',  ( -28.20849547050000083, 1509.668627049429915, 211.1040453917479738 ) ) ;
#84949=CARTESIAN_POINT ( 'NONE',  ( 1.123001734155827158, 1410.331803268985368, 185.2141170702371085 ) ) ;
#84951=CARTESIAN_POINT ( 'NONE',  ( -3.153913303612108532, 1425.996417847233033, 185.6247366075170646 ) ) ;
#84960=EDGE_LOOP ( 'NONE', ( #67159, #13963, #62724, #61876 ) ) ;
#84962=EDGE_CURVE ( 'NONE', #99871, #102807, #19221, .T. ) ;
#84968=DIRECTION ( 'NONE',  ( 1.000000000000000000, 0.000000000000000000, 0.000000000000000000 ) ) ;
#84970=CARTESIAN_POINT ( 'NONE',  ( 37.95268740653450124, 1438.587537029340183, 136.6052002288919880 ) ) ;
#84971=CARTESIAN_POINT ( 'NONE',  ( -11.43185072513739797, 1443.913060387330006, 147.9056598087979921 ) ) ;
#84977=ADVANCED_FACE ( 'NONE', ( #37163 ), #24924, .F. ) ;
#84978=CARTESIAN_POINT ( 'NONE',  ( 4.533938656610000173, 1410.006645354029843, 186.2297118026980058 ) ) ;
#84979=CARTESIAN_POINT ( 'NONE',  ( 4.304887325260000175, 1424.164641267230081, 184.8345661179979800 ) ) ;
#84982=CARTESIAN_POINT ( 'NONE',  ( -25.25200564400000047, 1450.804212513650100, 137.6134969548979825 ) ) ;
#84983=CARTESIAN_POINT ( 'NONE',  ( 1.440267586269999844, 1465.218598317130272, 235.8491212012980043 ) ) ;
#84985=EDGE_CURVE ( 'NONE', #100850, #86349, #49987, .T. ) ;
#84987=CARTESIAN_POINT ( 'NONE',  ( 12.19431714289060587, 1509.463056330486779, 236.6448779725608347 ) ) ;
#84989=CARTESIAN_POINT ( 'NONE',  ( 21.13431379670319998, 1409.651086887829933, 206.4149708788170301 ) ) ;
#84991=CARTESIAN_POINT ( 'NONE',  ( 14.68671602690000100, 1430.156356569229956, 190.6741761820979946 ) ) ;
#84992=CARTESIAN_POINT ( 'NONE',  ( -7.471909415769559706E-09, 1475.245055346789968, 265.8384215023410206 ) ) ;
#84993=CARTESIAN_POINT ( 'NONE',  ( 23.91303816115560466, 1436.560782071131371, 140.3770785067727616 ) ) ;
#84994=CARTESIAN_POINT ( 'NONE',  ( -1.546949757679999760, 1416.828040475729949, 228.0209010782980101 ) ) ;
#84995=CARTESIAN_POINT ( 'NONE',  ( -1.630423233649999970, 1417.460556004529963, 234.9148393419980039 ) ) ;
#84999=CARTESIAN_POINT ( 'NONE',  ( -0.5298339765193601503, 1485.566302121303579, 181.9011267176622084 ) ) ;
#85001=CARTESIAN_POINT ( 'NONE',  ( -45.80615043228049643, 1438.856719389719956, 266.4146728030800091 ) ) ;
#85002=CARTESIAN_POINT ( 'NONE',  ( 14.03164605154790223, 1509.388572056619978, 234.6445892514809941 ) ) ;
#85005=ORIENTED_EDGE ( 'NONE', *, *, #4126, .F. ) ;
#85007=FACE_BOUND ( 'NONE', #55994, .T. ) ;
#85008=B_SPLINE_SURFACE_WITH_KNOTS ( 'NONE', 5, 1, ( 
 ( #96468, #46635 ),
 ( #19173, #79133 ),
 ( #37659, #46085 ),
 ( #86955, #29258 ),
 ( #79682, #95365 ),
 ( #70753, #62343 ),
 ( #36015, #105982 ),
 ( #20840, #97568 ),
 ( #71306, #3534 ) ),
 .UNSPECIFIED., .F., .F., .F.,
 ( 6, 3, 6 ),
 ( 2, 2 ),
 ( 0.000000000000000000, 5.782490304330000441, 11.25975508159999983 ),
 ( -1.500000000000000000, 1.500000000000000000 ),
 .UNSPECIFIED. ) ;
#85009=CARTESIAN_POINT ( 'NONE',  ( -26.87832471722010297, 1441.334257773779882, 137.4807412269939846 ) ) ;
#85012=CARTESIAN_POINT ( 'NONE',  ( -26.26714492849760063, 1451.099761601440150, 136.4712888930870065 ) ) ;
#85014=CARTESIAN_POINT ( 'NONE',  ( 25.86260026069999896, 1440.913060418369923, 221.4996202440979971 ) ) ;
#85018=CARTESIAN_POINT ( 'NONE',  ( 3.203789175851970288E-09, 1424.294192408320214, 227.6053815985079893 ) ) ;
#85019=CARTESIAN_POINT ( 'NONE',  ( -24.04315183071442519, 1445.026065455099797, 213.4541038297220439 ) ) ;
#85022=EDGE_CURVE ( 'NONE', #44794, #105370, #50628, .T. ) ;
#85024=ORIENTED_EDGE ( 'NONE', *, *, #47341, .T. ) ;
#85025=CARTESIAN_POINT ( 'NONE',  ( -3.003389061728070075, 1410.104144440540040, 269.8660872768579679 ) ) ;
#85026=CARTESIAN_POINT ( 'NONE',  ( 10.71406017268189892, 1419.905362405259893, 231.5852711379240247 ) ) ;
#85028=ORIENTED_EDGE ( 'NONE', *, *, #31550, .F. ) ;
#85031=CARTESIAN_POINT ( 'NONE',  ( -23.69647183529550105, 1410.728790039680007, 210.2360925051529819 ) ) ;
#85034=CARTESIAN_POINT ( 'NONE',  ( -11.30500403589999792, 1428.976642997429963, 112.4493539157979995 ) ) ;
#85035=EDGE_CURVE ( 'NONE', #48892, #85148, #107919, .T. ) ;
#85036=CARTESIAN_POINT ( 'NONE',  ( -18.66712256547790005, 1432.215067861279977, 194.5764810006290020 ) ) ;
#85038=CARTESIAN_POINT ( 'NONE',  ( 36.73751017938760555, 1461.736580476300105, 266.4401257845650548 ) ) ;
#85041=CARTESIAN_POINT ( 'NONE',  ( -16.30652261508721423, 1421.098027771803800, 227.0172576140167848 ) ) ;
#85043=ORIENTED_EDGE ( 'NONE', *, *, #46053, .F. ) ;
#85044=CARTESIAN_POINT ( 'NONE',  ( 18.97915715501314793, 1457.436128530311407, 226.6750837173330240 ) ) ;
#85051=CARTESIAN_POINT ( 'NONE',  ( -1.544830625875079910, 1421.730119690919992, 228.2386301722320070 ) ) ;
#85054=CARTESIAN_POINT ( 'NONE',  ( 17.22592482065188335, 1443.913060387329779, 162.9227486220069352 ) ) ;
#85055=CARTESIAN_POINT ( 'NONE',  ( 1.014329838393059902, 1408.948481565789962, 186.6702704748330177 ) ) ;
#85056=CARTESIAN_POINT ( 'NONE',  ( 1.220948355079999992, 1416.360244924329891, 233.1251597269979925 ) ) ;
#85057=LINE ( 'NONE', #101288, #84830 ) ;
#85058=CARTESIAN_POINT ( 'NONE',  ( 12.86744022639999940, 1409.362401301430054, 227.0135731152979872 ) ) ;
#85063=CARTESIAN_POINT ( 'NONE',  ( 11.81416765884010012, 1432.336398938299908, 150.4603274062260141 ) ) ;
#85071=CARTESIAN_POINT ( 'NONE',  ( -10.04572263370000051, 1464.202968133530021, 255.3819207742980097 ) ) ;
#85072=CARTESIAN_POINT ( 'NONE',  ( -21.03123196678649975, 1507.789098018889945, 192.1781278620359785 ) ) ;
#85073=CARTESIAN_POINT ( 'NONE',  ( 11.91160370939999957, 1433.398298247449929, 150.1562357106980130 ) ) ;
#85074=CARTESIAN_POINT ( 'NONE',  ( 4.540901341789999712, 1462.614442898930065, 248.0989693021979861 ) ) ;
#85075=CARTESIAN_POINT ( 'NONE',  ( 12.87618670774100060, 1416.835419214280137, 196.3099906520550064 ) ) ;
#85083=CARTESIAN_POINT ( 'NONE',  ( 12.78677686703885996, 1398.292081298729045, 206.7702702667238555 ) ) ;
#85084=CARTESIAN_POINT ( 'NONE',  ( -7.510707159466901039, 1509.188756966919982, 238.7243973511239972 ) ) ;
#85085=CARTESIAN_POINT ( 'NONE',  ( 24.18568768079999742, 1430.355574605830043, 212.4850587644480129 ) ) ;
#85092=B_SPLINE_CURVE_WITH_KNOTS ( 'NONE', 3,
 ( #95743, #60507, #55833, #78395 ),
 .UNSPECIFIED., .F., .F.,
 ( 4, 4 ),
 ( 0.000000000000000000, 1.000000000000000000 ),
 .UNSPECIFIED. ) ;
#85094=CARTESIAN_POINT ( 'NONE',  ( 0.2056537491783179961, 1459.797042805989804, 182.9617855128460064 ) ) ;
#85095=CARTESIAN_POINT ( 'NONE',  ( -2.822331109926550230, 1407.946699431110119, 222.3121693578910083 ) ) ;
#85096=ORIENTED_EDGE ( 'NONE', *, *, #9303, .T. ) ;
#85097=CARTESIAN_POINT ( 'NONE',  ( -13.35741048202589809, 1443.913060387329324, 164.9741927960640453 ) ) ;
#85098=B_SPLINE_CURVE_WITH_KNOTS ( 'NONE', 3,
 ( #99542, #34006, #31802, #41859, #82761, #84947, #42407, #83857, #66542, #14983 ),
 .UNSPECIFIED., .F., .F.,
 ( 4, 2, 2, 2, 4 ),
 ( 0.000000000000000000, 0.2500000000000000000, 0.5000000000000000000, 0.7500000000000000000, 1.000000000000000000 ),
 .UNSPECIFIED. ) ;
#85099=EDGE_CURVE ( 'NONE', #98856, #61659, #17281, .T. ) ;
#85101=CARTESIAN_POINT ( 'NONE',  ( 13.50072690200000025, 1434.968958840149980, 149.8854961322979875 ) ) ;
#85102=CARTESIAN_POINT ( 'NONE',  ( -40.14707100610610269, 1448.397814784289949, 134.0999999982449822 ) ) ;
#85106=CYLINDRICAL_SURFACE ( 'NONE', #108236, 1.455175085939995450 ) ;
#85107=CARTESIAN_POINT ( 'NONE',  ( -16.09868638649999895, 1415.425582719929707, 216.6834975185180099 ) ) ;
#85111=CARTESIAN_POINT ( 'NONE',  ( -25.62237252300000279, 1435.677407238350042, 212.3102753037179866 ) ) ;
#85113=CARTESIAN_POINT ( 'NONE',  ( -22.57319772750419773, 1409.701314710050156, 209.4509374963450057 ) ) ;
#85119=CARTESIAN_POINT ( 'NONE',  ( -29.80701679760000289, 1450.584075178780267, 136.3662129318980192 ) ) ;
#85120=CARTESIAN_POINT ( 'NONE',  ( -15.69056619607619929, 1410.711084544529967, 226.7224086681349888 ) ) ;
#85122=CARTESIAN_POINT ( 'NONE',  ( 8.598096571001718758, 1427.995879741943554, 134.0999999980979567 ) ) ;
#85123=ORIENTED_EDGE ( 'NONE', *, *, #33786, .T. ) ;
#85129=CARTESIAN_POINT ( 'NONE',  ( 41.26946182738182500, 1446.774783179103224, 269.6336529072985400 ) ) ;
#85130=CARTESIAN_POINT ( 'NONE',  ( 22.12673984907599944, 1409.685743169220132, 208.3470065775269973 ) ) ;
#85131=CARTESIAN_POINT ( 'NONE',  ( 14.45242834458300862, 1430.060838702070441, 220.7992783074957401 ) ) ;
#85140=CARTESIAN_POINT ( 'NONE',  ( 3.654206554840000010, 1446.297061077269973, 167.4573428069980139 ) ) ;
#85145=EDGE_CURVE ( 'NONE', #91418, #105869, #9179, .T. ) ;
#85147=CARTESIAN_POINT ( 'NONE',  ( 3.055333763765900386E-13, 1547.913060387330006, 209.1218459616979999 ) ) ;
#85148=VERTEX_POINT ( 'NONE', #69963 ) ;
#85150=CARTESIAN_POINT ( 'NONE',  ( -23.95220588849999999, 1410.918936088230112, 208.0890925629879860 ) ) ;
#85151=CARTESIAN_POINT ( 'NONE',  ( -10.59742304113489908, 1425.359664718739850, 108.4540387853830055 ) ) ;
#85152=CARTESIAN_POINT ( 'NONE',  ( 17.08463325386040310, 1410.592669789649790, 192.1150242963900325 ) ) ;
#85154=CARTESIAN_POINT ( 'NONE',  ( 28.52891198672809736, 1510.020576512638172, 199.8347506128769169 ) ) ;
#85155=CARTESIAN_POINT ( 'NONE',  ( 1.532290126919999995, 1453.146242306529984, 188.6114051259980045 ) ) ;
#85156=CARTESIAN_POINT ( 'NONE',  ( -11.73700276120000119, 1426.696009609329849, 144.1682878321979899 ) ) ;
#85158=CARTESIAN_POINT ( 'NONE',  ( 12.75179305369680804, 1463.394816282316242, 231.2017325377458405 ) ) ;
#85161=CARTESIAN_POINT ( 'NONE',  ( -34.83764231434859937, 1437.110286233230227, 136.5404629688219984 ) ) ;
#85163=CARTESIAN_POINT ( 'NONE',  ( 8.897827345618869899, 1398.177211024679991, 219.0743639419499971 ) ) ;
#85166=CARTESIAN_POINT ( 'NONE',  ( 38.10537780832439836, 1442.926987427690165, 137.1117395883970005 ) ) ;
#85176=CARTESIAN_POINT ( 'NONE',  ( 27.06966409833973941, 1508.822567037296949, 206.2042575372482816 ) ) ;
#85181=VERTEX_POINT ( 'NONE', #110088 ) ;
#85186=CARTESIAN_POINT ( 'NONE',  ( 19.70018007940000260, 1487.524873918330059, 228.1714004993980041 ) ) ;
#85188=CARTESIAN_POINT ( 'NONE',  ( -13.76682154080000053, 1416.274718422629803, 221.8364419309980065 ) ) ;
#85189=CARTESIAN_POINT ( 'NONE',  ( -11.13648087572960144, 1432.345323104730141, 151.6342752581680031 ) ) ;
#85192=CARTESIAN_POINT ( 'NONE',  ( -4.848112173330000552, 1424.812407234129978, 186.1231568304979760 ) ) ;
#85193=CARTESIAN_POINT ( 'NONE',  ( -7.632823605539153178, 1446.706720026436187, 154.1366947371981837 ) ) ;
#85197=CARTESIAN_POINT ( 'NONE',  ( 24.02067050899190193, 1444.215366903609947, 206.2118375416320077 ) ) ;
#85198=CARTESIAN_POINT ( 'NONE',  ( 18.07930019940000221, 1457.670260863829981, 229.7183053948980103 ) ) ;
#85199=CARTESIAN_POINT ( 'NONE',  ( -1.757532416683340148, 1451.933574871519795, 184.1885909450070073 ) ) ;
#85200=CARTESIAN_POINT ( 'NONE',  ( -4.804557508719293324, 1423.543705180204142, 184.5808143603345002 ) ) ;
#85203=CARTESIAN_POINT ( 'NONE',  ( 18.08636941810240018, 1424.496041336439930, 224.1297234290499887 ) ) ;
#85205=CARTESIAN_POINT ( 'NONE',  ( -2.915526101786688251, 1484.840208661149063, 183.2060714930112511 ) ) ;
#85206=CARTESIAN_POINT ( 'NONE',  ( -9.047070658296459234E-06, 1407.650947979230068, 270.1377427408980338 ) ) ;
#85209=FACE_OUTER_BOUND ( 'NONE', #110019, .T. ) ;
#85211=CARTESIAN_POINT ( 'NONE',  ( -11.80513488090000074, 1428.473324687329978, 148.4494227052980193 ) ) ;
#85212=CARTESIAN_POINT ( 'NONE',  ( -14.87168881317970026, 1430.147188212150240, 221.8136313441650032 ) ) ;
#85216=CARTESIAN_POINT ( 'NONE',  ( 2.896431327470000205, 1410.394954567630066, 231.6349568340980056 ) ) ;
#85217=CARTESIAN_POINT ( 'NONE',  ( -20.47759437099999857, 1470.086929132030036, 225.5303694363980185 ) ) ;
#85220=ORIENTED_EDGE ( 'NONE', *, *, #67976, .T. ) ;
#85222=CARTESIAN_POINT ( 'NONE',  ( 18.31222429210000158, 1408.824700350729927, 268.9136943074980195 ) ) ;
#85224=CARTESIAN_POINT ( 'NONE',  ( 21.87475989109999830, 1430.294660538329936, 199.6850607904279968 ) ) ;
#85228=CARTESIAN_POINT ( 'NONE',  ( -1.275176580349999922, 1451.321844197929977, 183.5437223828979825 ) ) ;
#85231=CARTESIAN_POINT ( 'NONE',  ( -14.28540945339999979, 1444.019357213639978, 188.7049663577979857 ) ) ;
#85232=CARTESIAN_POINT ( 'NONE',  ( -18.07642520410000131, 1475.513060387329915, 220.4627547701979893 ) ) ;
#85236=CARTESIAN_POINT ( 'NONE',  ( 1.465037550250199994, 1491.117439488069977, 181.8109677011690053 ) ) ;
#85237=CARTESIAN_POINT ( 'NONE',  ( -13.23418824936010019, 1409.375208424609809, 216.0505887701349934 ) ) ;
#85240=CARTESIAN_POINT ( 'NONE',  ( -21.63439191490000368, 1471.040418176530011, 269.4983909155979518 ) ) ;
#85243=CARTESIAN_POINT ( 'NONE',  ( -24.07534640571084950, 1444.393242560262479, 211.9935189188719278 ) ) ;
#85246=CARTESIAN_POINT ( 'NONE',  ( 12.10884181136779958, 1416.007771869960152, 223.4226694167990104 ) ) ;
#85248=DIRECTION ( 'NONE',  ( 0.08340294689805435868, -0.004098122787127734569, 0.9965074780644357366 ) ) ;
#85249=CARTESIAN_POINT ( 'NONE',  ( -0.7910245917146945249, 1426.918876941764893, 137.0999999980979851 ) ) ;
#85250=CARTESIAN_POINT ( 'NONE',  ( -22.94104396079999830, 1409.714179296030125, 208.0443976299279996 ) ) ;
#85252=EDGE_CURVE ( 'NONE', #16145, #67278, #109336, .T. ) ;
#85261=CARTESIAN_POINT ( 'NONE',  ( -21.54410644429999877, 1409.665397162329782, 210.5639858174479855 ) ) ;
#85263=CARTESIAN_POINT ( 'NONE',  ( 11.73645003660239894, 1426.696353566730068, 144.1286464700729937 ) ) ;
#85267=CARTESIAN_POINT ( 'NONE',  ( -0.06333887091406470438, 1408.725629457220066, 223.1955288070940071 ) ) ;
#85269=CARTESIAN_POINT ( 'NONE',  ( -5.631861160212480399, 1398.080659042673688, 220.8446200131021726 ) ) ;
#85271=CARTESIAN_POINT ( 'NONE',  ( -17.64656215119999771, 1410.883670852830164, 194.5767827140980160 ) ) ;
#85275=ADVANCED_FACE ( 'NONE', ( #51850 ), #101867, .T. ) ;
#85277=CARTESIAN_POINT ( 'NONE',  ( 11.89750062909999961, 1433.907086374190158, 150.7125587214979987 ) ) ;
#85278=CARTESIAN_POINT ( 'NONE',  ( 28.15435480200000029, 1509.896243100630045, 217.4028989878879941 ) ) ;
#85280=CARTESIAN_POINT ( 'NONE',  ( -0.0002535134715325740242, 1396.409806809705060, 221.4414762769463039 ) ) ;
#85281=CARTESIAN_POINT ( 'NONE',  ( -23.95032396419999898, 1509.749424129729960, 192.7253573581980106 ) ) ;
#85284=CARTESIAN_POINT ( 'NONE',  ( 18.02057538510000256, 1424.315176607929743, 225.5995559224980127 ) ) ;
#85285=CARTESIAN_POINT ( 'NONE',  ( 14.93738999439999837, 1507.809955652629924, 232.3150682984980051 ) ) ;
#85286=CARTESIAN_POINT ( 'NONE',  ( 3.193178223990000397, 1449.236852389319893, 184.0465812473979952 ) ) ;
#85288=CARTESIAN_POINT ( 'NONE',  ( 15.52863166319999877, 1409.957043847029809, 226.9582993814979943 ) ) ;
#85291=CARTESIAN_POINT ( 'NONE',  ( 13.40958089240390017, 1414.996442620800053, 197.9133050684260127 ) ) ;
#85292=CARTESIAN_POINT ( 'NONE',  ( 11.28450772929999957, 1431.049583972360097, 151.4082744405979781 ) ) ;
#85295=CARTESIAN_POINT ( 'NONE',  ( 13.55393066989770112, 1434.957539567609956, 148.7506260606290027 ) ) ;
#85298=CARTESIAN_POINT ( 'NONE',  ( 13.26721377506743238, 1444.631487620105418, 169.3823617746430443 ) ) ;
#85299=CARTESIAN_POINT ( 'NONE',  ( -6.765101722839999887, 1464.003571155029931, 235.1670121008980345 ) ) ;
#85300=CARTESIAN_POINT ( 'NONE',  ( -13.97867491850210087, 1429.402194067919709, 222.2970902837259928 ) ) ;
#85304=EDGE_CURVE ( 'NONE', #56530, #22078, #30735, .T. ) ;
#85305=CARTESIAN_POINT ( 'NONE',  ( -18.97979506072560341, 1443.417780829110598, 211.6816736686500633 ) ) ;
#85306=CARTESIAN_POINT ( 'NONE',  ( -1.793335950739999962, 1419.496365638530051, 185.6406336190979971 ) ) ;
#85308=EDGE_CURVE ( 'NONE', #94675, #35766, #8495, .T. ) ;
#85309=EDGE_LOOP ( 'NONE', ( #57659, #77517, #52000, #63182 ) ) ;
#85312=CARTESIAN_POINT ( 'NONE',  ( 19.96317061269749971, 1440.913060387330006, 216.1997736411760229 ) ) ;
#85313=CARTESIAN_POINT ( 'NONE',  ( -19.60066770079999898, 1508.321169291629985, 229.5156755424980020 ) ) ;
#85314=CARTESIAN_POINT ( 'NONE',  ( -8.768908993999998458, 1409.219277437030087, 189.4712383907980211 ) ) ;
#85317=ORIENTED_EDGE ( 'NONE', *, *, #66723, .T. ) ;
#85318=CARTESIAN_POINT ( 'NONE',  ( 23.67158291440000184, 1434.407285501780052, 214.7094373112279868 ) ) ;
#85322=CARTESIAN_POINT ( 'NONE',  ( 5.386185205460879644, 1432.347042709529887, 154.6076275981190236 ) ) ;
#85324=AXIS2_PLACEMENT_3D ( 'NONE', #77794, #95696, #10592 ) ;
#85327=CARTESIAN_POINT ( 'NONE',  ( 22.80370854688087690, 1409.709376451625985, 209.3213601526881575 ) ) ;
#85330=CARTESIAN_POINT ( 'NONE',  ( 14.33610687090000013, 1409.413688268130045, 192.4637013132980030 ) ) ;
#85335=CARTESIAN_POINT ( 'NONE',  ( -2.370583552050000338E-08, 1473.529262908829878, 262.4990046775979522 ) ) ;
#85337=CARTESIAN_POINT ( 'NONE',  ( -28.95199422474000173, 1509.924086303959939, 213.9638677111150002 ) ) ;
#85338=B_SPLINE_CURVE_WITH_KNOTS ( 'NONE', 3,
 ( #94582, #1112, #35241, #26845, #61032, #87308, #71656, #37455, #104100, #87876, #105775, #10601 ),
 .UNSPECIFIED., .F., .F.,
 ( 4, 2, 2, 2, 2, 4 ),
 ( -0.1123552056311339920, -0.09789079770760569787, -0.08345975727310689374, -0.05408602631436299629, -0.02844277166354580721, 1.387778780781445676E-17 ),
 .UNSPECIFIED. ) ;
#85339=CARTESIAN_POINT ( 'NONE',  ( -2.757035807209109901, 1508.901542382500111, 238.0815734855640073 ) ) ;
#85344=CARTESIAN_POINT ( 'NONE',  ( 17.94190076916380150, 1410.493024420959955, 222.9337422920199856 ) ) ;
#85350=CARTESIAN_POINT ( 'NONE',  ( 29.15071166469999753, 1509.931025669929795, 206.3815615989880143 ) ) ;
#85352=FACE_OUTER_BOUND ( 'NONE', #29112, .T. ) ;
#85356=CARTESIAN_POINT ( 'NONE',  ( 24.59498489902570029, 1440.913044926110160, 213.3385239659299941 ) ) ;
#85357=CARTESIAN_POINT ( 'NONE',  ( 32.64372457531959526, 1436.966666287780072, 136.6006212270859805 ) ) ;
#85358=CARTESIAN_POINT ( 'NONE',  ( -38.63560630069969903, 1444.097728792060025, 137.1726987393469983 ) ) ;
#85359=CARTESIAN_POINT ( 'NONE',  ( 3.996802888650000299E-15, 1464.864131489809779, 254.9666375976830182 ) ) ;
#85361=CARTESIAN_POINT ( 'NONE',  ( -16.86767980680000178, 1410.829200352329963, 226.4168310385980192 ) ) ;
#85365=ORIENTED_EDGE ( 'NONE', *, *, #31306, .T. ) ;
#85366=CARTESIAN_POINT ( 'NONE',  ( -40.73184307449999864, 1436.263014496689948, 268.3665355199980240 ) ) ;
#85369=CARTESIAN_POINT ( 'NONE',  ( 15.14272559822449793, 1450.983108074159873, 189.8671428218680148 ) ) ;
#85370=CARTESIAN_POINT ( 'NONE',  ( 11.41065117167780762, 1425.709223140004497, 138.9050562313533419 ) ) ;
#85374=FACE_OUTER_BOUND ( 'NONE', #77754, .T. ) ;
#85377=FACE_OUTER_BOUND ( 'NONE', #46361, .T. ) ;
#85378=CARTESIAN_POINT ( 'NONE',  ( -19.32265508015788669, 1451.005352466662998, 146.2743915447199186 ) ) ;
#85379=CARTESIAN_POINT ( 'NONE',  ( -16.67301258007090325, 1414.971349104640012, 209.3683847725079943 ) ) ;
#85380=CARTESIAN_POINT ( 'NONE',  ( 24.29594634020000044, 1435.420522265349973, 137.1129172815979871 ) ) ;
#85381=CARTESIAN_POINT ( 'NONE',  ( -10.28643981572550103, 1396.272270782580108, 205.0450038041399807 ) ) ;
#85382=ORIENTED_EDGE ( 'NONE', *, *, #59619, .T. ) ;
#85384=CARTESIAN_POINT ( 'NONE',  ( -1.953612668519999707, 1408.981282045029957, 231.3328323811979885 ) ) ;
#85389=CARTESIAN_POINT ( 'NONE',  ( 11.02768931129999963, 1426.931661410030074, 92.69464464869780329 ) ) ;
#85391=CARTESIAN_POINT ( 'NONE',  ( 23.34379457190000196, 1410.649718844729932, 212.3615055056179983 ) ) ;
#85392=CARTESIAN_POINT ( 'NONE',  ( 4.156515053869860310, 1424.245343161929895, 184.5679882677330284 ) ) ;
#85394=CARTESIAN_POINT ( 'NONE',  ( -2.843812590201006518, 1419.747894056850782, 186.1690033552606849 ) ) ;
#85397=CARTESIAN_POINT ( 'NONE',  ( 8.664649168559998671, 1509.043694294030047, 182.0634189174980122 ) ) ;
#85400=CARTESIAN_POINT ( 'NONE',  ( -4.363122647530000009, 1423.854802298929826, 172.2701767054979882 ) ) ;
#85404=CARTESIAN_POINT ( 'NONE',  ( -11.81903391593660047, 1429.240617403939950, 149.0414667438120091 ) ) ;
#85406=CARTESIAN_POINT ( 'NONE',  ( -0.4918994192140000443, 1474.175172928430129, 270.1377426665980011 ) ) ;
#85411=EDGE_CURVE ( 'NONE', #38088, #2271, #18454, .T. ) ;
#85412=CARTESIAN_POINT ( 'NONE',  ( 22.77127579980000149, 1411.073674597329955, 206.9287118965879984 ) ) ;
#85413=CARTESIAN_POINT ( 'NONE',  ( -22.90620825977149977, 1507.562497965029934, 208.0767490477490185 ) ) ;
#85415=CARTESIAN_POINT ( 'NONE',  ( 10.10010064645940098, 1409.265763673950005, 197.6200419344060037 ) ) ;
#85416=CARTESIAN_POINT ( 'NONE',  ( -15.54429786038520156, 1407.696428880429949, 267.7515575858669763 ) ) ;
#85419=FACE_OUTER_BOUND ( 'NONE', #9837, .T. ) ;
#85420=CARTESIAN_POINT ( 'NONE',  ( 13.77182695930000023, 1443.992469818299924, 189.0025103208980113 ) ) ;
#85422=VERTEX_POINT ( 'NONE', #38551 ) ;
#85423=CARTESIAN_POINT ( 'NONE',  ( 4.653692642196047835, 1422.133935384945516, 184.1087935189646885 ) ) ;
#85426=CARTESIAN_POINT ( 'NONE',  ( -16.93220803830000065, 1485.485519723529933, 188.1884812454979965 ) ) ;
#85429=EDGE_LOOP ( 'NONE', ( #79691, #100307, #91872 ) ) ;
#85431=CIRCLE ( 'NONE', #21088, 1.999994602351862438 ) ;
#85432=CARTESIAN_POINT ( 'NONE',  ( -5.363939304704870459, 1424.918647691059959, 151.3386706125469914 ) ) ;
#85434=CARTESIAN_POINT ( 'NONE',  ( -26.55602695130000157, 1507.993014311030038, 202.0788793302480144 ) ) ;
#85435=CARTESIAN_POINT ( 'NONE',  ( -0.5846039405770000474, 1467.892742173730085, 230.0195927640980074 ) ) ;
#85437=CARTESIAN_POINT ( 'NONE',  ( -2.930050900409999937, 1409.015380019430040, 194.3093250809980077 ) ) ;
#85441=CARTESIAN_POINT ( 'NONE',  ( -28.15858260011039960, 1508.155820277190060, 209.9842769292959872 ) ) ;
#85442=CARTESIAN_POINT ( 'NONE',  ( 26.83695571220000176, 1488.686901729329747, 212.2842936355180257 ) ) ;
#85445=CARTESIAN_POINT ( 'NONE',  ( -23.77853211389999899, 1435.327860087930048, 137.1324111805979840 ) ) ;
#85452=ORIENTED_EDGE ( 'NONE', *, *, #73055, .F. ) ;
#85453=CARTESIAN_POINT ( 'NONE',  ( -36.37832876739999932, 1451.642701153929920, 134.0999999898979809 ) ) ;
#85454=CARTESIAN_POINT ( 'NONE',  ( 3.013238820032960064, 1440.805531895070089, 157.2037823681930320 ) ) ;
#85459=CARTESIAN_POINT ( 'NONE',  ( 12.28148677300000102, 1434.518492997930025, 150.4836546675979889 ) ) ;
#85460=CARTESIAN_POINT ( 'NONE',  ( -4.191720384344816530, 1441.591968528253801, 183.6965429472514302 ) ) ;
#85461=CARTESIAN_POINT ( 'NONE',  ( -22.75670083784289943, 1508.433586079999941, 224.9338270191400113 ) ) ;
#85463=CARTESIAN_POINT ( 'NONE',  ( -2.671306766649999886, 1410.383647693430021, 186.5757153796980106 ) ) ;
#85469=CARTESIAN_POINT ( 'NONE',  ( 21.19481749090000022, 1509.644157120430236, 188.6018308473980198 ) ) ;
#85470=DIRECTION ( 'NONE',  ( -1.000000000000000000, 0.000000000000000000, 0.000000000000000000 ) ) ;
#85471=ORIENTED_EDGE ( 'NONE', *, *, #72894, .F. ) ;
#85472=CARTESIAN_POINT ( 'NONE',  ( -12.61594209390000110, 1416.825532216630108, 194.9200742095979706 ) ) ;
#85482=CARTESIAN_POINT ( 'NONE',  ( 18.96271086799999850, 1416.819756528530206, 210.2433118287679861 ) ) ;
#85484=CARTESIAN_POINT ( 'NONE',  ( 11.86716023049999968, 1432.353341358199941, 147.6509521729980179 ) ) ;
#85486=CARTESIAN_POINT ( 'NONE',  ( 37.12039286075560085, 1440.913060386880034, 254.8318130490980309 ) ) ;
#85487=ADVANCED_FACE ( 'NONE', ( #20633 ), #25895, .F. ) ;
#85489=CARTESIAN_POINT ( 'NONE',  ( -22.91663120903140083, 1507.606285602550088, 207.6071078552859888 ) ) ;
#85490=CARTESIAN_POINT ( 'NONE',  ( 10.89381921772500839, 1427.223731764126796, 149.7143491514381708 ) ) ;
#85493=AXIS2_PLACEMENT_3D ( 'NONE', #7677, #110139, #41833 ) ;
#85496=CARTESIAN_POINT ( 'NONE',  ( 9.321267295856701551, 1447.491614812988928, 186.3095919917775518 ) ) ;
#85498=CARTESIAN_POINT ( 'NONE',  ( -4.146782895030730387, 1426.018316030089863, 186.1121555109529879 ) ) ;
#85502=CARTESIAN_POINT ( 'NONE',  ( 12.98226561589999939, 1414.913060387329779, 198.3280246956980193 ) ) ;
#85505=CARTESIAN_POINT ( 'NONE',  ( 21.89882296440000076, 1452.148336636630120, 141.7804002450980079 ) ) ;
#85506=DIRECTION ( 'NONE',  ( 0.000000000000000000, 0.000000000000000000, -1.000000000000000000 ) ) ;
#85509=EDGE_LOOP ( 'NONE', ( #60575, #54824, #22537, #79707, #20443 ) ) ;
#85511=CARTESIAN_POINT ( 'NONE',  ( -1.556370308520000023, 1414.996442553830093, 226.5294865815980074 ) ) ;
#85514=ORIENTED_EDGE ( 'NONE', *, *, #109332, .T. ) ;
#85516=CARTESIAN_POINT ( 'NONE',  ( 19.16562477733859993, 1509.252401821619969, 230.4506081681080047 ) ) ;
#85518=CARTESIAN_POINT ( 'NONE',  ( 36.70747090514399957, 1437.748585611690032, 136.5500148930220234 ) ) ;
#85519=CARTESIAN_POINT ( 'NONE',  ( 18.85453636469999950, 1434.822352678469997, 208.8963608210670202 ) ) ;
#85520=CARTESIAN_POINT ( 'NONE',  ( 4.500000000000000000, 1448.210448412289907, 182.3842140122979743 ) ) ;
#85521=B_SPLINE_CURVE_WITH_KNOTS ( 'NONE', 5,
 ( #67064, #16062, #58107, #58653, #49708, #93334 ),
 .UNSPECIFIED., .F., .F.,
 ( 6, 6 ),
 ( -107.6663712510000011, -41.52559413485549555 ),
 .UNSPECIFIED. ) ;
#85523=B_SPLINE_CURVE_WITH_KNOTS ( 'NONE', 5,
 ( #33329, #7042, #102195, #110605, #14875, #101625, #51251, #17054, #57474, #108402, #6491, #24914, #23823, #85384, #66970, #49067, #99986, #15969 ),
 .UNSPECIFIED., .F., .F.,
 ( 6, 3, 3, 3, 3, 6 ),
 ( 30.30137870641080156, 39.81263101060000054, 43.27628380800000230, 45.00811020669999607, 46.73993660539999695, 49.32388343160000233 ),
 .UNSPECIFIED. ) ;
#85525=CARTESIAN_POINT ( 'NONE',  ( -0.3328314641405109575, 1452.976685807730291, 183.2631399573310205 ) ) ;
#85526=LINE ( 'NONE', #45227, #4878 ) ;
#85527=CARTESIAN_POINT ( 'NONE',  ( 2.555976562930000195, 1409.169953449729974, 186.1677122907980220 ) ) ;
#85528=CARTESIAN_POINT ( 'NONE',  ( 11.22085815260450126, 1416.913060341609935, 197.6243702213470215 ) ) ;
#85529=CARTESIAN_POINT ( 'NONE',  ( 40.27219824716285501, 1443.778079288244953, 137.1299607049654128 ) ) ;
#85532=CARTESIAN_POINT ( 'NONE',  ( -2.383806472443930069, 1450.585402367019924, 184.2442155348799986 ) ) ;
#85533=CARTESIAN_POINT ( 'NONE',  ( 1.578863831189999845, 1464.872486508430029, 236.9579546960979997 ) ) ;
#85536=CARTESIAN_POINT ( 'NONE',  ( -43.71744118499999843, 1445.751715858400075, 270.2202180345980196 ) ) ;
#85538=CARTESIAN_POINT ( 'NONE',  ( 21.97938480441199971, 1506.433683733499947, 208.7396655020440051 ) ) ;
#85539=CARTESIAN_POINT ( 'NONE',  ( 15.68240438299999973, 1430.131679172730173, 190.9216979817980189 ) ) ;
#85540=CARTESIAN_POINT ( 'NONE',  ( -1.174542368893330082E-08, 1473.852152221930055, 263.0553943314729963 ) ) ;
#85542=CARTESIAN_POINT ( 'NONE',  ( -1.350316101520000256, 1416.274718424630009, 228.0027273083979935 ) ) ;
#85544=CARTESIAN_POINT ( 'NONE',  ( -4.956485740179999766, 1416.161662173230070, 232.1584812440979988 ) ) ;
#85547=CARTESIAN_POINT ( 'NONE',  ( -0.7507406189636354199, 1485.270421196727966, 181.9807069647154378 ) ) ;
#85549=CARTESIAN_POINT ( 'NONE',  ( -45.48544670104310228, 1437.736077969160078, 266.1937296958689672 ) ) ;
#85550=CARTESIAN_POINT ( 'NONE',  ( 13.91486264393430083, 1509.328966950709855, 234.3828252105219860 ) ) ;
#85552=ORIENTED_EDGE ( 'NONE', *, *, #76033, .T. ) ;
#85554=CARTESIAN_POINT ( 'NONE',  ( -5.397656279289999581, 1433.838088931449875, 154.6405518360980125 ) ) ;
#85555=B_SPLINE_CURVE_WITH_KNOTS ( 'NONE', 3,
 ( #1379, #52897, #44491, #71384 ),
 .UNSPECIFIED., .F., .F.,
 ( 4, 4 ),
 ( 0.000000000000000000, 1.000000000000000000 ),
 .UNSPECIFIED. ) ;
#85556=CARTESIAN_POINT ( 'NONE',  ( -26.46631751370579977, 1441.292691208669794, 137.7246565571259964 ) ) ;
#85558=CARTESIAN_POINT ( 'NONE',  ( -26.62761621350209751, 1450.720643774079917, 136.4854395823020070 ) ) ;
#85559=ORIENTED_EDGE ( 'NONE', *, *, #106208, .T. ) ;
#85560=CARTESIAN_POINT ( 'NONE',  ( 23.84883432139999826, 1428.816474285830054, 231.9514347523980291 ) ) ;
#85564=CARTESIAN_POINT ( 'NONE',  ( -22.15139830485364669, 1451.884836739148795, 222.5180298453051364 ) ) ;
#85568=VERTEX_POINT ( 'NONE', #4952 ) ;
#85569=CARTESIAN_POINT ( 'NONE',  ( -8.632231662151090390, 1408.838363546260098, 270.3814370203099884 ) ) ;
#85570=CARTESIAN_POINT ( 'NONE',  ( 9.106286253189209035, 1419.188153054899885, 232.8697977723819861 ) ) ;
#85575=CARTESIAN_POINT ( 'NONE',  ( -23.11517254792869736, 1409.837221116860064, 209.7713657907539755 ) ) ;
#85576=ADVANCED_FACE ( 'NONE', ( #13334 ), #58982, .T. ) ;
#85577=CARTESIAN_POINT ( 'NONE',  ( -0.8766014945788880297, 1410.319220143099983, 185.2092218620130097 ) ) ;
#85579=CARTESIAN_POINT ( 'NONE',  ( -4.418986906789999836, 1428.481734779130193, 91.31218443469779800 ) ) ;
#85580=AXIS2_PLACEMENT_3D ( 'NONE', #86111, #69337, #9953 ) ;
#85582=CARTESIAN_POINT ( 'NONE',  ( -19.36527534830760189, 1454.515909355379790, 193.8667981925449908 ) ) ;
#85583=CARTESIAN_POINT ( 'NONE',  ( -19.03679519810000187, 1420.834773504230043, 223.8082884180979875 ) ) ;
#85584=CARTESIAN_POINT ( 'NONE',  ( 41.21152668593589397, 1456.890786767240115, 267.1395868360899613 ) ) ;
#85585=CARTESIAN_POINT ( 'NONE',  ( -2.807011052872784962, 1466.843255166033032, 235.0768055671881029 ) ) ;
#85588=EDGE_LOOP ( 'NONE', ( #69761, #59120, #63463, #59145 ) ) ;
#85589=CARTESIAN_POINT ( 'NONE',  ( -11.39963766959999880, 1433.910854737510135, 151.4262557347980191 ) ) ;
#85591=DIRECTION ( 'NONE',  ( 0.1196801093690024326, -0.9928125056733640985, 0.000000000000000000 ) ) ;
#85594=CARTESIAN_POINT ( 'NONE',  ( 25.81862830083710136, 1451.947416646700049, 135.6228482220020055 ) ) ;
#85598=CARTESIAN_POINT ( 'NONE',  ( 18.67334359839999891, 1410.488446969229926, 194.6898139266980081 ) ) ;
#85600=CARTESIAN_POINT ( 'NONE',  ( 0.3071698501290910377, 1408.923786994839929, 186.4998763197650078 ) ) ;
#85601=CARTESIAN_POINT ( 'NONE',  ( 1.113930986489999775, 1416.316097248230108, 233.2037843969979747 ) ) ;
#85604=CARTESIAN_POINT ( 'NONE',  ( 10.96947504439999932, 1432.347663815810165, 151.7701302545979729 ) ) ;
#85607=CARTESIAN_POINT ( 'NONE',  ( 3.410069871122496821, 1417.828849658407762, 234.2623983030260320 ) ) ;
#85608=VERTEX_POINT ( 'NONE', #108521 ) ;
#85609=CARTESIAN_POINT ( 'NONE',  ( 12.18581614772429944, 1415.088012641449950, 220.9247406374639979 ) ) ;
#85613=EDGE_CURVE ( 'NONE', #41682, #102562, #48153, .T. ) ;
#85616=CARTESIAN_POINT ( 'NONE',  ( -34.03169827300909844, 1450.436082776269814, 136.2420522946879942 ) ) ;
#85617=EDGE_CURVE ( 'NONE', #98935, #84728, #53526, .T. ) ;
#85619=CARTESIAN_POINT ( 'NONE',  ( -28.52406121949999829, 1451.758636109829922, 255.3819207742980097 ) ) ;
#85621=ADVANCED_FACE ( 'NONE', ( #49189 ), #67948, .T. ) ;
#85622=CARTESIAN_POINT ( 'NONE',  ( 11.92834938799999911, 1433.441347791240105, 150.0273619249979902 ) ) ;
#85623=CARTESIAN_POINT ( 'NONE',  ( 20.41675352909999930, 1443.170379823910025, 219.6133835466979747 ) ) ;
#85630=CARTESIAN_POINT ( 'NONE',  ( -3.497240116209999972, 1486.046665812830042, 182.0896961123980020 ) ) ;
#85631=CARTESIAN_POINT ( 'NONE',  ( 8.792013403107649339, 1398.173719835249358, 218.8041918917098769 ) ) ;
#85632=CARTESIAN_POINT ( 'NONE',  ( -30.28584401579999863, 1510.098977584829981, 208.7842246005000106 ) ) ;
#85633=AXIS2_PLACEMENT_3D ( 'NONE', #7853, #16776, #92961 ) ;
#85634=CARTESIAN_POINT ( 'NONE',  ( 23.30790377549999803, 1410.912174208729766, 212.5128193344479826 ) ) ;
#85635=PLANE ( 'NONE',  #52085 ) ;
#85636=CARTESIAN_POINT ( 'NONE',  ( 2.310235562019999888E-16, 1426.500992774829911, 146.0666368882980066 ) ) ;
#85638=CARTESIAN_POINT ( 'NONE',  ( 11.62179174939422666, 1434.999149959319766, 151.3709551977956380 ) ) ;
#85643=CARTESIAN_POINT ( 'NONE',  ( 0.1730928914583289846, 1478.515575105890093, 182.1581534200829822 ) ) ;
#85646=CARTESIAN_POINT ( 'NONE',  ( -1.546896711300000060, 1416.831925149330118, 228.0210885246980297 ) ) ;
#85648=CARTESIAN_POINT ( 'NONE',  ( -38.51626067329515735, 1444.740067931809563, 136.9078731636151360 ) ) ;
#85651=ORIENTED_EDGE ( 'NONE', *, *, #100040, .T. ) ;
#85653=DIRECTION ( 'NONE',  ( 1.000000000000000000, 0.000000000000000000, 1.989556701369999986E-13 ) ) ;
#85656=CARTESIAN_POINT ( 'NONE',  ( -17.27701495550000033, 1415.425644477229980, 211.8855821374380071 ) ) ;
#85661=DIRECTION ( 'NONE',  ( -1.987898964669120000E-13, 0.000000000000000000, 1.000000000000000000 ) ) ;
#85664=B_SPLINE_SURFACE_WITH_KNOTS ( 'NONE', 5, 5, ( 
 ( #29116, #63302, #97420, #38607, #72786, #54887 ),
 ( #12301, #3940, #55435, #63845, #72245, #30201 ),
 ( #64392, #98513, #55983, #90106, #13389, #47577 ),
 ( #81701, #49240, #64940, #75547, #5571, #6663 ),
 ( #109144, #66051, #50352, #109683, #48692, #82816 ),
 ( #23990, #84477, #39722, #49788, #41383, #31310 ) ),
 .UNSPECIFIED., .F., .F., .F.,
 ( 6, 6 ),
 ( 6, 6 ),
 ( 8.912615240089998281, 11.89398684980000098 ),
 ( 0.000000000000000000, 1.457234320079999979 ),
 .UNSPECIFIED. ) ;
#85666=CARTESIAN_POINT ( 'NONE',  ( 13.01671764799699993, 1416.842625005220043, 196.3343525426479914 ) ) ;
#85670=ADVANCED_FACE ( 'NONE', ( #3213 ), #54717, .F. ) ;
#85671=DIRECTION ( 'NONE',  ( -1.000000000000000000, 0.000000000000000000, 0.000000000000000000 ) ) ;
#85672=CARTESIAN_POINT ( 'NONE',  ( 5.508554876272072853, 1427.333971811663332, 137.0999999980980135 ) ) ;
#85681=CARTESIAN_POINT ( 'NONE',  ( 38.96090183549657127, 1452.356242234835236, 269.5922817352261518 ) ) ;
#85682=CARTESIAN_POINT ( 'NONE',  ( -11.60004869885203682, 1428.983126981193436, 134.0999999980979851 ) ) ;
#85683=CARTESIAN_POINT ( 'NONE',  ( 13.40566205669149902, 1429.098591087019940, 222.0107402452829888 ) ) ;
#85692=B_SPLINE_SURFACE_WITH_KNOTS ( 'NONE', 5, 5, ( 
 ( #86489, #77553, #76436, #95452, #856, #78093, #34983, #110589, #103267 ),
 ( #97654, #36104, #97109, #98193, #27695, #96560, #20375, #11995, #105513 ),
 ( #104400, #4159, #70845, #12546, #87614, #104954, #54580, #3624, #38286 ),
 ( #88715, #61881, #71947, #46725, #55128, #19832, #45630, #21466, #46178 ),
 ( #72468, #80858, #80308, #106598, #88166, #37754, #47254, #36647, #70290 ),
 ( #28804, #79217, #95997, #106059, #55676, #29337, #63001, #63538, #29883 ),
 ( #89796, #28244, #20924, #89250, #64074, #11454, #45075, #13068, #62434 ),
 ( #71397, #1968, #3076, #19266, #53469, #10902, #2525, #54037, #79769 ),
 ( #37203, #82510, #14737, #40493, #98746, #107147, #75221, #15274, #30440 ),
 ( #73574, #64626, #92540, #99280, #22006, #23128, #73011, #74120, #66285 ),
 ( #13615, #107705, #56203, #109373, #99836, #57333, #41043, #6886, #49467 ),
 ( #15806, #91459, #32650, #58414, #48925, #56760, #57870, #108249, #47803 ),
 ( #83053, #24228, #6346, #31539, #65715, #83587, #4693, #100933, #30990 ),
 ( #74671, #108804, #90897, #81938, #66827, #39397, #14181, #39948, #92000 ),
 ( #32098, #81378, #100402, #38833, #90335, #5241, #65165, #48367, #5808 ),
 ( #23685, #22556, #75762, #43812, #94759, #109909, #24765, #42156, #33190 ),
 ( #67930, #67380, #102581, #41608, #42710, #34849, #60079, #93095, #76308 ),
 ( #77959, #68480, #69038, #110458, #51116, #1267, #50565, #16367, #103140 ),
 ( #86355, #85803, #9101, #50012, #94195, #102037, #84691, #7990, #25324 ),
 ( #101478, #59520, #58962, #18035, #26440, #33735, #93632, #35405, #17465 ),
 ( #25879, #69594, #60634, #16911, #52227, #84145, #34298, #103712, #85240 ),
 ( #7445, #43268, #8536, #9638, #76865, #51666, #177, #27013, #61202 ),
 ( #95317, #77414, #719, #4031, #10769, #105937, #80167, #11324, #54991 ),
 ( #2395, #72340, #46588, #29754, #53905, #63405, #1833, #11865, #38159 ),
 ( #29215, #3485, #45495, #89114, #97520, #36512, #106469, #20246, #20790 ),
 ( #37614, #71255, #63944, #37060, #12403, #18578, #28666, #104819, #80723 ),
 ( #95863, #86911, #54447, #52773, #96983, #79637, #2940, #10202, #44378 ),
 ( #44940, #88583, #46038, #71816, #28106, #61740, #78521, #87480, #62296 ),
 ( #35967, #19702, #62871, #70158, #104268, #27557, #19130, #53332, #79087 ),
 ( #88040, #70706, #96423, #105377, #12945, #91865, #31957, #47126, #72878 ) ),
 .UNSPECIFIED., .F., .F., .F.,
 ( 6, 3, 3, 3, 3, 3, 3, 3, 3, 6 ),
 ( 6, 3, 6 ),
 ( 24.21110745940000086, 25.10805053119999997, 26.03075347299999720, 28.79941466429999863, 31.56807585549999828, 38.94969915669999949, 55.51300259679999982, 72.07630603690000726, 88.69360427520000201, 143.4983655759999976 ),
 ( 0.000000000000000000, 1.000000000000000000, 2.000000000000000000 ),
 .UNSPECIFIED. ) ;
#85693=CARTESIAN_POINT ( 'NONE',  ( -15.79903022766779941, 1414.763965172529879, 226.8475472940190230 ) ) ;
#85694=CARTESIAN_POINT ( 'NONE',  ( 16.81223453394349932, 1414.913060391199906, 210.6693087035600058 ) ) ;
#85698=CARTESIAN_POINT ( 'NONE',  ( 0.000000000000000000, 1408.913060387329779, 217.9908631324380224 ) ) ;
#85701=CARTESIAN_POINT ( 'NONE',  ( -24.38832783710000029, 1430.357083412530073, 206.4809742753880073 ) ) ;
#85702=CARTESIAN_POINT ( 'NONE',  ( -10.94965103403530016, 1425.287425078169917, 130.8065909167059999 ) ) ;
#85703=CARTESIAN_POINT ( 'NONE',  ( 17.38138781036309766, 1410.742412905310175, 192.4657863012999712 ) ) ;
#85706=CARTESIAN_POINT ( 'NONE',  ( 28.64565192311250286, 1510.024564594433514, 200.2014960864728437 ) ) ;
#85708=CARTESIAN_POINT ( 'NONE',  ( -11.43729524049999924, 1425.481262536329950, 144.1593964292979990 ) ) ;
#85710=CARTESIAN_POINT ( 'NONE',  ( 17.11935957328527991, 1460.306514732013738, 228.6623330438524420 ) ) ;
#85712=CARTESIAN_POINT ( 'NONE',  ( -36.44137682827670233, 1437.619458494599712, 136.5441383857150015 ) ) ;
#85713=EDGE_LOOP ( 'NONE', ( #51513, #64016, #29976, #66687 ) ) ;
#85714=CARTESIAN_POINT ( 'NONE',  ( 7.050167510270000548, 1396.339668515729954, 198.4643683982980065 ) ) ;
#85716=CARTESIAN_POINT ( 'NONE',  ( -16.48650050839999892, 1458.966229476530089, 230.7111281069979896 ) ) ;
#85724=CARTESIAN_POINT ( 'NONE',  ( -19.34729233231120205, 1486.470064436709890, 189.5887045964369975 ) ) ;
#85726=CARTESIAN_POINT ( 'NONE',  ( 27.36889244077043415, 1509.257027140795799, 206.1683652123398645 ) ) ;
#85727=CARTESIAN_POINT ( 'NONE',  ( 1.026021462112689964, 1420.779496623759997, 182.9306845227040128 ) ) ;
#85735=CARTESIAN_POINT ( 'NONE',  ( 11.78683996080030028, 1427.664868936200037, 147.4634367502030159 ) ) ;
#85737=EDGE_CURVE ( 'NONE', #9923, #95978, #108954, .T. ) ;
#85740=CARTESIAN_POINT ( 'NONE',  ( -13.79047275900000002, 1415.263254653229978, 220.8845754465980065 ) ) ;
#85741=CARTESIAN_POINT ( 'NONE',  ( -12.53676446056685378, 1442.773887286369018, 169.5333422587011114 ) ) ;
#85744=CARTESIAN_POINT ( 'NONE',  ( -5.441602405930001218, 1420.475810304129936, 186.6133007815980136 ) ) ;
#85751=FACE_OUTER_BOUND ( 'NONE', #2292, .T. ) ;
#85752=CARTESIAN_POINT ( 'NONE',  ( 17.95976239040000166, 1458.835784221629865, 228.1005955696979868 ) ) ;
#85755=CARTESIAN_POINT ( 'NONE',  ( 15.52481336237690179, 1507.483737832699944, 225.9069234557499897 ) ) ;
#85761=EDGE_CURVE ( 'NONE', #37407, #38555, #24994, .T. ) ;
#85762=CARTESIAN_POINT ( 'NONE',  ( -2.925857677911992027, 1485.016887262468117, 183.1345334478515099 ) ) ;
#85768=ADVANCED_FACE ( 'NONE', ( #38969 ), #66117, .T. ) ;
#85769=CARTESIAN_POINT ( 'NONE',  ( -11.27131388419999958, 1430.079666422429909, 151.1567905714979929 ) ) ;
#85772=CARTESIAN_POINT ( 'NONE',  ( -3.696522336499820760, 1396.042145791810071, 198.5686952443658697 ) ) ;
#85775=CARTESIAN_POINT ( 'NONE',  ( 13.11746251490000148, 1410.400218127729886, 228.4678513248979925 ) ) ;
#85776=EDGE_CURVE ( 'NONE', #56530, #110307, #50697, .T. ) ;
#85779=CARTESIAN_POINT ( 'NONE',  ( -16.96848018825399862, 1460.581442102934261, 228.2620679135440014 ) ) ;
#85782=CARTESIAN_POINT ( 'NONE',  ( 23.45810927580000183, 1411.272422073929874, 269.3038011074980318 ) ) ;
#85783=DIRECTION ( 'NONE',  ( 0.000000000000000000, 0.000000000000000000, 1.000000000000000000 ) ) ;
#85784=B_SPLINE_SURFACE_WITH_KNOTS ( 'NONE', 5, 5, ( 
 ( #77916, #19649, #71764, #27505, #61692, #88527 ),
 ( #87989, #11277, #54395, #45440, #79583, #62813 ),
 ( #96929, #60588, #1223, #20196, #11812, #35358 ),
 ( #45982, #3433, #37564, #26393, #17984, #95270 ),
 ( #52180, #86311, #106419, #48735, #39768, #82317 ),
 ( #5615, #64981, #5053, #20737, #21825, #91268 ) ),
 .UNSPECIFIED., .F., .F., .F.,
 ( 6, 6 ),
 ( 6, 6 ),
 ( 29.50720980499999868, 158.0245753780000086 ),
 ( 0.000000000000000000, 1.000000000000000000 ),
 .UNSPECIFIED. ) ;
#85785=CARTESIAN_POINT ( 'NONE',  ( 21.04775274920000072, 1430.296917575329871, 197.6394114472979879 ) ) ;
#85787=EDGE_CURVE ( 'NONE', #38170, #56464, #99397, .T. ) ;
#85788=CARTESIAN_POINT ( 'NONE',  ( -0.1600598377913609871, 1508.974959163609810, 238.8730780788579864 ) ) ;
#85790=CARTESIAN_POINT ( 'NONE',  ( -41.66194398591169801, 1443.744947597720056, 136.1277479405200097 ) ) ;
#85794=CARTESIAN_POINT ( 'NONE',  ( -14.01419671689999902, 1443.250645178179866, 188.5336382816979892 ) ) ;
#85797=CARTESIAN_POINT ( 'NONE',  ( -5.486708004948176232, 1457.204336652478105, 228.5178868769606595 ) ) ;
#85798=ORIENTED_EDGE ( 'NONE', *, *, #82880, .F. ) ;
#85800=CARTESIAN_POINT ( 'NONE',  ( -11.72950371754490106, 1409.322663682899929, 199.8602493023269915 ) ) ;
#85802=CARTESIAN_POINT ( 'NONE',  ( -15.05358279999999915, 1410.831827720429828, 226.7261506157979909 ) ) ;
#85803=CARTESIAN_POINT ( 'NONE',  ( -14.61105931230000010, 1474.212000672530166, 267.1471378767980127 ) ) ;
#85807=CARTESIAN_POINT ( 'NONE',  ( -24.07979781585164503, 1444.275408748464088, 212.4814690993878230 ) ) ;
#85810=CARTESIAN_POINT ( 'NONE',  ( -13.96307519100000150, 1409.400661718330184, 225.8965666933980003 ) ) ;
#85811=CARTESIAN_POINT ( 'NONE',  ( 11.61894910093169919, 1415.258594622810051, 222.9409272062040088 ) ) ;
#85815=DIRECTION ( 'NONE',  ( 0.03489949670247352587, -0.9993908270190967613, -1.907370177224992791E-14 ) ) ;
#85816=CARTESIAN_POINT ( 'NONE',  ( -23.38374426929999927, 1411.089939434129974, 205.9489912828279898 ) ) ;
#85817=CARTESIAN_POINT ( 'NONE',  ( -1.465793917108519917, 1484.360957496709943, 182.4810413606819850 ) ) ;
#85819=VECTOR ( 'NONE', #33808, 1000.000000000000227 ) ;
#85822=CARTESIAN_POINT ( 'NONE',  ( 2.461716435160000049, 1435.943783413959864, 150.4083956814980070 ) ) ;
#85827=CARTESIAN_POINT ( 'NONE',  ( -22.63947967940000083, 1410.626538670930131, 211.5335619545579959 ) ) ;
#85830=DIRECTION ( 'NONE',  ( 1.000000000000000000, 0.000000000000000000, 0.000000000000000000 ) ) ;
#85831=VECTOR ( 'NONE', #97300, 1000.000000000000114 ) ;
#85834=CARTESIAN_POINT ( 'NONE',  ( -0.5941431873634029914, 1420.625254382509866, 182.8568024079209806 ) ) ;
#85836=CARTESIAN_POINT ( 'NONE',  ( -8.704519340914814052, 1398.171442848455627, 218.7793260591613489 ) ) ;
#85837=CARTESIAN_POINT ( 'NONE',  ( -4.283857371189049523, 1440.956241081810049, 155.9231041381889895 ) ) ;
#85839=FACE_OUTER_BOUND ( 'NONE', #20053, .T. ) ;
#85842=CARTESIAN_POINT ( 'NONE',  ( 40.44627699776750518, 1447.230319210510061, 136.4061566910979764 ) ) ;
#85844=VERTEX_POINT ( 'NONE', #5252 ) ;
#85846=CARTESIAN_POINT ( 'NONE',  ( 11.83189171497950021, 1433.731675027539950, 150.7538201803880042 ) ) ;
#85847=CARTESIAN_POINT ( 'NONE',  ( 28.41776274690000292, 1509.905438290129950, 216.6186804979880094 ) ) ;
#85852=DIRECTION ( 'NONE',  ( 0.000000000000000000, 0.000000000000000000, -1.000000000000000000 ) ) ;
#85853=CARTESIAN_POINT ( 'NONE',  ( 0.8262468554639167406, 1416.839570625587157, 190.2114392743267501 ) ) ;
#85854=CARTESIAN_POINT ( 'NONE',  ( 2.893254755770000131, 1507.808732218230034, 235.9747248503979904 ) ) ;
#85855=CARTESIAN_POINT ( 'NONE',  ( 3.328465976629999989, 1507.639111981630094, 181.4822836926979903 ) ) ;
#85856=CARTESIAN_POINT ( 'NONE',  ( -2.857575698580000267, 1416.519106787730152, 191.2889195365980015 ) ) ;
#85857=CARTESIAN_POINT ( 'NONE',  ( -24.09999474531229779, 1444.794386359630153, 211.7658029478569972 ) ) ;
#85860=CARTESIAN_POINT ( 'NONE',  ( 35.52558520626859462, 1435.900183204529867, 134.0999999974749812 ) ) ;
#85861=CARTESIAN_POINT ( 'NONE',  ( 11.30119660309999929, 1432.297823534569943, 151.5221481425980130 ) ) ;
#85864=CARTESIAN_POINT ( 'NONE',  ( 13.67949770404189991, 1434.971884691610285, 148.6456809700089821 ) ) ;
#85866=VERTEX_POINT ( 'NONE', #107715 ) ;
#85867=CARTESIAN_POINT ( 'NONE',  ( 12.96754954602891452, 1444.896177199393605, 169.4263590215614386 ) ) ;
#85868=CARTESIAN_POINT ( 'NONE',  ( -1.124593200380000102, 1465.369077680330065, 236.1474170825979968 ) ) ;
#85873=CARTESIAN_POINT ( 'NONE',  ( -19.07346239651989350, 1442.276001358560052, 210.5561030354247976 ) ) ;
#85876=B_SPLINE_CURVE_WITH_KNOTS ( 'NONE', 3,
 ( #15811, #92543, #5245, #39400, #31542, #73578, #32653, #50015, #48370, #99283, #30993, #74674, #100937, #100405, #84147, #49470, #58417, #39951, #7448, #48929, #41611 ),
 .UNSPECIFIED., .F., .F.,
 ( 4, 2, 2, 2, 1, 1, 1, 1, 1, 2, 2, 2, 4 ),
 ( 0.000000000000000000, 0.2499999999998419042, 0.3749999999997623013, 0.4374999999997226108, 0.4687499999997017941, 0.4843749999996903588, 0.4921874999996844746, 0.4960937499996817546, 0.4980468749996803668, 0.4990234374996797007, 0.4999999999996790345, 0.7499999999998394618, 1.000000000000000000 ),
 .UNSPECIFIED. ) ;
#85877=EDGE_LOOP ( 'NONE', ( #1750, #84867, #106738, #79333 ) ) ;
#85879=EDGE_LOOP ( 'NONE', ( #99557, #106433, #97260, #107318, #71696 ) ) ;
#85881=EDGE_CURVE ( 'NONE', #96030, #27055, #45085, .T. ) ;
#85884=CARTESIAN_POINT ( 'NONE',  ( -10.88545445589999972, 1409.460139157529966, 189.3640148419979994 ) ) ;
#85886=CARTESIAN_POINT ( 'NONE',  ( -11.60004869885203682, 1428.983126981193436, 137.0999999980979851 ) ) ;
#85887=VERTEX_POINT ( 'NONE', #108259 ) ;
#85889=CARTESIAN_POINT ( 'NONE',  ( 22.58319838150000081, 1431.951323673850084, 217.9369709904979970 ) ) ;
#85896=CARTESIAN_POINT ( 'NONE',  ( -20.59664500279999899, 1507.763472350329948, 190.3621299396980078 ) ) ;
#85899=CARTESIAN_POINT ( 'NONE',  ( 14.79761690939999852, 1410.816705308729979, 191.5180088111980012 ) ) ;
#85900=CARTESIAN_POINT ( 'NONE',  ( -16.14808375428494003, 1486.096392924785732, 187.0799805905815845 ) ) ;
#85902=ORIENTED_EDGE ( 'NONE', *, *, #32569, .T. ) ;
#85905=CARTESIAN_POINT ( 'NONE',  ( 40.44441459949999285, 1454.056682589430011, 264.0386555474980241 ) ) ;
#85907=CARTESIAN_POINT ( 'NONE',  ( 3.406945355383976359, 1451.023871256067878, 184.0267942193613919 ) ) ;
#85909=CARTESIAN_POINT ( 'NONE',  ( -7.877053409569999332, 1508.178149367029846, 235.5567789369980005 ) ) ;
#85910=EDGE_CURVE ( 'NONE', #62647, #41404, #8941, .T. ) ;
#85912=CARTESIAN_POINT ( 'NONE',  ( -23.83018590009999826, 1446.211104711980170, 214.0005792661480086 ) ) ;
#85915=CARTESIAN_POINT ( 'NONE',  ( 19.02906815400000440, 1456.981079902029933, 225.9142998226980126 ) ) ;
#85924=CARTESIAN_POINT ( 'NONE',  ( 12.36417386409999963, 1419.802638387629941, 223.6718635272980009 ) ) ;
#85926=LINE ( 'NONE', #9229, #41453 ) ;
#85928=B_SPLINE_CURVE_WITH_KNOTS ( 'NONE', 5,
 ( #100755, #93462, #57703, #77249, #15096, #68311 ),
 .UNSPECIFIED., .F., .F.,
 ( 6, 6 ),
 ( -167.5214209060000030, -95.54118702129999008 ),
 .UNSPECIFIED. ) ;
#85929=CARTESIAN_POINT ( 'NONE',  ( 32.64372691405990423, 1435.637504776599826, 135.1055159787700006 ) ) ;
#85930=CARTESIAN_POINT ( 'NONE',  ( -27.58798392020000279, 1447.300859615939999, 137.0122922810979844 ) ) ;
#85931=CARTESIAN_POINT ( 'NONE',  ( -40.44671179960830187, 1456.761851024655243, 269.1171488671376437 ) ) ;
#85937=CARTESIAN_POINT ( 'NONE',  ( 2.409586283469999923, 1426.663880916129983, 144.1938086916980239 ) ) ;
#85938=CARTESIAN_POINT ( 'NONE',  ( 2.982880056400492030, 1425.995092949923674, 184.8396490932583163 ) ) ;
#85940=CARTESIAN_POINT ( 'NONE',  ( 14.54091120785239788, 1432.075290591040130, 190.4591005668110029 ) ) ;
#85942=CARTESIAN_POINT ( 'NONE',  ( 11.43996310808473638, 1425.781067050057572, 139.0083090113801063 ) ) ;
#85946=CARTESIAN_POINT ( 'NONE',  ( -13.00518750807362167, 1444.872235629844454, 186.2927087732988412 ) ) ;
#85947=EDGE_CURVE ( 'NONE', #7508, #98070, #26794, .T. ) ;
#85950=CARTESIAN_POINT ( 'NONE',  ( -14.16989796120989986, 1420.440730658529901, 227.4201728071160176 ) ) ;
#85951=CARTESIAN_POINT ( 'NONE',  ( -24.22787522506175506, 1450.838946662983972, 139.9861787190485529 ) ) ;
#85953=CARTESIAN_POINT ( 'NONE',  ( 25.42198949309999989, 1436.467254550020016, 137.2714020107979991 ) ) ;
#85954=CARTESIAN_POINT ( 'NONE',  ( -9.150759623799741505, 1396.232611956530036, 202.9140964477350053 ) ) ;
#85955=ADVANCED_FACE ( 'NONE', ( #41617 ), #24775, .T. ) ;
#85957=CARTESIAN_POINT ( 'NONE',  ( -16.27483966040009733, 1409.481380779909841, 225.0625982544499948 ) ) ;
#85959=EDGE_LOOP ( 'NONE', ( #11798, #4473, #44288, #22305 ) ) ;
#85960=ORIENTED_EDGE ( 'NONE', *, *, #72139, .F. ) ;
#85963=CARTESIAN_POINT ( 'NONE',  ( 10.73151125300000075, 1425.688082741829930, 96.53145859069789481 ) ) ;
#85965=CARTESIAN_POINT ( 'NONE',  ( -11.16575615629999874, 1433.014654777279929, 151.6208054879980125 ) ) ;
#85966=CARTESIAN_POINT ( 'NONE',  ( -2.829822254990304042, 1419.790776434859481, 186.1587357482032985 ) ) ;
#85967=CARTESIAN_POINT ( 'NONE',  ( -2.745154014197499937, 1419.769956470485113, 137.0999999980979851 ) ) ;
#85969=CARTESIAN_POINT ( 'NONE',  ( 7.812988826530000708, 1507.598641535930028, 182.8715579098980015 ) ) ;
#85970=CARTESIAN_POINT ( 'NONE',  ( 3.237924447490000190, 1448.965650011070238, 183.9353614378979955 ) ) ;
#85975=CARTESIAN_POINT ( 'NONE',  ( -41.66043499930000138, 1443.874479658190012, 136.1362231440980111 ) ) ;
#85977=CARTESIAN_POINT ( 'NONE',  ( -1.408322393329999977, 1471.421866497730207, 269.3348812650980335 ) ) ;
#85978=CARTESIAN_POINT ( 'NONE',  ( -11.60004869885203682, 1428.983126981193436, 137.0999999980979851 ) ) ;
#85983=CARTESIAN_POINT ( 'NONE',  ( 22.15124694530000227, 1409.851347014229987, 206.9300461489279996 ) ) ;
#85984=CARTESIAN_POINT ( 'NONE',  ( -20.59684415639999955, 1507.762623716630060, 190.3921826403979765 ) ) ;
#85985=CARTESIAN_POINT ( 'NONE',  ( -15.96958168569999970, 1519.913060387329779, 193.1522642759980215 ) ) ;
#85987=CARTESIAN_POINT ( 'NONE',  ( 6.251338861372889966, 1407.163727730510118, 197.0599927605450148 ) ) ;
#85988=CARTESIAN_POINT ( 'NONE',  ( -15.50363298934050071, 1407.833641513950170, 267.1365089329019611 ) ) ;
#85989=CARTESIAN_POINT ( 'NONE',  ( -14.45330220633330143, 1435.576072362619925, 149.6094451218459938 ) ) ;
#85990=VERTEX_POINT ( 'NONE', #6897 ) ;
#85991=CARTESIAN_POINT ( 'NONE',  ( -11.86629849080000021, 1432.349867597430148, 149.9824147457980246 ) ) ;
#85992=CARTESIAN_POINT ( 'NONE',  ( 13.48364811319999923, 1443.577837597139933, 188.2168391137979881 ) ) ;
#85998=CARTESIAN_POINT ( 'NONE',  ( -17.86906774540000242, 1470.472114943930137, 189.5573397613979978 ) ) ;
#85999=CIRCLE ( 'NONE', #53823, 22.86690257359991207 ) ;
#86003=CARTESIAN_POINT ( 'NONE',  ( 11.74107766989999924, 1415.088275290230058, 222.6191883478979889 ) ) ;
#86005=CARTESIAN_POINT ( 'NONE',  ( -26.80691778309999762, 1509.168223069730175, 201.9730100476380130 ) ) ;
#86009=CARTESIAN_POINT ( 'NONE',  ( -7.121584090669999867, 1409.161751583729938, 195.9581075241979988 ) ) ;
#86012=CARTESIAN_POINT ( 'NONE',  ( -5.782709728270000404, 1448.056422632139856, 185.4008468919979862 ) ) ;
#86014=CARTESIAN_POINT ( 'NONE',  ( -28.30909971437809958, 1508.149945971400030, 209.2281912400019905 ) ) ;
#86015=CARTESIAN_POINT ( 'NONE',  ( 26.60955424469999997, 1469.249567702030163, 209.2992017010270160 ) ) ;
#86016=CARTESIAN_POINT ( 'NONE',  ( 20.01352635799040058, 1487.439253770349978, 226.1235325421299933 ) ) ;
#86017=CARTESIAN_POINT ( 'NONE',  ( -25.50964525599999888, 1435.388358958310164, 135.5743256029979875 ) ) ;
#86018=AXIS2_PLACEMENT_3D ( 'NONE', #110314, #26869, #94610 ) ;
#86021=CARTESIAN_POINT ( 'NONE',  ( -14.77492012620000139, 1418.010700285029998, 226.9887921092979752 ) ) ;
#86024=VERTEX_POINT ( 'NONE', #60088 ) ;
#86026=CARTESIAN_POINT ( 'NONE',  ( -1.731016753280000042, 1412.842784831929976, 232.9829570279979976 ) ) ;
#86029=VERTEX_POINT ( 'NONE', #25890 ) ;
#86034=CARTESIAN_POINT ( 'NONE',  ( 12.28522815033359983, 1434.206584240389930, 149.6310126879850202 ) ) ;
#86036=CARTESIAN_POINT ( 'NONE',  ( -4.072211398493276846, 1441.024307978096203, 184.8826053890980177 ) ) ;
#86038=CARTESIAN_POINT ( 'NONE',  ( -21.27928666812490022, 1509.330136533530094, 228.3541946679790158 ) ) ;
#86041=CARTESIAN_POINT ( 'NONE',  ( 4.221485129053400343, 1441.604895247859986, 169.6123329709060101 ) ) ;
#86043=CARTESIAN_POINT ( 'NONE',  ( -3.550567568200000412, 1421.681120215429701, 184.9649535313980095 ) ) ;
#86044=CARTESIAN_POINT ( 'NONE',  ( 20.52130897869999870, 1509.391296556930001, 188.5276697472980061 ) ) ;
#86046=ORIENTED_EDGE ( 'NONE', *, *, #55579, .F. ) ;
#86059=CARTESIAN_POINT ( 'NONE',  ( 15.10371960350000009, 1409.440493898030127, 192.9533952332979823 ) ) ;
#86060=CARTESIAN_POINT ( 'NONE',  ( 17.33159144739991575, 1507.668180251339209, 230.9408620993981458 ) ) ;
#86062=EDGE_CURVE ( 'NONE', #101516, #4376, #110505, .T. ) ;
#86063=CARTESIAN_POINT ( 'NONE',  ( -2.500000000000000000, 1443.913060387330006, 150.6726614421979775 ) ) ;
#86064=CARTESIAN_POINT ( 'NONE',  ( 38.99928884940030116, 1440.913060375190071, 257.8291480320509663 ) ) ;
#86066=LINE ( 'NONE', #78774, #60521 ) ;
#86069=CARTESIAN_POINT ( 'NONE',  ( 24.65551417620000407, 1449.825726189819989, 207.1786036389680135 ) ) ;
#86072=CARTESIAN_POINT ( 'NONE',  ( -4.059748297103329406, 1426.017828923427942, 186.0954046221966109 ) ) ;
#86074=CARTESIAN_POINT ( 'NONE',  ( -22.91361795061149920, 1509.842955864680107, 188.6798147461790052 ) ) ;
#86075=CARTESIAN_POINT ( 'NONE',  ( -1.530900592538410043, 1457.980095062469900, 229.8454460011110143 ) ) ;
#86078=CARTESIAN_POINT ( 'NONE',  ( 24.10320139190000432, 1451.260843396730024, 140.0407038608980201 ) ) ;
#86081=AXIS2_PLACEMENT_3D ( 'NONE', #8686, #18737, #44524 ) ;
#86085=CARTESIAN_POINT ( 'NONE',  ( -17.29937165656953013, 1460.725061093811519, 228.2665015787683274 ) ) ;
#86087=CARTESIAN_POINT ( 'NONE',  ( 20.25449715238289627, 1509.423786278329999, 230.0845035740109950 ) ) ;
#86088=EDGE_LOOP ( 'NONE', ( #97156, #87703, #58711, #42863, #3384, #106883 ) ) ;
#86089=ORIENTED_EDGE ( 'NONE', *, *, #46735, .F. ) ;
#86092=CARTESIAN_POINT ( 'NONE',  ( 40.24658834409459729, 1443.000124224550063, 137.0450759061350254 ) ) ;
#86093=CARTESIAN_POINT ( 'NONE',  ( 20.60842128290000019, 1470.808655614429881, 209.2898127946290003 ) ) ;
#86094=CARTESIAN_POINT ( 'NONE',  ( -38.63859217040000260, 1453.572267226629947, 261.7057268775980106 ) ) ;
#86097=AXIS2_PLACEMENT_3D ( 'NONE', #74416, #13911, #40233 ) ;
#86098=CARTESIAN_POINT ( 'NONE',  ( -11.51430234028174659, 1434.846150746961939, 151.4276967473332718 ) ) ;
#86100=CARTESIAN_POINT ( 'NONE',  ( 3.859899927900000360, 1409.047851062930022, 187.4971536713979958 ) ) ;
#86102=CARTESIAN_POINT ( 'NONE',  ( -6.907297315470000143, 1441.639242787609874, 154.4648440498980051 ) ) ;
#86105=CARTESIAN_POINT ( 'NONE',  ( -23.98473687499999940, 1450.847192898529784, 140.5494830415979948 ) ) ;
#86106=CARTESIAN_POINT ( 'NONE',  ( 0.3198754856440000349, 1465.430268038429858, 236.3116685324980040 ) ) ;
#86110=CARTESIAN_POINT ( 'NONE',  ( -44.13010932679999598, 1442.529835151319958, 270.2165850160980085 ) ) ;
#86111=CARTESIAN_POINT ( 'NONE',  ( 4.500000000000000000, 1448.210448412289907, 182.3842140122979743 ) ) ;
#86112=CARTESIAN_POINT ( 'NONE',  ( 17.99954499820000109, 1410.904693969529944, 222.9872228725980108 ) ) ;
#86113=CARTESIAN_POINT ( 'NONE',  ( 16.31021256559999699, 1449.492267977409711, 190.3239795148979852 ) ) ;
#86115=CARTESIAN_POINT ( 'NONE',  ( 0.9796450454589999968, 1519.913060387329779, 185.5578019107980197 ) ) ;
#86116=CARTESIAN_POINT ( 'NONE',  ( 2.877037746629070192, 1409.300644392530103, 231.0559814730769972 ) ) ;
#86118=CARTESIAN_POINT ( 'NONE',  ( -5.334367723879999801, 1417.997726539230143, 234.5082296770980008 ) ) ;
#86120=CARTESIAN_POINT ( 'NONE',  ( -0.3233743197617713894, 1485.844240999069598, 181.8492774525526272 ) ) ;
#86122=CARTESIAN_POINT ( 'NONE',  ( -45.41124627136969849, 1437.168790165909968, 266.1958325039140618 ) ) ;
#86125=ORIENTED_EDGE ( 'NONE', *, *, #22334, .T. ) ;
#86131=CARTESIAN_POINT ( 'NONE',  ( -26.88813706803909653, 1450.873201854049967, 136.4178382659040096 ) ) ;
#86133=CARTESIAN_POINT ( 'NONE',  ( -16.27487920219974171, 1409.481386702927466, 225.0626368816978982 ) ) ;
#86136=CARTESIAN_POINT ( 'NONE',  ( 1.798881530780000126, 1414.793106040730208, 232.3921639753980344 ) ) ;
#86139=CARTESIAN_POINT ( 'NONE',  ( -25.55352470659999753, 1439.395922612140112, 138.2402125053979773 ) ) ;
#86140=ORIENTED_EDGE ( 'NONE', *, *, #52178, .T. ) ;
#86141=CARTESIAN_POINT ( 'NONE',  ( -3.047457018506829485, 1409.276789394889875, 270.3711182856380333 ) ) ;
#86143=CARTESIAN_POINT ( 'NONE',  ( 4.825278127329029942, 1416.231055590679944, 231.5676602141780052 ) ) ;
#86146=ORIENTED_EDGE ( 'NONE', *, *, #100152, .F. ) ;
#86148=CARTESIAN_POINT ( 'NONE',  ( -23.73482365112180048, 1410.983419591109850, 210.2719065163740026 ) ) ;
#86149=CARTESIAN_POINT ( 'NONE',  ( -0.5842822571356600658, 1410.310976816329912, 185.0864727095799935 ) ) ;
#86150=CARTESIAN_POINT ( 'NONE',  ( 3.637347128655072481, 1424.394824945528399, 184.3428791968424036 ) ) ;
#86151=CARTESIAN_POINT ( 'NONE',  ( -11.59417695439999996, 1428.981093279630159, 133.6118001900980232 ) ) ;
#86154=CARTESIAN_POINT ( 'NONE',  ( -19.58644262093049804, 1461.583877449769943, 193.6422725452479767 ) ) ;
#86155=CARTESIAN_POINT ( 'NONE',  ( -20.42850894749999924, 1420.829206022629933, 220.9923232775979898 ) ) ;
#86156=CARTESIAN_POINT ( 'NONE',  ( 41.14170836581870105, 1456.835253165500035, 268.3722864362400173 ) ) ;
#86158=CARTESIAN_POINT ( 'NONE',  ( -16.94780996901901204, 1421.954292645319583, 226.8349865805433296 ) ) ;
#86160=ORIENTED_EDGE ( 'NONE', *, *, #97844, .F. ) ;
#86162=CARTESIAN_POINT ( 'NONE',  ( 1.525475311809489920, 1454.505970651009875, 183.4105038380650115 ) ) ;
#86163=CARTESIAN_POINT ( 'NONE',  ( 23.39550544339999760, 1409.988940844130184, 208.4616023169569985 ) ) ;
#86166=CARTESIAN_POINT ( 'NONE',  ( 25.40507033939829995, 1452.020727665570121, 135.4560029008310096 ) ) ;
#86170=CARTESIAN_POINT ( 'NONE',  ( 18.51573764629999630, 1410.055922931730038, 194.7836524695979961 ) ) ;
#86171=CARTESIAN_POINT ( 'NONE',  ( 20.24673233129999872, 1443.913060387330006, 162.1129423953979938 ) ) ;
#86172=CARTESIAN_POINT ( 'NONE',  ( -4.500000000000000000, 1425.929641636930000, 184.1455913746980002 ) ) ;
#86174=CARTESIAN_POINT ( 'NONE',  ( -22.68797206934306487, 1432.005947149859367, 215.9728551277908650 ) ) ;
#86175=CARTESIAN_POINT ( 'NONE',  ( 6.936014448009999889, 1409.155271349029817, 229.3511990319979930 ) ) ;
#86176=AXIS2_PLACEMENT_3D ( 'NONE', #52112, #58, #67813 ) ;
#86177=CARTESIAN_POINT ( 'NONE',  ( 19.53757103644559834, 1500.216194704430109, 229.0545849299770111 ) ) ;
#86178=CARTESIAN_POINT ( 'NONE',  ( 27.68516842258932087, 1508.595246554458527, 207.6423249480233437 ) ) ;
#86182=CARTESIAN_POINT ( 'NONE',  ( 11.40717599968280105, 1432.341607277799994, 151.3374035920139988 ) ) ;
#86186=CARTESIAN_POINT ( 'NONE',  ( 0.1166470182406819933, 1506.491018773052474, 231.1523900923795907 ) ) ;
#86187=CARTESIAN_POINT ( 'NONE',  ( -19.47651265109999841, 1455.559577374430091, 243.9198229294980251 ) ) ;
#86189=CARTESIAN_POINT ( 'NONE',  ( 11.52617294090000044, 1433.738990838459813, 151.2724044377980022 ) ) ;
#86190=CARTESIAN_POINT ( 'NONE',  ( 20.63825565839999854, 1456.438754565230056, 248.0989693098979956 ) ) ;
#86191=CARTESIAN_POINT ( 'NONE',  ( 12.73594778886240064, 1416.524489948229984, 196.2724390681139823 ) ) ;
#86194=CARTESIAN_POINT ( 'NONE',  ( 19.70594995229999924, 1434.992946305079840, 210.6610983617879924 ) ) ;
#86195=CARTESIAN_POINT ( 'NONE',  ( -13.58259380279999995, 1486.033890773129997, 185.4071426780979834 ) ) ;
#86196=CARTESIAN_POINT ( 'NONE',  ( -14.04637195990000009, 1416.570631226729802, 227.2989283747980096 ) ) ;
#86199=CARTESIAN_POINT ( 'NONE',  ( 22.66911695310000141, 1410.908238429030007, 214.4050216980779737 ) ) ;
#86200=CARTESIAN_POINT ( 'NONE',  ( 2.572472979250941538, 1447.610664903252655, 170.5280182008338272 ) ) ;
#86201=CARTESIAN_POINT ( 'NONE',  ( 26.23841509872854161, 1436.700912505007864, 136.8690137196103933 ) ) ;
#86209=CARTESIAN_POINT ( 'NONE',  ( 16.81223453394349932, 1414.913060391199906, 210.6693087035600058 ) ) ;
#86210=CARTESIAN_POINT ( 'NONE',  ( 22.86388144384979881, 1435.295931049420005, 134.1000000033949959 ) ) ;
#86211=CARTESIAN_POINT ( 'NONE',  ( 13.80504973719999917, 1434.979586003610166, 149.9810039891980011 ) ) ;
#86214=ORIENTED_EDGE ( 'NONE', *, *, #73558, .F. ) ;
#86218=CARTESIAN_POINT ( 'NONE',  ( 11.59121695358153303, 1426.214086040526126, 138.6115839517644304 ) ) ;
#86219=EDGE_CURVE ( 'NONE', #1439, #77110, #99769, .T. ) ;
#86220=CARTESIAN_POINT ( 'NONE',  ( 25.78167222729700114, 1509.813387082529971, 195.1140727163279962 ) ) ;
#86221=CARTESIAN_POINT ( 'NONE',  ( 0.4435022289555869968, 1418.672171135500093, 184.7048927309859891 ) ) ;
#86222=CARTESIAN_POINT ( 'NONE',  ( 14.25613302710000063, 1464.413060387330006, 224.0689215379980226 ) ) ;
#86228=VERTEX_POINT ( 'NONE', #729 ) ;
#86229=CARTESIAN_POINT ( 'NONE',  ( -15.72121095137550206, 1409.846661881940008, 226.2995151419540036 ) ) ;
#86230=CARTESIAN_POINT ( 'NONE',  ( 2.253566441613126910E-10, 1426.918876941764893, 137.0999999980979851 ) ) ;
#86233=ORIENTED_EDGE ( 'NONE', *, *, #81571, .T. ) ;
#86237=CARTESIAN_POINT ( 'NONE',  ( 38.91493664412075049, 1452.437576044287198, 269.5915040112719225 ) ) ;
#86239=CARTESIAN_POINT ( 'NONE',  ( 15.14181670882874187, 1430.803132298357241, 219.9013560687592985 ) ) ;
#86244=CARTESIAN_POINT ( 'NONE',  ( 10.78522152235938947, 1424.939302195395612, 142.2917100169879348 ) ) ;
#86246=CARTESIAN_POINT ( 'NONE',  ( 3.709912251430000030, 1447.069506931650039, 154.3963888670980111 ) ) ;
#86247=CARTESIAN_POINT ( 'NONE',  ( -2.500000000000000000, 1432.302173844710069, 157.4936352153980010 ) ) ;
#86250=ORIENTED_EDGE ( 'NONE', *, *, #90736, .F. ) ;
#86251=CARTESIAN_POINT ( 'NONE',  ( -33.91369110859999836, 1435.681798638700002, 135.0664268289980043 ) ) ;
#86253=CARTESIAN_POINT ( 'NONE',  ( 35.51625767599999506, 1423.702336106529856, 261.8360507833979796 ) ) ;
#86255=CARTESIAN_POINT ( 'NONE',  ( -25.05872055609999904, 1449.799157997629891, 205.7769664646480123 ) ) ;
#86256=CARTESIAN_POINT ( 'NONE',  ( -11.50904860320000012, 1426.838353685629954, 127.8453462649979997 ) ) ;
#86257=CARTESIAN_POINT ( 'NONE',  ( 17.16028268420890157, 1410.456713703000105, 192.2572872432389772 ) ) ;
#86258=EDGE_CURVE ( 'NONE', #1945, #43546, #78673, .T. ) ;
#86260=CARTESIAN_POINT ( 'NONE',  ( 4.034101557127501181, 1509.184792326690058, 179.3359848413445832 ) ) ;
#86261=ADVANCED_FACE ( 'NONE', ( #86368 ), #49117, .F. ) ;
#86262=CARTESIAN_POINT ( 'NONE',  ( -18.90776566690000138, 1416.839648768930147, 208.2177105294629769 ) ) ;
#86263=CARTESIAN_POINT ( 'NONE',  ( -27.41409751149999963, 1415.612339528129951, 262.1295707058980042 ) ) ;
#86264=CARTESIAN_POINT ( 'NONE',  ( 18.98069862813439812, 1509.597656182110086, 231.8600174792910025 ) ) ;
#86265=EDGE_CURVE ( 'NONE', #43307, #6784, #91133, .T. ) ;
#86266=CARTESIAN_POINT ( 'NONE',  ( 17.44123683046308315, 1460.026124469276283, 228.4392115393495715 ) ) ;
#86269=CARTESIAN_POINT ( 'NONE',  ( -34.95989591692970322, 1437.134820888970125, 136.5390585529150087 ) ) ;
#86271=CARTESIAN_POINT ( 'NONE',  ( 6.016803703712399809, 1396.654461611120041, 220.0432444583680081 ) ) ;
#86273=CARTESIAN_POINT ( 'NONE',  ( -17.31269850480000017, 1460.709739774729996, 228.2660248434980019 ) ) ;
#86278=B_SPLINE_CURVE_WITH_KNOTS ( 'NONE', 3,
 ( #91297, #6732, #48768, #40338, #31937, #41457, #56607, #58262, #74519, #31384, #30834, #92383, #100778, #5652, #22405, #66131, #15655, #91842 ),
 .UNSPECIFIED., .F., .F.,
 ( 4, 2, 2, 2, 2, 2, 2, 2, 4 ),
 ( 1.993915778357750142E-11, 0.07958679707882590493, 0.1577458553287279797, 0.2359250188071150001, 0.2750929174303070046, 0.2946670492092580140, 0.3044529509164879966, 0.3142986040616189691, 0.3151139619271109971 ),
 .UNSPECIFIED. ) ;
#86279=ORIENTED_EDGE ( 'NONE', *, *, #35986, .T. ) ;
#86283=CARTESIAN_POINT ( 'NONE',  ( -19.54170600522309797, 1486.310841334699035, 189.8199399202851225 ) ) ;
#86284=CARTESIAN_POINT ( 'NONE',  ( 27.12970368896878171, 1508.933966457487031, 206.1969555583084457 ) ) ;
#86293=VERTEX_POINT ( 'NONE', #55004 ) ;
#86296=ORIENTED_EDGE ( 'NONE', *, *, #60329, .T. ) ;
#86297=CARTESIAN_POINT ( 'NONE',  ( -1.443364724936080146, 1457.295864005700196, 183.6403006531590165 ) ) ;
#86299=CARTESIAN_POINT ( 'NONE',  ( 8.935643129749999858, 1508.218061432530021, 235.0249814686980017 ) ) ;
#86302=CARTESIAN_POINT ( 'NONE',  ( -4.997848117199999329, 1422.516530880429855, 184.8641170294979759 ) ) ;
#86303=CARTESIAN_POINT ( 'NONE',  ( 2.328498457451699810, 1407.969193676269924, 270.2917565518350216 ) ) ;
#86306=EDGE_CURVE ( 'NONE', #50150, #24414, #17811, .T. ) ;
#86311=CARTESIAN_POINT ( 'NONE',  ( 16.60581947120000024, 1489.466620109829819, 194.3878554425980099 ) ) ;
#86313=CARTESIAN_POINT ( 'NONE',  ( 17.93975917528049990, 1421.697473349219990, 225.1225136664709794 ) ) ;
#86314=CARTESIAN_POINT ( 'NONE',  ( -5.547914922874206844, 1506.428740433108715, 187.8549363882322893 ) ) ;
#86316=CARTESIAN_POINT ( 'NONE',  ( 18.39213345135680200, 1424.508846254459968, 223.4664176072620023 ) ) ;
#86318=CARTESIAN_POINT ( 'NONE',  ( -2.994403857541957592, 1485.695008466471108, 182.6247529937351146 ) ) ;
#86322=CARTESIAN_POINT ( 'NONE',  ( 17.11711237140000108, 1414.913528139930122, 210.6775764032980192 ) ) ;
#86323=CARTESIAN_POINT ( 'NONE',  ( -24.55197755740000076, 1443.533885484360098, 210.8939174055780086 ) ) ;
#86324=CARTESIAN_POINT ( 'NONE',  ( -11.71200338719999934, 1428.227207751029937, 149.3442601595979795 ) ) ;
#86325=CARTESIAN_POINT ( 'NONE',  ( 19.44117294853580091, 1456.941945407359981, 224.4539793896520052 ) ) ;
#86327=DIRECTION ( 'NONE',  ( 0.01430194279835390707, 0.9998977151197045998, -0.0001171775870170530692 ) ) ;
#86330=CARTESIAN_POINT ( 'NONE',  ( 15.87811701990000302, 1410.407893985029887, 226.9632077383980118 ) ) ;
#86332=CARTESIAN_POINT ( 'NONE',  ( -16.12591782766000037, 1459.081375581680049, 229.9878571019870037 ) ) ;
#86334=CARTESIAN_POINT ( 'NONE',  ( 31.62445009409999841, 1415.432857817130071, 268.6459320787980118 ) ) ;
#86335=CARTESIAN_POINT ( 'NONE',  ( 24.45980407890000308, 1436.162459971299768, 138.9323611871980120 ) ) ;
#86336=CARTESIAN_POINT ( 'NONE',  ( 19.47832335489999878, 1430.302475234229860, 194.3997851820979861 ) ) ;
#86338=CARTESIAN_POINT ( 'NONE',  ( -20.74894096239999897, 1428.237764131229824, 223.0444765198980122 ) ) ;
#86341=( BOUNDED_CURVE ( )  B_SPLINE_CURVE ( 3, ( #73860, #73300, #107435, #37489 ),
 .UNSPECIFIED., .F., .F. ) 
 B_SPLINE_CURVE_WITH_KNOTS ( ( 4, 4 ),
 ( 6.175716230969100273, 6.483011094422519882 ),
 .UNSPECIFIED. ) 
 CURVE ( )  GEOMETRIC_REPRESENTATION_ITEM ( )  RATIONAL_B_SPLINE_CURVE ( ( 1.000000000000000000, 0.9921462910537798274, 0.9921462910537798274, 1.000000000000000000 ) ) 
 REPRESENTATION_ITEM ( '' )  );
#86342=CARTESIAN_POINT ( 'NONE',  ( -41.15112175996920740, 1443.645559826710041, 136.9181504865389911 ) ) ;
#86343=CARTESIAN_POINT ( 'NONE',  ( 3.827327206003189985, 1424.046157813739910, 172.2701767048200168 ) ) ;
#86344=CARTESIAN_POINT ( 'NONE',  ( -18.34777493720000408, 1415.426952350729835, 207.7346860995480142 ) ) ;
#86345=CARTESIAN_POINT ( 'NONE',  ( -16.89684486387019291, 1409.672993099775113, 193.4350317905646364 ) ) ;
#86346=CARTESIAN_POINT ( 'NONE',  ( -18.48114474329999979, 1431.113060387329824, 212.6089797988180123 ) ) ;
#86347=CARTESIAN_POINT ( 'NONE',  ( -32.74366472130000716, 1435.640891862840135, 135.1028903260980201 ) ) ;
#86348=LINE ( 'NONE', #20239, #81830 ) ;
#86349=VERTEX_POINT ( 'NONE', #6217 ) ;
#86351=CARTESIAN_POINT ( 'NONE',  ( -14.93123092370299965, 1409.434470460630109, 208.8274998085580023 ) ) ;
#86354=CARTESIAN_POINT ( 'NONE',  ( -3.014945144310587022, 1420.039793247956595, 137.0999999980981272 ) ) ;
#86355=CARTESIAN_POINT ( 'NONE',  ( -14.57206770570000032, 1474.063984277629970, 266.8771244472980015 ) ) ;
#86357=CARTESIAN_POINT ( 'NONE',  ( 0.2861219874754159509, 1419.391003853660095, 184.4958517824849764 ) ) ;
#86359=CARTESIAN_POINT ( 'NONE',  ( 17.92086665490029773, 1421.088564386509915, 224.2530476824699974 ) ) ;
#86361=B_SPLINE_SURFACE_WITH_KNOTS ( 'NONE', 5, 5, ( 
 ( #90217, #89678, #12961, #4585, #98625, #13502, #47691, #73452, #107584 ),
 ( #19719, #43562, #30870, #34044, #77714, #5690, #68234, #6223, #82392 ),
 ( #59274, #39834, #67673, #94489, #86106, #65603, #25627, #16657, #102342 ),
 ( #101780, #73997, #22442, #50855, #17204, #473, #59819, #25071, #40375 ),
 ( #42443, #34597, #74554, #48248, #93392, #90778, #57212, #17761, #93938 ),
 ( #108127, #76601, #31979, #65047, #51401, #110753, #85533, #8828, #108686 ),
 ( #31421, #99162, #99716, #56644, #43013, #14061, #77170, #68783, #91337 ),
 ( #23009, #14621, #48808, #82931, #84983, #8279, #102882, #26180, #60368 ),
 ( #51965, #9400, #53640, #46345, #70445, #11064, #61483, #78255, #20536 ) ),
 .UNSPECIFIED., .F., .F., .F.,
 ( 6, 3, 6 ),
 ( 6, 3, 6 ),
 ( 2.710078270099999909, 5.432775312530000456, 8.155472354960000558 ),
 ( 0.000000000000000000, 1.000000000000000000, 2.000000000000000000 ),
 .UNSPECIFIED. ) ;
#86363=CARTESIAN_POINT ( 'NONE',  ( 17.96129668646389632, 1424.685407009209939, 227.4171637106319963 ) ) ;
#86364=CARTESIAN_POINT ( 'NONE',  ( 22.52609269710000106, 1509.699688877929930, 227.7124812497979747 ) ) ;
#86365=CARTESIAN_POINT ( 'NONE',  ( 11.20854089337319870, 1414.996442620860080, 222.5314268542019818 ) ) ;
#86368=FACE_OUTER_BOUND ( 'NONE', #85877, .T. ) ;
#86369=CARTESIAN_POINT ( 'NONE',  ( -23.03736570619999924, 1410.638942846430155, 204.9276098081979853 ) ) ;
#86370=CARTESIAN_POINT ( 'NONE',  ( 15.65413380780000097, 1416.520322350429979, 199.0527707490979878 ) ) ;
#86374=CARTESIAN_POINT ( 'NONE',  ( -4.122931283589999374E-15, 1438.194204504490017, 150.6035180695979818 ) ) ;
#86380=CARTESIAN_POINT ( 'NONE',  ( 0.3144575102820000301, 1415.740843721930105, 233.4848348588980116 ) ) ;
#86386=CARTESIAN_POINT ( 'NONE',  ( -4.219709396322937955, 1398.038964707169271, 221.4179454279745869 ) ) ;
#86387=CARTESIAN_POINT ( 'NONE',  ( -3.210056062782554065, 1440.596314194909610, 157.0444588582195422 ) ) ;
#86391=CARTESIAN_POINT ( 'NONE',  ( 41.08515758954219876, 1445.199432839919837, 136.7286086285029967 ) ) ;
#86395=CARTESIAN_POINT ( 'NONE',  ( 11.92740228873420172, 1433.690821784659875, 150.4649736788460075 ) ) ;
#86397=ORIENTED_EDGE ( 'NONE', *, *, #56592, .T. ) ;
#86402=CARTESIAN_POINT ( 'NONE',  ( -4.363122647530000009, 1418.913060387330006, 172.2701767054979882 ) ) ;
#86403=CARTESIAN_POINT ( 'NONE',  ( 8.828869558830000130, 1428.756629641229893, 91.31218443469779800 ) ) ;
#86404=CARTESIAN_POINT ( 'NONE',  ( 6.486837805662870160, 1498.104514242190135, 235.0024069431659939 ) ) ;
#86405=EDGE_CURVE ( 'NONE', #56812, #109512, #69363, .T. ) ;
#86406=CARTESIAN_POINT ( 'NONE',  ( 9.868861043749999951, 1507.633046480430039, 183.6677869673980013 ) ) ;
#86407=CARTESIAN_POINT ( 'NONE',  ( -2.525974214079999669, 1414.913060387329779, 193.2525438407980118 ) ) ;
#86408=DIRECTION ( 'NONE',  ( 0.000000000000000000, 0.000000000000000000, -1.000000000000000000 ) ) ;
#86410=CARTESIAN_POINT ( 'NONE',  ( 37.09403179586560384, 1436.457961864639856, 134.0999999968530005 ) ) ;
#86414=CARTESIAN_POINT ( 'NONE',  ( 14.06373079481629951, 1435.540244135899911, 149.8224532940170093 ) ) ;
#86421=LINE ( 'NONE', #41667, #36666 ) ;
#86425=CARTESIAN_POINT ( 'NONE',  ( -18.98057761230930396, 1443.411275185286968, 211.6743897324382147 ) ) ;
#86428=CARTESIAN_POINT ( 'NONE',  ( 0.8791005338980000250, 1507.105016923229869, 237.2044774393979765 ) ) ;
#86429=ORIENTED_EDGE ( 'NONE', *, *, #85787, .F. ) ;
#86432=CARTESIAN_POINT ( 'NONE',  ( 22.67290673576669846, 1440.913060387330006, 230.3840297054860002 ) ) ;
#86433=CARTESIAN_POINT ( 'NONE',  ( -20.30888048250000111, 1509.664622658930057, 230.8524508361979883 ) ) ;
#86434=ORIENTED_EDGE ( 'NONE', *, *, #25586, .F. ) ;
#86436=CARTESIAN_POINT ( 'NONE',  ( -15.37265973589999923, 1410.381991858130050, 190.9834082127980253 ) ) ;
#86437=FACE_OUTER_BOUND ( 'NONE', #30356, .T. ) ;
#86438=CARTESIAN_POINT ( 'NONE',  ( -11.33192160890000011, 1414.988015876730060, 195.9133765198980086 ) ) ;
#86439=ORIENTED_EDGE ( 'NONE', *, *, #5732, .T. ) ;
#86441=CARTESIAN_POINT ( 'NONE',  ( -11.93874601188699636, 1433.484590485582430, 147.6230866160556729 ) ) ;
#86446=CARTESIAN_POINT ( 'NONE',  ( -2.482751378362429762, 1484.258609237499968, 183.2201431065910242 ) ) ;
#86450=CARTESIAN_POINT ( 'NONE',  ( 22.90250767448596037, 1409.721554337538237, 209.3445789366613496 ) ) ;
#86451=CARTESIAN_POINT ( 'NONE',  ( 28.13497766429999913, 1508.084884363030142, 208.3112646548739804 ) ) ;
#86456=ORIENTED_EDGE ( 'NONE', *, *, #57636, .F. ) ;
#86457=CARTESIAN_POINT ( 'NONE',  ( 41.56056515450000433, 1443.484422632850055, 261.5690365361979275 ) ) ;
#86459=CARTESIAN_POINT ( 'NONE',  ( -28.36642185875479782, 1509.903637666350050, 216.6464846185489819 ) ) ;
#86460=CARTESIAN_POINT ( 'NONE',  ( -7.846811853963729710, 1509.181123880980067, 237.0925084584870035 ) ) ;
#86461=CARTESIAN_POINT ( 'NONE',  ( -20.96815884289999943, 1453.795197786730114, 223.9293672322979774 ) ) ;
#86462=CARTESIAN_POINT ( 'NONE',  ( 11.86735446070000144, 1432.439707097380051, 150.3969702326980098 ) ) ;
#86463=CARTESIAN_POINT ( 'NONE',  ( 16.91835387501690136, 1409.503862420059932, 222.1480345199989870 ) ) ;
#86466=VERTEX_POINT ( 'NONE', #4316 ) ;
#86468=CARTESIAN_POINT ( 'NONE',  ( 0.3381086166239999358, 1406.067103787530186, 269.0456609344980166 ) ) ;
#86469=DIRECTION ( 'NONE',  ( 0.5412924984493711067, 0.1391731009598990432, -0.8292365640103210866 ) ) ;
#86470=CARTESIAN_POINT ( 'NONE',  ( -5.013001780754789585E-06, 1474.175194961529996, 270.1377298905089788 ) ) ;
#86472=CARTESIAN_POINT ( 'NONE',  ( -39.52868828463210349, 1448.959389328290172, 136.3024939181339903 ) ) ;
#86474=CARTESIAN_POINT ( 'NONE',  ( -40.91681241450080364, 1440.913060407800003, 260.5474447294020024 ) ) ;
#86475=CARTESIAN_POINT ( 'NONE',  ( 34.49674184778439923, 1450.393187712189956, 136.2329864103040222 ) ) ;
#86481=CARTESIAN_POINT ( 'NONE',  ( -4.026786250540000722, 1418.591992575429913, 166.2922546441980103 ) ) ;
#86483=CARTESIAN_POINT ( 'NONE',  ( 2.541163892419999737, 1448.917481751670039, 182.8661774463979839 ) ) ;
#86484=CARTESIAN_POINT ( 'NONE',  ( 13.19903007109999926, 1434.900407346980046, 146.9206655066979863 ) ) ;
#86485=AXIS2_PLACEMENT_3D ( 'NONE', #104320, #19182, #2449 ) ;
#86486=EDGE_CURVE ( 'NONE', #16730, #54104, #42871, .T. ) ;
#86489=CARTESIAN_POINT ( 'NONE',  ( -2.816489208520000235E-09, 1475.837061348030147, 266.9611530681980298 ) ) ;
#86494=AXIS2_PLACEMENT_3D ( 'NONE', #105420, #104865, #70208 ) ;
#86495=CARTESIAN_POINT ( 'NONE',  ( -18.88088134670000073, 1416.274718424630009, 207.7715298601779921 ) ) ;
#86497=CARTESIAN_POINT ( 'NONE',  ( 26.81151128603429967, 1435.638944777679853, 136.0785659481259984 ) ) ;
#86498=CARTESIAN_POINT ( 'NONE',  ( -13.42972542437900252, 1443.473990538164571, 169.3652351402658383 ) ) ;
#86502=CARTESIAN_POINT ( 'NONE',  ( -16.37287785862759648, 1409.509946165770089, 225.2661112220829693 ) ) ;
#86504=ORIENTED_EDGE ( 'NONE', *, *, #97588, .T. ) ;
#86505=ORIENTED_EDGE ( 'NONE', *, *, #38378, .T. ) ;
#86508=CARTESIAN_POINT ( 'NONE',  ( 10.34843157210000086, 1425.420399904829992, 92.68902548569779754 ) ) ;
#86511=CARTESIAN_POINT ( 'NONE',  ( 0.9523195296171770297, 1507.123350973060269, 181.0287246982449858 ) ) ;
#86512=EDGE_CURVE ( 'NONE', #77650, #87081, #85092, .T. ) ;
#86514=CARTESIAN_POINT ( 'NONE',  ( 4.146638837207450301, 1424.545683129910230, 184.9058648655890238 ) ) ;
#86515=CARTESIAN_POINT ( 'NONE',  ( -2.580094527846787056, 1420.665232545646859, 185.6742284517313237 ) ) ;
#86524=CARTESIAN_POINT ( 'NONE',  ( 2.500000000000000000, 1440.913060387330006, 209.1218459616979999 ) ) ;
#86526=CARTESIAN_POINT ( 'NONE',  ( -0.9912863951520000105, 1474.170141985030114, 270.1376065698979687 ) ) ;
#86528=CARTESIAN_POINT ( 'NONE',  ( -1.315440798330000050, 1486.372475699629831, 181.7057967760979977 ) ) ;
#86533=CARTESIAN_POINT ( 'NONE',  ( -2.500000000000000000, 1448.240815252059747, 166.0716893801519802 ) ) ;
#86535=CARTESIAN_POINT ( 'NONE',  ( 15.58731231540000017, 1409.457381327729991, 212.3362532563479874 ) ) ;
#86536=CARTESIAN_POINT ( 'NONE',  ( -3.834048154244769968, 1405.884165538340085, 268.4780263706620076 ) ) ;
#86538=CARTESIAN_POINT ( 'NONE',  ( -5.343479917770609156, 1396.099658817820000, 199.4684377796870081 ) ) ;
#86541=CARTESIAN_POINT ( 'NONE',  ( 14.14641573409999964, 1442.793379590060113, 189.5788793805980106 ) ) ;
#86550=ORIENTED_EDGE ( 'NONE', *, *, #93352, .T. ) ;
#86552=CARTESIAN_POINT ( 'NONE',  ( 12.26359346369999948, 1416.522662137829911, 223.5679345147979973 ) ) ;
#86554=CARTESIAN_POINT ( 'NONE',  ( -28.49954575200000306, 1509.595654374630158, 206.6884919356779733 ) ) ;
#86555=CARTESIAN_POINT ( 'NONE',  ( -1.117992221519999996, 1457.942518689430244, 229.8927423682980020 ) ) ;
#86560=CARTESIAN_POINT ( 'NONE',  ( -12.02002183159999937, 1447.120369466030070, 187.5076504508980122 ) ) ;
#86562=EDGE_CURVE ( 'NONE', #74812, #53095, #22171, .T. ) ;
#86564=CARTESIAN_POINT ( 'NONE',  ( 28.00748489079999715, 1508.132844955729752, 210.8183952993380217 ) ) ;
#86566=FACE_OUTER_BOUND ( 'NONE', #34572, .T. ) ;
#86567=CARTESIAN_POINT ( 'NONE',  ( -24.67107306660000177, 1435.359038600570102, 135.9357527513979846 ) ) ;
#86568=EDGE_CURVE ( 'NONE', #71251, #85568, #109120, .T. ) ;
#86571=AXIS2_PLACEMENT_3D ( 'NONE', #40912, #42027, #5675 ) ;
#86573=CARTESIAN_POINT ( 'NONE',  ( -29.22959469711409852, 1509.933780326070064, 211.7723416727030212 ) ) ;
#86576=EDGE_CURVE ( 'NONE', #37815, #87917, #71890, .T. ) ;
#86577=EDGE_LOOP ( 'NONE', ( #93899, #18501, #3255, #108981, #80045 ) ) ;
#86578=CARTESIAN_POINT ( 'NONE',  ( 2.500000000000000000, 1433.033616087690007, 157.5151964473980115 ) ) ;
#86582=CARTESIAN_POINT ( 'NONE',  ( -3.171072485709999889, 1451.871858332230204, 182.7750508701979868 ) ) ;
#86584=CARTESIAN_POINT ( 'NONE',  ( 11.69975092292400021, 1434.958819240250023, 151.3101301185499779 ) ) ;
#86586=CARTESIAN_POINT ( 'NONE',  ( 17.89184398620259842, 1478.710743812830060, 229.0921243387979871 ) ) ;
#86587=CARTESIAN_POINT ( 'NONE',  ( -24.34268787264259970, 1442.549328851149994, 212.2035684885649687 ) ) ;
#86588=CARTESIAN_POINT ( 'NONE',  ( -2.196220669999999764, 1409.923853725629897, 186.4038509670979806 ) ) ;
#86590=CARTESIAN_POINT ( 'NONE',  ( -0.1500423873502870209, 1420.467040554029836, 182.7481543114539875 ) ) ;
#86594=CARTESIAN_POINT ( 'NONE',  ( 18.52345746076924016, 1425.819856484418779, 224.6762942409735899 ) ) ;
#86596=CARTESIAN_POINT ( 'NONE',  ( -11.01105141468870130, 1414.913060387399810, 197.2110468686490208 ) ) ;
#86599=CARTESIAN_POINT ( 'NONE',  ( 3.462763369819999770, 1420.996806472229991, 185.1667669751979872 ) ) ;
#86604=DIRECTION ( 'NONE',  ( 5.525335831609270812E-11, 0.9712045719081587869, 0.2382470975787324696 ) ) ;
#86605=CARTESIAN_POINT ( 'NONE',  ( -3.692944113110000259, 1446.771170833259930, 157.7765974131980045 ) ) ;
#86606=CARTESIAN_POINT ( 'NONE',  ( -18.06991754140000239, 1424.836194406330151, 226.5046235209979955 ) ) ;
#86608=CARTESIAN_POINT ( 'NONE',  ( 16.71292568740000206, 1489.452917662229993, 194.5586640803979890 ) ) ;
#86609=CARTESIAN_POINT ( 'NONE',  ( 17.94562356750000021, 1438.546729650309999, 191.2321735587979958 ) ) ;
#86612=CARTESIAN_POINT ( 'NONE',  ( 10.92532341640084326, 1429.179526204826971, 151.1050430757466074 ) ) ;
#86613=VERTEX_POINT ( 'NONE', #65333 ) ;
#86614=CARTESIAN_POINT ( 'NONE',  ( 1.278193956753560068, 1507.616839952949931, 186.1818873165319985 ) ) ;
#86615=CARTESIAN_POINT ( 'NONE',  ( 26.89254719910000091, 1508.005806001830024, 206.4982022804780115 ) ) ;
#86616=CARTESIAN_POINT ( 'NONE',  ( -23.96906971290000143, 1437.223344794849936, 211.5767061028579974 ) ) ;
#86618=CARTESIAN_POINT ( 'NONE',  ( -3.828803044467389949, 1426.014514409073172, 186.0276948169274931 ) ) ;
#86620=CARTESIAN_POINT ( 'NONE',  ( -9.845241469799999479, 1507.507259092430104, 182.3675330799979974 ) ) ;
#86621=DIRECTION ( 'NONE',  ( 1.000000000000000000, 0.000000000000000000, 0.000000000000000000 ) ) ;
#86623=CARTESIAN_POINT ( 'NONE',  ( 12.98226561589999939, 1414.913060387329779, 198.3280246956980193 ) ) ;
#86626=CARTESIAN_POINT ( 'NONE',  ( -15.27152961130000008, 1506.433683729329914, 224.9338604266980326 ) ) ;
#86627=DIRECTION ( 'NONE',  ( 0.7628756747269003213, -0.04363816414198476434, 0.6450708608674661226 ) ) ;
#86630=CARTESIAN_POINT ( 'NONE',  ( -1.527505831896529997, 1414.913527275050001, 226.2323514033340075 ) ) ;
#86632=CARTESIAN_POINT ( 'NONE',  ( 19.87374343083660122, 1508.662439912400032, 229.4870358833140074 ) ) ;
#86634=ORIENTED_EDGE ( 'NONE', *, *, #99663, .F. ) ;
#86635=CARTESIAN_POINT ( 'NONE',  ( 14.14641573409999964, 1442.793379590060113, 189.5788793805980106 ) ) ;
#86637=CARTESIAN_POINT ( 'NONE',  ( 37.57758922502669918, 1438.291453973320131, 136.5834610766669925 ) ) ;
#86638=CARTESIAN_POINT ( 'NONE',  ( 21.99590692650000179, 1506.811133726529988, 208.7395957790290026 ) ) ;
#86639=CARTESIAN_POINT ( 'NONE',  ( -45.31147984109999527, 1446.488572564270044, 266.2043212162980126 ) ) ;
#86640=AXIS2_PLACEMENT_3D ( 'NONE', #62935, #104331, #54513 ) ;
#86643=CARTESIAN_POINT ( 'NONE',  ( -12.82978874381982770, 1435.930450547085684, 150.8169046549416237 ) ) ;
#86645=CARTESIAN_POINT ( 'NONE',  ( 2.669285241919999940, 1410.384145046430149, 185.6213876249979933 ) ) ;
#86646=CARTESIAN_POINT ( 'NONE',  ( 4.902927094849999889, 1424.294896435129886, 185.5048746948980067 ) ) ;
#86648=CARTESIAN_POINT ( 'NONE',  ( -12.48849034979999928, 1435.526019791340104, 150.8975384341979975 ) ) ;
#86650=FACE_OUTER_BOUND ( 'NONE', #97785, .T. ) ;
#86651=CARTESIAN_POINT ( 'NONE',  ( -3.063989819839999740, 1452.806063505229986, 152.9802899940980296 ) ) ;
#86654=CARTESIAN_POINT ( 'NONE',  ( -26.35475552313950232, 1507.985742420310089, 201.5462045797129917 ) ) ;
#86657=CARTESIAN_POINT ( 'NONE',  ( -43.08606230889999722, 1445.624833271280295, 270.3368636273980314 ) ) ;
#86658=CARTESIAN_POINT ( 'NONE',  ( -12.27010794651660497, 1416.835807151113613, 194.6641343636595138 ) ) ;
#86659=CARTESIAN_POINT ( 'NONE',  ( 6.692947047070000544, 1442.760174925260117, 154.8612665581980252 ) ) ;
#86662=EDGE_CURVE ( 'NONE', #28587, #36324, #32156, .T. ) ;
#86663=CARTESIAN_POINT ( 'NONE',  ( 2.865137034695680374, 1409.233255452639924, 230.9592206399570102 ) ) ;
#86665=CARTESIAN_POINT ( 'NONE',  ( -4.309299583070000494, 1417.803906166430124, 233.7804493454979990 ) ) ;
#86666=CARTESIAN_POINT ( 'NONE',  ( 4.026786250540000722, 1432.413060387330006, 146.1721969590979882 ) ) ;
#86668=CARTESIAN_POINT ( 'NONE',  ( -46.22591519347989930, 1439.214963125549957, 267.5912708118539740 ) ) ;
#86669=CARTESIAN_POINT ( 'NONE',  ( -2.500000000000000000, 1418.913060387330006, 172.2701767054979882 ) ) ;
#86672=ORIENTED_EDGE ( 'NONE', *, *, #60271, .T. ) ;
#86675=CARTESIAN_POINT ( 'NONE',  ( 19.30779799461502932, 1456.580107245917134, 224.6839345049536121 ) ) ;
#86680=EDGE_CURVE ( 'NONE', #63865, #48606, #91845, .T. ) ;
#86681=CARTESIAN_POINT ( 'NONE',  ( -15.16694981760000083, 1488.813684182929819, 194.2846367734980220 ) ) ;
#86691=CARTESIAN_POINT ( 'NONE',  ( -4.798351648711870254, 1410.228040598270127, 269.8672392053869658 ) ) ;
#86693=CARTESIAN_POINT ( 'NONE',  ( 6.381981878911410000, 1416.920506164580047, 231.2616950943009897 ) ) ;
#86696=ORIENTED_EDGE ( 'NONE', *, *, #102147, .F. ) ;
#86697=EDGE_LOOP ( 'NONE', ( #11065, #93559, #108876, #53658 ) ) ;
#86699=CARTESIAN_POINT ( 'NONE',  ( -4.400277592110000136, 1425.922606744830091, 186.1626553210980148 ) ) ;
#86700=CARTESIAN_POINT ( 'NONE',  ( 3.627844022310690697, 1424.520533308087352, 184.5083861543649277 ) ) ;
#86701=CARTESIAN_POINT ( 'NONE',  ( -0.01068885454432250137, 1408.933329768819704, 186.2235385012060078 ) ) ;
#86703=CARTESIAN_POINT ( 'NONE',  ( -20.08296050208739914, 1477.456190548399945, 193.1386059401030195 ) ) ;
#86704=CARTESIAN_POINT ( 'NONE',  ( -18.89960126629999948, 1420.835424610929977, 224.0556394152980033 ) ) ;
#86706=CARTESIAN_POINT ( 'NONE',  ( 39.30292780399409480, 1459.546458005919931, 267.2018548829190081 ) ) ;
#86707=CARTESIAN_POINT ( 'NONE',  ( -5.924191439393101000, 1466.159508804048073, 234.1209534312763481 ) ) ;
#86708=CARTESIAN_POINT ( 'NONE',  ( 8.813431017979999282, 1446.116337443820157, 185.6059072443980256 ) ) ;
#86711=VERTEX_POINT ( 'NONE', #27170 ) ;
#86713=CARTESIAN_POINT ( 'NONE',  ( 1.479066938756839811, 1478.749526688280184, 182.3503021183099975 ) ) ;
#86714=CARTESIAN_POINT ( 'NONE',  ( 22.77629783569999944, 1409.717017837230060, 208.7225517380699955 ) ) ;
#86717=CARTESIAN_POINT ( 'NONE',  ( 26.22604730430230191, 1450.757778662670034, 136.6085202351380019 ) ) ;
#86721=CARTESIAN_POINT ( 'NONE',  ( 18.21434415869999768, 1409.713951146429963, 194.9538956094980335 ) ) ;
#86722=B_SPLINE_SURFACE_WITH_KNOTS ( 'NONE', 2, 1, ( 
 ( #85886, #104905 ),
 ( #69115, #43351 ),
 ( #77499, #34928 ),
 ( #28193, #102657 ),
 ( #1918, #19785 ) ),
 .UNSPECIFIED., .F., .F., .F.,
 ( 3, 2, 3 ),
 ( 2, 2 ),
 ( 0.000000000000000000, 0.5000000000000000000, 1.000000000000000000 ),
 ( 0.000000000000000000, 1.000000000000000000 ),
 .UNSPECIFIED. ) ;
#86723=CARTESIAN_POINT ( 'NONE',  ( 27.95977047539996718, 1444.740067931808653, 175.9996750486979238 ) ) ;
#86725=CARTESIAN_POINT ( 'NONE',  ( 3.089875597163601828, 1439.679630760519331, 184.1893751638651509 ) ) ;
#86727=CARTESIAN_POINT ( 'NONE',  ( -21.48378771895310990, 1429.065913162214201, 219.3372196911616356 ) ) ;
#86728=CARTESIAN_POINT ( 'NONE',  ( 1.167028762698379962, 1450.781002157910052, 181.8366260879649872 ) ) ;
#86734=ORIENTED_EDGE ( 'NONE', *, *, #13053, .T. ) ;
#86737=CARTESIAN_POINT ( 'NONE',  ( -0.2964179489810150336, 1408.950247830049875, 232.0370909886389938 ) ) ;
#86738=DIRECTION ( 'NONE',  ( 0.000000000000000000, 0.000000000000000000, -1.000000000000000000 ) ) ;
#86741=CARTESIAN_POINT ( 'NONE',  ( 1.332267629549999902E-15, 1453.913060387330006, 209.1218459616979999 ) ) ;
#86743=CARTESIAN_POINT ( 'NONE',  ( 11.89240926010000088, 1433.292849282470115, 150.1795062545980102 ) ) ;
#86744=CARTESIAN_POINT ( 'NONE',  ( 23.42675388609999843, 1440.913060387330006, 234.3916895593979746 ) ) ;
#86747=CARTESIAN_POINT ( 'NONE',  ( 26.10499783855849998, 1440.913060396819901, 222.4284486497450075 ) ) ;
#86749=CARTESIAN_POINT ( 'NONE',  ( 7.628773549489999972, 1416.913060387330006, 201.4930723711279938 ) ) ;
#86750=CARTESIAN_POINT ( 'NONE',  ( 22.11554775090000291, 1489.452917662729988, 210.6419443847580055 ) ) ;
#86751=CARTESIAN_POINT ( 'NONE',  ( -12.11110426309999966, 1485.984702322530211, 184.7620324990980123 ) ) ;
#86753=CARTESIAN_POINT ( 'NONE',  ( -25.60272812314580193, 1509.807125272330040, 193.2161752248550215 ) ) ;
#86754=B_SPLINE_CURVE_WITH_KNOTS ( 'NONE', 5,
 ( #98195, #74673, #89798, #5244, #73576, #108251, #64628, #107707, #40495 ),
 .UNSPECIFIED., .F., .F.,
 ( 6, 3, 6 ),
 ( -133.6064266969999892, -37.05188947199999916, -29.74344005870001695 ),
 .UNSPECIFIED. ) ;
#86755=CARTESIAN_POINT ( 'NONE',  ( 25.79285008279999758, 1449.806912616609907, 209.2669309290440083 ) ) ;
#86757=CARTESIAN_POINT ( 'NONE',  ( 25.08533235215197621, 1436.600044169495050, 137.7642755019057859 ) ) ;
#86765=CARTESIAN_POINT ( 'NONE',  ( 16.06428792994640276, 1414.913060387329779, 208.9262477894010033 ) ) ;
#86767=CARTESIAN_POINT ( 'NONE',  ( -5.429027349949509862, 1440.820888839999952, 154.8047238236129886 ) ) ;
#86768=CARTESIAN_POINT ( 'NONE',  ( -36.53452253901330238, 1451.194196174219996, 134.0999999986999853 ) ) ;
#86771=EDGE_LOOP ( 'NONE', ( #15663, #60572, #86634, #66632, #88798, #106796, #52576 ) ) ;
#86774=CARTESIAN_POINT ( 'NONE',  ( -15.58852115169999841, 1416.217772598429974, 219.1616263515979881 ) ) ;
#86775=CARTESIAN_POINT ( 'NONE',  ( -7.622164505680827595, 1509.179741253262137, 237.4777701423770111 ) ) ;
#86779=CARTESIAN_POINT ( 'NONE',  ( 14.02074821061520105, 1409.402675702379838, 214.2751657983629912 ) ) ;
#86782=CARTESIAN_POINT ( 'NONE',  ( 2.872763827723777919, 1464.652692434768142, 236.7382211450293426 ) ) ;
#86787=EDGE_LOOP ( 'NONE', ( #103778, #3952, #86233, #104081, #17706 ) ) ;
#86788=CARTESIAN_POINT ( 'NONE',  ( -16.93884325354670040, 1507.634939694479954, 230.1482608329069990 ) ) ;
#86793=CARTESIAN_POINT ( 'NONE',  ( 29.89039938633745308, 1462.329368749827381, 269.4696393147128219 ) ) ;
#86794=CARTESIAN_POINT ( 'NONE',  ( 21.24668427616252586, 1409.655010951418035, 207.1560907808110699 ) ) ;
#86795=CARTESIAN_POINT ( 'NONE',  ( -0.07152471987069999870, 1397.597829882229917, 222.1216538354979946 ) ) ;
#86796=CARTESIAN_POINT ( 'NONE',  ( 22.62861454470000311, 1507.212883763329955, 209.7205631874760172 ) ) ;
#86798=CARTESIAN_POINT ( 'NONE',  ( -22.73782204790000350, 1507.861822361731356, 224.9164116726981320 ) ) ;
#86800=CARTESIAN_POINT ( 'NONE',  ( -4.363122647530000009, 1407.471318475729959, 121.6099336315979969 ) ) ;
#86801=CARTESIAN_POINT ( 'NONE',  ( -15.74154698502330163, 1459.394320999469983, 230.7248352790539911 ) ) ;
#86804=CARTESIAN_POINT ( 'NONE',  ( -2.500000000000000000, 1438.044549794279874, 157.6830143192980245 ) ) ;
#86805=CARTESIAN_POINT ( 'NONE',  ( 14.35446001680000094, 1416.822692809430009, 196.6654167759980396 ) ) ;
#86808=DIRECTION ( 'NONE',  ( -1.065814103640000080E-14, -1.000000000000000000, -2.775557561560010037E-16 ) ) ;
#86812=CARTESIAN_POINT ( 'NONE',  ( -24.22746707429999802, 1430.355866426629973, 205.9027524981279953 ) ) ;
#86813=CARTESIAN_POINT ( 'NONE',  ( -11.01818088618090030, 1425.247880495119944, 135.2555266203450230 ) ) ;
#86815=CARTESIAN_POINT ( 'NONE',  ( 16.96718384375279953, 1410.138872099130140, 192.2499806778830020 ) ) ;
#86817=CARTESIAN_POINT ( 'NONE',  ( 2.070655153456132602, 1509.117836878747084, 179.1218456497088312 ) ) ;
#86818=CARTESIAN_POINT ( 'NONE',  ( -19.76088122879999887, 1434.994518314420247, 207.7852199276980230 ) ) ;
#86819=CARTESIAN_POINT ( 'NONE',  ( -34.21460435710000070, 1436.526926585939918, 250.0133502278980018 ) ) ;
#86820=CARTESIAN_POINT ( 'NONE',  ( 14.64682994990399933, 1509.425018640689814, 234.5784246007609966 ) ) ;
#86821=CARTESIAN_POINT ( 'NONE',  ( 28.46393112515930213, 1508.969040159859787, 209.4476463742820158 ) ) ;
#86824=CARTESIAN_POINT ( 'NONE',  ( 33.14938140729999816, 1451.300093685830007, 135.9684403000979955 ) ) ;
#86826=CARTESIAN_POINT ( 'NONE',  ( 5.343474245058209782, 1396.099658619720003, 218.7752572416549981 ) ) ;
#86828=CARTESIAN_POINT ( 'NONE',  ( -16.94140410150000164, 1460.101846531930050, 228.3559701019979968 ) ) ;
#86832=CARTESIAN_POINT ( 'NONE',  ( -6.330596753318919134, 1422.104800618580157, 147.4057733953199829 ) ) ;
#86833=ORIENTED_EDGE ( 'NONE', *, *, #35755, .F. ) ;
#86834=CARTESIAN_POINT ( 'NONE',  ( 0.1127810345220000010, 1412.052416346030213, 184.9056086049980081 ) ) ;
#86836=CARTESIAN_POINT ( 'NONE',  ( -12.10873113499999931, 1442.495059057370099, 187.0567141033980079 ) ) ;
#86837=CARTESIAN_POINT ( 'NONE',  ( -11.61555427849999944, 1470.475265069229863, 231.8199702359979710 ) ) ;
#86845=VERTEX_POINT ( 'NONE', #24873 ) ;
#86846=CARTESIAN_POINT ( 'NONE',  ( 11.83078866654130046, 1429.952306642770054, 149.4451526254590021 ) ) ;
#86847=CARTESIAN_POINT ( 'NONE',  ( 13.03352849233194632, 1444.854847888656423, 186.9825230085123167 ) ) ;
#86851=CARTESIAN_POINT ( 'NONE',  ( 8.903625402870000372, 1507.331954555630091, 234.8124830750979868 ) ) ;
#86854=CARTESIAN_POINT ( 'NONE',  ( -4.642209649809999839, 1422.070992366130213, 184.6618742118980094 ) ) ;
#86855=CARTESIAN_POINT ( 'NONE',  ( 4.854327180553859478, 1409.980837898999880, 270.0724508720410313 ) ) ;
#86863=CARTESIAN_POINT ( 'NONE',  ( -4.363123796622770278, 1423.854800546939941, 184.2546035468919854 ) ) ;
#86865=CARTESIAN_POINT ( 'NONE',  ( -2.499957339863959849, 1419.383168421049959, 144.0964016714840170 ) ) ;
#86867=CARTESIAN_POINT ( 'NONE',  ( 31.32742178079999462, 1437.308404694980027, 255.3819207742980097 ) ) ;
#86873=VERTEX_POINT ( 'NONE', #92107 ) ;
#86874=CARTESIAN_POINT ( 'NONE',  ( 17.09240173490840320, 1414.913527292460003, 210.5647920935599871 ) ) ;
#86875=CARTESIAN_POINT ( 'NONE',  ( -24.21003924839999755, 1443.294921534809873, 211.9567361259179847 ) ) ;
#86876=CARTESIAN_POINT ( 'NONE',  ( -2.278072849319670468, 1449.813593373988624, 154.3981412275377068 ) ) ;
#86878=CARTESIAN_POINT ( 'NONE',  ( -5.804923445810000082, 1441.820529667599885, 184.4027335045979896 ) ) ;
#86879=CARTESIAN_POINT ( 'NONE',  ( -1.876662632594598978, 1395.978594890587374, 198.1101541364135130 ) ) ;
#86882=CARTESIAN_POINT ( 'NONE',  ( 5.885111936350000406, 1415.073945855430111, 231.3228053793980052 ) ) ;
#86884=CARTESIAN_POINT ( 'NONE',  ( -16.85240214550000104, 1460.648904765030011, 228.2641506848979986 ) ) ;
#86886=CARTESIAN_POINT ( 'NONE',  ( 31.61313467960000168, 1415.423113773229716, 266.8259304570980248 ) ) ;
#86889=CARTESIAN_POINT ( 'NONE',  ( 22.92537184140000051, 1488.580164505829998, 195.5505115141980070 ) ) ;
#86890=CARTESIAN_POINT ( 'NONE',  ( -20.51879148909999984, 1428.070798452130020, 222.7953178437979886 ) ) ;
#86897=DIRECTION ( 'NONE',  ( 1.000000000000000000, 0.000000000000000000, 1.988211042460000085E-13 ) ) ;
#86899=CARTESIAN_POINT ( 'NONE',  ( -12.64870551279999944, 1442.301404759220077, 187.5798431206980013 ) ) ;
#86902=B_SPLINE_SURFACE_WITH_KNOTS ( 'NONE', 5, 5, ( 
 ( #44298, #95238, #95786, #1755, #10127, #53256 ),
 ( #78441, #86834, #12319, #52698, #19620, #96898 ),
 ( #105290, #54903, #20706, #105854, #80086, #97439 ),
 ( #11779, #2314, #19053, #70076, #89029, #10691 ),
 ( #3404, #29132, #18502, #63320, #35892, #104189 ),
 ( #80642, #27471, #2852, #70618, #3957, #20168 ) ),
 .UNSPECIFIED., .F., .F., .F.,
 ( 6, 6 ),
 ( 6, 6 ),
 ( 30.42592446739999801, 42.69308682570000002 ),
 ( 0.000000000000000000, 2.000000000000000000 ),
 .UNSPECIFIED. ) ;
#86904=CARTESIAN_POINT ( 'NONE',  ( -29.18328456680000116, 1435.993529926829979, 136.4438111567980059 ) ) ;
#86908=CARTESIAN_POINT ( 'NONE',  ( -11.93719948218080162, 1409.329916578820075, 200.1248561717409871 ) ) ;
#86911=CARTESIAN_POINT ( 'NONE',  ( -42.24861265719999892, 1455.960523536630035, 266.5276627523979869 ) ) ;
#86913=CARTESIAN_POINT ( 'NONE',  ( 0.1664555413521620064, 1420.066918388370141, 183.9183786667229867 ) ) ;
#86914=CARTESIAN_POINT ( 'NONE',  ( 17.81579863472509828, 1417.685313260180010, 224.1428778951429877 ) ) ;
#86916=CARTESIAN_POINT ( 'NONE',  ( 17.59742321542820065, 1423.715947681140051, 226.4556487353030150 ) ) ;
#86917=CARTESIAN_POINT ( 'NONE',  ( 17.05693858869999957, 1415.931669658029932, 215.3161187075879752 ) ) ;
#86918=CARTESIAN_POINT ( 'NONE',  ( -28.27864386137849806, 1508.411229484100204, 208.8441910969250159 ) ) ;
#86920=CARTESIAN_POINT ( 'NONE',  ( -26.30762031710139937, 1482.696347288150037, 210.8481448672619933 ) ) ;
#86922=CARTESIAN_POINT ( 'NONE',  ( -7.779176540490000846, 1507.931165456829831, 181.6769597819979936 ) ) ;
#86923=CARTESIAN_POINT ( 'NONE',  ( -22.57962297529999773, 1409.701558196430142, 208.4161775753709946 ) ) ;
#86927=CARTESIAN_POINT ( 'NONE',  ( -11.97668390569999985, 1433.616603791269881, 149.8660147765980071 ) ) ;
#86933=CARTESIAN_POINT ( 'NONE',  ( 1.356502502699999946, 1410.320696391030197, 232.6392733810980076 ) ) ;
#86936=CARTESIAN_POINT ( 'NONE',  ( -22.92154104720000163, 1411.040135743629889, 211.1056462352579786 ) ) ;
#86937=B_SPLINE_CURVE_WITH_KNOTS ( 'NONE', 3,
 ( #78914, #104090, #94574, #87867, #86186, #61022, #45864, #9478, #52604, #27382, #61562 ),
 .UNSPECIFIED., .F., .F.,
 ( 4, 2, 1, 2, 2, 4 ),
 ( 0.000000000000000000, 0.2500000000001444955, 0.3750000000003331224, 0.4375000000002918221, 0.5000000000002505773, 1.000000000000000000 ),
 .UNSPECIFIED. ) ;
#86942=CARTESIAN_POINT ( 'NONE',  ( -14.57927006065989950, 1484.949786830110043, 186.8775221956059909 ) ) ;
#86943=CARTESIAN_POINT ( 'NONE',  ( -18.20429502950000256, 1430.266005493330113, 193.4350815501980208 ) ) ;
#86944=CARTESIAN_POINT ( 'NONE',  ( 40.65306745188510007, 1445.156483018170093, 136.9198483831620194 ) ) ;
#86948=CARTESIAN_POINT ( 'NONE',  ( 11.23895917067440031, 1434.009643533409871, 151.5816975370499904 ) ) ;
#86950=EDGE_LOOP ( 'NONE', ( #93514, #101519, #36830, #26358, #33888, #30491, #13521 ) ) ;
#86951=CARTESIAN_POINT ( 'NONE',  ( 25.78167222729700114, 1509.813387082529971, 195.1140727163279962 ) ) ;
#86954=CARTESIAN_POINT ( 'NONE',  ( 13.88894654940479967, 1452.878337568840152, 223.9947615367189826 ) ) ;
#86955=CARTESIAN_POINT ( 'NONE',  ( 11.96519809220000141, 1440.444625599219989, 147.6189886498980002 ) ) ;
#86956=CARTESIAN_POINT ( 'NONE',  ( 11.84776047779999963, 1488.164498195129909, 185.6409340852979994 ) ) ;
#86957=CARTESIAN_POINT ( 'NONE',  ( -4.988720663300000524, 1414.971262582530017, 193.0978923767980007 ) ) ;
#86958=CARTESIAN_POINT ( 'NONE',  ( -24.28150245826429909, 1444.786156486610025, 211.3238323467629982 ) ) ;
#86959=EDGE_CURVE ( 'NONE', #97932, #50075, #66932, .T. ) ;
#86961=FACE_OUTER_BOUND ( 'NONE', #19421, .T. ) ;
#86965=CARTESIAN_POINT ( 'NONE',  ( 14.04488167959519984, 1435.070998900880113, 149.0410152460709980 ) ) ;
#86969=ORIENTED_EDGE ( 'NONE', *, *, #15359, .F. ) ;
#86972=CARTESIAN_POINT ( 'NONE',  ( 9.583090267181649580, 1451.335710444785946, 152.4223268313591859 ) ) ;
#86974=B_SPLINE_CURVE_WITH_KNOTS ( 'NONE', 5,
 ( #21450, #73001, #82494, #5796, #108237, #31525, #106587, #47240, #81368, #88702, #107135, #11983 ),
 .UNSPECIFIED., .F., .F.,
 ( 6, 3, 3, 6 ),
 ( 13.14991324430000041, 14.22551365930000067, 16.37671448909999938, 17.67668238079999909 ),
 .UNSPECIFIED. ) ;
#86979=CARTESIAN_POINT ( 'NONE',  ( 4.228534147342459804, 1446.279633625890028, 165.3434763453030030 ) ) ;
#86980=CARTESIAN_POINT ( 'NONE',  ( 0.8620940066740000463, 1508.701006820629800, 238.1167471285979786 ) ) ;
#86984=CARTESIAN_POINT ( 'NONE',  ( 31.37724852291990629, 1440.913060387330006, 254.8116090844129644 ) ) ;
#86985=CARTESIAN_POINT ( 'NONE',  ( -20.13259487519999880, 1508.866008678130129, 188.8141320356980088 ) ) ;
#86986=ORIENTED_EDGE ( 'NONE', *, *, #66493, .T. ) ;
#86987=CARTESIAN_POINT ( 'NONE',  ( 25.55809122598300220, 1449.022359460670032, 137.9040320589840292 ) ) ;
#86988=CARTESIAN_POINT ( 'NONE',  ( -14.18461090829999982, 1409.408397915129854, 191.4295514316980018 ) ) ;
#86989=CARTESIAN_POINT ( 'NONE',  ( -24.89775034519999863, 1442.835538705840008, 210.5176537872779932 ) ) ;
#86990=FACE_OUTER_BOUND ( 'NONE', #97991, .T. ) ;
#86993=CARTESIAN_POINT ( 'NONE',  ( -13.19837685220000090, 1434.900414701970021, 149.9808420605980075 ) ) ;
#86995=ADVANCED_FACE ( 'NONE', ( #24340 ), #60181, .T. ) ;
#86999=CARTESIAN_POINT ( 'NONE',  ( 24.08426584000000048, 1411.115194200730002, 209.6325720084630007 ) ) ;
#87006=CARTESIAN_POINT ( 'NONE',  ( -17.26876010021493713, 1486.136097085410938, 187.8972013554511875 ) ) ;
#87009=CARTESIAN_POINT ( 'NONE',  ( 26.69977470550000120, 1440.913060384380060, 225.7788486227980229 ) ) ;
#87012=CARTESIAN_POINT ( 'NONE',  ( -3.979020191233149539, 1509.031297583600008, 238.1276855365710219 ) ) ;
#87015=CARTESIAN_POINT ( 'NONE',  ( 11.77676742070000060, 1432.864137865029988, 150.8103446446980058 ) ) ;
#87016=CARTESIAN_POINT ( 'NONE',  ( 17.36536559375440092, 1409.655994655129916, 222.4839180234889966 ) ) ;
#87017=FACE_OUTER_BOUND ( 'NONE', #6639, .T. ) ;
#87019=ORIENTED_EDGE ( 'NONE', *, *, #81853, .F. ) ;
#87022=CARTESIAN_POINT ( 'NONE',  ( 0.5579742739800001017, 1405.845050212329852, 267.2348424307979826 ) ) ;
#87025=EDGE_CURVE ( 'NONE', #88136, #31171, #42815, .T. ) ;
#87026=CARTESIAN_POINT ( 'NONE',  ( 13.31649357393960109, 1472.985448371380016, 270.2713846310770123 ) ) ;
#87030=EDGE_CURVE ( 'NONE', #36359, #80118, #283, .T. ) ;
#87032=CARTESIAN_POINT ( 'NONE',  ( -27.15512466070000031, 1447.232094089440125, 137.0395159971979808 ) ) ;
#87037=EDGE_CURVE ( 'NONE', #87953, #64662, #12569, .T. ) ;
#87039=CARTESIAN_POINT ( 'NONE',  ( -38.89334934265168187, 1452.475886767586871, 269.5913128745133349 ) ) ;
#87041=CARTESIAN_POINT ( 'NONE',  ( 2.864767215090000096, 1448.949360505710047, 183.5737851087979777 ) ) ;
#87042=ADVANCED_FACE ( 'NONE', ( #97088 ), #41060, .T. ) ;
#87045=CARTESIAN_POINT ( 'NONE',  ( -0.4449673945539999731, 1417.362505061330012, 235.1883008639979948 ) ) ;
#87051=FACE_OUTER_BOUND ( 'NONE', #70943, .T. ) ;
#87053=CARTESIAN_POINT ( 'NONE',  ( 26.80685737241160282, 1436.288909910419989, 136.6593321135579799 ) ) ;
#87054=B_SPLINE_CURVE_WITH_KNOTS ( 'NONE', 5,
 ( #99148, #48234, #65587, #91321, #81255, #14044 ),
 .UNSPECIFIED., .F., .F.,
 ( 6, 6 ),
 ( 0.000000000000000000, 1.000000000000000000 ),
 .UNSPECIFIED. ) ;
#87055=CARTESIAN_POINT ( 'NONE',  ( -13.41929410752786822, 1443.449162763163940, 169.3662372747166387 ) ) ;
#87057=EDGE_CURVE ( 'NONE', #92171, #110603, #34125, .T. ) ;
#87058=CARTESIAN_POINT ( 'NONE',  ( -16.29829464476939904, 1409.490388075790179, 225.2024797511170107 ) ) ;
#87059=CARTESIAN_POINT ( 'NONE',  ( 7.467133905529999893, 1443.913060387330006, 149.7989312978980081 ) ) ;
#87060=ORIENTED_EDGE ( 'NONE', *, *, #72151, .F. ) ;
#87063=ADVANCED_FACE ( 'NONE', ( #3600 ), #100952, .F. ) ;
#87065=CARTESIAN_POINT ( 'NONE',  ( 11.05993000279999983, 1426.915704966229896, 94.99998741569790184 ) ) ;
#87068=B_SPLINE_CURVE_WITH_KNOTS ( 'NONE', 3,
 ( #108596, #31884, #107482, #65512 ),
 .UNSPECIFIED., .F., .F.,
 ( 4, 4 ),
 ( -128.3330504879999978, -82.60380882990649809 ),
 .UNSPECIFIED. ) ;
#87073=AXIS2_PLACEMENT_3D ( 'NONE', #62955, #35487, #69681 ) ;
#87076=CARTESIAN_POINT ( 'NONE',  ( 2.540129801540000010, 1449.030645993539792, 182.8575104869979953 ) ) ;
#87081=VERTEX_POINT ( 'NONE', #103116 ) ;
#87083=CARTESIAN_POINT ( 'NONE',  ( -15.77403878809999860, 1409.463901959830082, 192.8704306968979836 ) ) ;
#87084=CARTESIAN_POINT ( 'NONE',  ( -2.236976319609999653, 1471.546594272430184, 269.6154293286980419 ) ) ;
#87086=CARTESIAN_POINT ( 'NONE',  ( 0.1582547704020000057, 1486.366246513129909, 181.8206974649980054 ) ) ;
#87089=CARTESIAN_POINT ( 'NONE',  ( 12.63038619288439968, 1428.207532477410041, 223.9332333053530135 ) ) ;
#87090=CARTESIAN_POINT ( 'NONE',  ( 33.92723937951050317, 1435.682267998569841, 135.5036483818229840 ) ) ;
#87091=CARTESIAN_POINT ( 'NONE',  ( 7.079892945961029582, 1396.160295697190122, 217.6030398920230198 ) ) ;
#87092=CARTESIAN_POINT ( 'NONE',  ( 10.31428324521939821, 1409.273243095039788, 197.3781550435539884 ) ) ;
#87093=CARTESIAN_POINT ( 'NONE',  ( -2.300955939006319895, 1405.879429239740148, 267.2329980173330455 ) ) ;
#87094=CARTESIAN_POINT ( 'NONE',  ( -14.58077760642500031, 1436.114534100510127, 149.8442496726960087 ) ) ;
#87096=CARTESIAN_POINT ( 'NONE',  ( -18.64588652299999794, 1416.828040475229955, 208.5593769277110141 ) ) ;
#87097=CARTESIAN_POINT ( 'NONE',  ( 14.25940458439999858, 1444.037519612920050, 189.5923944946979987 ) ) ;
#87099=ORIENTED_EDGE ( 'NONE', *, *, #46651, .F. ) ;
#87102=CIRCLE ( 'NONE', #13776, 2.000000000549930324 ) ;
#87109=CARTESIAN_POINT ( 'NONE',  ( 7.561651663499999287, 1415.425582719929707, 225.2205323159980139 ) ) ;
#87111=CARTESIAN_POINT ( 'NONE',  ( -28.09217120239999943, 1508.632189896530008, 207.7571593959380039 ) ) ;
#87112=CARTESIAN_POINT ( 'NONE',  ( -0.9134622989720000419, 1487.754272106330063, 231.1436532359980163 ) ) ;
#87116=CARTESIAN_POINT ( 'NONE',  ( -9.701291430620001321, 1409.251836952829990, 228.6783269308979811 ) ) ;
#87117=CARTESIAN_POINT ( 'NONE',  ( -4.118684918089999591, 1446.308391630630013, 183.7684684173979974 ) ) ;
#87125=CARTESIAN_POINT ( 'NONE',  ( -24.45522160929999700, 1435.370145036180020, 136.4741062850980029 ) ) ;
#87129=CARTESIAN_POINT ( 'NONE',  ( -5.728574053214379624, 1424.937532576071590, 226.9478413594984545 ) ) ;
#87131=CARTESIAN_POINT ( 'NONE',  ( -11.60004869885203682, 1423.973206102290760, 135.9381536961890617 ) ) ;
#87133=ORIENTED_EDGE ( 'NONE', *, *, #66087, .T. ) ;
#87134=CARTESIAN_POINT ( 'NONE',  ( -1.787767503901650068, 1451.934961237370089, 184.2182930155049974 ) ) ;
#87135=CARTESIAN_POINT ( 'NONE',  ( -8.381285897630000647, 1412.830257829430138, 230.5949227061979911 ) ) ;
#87139=ADVANCED_FACE ( 'NONE', ( #48058 ), #22818, .F. ) ;
#87141=CARTESIAN_POINT ( 'NONE',  ( 12.49310090042409982, 1434.470230054580043, 149.8104293411710159 ) ) ;
#87142=CARTESIAN_POINT ( 'NONE',  ( 6.375428557307381006, 1488.402514618529722, 234.5820377068529865 ) ) ;
#87144=CARTESIAN_POINT ( 'NONE',  ( -23.30096132306110235, 1508.459748541459930, 223.9027429165689682 ) ) ;
#87146=CARTESIAN_POINT ( 'NONE',  ( -1.724134400390000099, 1408.973268486529832, 187.2669157652979948 ) ) ;
#87150=CARTESIAN_POINT ( 'NONE',  ( 16.08564639389649997, 1496.414352768219942, 193.8777386732119794 ) ) ;
#87154=CARTESIAN_POINT ( 'NONE',  ( -12.21873817507669990, 1415.431750870129918, 196.1844242608510172 ) ) ;
#87156=VERTEX_POINT ( 'NONE', #9360 ) ;
#87157=CARTESIAN_POINT ( 'NONE',  ( 3.903606122229999809, 1420.588980623530006, 185.5382139491979956 ) ) ;
#87164=CARTESIAN_POINT ( 'NONE',  ( 17.64235773549999919, 1415.063410501330054, 210.6787325816779912 ) ) ;
#87167=CARTESIAN_POINT ( 'NONE',  ( -14.03269008360000036, 1434.988272402140183, 148.9022108617980109 ) ) ;
#87168=CARTESIAN_POINT ( 'NONE',  ( 33.93392607710000419, 1451.271780568129998, 135.9464999937979997 ) ) ;
#87170=FACE_OUTER_BOUND ( 'NONE', #34491, .T. ) ;
#87171=CARTESIAN_POINT ( 'NONE',  ( -19.04163037422885552, 1439.995762762720460, 209.8507536649994165 ) ) ;
#87172=CARTESIAN_POINT ( 'NONE',  ( 10.84538211560184351, 1425.248158932944079, 146.5362285467592756 ) ) ;
#87173=ORIENTED_EDGE ( 'NONE', *, *, #81452, .F. ) ;
#87174=CARTESIAN_POINT ( 'NONE',  ( 1.556610602838379931, 1415.059973079630026, 191.5211804267419780 ) ) ;
#87176=EDGE_CURVE ( 'NONE', #72398, #90951, #19444, .T. ) ;
#87178=CARTESIAN_POINT ( 'NONE',  ( -11.87550762067749943, 1433.043840718726415, 149.9802264065416750 ) ) ;
#87181=CARTESIAN_POINT ( 'NONE',  ( -20.59684415639999955, 1507.762623717429960, 190.9355247910979756 ) ) ;
#87185=CARTESIAN_POINT ( 'NONE',  ( 13.25967441340000086, 1414.983771848829747, 197.8194332372980000 ) ) ;
#87192=CARTESIAN_POINT ( 'NONE',  ( -17.89145751773400761, 1459.891188655622500, 228.0875397610878963 ) ) ;
#87194=CARTESIAN_POINT ( 'NONE',  ( 20.08991052607950323, 1509.197173136989932, 229.8362170949519907 ) ) ;
#87197=CARTESIAN_POINT ( 'NONE',  ( 17.13546961575789851, 1509.208612314439961, 231.8360975173889926 ) ) ;
#87199=CARTESIAN_POINT ( 'NONE',  ( 12.95646782890822024, 1442.923247039539092, 169.4280525748522450 ) ) ;
#87200=CARTESIAN_POINT ( 'NONE',  ( 20.46400528219999870, 1470.815019615230085, 209.0339138421799987 ) ) ;
#87201=CARTESIAN_POINT ( 'NONE',  ( -4.495633307820000005E-08, 1473.529235887330060, 262.4989462860979756 ) ) ;
#87205=CARTESIAN_POINT ( 'NONE',  ( 25.66085765329999901, 1508.559638121829948, 199.8979669743779937 ) ) ;
#87206=CARTESIAN_POINT ( 'NONE',  ( -20.74297378600000030, 1486.050832587129889, 191.3292126814980065 ) ) ;
#87208=CARTESIAN_POINT ( 'NONE',  ( 5.480463564019999900, 1422.526046715330040, 185.8321080085979986 ) ) ;
#87209=CARTESIAN_POINT ( 'NONE',  ( -11.39453227890000164, 1435.362097301539961, 151.5417150060980020 ) ) ;
#87211=CARTESIAN_POINT ( 'NONE',  ( 11.55343380559999922, 1436.871189967930150, 151.7006543630979820 ) ) ;
#87214=CARTESIAN_POINT ( 'NONE',  ( 1.151838181399999828, 1507.064426625830038, 237.0475204680980141 ) ) ;
#87219=CARTESIAN_POINT ( 'NONE',  ( -42.45911994060000438, 1445.498763873839835, 270.1977472527979671 ) ) ;
#87220=CARTESIAN_POINT ( 'NONE',  ( -23.70138498562419471, 1436.173432996585234, 212.0448533859750739 ) ) ;
#87221=CARTESIAN_POINT ( 'NONE',  ( 17.67654200049999957, 1410.026337379229972, 223.0785978711979851 ) ) ;
#87222=CARTESIAN_POINT ( 'NONE',  ( -14.72117515839999946, 1485.050094052629902, 224.1720311065980127 ) ) ;
#87224=CARTESIAN_POINT ( 'NONE',  ( 2.925928197532340125, 1410.286699746360227, 231.6216146004889822 ) ) ;
#87225=CARTESIAN_POINT ( 'NONE',  ( -1.270728274629999932, 1414.996444518330009, 226.4582995714980029 ) ) ;
#87226=CARTESIAN_POINT ( 'NONE',  ( -3.167625933140000072, 1417.589985715129842, 234.1420239621979817 ) ) ;
#87227=DIRECTION ( 'NONE',  ( 1.000000000000000000, 3.152985556228405519E-15, -4.340229276715479857E-15 ) ) ;
#87230=CARTESIAN_POINT ( 'NONE',  ( -43.73454037239169878, 1430.821798806799961, 266.2441235663050065 ) ) ;
#87231=CARTESIAN_POINT ( 'NONE',  ( -4.146782939769999565, 1426.018316117329960, 186.1121555218979893 ) ) ;
#87232=ORIENTED_EDGE ( 'NONE', *, *, #5421, .T. ) ;
#87236=FACE_OUTER_BOUND ( 'NONE', #108570, .T. ) ;
#87238=CARTESIAN_POINT ( 'NONE',  ( -20.86054011779999939, 1508.959477709830026, 190.3575368027980232 ) ) ;
#87239=CARTESIAN_POINT ( 'NONE',  ( -5.601667600379999890, 1410.392892709329772, 187.0683166722980104 ) ) ;
#87242=CARTESIAN_POINT ( 'NONE',  ( 20.57759936150000257, 1430.447427346229915, 213.0442855874480017 ) ) ;
#87246=DIRECTION ( 'NONE',  ( 3.331145804512843979E-08, 5.455889386854617429E-11, 0.9999999999999995559 ) ) ;
#87250=CARTESIAN_POINT ( 'NONE',  ( -28.33587269610449866, 1415.670569832889896, 270.2700704253879849 ) ) ;
#87252=CARTESIAN_POINT ( 'NONE',  ( 4.196431865958829555, 1416.112438447810064, 231.6845605219920117 ) ) ;
#87255=EDGE_LOOP ( 'NONE', ( #14640, #26790 ) ) ;
#87257=CARTESIAN_POINT ( 'NONE',  ( -22.67952439726359870, 1409.704860892969918, 209.4938531156840043 ) ) ;
#87258=CARTESIAN_POINT ( 'NONE',  ( -0.8807669020151700501, 1409.878743503689975, 185.2313411206270075 ) ) ;
#87262=CARTESIAN_POINT ( 'NONE',  ( -18.80861391721730058, 1416.321686226169959, 207.5736137325899904 ) ) ;
#87263=CARTESIAN_POINT ( 'NONE',  ( -17.84981256740000077, 1425.821171079729993, 226.1975678583979743 ) ) ;
#87264=CARTESIAN_POINT ( 'NONE',  ( 40.67628413852310132, 1456.517704155799947, 269.1116589114889734 ) ) ;
#87266=CARTESIAN_POINT ( 'NONE',  ( 5.515204341519999609, 1447.426897563979992, 184.7404326633980247 ) ) ;
#87270=CARTESIAN_POINT ( 'NONE',  ( 1.490044353047579984, 1471.418353334920084, 182.6703762986020081 ) ) ;
#87272=CARTESIAN_POINT ( 'NONE',  ( 23.47355847000000040, 1409.990881410429893, 208.6231098356030031 ) ) ;
#87274=CARTESIAN_POINT ( 'NONE',  ( -1.530900592538410043, 1457.980095062469900, 229.8454460011110143 ) ) ;
#87275=CARTESIAN_POINT ( 'NONE',  ( 25.68381050121670128, 1452.010962298709956, 135.3221168002480113 ) ) ;
#87279=CARTESIAN_POINT ( 'NONE',  ( 17.24303251159999917, 1409.680293628830213, 193.2722534259980307 ) ) ;
#87280=CARTESIAN_POINT ( 'NONE',  ( 18.57285056714469107, 1444.740067931810245, 161.9794701184630696 ) ) ;
#87281=FACE_OUTER_BOUND ( 'NONE', #78741, .T. ) ;
#87283=CARTESIAN_POINT ( 'NONE',  ( -21.14513965206749901, 1428.384847628398347, 220.1321864412567209 ) ) ;
#87285=CARTESIAN_POINT ( 'NONE',  ( 0.4493958440627169870, 1451.091564611090007, 182.2331086531640096 ) ) ;
#87291=CARTESIAN_POINT ( 'NONE',  ( -45.63712966311000230, 1440.913059426480004, 268.9747523979869470 ) ) ;
#87293=AXIS2_PLACEMENT_3D ( 'NONE', #67353, #67903, #101451 ) ;
#87294=CARTESIAN_POINT ( 'NONE',  ( -0.5107086395123420219, 1409.923861741519886, 233.1022952685189864 ) ) ;
#87299=ADVANCED_FACE ( 'NONE', ( #87170 ), #24969, .F. ) ;
#87300=CARTESIAN_POINT ( 'NONE',  ( -28.02005516190000023, 1440.913060387330006, 248.0989693021979861 ) ) ;
#87304=CARTESIAN_POINT ( 'NONE',  ( 26.42714720800000094, 1440.913060387330006, 243.9198229517980110 ) ) ;
#87308=CARTESIAN_POINT ( 'NONE',  ( 22.92822468965760407, 1507.593738162489899, 210.2569774338279842 ) ) ;
#87310=CARTESIAN_POINT ( 'NONE',  ( -5.846647695999999783, 1486.134888885630062, 182.3486960385980069 ) ) ;
#87312=CARTESIAN_POINT ( 'NONE',  ( -27.94862287022959890, 1509.902053760850094, 222.3787653423719917 ) ) ;
#87313=CARTESIAN_POINT ( 'NONE',  ( 25.57225985780000244, 1469.240968286530006, 213.7224825415979979 ) ) ;
#87316=CARTESIAN_POINT ( 'NONE',  ( -15.94609539910000073, 1509.299602945830202, 232.2985042022980053 ) ) ;
#87319=CARTESIAN_POINT ( 'NONE',  ( 20.99597493542299986, 1506.660869835769972, 226.0298841686729929 ) ) ;
#87320=CARTESIAN_POINT ( 'NONE',  ( 2.499940070885770194, 1420.000201147749976, 104.0331098325849979 ) ) ;
#87322=CARTESIAN_POINT ( 'NONE',  ( 0.1645172808354759819, 1483.564749894839906, 181.9412502021760076 ) ) ;
#87327=CARTESIAN_POINT ( 'NONE',  ( -20.59469742430000139, 1507.767255104930200, 190.2244918928979871 ) ) ;
#87331=EDGE_LOOP ( 'NONE', ( #32167, #82064, #6528, #91002 ) ) ;
#87333=CARTESIAN_POINT ( 'NONE',  ( -17.48265376240000180, 1415.426210663629945, 209.4361207452480187 ) ) ;
#87334=CARTESIAN_POINT ( 'NONE',  ( 11.50644271998659285, 1425.933145223276142, 139.0407033083927786 ) ) ;
#87338=CARTESIAN_POINT ( 'NONE',  ( 14.93195572412279937, 1409.434495771229876, 208.8832241306849937 ) ) ;
#87342=CARTESIAN_POINT ( 'NONE',  ( -17.09359705219999981, 1424.173446424729946, 191.3645022196980108 ) ) ;
#87344=EDGE_LOOP ( 'NONE', ( #45455, #58929, #56971 ) ) ;
#87349=ORIENTED_EDGE ( 'NONE', *, *, #85252, .T. ) ;
#87353=CARTESIAN_POINT ( 'NONE',  ( -11.73858749130000056, 1433.859640885310228, 151.0726002451980037 ) ) ;
#87354=CARTESIAN_POINT ( 'NONE',  ( 29.48235791214129620, 1509.960495255634896, 211.9272200838070717 ) ) ;
#87356=CARTESIAN_POINT ( 'NONE',  ( 1.244907802569999999, 1397.637435234229997, 222.1288968301979878 ) ) ;
#87359=CARTESIAN_POINT ( 'NONE',  ( -1.200783037039999890, 1471.157679959530014, 182.7924989298979881 ) ) ;
#87361=CARTESIAN_POINT ( 'NONE',  ( -18.34590456075780196, 1416.851343895820037, 208.8605686865189739 ) ) ;
#87362=CARTESIAN_POINT ( 'NONE',  ( 21.33070998324595280, 1509.431296620648936, 227.6602567490701574 ) ) ;
#87363=B_SPLINE_CURVE_WITH_KNOTS ( 'NONE', 5,
 ( #35896, #61127, #11252, #86836, #43739, #35330 ),
 .UNSPECIFIED., .F., .F.,
 ( 6, 6 ),
 ( 0.000000000000000000, 1.000000000000000000 ),
 .UNSPECIFIED. ) ;
#87367=CARTESIAN_POINT ( 'NONE',  ( -15.91482500274329936, 1418.747949750289990, 226.9705446459220184 ) ) ;
#87368=CARTESIAN_POINT ( 'NONE',  ( 19.90544086846439953, 1485.367507128069974, 226.9947249633279966 ) ) ;
#87371=ORIENTED_EDGE ( 'NONE', *, *, #80486, .F. ) ;
#87372=CARTESIAN_POINT ( 'NONE',  ( 12.84239221398829933, 1435.935692713660046, 150.8114773724069835 ) ) ;
#87373=ORIENTED_EDGE ( 'NONE', *, *, #68587, .T. ) ;
#87375=CARTESIAN_POINT ( 'NONE',  ( 43.15848742349999867, 1435.559015236269943, 263.9122469287980266 ) ) ;
#87376=CARTESIAN_POINT ( 'NONE',  ( -27.25446695549999987, 1488.690170598729765, 207.9119471468479787 ) ) ;
#87377=CARTESIAN_POINT ( 'NONE',  ( -11.03966253259999952, 1426.925357892029979, 93.54906076669780646 ) ) ;
#87378=CARTESIAN_POINT ( 'NONE',  ( 17.10041881072790204, 1410.877218605189910, 192.0891696896890153 ) ) ;
#87380=CARTESIAN_POINT ( 'NONE',  ( 2.811464099758409940, 1396.011238877079904, 198.4687896839119787 ) ) ;
#87381=CARTESIAN_POINT ( 'NONE',  ( -20.51078616439999891, 1453.154034703630032, 207.5895588249879893 ) ) ;
#87382=CARTESIAN_POINT ( 'NONE',  ( -29.79081509929999783, 1435.029579668969973, 240.1465591147980092 ) ) ;
#87384=CARTESIAN_POINT ( 'NONE',  ( 28.81018896693269582, 1509.453431478040102, 209.5184652127150002 ) ) ;
#87386=CARTESIAN_POINT ( 'NONE',  ( 32.75710557470000595, 1451.313526626729981, 135.9801501586979953 ) ) ;
#87388=CARTESIAN_POINT ( 'NONE',  ( 11.07094430326320023, 1396.299666280629935, 213.3550120317470089 ) ) ;
#87396=CARTESIAN_POINT ( 'NONE',  ( -17.27558692971449972, 1507.606285623229951, 224.2552697136770234 ) ) ;
#87398=CARTESIAN_POINT ( 'NONE',  ( 8.683531591982326603, 1446.645667073313916, 153.8370100282342037 ) ) ;
#87404=CARTESIAN_POINT ( 'NONE',  ( 14.95878199090000038, 1496.663429984430195, 225.9504587705980043 ) ) ;
#87409=CARTESIAN_POINT ( 'NONE',  ( 11.86409049007759897, 1432.195540099199889, 149.9805507428490046 ) ) ;
#87410=CARTESIAN_POINT ( 'NONE',  ( 12.89309554127431667, 1444.938028831528982, 186.7183914381823513 ) ) ;
#87412=CARTESIAN_POINT ( 'NONE',  ( -15.57930627156463288, 1506.606278688346947, 193.4080148037165827 ) ) ;
#87414=CARTESIAN_POINT ( 'NONE',  ( 10.98671988040000080, 1508.791612297629854, 234.6950353958980031 ) ) ;
#87416=CARTESIAN_POINT ( 'NONE',  ( -5.851186079629999703, 1425.133448028729845, 186.4975221530980036 ) ) ;
#87417=CARTESIAN_POINT ( 'NONE',  ( 3.081956807038389812, 1409.860509536320251, 270.0718037183509637 ) ) ;
#87418=CARTESIAN_POINT ( 'NONE',  ( -11.60004869885203682, 1428.983126981193436, 137.0999999980979851 ) ) ;
#87429=CARTESIAN_POINT ( 'NONE',  ( 6.092217268310000655, 1412.362567999629846, 265.6112251771979800 ) ) ;
#87431=CARTESIAN_POINT ( 'NONE',  ( 13.76344037756659944, 1434.978125283600093, 148.5738572365669938 ) ) ;
#87433=CARTESIAN_POINT ( 'NONE',  ( 40.04386419106696593, 1448.778254206540169, 134.9801842265818550 ) ) ;
#87440=CARTESIAN_POINT ( 'NONE',  ( -24.16388973340000135, 1443.918222318679909, 212.4831360045579913 ) ) ;
#87441=CARTESIAN_POINT ( 'NONE',  ( -2.016955699854175776, 1450.205627335352347, 154.3312174505059033 ) ) ;
#87445=CARTESIAN_POINT ( 'NONE',  ( 19.28837017967479994, 1509.586622668500013, 231.7115921283199782 ) ) ;
#87448=CARTESIAN_POINT ( 'NONE',  ( 11.99684948639972859, 1433.670360444001972, 149.8496142774944531 ) ) ;
#87449=CARTESIAN_POINT ( 'NONE',  ( 13.18956788129999858, 1412.740670877530192, 228.5450254855980177 ) ) ;
#87451=CARTESIAN_POINT ( 'NONE',  ( -15.74154664829999994, 1459.394320478729924, 230.7248325767979793 ) ) ;
#87454=CARTESIAN_POINT ( 'NONE',  ( 41.47797487389999560, 1425.138039607129713, 268.3622462469979837 ) ) ;
#87456=CARTESIAN_POINT ( 'NONE',  ( 13.80545266760000089, 1434.979654225609920, 148.5370281251980202 ) ) ;
#87457=CIRCLE ( 'NONE', #39148, 1.000002395376709652 ) ;
#87458=CARTESIAN_POINT ( 'NONE',  ( 20.44074684259999941, 1488.586588146029953, 191.1769514407980068 ) ) ;
#87460=CARTESIAN_POINT ( 'NONE',  ( -21.80812349030000163, 1430.398269787930076, 219.2188554248980097 ) ) ;
#87463=CARTESIAN_POINT ( 'NONE',  ( 0.03697543579222300342, 1507.626287098129751, 237.3745122006210124 ) ) ;
#87464=CARTESIAN_POINT ( 'NONE',  ( -16.30647051440000084, 1418.357332664029855, 226.9584847186979744 ) ) ;
#87466=CARTESIAN_POINT ( 'NONE',  ( -41.44601667217140317, 1442.603978534169983, 136.4469555575219886 ) ) ;
#87467=CARTESIAN_POINT ( 'NONE',  ( -13.04207679966010147, 1409.368499744919745, 225.9431846064669855 ) ) ;
#87469=CARTESIAN_POINT ( 'NONE',  ( -12.73158637370000079, 1442.742385989480226, 186.8996798116980074 ) ) ;
#87471=CARTESIAN_POINT ( 'NONE',  ( -27.78496691744659941, 1508.044397529670050, 210.4698789973389808 ) ) ;
#87472=CARTESIAN_POINT ( 'NONE',  ( -31.77787458389999387, 1435.606731000560103, 135.5694218124980068 ) ) ;
#87473=DIRECTION ( 'NONE',  ( 0.000000000000000000, 1.000000000000000000, 0.000000000000000000 ) ) ;
#87474=ORIENTED_EDGE ( 'NONE', *, *, #37831, .T. ) ;
#87475=DIRECTION ( 'NONE',  ( 0.000000000000000000, 0.000000000000000000, -1.000000000000000000 ) ) ;
#87476=CARTESIAN_POINT ( 'NONE',  ( -14.87542623989530099, 1409.432521718130147, 207.7979172480029888 ) ) ;
#87477=CARTESIAN_POINT ( 'NONE',  ( -5.494437299350000359, 1439.687232799670255, 154.7535679683980163 ) ) ;
#87480=CARTESIAN_POINT ( 'NONE',  ( -44.60802269250000052, 1451.081273266829839, 268.7932458390980059 ) ) ;
#87483=CARTESIAN_POINT ( 'NONE',  ( 0.1826205922680210203, 1420.410877725119917, 183.2589509447180092 ) ) ;
#87484=CARTESIAN_POINT ( 'NONE',  ( -26.88785758550000082, 1509.181462003529987, 214.1987029181680100 ) ) ;
#87487=CARTESIAN_POINT ( 'NONE',  ( 17.33264729495500234, 1424.042909391080002, 227.4554219137819757 ) ) ;
#87488=CARTESIAN_POINT ( 'NONE',  ( 14.46594802229999921, 1415.931784856029935, 219.5940544748980301 ) ) ;
#87489=CARTESIAN_POINT ( 'NONE',  ( 14.89315775630000083, 1485.046810827629997, 224.2543386747979923 ) ) ;
#87493=CARTESIAN_POINT ( 'NONE',  ( 4.433889532992436600, 1421.449000901995305, 137.6338609017415422 ) ) ;
#87494=CARTESIAN_POINT ( 'NONE',  ( 16.06428786779999740, 1414.913060387329779, 208.9262477901120008 ) ) ;
#87497=CARTESIAN_POINT ( 'NONE',  ( 23.87472870330000063, 1411.107469451229917, 210.5066206584180009 ) ) ;
#87500=CARTESIAN_POINT ( 'NONE',  ( -16.40900118989999967, 1421.678299158230175, 227.0581239876979964 ) ) ;
#87511=CARTESIAN_POINT ( 'NONE',  ( -14.13260639439999977, 1484.576036422829930, 186.6695759715979932 ) ) ;
#87514=CARTESIAN_POINT ( 'NONE',  ( 41.48258358977700055, 1444.135548109920137, 136.5500177229649807 ) ) ;
#87517=ORIENTED_EDGE ( 'NONE', *, *, #20118, .T. ) ;
#87518=CARTESIAN_POINT ( 'NONE',  ( 11.74950119094600076, 1433.770027978590178, 150.9361992396719927 ) ) ;
#87519=CARTESIAN_POINT ( 'NONE',  ( 0.07152473094740001425, 1397.597829882229917, 222.1216538301979995 ) ) ;
#87520=VERTEX_POINT ( 'NONE', #104393 ) ;
#87523=CARTESIAN_POINT ( 'NONE',  ( -15.73574044604409927, 1409.462552572229924, 225.2910003602459881 ) ) ;
#87524=CARTESIAN_POINT ( 'NONE',  ( 0.1999013110879999944, 1508.573951179030018, 180.3597275294980022 ) ) ;
#87525=CARTESIAN_POINT ( 'NONE',  ( -0.5392968480769999573, 1417.272289817929959, 235.8882545161980033 ) ) ;
#87527=CARTESIAN_POINT ( 'NONE',  ( 2.495004647950000098, 1488.172775063030031, 182.1516654459980202 ) ) ;
#87528=CARTESIAN_POINT ( 'NONE',  ( 9.687429786604399240, 1439.765094063396873, 153.1584582019008849 ) ) ;
#87530=FILL_AREA_STYLE_COLOUR ( '', #96873 ) ;
#87533=CARTESIAN_POINT ( 'NONE',  ( 38.19279632128629487, 1437.094169275030026, 134.0999999969999692 ) ) ;
#87535=CARTESIAN_POINT ( 'NONE',  ( -15.82483088085467138, 1509.465675743439988, 234.0825299431272128 ) ) ;
#87536=ORIENTED_EDGE ( 'NONE', *, *, #53583, .T. ) ;
#87537=CARTESIAN_POINT ( 'NONE',  ( 14.45648542637160006, 1435.815601845680021, 149.7795650820339972 ) ) ;
#87542=CARTESIAN_POINT ( 'NONE',  ( 12.66043128553913810, 1445.026948396785428, 169.4635460886795784 ) ) ;
#87547=VECTOR ( 'NONE', #20493, 1000.000000000000000 ) ;
#87550=CARTESIAN_POINT ( 'NONE',  ( 4.231248707956949850, 1446.302976782659925, 164.6656280576010261 ) ) ;
#87555=ORIENTED_EDGE ( 'NONE', *, *, #52259, .F. ) ;
#87556=CARTESIAN_POINT ( 'NONE',  ( 33.36397945909019569, 1440.913060387330006, 258.2907522413270271 ) ) ;
#87560=CARTESIAN_POINT ( 'NONE',  ( -14.78674196459999912, 1410.361681208129994, 190.6508623267980056 ) ) ;
#87565=CARTESIAN_POINT ( 'NONE',  ( 0.0002644827706587799215, 1396.374078736850834, 196.8444724510774222 ) ) ;
#87567=CARTESIAN_POINT ( 'NONE',  ( -12.91292777029999961, 1434.774376582520063, 149.2723726445979935 ) ) ;
#87569=CARTESIAN_POINT ( 'NONE',  ( 2.824784936839999983, 1465.895815560630126, 234.2053348773979735 ) ) ;
#87572=B_SPLINE_SURFACE_WITH_KNOTS ( 'NONE', 5, 5, ( 
 ( #62672, #20063, #21140, #87851, #29034, #63219 ),
 ( #12212, #53713, #80540, #3855, #37982, #72164 ),
 ( #106281, #55347, #29567, #11139, #96039, #85412 ),
 ( #77593, #43443, #85983, #70884, #9826, #8711 ),
 ( #62482, #61371, #87655, #42889, #52954, #26620 ),
 ( #60816, #104441, #78129, #18211, #354, #10373 ) ),
 .UNSPECIFIED., .F., .F., .F.,
 ( 6, 6 ),
 ( 6, 6 ),
 ( 8.878996031149998913, 11.86168502449999984 ),
 ( 0.000000000000000000, 1.459712257500000110 ),
 .UNSPECIFIED. ) ;
#87574=CARTESIAN_POINT ( 'NONE',  ( 11.43741207009999883, 1425.481177415629872, 144.1677667564979970 ) ) ;
#87578=CARTESIAN_POINT ( 'NONE',  ( -21.31156959599999823, 1488.809466529130077, 209.0743529571010129 ) ) ;
#87579=CARTESIAN_POINT ( 'NONE',  ( -17.25653015495222675, 1486.135578907454601, 187.8878648081120559 ) ) ;
#87584=CARTESIAN_POINT ( 'NONE',  ( 22.60664681420000122, 1452.395138154029837, 225.7920039562980037 ) ) ;
#87587=CARTESIAN_POINT ( 'NONE',  ( -7.840274410260001048, 1507.896958070730079, 235.4362243845980061 ) ) ;
#87588=CARTESIAN_POINT ( 'NONE',  ( -21.79827285660000058, 1452.321708545830006, 222.0267583476980064 ) ) ;
#87589=B_SPLINE_CURVE_WITH_KNOTS ( 'NONE', 3,
 ( #6473, #7021, #101063, #15405, #22135, #82636, #57996, #100525, #24359, #31665, #39527, #14857, #82063, #48496, #7572, #23804, #33310, #73702, #32227, #23257, #67504, #40623, #49047, #57456, #58545, #84278, #107828, #65846, #41179, #5927, #14306, #5368, #40073, #66407, #56335, #74794, #108384, #50149, #108938, #92130, #74253, #32769, #56887, #31116, #99408, #13743, #49594, #90467, #91583, #83726, #99965, #83184, #75353, #92671, #15948, #22688, #91017, #41726, #75886, #110036, #47927, #69724, #76997, #87039, #26570, #110583, #101608, #51231, #60766, #69157, #103843 ),
 .UNSPECIFIED., .F., .F.,
 ( 4, 2, 2, 2, 1, 1, 1, 1, 1, 2, 2, 2, 2, 2, 1, 1, 1, 1, 1, 1, 1, 2, 2, 2, 2, 2, 2, 2, 1, 1, 1, 1, 2, 2, 2, 2, 2, 1, 1, 1, 1, 1, 2, 2, 2, 4 ),
 ( 0.000000000000000000, 0.1250000000075510986, 0.1875000000113273835, 0.2187500000132166778, 0.2343750000141613110, 0.2421875000146322121, 0.2460937500148676349, 0.2480468750149853463, 0.2490234375150427171, 0.2495117187650713608, 0.2500000000151000323, 0.3750000000222334373, 0.4375000000258001953, 0.4687500000275862111, 0.4843750000284820501, 0.4921875000289330226, 0.4960937500291585645, 0.4980468750292713631, 0.4990234375293277069, 0.4995117187793529090, 0.4997558594043624014, 0.4998779297168672309, 0.5000000000293720603, 0.5312500000262170285, 0.5625000000230618857, 0.5937500000199068539, 0.6093750000183260074, 0.6171875000175328640, 0.6210937500171362924, 0.6230468750169378955, 0.6240234375168386416, 0.6245117187667917902, 0.6247558593917682535, 0.6250000000167448277, 0.6875000000123349109, 0.7187500000101351150, 0.7343750000090352170, 0.7421875000084852125, 0.7460937500082102103, 0.7480468750080800922, 0.7490234375080077056, 0.7495117187579714013, 0.7497558593829608542, 0.7500000000079501961, 0.8750000000039751535, 1.000000000000000000 ),
 .UNSPECIFIED. ) ;
#87590=CARTESIAN_POINT ( 'NONE',  ( 11.57799745920000056, 1432.441881432899891, 151.1964746161979747 ) ) ;
#87591=CARTESIAN_POINT ( 'NONE',  ( 17.97731455220759855, 1410.660655195440086, 222.9643864582139940 ) ) ;
#87594=EDGE_LOOP ( 'NONE', ( #95519, #7348, #91600, #47044 ) ) ;
#87596=CARTESIAN_POINT ( 'NONE',  ( 1.764049411440000048, 1406.288942863529883, 269.2935851124980218 ) ) ;
#87598=CARTESIAN_POINT ( 'NONE',  ( 44.70565502892719678, 1446.408339148580126, 269.9105772414620219 ) ) ;
#87599=CARTESIAN_POINT ( 'NONE',  ( 2.478937890449999681, 1432.468588061860146, 157.5195758061979916 ) ) ;
#87600=CARTESIAN_POINT ( 'NONE',  ( -27.28327444803209900, 1449.032218191109905, 136.7238657257040018 ) ) ;
#87601=CARTESIAN_POINT ( 'NONE',  ( -42.09825630726439272, 1440.913060411040078, 262.0793472720840214 ) ) ;
#87602=AXIS2_PLACEMENT_3D ( 'NONE', #90665, #13393, #73333 ) ;
#87603=CARTESIAN_POINT ( 'NONE',  ( -27.74152905169999883, 1446.393006942010061, 137.1637342961979869 ) ) ;
#87604=CARTESIAN_POINT ( 'NONE',  ( 2.017821789106273744, 1450.204743078944830, 154.3313547465386080 ) ) ;
#87606=CARTESIAN_POINT ( 'NONE',  ( 1.958645842704549889, 1450.346086676289815, 154.2463840790279903 ) ) ;
#87608=CARTESIAN_POINT ( 'NONE',  ( -1.546896723439913135, 1416.831923553206025, 228.0210884502933482 ) ) ;
#87609=ORIENTED_EDGE ( 'NONE', *, *, #49688, .F. ) ;
#87611=CARTESIAN_POINT ( 'NONE',  ( -3.946018174590000300E-15, 1427.166763959530044, 147.9649995502979891 ) ) ;
#87614=CARTESIAN_POINT ( 'NONE',  ( -0.2161462641430000053, 1476.049917889630024, 268.4837592950979683 ) ) ;
#87615=CARTESIAN_POINT ( 'NONE',  ( 10.73506988043325627, 1424.972993549859893, 139.1354236083641922 ) ) ;
#87617=CARTESIAN_POINT ( 'NONE',  ( -3.825775683770979985, 1448.295119309961819, 185.0228311757895483 ) ) ;
#87619=CIRCLE ( 'NONE', #51882, 2.000000000015774049 ) ;
#87620=CARTESIAN_POINT ( 'NONE',  ( -18.88752285780000051, 1416.568813549730066, 207.5747269755180184 ) ) ;
#87622=CARTESIAN_POINT ( 'NONE',  ( 26.38682956852759887, 1435.721715954939782, 136.2459471611129800 ) ) ;
#87623=CARTESIAN_POINT ( 'NONE',  ( -6.669055308816830063, 1396.145948930530039, 200.3212403031140241 ) ) ;
#87624=CARTESIAN_POINT ( 'NONE',  ( -15.51029599480000165, 1420.880494488829981, 227.0363825903980057 ) ) ;
#87625=CARTESIAN_POINT ( 'NONE',  ( -17.38485670972179875, 1410.884453452420075, 225.7833130266830040 ) ) ;
#87626=CARTESIAN_POINT ( 'NONE',  ( 22.09302970059145821, 1509.609508200493792, 226.9617867963430058 ) ) ;
#87627=ORIENTED_EDGE ( 'NONE', *, *, #93360, .T. ) ;
#87629=CARTESIAN_POINT ( 'NONE',  ( 2.370746254249999740, 1409.499373740729880, 231.5443631752980025 ) ) ;
#87631=CARTESIAN_POINT ( 'NONE',  ( 11.20602548229999940, 1425.617270592030081, 128.4886806428979753 ) ) ;
#87635=EDGE_CURVE ( 'NONE', #6139, #36366, #74219, .T. ) ;
#87639=CARTESIAN_POINT ( 'NONE',  ( -14.87168881317970026, 1430.147188212150240, 221.8136313441650032 ) ) ;
#87640=CARTESIAN_POINT ( 'NONE',  ( 8.991748181960000252, 1509.227061564030009, 181.2342630857980055 ) ) ;
#87642=CARTESIAN_POINT ( 'NONE',  ( 3.932775215530000423, 1448.980695957309990, 184.2693358957980081 ) ) ;
#87646=ORIENTED_EDGE ( 'NONE', *, *, #38173, .F. ) ;
#87647=CARTESIAN_POINT ( 'NONE',  ( -41.14739979139999804, 1443.970064379710038, 136.9302418245979709 ) ) ;
#87648=CARTESIAN_POINT ( 'NONE',  ( 0.8306043666373410517, 1482.868851409599984, 236.2037489664579937 ) ) ;
#87649=CARTESIAN_POINT ( 'NONE',  ( -20.19975713530000050, 1435.203085175508932, 142.9756137166980068 ) ) ;
#87651=CARTESIAN_POINT ( 'NONE',  ( -1.356522590142140050, 1410.335674017130032, 185.6037846924129724 ) ) ;
#87652=CIRCLE ( 'NONE', #52, 12.50000000000001066 ) ;
#87655=CARTESIAN_POINT ( 'NONE',  ( 22.04779549230000057, 1409.847308075230103, 206.6119095045879988 ) ) ;
#87656=CARTESIAN_POINT ( 'NONE',  ( -2.500000000000000000, 1448.261011210099923, 165.3792834674099765 ) ) ;
#87657=CARTESIAN_POINT ( 'NONE',  ( 8.407436659505169274, 1396.206654546769869, 216.2971811410959901 ) ) ;
#87658=CARTESIAN_POINT ( 'NONE',  ( 14.64909617470000214, 1409.247894962230021, 212.1421858282079711 ) ) ;
#87659=CARTESIAN_POINT ( 'NONE',  ( -2.295142876860809977, 1406.025848543300071, 266.9592563235519833 ) ) ;
#87660=CARTESIAN_POINT ( 'NONE',  ( 41.66043411209999903, 1443.874408430530139, 136.1362219313979836 ) ) ;
#87661=ORIENTED_EDGE ( 'NONE', *, *, #106208, .F. ) ;
#87663=CARTESIAN_POINT ( 'NONE',  ( 11.75889809420000098, 1441.171049811090143, 188.0932782936979777 ) ) ;
#87664=ORIENTED_EDGE ( 'NONE', *, *, #12306, .T. ) ;
#87678=CARTESIAN_POINT ( 'NONE',  ( 7.681065654920000263, 1415.931669658129977, 225.5629348723979888 ) ) ;
#87681=CARTESIAN_POINT ( 'NONE',  ( -28.26971619810000291, 1508.651289824929790, 208.8373429800469978 ) ) ;
#87683=B_SPLINE_SURFACE_WITH_KNOTS ( 'NONE', 3, 1, ( 
 ( #68916, #70572 ),
 ( #27985, #87915 ),
 ( #45367, #52100 ),
 ( #86230, #103017 ) ),
 .UNSPECIFIED., .F., .F., .F.,
 ( 4, 4 ),
 ( 2, 2 ),
 ( 0.000000000000000000, 1.000000000000000000 ),
 ( 0.000000000000000000, 1.000000000000000000 ),
 .UNSPECIFIED. ) ;
#87684=CARTESIAN_POINT ( 'NONE',  ( -41.32341301190928107, 1435.252038220275381, 269.6346703354698775 ) ) ;
#87686=CARTESIAN_POINT ( 'NONE',  ( -3.945491179890000311, 1409.050839975730014, 231.1832439529980263 ) ) ;
#87688=CARTESIAN_POINT ( 'NONE',  ( -10.44960420120000144, 1446.424728451650026, 186.6666287116979959 ) ) ;
#87694=CARTESIAN_POINT ( 'NONE',  ( -25.23898257620000152, 1435.663290897030038, 136.6833633521980005 ) ) ;
#87695=B_SPLINE_CURVE_WITH_KNOTS ( 'NONE', 3,
 ( #26172, #110191, #50316, #68227, #93930, #86643, #51956, #51392, #42435, #77704, #60358, #77162, #68773, #110744, #8819, #69323, #43004, #18322, #103429, #24513, #94480, #464, #58702, #17753, #16111, #76593, #86098, #26737, #9939, #101215, #33464, #44111, #16650, #84444 ),
 .UNSPECIFIED., .F., .F.,
 ( 4, 2, 2, 2, 2, 2, 2, 2, 2, 1, 1, 2, 2, 2, 1, 1, 2, 2, 4 ),
 ( 0.000000000000000000, 0.001953124999952264747, 0.003906249999904529493, 0.007812499999882994636, 0.01562499999985087623, 0.03124999999978504694, 0.06249999999966276976, 0.1249999999995043132, 0.2499999999992956745, 0.3749999999990870081, 0.4374999999989006572, 0.4687499999988947730, 0.4999999999988888888, 0.6249999999992073008, 0.6874999999993666178, 0.7187499999994462208, 0.7343749999994860778, 0.7499999999995258237, 1.000000000000000000 ),
 .UNSPECIFIED. ) ;
#87696=CONICAL_SURFACE ( 'NONE', #43011, 24.00000000000002132, 0.3430239404209998177 ) ;
#87703=ORIENTED_EDGE ( 'NONE', *, *, #31211, .F. ) ;
#87704=CARTESIAN_POINT ( 'NONE',  ( -1.803460047120530207, 1451.935679885149966, 184.2329819486090230 ) ) ;
#87705=CARTESIAN_POINT ( 'NONE',  ( -1.699922289799999930, 1417.915507289630114, 233.2101064502979852 ) ) ;
#87709=CARTESIAN_POINT ( 'NONE',  ( 25.25200551730000242, 1450.804230319249882, 137.6134878989979882 ) ) ;
#87710=B_SPLINE_CURVE_WITH_KNOTS ( 'NONE', 3,
 ( #94008, #85051, #25688, #67734 ),
 .UNSPECIFIED., .F., .F.,
 ( 4, 4 ),
 ( -17.00590611422270015, -6.621488669319999687 ),
 .UNSPECIFIED. ) ;
#87712=CARTESIAN_POINT ( 'NONE',  ( 2.779535121191639924, 1478.702761277170111, 234.6945779322839769 ) ) ;
#87713=EDGE_CURVE ( 'NONE', #96354, #33795, #110277, .T. ) ;
#87714=CARTESIAN_POINT ( 'NONE',  ( -24.04911046563629995, 1508.500148083520116, 222.3301988378860301 ) ) ;
#87715=CARTESIAN_POINT ( 'NONE',  ( -1.984520192970000263, 1409.916377354330052, 186.2507124829979830 ) ) ;
#87717=CARTESIAN_POINT ( 'NONE',  ( -0.5133565506310000526, 1410.311096912230141, 233.1717002627980264 ) ) ;
#87718=CARTESIAN_POINT ( 'NONE',  ( -0.005886490086299069752, 1420.444031316269729, 182.6735942328060105 ) ) ;
#87725=CARTESIAN_POINT ( 'NONE',  ( -12.60587301698909890, 1415.938742849230039, 196.3044052707020057 ) ) ;
#87727=ORIENTED_EDGE ( 'NONE', *, *, #77712, .F. ) ;
#87729=CARTESIAN_POINT ( 'NONE',  ( -2.713960167710639967E-10, 1417.262443616730025, 235.9145977375980010 ) ) ;
#87735=CARTESIAN_POINT ( 'NONE',  ( 17.97556616420000353, 1415.263254644529979, 210.1863902027079973 ) ) ;
#87736=CARTESIAN_POINT ( 'NONE',  ( -18.37606861500000122, 1424.967732719430160, 227.5064700491979863 ) ) ;
#87737=CARTESIAN_POINT ( 'NONE',  ( -22.92800964410000120, 1436.527409660840021, 141.8297638279979935 ) ) ;
#87738=CARTESIAN_POINT ( 'NONE',  ( -11.88140585900000090, 1433.447543843229823, 147.6490162021979984 ) ) ;
#87739=CARTESIAN_POINT ( 'NONE',  ( 15.76350792579999904, 1413.541987861329972, 191.4338706723980010 ) ) ;
#87742=CARTESIAN_POINT ( 'NONE',  ( 27.69925877688100258, 1441.434395746940027, 137.3015763641899980 ) ) ;
#87744=CARTESIAN_POINT ( 'NONE',  ( 1.556549595879139991, 1415.034069327939960, 191.5954303787009962 ) ) ;
#87745=CARTESIAN_POINT ( 'NONE',  ( 23.52041813219999966, 1430.461288272430238, 206.7123354197679816 ) ) ;
#87746=CARTESIAN_POINT ( 'NONE',  ( -23.77394755739999965, 1436.009596247230093, 211.4729698866979959 ) ) ;
#87748=CARTESIAN_POINT ( 'NONE',  ( -18.57349606690000243, 1508.241272120329995, 229.7340498379979863 ) ) ;
#87749=CARTESIAN_POINT ( 'NONE',  ( -2.976203730276889114, 1425.987994125993964, 185.4396839897474649 ) ) ;
#87750=CARTESIAN_POINT ( 'NONE',  ( 11.76054352614784548, 1435.168637047273251, 151.3007564940777741 ) ) ;
#87757=CARTESIAN_POINT ( 'NONE',  ( -15.83141035718888645, 1506.691119452811790, 224.6832273421007642 ) ) ;
#87758=CARTESIAN_POINT ( 'NONE',  ( -22.70290513515956832, 1409.705865905418023, 209.5810033907468721 ) ) ;
#87759=CARTESIAN_POINT ( 'NONE',  ( 24.02863965889999776, 1507.902931924930044, 195.9323066764980013 ) ) ;
#87761=CARTESIAN_POINT ( 'NONE',  ( -17.14943674877569890, 1460.897686246159992, 228.2718295297070199 ) ) ;
#87767=CARTESIAN_POINT ( 'NONE',  ( 17.57493253053520021, 1415.090956648730071, 210.1540952727430067 ) ) ;
#87769=CARTESIAN_POINT ( 'NONE',  ( 13.43245946205634667, 1443.480739768224339, 169.3649759703340294 ) ) ;
#87770=CARTESIAN_POINT ( 'NONE',  ( 19.63212482909999679, 1452.819910076630094, 208.7504658628519962 ) ) ;
#87771=CARTESIAN_POINT ( 'NONE',  ( -39.71667984470000334, 1443.385947343989756, 259.0958842110979958 ) ) ;
#87773=CARTESIAN_POINT ( 'NONE',  ( -11.23615794200000018, 1433.983026149579928, 151.5834757130979824 ) ) ;
#87776=CARTESIAN_POINT ( 'NONE',  ( -20.03090002299999739, 1485.143653381429885, 191.6176849518980134 ) ) ;
#87777=CARTESIAN_POINT ( 'NONE',  ( 13.55936921520000027, 1409.552479627430102, 191.5919583953979952 ) ) ;
#87779=CARTESIAN_POINT ( 'NONE',  ( 4.891644445989999923, 1423.483205933229783, 184.7436577964980131 ) ) ;
#87780=CARTESIAN_POINT ( 'NONE',  ( -11.36665844790000079, 1437.938651746620053, 152.0461524611979769 ) ) ;
#87781=CARTESIAN_POINT ( 'NONE',  ( 11.26681265989999936, 1433.831805099620169, 151.5577295601979984 ) ) ;
#87786=CARTESIAN_POINT ( 'NONE',  ( -2.382436964801009083, 1426.901689560119166, 137.0999999980979567 ) ) ;
#87788=CARTESIAN_POINT ( 'NONE',  ( -38.10549725089999384, 1456.559844724929917, 270.3402585752979803 ) ) ;
#87790=CARTESIAN_POINT ( 'NONE',  ( 17.22540035980000184, 1409.514584625130055, 222.3763175275979904 ) ) ;
#87792=EDGE_CURVE ( 'NONE', #94490, #35126, #16903, .T. ) ;
#87793=CARTESIAN_POINT ( 'NONE',  ( 8.407921469289998839, 1475.513060387329915, 189.8056153727980018 ) ) ;
#87794=CARTESIAN_POINT ( 'NONE',  ( 2.858803364451159901, 1409.202624393130009, 230.9089643516309991 ) ) ;
#87795=FACE_OUTER_BOUND ( 'NONE', #14458, .T. ) ;
#87796=CARTESIAN_POINT ( 'NONE',  ( -11.46248030930000006, 1419.039353461930205, 229.2066792439979963 ) ) ;
#87800=CARTESIAN_POINT ( 'NONE',  ( -44.72192564158709871, 1433.780113820020233, 266.2155848715870547 ) ) ;
#87801=CARTESIAN_POINT ( 'NONE',  ( -2.500000000000000000, 1425.954745500930130, 184.7023283137979774 ) ) ;
#87803=CARTESIAN_POINT ( 'NONE',  ( 23.71772659069999989, 1435.325744483010112, 137.0491500660980080 ) ) ;
#87808=CARTESIAN_POINT ( 'NONE',  ( -21.33070998720000233, 1509.431296620130070, 190.3921826451980053 ) ) ;
#87809=CARTESIAN_POINT ( 'NONE',  ( -2.610074113990000111, 1410.395240763830088, 186.5675311192979962 ) ) ;
#87811=EDGE_LOOP ( 'NONE', ( #53738, #36813, #68133, #62358 ) ) ;
#87812=CARTESIAN_POINT ( 'NONE',  ( 23.88021423819999711, 1436.089573992459918, 213.0827210816779882 ) ) ;
#87814=CARTESIAN_POINT ( 'NONE',  ( 12.87559654649999885, 1416.820969729830040, 196.3104025333980189 ) ) ;
#87816=CARTESIAN_POINT ( 'NONE',  ( 11.60004869885203505, 1425.456391939635751, 136.9368493822784671 ) ) ;
#87822=CARTESIAN_POINT ( 'NONE',  ( -22.51472004476610067, 1414.327503631689979, 270.0970517051659385 ) ) ;
#87824=CARTESIAN_POINT ( 'NONE',  ( 2.840174497108410634, 1416.937576063520055, 232.1670866114159821 ) ) ;
#87829=CARTESIAN_POINT ( 'NONE',  ( 45.62288738355533724, 1441.767032437498983, 268.9751391232022684 ) ) ;
#87833=CARTESIAN_POINT ( 'NONE',  ( -0.03032924301457349744, 1409.189327868429928, 185.6174390816690050 ) ) ;
#87836=CARTESIAN_POINT ( 'NONE',  ( -18.11774863200000141, 1420.839368349930055, 225.3824726533979970 ) ) ;
#87837=CARTESIAN_POINT ( 'NONE',  ( -0.0001178445682933130075, 1475.048122365760037, 269.6502183532239769 ) ) ;
#87838=CARTESIAN_POINT ( 'NONE',  ( -4.377444850077553795, 1466.548242231658151, 234.6382214351334028 ) ) ;
#87839=CARTESIAN_POINT ( 'NONE',  ( 5.684860708799999607, 1446.208771210280020, 183.7854341813980170 ) ) ;
#87841=VERTEX_POINT ( 'NONE', #10763 ) ;
#87842=CARTESIAN_POINT ( 'NONE',  ( 21.54081683246133849, 1411.025740448911392, 217.0790126318913451 ) ) ;
#87843=CARTESIAN_POINT ( 'NONE',  ( 1.516162725629030206, 1458.382341108720084, 183.2406470817350055 ) ) ;
#87844=VERTEX_POINT ( 'NONE', #18028 ) ;
#87846=CARTESIAN_POINT ( 'NONE',  ( 25.36371696672659937, 1452.027352620659940, 135.3832310289139969 ) ) ;
#87850=CARTESIAN_POINT ( 'NONE',  ( 18.26694772049999926, 1410.474778457329876, 193.9644247597979927 ) ) ;
#87851=CARTESIAN_POINT ( 'NONE',  ( 22.98253439269999987, 1410.218983183530099, 207.4712557340779995 ) ) ;
#87852=CARTESIAN_POINT ( 'NONE',  ( 16.19492570339999915, 1409.478599654730033, 224.8086529783979870 ) ) ;
#87853=CARTESIAN_POINT ( 'NONE',  ( -19.34609354041575813, 1425.420091874406125, 223.6468805313006669 ) ) ;
#87854=ADVANCED_FACE ( 'NONE', ( #28098 ), #31423, .T. ) ;
#87855=CARTESIAN_POINT ( 'NONE',  ( 0.6086926234157500337, 1452.967218034779989, 183.3063368812749729 ) ) ;
#87858=EDGE_CURVE ( 'NONE', #104164, #4923, #78751, .T. ) ;
#87860=EDGE_LOOP ( 'NONE', ( #1050, #66968, #71378, #75281 ) ) ;
#87861=CARTESIAN_POINT ( 'NONE',  ( -14.35518320136639936, 1509.483853104240097, 182.9676327163749932 ) ) ;
#87862=DIRECTION ( 'NONE',  ( 0.3363363969979655810, -0.9417419115949056119, 0.000000000000000000 ) ) ;
#87864=CARTESIAN_POINT ( 'NONE',  ( -9829.078716724869082, 2833.596074015789782, -1083.720023828399917 ) ) ;
#87866=CARTESIAN_POINT ( 'NONE',  ( -36.44972635297019536, 1449.829476660199816, 136.2612135086269802 ) ) ;
#87867=CARTESIAN_POINT ( 'NONE',  ( 0.1622545933607045798, 1506.474306115611853, 231.1380631582393903 ) ) ;
#87868=CARTESIAN_POINT ( 'NONE',  ( 4.884981308350000102E-15, 1454.846680951630105, 214.3676144195279676 ) ) ;
#87869=CARTESIAN_POINT ( 'NONE',  ( -2.391326140863789806, 1458.414063273499778, 184.3573557473769995 ) ) ;
#87870=CARTESIAN_POINT ( 'NONE',  ( 11.14340129720000050, 1433.162048341109994, 151.6428083595979786 ) ) ;
#87871=CARTESIAN_POINT ( 'NONE',  ( -4.227836598029999671, 1474.916636390029907, 269.6389068554980213 ) ) ;
#87872=CARTESIAN_POINT ( 'NONE',  ( 25.99288283567859636, 1440.913060397479967, 221.8287371291170018 ) ) ;
#87875=ORIENTED_EDGE ( 'NONE', *, *, #100138, .T. ) ;
#87876=CARTESIAN_POINT ( 'NONE',  ( 22.72903601766490311, 1507.336004462970095, 209.8256819690419945 ) ) ;
#87878=CARTESIAN_POINT ( 'NONE',  ( -5.823492620599999725, 1486.046966802129873, 182.4545651139980009 ) ) ;
#87882=CARTESIAN_POINT ( 'NONE',  ( 19.72588039849999930, 1469.237837315330125, 224.9730300090979824 ) ) ;
#87884=CARTESIAN_POINT ( 'NONE',  ( 2.557733547691819709, 1428.430169347510173, 224.8392532217209805 ) ) ;
#87887=CARTESIAN_POINT ( 'NONE',  ( 9.509570154840000455, 1407.604192000429975, 218.7432867935780223 ) ) ;
#87889=CARTESIAN_POINT ( 'NONE',  ( 0.1659333737283860133, 1482.725682766760201, 181.9772994460549853 ) ) ;
#87892=CARTESIAN_POINT ( 'NONE',  ( -16.68463233076019492, 1445.052233488289630, 162.0935120523188857 ) ) ;
#87894=CARTESIAN_POINT ( 'NONE',  ( 4.424121880270347695, 1432.332071595964408, 155.5695889658696274 ) ) ;
#87895=CARTESIAN_POINT ( 'NONE',  ( -38.37377460175660104, 1450.184294006830214, 134.0999999983419855 ) ) ;
#87896=ORIENTED_EDGE ( 'NONE', *, *, #39113, .T. ) ;
#87898=ORIENTED_EDGE ( 'NONE', *, *, #64602, .T. ) ;
#87902=DIRECTION ( 'NONE',  ( 0.000000000000000000, 0.000000000000000000, 1.000000000000000000 ) ) ;
#87904=ADVANCED_FACE ( 'NONE', ( #71808 ), #47664, .T. ) ;
#87907=CARTESIAN_POINT ( 'NONE',  ( 12.40624418351419855, 1409.346295973229871, 217.4486123556800408 ) ) ;
#87910=CARTESIAN_POINT ( 'NONE',  ( -17.71469135509999759, 1424.169313328530052, 191.8806465351980250 ) ) ;
#87911=FACE_OUTER_BOUND ( 'NONE', #47583, .T. ) ;
#87915=CARTESIAN_POINT ( 'NONE',  ( -1.581901184577762409, 1426.946688134061105, 134.0999999980979567 ) ) ;
#87917=VERTEX_POINT ( 'NONE', #3478 ) ;
#87918=CARTESIAN_POINT ( 'NONE',  ( 17.74362484289149933, 1457.960420730979877, 228.9108169342899828 ) ) ;
#87921=EDGE_CURVE ( 'NONE', #12979, #39452, #3413, .T. ) ;
#87922=CARTESIAN_POINT ( 'NONE',  ( 29.52154479088818562, 1509.964009467801588, 211.6628974038054594 ) ) ;
#87924=CARTESIAN_POINT ( 'NONE',  ( 2.495059952650000135, 1396.538088716130005, 221.4303740941980152 ) ) ;
#87927=CARTESIAN_POINT ( 'NONE',  ( -0.8705189345459999339, 1455.061689295130009, 183.2811947162979891 ) ) ;
#87929=CARTESIAN_POINT ( 'NONE',  ( -26.07931670434293281, 1436.684335497711118, 136.9216750084780756 ) ) ;
#87931=CARTESIAN_POINT ( 'NONE',  ( -13.11326399589999880, 1435.169422440890003, 150.1511621572980175 ) ) ;
#87932=CARTESIAN_POINT ( 'NONE',  ( 17.09517797430000030, 1409.510037156830094, 194.7435863138979926 ) ) ;
#87938=CARTESIAN_POINT ( 'NONE',  ( -22.23102603839999958, 1508.124938942629797, 193.6648602066980231 ) ) ;
#87939=CARTESIAN_POINT ( 'NONE',  ( -10.33698045908790064, 1425.426606213330160, 91.95338683678188829 ) ) ;
#87940=CARTESIAN_POINT ( 'NONE',  ( 5.451195050909999503E-14, 1410.389826760030019, 269.3346704430979912 ) ) ;
#87942=PLANE ( 'NONE',  #22998 ) ;
#87943=CARTESIAN_POINT ( 'NONE',  ( -33.33289073560000304, 1436.626756254900101, 248.0947902376980210 ) ) ;
#87944=CARTESIAN_POINT ( 'NONE',  ( 19.95713565929469979, 1509.643969355689933, 231.1087739065170013 ) ) ;
#87946=CARTESIAN_POINT ( 'NONE',  ( -13.40958089250450058, 1414.996442620860080, 220.3303868550709694 ) ) ;
#87947=CARTESIAN_POINT ( 'NONE',  ( -24.06079138099230263, 1410.858125179654508, 208.6187266795722621 ) ) ;
#87949=CARTESIAN_POINT ( 'NONE',  ( -2.500000000000000000, 1432.325347410999711, 157.4940207838979802 ) ) ;
#87953=VERTEX_POINT ( 'NONE', #97371 ) ;
#87955=CARTESIAN_POINT ( 'NONE',  ( -29.28608745770604216, 1509.936230668231474, 211.6463041379158199 ) ) ;
#87958=ORIENTED_EDGE ( 'NONE', *, *, #42808, .T. ) ;
#87960=CARTESIAN_POINT ( 'NONE',  ( 0.08511096936709999783, 1424.315873630530177, 227.5527473093980007 ) ) ;
#87962=DIRECTION ( 'NONE',  ( 0.9401064050714854625, -0.2476038110569656059, -0.2342910580744280991 ) ) ;
#87964=CARTESIAN_POINT ( 'NONE',  ( -3.374329543420000022, 1470.482678873730038, 235.0946326950979994 ) ) ;
#87965=CARTESIAN_POINT ( 'NONE',  ( 1.398466363930680023, 1420.912512660129778, 183.0157344917449791 ) ) ;
#87966=CARTESIAN_POINT ( 'NONE',  ( 45.85445519596599695, 1441.844569312759859, 268.7564833741089956 ) ) ;
#87968=CARTESIAN_POINT ( 'NONE',  ( 0.2192230774779999891, 1419.198292138529951, 184.6432371525980045 ) ) ;
#87973=CARTESIAN_POINT ( 'NONE',  ( 11.85573241129629984, 1431.613746796120040, 149.9352766684680205 ) ) ;
#87975=CARTESIAN_POINT ( 'NONE',  ( 13.13407055734306006, 1444.772519759580291, 187.1788395466846850 ) ) ;
#87979=CARTESIAN_POINT ( 'NONE',  ( 4.910254292329999437, 1507.788984001429981, 235.8016783594979700 ) ) ;
#87981=CARTESIAN_POINT ( 'NONE',  ( 16.18847201900799959, 1452.347746487550012, 146.9707830506359869 ) ) ;
#87982=CARTESIAN_POINT ( 'NONE',  ( 3.165485043389999920, 1408.317885794130007, 270.3910588707980196 ) ) ;
#87987=CARTESIAN_POINT ( 'NONE',  ( 0.02828745832028754098, 1410.214488029192353, 233.2162056590676684 ) ) ;
#87989=CARTESIAN_POINT ( 'NONE',  ( 15.02274787390000022, 1434.996842493880195, 196.2759273980980197 ) ) ;
#87991=CARTESIAN_POINT ( 'NONE',  ( 17.77755434120550149, 1416.443526435939930, 224.9696923782719864 ) ) ;
#87995=CARTESIAN_POINT ( 'NONE',  ( 25.65427092280000210, 1434.769004650220268, 243.9198229472980017 ) ) ;
#87997=CARTESIAN_POINT ( 'NONE',  ( 41.49255935287312269, 1443.690926113407841, 136.5669747823052376 ) ) ;
#87999=CARTESIAN_POINT ( 'NONE',  ( 41.65675406397859604, 1443.992462633329978, 135.6790809494980010 ) ) ;
#88008=CARTESIAN_POINT ( 'NONE',  ( -24.09814796439999895, 1444.255765020069930, 212.5772278521379803 ) ) ;
#88009=CARTESIAN_POINT ( 'NONE',  ( -1.426943104832486098, 1450.672165367667276, 154.2643989290685909 ) ) ;
#88012=CARTESIAN_POINT ( 'NONE',  ( 28.00492654830749828, 1509.968806677990187, 194.4672643161270003 ) ) ;
#88014=CARTESIAN_POINT ( 'NONE',  ( -13.53916864874639892, 1429.119333790580185, 222.2883575635510169 ) ) ;
#88015=CARTESIAN_POINT ( 'NONE',  ( 13.33339459179999942, 1417.421582639030021, 228.6994961110980000 ) ) ;
#88017=CARTESIAN_POINT ( 'NONE',  ( -16.78296769010000133, 1460.265262334630279, 228.3353431369980058 ) ) ;
#88019=CARTESIAN_POINT ( 'NONE',  ( 43.71400391259999907, 1430.030208370729952, 266.2448334172979685 ) ) ;
#88020=CARTESIAN_POINT ( 'NONE',  ( -17.58047195769999860, 1409.526983996129957, 222.6194513965980093 ) ) ;
#88021=CARTESIAN_POINT ( 'NONE',  ( 16.98962153889999627, 1435.906362427300110, 148.1094881728979828 ) ) ;
#88022=CARTESIAN_POINT ( 'NONE',  ( 22.63564133870000106, 1508.009850363030182, 193.1501364738980158 ) ) ;
#88023=CARTESIAN_POINT ( 'NONE',  ( 29.43773002077689682, 1509.946928101494450, 206.9696982396478688 ) ) ;
#88027=CARTESIAN_POINT ( 'NONE',  ( -40.99906703070779912, 1440.733582855520126, 136.2526507852639952 ) ) ;
#88028=CARTESIAN_POINT ( 'NONE',  ( -8.345511106849999194, 1409.144376880429945, 197.3321607578980093 ) ) ;
#88030=CARTESIAN_POINT ( 'NONE',  ( -12.01638140429999879, 1440.881463611970048, 187.8051733414979765 ) ) ;
#88032=CARTESIAN_POINT ( 'NONE',  ( -33.13365747560000329, 1435.654560788539811, 135.0902693358980287 ) ) ;
#88034=ORIENTED_EDGE ( 'NONE', *, *, #23088, .F. ) ;
#88036=CARTESIAN_POINT ( 'NONE',  ( -12.13069928485440130, 1409.336673740850074, 217.8481747060740190 ) ) ;
#88039=CARTESIAN_POINT ( 'NONE',  ( -3.804428602223190126, 1420.825805556418345, 137.2934056698748861 ) ) ;
#88040=CARTESIAN_POINT ( 'NONE',  ( -45.67177334430000712, 1440.913039353769818, 266.1885934045980093 ) ) ;
#88048=CARTESIAN_POINT ( 'NONE',  ( 13.88551022039999872, 1452.408285299329918, 223.3855399223979816 ) ) ;
#88049=CARTESIAN_POINT ( 'NONE',  ( 1.581901184577762853, 1426.946688134061105, 137.0999999980979851 ) ) ;
#88052=CARTESIAN_POINT ( 'NONE',  ( -23.95637140939999910, 1411.110463997629950, 208.0703336090279834 ) ) ;
#88053=CARTESIAN_POINT ( 'NONE',  ( 17.37509876899999739, 1416.823418193329871, 203.7862089741079785 ) ) ;
#88055=CARTESIAN_POINT ( 'NONE',  ( -11.95789827870000011, 1415.263254644529979, 195.6584547795980029 ) ) ;
#88057=CARTESIAN_POINT ( 'NONE',  ( 23.48803479300000063, 1409.897858449729938, 209.7858158176040035 ) ) ;
#88058=CARTESIAN_POINT ( 'NONE',  ( 11.43185072513739797, 1443.913060387330006, 147.9056598087979921 ) ) ;
#88060=CARTESIAN_POINT ( 'NONE',  ( -5.360200749763491146, 1422.242249887159915, 144.4955016248619870 ) ) ;
#88061=CARTESIAN_POINT ( 'NONE',  ( -11.86563472409999953, 1432.300011745260008, 149.9825370587979876 ) ) ;
#88066=CARTESIAN_POINT ( 'NONE',  ( -15.36549427709999982, 1420.352425059129928, 229.0210324418980008 ) ) ;
#88070=CARTESIAN_POINT ( 'NONE',  ( -15.44463253599880126, 1485.324514085619967, 187.2482728325680057 ) ) ;
#88077=CARTESIAN_POINT ( 'NONE',  ( 26.88905145119999673, 1508.006187447730099, 215.2211436898180068 ) ) ;
#88078=ORIENTED_EDGE ( 'NONE', *, *, #58323, .T. ) ;
#88080=CARTESIAN_POINT ( 'NONE',  ( 1.499137301480000017, 1414.988015881329829, 191.7262494052980060 ) ) ;
#88081=CARTESIAN_POINT ( 'NONE',  ( -15.69204124918606169, 1410.669730017232723, 226.7211433092322466 ) ) ;
#88082=CARTESIAN_POINT ( 'NONE',  ( 1.448681958479999921, 1507.129709326030024, 181.1126016739980003 ) ) ;
#88083=CARTESIAN_POINT ( 'NONE',  ( -2.713960167710639967E-10, 1417.262443616730025, 235.9145977375980010 ) ) ;
#88084=CARTESIAN_POINT ( 'NONE',  ( -24.06633326386470273, 1452.067469986559900, 136.8844249806119819 ) ) ;
#88086=CARTESIAN_POINT ( 'NONE',  ( 12.86744022639999940, 1409.362401301430054, 227.0135731152979872 ) ) ;
#88087=EDGE_CURVE ( 'NONE', #41783, #54360, #2242, .T. ) ;
#88089=CARTESIAN_POINT ( 'NONE',  ( 39.02661178044039758, 1437.758897875479761, 134.0999999974839909 ) ) ;
#88091=CARTESIAN_POINT ( 'NONE',  ( -8.991629940588330427, 1509.227055023859975, 237.0095830223739881 ) ) ;
#88096=ORIENTED_EDGE ( 'NONE', *, *, #41297, .T. ) ;
#88099=CARTESIAN_POINT ( 'NONE',  ( -0.3530891476770000037, 1467.116854362329832, 235.6078141479979990 ) ) ;
#88101=CARTESIAN_POINT ( 'NONE',  ( -2.903124885889999618, 1484.703481644929980, 183.2972796410979868 ) ) ;
#88105=CARTESIAN_POINT ( 'NONE',  ( 4.222485211202849698, 1446.229405227499910, 167.6248456503689681 ) ) ;
#88106=ADVANCED_FACE ( 'NONE', ( #80581 ), #107396, .F. ) ;
#88107=CARTESIAN_POINT ( 'NONE',  ( 0.3138303437369999727, 1507.644171354529817, 237.4220927994979888 ) ) ;
#88110=ORIENTED_EDGE ( 'NONE', *, *, #104508, .F. ) ;
#88111=CARTESIAN_POINT ( 'NONE',  ( 27.15528332431300029, 1440.913060387330006, 245.4436605369820086 ) ) ;
#88113=EDGE_LOOP ( 'NONE', ( #72291, #98989, #82295, #77114 ) ) ;
#88116=CARTESIAN_POINT ( 'NONE',  ( -15.00325987230000102, 1410.369181960630158, 190.7724269911979889 ) ) ;
#88118=CARTESIAN_POINT ( 'NONE',  ( -24.49730784189999966, 1441.139193927939914, 211.0002140101279906 ) ) ;
#88120=CARTESIAN_POINT ( 'NONE',  ( 22.52079200403399994, 1410.876293387520036, 206.2022394633299882 ) ) ;
#88121=CARTESIAN_POINT ( 'NONE',  ( -4.803664197750522748E-06, 1397.577875906359623, 196.1218455414115738 ) ) ;
#88122=CARTESIAN_POINT ( 'NONE',  ( -12.69533288745581068, 1434.600403889475274, 147.1709292336272483 ) ) ;
#88125=CARTESIAN_POINT ( 'NONE',  ( 9.935511340089998811, 1462.885007474029862, 233.7276471281980150 ) ) ;
#88132=CARTESIAN_POINT ( 'NONE',  ( -20.42904319129999635, 1470.816572149929925, 209.3526706922980054 ) ) ;
#88133=EDGE_CURVE ( 'NONE', #74812, #40553, #68695, .T. ) ;
#88136=VERTEX_POINT ( 'NONE', #33324 ) ;
#88138=CARTESIAN_POINT ( 'NONE',  ( -1.296432797589999879E-09, 1463.596605969329858, 232.0486588194980015 ) ) ;
#88141=CARTESIAN_POINT ( 'NONE',  ( 2.921722053920000395, 1414.540823234730169, 231.8164568075980014 ) ) ;
#88142=CARTESIAN_POINT ( 'NONE',  ( -18.76806136029999905, 1457.583373696730177, 227.2045900892980228 ) ) ;
#88143=CARTESIAN_POINT ( 'NONE',  ( 11.58007378539999976, 1432.582704238630186, 151.1961013072979938 ) ) ;
#88144=CARTESIAN_POINT ( 'NONE',  ( 5.379505748067900051, 1430.582098177589842, 154.4820892377710209 ) ) ;
#88149=CARTESIAN_POINT ( 'NONE',  ( 0.7720380218979999709, 1406.269671972929928, 269.2944987139979958 ) ) ;
#88151=CARTESIAN_POINT ( 'NONE',  ( 12.75661095148570112, 1470.549711631520040, 269.3476708060779856 ) ) ;
#88152=CARTESIAN_POINT ( 'NONE',  ( 2.478043214419999973, 1440.127217985849938, 157.7918389896980216 ) ) ;
#88153=CARTESIAN_POINT ( 'NONE',  ( 10.33594274554624803, 1423.067651820833134, 137.1941078872085882 ) ) ;
#88154=CARTESIAN_POINT ( 'NONE',  ( -38.15894704684880168, 1440.913060390959799, 256.5354463518759758 ) ) ;
#88155=CARTESIAN_POINT ( 'NONE',  ( 37.12869866823530174, 1449.463881992789993, 136.3003431950029949 ) ) ;
#88156=CARTESIAN_POINT ( 'NONE',  ( 1.425556924595323238, 1450.669415802774438, 154.2648944982862247 ) ) ;
#88157=CARTESIAN_POINT ( 'NONE',  ( 0.0001408309371566590163, 1408.913070111550269, 186.4658721391990071 ) ) ;
#88158=CARTESIAN_POINT ( 'NONE',  ( 0.8736373785452179463, 1450.882552294920060, 154.7893692902700025 ) ) ;
#88159=B_SPLINE_CURVE_WITH_KNOTS ( 'NONE', 3,
 ( #29185, #95835, #79062, #36481 ),
 .UNSPECIFIED., .F., .F.,
 ( 4, 4 ),
 ( 0.000000000000000000, 1.000000000000000000 ),
 .UNSPECIFIED. ) ;
#88163=CARTESIAN_POINT ( 'NONE',  ( -36.06124927020000115, 1436.776486029860052, 262.6648722463980334 ) ) ;
#88166=CARTESIAN_POINT ( 'NONE',  ( -0.5589532248799999881, 1476.047851565629799, 268.4836504708979987 ) ) ;
#88167=CARTESIAN_POINT ( 'NONE',  ( -4.291175242752039765, 1446.971469842819943, 154.7965863647420122 ) ) ;
#88169=CARTESIAN_POINT ( 'NONE',  ( -2.973630401571459636, 1448.268562863430816, 184.4328599109281299 ) ) ;
#88171=CARTESIAN_POINT ( 'NONE',  ( -2.500000000000000000, 1448.894380913990062, 169.3595559471979755 ) ) ;
#88172=CARTESIAN_POINT ( 'NONE',  ( 26.45092774933420188, 1436.256316748539803, 136.6768279046889916 ) ) ;
#88173=CARTESIAN_POINT ( 'NONE',  ( -4.353139012478820291, 1396.065075352050144, 219.2571886206609975 ) ) ;
#88174=CARTESIAN_POINT ( 'NONE',  ( -15.34713811569999997, 1421.556258866430198, 227.2905572623980106 ) ) ;
#88175=CARTESIAN_POINT ( 'NONE',  ( -16.65620699048979603, 1409.595037377370090, 225.3660632515070290 ) ) ;
#88176=FACE_OUTER_BOUND ( 'NONE', #7179, .T. ) ;
#88178=CARTESIAN_POINT ( 'NONE',  ( -20.86054011819999943, 1508.959477709930070, 190.3575368045979985 ) ) ;
#88179=CARTESIAN_POINT ( 'NONE',  ( 1.498833634909999990, 1408.965400811229983, 230.5914988299979882 ) ) ;
#88180=CARTESIAN_POINT ( 'NONE',  ( -12.71625625589999942, 1484.464918063330060, 185.9897890590980012 ) ) ;
#88181=CARTESIAN_POINT ( 'NONE',  ( 11.38204197729999834, 1426.011755914629930, 126.2834675746979940 ) ) ;
#88183=CARTESIAN_POINT ( 'NONE',  ( 11.60004869885203682, 1428.983126981193436, 134.0999999980966777 ) ) ;
#88184=CARTESIAN_POINT ( 'NONE',  ( -13.51610093808350577, 1445.063428794548372, 151.4871142704430156 ) ) ;
#88187=CARTESIAN_POINT ( 'NONE',  ( -7.320561577120000329, 1432.353341358199941, 149.5448088695980005 ) ) ;
#88188=CARTESIAN_POINT ( 'NONE',  ( 2.588559417869999546, 1508.984568548630023, 179.8910387445980064 ) ) ;
#88189=DIRECTION ( 'NONE',  ( -0.8926073982886787439, 0.000000000000000000, -0.4508348173337058951 ) ) ;
#88192=CARTESIAN_POINT ( 'NONE',  ( -13.14000761400309969, 1461.232465202761659, 232.8227669047252846 ) ) ;
#88193=ORIENTED_EDGE ( 'NONE', *, *, #12306, .F. ) ;
#88195=CARTESIAN_POINT ( 'NONE',  ( 0.3722769099684289928, 1457.826255237599980, 228.9731060096619899 ) ) ;
#88196=CARTESIAN_POINT ( 'NONE',  ( -13.51610093809999924, 1443.913060387330006, 169.3501091259980171 ) ) ;
#88197=CARTESIAN_POINT ( 'NONE',  ( -22.37341732390000004, 1435.279001492648831, 139.8076879873978839 ) ) ;
#88200=CARTESIAN_POINT ( 'NONE',  ( -1.318069841409999832, 1486.109660646130123, 181.8447665737980117 ) ) ;
#88203=CARTESIAN_POINT ( 'NONE',  ( -41.65674201940959875, 1443.992456074669917, 135.6790666823760034 ) ) ;
#88205=CARTESIAN_POINT ( 'NONE',  ( -2.500000000000000000, 1448.711455262680147, 157.7219972398099799 ) ) ;
#88208=CARTESIAN_POINT ( 'NONE',  ( 5.200164090505730256E-05, 1406.777850256470174, 269.6501335340969945 ) ) ;
#88209=CARTESIAN_POINT ( 'NONE',  ( 40.71480606090000265, 1443.734517994560065, 137.1148378138979922 ) ) ;
#88211=CARTESIAN_POINT ( 'NONE',  ( -11.57603212119999903, 1432.304338525750154, 151.1967213783980242 ) ) ;
#88212=CARTESIAN_POINT ( 'NONE',  ( 12.25335341949999979, 1440.953202899389908, 188.4028591661979704 ) ) ;
#88220=B_SPLINE_CURVE_WITH_KNOTS ( 'NONE', 3,
 ( #109856, #16311, #84089, #51607 ),
 .UNSPECIFIED., .F., .F.,
 ( 4, 4 ),
 ( -96.65569485166331276, -19.64510849129999315 ),
 .UNSPECIFIED. ) ;
#88225=CARTESIAN_POINT ( 'NONE',  ( 12.22918761389999887, 1416.219761280829971, 223.5054628756979866 ) ) ;
#88228=EDGE_CURVE ( 'NONE', #64952, #81429, #66297, .T. ) ;
#88229=CARTESIAN_POINT ( 'NONE',  ( -42.06231979437640689, 1440.913089571769888, 269.6487552725350270 ) ) ;
#88231=CARTESIAN_POINT ( 'NONE',  ( -11.34430840129999929, 1409.809597392229989, 228.6274365818979959 ) ) ;
#88232=CARTESIAN_POINT ( 'NONE',  ( -7.313096896839999417, 1447.188565721670102, 185.7316950759980045 ) ) ;
#88234=CARTESIAN_POINT ( 'NONE',  ( 2.446787376320000096, 1432.353341358199941, 150.2884730787980061 ) ) ;
#88235=CARTESIAN_POINT ( 'NONE',  ( -25.97046658602729963, 1440.913060480119839, 221.7145558740930085 ) ) ;
#88237=CARTESIAN_POINT ( 'NONE',  ( 16.76344481147369336, 1422.586955737515609, 227.0118626232063832 ) ) ;
#88238=CARTESIAN_POINT ( 'NONE',  ( 41.65086068609159753, 1427.189777683049897, 269.7492451942990215 ) ) ;
#88241=CARTESIAN_POINT ( 'NONE',  ( -25.78156655170059608, 1509.813372604039841, 223.1298223243570078 ) ) ;
#88243=CARTESIAN_POINT ( 'NONE',  ( 19.18685276606920453, 1410.944740066537406, 195.6341497936866176 ) ) ;
#88245=ORIENTED_EDGE ( 'NONE', *, *, #100687, .T. ) ;
#88247=CARTESIAN_POINT ( 'NONE',  ( -0.8146824607389999695, 1415.382299376130049, 233.3155241476979995 ) ) ;
#88252=CARTESIAN_POINT ( 'NONE',  ( 18.49907080295740158, 1478.712406274740033, 228.6789878470059989 ) ) ;
#88253=CARTESIAN_POINT ( 'NONE',  ( -24.68077630836099701, 1437.736159206269804, 210.5119845322900005 ) ) ;
#88255=CARTESIAN_POINT ( 'NONE',  ( -0.3485419179389999678, 1410.306756102429972, 233.2101795455980096 ) ) ;
#88256=CARTESIAN_POINT ( 'NONE',  ( 0.03428106877207290348, 1420.445078887740010, 182.6743165705210004 ) ) ;
#88261=ORIENTED_EDGE ( 'NONE', *, *, #39236, .F. ) ;
#88262=CARTESIAN_POINT ( 'NONE',  ( -11.46011354710740093, 1414.971717244360207, 196.6341504491270200 ) ) ;
#88263=CARTESIAN_POINT ( 'NONE',  ( -11.54918848589999847, 1490.513422156330080, 183.1734117734980316 ) ) ;
#88264=EDGE_LOOP ( 'NONE', ( #95391, #57550, #82656, #34640 ) ) ;
#88265=CARTESIAN_POINT ( 'NONE',  ( 0.2353198783969999985, 1506.810797463830113, 231.1250055480980166 ) ) ;
#88266=CARTESIAN_POINT ( 'NONE',  ( 10.58000746958911797, 1434.869963651638045, 152.0831908380279458 ) ) ;
#88270=CARTESIAN_POINT ( 'NONE',  ( 16.92416502119278121, 1422.029238661900536, 226.8824423085827391 ) ) ;
#88271=CARTESIAN_POINT ( 'NONE',  ( 22.37934203670000244, 1410.866856972729920, 205.0809305166880279 ) ) ;
#88272=CARTESIAN_POINT ( 'NONE',  ( 17.33645360970000127, 1414.996444518330009, 210.3925742363780103 ) ) ;
#88276=CARTESIAN_POINT ( 'NONE',  ( 16.60587746830000100, 1428.779800883930193, 190.9634344794979768 ) ) ;
#88277=CARTESIAN_POINT ( 'NONE',  ( -19.07391236770194354, 1440.581610101740807, 209.7732386265107039 ) ) ;
#88278=CARTESIAN_POINT ( 'NONE',  ( -0.2282227750583530057, 1457.883215173980034, 229.2261862118490114 ) ) ;
#88279=ORIENTED_EDGE ( 'NONE', *, *, #55126, .T. ) ;
#88280=CARTESIAN_POINT ( 'NONE',  ( 1.045121606856920016, 1507.562507626550087, 186.2156307130109951 ) ) ;
#88282=CARTESIAN_POINT ( 'NONE',  ( -11.90000809277082183, 1434.914618699171342, 147.6452175350320317 ) ) ;
#88284=DIRECTION ( 'NONE',  ( 0.000000000000000000, 1.000000000000000000, 0.000000000000000000 ) ) ;
#88285=CARTESIAN_POINT ( 'NONE',  ( -2.771042439397337631, 1425.976720272856255, 185.1763243323314043 ) ) ;
#88286=CARTESIAN_POINT ( 'NONE',  ( 12.54268436849999979, 1408.913060387329779, 221.6645303301980050 ) ) ;
#88287=CARTESIAN_POINT ( 'NONE',  ( 26.80766621430014496, 1435.433710258606880, 135.7240550330992903 ) ) ;
#88292=EDGE_CURVE ( 'NONE', #76159, #68958, #103781, .T. ) ;
#88294=CARTESIAN_POINT ( 'NONE',  ( -15.49546525088307192, 1506.491018773352152, 224.7822750072435838 ) ) ;
#88296=CARTESIAN_POINT ( 'NONE',  ( 20.76477904309999900, 1508.884216872730121, 189.8073430845979885 ) ) ;
#88297=ORIENTED_EDGE ( 'NONE', *, *, #18796, .F. ) ;
#88302=EDGE_LOOP ( 'NONE', ( #105528, #9056, #40320, #101537 ) ) ;
#88304=CARTESIAN_POINT ( 'NONE',  ( 27.17824031941000129, 1496.227206563929940, 207.6753971228399962 ) ) ;
#88305=CARTESIAN_POINT ( 'NONE',  ( 13.12077080189999911, 1508.676888898530024, 233.4678022570980147 ) ) ;
#88306=CARTESIAN_POINT ( 'NONE',  ( 13.48138647031106352, 1443.612224725923852, 169.3589832081940756 ) ) ;
#88307=CARTESIAN_POINT ( 'NONE',  ( 35.02402602625965500, 1424.077443822751775, 269.5318445452296032 ) ) ;
#88308=CARTESIAN_POINT ( 'NONE',  ( -24.26836172750000031, 1463.758689926529996, 255.0044385419980131 ) ) ;
#88312=CARTESIAN_POINT ( 'NONE',  ( 11.68583270360880100, 1426.729740719480105, 140.5078102237010000 ) ) ;
#88313=CARTESIAN_POINT ( 'NONE',  ( 6.165765019510000222, 1409.128373646630052, 187.8915199111979746 ) ) ;
#88315=CARTESIAN_POINT ( 'NONE',  ( -12.03552277399999859, 1436.199553089340043, 151.3007237992979981 ) ) ;
#88316=DIRECTION ( 'NONE',  ( 4.973799150213359420E-14, 0.8730714504308808577, -0.4875922912049759361 ) ) ;
#88320=ORIENTED_EDGE ( 'NONE', *, *, #105531, .F. ) ;
#88324=CARTESIAN_POINT ( 'NONE',  ( -10.53025827939999992, 1470.866850696130086, 269.8740970541979323 ) ) ;
#88327=( BOUNDED_CURVE ( )  B_SPLINE_CURVE ( 3, ( #81420, #45672, #20415, #3116 ),
 .UNSPECIFIED., .F., .T. ) 
 B_SPLINE_CURVE_WITH_KNOTS ( ( 4, 4 ),
 ( 1.530699404089715943, 1.539816210893797388 ),
 .UNSPECIFIED. ) 
 CURVE ( )  GEOMETRIC_REPRESENTATION_ITEM ( )  RATIONAL_B_SPLINE_CURVE ( ( 1.000000000000000000, 0.9999930736648015017, 0.9999930736648015017, 1.000000000000000000 ) ) 
 REPRESENTATION_ITEM ( '' )  );
#88328=CARTESIAN_POINT ( 'NONE',  ( 16.69108863619999994, 1409.495926044930002, 223.4055895545979809 ) ) ;
#88329=CARTESIAN_POINT ( 'NONE',  ( -15.28316321820000034, 1506.811133768429954, 224.9455926307979894 ) ) ;
#88331=CARTESIAN_POINT ( 'NONE',  ( 18.22873622136830107, 1457.634151734390116, 229.9687917111629929 ) ) ;
#88335=CARTESIAN_POINT ( 'NONE',  ( -45.32983761869079586, 1435.629079562749894, 268.7723279587979732 ) ) ;
#88336=ORIENTED_EDGE ( 'NONE', *, *, #101405, .F. ) ;
#88338=AXIS2_PLACEMENT_3D ( 'NONE', #71972, #79796, #88189 ) ;
#88339=VERTEX_POINT ( 'NONE', #28250 ) ;
#88341=DIRECTION ( 'NONE',  ( 0.7074300732568278294, 0.02470400251969403355, 0.7063514732138287400 ) ) ;
#88342=CARTESIAN_POINT ( 'NONE',  ( -20.59685312390000078, 1507.762914164829908, 190.3821647269979849 ) ) ;
#88346=B_SPLINE_SURFACE_WITH_KNOTS ( 'NONE', 5, 5, ( 
 ( #31850, #48117, #81685, #40252, #73872, #22318, #90091, #15028, #32946 ),
 ( #92303, #83906, #40804, #55968, #67136, #82256, #109131, #57082, #74434 ),
 ( #107450, #4991, #30746, #5557, #7212, #65481, #21767, #108560, #13375 ),
 ( #56520, #90647, #39706, #108000, #31297, #99590, #22873, #91206, #14488 ),
 ( #50340, #35162, #84465, #76073, #93408, #9416, #44135, #78269, #8296 ),
 ( #18344, #68252, #60385, #7752, #110214, #68798, #94506, #26197, #60951 ),
 ( #101234, #34612, #17780, #16673, #86668, #33487, #92857, #110769, #1583 ),
 ( #41917, #85001, #67689, #17222, #50871, #103456, #101797, #25087, #43578 ),
 ( #59291, #77727, #42458, #16133, #69346, #25643, #76617, #34059, #102359 ),
 ( #59834, #93957, #35718, #9964, #51418, #24534, #1040, #58722, #95078 ),
 ( #85549, #8845, #43028, #26762, #77186, #489, #102899, #52535, #51981 ),
 ( #86122, #36826, #29520, #19456, #63711, #12168, #27316, #106234, #80492 ),
 ( #28427, #53655, #69907, #97821, #97277, #105703, #21099, #12726, #71016 ),
 ( #3254, #78840, #63173, #2151, #55301, #89434, #20550, #88335, #54754 ),
 ( #79938, #37381, #70459, #27875, #46907, #11627, #18896, #10519, #105137 ),
 ( #87800, #62626, #96744, #53091, #88884, #54210, #81030, #95627, #11084 ),
 ( #71581, #4339, #3808, #72119, #61497, #104021, #44693, #37939, #46358 ),
 ( #87230, #28985, #36269, #104580, #45251, #20015, #79387, #45805, #2701 ),
 ( #62056, #96181, #66465, #74851, #83234, #5977, #49099, #58048, #4867 ),
 ( #47986, #82123, #40677, #73755, #39583, #56392, #82687, #39010, #108995 ),
 ( #40122, #5425, #100022, #22742, #21649, #56946, #92184, #23856, #72647 ),
 ( #98377, #55857, #98924, #32281, #107878, #74307, #91075, #14358, #31718 ),
 ( #15455, #49647, #108437, #83783, #31166, #13800, #64254, #48550, #47440 ),
 ( #100574, #65904, #23314, #57507, #90524, #91632, #14908, #73187, #107332 ),
 ( #6525, #89976, #13250, #65356, #38470, #99464, #106772, #30063, #81564 ),
 ( #64816, #30628, #22194, #60821, #903, #68660, #58596, #33921, #50732 ),
 ( #41779, #8163, #77597, #69208, #42894, #102760, #42332, #75934, #67005 ),
 ( #8715, #17090, #93811, #94368, #59158, #110636, #33364, #51851, #26056 ),
 ( #59698, #85988, #51282, #85416, #77052, #67557, #32818, #25508, #93278 ),
 ( #75406, #358, #94946, #41234, #9286, #35029, #34485, #109545, #26625 ),
 ( #60251, #76484, #17650, #16541, #24411, #101115, #92727, #101660, #103317 ),
 ( #43448, #102229, #18215, #24947, #52411, #7078, #16003, #110089, #84865 ),
 ( #50206, #84331, #68116, #7621, #63046, #45120, #63582, #62487, #88759 ),
 ( #36149, #28851, #97152, #53516, #46224, #70333, #80358, #20421, #43999 ),
 ( #54626, #3674, #79262, #104445, #86536, #37802, #3122, #11502, #71990 ),
 ( #87659, #87093, #19876, #95494, #79816, #97699, #12042, #106104, #78134 ),
 ( #27192, #29381, #105565, #105002, #69775, #54083, #45678, #20971, #61927 ),
 ( #96044, #2572, #19315, #18762, #9830, #36694, #1437, #35583, #103893 ),
 ( #61375, #52959, #10378, #70888, #10948, #28291, #44551, #96607, #88208 ) ),
 .UNSPECIFIED., .F., .F., .F.,
 ( 6, 3, 3, 3, 3, 3, 3, 3, 3, 3, 3, 3, 6 ),
 ( 6, 3, 6 ),
 ( 24.04728406787560147, 26.41731193910000286, 28.47858422270000034, 30.53985650629999782, 34.66240107340000520, 42.94082674090000040, 51.21925240840000271, 84.61883450350001112, 101.2490010300000023, 117.8791675569999882, 130.6181505580000248, 136.9876420589999952, 143.3571909864640190 ),
 ( -7.608642969747240396E-05, 1.000000000000000000, 2.000086805724440087 ),
 .UNSPECIFIED. ) ;
#88350=EDGE_CURVE ( 'NONE', #88970, #98935, #62442, .T. ) ;
#88354=ORIENTED_EDGE ( 'NONE', *, *, #28772, .T. ) ;
#88355=CARTESIAN_POINT ( 'NONE',  ( -8.402618400705980761, 1410.369408431269903, 270.0745577945219793 ) ) ;
#88357=CARTESIAN_POINT ( 'NONE',  ( 3.515433849202130201, 1416.356576007590093, 231.8113076371539876 ) ) ;
#88360=EDGE_LOOP ( 'NONE', ( #107420, #80784, #50467, #95007, #72002 ) ) ;
#88362=CARTESIAN_POINT ( 'NONE',  ( 45.58870143954486309, 1442.488502812692332, 268.9760731915026213 ) ) ;
#88364=CARTESIAN_POINT ( 'NONE',  ( 3.625818218658252157, 1424.595510787312151, 184.5955723309376992 ) ) ;
#88365=CARTESIAN_POINT ( 'NONE',  ( -24.04208912931621711, 1411.123052270208063, 266.7327788561432271 ) ) ;
#88367=CARTESIAN_POINT ( 'NONE',  ( -18.69712754293130175, 1416.051481372519902, 207.5721598449429735 ) ) ;
#88368=CARTESIAN_POINT ( 'NONE',  ( 2.500000047107329593, 1439.241554657300185, 157.7315143162209949 ) ) ;
#88369=CARTESIAN_POINT ( 'NONE',  ( -0.0001195472470990460034, 1475.319258240860108, 269.4988494337139855 ) ) ;
#88370=CARTESIAN_POINT ( 'NONE',  ( 12.71459596929999947, 1416.274718422629803, 222.8886675024980093 ) ) ;
#88371=CARTESIAN_POINT ( 'NONE',  ( 7.138945119869999800, 1447.187254549259933, 185.3421223705979912 ) ) ;
#88374=CARTESIAN_POINT ( 'NONE',  ( 21.31045967363568749, 1411.017795812226268, 217.5615436375129264 ) ) ;
#88375=CARTESIAN_POINT ( 'NONE',  ( 1.480860223639280049, 1477.429525514950001, 182.4079029408990209 ) ) ;
#88377=CARTESIAN_POINT ( 'NONE',  ( 18.22873622136830107, 1457.634151734390116, 229.9687917111629929 ) ) ;
#88378=CARTESIAN_POINT ( 'NONE',  ( 24.39998090177769896, 1451.998272387500037, 136.9252543644830098 ) ) ;
#88382=CARTESIAN_POINT ( 'NONE',  ( 18.53966907490000082, 1409.560479898229914, 196.5394618705980179 ) ) ;
#88383=CARTESIAN_POINT ( 'NONE',  ( 27.73483395940000307, 1444.994950788470987, 161.2078980334979690 ) ) ;
#88384=CARTESIAN_POINT ( 'NONE',  ( 17.58997750089999812, 1410.451595763729983, 225.2085130754979900 ) ) ;
#88385=CARTESIAN_POINT ( 'NONE',  ( -19.76302329002471936, 1426.035389032143939, 222.9111529220132866 ) ) ;
#88386=CARTESIAN_POINT ( 'NONE',  ( 21.64192060530918482, 1453.490330227820550, 220.9236656602734001 ) ) ;
#88392=ORIENTED_EDGE ( 'NONE', *, *, #103127, .T. ) ;
#88397=CARTESIAN_POINT ( 'NONE',  ( -39.96604417509509943, 1445.822677059940133, 136.8290734187280009 ) ) ;
#88399=CARTESIAN_POINT ( 'NONE',  ( 1.576516694969999887E-14, 1462.614442895030152, 248.0989693021979861 ) ) ;
#88402=CARTESIAN_POINT ( 'NONE',  ( -42.19478785709999613, 1454.283011521129993, 269.0694631118980169 ) ) ;
#88404=CARTESIAN_POINT ( 'NONE',  ( -22.67178350569999878, 1508.009769414930133, 225.0292584458980230 ) ) ;
#88405=CARTESIAN_POINT ( 'NONE',  ( 13.16561200850000013, 1429.090194843729932, 222.5186421963979910 ) ) ;
#88406=ORIENTED_EDGE ( 'NONE', *, *, #48788, .F. ) ;
#88413=CARTESIAN_POINT ( 'NONE',  ( 25.36027075109999984, 1449.801358167649823, 211.2972422996380146 ) ) ;
#88414=VECTOR ( 'NONE', #105563, 1000.000000000000114 ) ;
#88415=B_SPLINE_CURVE_WITH_KNOTS ( 'NONE', 3,
 ( #30913, #107076, #39873, #30362, #74041, #80785, #21934, #31462, #38217, #72399, #13000, #108171, #65642, #99204, #89725, #106530, #98116, #23048, #56127, #90262, #91382, #13545, #73493, #3553, #107629, #22483, #65092, #14101, #32017, #16833, #48849 ),
 .UNSPECIFIED., .F., .F.,
 ( 4, 2, 2, 1, 1, 1, 1, 2, 2, 2, 1, 1, 1, 1, 1, 2, 2, 2, 2, 4 ),
 ( 0.000000000000000000, 0.2500000000000182632, 0.3750000000000275335, 0.4375000000000320854, 0.4687500000000326406, 0.4843750000000336398, 0.4921875000000361933, 0.4960937500000365818, 0.5000000000000369704, 0.6250000000000401901, 0.6875000000000419664, 0.7187500000000440759, 0.7343750000000441869, 0.7421875000000438538, 0.7460937500000442979, 0.7480468750000439648, 0.7500000000000436318, 0.8125000000000325295, 0.8750000000000213163, 1.000000000000000000 ),
 .UNSPECIFIED. ) ;
#88422=CARTESIAN_POINT ( 'NONE',  ( -3.482404828285579956, 1485.996524617339901, 182.2044860649310181 ) ) ;
#88423=CARTESIAN_POINT ( 'NONE',  ( 2.994687979099999620, 1464.609795697029995, 236.6065847252980063 ) ) ;
#88427=CARTESIAN_POINT ( 'NONE',  ( -1.535065677160000197, 1450.609239756710167, 182.1703775756980122 ) ) ;
#88430=CARTESIAN_POINT ( 'NONE',  ( -17.13018491839999768, 1414.971993471370070, 208.1178512858780039 ) ) ;
#88433=EDGE_LOOP ( 'NONE', ( #59844, #18920, #54117, #62130, #4826, #23355, #66226, #26659, #7969, #38480, #97171, #26158, #49103, #14635, #10882, #5948 ) ) ;
#88437=CARTESIAN_POINT ( 'NONE',  ( -2.760778634279479782, 1409.009468901610035, 188.0459411385839985 ) ) ;
#88442=CARTESIAN_POINT ( 'NONE',  ( 14.91350687018140064, 1409.433851523019939, 209.9051533666169860 ) ) ;
#88446=CARTESIAN_POINT ( 'NONE',  ( -17.63801041889999865, 1411.923586951229936, 192.9996560761979936 ) ) ;
#88450=ORIENTED_EDGE ( 'NONE', *, *, #89984, .T. ) ;
#88451=ORIENTED_EDGE ( 'NONE', *, *, #93991, .T. ) ;
#88453=CARTESIAN_POINT ( 'NONE',  ( -11.94908641619550060, 1415.673583083980020, 194.9773138209209833 ) ) ;
#88456=CARTESIAN_POINT ( 'NONE',  ( 34.37943628549087549, 1458.453385912395106, 269.5229009448329407 ) ) ;
#88458=CARTESIAN_POINT ( 'NONE',  ( 3.502832715609999870, 1396.096283016630196, 220.3210214699980156 ) ) ;
#88460=EDGE_CURVE ( 'NONE', #41682, #98399, #94203, .T. ) ;
#88461=CARTESIAN_POINT ( 'NONE',  ( -0.1433134854889999976, 1453.573377095430260, 183.1846218448980039 ) ) ;
#88464=B_SPLINE_CURVE_WITH_KNOTS ( 'NONE', 3,
 ( #77330, #86820, #59439, #1183, #104174, #34210, #76769, #16821, #44284, #17377, #10112, #51576, #110364, #77875, #78428, #35878, #70062, #86264, #33642, #69500, #51022, #631, #68949, #104722, #62769, #46497, #105277, #20694, #87944, #47041, #54890, #36961, #28571, #54350, #71724, #70604, #105841 ),
 .UNSPECIFIED., .F., .F.,
 ( 4, 3, 3, 3, 3, 3, 3, 3, 3, 3, 3, 3, 4 ),
 ( 0.000000000000000000, 2.822161410921079749, 4.695069562297280008, 5.748948128523428736, 7.569543626606720643, 8.522194890855359972, 9.390139124690000116, 9.765848498500000474, 10.24736818868129973, 10.79639064002810045, 11.59603149051410043, 12.12355864179750142, 12.39567234100000093 ),
 .UNSPECIFIED. ) ;
#88468=B_SPLINE_SURFACE_WITH_KNOTS ( 'NONE', 5, 5, ( 
 ( #26425, #8517, #100915, #25861, #9085, #51649 ),
 ( #93079, #32637, #160, #77400, #17450, #94180 ),
 ( #66814, #16895, #60620, #67365, #34283, #7974 ),
 ( #85788, #34833, #60062, #69021, #24751, #94740 ),
 ( #58948, #42141, #76292, #110443, #33722, #67914 ),
 ( #102021, #25306, #59506, #93617, #87463, #98995 ) ),
 .UNSPECIFIED., .F., .F., .F.,
 ( 6, 6 ),
 ( 6, 6 ),
 ( 1.117146821299999981, 1.987971636789739982 ),
 ( 0.000000000000000000, 2.000000000000000000 ),
 .UNSPECIFIED. ) ;
#88469=CARTESIAN_POINT ( 'NONE',  ( 17.64995062490000066, 1409.529410244630071, 195.7212478390979982 ) ) ;
#88472=EDGE_CURVE ( 'NONE', #69919, #5765, #32233, .T. ) ;
#88473=DIRECTION ( 'NONE',  ( 0.9930361521007663450, 0.03467758656449191484, -0.1125906994869730476 ) ) ;
#88476=CARTESIAN_POINT ( 'NONE',  ( -25.53333737259999836, 1449.803091291330020, 207.7075060623679974 ) ) ;
#88477=CARTESIAN_POINT ( 'NONE',  ( -3.549608295209999653, 1507.276800932030028, 180.9704960860979952 ) ) ;
#88480=CARTESIAN_POINT ( 'NONE',  ( -31.18244400340000055, 1434.782053685539950, 244.2061907853979790 ) ) ;
#88483=DIRECTION ( 'NONE',  ( -0.7067700949440681724, -0.03085664260706927689, -0.7067700478230329875 ) ) ;
#88485=CARTESIAN_POINT ( 'NONE',  ( -5.381406753977029389, 1431.114362971160062, 154.5700877874419916 ) ) ;
#88489=ORIENTED_EDGE ( 'NONE', *, *, #103127, .F. ) ;
#88492=CARTESIAN_POINT ( 'NONE',  ( -24.06249508630390110, 1410.733114950599884, 208.7965224760120009 ) ) ;
#88493=ORIENTED_EDGE ( 'NONE', *, *, #43968, .F. ) ;
#88494=CARTESIAN_POINT ( 'NONE',  ( -0.04553580890769999556, 1421.815794421829878, 227.5038027964980074 ) ) ;
#88496=AXIS2_PLACEMENT_3D ( 'NONE', #147, #109881, #9611 ) ;
#88498=VECTOR ( 'NONE', #62433, 1000.000000000000000 ) ;
#88499=CARTESIAN_POINT ( 'NONE',  ( -16.41268168250000059, 1489.056318670530118, 229.5189257191980232 ) ) ;
#88504=CARTESIAN_POINT ( 'NONE',  ( -12.71641934408000019, 1415.429375168339902, 221.3762486804189962 ) ) ;
#88506=CARTESIAN_POINT ( 'NONE',  ( 14.18404988999999894, 1463.784527685830199, 224.5937116242980096 ) ) ;
#88507=VERTEX_POINT ( 'NONE', #70717 ) ;
#88510=CARTESIAN_POINT ( 'NONE',  ( 11.84405349179480105, 1430.816400222050106, 149.7709986801920081 ) ) ;
#88511=B_SPLINE_CURVE_WITH_KNOTS ( 'NONE', 5,
 ( #21871, #91316, #73977, #48230, #39816, #108107, #81799, #39254, #14598 ),
 .UNSPECIFIED., .F., .F.,
 ( 6, 3, 6 ),
 ( 0.000000000000000000, 0.4996938382793605915, 1.000000000000000000 ),
 .UNSPECIFIED. ) ;
#88512=CARTESIAN_POINT ( 'NONE',  ( 13.42720001465534629, 1444.358310982252533, 187.7973124303245811 ) ) ;
#88513=ORIENTED_EDGE ( 'NONE', *, *, #91348, .F. ) ;
#88514=EDGE_LOOP ( 'NONE', ( #57564, #92885, #46944, #1610 ) ) ;
#88515=CARTESIAN_POINT ( 'NONE',  ( -1.455133652010000000, 1471.168344426330123, 183.0463840045979964 ) ) ;
#88520=CARTESIAN_POINT ( 'NONE',  ( 0.4918853724044109921, 1407.650947704770033, 270.1377426703190281 ) ) ;
#88527=CARTESIAN_POINT ( 'NONE',  ( 13.58268853709999924, 1416.851343898729965, 196.3340833726979895 ) ) ;
#88530=CARTESIAN_POINT ( 'NONE',  ( 17.65466472533700326, 1412.463031515849934, 224.8541166168249958 ) ) ;
#88532=EDGE_LOOP ( 'NONE', ( #327, #2612, #17325, #75564 ) ) ;
#88533=CARTESIAN_POINT ( 'NONE',  ( 5.052203703969999182, 1416.825952163429974, 255.3819207742980097 ) ) ;
#88534=CARTESIAN_POINT ( 'NONE',  ( 18.65749896656096496, 1509.387464492215713, 187.4422726699444866 ) ) ;
#88541=ORIENTED_EDGE ( 'NONE', *, *, #42666, .T. ) ;
#88542=CARTESIAN_POINT ( 'NONE',  ( 17.35267692490000258, 1414.988015876730060, 210.4487656595580063 ) ) ;
#88544=CARTESIAN_POINT ( 'NONE',  ( -2.434657972054051100, 1449.456394606908361, 154.4645640298018918 ) ) ;
#88549=CARTESIAN_POINT ( 'NONE',  ( 17.06735424545500024, 1509.588153667619963, 233.8544743334759914 ) ) ;
#88551=CARTESIAN_POINT ( 'NONE',  ( -40.27308906366239682, 1443.612067134240078, 137.1163379626329970 ) ) ;
#88552=CARTESIAN_POINT ( 'NONE',  ( -11.73230603450000054, 1475.513060387329915, 226.3291547820980156 ) ) ;
#88553=CARTESIAN_POINT ( 'NONE',  ( 15.64385495210000165, 1412.747091720930030, 227.2162067996979999 ) ) ;
#88554=B_SPLINE_CURVE_WITH_KNOTS ( 'NONE', 5,
 ( #66642, #92909, #94011, #101284, #8343, #31902, #49829, #24579, #41422, #59341, #57689, #15082, #91804, #25138 ),
 .UNSPECIFIED., .F., .F.,
 ( 6, 2, 3, 3, 6 ),
 ( -60.28232112689999411, -50.75108181390000084, -43.93735686660000539, -43.22195389150000011, -41.21984250090000046 ),
 .UNSPECIFIED. ) ;
#88556=CARTESIAN_POINT ( 'NONE',  ( -16.96620414819999922, 1460.582764900229904, 228.2621087521980030 ) ) ;
#88558=CARTESIAN_POINT ( 'NONE',  ( 45.32382092809999818, 1434.935672970719907, 266.4295321061979962 ) ) ;
#88559=CARTESIAN_POINT ( 'NONE',  ( -18.35086141989999931, 1409.718682756730004, 223.0331779077980059 ) ) ;
#88560=CARTESIAN_POINT ( 'NONE',  ( 21.21222413589999789, 1436.051885491429857, 143.9410731133980050 ) ) ;
#88561=CARTESIAN_POINT ( 'NONE',  ( 19.17287356779999996, 1469.162364348330129, 190.7723560717980149 ) ) ;
#88562=CARTESIAN_POINT ( 'NONE',  ( 5.369163426388340099, 1427.167559700779975, 153.2169079524520043 ) ) ;
#88564=CARTESIAN_POINT ( 'NONE',  ( -16.85082183769999986, 1423.343525757829866, 227.0118847376980113 ) ) ;
#88567=CARTESIAN_POINT ( 'NONE',  ( -13.82235482710600039, 1408.877038801369963, 210.6069041857849697 ) ) ;
#88568=CARTESIAN_POINT ( 'NONE',  ( -15.44258166179999847, 1414.913060387329779, 203.7071583754979827 ) ) ;
#88569=CARTESIAN_POINT ( 'NONE',  ( -12.65658667800000003, 1442.791283154439952, 186.1190103994979950 ) ) ;
#88571=CARTESIAN_POINT ( 'NONE',  ( -27.93079119180610093, 1508.830486288999964, 210.6192819018250191 ) ) ;
#88572=CARTESIAN_POINT ( 'NONE',  ( 13.80595060949999997, 1434.979618316850065, 146.5972947611979862 ) ) ;
#88573=CARTESIAN_POINT ( 'NONE',  ( -33.91369292130000446, 1435.681789575369976, 135.0664759990980315 ) ) ;
#88574=CARTESIAN_POINT ( 'NONE',  ( -7.743156676465178911, 1456.414080484902570, 227.4372369063648591 ) ) ;
#88577=CARTESIAN_POINT ( 'NONE',  ( -1.565132884227080190, 1408.967716032030012, 224.0361922849110101 ) ) ;
#88579=ORIENTED_EDGE ( 'NONE', *, *, #26729, .F. ) ;
#88582=CARTESIAN_POINT ( 'NONE',  ( -17.22592475669953416, 1443.913060387330688, 162.9227486557969655 ) ) ;
#88583=CARTESIAN_POINT ( 'NONE',  ( -44.66932832909999718, 1451.100843914730149, 266.4486768909980015 ) ) ;
#88585=CARTESIAN_POINT ( 'NONE',  ( 0.4599152650301550072, 1418.782133919569787, 184.7029683564409765 ) ) ;
#88586=CARTESIAN_POINT ( 'NONE',  ( -27.48211786359999920, 1509.872757090430014, 218.9219095898779983 ) ) ;
#88591=CARTESIAN_POINT ( 'NONE',  ( 2.553512956640000223E-15, 1433.447556881219953, 155.4376913957980264 ) ) ;
#88595=VERTEX_POINT ( 'NONE', #27568 ) ;
#88596=CARTESIAN_POINT ( 'NONE',  ( -5.682125987650000098, 1507.354943063129895, 181.2351845632980201 ) ) ;
#88597=VECTOR ( 'NONE', #94474, 1000.000000000000114 ) ;
#88598=CARTESIAN_POINT ( 'NONE',  ( 5.371102036599521234, 1422.361277206714249, 138.9487451065114954 ) ) ;
#88600=CARTESIAN_POINT ( 'NONE',  ( -11.50684714910000039, 1415.041103189330215, 195.7533805636979878 ) ) ;
#88602=CARTESIAN_POINT ( 'NONE',  ( 22.18009780759999927, 1409.687606470130049, 211.3518347607079875 ) ) ;
#88603=B_SPLINE_SURFACE_WITH_KNOTS ( 'NONE', 5, 1, ( 
 ( #71127, #26313 ),
 ( #43689, #104486 ),
 ( #77093, #36187 ),
 ( #35619, #8200 ),
 ( #85454, #69251 ),
 ( #44594, #402 ) ),
 .UNSPECIFIED., .F., .F., .F.,
 ( 6, 6 ),
 ( 2, 2 ),
 ( 65.12638661990000344, 66.80157803080371082 ),
 ( 0.6126846217289999563, 3.463904735919999922 ),
 .UNSPECIFIED. ) ;
#88606=CARTESIAN_POINT ( 'NONE',  ( -3.567499890613730074, 1508.690874479150125, 180.4371998924179934 ) ) ;
#88607=CARTESIAN_POINT ( 'NONE',  ( -11.58215570839999842, 1432.723904499930086, 151.1956759123980021 ) ) ;
#88616=CARTESIAN_POINT ( 'NONE',  ( -20.74894096239999897, 1428.237764131229824, 223.0444765198980122 ) ) ;
#88617=CARTESIAN_POINT ( 'NONE',  ( -16.67123089062359753, 1485.152086820359955, 188.0413787914010015 ) ) ;
#88624=CARTESIAN_POINT ( 'NONE',  ( 27.67579904629999987, 1509.157128445930084, 213.4451930261979840 ) ) ;
#88628=CARTESIAN_POINT ( 'NONE',  ( 1.555730441589999957, 1414.913528139930122, 192.0047335902979739 ) ) ;
#88629=CARTESIAN_POINT ( 'NONE',  ( 0.7904366496569998901, 1426.935925255829943, 133.6118001900980232 ) ) ;
#88630=CARTESIAN_POINT ( 'NONE',  ( 23.03439503529999755, 1449.683642696550123, 219.5641606253980171 ) ) ;
#88631=CARTESIAN_POINT ( 'NONE',  ( 2.500000000000000000, 1417.575542695230070, 161.0097146487299824 ) ) ;
#88632=CARTESIAN_POINT ( 'NONE',  ( -23.99188238352159885, 1452.075290040919981, 136.8468086068940295 ) ) ;
#88634=CARTESIAN_POINT ( 'NONE',  ( 7.252569847259999314, 1409.670284998229818, 230.5441453657980162 ) ) ;
#88636=( NAMED_UNIT ( * ) PLANE_ANGLE_UNIT ( ) SI_UNIT ( $, .RADIAN. ) );
#88638=CARTESIAN_POINT ( 'NONE',  ( 40.76227011262719202, 1440.007145189029870, 134.0999999980880091 ) ) ;
#88641=EDGE_LOOP ( 'NONE', ( #14552, #62500, #77099, #40606 ) ) ;
#88648=CARTESIAN_POINT ( 'NONE',  ( 36.02435014169089555, 1445.276583512550133, 137.0631246346559919 ) ) ;
#88649=CARTESIAN_POINT ( 'NONE',  ( 15.09916686074197578, 1451.148571410817340, 149.6580463515937822 ) ) ;
#88652=CARTESIAN_POINT ( 'NONE',  ( -16.73703974548556417, 1449.615440745906653, 220.0451451102140368 ) ) ;
#88654=CARTESIAN_POINT ( 'NONE',  ( 4.262306684643539789, 1446.607359238689924, 159.1811806424360043 ) ) ;
#88656=CARTESIAN_POINT ( 'NONE',  ( 0.01130987586839999996, 1507.369121482229957, 237.3632175159979738 ) ) ;
#88659=ORIENTED_EDGE ( 'NONE', *, *, #16624, .T. ) ;
#88660=CARTESIAN_POINT ( 'NONE',  ( 27.83576393251260228, 1440.913060387330006, 247.1867187401149977 ) ) ;
#88661=CARTESIAN_POINT ( 'NONE',  ( -2.348318232329873353E-05, 1452.887054547371918, 152.8599681479486776 ) ) ;
#88664=CARTESIAN_POINT ( 'NONE',  ( -15.10863497539999933, 1409.942448651430141, 191.0446830422980042 ) ) ;
#88666=CARTESIAN_POINT ( 'NONE',  ( -24.90528981920000007, 1441.263847370060148, 210.4373564352579820 ) ) ;
#88668=CARTESIAN_POINT ( 'NONE',  ( 22.31280560966569837, 1410.332809971110009, 206.2360209584310269 ) ) ;
#88673=CARTESIAN_POINT ( 'NONE',  ( 6.162479943850000197, 1464.100498801029971, 234.9357781952980133 ) ) ;
#88678=CARTESIAN_POINT ( 'NONE',  ( 28.31864921020000025, 1509.156311056829963, 208.1546065555820064 ) ) ;
#88681=CARTESIAN_POINT ( 'NONE',  ( -19.73776679940000278, 1452.815214894829978, 209.0753000189979787 ) ) ;
#88684=ORIENTED_EDGE ( 'NONE', *, *, #46053, .T. ) ;
#88686=CARTESIAN_POINT ( 'NONE',  ( 30.53571888249999944, 1440.913060384770006, 240.1260121784980015 ) ) ;
#88687=CARTESIAN_POINT ( 'NONE',  ( -10.97019733509999995, 1432.400418277960171, 151.7699536590980074 ) ) ;
#88689=CARTESIAN_POINT ( 'NONE',  ( -1.423894748726279857, 1507.656498555010103, 237.2172253236890072 ) ) ;
#88690=B_SPLINE_CURVE_WITH_KNOTS ( 'NONE', 5,
 ( #65436, #58129, #23399, #58678, #74936, #14436, #99545, #7162, #57035 ),
 .UNSPECIFIED., .F., .F.,
 ( 6, 3, 6 ),
 ( 0.000000000000000000, 0.5000000000000000000, 1.000000000000000000 ),
 .UNSPECIFIED. ) ;
#88691=CARTESIAN_POINT ( 'NONE',  ( -22.89636893299999798, 1449.797811951130143, 219.2674029246980183 ) ) ;
#88692=CARTESIAN_POINT ( 'NONE',  ( 11.87490714379999979, 1433.006767503300125, 150.3951466330979940 ) ) ;
#88693=CARTESIAN_POINT ( 'NONE',  ( 19.46657980040000169, 1455.632578195829865, 226.1434856801980118 ) ) ;
#88694=CARTESIAN_POINT ( 'NONE',  ( -0.2353198522280000038, 1506.810797420529980, 187.1186863663980091 ) ) ;
#88696=EDGE_LOOP ( 'NONE', ( #85365, #87958, #59447, #84333, #41670, #64680, #73932, #12598, #108287, #22846, #106008, #9683, #3916, #97241, #50734, #43069, #59007, #92771, #22345, #59779, #63655 ) ) ;
#88698=CARTESIAN_POINT ( 'NONE',  ( 1.323291931630000029, 1406.278073745629854, 269.2941001024979641 ) ) ;
#88701=CARTESIAN_POINT ( 'NONE',  ( 31.66981299747059708, 1465.623440352080024, 270.1133457425380016 ) ) ;
#88702=CARTESIAN_POINT ( 'NONE',  ( -26.56014455169999877, 1451.985525993130068, 134.9308153408980218 ) ) ;
#88713=CARTESIAN_POINT ( 'NONE',  ( -6.850948847420000654, 1425.447270615729849, 224.8635561966979708 ) ) ;
#88715=CARTESIAN_POINT ( 'NONE',  ( -0.3382973561789999750, 1475.836249162829972, 266.9611136385980217 ) ) ;
#88716=CARTESIAN_POINT ( 'NONE',  ( -4.262501422047650479, 1446.609523482700070, 159.1513637479519900 ) ) ;
#88717=CARTESIAN_POINT ( 'NONE',  ( -28.26084321609999961, 1508.649017708029987, 209.6368911950440008 ) ) ;
#88721=CARTESIAN_POINT ( 'NONE',  ( -17.92792478850000037, 1415.296882282229944, 208.1699612212720183 ) ) ;
#88723=CARTESIAN_POINT ( 'NONE',  ( 26.79415489093269898, 1435.433178437559945, 135.2874578969010031 ) ) ;
#88724=CARTESIAN_POINT ( 'NONE',  ( -2.574213757757640053, 1396.002953912619887, 219.8362960026119879 ) ) ;
#88725=CARTESIAN_POINT ( 'NONE',  ( -14.90609184490000061, 1421.333676412129989, 227.2836066624979878 ) ) ;
#88726=CARTESIAN_POINT ( 'NONE',  ( 9.660544699540000835, 1432.353341358199941, 148.7316627034979888 ) ) ;
#88730=CARTESIAN_POINT ( 'NONE',  ( -4.338670661869993062, 1484.259043665225363, 183.5078876442977389 ) ) ;
#88731=CARTESIAN_POINT ( 'NONE',  ( 11.12283182329999853, 1426.473557707429791, 99.60385865669789496 ) ) ;
#88734=CARTESIAN_POINT ( 'NONE',  ( -13.51610093808349866, 1443.913060387330006, 151.4871142704430156 ) ) ;
#88738=CARTESIAN_POINT ( 'NONE',  ( 6.951567194469999933, 1508.626707931329747, 181.9880926591980312 ) ) ;
#88745=CARTESIAN_POINT ( 'NONE',  ( -14.66018946070000162, 1444.034773379980152, 188.9384452558980172 ) ) ;
#88746=CARTESIAN_POINT ( 'NONE',  ( 1.420260137469999906, 1466.712984991329904, 235.0376562393980180 ) ) ;
#88747=LINE ( 'NONE', #38324, #24303 ) ;
#88750=CARTESIAN_POINT ( 'NONE',  ( -1.364645589921620106, 1416.551493819629968, 185.3405191386750062 ) ) ;
#88752=CARTESIAN_POINT ( 'NONE',  ( 2.011589696679999761, 1429.772212105730205, 184.5964239730980125 ) ) ;
#88754=CARTESIAN_POINT ( 'NONE',  ( -41.38883695897280290, 1445.149448330730138, 136.3871248988700131 ) ) ;
#88756=CARTESIAN_POINT ( 'NONE',  ( -2.500000000000000000, 1448.435833742209979, 161.6007892298630111 ) ) ;
#88757=CARTESIAN_POINT ( 'NONE',  ( -12.84239665067440050, 1435.935719077439899, 150.8114796122480072 ) ) ;
#88758=CARTESIAN_POINT ( 'NONE',  ( -27.84617737330000153, 1442.188138044959942, 137.3853255075979973 ) ) ;
#88759=CARTESIAN_POINT ( 'NONE',  ( -6.024456086116980025, 1407.067997541940031, 269.6384956777279740 ) ) ;
#88760=CARTESIAN_POINT ( 'NONE',  ( 41.48601861270000057, 1444.048396303439858, 136.5661520294979709 ) ) ;
#88761=ORIENTED_EDGE ( 'NONE', *, *, #51557, .T. ) ;
#88762=CARTESIAN_POINT ( 'NONE',  ( 4.187049558480000044, 1423.917685550429951, 184.1424272131979762 ) ) ;
#88767=CARTESIAN_POINT ( 'NONE',  ( -13.61466181890000016, 1460.855063855429762, 231.3360755285980019 ) ) ;
#88772=CARTESIAN_POINT ( 'NONE',  ( 0.05087345101610000336, 1508.993291644029796, 179.2717210570979773 ) ) ;
#88775=CARTESIAN_POINT ( 'NONE',  ( 17.66282533229999885, 1415.426091369230107, 212.8695664232880063 ) ) ;
#88779=AXIS2_PLACEMENT_3D ( 'NONE', #66750, #67298, #99755 ) ;
#88780=CARTESIAN_POINT ( 'NONE',  ( -4.181137680949999158, 1409.562970863930104, 231.9380548681980088 ) ) ;
#88781=DIRECTION ( 'NONE',  ( 0.7067701472209363400, 0.03085807451170261353, 0.7067699330296433047 ) ) ;
#88783=CARTESIAN_POINT ( 'NONE',  ( -14.25058219265448045, 1435.219475802135548, 149.2644305274596945 ) ) ;
#88784=CARTESIAN_POINT ( 'NONE',  ( 1.742626220133139947, 1466.605724716640225, 234.7106070719929960 ) ) ;
#88787=CARTESIAN_POINT ( 'NONE',  ( 28.70938062880000174, 1416.088826313630079, 270.3384725155980277 ) ) ;
#88790=CARTESIAN_POINT ( 'NONE',  ( -1.543833121739990100, 1424.175334750540060, 228.3471663839470125 ) ) ;
#88792=CARTESIAN_POINT ( 'NONE',  ( 22.53878404599999641, 1411.058442739730026, 206.1986151668880041 ) ) ;
#88795=CARTESIAN_POINT ( 'NONE',  ( 4.343520079308760273, 1421.964317546590109, 183.8964818372369905 ) ) ;
#88796=DIRECTION ( 'NONE',  ( 0.9993908270190849930, -0.03489949670280780014, 8.033055426964939564E-16 ) ) ;
#88797=CARTESIAN_POINT ( 'NONE',  ( 8.141878239905574688, 1423.434623704914429, 137.0999999979602535 ) ) ;
#88798=ORIENTED_EDGE ( 'NONE', *, *, #83267, .F. ) ;
#88803=CARTESIAN_POINT ( 'NONE',  ( -0.08328763183689999461, 1408.915968883630057, 232.2275454037979898 ) ) ;
#88804=CARTESIAN_POINT ( 'NONE',  ( 0.1681674884180490159, 1420.473121907760060, 182.7464979049940155 ) ) ;
#88812=EDGE_LOOP ( 'NONE', ( #100577, #11650, #64295, #36700, #80063 ) ) ;
#88813=CARTESIAN_POINT ( 'NONE',  ( 11.60004869884835621, 1426.567385858177886, 135.1569352595896589 ) ) ;
#88818=CARTESIAN_POINT ( 'NONE',  ( 15.70386933114422590, 1421.083856898652130, 227.5869605700097509 ) ) ;
#88819=CARTESIAN_POINT ( 'NONE',  ( 5.950109296629999989, 1421.372702594429938, 186.2244564570979719 ) ) ;
#88820=CARTESIAN_POINT ( 'NONE',  ( -18.07122677940000344, 1424.826032087529939, 227.1937097634979921 ) ) ;
#88821=CARTESIAN_POINT ( 'NONE',  ( -15.42782019790000092, 1435.461599119239963, 148.9396145078979998 ) ) ;
#88823=CARTESIAN_POINT ( 'NONE',  ( 17.16923421059999910, 1410.829425249829910, 192.1173138142980008 ) ) ;
#88825=CARTESIAN_POINT ( 'NONE',  ( -17.29437801252285922, 1433.661299895118873, 216.7949840967941100 ) ) ;
#88835=CARTESIAN_POINT ( 'NONE',  ( -2.971820252585304800, 1425.987760232464780, 185.4345033297641692 ) ) ;
#88836=CARTESIAN_POINT ( 'NONE',  ( 11.40030748711895825, 1434.654611036206006, 151.4913564614089125 ) ) ;
#88838=CARTESIAN_POINT ( 'NONE',  ( -2.551544005433064477, 1507.143443351390488, 236.9472590348812275 ) ) ;
#88840=B_SPLINE_CURVE_WITH_KNOTS ( 'NONE', 3,
 ( #93934, #91332, #100286, #82927, #17200, #51396, #85529, #107031, #21886, #23005, #57208 ),
 .UNSPECIFIED., .F., .F.,
 ( 4, 2, 1, 1, 1, 2, 4 ),
 ( 0.000000000000000000, 0.03125000000040171338, 0.06250000000080342677, 0.1250000000016067148, 0.2500000000020394242, 0.5000000000017441604, 1.000000000000000000 ),
 .UNSPECIFIED. ) ;
#88846=CARTESIAN_POINT ( 'NONE',  ( 21.42336641369999839, 1508.384612396429930, 191.1046303810979907 ) ) ;
#88847=VERTEX_POINT ( 'NONE', #29765 ) ;
#88850=EDGE_CURVE ( 'NONE', #24399, #12743, #51371, .T. ) ;
#88855=CARTESIAN_POINT ( 'NONE',  ( 13.35954871928184318, 1443.329911868641602, 169.3723227893304113 ) ) ;
#88856=CARTESIAN_POINT ( 'NONE',  ( 30.16113214930838993, 1419.695379429048671, 269.4725258538827006 ) ) ;
#88857=CARTESIAN_POINT ( 'NONE',  ( -9.545816650640000844, 1464.920850551829744, 240.4008508568979892 ) ) ;
#88858=CARTESIAN_POINT ( 'NONE',  ( -19.82279908859999651, 1484.712476145529990, 190.4276546656979860 ) ) ;
#88859=CARTESIAN_POINT ( 'NONE',  ( -11.92780736370000128, 1433.439050768640072, 150.0136606030979749 ) ) ;
#88861=CARTESIAN_POINT ( 'NONE',  ( -19.42119839770000311, 1486.154863920830167, 189.7844104138979731 ) ) ;
#88864=CARTESIAN_POINT ( 'NONE',  ( 4.992020700599999472, 1423.657950984729951, 185.2360043649980241 ) ) ;
#88866=CARTESIAN_POINT ( 'NONE',  ( 8.251909802380000158, 1439.861449115349842, 153.7181668371979981 ) ) ;
#88867=LINE ( 'NONE', #37364, #25130 ) ;
#88868=CARTESIAN_POINT ( 'NONE',  ( -9.470856273389999913, 1451.339473522230037, 152.7638238112979820 ) ) ;
#88875=CARTESIAN_POINT ( 'NONE',  ( -10.97762738589999998, 1473.214251705830065, 270.1116084939980055 ) ) ;
#88878=CARTESIAN_POINT ( 'NONE',  ( -15.39218706910000023, 1506.810797462329901, 224.8468255945980161 ) ) ;
#88879=CARTESIAN_POINT ( 'NONE',  ( 0.3240298866389390020, 1450.984562072739891, 181.8401462983730141 ) ) ;
#88880=CARTESIAN_POINT ( 'NONE',  ( -13.51720310719999851, 1421.523852283830138, 229.8336178099980032 ) ) ;
#88884=CARTESIAN_POINT ( 'NONE',  ( -45.29232520150449659, 1433.625543105270026, 267.6243001420129985 ) ) ;
#88885=ORIENTED_EDGE ( 'NONE', *, *, #102328, .F. ) ;
#88890=CARTESIAN_POINT ( 'NONE',  ( -22.52609270419999987, 1509.699688878229836, 190.3921826525979952 ) ) ;
#88891=CARTESIAN_POINT ( 'NONE',  ( -15.23280641220000220, 1410.405619594230075, 190.9016463256980103 ) ) ;
#88892=CIRCLE ( 'NONE', #54940, 29.84605316883209625 ) ;
#88897=CARTESIAN_POINT ( 'NONE',  ( -3.206876023490000005, 1419.434649146130141, 184.2270935463979811 ) ) ;
#88899=ORIENTED_EDGE ( 'NONE', *, *, #8893, .T. ) ;
#88900=CARTESIAN_POINT ( 'NONE',  ( -26.02511763151360213, 1416.147910639220072, 270.1077897879640091 ) ) ;
#88901=CARTESIAN_POINT ( 'NONE',  ( -1.608351468689999786, 1426.598937817530214, 144.1938086916980239 ) ) ;
#88902=LINE ( 'NONE', #106256, #85831 ) ;
#88906=CARTESIAN_POINT ( 'NONE',  ( 45.42636855331534917, 1444.198313664763418, 268.9805725394130604 ) ) ;
#88911=CARTESIAN_POINT ( 'NONE',  ( -17.40764085468179800, 1414.996442620800053, 207.5654756526599840 ) ) ;
#88912=CARTESIAN_POINT ( 'NONE',  ( 2.689507531282340214, 1439.963205020849955, 157.5730311057610038 ) ) ;
#88913=CARTESIAN_POINT ( 'NONE',  ( 10.54362614759770089, 1474.753171831259806, 269.4739217683639936 ) ) ;
#88914=CARTESIAN_POINT ( 'NONE',  ( 11.46423597849999965, 1415.041103191730144, 222.5613496819979957 ) ) ;
#88915=CARTESIAN_POINT ( 'NONE',  ( -17.36636230016033267, 1422.631182428599232, 226.5763293091231390 ) ) ;
#88917=EDGE_LOOP ( 'NONE', ( #66893, #24803, #47928, #109985 ) ) ;
#88919=CARTESIAN_POINT ( 'NONE',  ( -23.61303499308581166, 1447.799747876519405, 215.1558229191804514 ) ) ;
#88921=CARTESIAN_POINT ( 'NONE',  ( 10.59300109150884239, 1455.143630007434922, 226.2791905348894090 ) ) ;
#88922=CARTESIAN_POINT ( 'NONE',  ( -28.17856943518795276, 1509.667335740066619, 211.1330165289786294 ) ) ;
#88925=CARTESIAN_POINT ( 'NONE',  ( 19.74363812609999869, 1410.524512607730230, 196.8232449923980028 ) ) ;
#88926=CARTESIAN_POINT ( 'NONE',  ( 28.46619500829999794, 1445.052233488290085, 168.7181723459979992 ) ) ;
#88927=CARTESIAN_POINT ( 'NONE',  ( 16.64312535719999886, 1409.659826693630066, 225.8601930648979987 ) ) ;
#88929=CARTESIAN_POINT ( 'NONE',  ( 20.85017764587675515, 1454.877224260557341, 222.3149521191053850 ) ) ;
#88936=FACE_OUTER_BOUND ( 'NONE', #37469, .T. ) ;
#88938=CARTESIAN_POINT ( 'NONE',  ( -37.45632682353310372, 1449.248250845319944, 136.3260026918899825 ) ) ;
#88939=CARTESIAN_POINT ( 'NONE',  ( 11.01785724859542626, 1425.018945203718204, 138.3717623160356709 ) ) ;
#88940=CARTESIAN_POINT ( 'NONE',  ( 2.182839453575158295, 1417.483061668222035, 233.3517557601115300 ) ) ;
#88941=CARTESIAN_POINT ( 'NONE',  ( 17.90144918474177160, 1423.842768551787003, 225.8231199409207477 ) ) ;
#88942=CARTESIAN_POINT ( 'NONE',  ( 11.68841187039999951, 1433.169245300249941, 150.9165344040980017 ) ) ;
#88943=CARTESIAN_POINT ( 'NONE',  ( -4.168267939633230057, 1474.036593221349904, 270.1339685919859903 ) ) ;
#88946=CARTESIAN_POINT ( 'NONE',  ( 1.420259601960000229, 1466.712985171129958, 235.0376566307980113 ) ) ;
#88947=ORIENTED_EDGE ( 'NONE', *, *, #48415, .T. ) ;
#88948=DIRECTION ( 'NONE',  ( 0.000000000000000000, -1.000000000000000000, 0.000000000000000000 ) ) ;
#88951=CARTESIAN_POINT ( 'NONE',  ( -19.41856793929088099, 1485.592250299008128, 189.9265828168643395 ) ) ;
#88953=CARTESIAN_POINT ( 'NONE',  ( -11.74015320060000001, 1428.979986575930070, 144.1938086916980239 ) ) ;
#88956=CARTESIAN_POINT ( 'NONE',  ( -10.95472753179999970, 1509.295607902330175, 236.2198715736980148 ) ) ;
#88959=CARTESIAN_POINT ( 'NONE',  ( 2.499944437997340341, 1419.584213655310123, 133.9247507763970191 ) ) ;
#88961=( BOUNDED_CURVE ( )  B_SPLINE_CURVE ( 3, ( #9612, #86879, #85772, #25293 ),
 .UNSPECIFIED., .F., .F. ) 
 B_SPLINE_CURVE_WITH_KNOTS ( ( 4, 4 ),
 ( 1.478867175770939957, 1.985375841758659998 ),
 .UNSPECIFIED. ) 
 CURVE ( )  GEOMETRIC_REPRESENTATION_ITEM ( )  RATIONAL_B_SPLINE_CURVE ( ( 1.000000000000000000, 0.9787347716977619072, 0.9787347716977619072, 1.000000000000000000 ) ) 
 REPRESENTATION_ITEM ( '' )  );
#88962=CARTESIAN_POINT ( 'NONE',  ( 1.458694644860000000, 1465.700659552730031, 235.2691402379979877 ) ) ;
#88964=ORIENTED_EDGE ( 'NONE', *, *, #48851, .T. ) ;
#88965=CARTESIAN_POINT ( 'NONE',  ( -1.129710524660000104, 1450.979185682630032, 182.6858286092979995 ) ) ;
#88968=ADVANCED_FACE ( 'NONE', ( #42034 ), #105586, .T. ) ;
#88970=VERTEX_POINT ( 'NONE', #34726 ) ;
#88972=ORIENTED_EDGE ( 'NONE', *, *, #72108, .T. ) ;
#88974=DIRECTION ( 'NONE',  ( 0.9993902469226793039, -0.03489947646363077138, -0.001077449947926189004 ) ) ;
#88975=CARTESIAN_POINT ( 'NONE',  ( 11.60004869885204570, 1426.273943615695998, 138.2686089212693332 ) ) ;
#88980=CARTESIAN_POINT ( 'NONE',  ( 14.77784225791719841, 1409.429114010250032, 211.2770915593420114 ) ) ;
#88983=CARTESIAN_POINT ( 'NONE',  ( -17.96086529829999989, 1440.788139876609876, 191.1125201911979730 ) ) ;
#88989=CARTESIAN_POINT ( 'NONE',  ( 18.24033452539389799, 1459.341357182790034, 227.8698260022179909 ) ) ;
#88991=CARTESIAN_POINT ( 'NONE',  ( 29.98468393967828050, 1462.259853740634071, 269.4706430128066472 ) ) ;
#88992=CARTESIAN_POINT ( 'NONE',  ( -20.59032573514600273, 1507.551486734899981, 190.3983201303999806 ) ) ;
#88993=CARTESIAN_POINT ( 'NONE',  ( 4.365782049980000856, 1396.065516855929900, 219.3093729220980208 ) ) ;
#88997=CARTESIAN_POINT ( 'NONE',  ( -26.59801442624275580, 1436.739763347805138, 136.7954695389641699 ) ) ;
#88998=CARTESIAN_POINT ( 'NONE',  ( -19.16007793760780231, 1428.477562982570134, 208.5540069974889832 ) ) ;
#88999=EDGE_CURVE ( 'NONE', #15749, #87844, #107429, .T. ) ;
#89004=CARTESIAN_POINT ( 'NONE',  ( 16.19087789078229989, 1409.478458302130093, 193.2334102746530107 ) ) ;
#89005=DIRECTION ( 'NONE',  ( 0.000000000000000000, 1.000000000000000000, 0.000000000000000000 ) ) ;
#89007=CARTESIAN_POINT ( 'NONE',  ( 41.58338113919019463, 1444.065857391419968, 136.1223126983269935 ) ) ;
#89009=CARTESIAN_POINT ( 'NONE',  ( 33.60183515439999979, 1440.913060392849957, 248.0844435622979915 ) ) ;
#89010=CARTESIAN_POINT ( 'NONE',  ( -25.81147510950000168, 1488.682669034729997, 202.5064507356880199 ) ) ;
#89011=CARTESIAN_POINT ( 'NONE',  ( -11.08316036037830088, 1426.485585298449905, 96.72966585604500267 ) ) ;
#89012=CARTESIAN_POINT ( 'NONE',  ( 13.35004134540000109, 1415.296882282229944, 197.1179729259980036 ) ) ;
#89013=CARTESIAN_POINT ( 'NONE',  ( -17.14220118670536763, 1410.074716354810107, 270.0732288711442948 ) ) ;
#89014=CARTESIAN_POINT ( 'NONE',  ( -6.248994202630000494, 1409.477339443830033, 259.9484415741980001 ) ) ;
#89016=CARTESIAN_POINT ( 'NONE',  ( 2.500574528909250027, 1448.942056006560051, 154.5733147652059927 ) ) ;
#89017=CARTESIAN_POINT ( 'NONE',  ( -23.71385545433166797, 1410.153949831662885, 208.7056953457179418 ) ) ;
#89018=ORIENTED_EDGE ( 'NONE', *, *, #96960, .F. ) ;
#89019=CARTESIAN_POINT ( 'NONE',  ( 3.657048081452280108, 1396.576469495309993, 196.6488135896609890 ) ) ;
#89021=B_SPLINE_CURVE_WITH_KNOTS ( 'NONE', 3,
 ( #87615, #106060, #29338, #70846 ),
 .UNSPECIFIED., .F., .F.,
 ( 4, 4 ),
 ( 0.000000000000000000, 0.3624990114314036171 ),
 .UNSPECIFIED. ) ;
#89029=CARTESIAN_POINT ( 'NONE',  ( -1.077779315100000135, 1415.654178936130165, 185.0928310270980148 ) ) ;
#89032=CARTESIAN_POINT ( 'NONE',  ( -0.3620056675250000189, 1489.066376473530227, 236.5422289001979834 ) ) ;
#89034=ORIENTED_EDGE ( 'NONE', *, *, #56189, .F. ) ;
#89035=EDGE_CURVE ( 'NONE', #92712, #43923, #109212, .T. ) ;
#89037=CARTESIAN_POINT ( 'NONE',  ( -12.13987205284939996, 1415.426207913209964, 221.7061766877399975 ) ) ;
#89038=CARTESIAN_POINT ( 'NONE',  ( 14.57546012949999970, 1474.756325762929919, 224.5278850946980072 ) ) ;
#89042=CARTESIAN_POINT ( 'NONE',  ( 11.85702737606739987, 1431.703556386109994, 149.9456834834640233 ) ) ;
#89044=CARTESIAN_POINT ( 'NONE',  ( 12.70925652983267895, 1445.012977275617231, 186.3879696001495176 ) ) ;
#89053=CARTESIAN_POINT ( 'NONE',  ( 26.27891900751420096, 1507.831017877699878, 209.0944339814940065 ) ) ;
#89058=CARTESIAN_POINT ( 'NONE',  ( 0.03679684590394945165, 1409.773880882323510, 233.0990921512198213 ) ) ;
#89067=CARTESIAN_POINT ( 'NONE',  ( 39.48812356990000438, 1431.587789823920048, 268.3665355202980436 ) ) ;
#89070=CARTESIAN_POINT ( 'NONE',  ( 35.95604727100876374, 1451.436200009825143, 134.6958367465652202 ) ) ;
#89072=CARTESIAN_POINT ( 'NONE',  ( 45.63713829939310074, 1440.913067348179993, 268.9747433721050243 ) ) ;
#89075=ORIENTED_EDGE ( 'NONE', *, *, #97262, .F. ) ;
#89076=CARTESIAN_POINT ( 'NONE',  ( 8.598096571001718758, 1427.995879741943554, 137.0999999980979567 ) ) ;
#89077=CARTESIAN_POINT ( 'NONE',  ( -2.511980889886960000, 1439.367824232180055, 157.7248736099130042 ) ) ;
#89083=CARTESIAN_POINT ( 'NONE',  ( 27.67618890949159649, 1509.957365838989972, 222.7461888534850232 ) ) ;
#89085=CARTESIAN_POINT ( 'NONE',  ( -8.805428988939999257, 1497.713060387329961, 229.3821491682979854 ) ) ;
#89091=CARTESIAN_POINT ( 'NONE',  ( 43.82551825799999534, 1429.987201715729952, 268.8187383044979697 ) ) ;
#89092=CARTESIAN_POINT ( 'NONE',  ( -18.29824102079999903, 1410.475830671229915, 224.2242554351979891 ) ) ;
#89093=CARTESIAN_POINT ( 'NONE',  ( 19.22696748599999950, 1435.168248072100141, 144.6563286545979850 ) ) ;
#89095=CARTESIAN_POINT ( 'NONE',  ( 20.12413710170000414, 1488.587669296430022, 190.7085797787979971 ) ) ;
#89096=CARTESIAN_POINT ( 'NONE',  ( 5.359753019955250330, 1422.468040155149993, 146.8791528727659852 ) ) ;
#89097=CARTESIAN_POINT ( 'NONE',  ( -4.970712357689999195, 1475.638404632529955, 266.9514863814980004 ) ) ;
#89099=CARTESIAN_POINT ( 'NONE',  ( -36.85982855397319469, 1436.428218451429984, 135.9089977690080104 ) ) ;
#89100=CARTESIAN_POINT ( 'NONE',  ( 0.2124338303341239964, 1455.982566712989865, 183.1254455901450058 ) ) ;
#89101=CARTESIAN_POINT ( 'NONE',  ( -11.97297630299070015, 1408.007688502349993, 215.8652761565809897 ) ) ;
#89102=CARTESIAN_POINT ( 'NONE',  ( 0.7950258152958181723, 1426.814114633998997, 137.0999999982234385 ) ) ;
#89105=CARTESIAN_POINT ( 'NONE',  ( 11.87582791709999874, 1433.006487889580058, 146.9202945366980089 ) ) ;
#89106=CARTESIAN_POINT ( 'NONE',  ( -36.51516363092789419, 1436.208852636029860, 134.0999999969979797 ) ) ;
#89107=CARTESIAN_POINT ( 'NONE',  ( 10.29822466560000116, 1441.809080340180117, 186.9379677964980146 ) ) ;
#89108=ORIENTED_EDGE ( 'NONE', *, *, #48120, .T. ) ;
#89109=CARTESIAN_POINT ( 'NONE',  ( -7.114141310732409629, 1427.484008838899626, 137.0999999980979567 ) ) ;
#89110=CARTESIAN_POINT ( 'NONE',  ( -7.000838161960609263, 1409.157535043050075, 222.3551060745959944 ) ) ;
#89112=CARTESIAN_POINT ( 'NONE',  ( -2.478156609180000025, 1439.614611698830231, 157.7689743226979999 ) ) ;
#89113=CARTESIAN_POINT ( 'NONE',  ( 14.65718418945929891, 1509.165728398129886, 233.2531174127820179 ) ) ;
#89114=CARTESIAN_POINT ( 'NONE',  ( -31.73415138219999676, 1466.561829745230170, 267.4236068477979984 ) ) ;
#89118=CARTESIAN_POINT ( 'NONE',  ( -25.59999408250000030, 1509.583809833630085, 220.6387430072979896 ) ) ;
#89124=CARTESIAN_POINT ( 'NONE',  ( -29.61157949331689920, 1509.955833110559979, 208.5825572949630100 ) ) ;
#89125=EDGE_CURVE ( 'NONE', #76827, #91492, #62730, .T. ) ;
#89129=DIRECTION ( 'NONE',  ( -1.000000000000000000, 0.000000000000000000, 0.000000000000000000 ) ) ;
#89131=CARTESIAN_POINT ( 'NONE',  ( 1.455000209906389896, 1507.073729425429974, 236.7651043255590082 ) ) ;
#89132=EDGE_CURVE ( 'NONE', #94873, #11858, #80737, .T. ) ;
#89136=CARTESIAN_POINT ( 'NONE',  ( 22.63852601520000007, 1409.703615135929795, 209.5818420717589845 ) ) ;
#89139=CARTESIAN_POINT ( 'NONE',  ( -5.362414201681900749, 1424.198757875690035, 150.5191954795400022 ) ) ;
#89140=CARTESIAN_POINT ( 'NONE',  ( -11.77874533540000002, 1433.007533761370041, 150.8097953740980017 ) ) ;
#89142=CARTESIAN_POINT ( 'NONE',  ( 25.68368308515399789, 1449.916366644430127, 208.3382958551559909 ) ) ;
#89149=CARTESIAN_POINT ( 'NONE',  ( 13.37450925738970042, 1507.663501308599962, 233.0614823370259785 ) ) ;
#89150=CARTESIAN_POINT ( 'NONE',  ( -18.71617348083620058, 1485.537080198780131, 189.3638635336550067 ) ) ;
#89154=ORIENTED_EDGE ( 'NONE', *, *, #49368, .T. ) ;
#89156=CARTESIAN_POINT ( 'NONE',  ( 29.17336346449999951, 1509.870405656429966, 210.3367036282079994 ) ) ;
#89157=ORIENTED_EDGE ( 'NONE', *, *, #32405, .F. ) ;
#89160=CARTESIAN_POINT ( 'NONE',  ( 1.496858517070000172, 1428.056401037730211, 101.8807690336980016 ) ) ;
#89161=CARTESIAN_POINT ( 'NONE',  ( 1.716050170100000161, 1509.007692890629869, 179.5167852785979790 ) ) ;
#89162=CARTESIAN_POINT ( 'NONE',  ( -0.1798688738929999642, 1417.261861208530263, 235.9169760632979944 ) ) ;
#89164=CARTESIAN_POINT ( 'NONE',  ( -24.10240618318239925, 1452.071386932320138, 136.4706332069859798 ) ) ;
#89166=CARTESIAN_POINT ( 'NONE',  ( 8.774939133739998454, 1409.219488014130093, 228.7704650873980086 ) ) ;
#89169=CARTESIAN_POINT ( 'NONE',  ( 41.50828902763819173, 1442.131284356850074, 134.0999999980909934 ) ) ;
#89171=ORIENTED_EDGE ( 'NONE', *, *, #32476, .T. ) ;
#89175=VERTEX_POINT ( 'NONE', #78393 ) ;
#89180=CARTESIAN_POINT ( 'NONE',  ( 8.173996330113771691, 1451.383476035822923, 152.8928977840655818 ) ) ;
#89182=CARTESIAN_POINT ( 'NONE',  ( -17.48410805928437384, 1448.286856264058997, 218.1600271269404629 ) ) ;
#89184=FACE_OUTER_BOUND ( 'NONE', #89264, .T. ) ;
#89187=CARTESIAN_POINT ( 'NONE',  ( 6.036596006619999955, 1415.425582719929707, 192.3914609787979941 ) ) ;
#89189=ORIENTED_EDGE ( 'NONE', *, *, #93360, .F. ) ;
#89191=ORIENTED_EDGE ( 'NONE', *, *, #64561, .F. ) ;
#89192=CARTESIAN_POINT ( 'NONE',  ( 25.26674768904949886, 1440.913060387330006, 239.9653784531180065 ) ) ;
#89194=ADVANCED_FACE ( 'NONE', ( #36384 ), #87683, .T. ) ;
#89195=EDGE_LOOP ( 'NONE', ( #48080, #35257, #10297, #11129 ) ) ;
#89196=CARTESIAN_POINT ( 'NONE',  ( -0.3328315121010000377, 1452.976685501030261, 183.2631392977980056 ) ) ;
#89197=CARTESIAN_POINT ( 'NONE',  ( -16.48988658240000049, 1410.421086167129943, 191.6528615609980193 ) ) ;
#89199=CARTESIAN_POINT ( 'NONE',  ( -24.90364451589999817, 1441.171407319239961, 210.4346984424180107 ) ) ;
#89203=CARTESIAN_POINT ( 'NONE',  ( 0.8854628104720000392, 1405.995467260429905, 266.9608410729979937 ) ) ;
#89205=CARTESIAN_POINT ( 'NONE',  ( 15.69844654775839921, 1410.486775117663228, 191.5641288874454631 ) ) ;
#89206=CARTESIAN_POINT ( 'NONE',  ( -11.60004869885203860, 1425.163648261535172, 137.9639116715027853 ) ) ;
#89207=CIRCLE ( 'NONE', #48040, 20.98341875040010507 ) ;
#89210=ADVANCED_FACE ( 'NONE', ( #2811 ), #88603, .F. ) ;
#89211=CARTESIAN_POINT ( 'NONE',  ( 7.105427357599999217E-15, 1425.413060387329779, 188.2701767054980166 ) ) ;
#89213=VECTOR ( 'NONE', #58237, 1000.000000000000000 ) ;
#89216=CARTESIAN_POINT ( 'NONE',  ( -22.09833645820000214, 1506.806593688730118, 209.0739427216549871 ) ) ;
#89220=CARTESIAN_POINT ( 'NONE',  ( -0.5679639878839999323, 1416.568813547830132, 227.7576290933980090 ) ) ;
#89221=CARTESIAN_POINT ( 'NONE',  ( 29.87497052560000199, 1440.913060386509869, 238.0574391280980251 ) ) ;
#89224=CARTESIAN_POINT ( 'NONE',  ( 1.980002924110000118, 1414.522533370030033, 232.1992291241980126 ) ) ;
#89226=CARTESIAN_POINT ( 'NONE',  ( -24.11883138550000183, 1457.436797524329904, 215.1402808420379813 ) ) ;
#89228=CARTESIAN_POINT ( 'NONE',  ( -2.845522529430000169, 1486.018762278030181, 182.0897997094980099 ) ) ;
#89230=CIRCLE ( 'NONE', #98173, 30.00000000000000000 ) ;
#89233=CARTESIAN_POINT ( 'NONE',  ( 2.112228378390000216, 1405.752148843630039, 267.8521524492979893 ) ) ;
#89236=CARTESIAN_POINT ( 'NONE',  ( 30.92651641011650199, 1464.557726000649836, 270.3478336023849806 ) ) ;
#89237=B_SPLINE_CURVE_WITH_KNOTS ( 'NONE', 3,
 ( #88196, #55714, #5845, #6387, #39437, #75264, #73612, #64666, #74711, #92044, #98232, #90372, #32139, #64111, #73048, #23171, #13650, #15316, #66324, #47840, #99872, #49509, #40535, #107741, #81973, #98783, #83634, #5281, #22046, #108842, #23725, #13107, #100442, #31025, #109413, #6930, #21501, #56243, #65207, #65755, #99320, #57371, #108292, #57910, #82551, #41087, #22594, #48963, #89835, #56797, #47290, #74161, #83094, #90934, #14221, #107189, #48407, #39985, #91498, #81413, #14777 ),
 .UNSPECIFIED., .F., .F.,
 ( 4, 2, 2, 2, 2, 2, 1, 2, 2, 2, 1, 2, 2, 2, 2, 1, 1, 1, 2, 2, 2, 2, 2, 1, 2, 2, 2, 1, 2, 2, 2, 2, 2, 4 ),
 ( 0.000000000000000000, 0.06249999999394668937, 0.09374999999092048508, 0.1093749999892469627, 0.1249999999875734263, 0.1874999999799758787, 0.2187499999763425629, 0.2343749999743528212, 0.2499999999723631072, 0.3124999999644023640, 0.3437499999604230472, 0.3593749999585725274, 0.3749999999567220632, 0.4374999999493155989, 0.4687499999456131716, 0.4843749999436541276, 0.4921874999427758302, 0.4960937499424362129, 0.4980468749422645725, 0.4999999999420928765, 0.5624999999485508217, 0.5937499999517797944, 0.6093749999533922823, 0.6171874999542571461, 0.6210937499547435348, 0.6249999999552299235, 0.6874999999624902269, 0.7187499999661217664, 0.7343749999679390905, 0.7499999999697564146, 0.8124999999772816173, 0.8437499999811264306, 0.8749999999849713550, 1.000000000000000000 ),
 .UNSPECIFIED. ) ;
#89242=CARTESIAN_POINT ( 'NONE',  ( 9.923338817417189262, 1442.404032688280040, 184.8562081593751429 ) ) ;
#89243=CARTESIAN_POINT ( 'NONE',  ( 1.962873812034300114, 1450.341737227420026, 154.5188752846379714 ) ) ;
#89244=CARTESIAN_POINT ( 'NONE',  ( -13.81908124539619998, 1415.258594623649969, 220.7407950635269742 ) ) ;
#89245=CARTESIAN_POINT ( 'NONE',  ( 18.35614473481600584, 1445.354571529838722, 191.3429017698720145 ) ) ;
#89246=EDGE_LOOP ( 'NONE', ( #10639, #91377, #94057, #25261, #101626, #45895, #109157, #73212, #48225, #44979, #68381, #46817, #104060, #95374 ) ) ;
#89247=CARTESIAN_POINT ( 'NONE',  ( -37.18025140759999658, 1432.092748029830091, 265.6112249940979950 ) ) ;
#89250=CARTESIAN_POINT ( 'NONE',  ( -0.8899015605279998464, 1476.102961708030080, 267.8536994237979911 ) ) ;
#89251=CARTESIAN_POINT ( 'NONE',  ( -12.98226713004480004, 1414.913060387349788, 219.9156686614909972 ) ) ;
#89253=CARTESIAN_POINT ( 'NONE',  ( 16.19492570339999915, 1409.478599654730033, 224.8086529783979870 ) ) ;
#89256=B_SPLINE_SURFACE_WITH_KNOTS ( 'NONE', 5, 5, ( 
 ( #102145, #83699, #67481, #32202, #7549, #68580 ),
 ( #33289, #60179, #50124, #50660, #76974, #34407 ),
 ( #92105, #9216, #85912, #41153, #110560, #59621 ),
 ( #281, #43375, #8090, #102684, #110013, #15382 ),
 ( #77523, #25426, #93732, #17011, #66384, #100503 ),
 ( #49571, #75328, #109470, #58519, #88691, #60745 ),
 ( #35510, #10305, #54011, #79193, #53443, #19233 ),
 ( #45600, #18143, #52340, #87588, #46153, #43918 ),
 ( #103822, #71371, #3050, #86461, #61853, #37175 ),
 ( #10877, #27667, #79742, #61307, #94867, #78625 ),
 ( #1367, #78065, #11970, #36077, #823, #95426 ),
 ( #62974, #104930, #19806, #70818, #105484, #34953 ),
 ( #28774, #45048, #69703, #104371, #9752, #2499 ),
 ( #95972, #88142, #36618, #97087, #44479, #28215 ),
 ( #27121, #18687, #62404, #96532, #11430, #52885 ) ),
 .UNSPECIFIED., .F., .F., .F.,
 ( 6, 3, 3, 3, 6 ),
 ( 6, 6 ),
 ( 44.15568540390000152, 56.49823163619999633, 69.80263562410000588, 81.33849626609999461, 85.77622357600000669 ),
 ( 0.000000000000000000, 2.000000000000000000 ),
 .UNSPECIFIED. ) ;
#89260=CARTESIAN_POINT ( 'NONE',  ( -11.07268104156529986, 1396.299726929629969, 209.2078313262790061 ) ) ;
#89261=CARTESIAN_POINT ( 'NONE',  ( -15.67023493909999665, 1420.566432160730074, 227.0266865602980033 ) ) ;
#89262=VECTOR ( 'NONE', #69579, 1000.000000000000341 ) ;
#89263=CARTESIAN_POINT ( 'NONE',  ( 19.56650236141162935, 1455.497407615608608, 225.8439199820629142 ) ) ;
#89264=EDGE_LOOP ( 'NONE', ( #33231, #55325, #12868, #100131, #53577 ) ) ;
#89266=CARTESIAN_POINT ( 'NONE',  ( 1.137831829869999867, 1408.952794351630018, 231.4765879240979984 ) ) ;
#89267=CARTESIAN_POINT ( 'NONE',  ( -6.358358198699995967, 1484.270642863229568, 183.8946942232976483 ) ) ;
#89268=CARTESIAN_POINT ( 'NONE',  ( 11.01694515279999997, 1425.660268107129923, 115.7225178154979943 ) ) ;
#89270=CARTESIAN_POINT ( 'NONE',  ( 5399.190776299724348, 2837.541834147233658, -8134.792049093189235 ) ) ;
#89271=CARTESIAN_POINT ( 'NONE',  ( -13.51610093808349866, 1443.913060387330006, 205.0760988357349959 ) ) ;
#89275=CARTESIAN_POINT ( 'NONE',  ( -2.439001525050000119, 1430.488531030629929, 150.2249694046979869 ) ) ;
#89276=CARTESIAN_POINT ( 'NONE',  ( 4.287256129599999355, 1508.836301919430298, 180.7363543702979882 ) ) ;
#89279=AXIS2_PLACEMENT_3D ( 'NONE', #105870, #57129, #13981 ) ;
#89282=ORIENTED_EDGE ( 'NONE', *, *, #17992, .F. ) ;
#89286=CARTESIAN_POINT ( 'NONE',  ( 0.4654153100249480146, 1490.951906556200129, 236.6680651313590147 ) ) ;
#89287=CARTESIAN_POINT ( 'NONE',  ( 15.28420222189999933, 1497.713060387329961, 225.7900586086979899 ) ) ;
#89289=( BOUNDED_CURVE ( )  B_SPLINE_CURVE ( 3, ( #50500, #75153, #33662, #101967 ),
 .UNSPECIFIED., .F., .F. ) 
 B_SPLINE_CURVE_WITH_KNOTS ( ( 4, 4 ),
 ( 4.834686371853470277, 5.479655915121550258 ),
 .UNSPECIFIED. ) 
 CURVE ( )  GEOMETRIC_REPRESENTATION_ITEM ( )  RATIONAL_B_SPLINE_CURVE ( ( 1.000000000000000000, 0.9656339083259537492, 0.9656339083259537492, 1.000000000000000000 ) ) 
 REPRESENTATION_ITEM ( '' )  );
#89291=CARTESIAN_POINT ( 'NONE',  ( -1.360610103134009874, 1413.432550495719852, 185.4726596582680145 ) ) ;
#89292=ADVANCED_FACE ( 'NONE', ( #9871 ), #71650, .F. ) ;
#89293=CARTESIAN_POINT ( 'NONE',  ( 2.982689009480000486, 1410.303126873030124, 185.7169846868979732 ) ) ;
#89297=CARTESIAN_POINT ( 'NONE',  ( 40.45017409928269814, 1439.698990137739884, 136.1552142357990078 ) ) ;
#89298=CARTESIAN_POINT ( 'NONE',  ( 7.675121520048339363, 1396.181081537549971, 217.0737066862720042 ) ) ;
#89299=CARTESIAN_POINT ( 'NONE',  ( -19.25375188179999952, 1464.258769156330118, 194.1747703853979772 ) ) ;
#89300=CARTESIAN_POINT ( 'NONE',  ( 11.74760992340000065, 1430.665155385330081, 150.5937701333980101 ) ) ;
#89301=CARTESIAN_POINT ( 'NONE',  ( 41.66194051640000140, 1443.744879019749987, 136.1277437682980178 ) ) ;
#89303=CARTESIAN_POINT ( 'NONE',  ( 3.957454374529999708, 1424.240901629729933, 184.6710418408979990 ) ) ;
#89304=CARTESIAN_POINT ( 'NONE',  ( 12.16634552240000033, 1441.485087603719876, 188.2667282966980338 ) ) ;
#89305=B_SPLINE_CURVE_WITH_KNOTS ( 'NONE', 3,
 ( #79435, #27921, #79978, #35770, #69953, #3297, #36312 ),
 .UNSPECIFIED., .F., .F.,
 ( 4, 3, 4 ),
 ( -157.7844419369999969, -101.5360198676929997, -30.93609007920730392 ),
 .UNSPECIFIED. ) ;
#89308=CARTESIAN_POINT ( 'NONE',  ( -17.65750842319999947, 1478.114914029529928, 228.8033778946980021 ) ) ;
#89316=CARTESIAN_POINT ( 'NONE',  ( 5.281924519060000378, 1415.931391677329884, 226.2877012803980108 ) ) ;
#89318=AXIS2_PLACEMENT_3D ( 'NONE', #67962, #6917, #15840 ) ;
#89319=CARTESIAN_POINT ( 'NONE',  ( -37.61786880320000392, 1440.913060387330006, 264.6588860065979816 ) ) ;
#89320=EDGE_CURVE ( 'NONE', #12979, #40553, #80944, .T. ) ;
#89321=CARTESIAN_POINT ( 'NONE',  ( 11.86794117217350397, 1433.007090821210568, 150.2053110587648632 ) ) ;
#89322=CARTESIAN_POINT ( 'NONE',  ( -10.07203899970000016, 1409.765688315129864, 229.3746300812979939 ) ) ;
#89324=CARTESIAN_POINT ( 'NONE',  ( -12.54268436849999979, 1408.913060387329779, 195.2008187059980173 ) ) ;
#89327=CARTESIAN_POINT ( 'NONE',  ( -25.24317812581459819, 1440.913060497079869, 217.5666783990430133 ) ) ;
#89328=CARTESIAN_POINT ( 'NONE',  ( 20.64229337434479561, 1507.778434579259965, 226.7718724856480037 ) ) ;
#89330=ADVANCED_FACE ( 'NONE', ( #74220 ), #89500, .T. ) ;
#89331=CARTESIAN_POINT ( 'NONE',  ( 44.43452778323990060, 1436.360229837989891, 270.0922544047889460 ) ) ;
#89335=CARTESIAN_POINT ( 'NONE',  ( 23.33118560439999811, 1410.121805423329988, 208.1130523111279729 ) ) ;
#89336=CARTESIAN_POINT ( 'NONE',  ( 0.009105150452084580931, 1508.374673153829917, 237.8724040003439768 ) ) ;
#89340=CARTESIAN_POINT ( 'NONE',  ( 4.172120233436539927, 1421.397866124950042, 185.0689737346249899 ) ) ;
#89341=CARTESIAN_POINT ( 'NONE',  ( -1.884384940320000146, 1417.914943765129919, 233.1634843046979881 ) ) ;
#89348=CARTESIAN_POINT ( 'NONE',  ( 19.59880151960000205, 1507.802454151830034, 188.8055342685979952 ) ) ;
#89349=AXIS2_PLACEMENT_3D ( 'NONE', #95747, #71699, #44257 ) ;
#89350=CARTESIAN_POINT ( 'NONE',  ( -24.90171366722389834, 1441.078953672730222, 210.4323502101370025 ) ) ;
#89352=CARTESIAN_POINT ( 'NONE',  ( 0.4110931836658809901, 1452.974865402240084, 183.2795641384469718 ) ) ;
#89355=CARTESIAN_POINT ( 'NONE',  ( 18.64442764509999861, 1507.939506224430033, 188.5219863284980022 ) ) ;
#89356=CARTESIAN_POINT ( 'NONE',  ( -11.44665353847253186, 1425.798163151176823, 139.1345268192609126 ) ) ;
#89361=ORIENTED_EDGE ( 'NONE', *, *, #69020, .F. ) ;
#89363=CARTESIAN_POINT ( 'NONE',  ( 11.60004869885203327, 1426.765776710964019, 134.3812685280135497 ) ) ;
#89364=CARTESIAN_POINT ( 'NONE',  ( 9.940067125116463842, 1435.763642648871837, 152.5323839883900803 ) ) ;
#89367=UNCERTAINTY_MEASURE_WITH_UNIT (LENGTH_MEASURE( 1.000000000000000082E-05 ), #19752, 'distance_accuracy_value', 'NONE');
#89369=CARTESIAN_POINT ( 'NONE',  ( -26.95412021097830291, 1509.373492805739943, 201.3014358241730122 ) ) ;
#89370=FACE_OUTER_BOUND ( 'NONE', #108045, .T. ) ;
#89371=CARTESIAN_POINT ( 'NONE',  ( -19.24890086970000169, 1426.049025734429961, 226.0195547209980305 ) ) ;
#89372=CARTESIAN_POINT ( 'NONE',  ( -21.13920444840000101, 1435.664861300689836, 143.7512800368980095 ) ) ;
#89374=CARTESIAN_POINT ( 'NONE',  ( 16.27871131059999854, 1509.481525512630014, 185.4630867003979802 ) ) ;
#89376=CARTESIAN_POINT ( 'NONE',  ( -18.71783619763316509, 1437.581472098226641, 211.6929844148049824 ) ) ;
#89377=CARTESIAN_POINT ( 'NONE',  ( -0.2682795917991919743, 1457.891717849350016, 229.2666142623699841 ) ) ;
#89380=CARTESIAN_POINT ( 'NONE',  ( -0.3621993323151809774, 1416.825784014559986, 191.0664209890499876 ) ) ;
#89385=CARTESIAN_POINT ( 'NONE',  ( -18.56428495200000128, 1507.623776005530090, 229.7144034790980243 ) ) ;
#89387=CARTESIAN_POINT ( 'NONE',  ( 21.20437582439999957, 1519.913060387329779, 218.3247824702980040 ) ) ;
#89389=CARTESIAN_POINT ( 'NONE',  ( -16.81223226430000039, 1414.913060387329779, 207.5743821216680089 ) ) ;
#89396=CARTESIAN_POINT ( 'NONE',  ( 20.99191170940000362, 1509.583341178129785, 188.7493971674979889 ) ) ;
#89403=CARTESIAN_POINT ( 'NONE',  ( 12.25335341949999979, 1440.953202899389908, 188.4028591661979704 ) ) ;
#89404=CARTESIAN_POINT ( 'NONE',  ( 14.12038737319999804, 1509.406339941330089, 234.8413163218980060 ) ) ;
#89405=CARTESIAN_POINT ( 'NONE',  ( 12.88090278901364094, 1442.881791335779553, 169.4390353358178345 ) ) ;
#89406=CARTESIAN_POINT ( 'NONE',  ( 29.35424698433324053, 1419.108688181071784, 269.4640726278769307 ) ) ;
#89407=CARTESIAN_POINT ( 'NONE',  ( -34.21460436289999762, 1445.299194188719866, 250.0133502388980276 ) ) ;
#89408=CARTESIAN_POINT ( 'NONE',  ( -19.79895059749999930, 1487.981277986430086, 190.0341339962980101 ) ) ;
#89409=CARTESIAN_POINT ( 'NONE',  ( -11.77426720859999953, 1433.514918800020041, 150.7945381811979928 ) ) ;
#89410=CARTESIAN_POINT ( 'NONE',  ( 28.08606285309999961, 1509.893847314130198, 201.5170686698379825 ) ) ;
#89411=CARTESIAN_POINT ( 'NONE',  ( -19.13600947890000015, 1486.262565671930133, 189.4467765145979854 ) ) ;
#89413=CARTESIAN_POINT ( 'NONE',  ( -26.64345414829999825, 1440.570068888169999, 137.3587798196979861 ) ) ;
#89415=FACE_OUTER_BOUND ( 'NONE', #73285, .T. ) ;
#89418=CARTESIAN_POINT ( 'NONE',  ( 3.622743996232769967E-09, 1410.219912027380133, 258.0694156936299919 ) ) ;
#89423=CARTESIAN_POINT ( 'NONE',  ( -20.84494148259999946, 1470.316654825529895, 270.2130226670980164 ) ) ;
#89427=AXIS2_PLACEMENT_3D ( 'NONE', #75273, #109420, #66876 ) ;
#89428=CARTESIAN_POINT ( 'NONE',  ( 0.2060742663968820054, 1452.528028601769847, 183.2209051729230112 ) ) ;
#89429=CARTESIAN_POINT ( 'NONE',  ( -14.09400383010000013, 1421.906236174930200, 228.7093513157980169 ) ) ;
#89430=CARTESIAN_POINT ( 'NONE',  ( 10.73506988043325627, 1424.972993549859893, 139.1354236083641922 ) ) ;
#89434=CARTESIAN_POINT ( 'NONE',  ( -45.62535461455620123, 1435.567858674460012, 268.2222749696159667 ) ) ;
#89437=CARTESIAN_POINT ( 'NONE',  ( -3.531632230717580256, 1490.204869628420056, 181.6974446958380156 ) ) ;
#89443=CARTESIAN_POINT ( 'NONE',  ( -15.84954036500000107, 1425.421969000529998, 190.5298818713980040 ) ) ;
#89445=CARTESIAN_POINT ( 'NONE',  ( 4.406802116531240543, 1421.289453786690501, 144.1378412804505160 ) ) ;
#89448=ADVANCED_FACE ( 'NONE', ( #47893 ), #54647, .T. ) ;
#89450=CARTESIAN_POINT ( 'NONE',  ( 0.8087773895360982346, 1508.989140809515220, 238.8276268623044132 ) ) ;
#89451=VERTEX_POINT ( 'NONE', #103813 ) ;
#89452=CARTESIAN_POINT ( 'NONE',  ( -13.46173026269689998, 1409.689012232490086, 270.3660067276319978 ) ) ;
#89453=CARTESIAN_POINT ( 'NONE',  ( -33.13365747560000329, 1435.654560788539811, 135.0902693358980287 ) ) ;
#89454=CARTESIAN_POINT ( 'NONE',  ( 2.903721707529999602E-11, 1395.913060387330006, 198.1220674040980043 ) ) ;
#89456=ORIENTED_EDGE ( 'NONE', *, *, #77742, .T. ) ;
#89458=CARTESIAN_POINT ( 'NONE',  ( 43.59041716596218663, 1451.056131081360263, 269.0321477434157487 ) ) ;
#89462=CARTESIAN_POINT ( 'NONE',  ( -0.9471777936590000113, 1485.704136142530160, 181.8966647610979805 ) ) ;
#89463=CARTESIAN_POINT ( 'NONE',  ( -18.38499229356419917, 1415.595619977600109, 207.5688028031409829 ) ) ;
#89466=CARTESIAN_POINT ( 'NONE',  ( -0.0001241292207142050271, 1476.050175603799744, 268.4837846581640406 ) ) ;
#89467=CARTESIAN_POINT ( 'NONE',  ( 12.45642902069999991, 1416.822690122629865, 223.4763059356979795 ) ) ;
#89471=CARTESIAN_POINT ( 'NONE',  ( -40.71747595459120106, 1438.773003512900004, 135.6928028942980120 ) ) ;
#89472=CARTESIAN_POINT ( 'NONE',  ( -23.89217091865537768, 1446.185953660134601, 213.4188154793815784 ) ) ;
#89474=CARTESIAN_POINT ( 'NONE',  ( 1.577711128016545006, 1457.769755330347834, 228.8717772423867700 ) ) ;
#89476=CARTESIAN_POINT ( 'NONE',  ( 25.37853710749670100, 1450.982216501690118, 137.2656895386909923 ) ) ;
#89478=CARTESIAN_POINT ( 'NONE',  ( 14.08840122829999864, 1415.996778985530000, 196.6785942718979925 ) ) ;
#89480=CARTESIAN_POINT ( 'NONE',  ( 21.45434793639999782, 1410.156528989129811, 201.8904129172080104 ) ) ;
#89481=CARTESIAN_POINT ( 'NONE',  ( 28.84486411959998975, 1445.052233488288948, 176.6843673542979332 ) ) ;
#89482=CARTESIAN_POINT ( 'NONE',  ( 16.98922847780000112, 1409.671041244329899, 225.3825873552979999 ) ) ;
#89484=CARTESIAN_POINT ( 'NONE',  ( 21.03221526084817583, 1454.576107912622774, 222.0093531227894061 ) ) ;
#89485=CARTESIAN_POINT ( 'NONE',  ( 2.500000000000000000, 1439.390253026290111, 161.6061712116469948 ) ) ;
#89487=ORIENTED_EDGE ( 'NONE', *, *, #61139, .F. ) ;
#89490=CARTESIAN_POINT ( 'NONE',  ( -3.609044149889999886, 1448.294815638699902, 185.0160860582980149 ) ) ;
#89491=CARTESIAN_POINT ( 'NONE',  ( 1.154619285495940073E-14, 1421.542801637179991, 144.1895650386140062 ) ) ;
#89492=CARTESIAN_POINT ( 'NONE',  ( -40.26102048347320306, 1444.237160703029986, 137.0925857260259875 ) ) ;
#89493=EDGE_CURVE ( 'NONE', #105791, #55354, #25165, .T. ) ;
#89494=CARTESIAN_POINT ( 'NONE',  ( 10.98404765546614215, 1424.970519178970562, 138.3342105157259425 ) ) ;
#89495=CARTESIAN_POINT ( 'NONE',  ( 1.854797713449190644, 1416.891245252034878, 232.8243438672992909 ) ) ;
#89497=CARTESIAN_POINT ( 'NONE',  ( -2.634342770595469840, 1484.261925542240078, 183.2842859132129831 ) ) ;
#89498=CARTESIAN_POINT ( 'NONE',  ( 11.87548778179999864, 1433.045415409350198, 150.0930343713980051 ) ) ;
#89499=CARTESIAN_POINT ( 'NONE',  ( -27.00409795999999929, 1468.895988936930280, 269.4154629628980047 ) ) ;
#89500=B_SPLINE_SURFACE_WITH_KNOTS ( 'NONE', 4, 5, ( 
 ( #101028, #99374, #40589, #90984, #23222, #14272 ),
 ( #22648, #31630, #110003, #39493, #6985, #65810 ),
 ( #109460, #75317, #57422, #6443, #83148, #56298 ),
 ( #41138, #49561, #91548, #14825, #74760, #32189 ),
 ( #108898, #73664, #66373, #90428, #33280, #49012 ) ),
 .UNSPECIFIED., .F., .F., .F.,
 ( 5, 5 ),
 ( 6, 6 ),
 ( 5.896863119889999894, 6.006609908439999757 ),
 ( 0.000000000000000000, 2.000000000000000000 ),
 .UNSPECIFIED. ) ;
#89501=CARTESIAN_POINT ( 'NONE',  ( 28.90001227645370108, 1440.913060387309997, 234.6055553947669807 ) ) ;
#89504=EDGE_LOOP ( 'NONE', ( #75856, #101721, #76413, #81567, #68823 ) ) ;
#89510=CARTESIAN_POINT ( 'NONE',  ( -8.326400914709999768, 1507.918721568629962, 235.2420587249980031 ) ) ;
#89513=CARTESIAN_POINT ( 'NONE',  ( 5.703571544217409972, 1423.268783014629889, 97.22701424869330822 ) ) ;
#89515=CARTESIAN_POINT ( 'NONE',  ( 1.486914849300000174, 1466.335769990830158, 234.9545319649979831 ) ) ;
#89517=ORIENTED_EDGE ( 'NONE', *, *, #66450, .F. ) ;
#89518=CARTESIAN_POINT ( 'NONE',  ( -0.4497180320269999476, 1451.473261245730100, 182.7775570608980047 ) ) ;
#89524=EDGE_LOOP ( 'NONE', ( #46628, #21703, #90673, #90674 ) ) ;
#89529=CARTESIAN_POINT ( 'NONE',  ( 3.156166260290000025, 1466.544008048530031, 236.1241471695980181 ) ) ;
#89530=CARTESIAN_POINT ( 'NONE',  ( -11.60004869885203860, 1426.730434967580550, 134.4361580478455949 ) ) ;
#89532=AXIS2_PLACEMENT_3D ( 'NONE', #92414, #110333, #58290 ) ;
#89533=CARTESIAN_POINT ( 'NONE',  ( 19.53037967897675387, 1509.610924284994326, 186.9102273450286305 ) ) ;
#89534=CARTESIAN_POINT ( 'NONE',  ( 2.629053311723080100, 1409.004868951980143, 194.3627930264940176 ) ) ;
#89537=CARTESIAN_POINT ( 'NONE',  ( -18.35381443609999863, 1463.216262999530045, 190.2560332892980171 ) ) ;
#89539=CARTESIAN_POINT ( 'NONE',  ( -3.259594021489010007, 1449.992738614869950, 184.7284798427360215 ) ) ;
#89543=CARTESIAN_POINT ( 'NONE',  ( -11.66418951239869983, 1415.301705643500100, 195.2579644112690289 ) ) ;
#89544=CARTESIAN_POINT ( 'NONE',  ( -11.96285889400000002, 1434.857482882780005, 151.1275188542980175 ) ) ;
#89547=CARTESIAN_POINT ( 'NONE',  ( -7.765407202818009861E-10, 1467.540443453480066, 246.7923564290519778 ) ) ;
#89548=CARTESIAN_POINT ( 'NONE',  ( -20.54913697329470068, 1506.217349134330107, 190.4370943769829978 ) ) ;
#89549=CARTESIAN_POINT ( 'NONE',  ( 10.07328664426130516, 1509.264827308277518, 236.8976276071642246 ) ) ;
#89551=CARTESIAN_POINT ( 'NONE',  ( 0.2192852207989999802, 1452.168323573130010, 183.2890642940980115 ) ) ;
#89553=CARTESIAN_POINT ( 'NONE',  ( -26.43279506992269390, 1436.721711417935239, 136.8206605300602234 ) ) ;
#89556=CARTESIAN_POINT ( 'NONE',  ( 11.14607745555529839, 1434.019391663140141, 151.6534738377419842 ) ) ;
#89557=CARTESIAN_POINT ( 'NONE',  ( -13.52799278891819945, 1434.953562907949845, 148.7718104166640103 ) ) ;
#89560=CARTESIAN_POINT ( 'NONE',  ( 19.03110457515579768, 1457.047041246000163, 226.1578386336209974 ) ) ;
#89561=FACE_OUTER_BOUND ( 'NONE', #40529, .T. ) ;
#89563=CARTESIAN_POINT ( 'NONE',  ( 34.48978216879999792, 1440.913060389390012, 250.0021841763980319 ) ) ;
#89565=CARTESIAN_POINT ( 'NONE',  ( -9.984537528192330313, 1425.226300119460120, 93.54765018715950475 ) ) ;
#89566=DIRECTION ( 'NONE',  ( 0.000000000000000000, 1.000000000000000000, 0.000000000000000000 ) ) ;
#89568=CARTESIAN_POINT ( 'NONE',  ( -25.05703569219999949, 1435.888271332780050, 220.8261789359980014 ) ) ;
#89570=CARTESIAN_POINT ( 'NONE',  ( -13.12775437379390020, 1414.913060581094669, 220.0542260670848123 ) ) ;
#89571=CARTESIAN_POINT ( 'NONE',  ( 29.24087205800000078, 1450.603665907289951, 136.3826361771980089 ) ) ;
#89575=CARTESIAN_POINT ( 'NONE',  ( 11.51728378950000042, 1509.315252799729933, 236.2324387071979857 ) ) ;
#89577=ORIENTED_EDGE ( 'NONE', *, *, #93787, .F. ) ;
#89579=CARTESIAN_POINT ( 'NONE',  ( -24.04783088717389816, 1410.733285934720243, 208.7113026174390029 ) ) ;
#89580=ORIENTED_EDGE ( 'NONE', *, *, #62089, .T. ) ;
#89583=VECTOR ( 'NONE', #75930, 1000.000000000000000 ) ;
#89584=B_SPLINE_CURVE_WITH_KNOTS ( 'NONE', 3,
 ( #51053, #658, #51602, #25816, #8471, #60014, #43750, #77901, #1208, #41549, #33673, #67865, #34236, #92477, #42644, #109852, #15747, #34789, #49948, #75705, #16305, #68422, #7384, #84086, #25262, #42098, #85735, #76797, #110393, #101413, #94135, #24705, #9034, #94693, #43206, #50509, #66772, #68976, #103077, #26378, #60573, #17966, #52161, #100871, #24162, #58352, #19065, #86846, #37547, #35342, #28594, #63333, #52711, #88510, #97453, #44310, #11794, #78454, #61137, #80098, #54916, #45961, #87973, #89042, #28039, #62229, #18514, #20180, #19633, #20721, #95251, #53270, #53834, #45424, #96355, #12330, #36437, #70088, #10702, #1767, #3418, #46520, #71182, #10139, #62796, #80655, #27486, #44874, #36988, #79566, #11262, #71749, #87409, #2867, #61675, #105866, #54378, #29145, #105304, #69530, #96910, #103650, #79025, #26948, #35905, #104201, #95798, #2327, #70634 ),
 .UNSPECIFIED., .F., .F.,
 ( 4, 3, 3, 3, 3, 3, 3, 3, 3, 3, 3, 3, 3, 3, 3, 3, 3, 3, 3, 3, 3, 3, 3, 3, 3, 3, 3, 3, 3, 3, 3, 3, 3, 3, 3, 3, 4 ),
 ( 3.497608506310000198, 4.529268212650570113, 4.673809866680000091, 5.552633724228540402, 5.850011227059999541, 6.748642867657440370, 7.649943429611059997, 8.202413947820000217, 9.104080493403879260, 10.00194339904189889, 10.89091721172289873, 11.77326960059560079, 12.64490599439209895, 12.90721938930000157, 13.77712401890710048, 14.64888018335460096, 15.52348301336279945, 16.34806929659060160, 17.19513031426199845, 18.01644611260000062, 18.06848103991510257, 18.56473004397999915, 18.75451818430730100, 18.85043071655640290, 18.86798389980000223, 18.98461694718449877, 19.11219043176969734, 19.21468060761500141, 19.30785973235489905, 19.39334657279270147, 19.44079725900000000, 19.48296743266269715, 19.52937033080259965, 19.59042956274780067, 19.64886608588970063, 19.69360426244629991, 19.71952168709999853 ),
 .UNSPECIFIED. ) ;
#89585=CARTESIAN_POINT ( 'NONE',  ( -1.618414601050000012, 1489.063570503329856, 236.3146473097979765 ) ) ;
#89588=CARTESIAN_POINT ( 'NONE',  ( 45.63691321389429589, 1440.912969052420067, 268.9749694736630090 ) ) ;
#89589=CARTESIAN_POINT ( 'NONE',  ( -12.56955872635460025, 1415.089118586279938, 220.8661684437149972 ) ) ;
#89594=CARTESIAN_POINT ( 'NONE',  ( 13.08711526621821442, 1443.014180111750193, 187.3495770229439188 ) ) ;
#89599=CARTESIAN_POINT ( 'NONE',  ( 12.72577279029999886, 1508.073447237130040, 233.4251884259979875 ) ) ;
#89601=CARTESIAN_POINT ( 'NONE',  ( 22.98351633743509836, 1452.110458311199864, 138.7999742373860101 ) ) ;
#89604=CARTESIAN_POINT ( 'NONE',  ( 10.99924977368306145, 1433.357864536487796, 151.7593666591178021 ) ) ;
#89605=CARTESIAN_POINT ( 'NONE',  ( -21.21787123920067586, 1509.703102098133513, 230.0033421491306740 ) ) ;
#89606=CARTESIAN_POINT ( 'NONE',  ( 0.02456836867461557536, 1409.062161665360918, 232.4158905231754488 ) ) ;
#89607=CARTESIAN_POINT ( 'NONE',  ( -18.39585571575249645, 1464.527486176419870, 190.2183615832909993 ) ) ;
#89608=CARTESIAN_POINT ( 'NONE',  ( -3.482404828285579956, 1485.996524617339901, 182.2044860649310181 ) ) ;
#89610=VECTOR ( 'NONE', #84560, 1000.000000000000114 ) ;
#89619=( BOUNDED_CURVE ( )  B_SPLINE_CURVE ( 3, ( #97754, #5910, #21580, #14291 ),
 .UNSPECIFIED., .F., .F. ) 
 B_SPLINE_CURVE_WITH_KNOTS ( ( 4, 4 ),
 ( 1.569654617349090175, 1.584186644469695038 ),
 .UNSPECIFIED. ) 
 CURVE ( )  GEOMETRIC_REPRESENTATION_ITEM ( )  RATIONAL_B_SPLINE_CURVE ( ( 1.000000000000000000, 0.9999824017597387371, 0.9999824017597387371, 1.000000000000000000 ) ) 
 REPRESENTATION_ITEM ( '' )  );
#89622=CARTESIAN_POINT ( 'NONE',  ( 16.81223226430000039, 1414.913060387329779, 210.6693098017280192 ) ) ;
#89628=CARTESIAN_POINT ( 'NONE',  ( 12.86384817108610079, 1415.089948427380023, 197.4268898898679936 ) ) ;
#89632=CARTESIAN_POINT ( 'NONE',  ( 13.73047359140000090, 1422.103018753830156, 228.7261909963979747 ) ) ;
#89636=CARTESIAN_POINT ( 'NONE',  ( 41.46315275289999391, 1425.141660529629917, 266.8282284094979673 ) ) ;
#89637=CARTESIAN_POINT ( 'NONE',  ( -18.88903524680000245, 1410.934759576429997, 223.1880985098980261 ) ) ;
#89638=CARTESIAN_POINT ( 'NONE',  ( 16.06624336259999808, 1435.502499720209926, 148.4819144917980225 ) ) ;
#89640=CARTESIAN_POINT ( 'NONE',  ( 19.93032256160000415, 1508.017639892230136, 189.0239162005979949 ) ) ;
#89641=CARTESIAN_POINT ( 'NONE',  ( 22.91663120903140083, 1507.606285602550088, 210.6365840681099826 ) ) ;
#89642=CARTESIAN_POINT ( 'NONE',  ( 12.78755496029999961, 1416.844618638430120, 222.9177554082980066 ) ) ;
#89645=CARTESIAN_POINT ( 'NONE',  ( 0.2148841057284759937, 1454.612562414240074, 183.1842180022130151 ) ) ;
#89646=CARTESIAN_POINT ( 'NONE',  ( -11.92254695265209996, 1407.392238798829794, 215.8238487423210188 ) ) ;
#89647=CARTESIAN_POINT ( 'NONE',  ( 0.3152240322409999851, 1418.590776207229965, 184.6848380081979997 ) ) ;
#89650=CARTESIAN_POINT ( 'NONE',  ( 11.94155113780000121, 1433.614991520300009, 147.2728962421979872 ) ) ;
#89651=CARTESIAN_POINT ( 'NONE',  ( -28.14953226589999957, 1435.638849176820031, 136.1223312599980204 ) ) ;
#89652=CARTESIAN_POINT ( 'NONE',  ( 5.501991724969999886, 1440.536034637450030, 185.1205903260980108 ) ) ;
#89653=ORIENTED_EDGE ( 'NONE', *, *, #58907, .F. ) ;
#89655=CARTESIAN_POINT ( 'NONE',  ( -1.235199885961179911, 1408.956194517850008, 224.0686660204410146 ) ) ;
#89659=CARTESIAN_POINT ( 'NONE',  ( 40.56704996976148436, 1425.248325938897096, 269.1138862120274666 ) ) ;
#89660=CARTESIAN_POINT ( 'NONE',  ( -11.84289190199999986, 1435.906080920110071, 147.6777950973980182 ) ) ;
#89661=CARTESIAN_POINT ( 'NONE',  ( 19.70612301839999958, 1434.996842493730128, 210.6610967273779806 ) ) ;
#89662=CARTESIAN_POINT ( 'NONE',  ( -28.77730028790000105, 1509.917985857229951, 212.2396942694179813 ) ) ;
#89667=CARTESIAN_POINT ( 'NONE',  ( -27.53433169550000059, 1451.090186181929994, 136.3574917508980207 ) ) ;
#89672=ADVANCED_FACE ( 'NONE', ( #20342 ), #70726, .F. ) ;
#89673=CARTESIAN_POINT ( 'NONE',  ( -23.13309514930000077, 1409.720885870030088, 208.8451414652710127 ) ) ;
#89676=CARTESIAN_POINT ( 'NONE',  ( -25.25200574389469921, 1450.804213008409988, 137.6134964715130025 ) ) ;
#89677=CARTESIAN_POINT ( 'NONE',  ( -11.75715125319999999, 1415.140114695929924, 195.7397137993980039 ) ) ;
#89678=CARTESIAN_POINT ( 'NONE',  ( 0.003765252625069999848, 1466.769817372230136, 235.6257278897980143 ) ) ;
#89679=ADVANCED_FACE ( 'NONE', ( #56722 ), #38537, .F. ) ;
#89680=CARTESIAN_POINT ( 'NONE',  ( 18.88559166019999935, 1410.934781852329934, 221.7939351717979832 ) ) ;
#89681=CARTESIAN_POINT ( 'NONE',  ( -2.421689921559070147, 1414.941989913409998, 186.2944651685450026 ) ) ;
#89683=CARTESIAN_POINT ( 'NONE',  ( -5.376483239217891175, 1429.660786141449762, 154.2333551657499982 ) ) ;
#89684=CARTESIAN_POINT ( 'NONE',  ( -11.86750609110000099, 1432.440555272449956, 149.9822222932980083 ) ) ;
#89686=CARTESIAN_POINT ( 'NONE',  ( 25.82124364776869641, 1449.911324753369854, 209.1312396996160032 ) ) ;
#89689=CARTESIAN_POINT ( 'NONE',  ( -1.883560539969999947, 1415.581158730429934, 233.0664532878980140 ) ) ;
#89693=CARTESIAN_POINT ( 'NONE',  ( -3.379827007410890261, 1485.523830331509998, 182.9521946713460068 ) ) ;
#89696=CARTESIAN_POINT ( 'NONE',  ( 17.86855543449999928, 1415.163755998629995, 210.6784302842380043 ) ) ;
#89699=ORIENTED_EDGE ( 'NONE', *, *, #82941, .F. ) ;
#89700=CARTESIAN_POINT ( 'NONE',  ( 27.93707802169999965, 1509.154714909829863, 212.3148866501879866 ) ) ;
#89701=ORIENTED_EDGE ( 'NONE', *, *, #68742, .T. ) ;
#89704=CARTESIAN_POINT ( 'NONE',  ( -1.610281973209999908E-15, 1427.674934138829940, 112.4493539157979995 ) ) ;
#89707=EDGE_CURVE ( 'NONE', #50703, #77021, #58137, .T. ) ;
#89710=CARTESIAN_POINT ( 'NONE',  ( -24.55869259776619984, 1452.050375068560015, 136.1074992667110166 ) ) ;
#89711=CARTESIAN_POINT ( 'NONE',  ( -11.15480544429999910, 1425.160630053029990, 144.1619436909979868 ) ) ;
#89712=CARTESIAN_POINT ( 'NONE',  ( 14.12491358549999987, 1409.406313238730036, 226.3524348291979891 ) ) ;
#89716=CARTESIAN_POINT ( 'NONE',  ( 41.65030538173530061, 1443.228731902989921, 134.0999999981379744 ) ) ;
#89719=CARTESIAN_POINT ( 'NONE',  ( -16.94109862351797346, 1410.873590852185316, 226.2869239458361790 ) ) ;
#89725=CARTESIAN_POINT ( 'NONE',  ( 11.23374711189292618, 1410.679338792965154, 229.3371837158982203 ) ) ;
#89728=CARTESIAN_POINT ( 'NONE',  ( -3.140448395399999537, 1485.996777215629891, 182.1629481133980164 ) ) ;
#89733=CARTESIAN_POINT ( 'NONE',  ( -0.9145582870020000366, 1497.690648267530150, 231.5795319701980191 ) ) ;
#89734=CARTESIAN_POINT ( 'NONE',  ( 9.612666450629999915, 1414.913060387329779, 195.8647609382979908 ) ) ;
#89740=CARTESIAN_POINT ( 'NONE',  ( 38.06114384108260396, 1440.913060387330006, 265.0356504283799950 ) ) ;
#89742=ORIENTED_EDGE ( 'NONE', *, *, #76298, .F. ) ;
#89743=CARTESIAN_POINT ( 'NONE',  ( -0.4429558866438589870, 1450.897592026909933, 181.2687265345639958 ) ) ;
#89744=CARTESIAN_POINT ( 'NONE',  ( -14.38276615811366810, 1518.913060387330006, 182.7943691050095367 ) ) ;
#89745=CARTESIAN_POINT ( 'NONE',  ( -8.881784196999999612E-15, 1452.913060387330006, 126.8032249175980155 ) ) ;
#89750=CARTESIAN_POINT ( 'NONE',  ( 18.29857331400000220, 1408.824872542730191, 266.8292035143980456 ) ) ;
#89751=CARTESIAN_POINT ( 'NONE',  ( -11.87984373480000144, 1433.310963811260081, 146.4341628266979853 ) ) ;
#89752=CARTESIAN_POINT ( 'NONE',  ( 11.73605004184446976, 1425.975720587435035, 144.1605505835322560 ) ) ;
#89753=CARTESIAN_POINT ( 'NONE',  ( 2.937605202049999864, 1464.526028384730125, 236.2516354109980057 ) ) ;
#89754=CARTESIAN_POINT ( 'NONE',  ( 0.05885997228641060702, 1457.844234150280045, 229.0443196536700157 ) ) ;
#89755=B_SPLINE_CURVE_WITH_KNOTS ( 'NONE', 5,
 ( #29356, #64648, #36670, #63557, #47823, #98767, #70863, #31010, #6369, #75783, #16389, #6911 ),
 .UNSPECIFIED., .F., .F.,
 ( 6, 3, 3, 6 ),
 ( 0.000000000000000000, 0.2378339703147543949, 0.7135077814956326536, 1.000000000000000000 ),
 .UNSPECIFIED. ) ;
#89758=CARTESIAN_POINT ( 'NONE',  ( -0.1538198133092779918, 1507.373913156659910, 180.8743467545279771 ) ) ;
#89759=CARTESIAN_POINT ( 'NONE',  ( 19.12527834899882606, 1443.894831870294183, 213.6836570825134629 ) ) ;
#89761=CARTESIAN_POINT ( 'NONE',  ( -21.21614429629999776, 1488.813684182929819, 209.3550077978840136 ) ) ;
#89766=CARTESIAN_POINT ( 'NONE',  ( 2.339444114659999990E-09, 1462.218800619629974, 225.7558667929980061 ) ) ;
#89767=CARTESIAN_POINT ( 'NONE',  ( -11.76643225729999997, 1432.100642793779798, 150.8086033765980289 ) ) ;
#89774=CARTESIAN_POINT ( 'NONE',  ( -19.70972463880000092, 1444.803624437849976, 224.6978511680979977 ) ) ;
#89775=CARTESIAN_POINT ( 'NONE',  ( 5.386383302847690402, 1432.333871934329864, 154.6074109928329960 ) ) ;
#89776=CARTESIAN_POINT ( 'NONE',  ( -1.465804341989999982, 1484.360936341829984, 182.4810536920979871 ) ) ;
#89779=CARTESIAN_POINT ( 'NONE',  ( 3.435598742629999869, 1405.939636272029929, 267.2300248611979896 ) ) ;
#89781=CARTESIAN_POINT ( 'NONE',  ( -16.42420382550000113, 1507.212883782629888, 224.6993357452979865 ) ) ;
#89782=CARTESIAN_POINT ( 'NONE',  ( 23.52024624973322986, 1433.790221880693707, 214.9612971668913133 ) ) ;
#89788=CARTESIAN_POINT ( 'NONE',  ( -0.5699886577095060192, 1450.893155944799901, 155.0620570460170029 ) ) ;
#89789=CARTESIAN_POINT ( 'NONE',  ( -1.609652689937413061, 1451.521214583105120, 183.9748645127235420 ) ) ;
#89790=CARTESIAN_POINT ( 'NONE',  ( 1.981093176729999739, 1450.324655956839933, 155.6080914326980178 ) ) ;
#89791=CARTESIAN_POINT ( 'NONE',  ( -13.90692152972509987, 1415.348334734779883, 220.8295855263409919 ) ) ;
#89792=FACE_OUTER_BOUND ( 'NONE', #38815, .T. ) ;
#89793=CARTESIAN_POINT ( 'NONE',  ( -25.52872275889999898, 1431.191366577369990, 248.0989693098979956 ) ) ;
#89794=CARTESIAN_POINT ( 'NONE',  ( 11.18156373363127720, 1425.045528541028943, 138.1873464159537832 ) ) ;
#89795=CARTESIAN_POINT ( 'NONE',  ( 3.702277819670000358, 1440.893270118220016, 155.9286631201980242 ) ) ;
#89796=CARTESIAN_POINT ( 'NONE',  ( -0.8855859651640000108, 1475.830651730830141, 266.9608409856979847 ) ) ;
#89797=CARTESIAN_POINT ( 'NONE',  ( -4.251778211643499894, 1446.495381983220113, 160.8243770259319945 ) ) ;
#89798=CARTESIAN_POINT ( 'NONE',  ( -19.02991910360000105, 1457.008642855029848, 192.0880663617980133 ) ) ;
#89799=ADVANCED_FACE ( 'NONE', ( #109732 ), #11464, .T. ) ;
#89802=AXIS2_PLACEMENT_3D ( 'NONE', #80955, #21571, #14835 ) ;
#89803=CARTESIAN_POINT ( 'NONE',  ( 16.56954271164469716, 1507.336004463039899, 193.5476776774169707 ) ) ;
#89808=CARTESIAN_POINT ( 'NONE',  ( -7.863301563632830948, 1396.187652929399974, 216.8893108632619828 ) ) ;
#89811=CARTESIAN_POINT ( 'NONE',  ( -44.88917860750000699, 1439.584993159529859, 269.6920180689979247 ) ) ;
#89812=VERTEX_POINT ( 'NONE', #105762 ) ;
#89813=CARTESIAN_POINT ( 'NONE',  ( -2.451711519242490311, 1410.376778189126981, 232.6822308553063294 ) ) ;
#89814=CARTESIAN_POINT ( 'NONE',  ( 2.825023614729999633, 1409.011712385729879, 230.6344011842979853 ) ) ;
#89816=CARTESIAN_POINT ( 'NONE',  ( 10.56488187690000125, 1425.074640677629986, 128.4926088604979952 ) ) ;
#89818=CARTESIAN_POINT ( 'NONE',  ( -0.2981780139620000547, 1491.118694209130126, 236.6398961300979806 ) ) ;
#89824=CARTESIAN_POINT ( 'NONE',  ( 3.510779589379999788, 1509.015428989629982, 180.0383898831980218 ) ) ;
#89834=CARTESIAN_POINT ( 'NONE',  ( -1.477202341559999965, 1415.048591094029916, 226.7491272332979975 ) ) ;
#89835=CARTESIAN_POINT ( 'NONE',  ( -12.82920166685754815, 1444.968562662791328, 169.4458598129212419 ) ) ;
#89839=CARTESIAN_POINT ( 'NONE',  ( 11.68659302070000194, 1410.292622361829899, 189.6048334739980135 ) ) ;
#89841=CARTESIAN_POINT ( 'NONE',  ( -40.57136080872869854, 1447.824542289230067, 135.5531601139149984 ) ) ;
#89843=CARTESIAN_POINT ( 'NONE',  ( 11.05891918951989972, 1396.299246355200239, 209.6785178209389926 ) ) ;
#89845=CARTESIAN_POINT ( 'NONE',  ( 11.84502656599999959, 1430.880975159330092, 149.7917605896980149 ) ) ;
#89846=DIRECTION ( 'NONE',  ( 0.000000000000000000, 1.000000000000000000, 0.000000000000000000 ) ) ;
#89847=ORIENTED_EDGE ( 'NONE', *, *, #8293, .T. ) ;
#89848=CARTESIAN_POINT ( 'NONE',  ( 4.282619229829998986, 1425.872306577030031, 185.4231226939979820 ) ) ;
#89849=CARTESIAN_POINT ( 'NONE',  ( 12.16249367390000025, 1441.737599154800137, 188.1412300377979818 ) ) ;
#89850=B_SPLINE_CURVE_WITH_KNOTS ( 'NONE', 5,
 ( #31846, #108556, #13370, #81143, #23440, #100692 ),
 .UNSPECIFIED., .F., .F.,
 ( 6, 6 ),
 ( 0.000000000000000000, 1.000000000000000000 ),
 .UNSPECIFIED. ) ;
#89852=ADVANCED_FACE ( 'NONE', ( #11685 ), #69914, .T. ) ;
#89853=ORIENTED_EDGE ( 'NONE', *, *, #97902, .F. ) ;
#89856=CARTESIAN_POINT ( 'NONE',  ( 24.55901760849999960, 1440.913060394469994, 213.0859796112679874 ) ) ;
#89857=CARTESIAN_POINT ( 'NONE',  ( 13.29676293300000012, 1434.820761659849950, 195.7037073619979992 ) ) ;
#89861=ORIENTED_EDGE ( 'NONE', *, *, #14706, .F. ) ;
#89863=CARTESIAN_POINT ( 'NONE',  ( -14.37487418797869942, 1509.495309192210016, 182.9308568162230131 ) ) ;
#89865=CARTESIAN_POINT ( 'NONE',  ( 4.836108313140000448, 1414.913060387329779, 224.5514542965979956 ) ) ;
#89868=CARTESIAN_POINT ( 'NONE',  ( -28.45308972560000171, 1509.159845678530019, 208.7911871173449754 ) ) ;
#89869=CARTESIAN_POINT ( 'NONE',  ( -38.90379940696828243, 1429.368923031839358, 269.5913158308796369 ) ) ;
#89870=CARTESIAN_POINT ( 'NONE',  ( -0.8669575069650000687, 1409.449195270830160, 232.8795264863980208 ) ) ;
#89871=CARTESIAN_POINT ( 'NONE',  ( -4.063550476549999679, 1497.713060387329961, 187.6673214695979937 ) ) ;
#89874=CARTESIAN_POINT ( 'NONE',  ( -35.16444583816929992, 1440.913060388340000, 251.2596977943379954 ) ) ;
#89876=CARTESIAN_POINT ( 'NONE',  ( -0.4289664345794019784, 1465.008324844339995, 237.3601925583080003 ) ) ;
#89877=CARTESIAN_POINT ( 'NONE',  ( 28.03275775867099995, 1417.152506600500146, 270.1137522001889693 ) ) ;
#89880=CARTESIAN_POINT ( 'NONE',  ( 23.48437040230000150, 1410.391238764530044, 207.9633649421280097 ) ) ;
#89881=CARTESIAN_POINT ( 'NONE',  ( 0.02088113289338846754, 1507.124156042135382, 237.3527289089472845 ) ) ;
#89885=CARTESIAN_POINT ( 'NONE',  ( 4.247639483515419201, 1421.862531007339840, 184.3113611789599986 ) ) ;
#89886=CARTESIAN_POINT ( 'NONE',  ( -3.082646531299999992, 1415.375634542629996, 232.7232394780980087 ) ) ;
#89890=CARTESIAN_POINT ( 'NONE',  ( 18.96325319869999859, 1416.831305841230005, 210.2431144155779918 ) ) ;
#89892=CARTESIAN_POINT ( 'NONE',  ( 20.15452300067990166, 1507.845791525220193, 189.3412703910400126 ) ) ;
#89893=CARTESIAN_POINT ( 'NONE',  ( -24.89775034519999863, 1442.835538705840008, 210.5176537872779932 ) ) ;
#89896=ADVANCED_FACE ( 'NONE', ( #20608 ), #71642, .F. ) ;
#89898=CARTESIAN_POINT ( 'NONE',  ( 18.34590456075850184, 1416.851343895820037, 209.3831232368769975 ) ) ;
#89899=DIRECTION ( 'NONE',  ( 1.000000000000000000, 0.000000000000000000, 0.000000000000000000 ) ) ;
#89901=EDGE_LOOP ( 'NONE', ( #71917, #18451, #8187, #61510 ) ) ;
#89905=CARTESIAN_POINT ( 'NONE',  ( 11.60004869885205459, 1426.591397983647767, 134.9942396637077024 ) ) ;
#89906=CARTESIAN_POINT ( 'NONE',  ( 10.59993614363193970, 1434.841029502628317, 152.0686027719855531 ) ) ;
#89909=CARTESIAN_POINT ( 'NONE',  ( -27.88505092258619911, 1509.867173926660143, 200.9431876222099902 ) ) ;
#89911=CARTESIAN_POINT ( 'NONE',  ( -4.260142627790000525, 1446.575473928930023, 159.4573725592980225 ) ) ;
#89912=CARTESIAN_POINT ( 'NONE',  ( -18.95264117809999860, 1425.362752766330232, 224.3521994502980021 ) ) ;
#89917=CARTESIAN_POINT ( 'NONE',  ( 28.29412261439999909, 1508.657108462829910, 209.2602327817579919 ) ) ;
#89920=CARTESIAN_POINT ( 'NONE',  ( -2.923521517025829741, 1410.394928878200062, 186.6127595807840009 ) ) ;
#89921=EDGE_CURVE ( 'NONE', #80100, #57683, #23534, .T. ) ;
#89925=CARTESIAN_POINT ( 'NONE',  ( -14.59882275830000076, 1475.513060387329915, 223.7206687204979971 ) ) ;
#89926=CARTESIAN_POINT ( 'NONE',  ( -18.55728995089999955, 1509.324399913130037, 230.4821994879980025 ) ) ;
#89928=CARTESIAN_POINT ( 'NONE',  ( -13.05831431138886956, 1442.991492262945712, 186.6128402540535092 ) ) ;
#89929=CARTESIAN_POINT ( 'NONE',  ( 26.79414481833639883, 1435.433178084320161, 135.2874577367330176 ) ) ;
#89942=VERTEX_POINT ( 'NONE', #48049 ) ;
#89944=CARTESIAN_POINT ( 'NONE',  ( 13.04304233460000084, 1507.484018513129968, 233.1962564005980028 ) ) ;
#89946=CARTESIAN_POINT ( 'NONE',  ( 38.63445848827170437, 1428.905190833854476, 269.5867826533756215 ) ) ;
#89947=CARTESIAN_POINT ( 'NONE',  ( 4.840407647989999825E-09, 1466.838857907629972, 244.5742075736980041 ) ) ;
#89950=CARTESIAN_POINT ( 'NONE',  ( -11.92436129959999924, 1433.423661116180028, 149.9160561082979939 ) ) ;
#89951=ADVANCED_FACE ( 'NONE', ( #4402 ), #11696, .T. ) ;
#89953=CARTESIAN_POINT ( 'NONE',  ( 11.60536311244090513, 1426.783531571186131, 134.7591166632975899 ) ) ;
#89955=CARTESIAN_POINT ( 'NONE',  ( -25.79175640970000316, 1440.622088907729903, 138.3748975615980044 ) ) ;
#89956=CARTESIAN_POINT ( 'NONE',  ( -24.41186851410000003, 1440.913063283769816, 212.0284779319380277 ) ) ;
#89957=DIRECTION ( 'NONE',  ( 0.000000000000000000, 0.7071067811865475727, 0.7071067811865475727 ) ) ;
#89961=CARTESIAN_POINT ( 'NONE',  ( -20.32885181593275448, 1509.740925697234843, 231.1842896567873140 ) ) ;
#89962=CARTESIAN_POINT ( 'NONE',  ( 1.124394224133599967E-08, 1406.771932233190000, 265.4689318986550006 ) ) ;
#89967=CARTESIAN_POINT ( 'NONE',  ( -28.70951102109999908, 1465.737235724629954, 270.3384643691979932 ) ) ;
#89971=CARTESIAN_POINT ( 'NONE',  ( 0.2292726218886919909, 1451.597858639469905, 182.7735418884959699 ) ) ;
#89972=CARTESIAN_POINT ( 'NONE',  ( -14.16989755279999841, 1420.440733325929841, 227.4201777901979824 ) ) ;
#89973=CARTESIAN_POINT ( 'NONE',  ( -16.17568153084674520, 1459.146937367386045, 230.7169172031621542 ) ) ;
#89976=CARTESIAN_POINT ( 'NONE',  ( -27.41102939123420157, 1412.722695273399950, 266.9253032451249510 ) ) ;
#89977=ORIENTED_EDGE ( 'NONE', *, *, #18142, .F. ) ;
#89978=CARTESIAN_POINT ( 'NONE',  ( -3.528579519175909951, 1487.425795918970152, 181.8155835057870036 ) ) ;
#89979=ADVANCED_FACE ( 'NONE', ( #61860 ), #28687, .T. ) ;
#89981=VERTEX_POINT ( 'NONE', #91292 ) ;
#89984=EDGE_CURVE ( 'NONE', #43805, #45625, #2028, .T. ) ;
#89986=CARTESIAN_POINT ( 'NONE',  ( -2.499999999999998668, 1439.922964613317845, 170.5265280277067461 ) ) ;
#89987=CARTESIAN_POINT ( 'NONE',  ( -16.29048445220000119, 1440.437958515699847, 190.0548704972979976 ) ) ;
#89988=DIRECTION ( 'NONE',  ( 0.000000000000000000, 0.000000000000000000, 1.000000000000000000 ) ) ;
#89989=ORIENTED_EDGE ( 'NONE', *, *, #16880, .T. ) ;
#89990=LINE ( 'NONE', #13265, #43942 ) ;
#89991=EDGE_CURVE ( 'NONE', #12156, #57816, #30828, .T. ) ;
#89995=CARTESIAN_POINT ( 'NONE',  ( -38.39577626298080304, 1426.808633107450078, 269.8162326586069639 ) ) ;
#89996=CARTESIAN_POINT ( 'NONE',  ( -31.76432722529999708, 1435.606706419230022, 135.1329931210979964 ) ) ;
#89997=CARTESIAN_POINT ( 'NONE',  ( -3.320612525290000061, 1396.029018731929909, 198.5240420177980241 ) ) ;
#90000=ORIENTED_EDGE ( 'NONE', *, *, #29727, .T. ) ;
#90001=CARTESIAN_POINT ( 'NONE',  ( 34.55717928115133475, 1463.247045597946226, 269.2604522464154684 ) ) ;
#90004=CARTESIAN_POINT ( 'NONE',  ( -0.03316221134518849978, 1410.241317949180257, 185.0241807165079990 ) ) ;
#90006=CARTESIAN_POINT ( 'NONE',  ( -19.78000735379999853, 1435.771566308190131, 223.7853677692980057 ) ) ;
#90007=CARTESIAN_POINT ( 'NONE',  ( 10.66803740613750051, 1475.468785709809936, 268.4528686381480043 ) ) ;
#90008=CARTESIAN_POINT ( 'NONE',  ( -1.587029028349338455, 1467.007754443978001, 235.3619703211468561 ) ) ;
#90011=ORIENTED_EDGE ( 'NONE', *, *, #30425, .T. ) ;
#90012=CARTESIAN_POINT ( 'NONE',  ( -33.91369107994319876, 1451.728768198530133, 135.3761648363289964 ) ) ;
#90013=CARTESIAN_POINT ( 'NONE',  ( -22.96340384543530178, 1450.270798277949325, 217.9471854896650882 ) ) ;
#90016=CARTESIAN_POINT ( 'NONE',  ( 24.63819526104030189, 1451.813975265550198, 137.3334418279220017 ) ) ;
#90017=CARTESIAN_POINT ( 'NONE',  ( 13.45946769660000086, 1415.628674266529742, 196.7502466371980177 ) ) ;
#90019=CARTESIAN_POINT ( 'NONE',  ( 21.64785686290000299, 1411.027693062930211, 201.8270548794779984 ) ) ;
#90023=CARTESIAN_POINT ( 'NONE',  ( 24.53302258951347525, 1443.964919931875556, 213.3614358596423983 ) ) ;
#90024=CARTESIAN_POINT ( 'NONE',  ( 2.500000000000000000, 1439.621629183889809, 170.0481663565560098 ) ) ;
#90028=CARTESIAN_POINT ( 'NONE',  ( -3.196891731540000059, 1474.092834640029878, 270.1354749226979379 ) ) ;
#90030=CARTESIAN_POINT ( 'NONE',  ( -6.160533402158700156, 1422.363863605520010, 133.5162229238370060 ) ) ;
#90031=CARTESIAN_POINT ( 'NONE',  ( -37.03079991490060507, 1449.523054757250065, 136.2935849128809878 ) ) ;
#90032=CARTESIAN_POINT ( 'NONE',  ( 11.60004869885203682, 1426.073251783285741, 137.8255840559769183 ) ) ;
#90033=B_SPLINE_CURVE_WITH_KNOTS ( 'NONE', 3,
 ( #96190, #79944, #46365, #96752 ),
 .UNSPECIFIED., .F., .F.,
 ( 4, 4 ),
 ( -23.51228018140000131, -6.734755223260002310 ),
 .UNSPECIFIED. ) ;
#90034=CARTESIAN_POINT ( 'NONE',  ( 1.833592485732214783, 1416.810683918116865, 232.7762320029798389 ) ) ;
#90035=CARTESIAN_POINT ( 'NONE',  ( -2.500000000000000000, 1419.382839383030159, 144.1073686758980159 ) ) ;
#90037=CARTESIAN_POINT ( 'NONE',  ( 1.191993025707729934E-05, 1406.952180159080172, 222.1219960650689984 ) ) ;
#90038=CARTESIAN_POINT ( 'NONE',  ( 34.25124623592680706, 1440.913060384829805, 249.3947555928999975 ) ) ;
#90040=ORIENTED_EDGE ( 'NONE', *, *, #20547, .F. ) ;
#90042=B_SPLINE_CURVE_WITH_KNOTS ( 'NONE', 5,
 ( #33440, #40208, #24490, #109624, #40759, #84418 ),
 .UNSPECIFIED., .F., .F.,
 ( 6, 6 ),
 ( 0.000000000000000000, 1.000000000000000000 ),
 .UNSPECIFIED. ) ;
#90043=CARTESIAN_POINT ( 'NONE',  ( 12.37499353609999986, 1442.762691980110048, 150.7815459944920065 ) ) ;
#90045=CARTESIAN_POINT ( 'NONE',  ( -1.330041464690565611, 1409.969616266280809, 185.6431087925785164 ) ) ;
#90046=CARTESIAN_POINT ( 'NONE',  ( 1.705087066220000169, 1507.082462650630077, 236.5153987699980007 ) ) ;
#90048=CARTESIAN_POINT ( 'NONE',  ( -5.496544701782279496, 1440.579441524449976, 154.7743156926269705 ) ) ;
#90051=CARTESIAN_POINT ( 'NONE',  ( 23.21626404799999932, 1452.102330582029936, 139.5326100675980001 ) ) ;
#90053=CARTESIAN_POINT ( 'NONE',  ( 1.420260064800000110, 1466.712984990630048, 235.0376563120979938 ) ) ;
#90056=CARTESIAN_POINT ( 'NONE',  ( -0.6686366138079999910, 1452.253038997929934, 183.3051521255979992 ) ) ;
#90066=CARTESIAN_POINT ( 'NONE',  ( 35.97546153048689632, 1437.423085270620049, 136.5373550775509841 ) ) ;
#90070=DIRECTION ( 'NONE',  ( -0.6906235816661248084, 0.2466512791670449067, 0.6798545542481227999 ) ) ;
#90071=CARTESIAN_POINT ( 'NONE',  ( 21.39771952614790251, 1509.704955107219803, 188.4542851670070149 ) ) ;
#90072=CYLINDRICAL_SURFACE ( 'NONE', #86097, 1.638701816490922836 ) ;
#90073=CARTESIAN_POINT ( 'NONE',  ( 18.29046601820000006, 1425.439462508929864, 225.0338555594980221 ) ) ;
#90075=CARTESIAN_POINT ( 'NONE',  ( -19.45301492749999994, 1470.713061780830230, 191.6830327524980078 ) ) ;
#90078=CARTESIAN_POINT ( 'NONE',  ( -2.928230722141350384, 1449.385141265240009, 184.4057003796210097 ) ) ;
#90084=B_SPLINE_CURVE_WITH_KNOTS ( 'NONE', 3,
 ( #87274, #102942, #1631, #8889, #94005, #43070, #35767, #35208, #79433, #43623 ),
 .UNSPECIFIED., .F., .F.,
 ( 4, 2, 2, 2, 4 ),
 ( -0.1037542911854470035, -0.07904524408052189532, -0.05440765139039069331, -0.02871539828174819731, -5.298799732322834188E-10 ),
 .UNSPECIFIED. ) ;
#90085=CARTESIAN_POINT ( 'NONE',  ( -3.261635522710140146E-10, 1469.285592605210240, 252.0667581022420052 ) ) ;
#90086=CARTESIAN_POINT ( 'NONE',  ( -20.05210432756090100, 1490.118056226199997, 190.9036615977489930 ) ) ;
#90089=CARTESIAN_POINT ( 'NONE',  ( -1.467496020479999830, 1486.532142015430054, 182.3879484836979827 ) ) ;
#90091=CARTESIAN_POINT ( 'NONE',  ( -46.02995229330920068, 1440.913068804449949, 268.4959856126969839 ) ) ;
#90093=CARTESIAN_POINT ( 'NONE',  ( 14.13195592840999915, 1452.421092199690065, 222.7290593210850034 ) ) ;
#90096=CARTESIAN_POINT ( 'NONE',  ( 3.985678545446159848, 1408.516722457220112, 222.1641616639979873 ) ) ;
#90097=CARTESIAN_POINT ( 'NONE',  ( -13.34678598724409859, 1434.913712705049875, 149.0316152958799876 ) ) ;
#90100=CARTESIAN_POINT ( 'NONE',  ( 3.134082760970000159, 1421.411057458130017, 144.1516174827979739 ) ) ;
#90102=EDGE_LOOP ( 'NONE', ( #102216, #84433, #107220, #82124, #42231 ) ) ;
#90103=CARTESIAN_POINT ( 'NONE',  ( 5.442004251710000240, 1413.088571896030089, 250.5651368636980294 ) ) ;
#90105=CARTESIAN_POINT ( 'NONE',  ( 1.530048329109999994, 1452.704402376130020, 183.4894930016980084 ) ) ;
#90106=CARTESIAN_POINT ( 'NONE',  ( -17.54329334670000051, 1410.021607005030091, 194.9097843735980007 ) ) ;
#90108=CARTESIAN_POINT ( 'NONE',  ( -28.62989887450860138, 1415.197388761415141, 269.9536704965778426 ) ) ;
#90109=CARTESIAN_POINT ( 'NONE',  ( -16.58223822780000134, 1424.948544771930074, 220.7841459318979958 ) ) ;
#90111=CARTESIAN_POINT ( 'NONE',  ( -6.452039925207460946, 1452.687750188360042, 151.7627216464220226 ) ) ;
#90112=CARTESIAN_POINT ( 'NONE',  ( 28.25319066630000009, 1451.926638454029899, 134.8820817050979883 ) ) ;
#90113=VERTEX_POINT ( 'NONE', #64469 ) ;
#90114=CARTESIAN_POINT ( 'NONE',  ( -0.04898430503675949704, 1396.985968514940168, 196.3070536892440145 ) ) ;
#90116=CARTESIAN_POINT ( 'NONE',  ( -0.04569930594200000140, 1508.911464532430273, 238.4016181626980142 ) ) ;
#90120=CARTESIAN_POINT ( 'NONE',  ( -24.02848715508979893, 1410.733037965189851, 208.6273024917730083 ) ) ;
#90121=B_SPLINE_CURVE_WITH_KNOTS ( 'NONE', 3,
 ( #91577, #92123, #7565, #85358, #50143, #102165 ),
 .UNSPECIFIED., .F., .F.,
 ( 4, 2, 4 ),
 ( 0.000000000000000000, 0.01392848930680899884, 0.02784760531277210086 ),
 .UNSPECIFIED. ) ;
#90125=CARTESIAN_POINT ( 'NONE',  ( -7.332328763730000531, 1479.766960287329994, 234.2465134582980113 ) ) ;
#90126=DIRECTION ( 'NONE',  ( -1.962483594669999970E-13, -8.350994019880001345E-15, 1.000000000000000000 ) ) ;
#90127=ORIENTED_EDGE ( 'NONE', *, *, #97559, .F. ) ;
#90128=CARTESIAN_POINT ( 'NONE',  ( 10.81518740880000173, 1424.921099675630103, 144.1705347732979874 ) ) ;
#90129=CARTESIAN_POINT ( 'NONE',  ( -12.57270521884790071, 1416.218865267220053, 221.9821426913590017 ) ) ;
#90134=CARTESIAN_POINT ( 'NONE',  ( 13.25261745213164843, 1443.177766318758358, 187.6357070691568936 ) ) ;
#90140=CARTESIAN_POINT ( 'NONE',  ( -4.271147774425892329, 1424.301298031622082, 185.4449705293434931 ) ) ;
#90141=CARTESIAN_POINT ( 'NONE',  ( -4.550427519660000364, 1425.535076783930208, 186.2088322612979994 ) ) ;
#90142=CARTESIAN_POINT ( 'NONE',  ( -1.709436532471480112E-05, 1408.236684775530193, 270.3925729408980487 ) ) ;
#90145=CARTESIAN_POINT ( 'NONE',  ( -19.21356996290061758, 1509.590333268685981, 231.5036793335008838 ) ) ;
#90147=CARTESIAN_POINT ( 'NONE',  ( 0.03685098609671132869, 1409.759219108942716, 233.0924633182313812 ) ) ;
#90151=CARTESIAN_POINT ( 'NONE',  ( -25.13357330590289962, 1509.659395417869973, 222.8360384651579693 ) ) ;
#90152=CARTESIAN_POINT ( 'NONE',  ( 11.58690141939999840, 1425.690684998030292, 133.5558073867980227 ) ) ;
#90153=ORIENTED_EDGE ( 'NONE', *, *, #69962, .F. ) ;
#90154=CARTESIAN_POINT ( 'NONE',  ( 3.114882401830000092, 1426.979439823129951, 214.3676144192479853 ) ) ;
#90156=DIRECTION ( 'NONE',  ( 0.000000000000000000, 0.000000000000000000, -1.000000000000000000 ) ) ;
#90158=B_SPLINE_SURFACE_WITH_KNOTS ( 'NONE', 2, 5, ( 
 ( #63988, #88080, #2438, #46082, #4609, #62340 ),
 ( #88628, #12448, #98098, #55032, #45539, #79679 ),
 ( #29255, #21371, #105417, #44981, #20286, #61787 ) ),
 .UNSPECIFIED., .F., .F., .F.,
 ( 3, 3 ),
 ( 6, 6 ),
 ( 1.399803019409999960, 2.016961153140000018 ),
 ( 0.000000000000000000, 1.000000000000000000 ),
 .UNSPECIFIED. ) ;
#90164=CARTESIAN_POINT ( 'NONE',  ( -0.8217888514169999770, 1435.943783413959864, 150.5249316333980119 ) ) ;
#90166=CARTESIAN_POINT ( 'NONE',  ( 11.93572966800000046, 1433.501285843680080, 150.1252694811980177 ) ) ;
#90168=CARTESIAN_POINT ( 'NONE',  ( 12.98785519611789852, 1415.943166310999914, 196.5430628610019994 ) ) ;
#90171=CARTESIAN_POINT ( 'NONE',  ( 5.943213857399999966, 1419.755023743430002, 231.5246200396979930 ) ) ;
#90175=CARTESIAN_POINT ( 'NONE',  ( -18.22459200680000180, 1409.714306415329929, 223.2691318219980019 ) ) ;
#90176=CARTESIAN_POINT ( 'NONE',  ( 14.55375838210000161, 1435.825272921289979, 149.7847056613980214 ) ) ;
#90178=CARTESIAN_POINT ( 'NONE',  ( 37.65047687761219919, 1442.773887286080026, 137.1096749932030150 ) ) ;
#90179=CARTESIAN_POINT ( 'NONE',  ( 18.80339027203730140, 1425.953307585449693, 225.0197318394450008 ) ) ;
#90182=CARTESIAN_POINT ( 'NONE',  ( -39.82448890266579866, 1438.723056497909965, 136.0668919366270018 ) ) ;
#90183=CARTESIAN_POINT ( 'NONE',  ( -3.236789229669999823, 1414.913060387329779, 225.4509929012980081 ) ) ;
#90184=CARTESIAN_POINT ( 'NONE',  ( 0.2157156553116409969, 1454.149060955749974, 183.2041011444529772 ) ) ;
#90185=CARTESIAN_POINT ( 'NONE',  ( -11.92059014628319957, 1407.699961494269928, 215.8293613729719880 ) ) ;
#90186=CARTESIAN_POINT ( 'NONE',  ( 0.05678182167189999713, 1418.511462927230014, 184.6660934127980340 ) ) ;
#90189=CARTESIAN_POINT ( 'NONE',  ( 13.19858043940000059, 1434.900412407629801, 149.0260047559980023 ) ) ;
#90190=CARTESIAN_POINT ( 'NONE',  ( -36.31760351699959699, 1436.138747409269854, 134.0999999970809995 ) ) ;
#90191=CARTESIAN_POINT ( 'NONE',  ( 9.343523557230000165, 1442.321883629180093, 184.6435794382980191 ) ) ;
#90195=CARTESIAN_POINT ( 'NONE',  ( 40.22845519509999690, 1442.699277658399978, 137.0102247757980081 ) ) ;
#90198=CARTESIAN_POINT ( 'NONE',  ( 14.39191247257890183, 1509.401575546390177, 234.0412317446419763 ) ) ;
#90199=CARTESIAN_POINT ( 'NONE',  ( 11.43304550802769626, 1407.789912946944924, 269.6098866619304317 ) ) ;
#90206=CARTESIAN_POINT ( 'NONE',  ( -27.28054590290000192, 1451.100206374529989, 136.3683869527979766 ) ) ;
#90207=LINE ( 'NONE', #4040, #49969 ) ;
#90208=CARTESIAN_POINT ( 'NONE',  ( -17.02125645528619913, 1410.875184141109912, 226.2353266115079862 ) ) ;
#90210=CARTESIAN_POINT ( 'NONE',  ( 0.5088547212972790446, 1411.680041637540171, 185.0134109359660215 ) ) ;
#90216=CARTESIAN_POINT ( 'NONE',  ( -0.2866861870901689646, 1419.027722853580144, 184.6389722060440022 ) ) ;
#90217=CARTESIAN_POINT ( 'NONE',  ( 0.003562172589289999778, 1467.142144095830190, 235.6416276042979803 ) ) ;
#90219=CARTESIAN_POINT ( 'NONE',  ( 19.99392930349999986, 1409.775846518530216, 218.9826064745180076 ) ) ;
#90220=CARTESIAN_POINT ( 'NONE',  ( -1.798624549303609932, 1414.921120847540124, 185.8456817132880019 ) ) ;
#90222=CARTESIAN_POINT ( 'NONE',  ( -17.54372176839999753, 1423.780072466529873, 226.6776802473979728 ) ) ;
#90223=LINE ( 'NONE', #49901, #33549 ) ;
#90229=VECTOR ( 'NONE', #27230, 1000.000000000000000 ) ;
#90232=CARTESIAN_POINT ( 'NONE',  ( -17.86706492440000105, 1424.552609962230008, 227.1966067826979838 ) ) ;
#90235=LINE ( 'NONE', #47706, #70975 ) ;
#90236=CARTESIAN_POINT ( 'NONE',  ( -4.258475691689660003, 1441.254861102220048, 159.6897597212040125 ) ) ;
#90240=ORIENTED_EDGE ( 'NONE', *, *, #19298, .F. ) ;
#90242=ORIENTED_EDGE ( 'NONE', *, *, #99080, .T. ) ;
#90245=( BOUNDED_SURFACE ( )  B_SPLINE_SURFACE ( 3, 2, ( 
 ( #75219, #39946, #55673 ),
 ( #74118, #41041, #109370 ),
 ( #47252, #21464, #89794 ),
 ( #103137, #52225, #51663 ),
 ( #75760, #24226, #84143 ),
 ( #110456, #66825, #7442 ) ),
 .UNSPECIFIED., .F., .F., .F. ) 
 B_SPLINE_SURFACE_WITH_KNOTS ( ( 4, 2, 4 ),
 ( 3, 3 ),
 ( -1.896842529429832586E-07, 0.001072165293717367192, 0.002144520271687677150 ),
 ( 0.000000000000000000, 0.3183217140536988010 ),
 .UNSPECIFIED. ) 
 GEOMETRIC_REPRESENTATION_ITEM ( )  RATIONAL_B_SPLINE_SURFACE ( (
 ( 1.000000000000000000, 0.9047634226006637803, 0.8701585863180565372),
 ( 1.000000000000000000, 0.9047376462424103760, 0.8701234439506322360),
 ( 1.000000000000000000, 0.9047290734635364817, 0.8701117561962150582),
 ( 1.000000000000000000, 0.9047473679512488820, 0.8701366981062672590),
 ( 1.000000000000000000, 0.9047738115176444662, 0.8701727501162970224),
 ( 1.000000000000000000, 0.9048167665816072569, 0.8702313131850467620) ) ) 
 REPRESENTATION_ITEM ( '' )  SURFACE ( )  );
#90246=CARTESIAN_POINT ( 'NONE',  ( -11.73701142390000030, 1426.696005485330033, 144.1689090389980095 ) ) ;
#90247=CARTESIAN_POINT ( 'NONE',  ( 0.5363933160299999559, 1508.586927071130049, 180.3878905387979898 ) ) ;
#90250=CARTESIAN_POINT ( 'NONE',  ( -25.21718682590210037, 1450.979587312889862, 137.5960344802909958 ) ) ;
#90252=CARTESIAN_POINT ( 'NONE',  ( 13.94439657179999870, 1410.332512878529997, 228.0517289727980312 ) ) ;
#90255=CARTESIAN_POINT ( 'NONE',  ( 41.40218316853920300, 1445.741963847480065, 134.0999999985380100 ) ) ;
#90256=CARTESIAN_POINT ( 'NONE',  ( -40.24748973017329945, 1443.039696951350152, 137.0497123184690054 ) ) ;
#90262=CARTESIAN_POINT ( 'NONE',  ( 13.35890006641605865, 1410.752511746112077, 228.3639459599291968 ) ) ;
#90263=CARTESIAN_POINT ( 'NONE',  ( 31.06561166658629958, 1445.948172529730073, 137.1228041004679881 ) ) ;
#90264=CARTESIAN_POINT ( 'NONE',  ( -0.005696459569060000581, 1451.697357073530156, 183.0329412725980092 ) ) ;
#90265=CARTESIAN_POINT ( 'NONE',  ( -3.258850095529999713, 1485.815288458330087, 182.5815364463979904 ) ) ;
#90266=CARTESIAN_POINT ( 'NONE',  ( 12.24860663770000002, 1442.680101602390096, 186.9125332272980131 ) ) ;
#90270=FACE_OUTER_BOUND ( 'NONE', #34084, .T. ) ;
#90271=CARTESIAN_POINT ( 'NONE',  ( 10.59708812170000058, 1416.824060884929850, 194.4803559377980093 ) ) ;
#90274=( BOUNDED_CURVE ( )  B_SPLINE_CURVE ( 3, ( #69825, #96092, #79309, #61422 ),
 .UNSPECIFIED., .F., .T. ) 
 B_SPLINE_CURVE_WITH_KNOTS ( ( 4, 4 ),
 ( 1.036126831488924926, 2.105455280819345631 ),
 .UNSPECIFIED. ) 
 CURVE ( )  GEOMETRIC_REPRESENTATION_ITEM ( )  RATIONAL_B_SPLINE_CURVE ( ( 1.000000000000000000, 0.9069598485478114203, 0.9069598485478114203, 1.000000000000000000 ) ) 
 REPRESENTATION_ITEM ( '' )  );
#90278=CARTESIAN_POINT ( 'NONE',  ( 35.20572477793839994, 1440.913060387330006, 261.1485995943819489 ) ) ;
#90279=CARTESIAN_POINT ( 'NONE',  ( 19.65855403599999818, 1477.370641617730143, 227.1408115753980042 ) ) ;
#90281=CARTESIAN_POINT ( 'NONE',  ( -0.03743758868163819808, 1451.696053065270007, 183.0324010646019985 ) ) ;
#90282=CARTESIAN_POINT ( 'NONE',  ( -15.74506077599999898, 1409.964630928229781, 191.4165501260980022 ) ) ;
#90283=DIRECTION ( 'NONE',  ( 0.3363363969979660806, -0.9417419115949053898, 0.000000000000000000 ) ) ;
#90284=CIRCLE ( 'NONE', #67133, 2.000000002117825915 ) ;
#90288=CARTESIAN_POINT ( 'NONE',  ( 0.7748160517030000527, 1405.993929547030120, 266.9609161638979913 ) ) ;
#90291=CARTESIAN_POINT ( 'NONE',  ( 12.09637707030000087, 1463.380942464329792, 231.4947967239980073 ) ) ;
#90292=CARTESIAN_POINT ( 'NONE',  ( -10.33597699569439676, 1423.067771114430570, 137.1941345535399535 ) ) ;
#90293=B_SPLINE_SURFACE_WITH_KNOTS ( 'NONE', 5, 5, ( 
 ( #105407, #97015, #4064, #36542, #11358, #70741 ),
 ( #28140, #104300, #63436, #19735, #89150, #97554 ),
 ( #28699, #71852, #38189, #27589, #53936, #72371 ),
 ( #62905, #62331, #11898, #45528, #44409, #79669 ),
 ( #46624, #95350, #46072, #106501, #18610, #36000 ),
 ( #20277, #79118, #20827, #2974, #88617, #10800 ),
 ( #37092, #71294, #55023, #54481, #80205, #3521 ),
 ( #96455, #70191, #37646, #88070, #61235, #105968 ),
 ( #29246, #44971, #12436, #52810, #86942, #10232 ),
 ( #78549, #1866, #61774, #95898, #19159, #87511 ),
 ( #2426, #29789, #100299, #57225, #65617, #23583 ),
 ( #39292, #6779, #99176, #47157, #13516, #81283 ),
 ( #21906, #31991, #4599, #38733, #82944, #57773 ),
 ( #6234, #72909, #55568, #74564, #49355, #12974 ),
 ( #74011, #108143, #81833, #73466, #75118, #15167 ),
 ( #83484, #40387, #40941, #91892, #91354, #107048 ),
 ( #64524, #108699, #98090, #30882, #63976, #21361 ),
 ( #31436, #99730, #89693, #5138, #90792, #107599 ) ),
 .UNSPECIFIED., .F., .F., .F.,
 ( 6, 3, 3, 3, 3, 6 ),
 ( 6, 6 ),
 ( 3.688330952486170045, 6.839513527549999417, 10.63598301710000094, 15.04879579270000001, 24.05445287550000089, 33.17986963567380343 ),
 ( -0.001310986273832020089, 2.000000000000000000 ),
 .UNSPECIFIED. ) ;
#90295=CARTESIAN_POINT ( 'NONE',  ( 22.51756156282889876, 1509.699390964210124, 227.9212218486820234 ) ) ;
#90297=CARTESIAN_POINT ( 'NONE',  ( 18.91907327681788686, 1444.756048487146472, 214.3158972188605844 ) ) ;
#90301=CARTESIAN_POINT ( 'NONE',  ( -10.10004869884733125, 1422.222932908416851, 137.0999999980979851 ) ) ;
#90303=ORIENTED_EDGE ( 'NONE', *, *, #87792, .T. ) ;
#90305=CARTESIAN_POINT ( 'NONE',  ( 20.03600803810000031, 1452.959368570329843, 217.4640555505980046 ) ) ;
#90307=CARTESIAN_POINT ( 'NONE',  ( -11.56636936299999974, 1431.560971557430094, 151.1549291175980159 ) ) ;
#90309=EDGE_CURVE ( 'NONE', #85990, #5142, #59369, .T. ) ;
#90311=CARTESIAN_POINT ( 'NONE',  ( 2.668886676840000138, 1414.538856421429955, 231.8535933046979949 ) ) ;
#90313=CARTESIAN_POINT ( 'NONE',  ( 12.20364748979999980, 1447.059433187239847, 188.0531537431980098 ) ) ;
#90314=CARTESIAN_POINT ( 'NONE',  ( -25.19387440899999930, 1470.081153789430118, 211.8647355342179992 ) ) ;
#90315=CARTESIAN_POINT ( 'NONE',  ( 19.08819056019999749, 1456.247773388830183, 225.9807996138980002 ) ) ;
#90316=CARTESIAN_POINT ( 'NONE',  ( -1.948797609489999916, 1485.180374433429961, 182.7287261531979823 ) ) ;
#90317=ORIENTED_EDGE ( 'NONE', *, *, #94887, .F. ) ;
#90319=CARTESIAN_POINT ( 'NONE',  ( 7.084264032569999259, 1406.157124000829981, 267.5158752688980144 ) ) ;
#90321=CARTESIAN_POINT ( 'NONE',  ( 18.87778356449999961, 1410.875542549930287, 195.0395779401980292 ) ) ;
#90322=CARTESIAN_POINT ( 'NONE',  ( 21.04721947777625246, 1428.203262266114280, 219.7000736795839657 ) ) ;
#90325=CARTESIAN_POINT ( 'NONE',  ( 11.60004869885203682, 1424.304602974221552, 137.2803358174371056 ) ) ;
#90327=CARTESIAN_POINT ( 'NONE',  ( -1.181727161079999977, 1450.812795825409921, 155.6080925169979707 ) ) ;
#90328=CARTESIAN_POINT ( 'NONE',  ( -1.591694425982771888, 1451.443140916882612, 183.9247936146681752 ) ) ;
#90329=CARTESIAN_POINT ( 'NONE',  ( 2.500000000000000000, 1448.894380896710118, 155.6080914321979947 ) ) ;
#90330=CARTESIAN_POINT ( 'NONE',  ( -14.25441464927300039, 1415.890045859280008, 221.1831556969420092 ) ) ;
#90331=CARTESIAN_POINT ( 'NONE',  ( 25.91590772989999891, 1441.261220175949802, 138.4451201509980365 ) ) ;
#90332=CARTESIAN_POINT ( 'NONE',  ( -6.092217317660000298, 1412.362567936729874, 265.6112251771979800 ) ) ;
#90334=CARTESIAN_POINT ( 'NONE',  ( 4.242727252399999927, 1441.427684323080030, 162.1744802195979958 ) ) ;
#90335=CARTESIAN_POINT ( 'NONE',  ( -6.205475772959999858, 1475.744157773729967, 268.4675638380979876 ) ) ;
#90341=CARTESIAN_POINT ( 'NONE',  ( 12.26778636213749962, 1416.765224586259819, 223.5774076447450227 ) ) ;
#90346=CARTESIAN_POINT ( 'NONE',  ( -20.46201241340000010, 1410.988590480530092, 198.9701274117980176 ) ) ;
#90348=CARTESIAN_POINT ( 'NONE',  ( 19.52361536739011427, 1455.536307519420234, 225.7780045410000582 ) ) ;
#90351=CARTESIAN_POINT ( 'NONE',  ( -4.049338806867527119, 1410.430873130929967, 232.1965388422846388 ) ) ;
#90353=AXIS2_PLACEMENT_3D ( 'NONE', #63738, #12198, #98409 ) ;
#90355=CARTESIAN_POINT ( 'NONE',  ( 11.70462718329999952, 1426.716940587629779, 141.8502512716979993 ) ) ;
#90357=CARTESIAN_POINT ( 'NONE',  ( 2.500000000000000000, 1425.929641636930000, 172.2701767017979932 ) ) ;
#90362=CARTESIAN_POINT ( 'NONE',  ( 4.090276254750000007, 1507.742068723129933, 181.5992713909979841 ) ) ;
#90368=ORIENTED_EDGE ( 'NONE', *, *, #32715, .F. ) ;
#90369=CARTESIAN_POINT ( 'NONE',  ( -5.492330872600000191, 1396.104856807829947, 199.1956357395080204 ) ) ;
#90370=CARTESIAN_POINT ( 'NONE',  ( -19.72217329349999915, 1410.523787867230112, 221.4680334561980146 ) ) ;
#90371=CARTESIAN_POINT ( 'NONE',  ( 1.400808531280000047, 1507.374882240629859, 236.8304372384980070 ) ) ;
#90372=CARTESIAN_POINT ( 'NONE',  ( -13.46505473512351081, 1444.253858681032625, 169.3609527546826712 ) ) ;
#90376=CARTESIAN_POINT ( 'NONE',  ( 17.50240768599999797, 1410.866981087730210, 225.6197211887979961 ) ) ;
#90378=CARTESIAN_POINT ( 'NONE',  ( -10.06907521269999961, 1416.520322350429979, 193.4677121538979918 ) ) ;
#90379=CARTESIAN_POINT ( 'NONE',  ( -40.60083016280549373, 1447.775073852730202, 135.1193631031219979 ) ) ;
#90380=CARTESIAN_POINT ( 'NONE',  ( 10.25097305582739970, 1396.271032255460113, 213.2864649067509788 ) ) ;
#90381=CARTESIAN_POINT ( 'NONE',  ( 0.9088213736110000163, 1416.535385209229844, 190.2286903860979805 ) ) ;
#90382=CARTESIAN_POINT ( 'NONE',  ( 11.26739317570000054, 1429.793092966730001, 151.0732202328979952 ) ) ;
#90384=EDGE_LOOP ( 'NONE', ( #45717, #17900, #57426, #3257 ) ) ;
#90389=EDGE_CURVE ( 'NONE', #70841, #8770, #17304, .T. ) ;
#90390=CARTESIAN_POINT ( 'NONE',  ( -19.35824286299009955, 1488.013120477789926, 228.5799778352339899 ) ) ;
#90391=CARTESIAN_POINT ( 'NONE',  ( -15.31141905560000005, 1459.632573421429925, 229.9709746414979747 ) ) ;
#90400=B_SPLINE_CURVE_WITH_KNOTS ( 'NONE', 3,
 ( #60982, #69380, #1615, #18372, #26793, #69938, #36298, #95106, #103489, #29015, #52567, #27903, #79419, #62086, #45280, #71609, #88364, #54238, #62651, #86700, #37410, #11654, #2730, #86150, #104052, #36852, #53690, #63200, #95657, #9994, #78877, #20577, #27343, #18924, #97307, #43607 ),
 .UNSPECIFIED., .F., .F.,
 ( 4, 2, 2, 1, 1, 1, 2, 2, 2, 2, 1, 1, 2, 2, 2, 2, 1, 1, 1, 2, 2, 4 ),
 ( 0.1904315896942847253, 0.2916276409813860493, 0.3422256666249366974, 0.3675246794466333067, 0.3801741858573954302, 0.3864989390627698862, 0.3896613156655327481, 0.3928236922682955545, 0.4940197435555052641, 0.5446177691992000192, 0.5699167820210474522, 0.5825662884320258472, 0.5888910416374537604, 0.5952157948428816736, 0.6964118461295565332, 0.7470098717728940185, 0.7723088845945627057, 0.7849583910053672398, 0.7912831442107969293, 0.7944455208135379198, 0.7976078974162790214, 1.000000000000000000 ),
 .UNSPECIFIED. ) ;
#90402=CARTESIAN_POINT ( 'NONE',  ( 17.27338612379999816, 1414.913060387329779, 210.1977510952380044 ) ) ;
#90408=CARTESIAN_POINT ( 'NONE',  ( -39.14106390295368243, 1429.794342911720378, 269.5953431606081949 ) ) ;
#90409=CARTESIAN_POINT ( 'NONE',  ( -0.7002101091710001279, 1408.937512263330063, 232.1050833052979954 ) ) ;
#90412=CARTESIAN_POINT ( 'NONE',  ( -0.01152932003563050117, 1451.938819355580108, 183.0054112925830054 ) ) ;
#90413=CARTESIAN_POINT ( 'NONE',  ( -31.61895657298340012, 1440.913060388849999, 243.1029565790050242 ) ) ;
#90415=CARTESIAN_POINT ( 'NONE',  ( -0.1062606726760350062, 1465.018637258840045, 237.3905034661050024 ) ) ;
#90416=CARTESIAN_POINT ( 'NONE',  ( 15.45910333959999861, 1409.623955960430067, 270.0849031534979758 ) ) ;
#90419=B_SPLINE_CURVE_WITH_KNOTS ( 'NONE', 3,
 ( #32067, #15245, #31507, #58384, #49437, #75736, #109880, #33160, #24736, #65687, #91432, #14708, #58933, #48897, #93065, #83024, #47775, #5214, #34819, #110426, #77386, #52196, #35938, #103110, #86325 ),
 .UNSPECIFIED., .F., .F.,
 ( 4, 3, 3, 3, 3, 3, 3, 3, 4 ),
 ( -1.000000000000000000, -0.8761102852806710306, -0.6239390062907779200, -0.3603953910640009806, -0.09086183696110827768, 0.1830679867661229032, 0.4571305125683509107, 0.7297053856717570230, 0.9999610272373291586 ),
 .UNSPECIFIED. ) ;
#90420=CARTESIAN_POINT ( 'NONE',  ( 22.82103900350000103, 1409.709957859030055, 209.1787568684370058 ) ) ;
#90427=EDGE_CURVE ( 'NONE', #76272, #102730, #45836, .T. ) ;
#90428=CARTESIAN_POINT ( 'NONE',  ( 0.1674519188599999930, 1419.793575726829886, 184.3767552697979966 ) ) ;
#90429=CARTESIAN_POINT ( 'NONE',  ( 6.061196268494501105, 1422.611301504031417, 137.0999999981671635 ) ) ;
#90430=ADVANCED_FACE ( 'NONE', ( #67761 ), #76694, .F. ) ;
#90432=ORIENTED_EDGE ( 'NONE', *, *, #15951, .F. ) ;
#90435=EDGE_CURVE ( 'NONE', #56546, #28026, #81900, .T. ) ;
#90436=CARTESIAN_POINT ( 'NONE',  ( 0.7436338729729999875, 1415.853947014629966, 233.3108650019980246 ) ) ;
#90438=VECTOR ( 'NONE', #25278, 1000.000000000000000 ) ;
#90446=CARTESIAN_POINT ( 'NONE',  ( 10.43242597914977665, 1423.400858002167979, 137.2800370846200337 ) ) ;
#90450=VERTEX_POINT ( 'NONE', #63247 ) ;
#90452=CARTESIAN_POINT ( 'NONE',  ( 20.34226454299999887, 1454.597587043530211, 225.1509561457980340 ) ) ;
#90457=CARTESIAN_POINT ( 'NONE',  ( 16.63417907921860106, 1421.797052956256721, 227.0536667165849849 ) ) ;
#90459=CARTESIAN_POINT ( 'NONE',  ( -2.499999995990000112, 1447.656584094229856, 165.9523979493980050 ) ) ;
#90460=CARTESIAN_POINT ( 'NONE',  ( -20.07368861760000200, 1427.190829891029807, 224.4645657875979907 ) ) ;
#90463=CARTESIAN_POINT ( 'NONE',  ( 18.62849171730000108, 1498.094182759829891, 188.8234950878980101 ) ) ;
#90464=CARTESIAN_POINT ( 'NONE',  ( 0.2881515426530549817, 1409.862531727490023, 233.1990202907039986 ) ) ;
#90465=CARTESIAN_POINT ( 'NONE',  ( -18.52077958148023029, 1436.768619839807798, 212.6474277558114636 ) ) ;
#90466=EDGE_CURVE ( 'NONE', #57273, #6602, #97957, .T. ) ;
#90467=CARTESIAN_POINT ( 'NONE',  ( -35.00793662113747473, 1457.766281221113786, 269.5316643497311020 ) ) ;
#90472=EDGE_CURVE ( 'NONE', #86613, #3072, #70031, .T. ) ;
#90474=CARTESIAN_POINT ( 'NONE',  ( -15.28420222199999934, 1497.713060387329961, 224.4060481839979957 ) ) ;
#90475=CARTESIAN_POINT ( 'NONE',  ( 1.454962978634650073, 1500.859017483070147, 181.3861282941270190 ) ) ;
#90477=CARTESIAN_POINT ( 'NONE',  ( -12.91165256927668992, 1442.897813290883278, 186.4311288414393175 ) ) ;
#90478=CARTESIAN_POINT ( 'NONE',  ( 2.566893074593609807E-08, 1406.911841303630126, 196.1218459607310081 ) ) ;
#90479=DIRECTION ( 'NONE',  ( 0.000000000000000000, 1.000000000000000000, 0.000000000000000000 ) ) ;
#90480=ADVANCED_FACE ( 'NONE', ( #108513 ), #46611, .T. ) ;
#90481=DIRECTION ( 'NONE',  ( 0.000000000000000000, 1.000000000000000000, 0.000000000000000000 ) ) ;
#90484=CARTESIAN_POINT ( 'NONE',  ( 23.95468325570000090, 1435.352574582540001, 137.1777079961979950 ) ) ;
#90491=ORIENTED_EDGE ( 'NONE', *, *, #28433, .F. ) ;
#90494=CARTESIAN_POINT ( 'NONE',  ( 35.97184424755489829, 1425.113701170736931, 269.5449737053726267 ) ) ;
#90495=CARTESIAN_POINT ( 'NONE',  ( -32.03901054920000036, 1451.703008381130076, 250.0966427714979545 ) ) ;
#90496=CARTESIAN_POINT ( 'NONE',  ( -19.96856953369999843, 1506.518496045629945, 189.0102800763980042 ) ) ;
#90497=CARTESIAN_POINT ( 'NONE',  ( -11.23122559239999951, 1433.609634981740101, 151.5769196124979885 ) ) ;
#90498=CARTESIAN_POINT ( 'NONE',  ( 3.827327205999999649, 1422.542708386029972, 168.6405287067979941 ) ) ;
#90499=CARTESIAN_POINT ( 'NONE',  ( -19.39146514529999976, 1486.028937747929831, 189.8083660822979937 ) ) ;
#90500=CARTESIAN_POINT ( 'NONE',  ( -13.80543374319990058, 1434.979599778060219, 148.5369743065390082 ) ) ;
#90501=PLANE ( 'NONE',  #64320 ) ;
#90506=CARTESIAN_POINT ( 'NONE',  ( -11.01313281335095873, 1509.422798596149732, 237.0272438081198345 ) ) ;
#90509=CARTESIAN_POINT ( 'NONE',  ( 8.938783782526350941E-09, 1406.490650553919977, 266.0111486438349857 ) ) ;
#90510=VERTEX_POINT ( 'NONE', #83858 ) ;
#90515=CARTESIAN_POINT ( 'NONE',  ( -13.52613638759999937, 1472.406022870030029, 270.2585879644979627 ) ) ;
#90517=CARTESIAN_POINT ( 'NONE',  ( 3.229222591820000154, 1433.444289491620111, 155.4497426196979859 ) ) ;
#90518=CARTESIAN_POINT ( 'NONE',  ( 34.55890087717340009, 1451.246761928099886, 135.9292514245820200 ) ) ;
#90524=CARTESIAN_POINT ( 'NONE',  ( -29.10623605396180125, 1413.506399245979992, 268.1222045722540201 ) ) ;
#90528=ORIENTED_EDGE ( 'NONE', *, *, #71923, .T. ) ;
#90530=EDGE_CURVE ( 'NONE', #48829, #60488, #73993, .T. ) ;
#90531=CARTESIAN_POINT ( 'NONE',  ( 33.82133213608769751, 1444.740067931810017, 154.8032509060861912 ) ) ;
#90534=CARTESIAN_POINT ( 'NONE',  ( -6.133587857060000204, 1455.443851699130164, 185.1190063763980049 ) ) ;
#90535=CARTESIAN_POINT ( 'NONE',  ( -2.080511716054991744, 1450.122691195282641, 182.8668332015829208 ) ) ;
#90537=CARTESIAN_POINT ( 'NONE',  ( -26.28380303640000193, 1435.415400226489737, 135.3026382325979853 ) ) ;
#90540=DIRECTION ( 'NONE',  ( -0.7067635638050681068, 0.03085854333205623190, -0.7067764959171910499 ) ) ;
#90541=CARTESIAN_POINT ( 'NONE',  ( -12.94448954231350868, 1512.413060387330006, 185.4271167906579478 ) ) ;
#90542=CARTESIAN_POINT ( 'NONE',  ( -41.23699424981570161, 1431.252039966480197, 270.0532253150080351 ) ) ;
#90544=CARTESIAN_POINT ( 'NONE',  ( 0.07152419878080000515, 1397.597829884029807, 196.1220380877979892 ) ) ;
#90547=ORIENTED_EDGE ( 'NONE', *, *, #56189, .T. ) ;
#90549=CARTESIAN_POINT ( 'NONE',  ( 0.2777695833849999629, 1451.683731431829756, 183.0558775174980042 ) ) ;
#90552=CARTESIAN_POINT ( 'NONE',  ( -2.500000000000000000, 1419.383211070329935, 144.0964026338980091 ) ) ;
#90553=CARTESIAN_POINT ( 'NONE',  ( -0.03226023477341029982, 1410.297896964309984, 185.0217421575940193 ) ) ;
#90556=CARTESIAN_POINT ( 'NONE',  ( 2.746150429200790111, 1440.068830608010103, 157.5210337837320083 ) ) ;
#90558=CARTESIAN_POINT ( 'NONE',  ( 11.59504266670000128, 1415.140114704729967, 222.7749241790980079 ) ) ;
#90560=CARTESIAN_POINT ( 'NONE',  ( 12.09590736490000040, 1445.294669480289940, 186.8687466626980154 ) ) ;
#90562=ORIENTED_EDGE ( 'NONE', *, *, #15514, .T. ) ;
#90563=CARTESIAN_POINT ( 'NONE',  ( -40.71747596209480236, 1438.773003613870060, 135.0584847165220026 ) ) ;
#90564=CARTESIAN_POINT ( 'NONE',  ( -22.46490035622105452, 1451.676372061169559, 219.5715471896962185 ) ) ;
#90566=CARTESIAN_POINT ( 'NONE',  ( 6.714078785831339324, 1456.768705330869352, 227.7987839437156765 ) ) ;
#90567=EDGE_CURVE ( 'NONE', #94251, #24298, #64695, .T. ) ;
#90569=CARTESIAN_POINT ( 'NONE',  ( 13.35004134540000109, 1415.296882282229944, 197.1179729259980036 ) ) ;
#90571=CARTESIAN_POINT ( 'NONE',  ( 21.56891374070000111, 1409.666263453530291, 206.3502062819679850 ) ) ;
#90572=CARTESIAN_POINT ( 'NONE',  ( 16.66257059149999975, 1410.427173608229850, 226.4839827083980026 ) ) ;
#90575=CARTESIAN_POINT ( 'NONE',  ( 23.34191689203280973, 1449.544838690270126, 217.2362966351278430 ) ) ;
#90577=CARTESIAN_POINT ( 'NONE',  ( 2.500000000000039968, 1439.311174638779903, 160.3626073483409868 ) ) ;
#90582=CARTESIAN_POINT ( 'NONE',  ( -2.500000000000000000, 1448.919575512349866, 183.6707651433980004 ) ) ;
#90583=EDGE_CURVE ( 'NONE', #109869, #74855, #65861, .T. ) ;
#90584=ADVANCED_FACE ( 'NONE', ( #71527 ), #20616, .F. ) ;
#90589=CARTESIAN_POINT ( 'NONE',  ( 11.60004869885197110, 1426.057405506147461, 138.8677241012580907 ) ) ;
#90590=CYLINDRICAL_SURFACE ( 'NONE', #65743, 2.000000000000000000 ) ;
#90591=CARTESIAN_POINT ( 'NONE',  ( 17.80628076561068340, 1423.588752249659819, 226.0326016818666233 ) ) ;
#90594=CARTESIAN_POINT ( 'NONE',  ( 30.04265233421849857, 1440.913060385890049, 238.4851536875560214 ) ) ;
#90601=CARTESIAN_POINT ( 'NONE',  ( -19.09820918671905332, 1485.515190164787555, 189.6361271261989714 ) ) ;
#90606=CARTESIAN_POINT ( 'NONE',  ( 15.10371975099999986, 1409.440493903229935, 192.9533947891980006 ) ) ;
#90610=CARTESIAN_POINT ( 'NONE',  ( 5.360860135257599524, 1422.261831586439939, 143.3181667732210087 ) ) ;
#90612=CARTESIAN_POINT ( 'NONE',  ( 1.615419329660000125, 1466.293469222530121, 234.8241805934979993 ) ) ;
#90615=CARTESIAN_POINT ( 'NONE',  ( -0.3241128057579999999, 1452.022536283230238, 183.1062973747980038 ) ) ;
#90618=CARTESIAN_POINT ( 'NONE',  ( -17.57493253053520021, 1415.090956648730071, 208.0895966506530215 ) ) ;
#90625=CARTESIAN_POINT ( 'NONE',  ( -11.60004869885203860, 1426.752153102204375, 134.4009884339467931 ) ) ;
#90630=CARTESIAN_POINT ( 'NONE',  ( 18.28845792193000364, 1425.324260404669985, 225.4739065078200042 ) ) ;
#90633=CARTESIAN_POINT ( 'NONE',  ( -24.04659120089169733, 1444.796772349889807, 212.0316830080810178 ) ) ;
#90635=CARTESIAN_POINT ( 'NONE',  ( -4.161598017608739930, 1448.982982409190072, 185.0801973001829879 ) ) ;
#90639=CARTESIAN_POINT ( 'NONE',  ( 18.80348473439820012, 1458.103780993950068, 227.2192783789020041 ) ) ;
#90640=CARTESIAN_POINT ( 'NONE',  ( -12.47168581320000058, 1435.763300496210150, 150.9715321517980158 ) ) ;
#90641=CARTESIAN_POINT ( 'NONE',  ( 2.842584659965070124E-10, 1465.638316924609853, 240.1326368917110301 ) ) ;
#90642=CARTESIAN_POINT ( 'NONE',  ( -20.59684415639999955, 1507.762623716630060, 190.3921826403979765 ) ) ;
#90647=CARTESIAN_POINT ( 'NONE',  ( -45.87688764550289733, 1440.254748464500153, 266.4125321213890061 ) ) ;
#90652=CARTESIAN_POINT ( 'NONE',  ( 3.870734350961310355, 1407.691698232470117, 221.6993045718820099 ) ) ;
#90653=CARTESIAN_POINT ( 'NONE',  ( -13.12797199115260227, 1435.680278977339867, 150.5510888193360017 ) ) ;
#90656=CARTESIAN_POINT ( 'NONE',  ( 8.320723051859999941, 1424.406562835429895, 91.09139192869778867 ) ) ;
#90659=CARTESIAN_POINT ( 'NONE',  ( 24.64758684659999943, 1426.171069948330114, 240.2509105673979946 ) ) ;
#90660=CARTESIAN_POINT ( 'NONE',  ( -28.07142279760000037, 1508.133443487129853, 207.7742737906680190 ) ) ;
#90661=CARTESIAN_POINT ( 'NONE',  ( -3.541507727459999977, 1499.396715322330010, 181.3063315952979906 ) ) ;
#90663=CARTESIAN_POINT ( 'NONE',  ( 20.74431190377872269, 1506.539416727910066, 201.5807876387586077 ) ) ;
#90664=CARTESIAN_POINT ( 'NONE',  ( -4.374510219029999369, 1418.297051469029839, 231.7760247135979910 ) ) ;
#90665=CARTESIAN_POINT ( 'NONE',  ( 21.03036721537930376, 1456.985417876070187, 226.1578115872349883 ) ) ;
#90666=CARTESIAN_POINT ( 'NONE',  ( -7.429844844193369546, 1452.653604488170004, 151.4931312769679721 ) ) ;
#90667=CARTESIAN_POINT ( 'NONE',  ( -18.79678650740000023, 1416.830000968129980, 208.4086244650179935 ) ) ;
#90669=CARTESIAN_POINT ( 'NONE',  ( -5.359834938588759812, 1422.451238776880018, 146.6367341849590105 ) ) ;
#90671=CARTESIAN_POINT ( 'NONE',  ( 15.88607233163610211, 1422.777081491979970, 229.6788727262410248 ) ) ;
#90673=ORIENTED_EDGE ( 'NONE', *, *, #102049, .F. ) ;
#90674=ORIENTED_EDGE ( 'NONE', *, *, #66723, .F. ) ;
#90675=CARTESIAN_POINT ( 'NONE',  ( -10.36554740068187108, 1423.171634364120564, 137.2136980898112313 ) ) ;
#90676=CARTESIAN_POINT ( 'NONE',  ( -23.56284583309999903, 1410.013091502230054, 209.4388942478690012 ) ) ;
#90677=CARTESIAN_POINT ( 'NONE',  ( -3.775288954430000121, 1424.836333284029934, 185.8533989989979887 ) ) ;
#90681=CARTESIAN_POINT ( 'NONE',  ( -15.23964492230000012, 1498.344222354329986, 230.9699155403980058 ) ) ;
#90683=ORIENTED_EDGE ( 'NONE', *, *, #36631, .T. ) ;
#90684=CARTESIAN_POINT ( 'NONE',  ( 45.92877942503140076, 1443.730784468270031, 266.6808678471329586 ) ) ;
#90685=CARTESIAN_POINT ( 'NONE',  ( -12.50317167495700055, 1415.933499560010205, 221.8717862475229765 ) ) ;
#90686=CARTESIAN_POINT ( 'NONE',  ( -0.2148604818640000025, 1419.222391940929811, 184.6498075250980264 ) ) ;
#90690=CARTESIAN_POINT ( 'NONE',  ( 13.46741876155364359, 1443.580133104905826, 187.9916346024478457 ) ) ;
#90691=ORIENTED_EDGE ( 'NONE', *, *, #20066, .T. ) ;
#90692=VERTEX_POINT ( 'NONE', #30011 ) ;
#90697=CARTESIAN_POINT ( 'NONE',  ( 9.593413928111729660, 1452.578050990920019, 150.7562495203559934 ) ) ;
#90699=CARTESIAN_POINT ( 'NONE',  ( -1.664499176201119805E-05, 1409.781082070230013, 270.0713786264859664 ) ) ;
#90701=CARTESIAN_POINT ( 'NONE',  ( 19.07040306792730888, 1456.402085735674746, 225.8083803216468084 ) ) ;
#90702=CARTESIAN_POINT ( 'NONE',  ( -10.97972313751300177, 1432.951242176940013, 151.7695334411729959 ) ) ;
#90703=CARTESIAN_POINT ( 'NONE',  ( 0.03404606575480032676, 1410.028338985503296, 233.1847745296862513 ) ) ;
#90704=CARTESIAN_POINT ( 'NONE',  ( -2.198507585695390212E-07, 1408.626123741879837, 268.3915997536489613 ) ) ;
#90711=CARTESIAN_POINT ( 'NONE',  ( 11.79165762230000070, 1429.416862815430022, 146.4064176768980019 ) ) ;
#90713=CARTESIAN_POINT ( 'NONE',  ( 19.02913997119999934, 1436.609546585119915, 214.3676144198679765 ) ) ;
#90723=CARTESIAN_POINT ( 'NONE',  ( -0.8348477807080000312, 1443.913060387330006, 150.8032249175980155 ) ) ;
#90726=CARTESIAN_POINT ( 'NONE',  ( 11.49747572422220188, 1414.913060387329779, 220.3427040978150160 ) ) ;
#90727=CARTESIAN_POINT ( 'NONE',  ( 13.15726446870029953, 1414.972329067380088, 197.7171628163160051 ) ) ;
#90734=CARTESIAN_POINT ( 'NONE',  ( -17.32164063149999933, 1410.015194788730014, 225.5041473358979829 ) ) ;
#90736=EDGE_CURVE ( 'NONE', #41530, #75664, #84371, .T. ) ;
#90744=CARTESIAN_POINT ( 'NONE',  ( -8.886125802571559262, 1432.346591486940042, 153.1913712024140182 ) ) ;
#90746=CARTESIAN_POINT ( 'NONE',  ( -1.387158262170000045, 1415.426952351230057, 227.4696213630980139 ) ) ;
#90748=CARTESIAN_POINT ( 'NONE',  ( -13.32225628249999971, 1409.200806412430211, 203.4621145805880076 ) ) ;
#90749=CARTESIAN_POINT ( 'NONE',  ( -17.25136325379999747, 1416.823872462129884, 202.8337460093080153 ) ) ;
#90750=CARTESIAN_POINT ( 'NONE',  ( -28.49243283392089765, 1509.649079667319938, 211.1281934096199961 ) ) ;
#90751=CARTESIAN_POINT ( 'NONE',  ( 11.87541216019999979, 1433.006892857880075, 148.5014493308979979 ) ) ;
#90752=CARTESIAN_POINT ( 'NONE',  ( -28.14147886860000369, 1436.374928695000108, 136.6909279132979975 ) ) ;
#90756=CARTESIAN_POINT ( 'NONE',  ( -4.758677794462281341, 1427.076634120264089, 137.0999999980979567 ) ) ;
#90759=CARTESIAN_POINT ( 'NONE',  ( 21.97938480441199971, 1506.433683733499947, 208.7396655020440051 ) ) ;
#90760=CARTESIAN_POINT ( 'NONE',  ( 13.87299426750780107, 1509.389572371919940, 234.2955350557650149 ) ) ;
#90762=CARTESIAN_POINT ( 'NONE',  ( 40.50390548520631029, 1425.157017824941704, 269.1155397953845636 ) ) ;
#90765=CARTESIAN_POINT ( 'NONE',  ( 2.500000015409999943, 1439.638673630699941, 183.2818205602979731 ) ) ;
#90769=CARTESIAN_POINT ( 'NONE',  ( -27.52167012590000184, 1451.951932214330100, 134.9033768147980084 ) ) ;
#90770=CARTESIAN_POINT ( 'NONE',  ( -15.99309461030230040, 1409.852751965980133, 226.2723575830249843 ) ) ;
#90773=DIRECTION ( 'NONE',  ( 0.3363363926273127968, -0.9417419131558525391, -2.375999277009924068E-08 ) ) ;
#90777=CARTESIAN_POINT ( 'NONE',  ( -0.1321314129836040074, 1420.447759805389978, 182.9787002574440180 ) ) ;
#90778=CARTESIAN_POINT ( 'NONE',  ( 1.010913760600000044, 1465.039206930530099, 236.8418874943980086 ) ) ;
#90779=CARTESIAN_POINT ( 'NONE',  ( 23.03460887469999818, 1411.077649166529909, 213.3831903349580159 ) ) ;
#90782=CARTESIAN_POINT ( 'NONE',  ( -17.64330431710000013, 1423.732166419529904, 226.4225726569979997 ) ) ;
#90785=CARTESIAN_POINT ( 'NONE',  ( 26.64849719969200237, 1469.324131025480028, 209.0880383046890074 ) ) ;
#90788=CARTESIAN_POINT ( 'NONE',  ( -23.42267346790000104, 1430.824238628630155, 212.0368849710979759 ) ) ;
#90792=CARTESIAN_POINT ( 'NONE',  ( -3.324249965575039933, 1484.702398424410148, 183.3514200912059664 ) ) ;
#90795=CARTESIAN_POINT ( 'NONE',  ( -4.222047166393189777, 1441.600308170239941, 167.9930962660010039 ) ) ;
#90798=ORIENTED_EDGE ( 'NONE', *, *, #68643, .T. ) ;
#90800=CARTESIAN_POINT ( 'NONE',  ( -17.31663237150539558, 1423.877172976356860, 228.8047162730268838 ) ) ;
#90803=CARTESIAN_POINT ( 'NONE',  ( 7.817147020270110325, 1507.298329231454545, 182.8873992028549651 ) ) ;
#90805=CARTESIAN_POINT ( 'NONE',  ( -11.74384639166921218, 1426.275853339841206, 144.6945198498246725 ) ) ;
#90806=CARTESIAN_POINT ( 'NONE',  ( 16.06732615789859508, 1409.482374878060000, 192.8457122857769832 ) ) ;
#90808=CARTESIAN_POINT ( 'NONE',  ( 33.92724809123075858, 1436.576393223097966, 136.5094752661439657 ) ) ;
#90812=CARTESIAN_POINT ( 'NONE',  ( 38.37377460181989619, 1450.184294006789969, 134.0999999983419855 ) ) ;
#90817=ORIENTED_EDGE ( 'NONE', *, *, #13025, .F. ) ;
#90821=CARTESIAN_POINT ( 'NONE',  ( -0.03576358831780000053, 1452.355416418630057, 183.2659201527980031 ) ) ;
#90823=CARTESIAN_POINT ( 'NONE',  ( -3.156350064089999741, 1484.702381841229908, 183.3290672668979937 ) ) ;
#90824=CARTESIAN_POINT ( 'NONE',  ( -2.500000000000000000, 1439.547542131649834, 164.8613965946329927 ) ) ;
#90826=CARTESIAN_POINT ( 'NONE',  ( 38.81202645930000017, 1436.797832437240231, 134.0999985825980332 ) ) ;
#90828=FACE_OUTER_BOUND ( 'NONE', #23202, .T. ) ;
#90834=ORIENTED_EDGE ( 'NONE', *, *, #72040, .T. ) ;
#90835=CARTESIAN_POINT ( 'NONE',  ( 33.89753131429299771, 1440.913060387330006, 259.1515849714069759 ) ) ;
#90836=CARTESIAN_POINT ( 'NONE',  ( -0.0002035883165944741776, 1452.365207701825739, 153.7261367825575178 ) ) ;
#90838=CARTESIAN_POINT ( 'NONE',  ( 0.05421983196053539733, 1451.175530199109971, 182.5313573697069955 ) ) ;
#90839=CARTESIAN_POINT ( 'NONE',  ( -16.66257565289999931, 1410.427174256630224, 191.7597267753979793 ) ) ;
#90842=CARTESIAN_POINT ( 'NONE',  ( 21.13431379670319998, 1409.651086887829933, 206.4149708788170301 ) ) ;
#90844=CARTESIAN_POINT ( 'NONE',  ( -1.449529204450000108, 1508.614376975429877, 180.2799702684980048 ) ) ;
#90847=CARTESIAN_POINT ( 'NONE',  ( 12.94229023090000119, 1461.456462053329915, 233.4393938603979848 ) ) ;
#90848=CARTESIAN_POINT ( 'NONE',  ( -11.60004869886543410, 1424.050231871397045, 137.1752122141798225 ) ) ;
#90849=CARTESIAN_POINT ( 'NONE',  ( -0.3402596924234728704, 1410.306538769425742, 233.2121123280315942 ) ) ;
#90852=CARTESIAN_POINT ( 'NONE',  ( -0.4586520875518777518, 1486.396701128719542, 181.7766115271735714 ) ) ;
#90854=CARTESIAN_POINT ( 'NONE',  ( -0.1511123393328930031, 1507.449223653020226, 180.8591688853359756 ) ) ;
#90861=ORIENTED_EDGE ( 'NONE', *, *, #42023, .F. ) ;
#90862=LINE ( 'NONE', #100372, #28105 ) ;
#90863=CARTESIAN_POINT ( 'NONE',  ( 20.68004892169999920, 1453.350765365529924, 221.6396287865980241 ) ) ;
#90865=CARTESIAN_POINT ( 'NONE',  ( -11.84725155179999945, 1430.949263877939984, 150.2388512889980063 ) ) ;
#90868=CARTESIAN_POINT ( 'NONE',  ( 9.330551562259142173, 1426.784206974829885, 151.9956406576650352 ) ) ;
#90870=CARTESIAN_POINT ( 'NONE',  ( 12.59633922020000085, 1445.148044568509931, 187.0941081104979844 ) ) ;
#90871=CARTESIAN_POINT ( 'NONE',  ( -20.34050849710000008, 1457.444417593830167, 224.6898825346980288 ) ) ;
#90874=EDGE_LOOP ( 'NONE', ( #33653, #99343, #3480, #9382 ) ) ;
#90877=CARTESIAN_POINT ( 'NONE',  ( 4.994452949999999447, 1405.913965673130178, 267.8435537567980305 ) ) ;
#90878=CARTESIAN_POINT ( 'NONE',  ( 0.09447546337450000997, 1408.916359543229873, 186.4601785166979937 ) ) ;
#90881=CARTESIAN_POINT ( 'NONE',  ( 23.62109726877421423, 1434.135449394258558, 214.7287868320940447 ) ) ;
#90883=CARTESIAN_POINT ( 'NONE',  ( -1.594806016870000009, 1450.591479615480011, 183.0618219514980183 ) ) ;
#90884=EDGE_CURVE ( 'NONE', #78014, #72991, #423, .T. ) ;
#90887=CARTESIAN_POINT ( 'NONE',  ( -2.428387260106030343, 1449.547206808950023, 154.5200478772810015 ) ) ;
#90888=CARTESIAN_POINT ( 'NONE',  ( -1.569676819536519385, 1450.891569726948546, 183.4696716048479459 ) ) ;
#90889=CARTESIAN_POINT ( 'NONE',  ( -19.87804702706843685, 1485.311229468551801, 190.7217664356889486 ) ) ;
#90890=CARTESIAN_POINT ( 'NONE',  ( -14.45750500688560081, 1416.828039245989885, 221.3916439204320170 ) ) ;
#90892=CARTESIAN_POINT ( 'NONE',  ( -5.969073325650000150, 1428.313923095629889, 209.1218459616979999 ) ) ;
#90896=CARTESIAN_POINT ( 'NONE',  ( 13.04207810306199988, 1409.368499790489750, 192.3005055522939983 ) ) ;
#90897=CARTESIAN_POINT ( 'NONE',  ( -4.991737838419999740, 1475.878694619930002, 267.5267923144979818 ) ) ;
#90898=DIRECTION ( 'NONE',  ( -0.7636119845522929550, -0.004098122786836628888, -0.6456624059349689304 ) ) ;
#90908=( BOUNDED_CURVE ( )  B_SPLINE_CURVE ( 3, ( #95639, #96195, #37394, #44148 ),
 .UNSPECIFIED., .F., .F. ) 
 B_SPLINE_CURVE_WITH_KNOTS ( ( 4, 4 ),
 ( 6.251003116154824291, 6.262497214195333228 ),
 .UNSPECIFIED. ) 
 CURVE ( )  GEOMETRIC_REPRESENTATION_ITEM ( )  RATIONAL_B_SPLINE_CURVE ( ( 1.000000000000000000, 0.9999889905061551953, 0.9999889905061551953, 1.000000000000000000 ) ) 
 REPRESENTATION_ITEM ( '' )  );
#90909=CARTESIAN_POINT ( 'NONE',  ( -18.08393550219999923, 1409.544565332530055, 197.0250912618979839 ) ) ;
#90911=CARTESIAN_POINT ( 'NONE',  ( 19.28229067004766861, 1456.003485696241569, 225.1845458337684249 ) ) ;
#90913=CARTESIAN_POINT ( 'NONE',  ( -2.642706046298320732, 1410.383226565404584, 232.6286052421928048 ) ) ;
#90916=CARTESIAN_POINT ( 'NONE',  ( 10.74308370929999867, 1424.967654141830053, 139.6357132919980018 ) ) ;
#90923=CARTESIAN_POINT ( 'NONE',  ( -2.409586283469999923, 1426.663880916129983, 144.1938086916980239 ) ) ;
#90927=CARTESIAN_POINT ( 'NONE',  ( 21.91792290201540183, 1509.678451720530120, 227.8819227092559743 ) ) ;
#90929=ORIENTED_EDGE ( 'NONE', *, *, #9658, .F. ) ;
#90931=CARTESIAN_POINT ( 'NONE',  ( -5.776215096199999621, 1396.296062264229931, 198.6637670462979770 ) ) ;
#90932=CARTESIAN_POINT ( 'NONE',  ( -21.01722066690000190, 1410.567592102230037, 218.3378942615279925 ) ) ;
#90934=CARTESIAN_POINT ( 'NONE',  ( -12.73809752124026495, 1445.003929500445793, 169.4561374448583990 ) ) ;
#90935=CARTESIAN_POINT ( 'NONE',  ( -25.23570363969999875, 1509.794310577129863, 194.6260395679979922 ) ) ;
#90937=CARTESIAN_POINT ( 'NONE',  ( 0.7910245917146940808, 1426.918876941764893, 134.0999999980980135 ) ) ;
#90938=CARTESIAN_POINT ( 'NONE',  ( 17.60601737500000041, 1410.887304148830026, 224.8084147167980120 ) ) ;
#90939=B_SPLINE_CURVE_WITH_KNOTS ( 'NONE', 3,
 ( #57488, #82669, #32800, #67540 ),
 .UNSPECIFIED., .F., .F.,
 ( 4, 4 ),
 ( 0.000000000000000000, 1.000000000000000000 ),
 .UNSPECIFIED. ) ;
#90941=CARTESIAN_POINT ( 'NONE',  ( -7.723894028380000165, 1416.216596894529857, 192.5579729901980102 ) ) ;
#90943=CARTESIAN_POINT ( 'NONE',  ( 11.06592217088270047, 1396.299490904690174, 209.4166363852829988 ) ) ;
#90944=CARTESIAN_POINT ( 'NONE',  ( 1.326919707080000066, 1414.988017870030035, 191.7691690602979691 ) ) ;
#90945=CARTESIAN_POINT ( 'NONE',  ( 11.25166810410000018, 1428.703240696229841, 150.5458012123980041 ) ) ;
#90946=CARTESIAN_POINT ( 'NONE',  ( 5.938657822353222038, 1509.124927619275013, 180.2982783801607525 ) ) ;
#90948=CARTESIAN_POINT ( 'NONE',  ( 13.46829667242139905, 1436.161474321959986, 150.5249941659139949 ) ) ;
#90951=VERTEX_POINT ( 'NONE', #72872 ) ;
#90953=CARTESIAN_POINT ( 'NONE',  ( -14.92438935200000039, 1460.034730670430008, 231.4439065160979965 ) ) ;
#90955=CARTESIAN_POINT ( 'NONE',  ( -13.49161259159999915, 1434.822352678170091, 195.9491175140979919 ) ) ;
#90960=CARTESIAN_POINT ( 'NONE',  ( 2.500000000000000000, 1448.534146728170072, 160.0811088377199951 ) ) ;
#90962=AXIS2_PLACEMENT_3D ( 'NONE', #14000, #82325, #22943 ) ;
#90967=CARTESIAN_POINT ( 'NONE',  ( -10.92882029718542825, 1411.379195557904040, 269.3492646456201669 ) ) ;
#90972=CARTESIAN_POINT ( 'NONE',  ( -28.02863369646679814, 1440.913060388819986, 231.2731264215370004 ) ) ;
#90974=CARTESIAN_POINT ( 'NONE',  ( -0.1290038325305789824, 1466.767347909359842, 235.6227026514060015 ) ) ;
#90976=CARTESIAN_POINT ( 'NONE',  ( 13.22859383683809931, 1410.662777231539849, 270.3663857566149886 ) ) ;
#90978=CARTESIAN_POINT ( 'NONE',  ( 23.93604199780000030, 1410.398478142230033, 208.8934000136680140 ) ) ;
#90979=CYLINDRICAL_SURFACE ( 'NONE', #55351, 1.463110112870021462 ) ;
#90981=CARTESIAN_POINT ( 'NONE',  ( -11.60004869885203682, 1425.894669202444675, 137.5118601406020673 ) ) ;
#90983=CARTESIAN_POINT ( 'NONE',  ( 4.254228409968599856, 1420.739899128549951, 185.5486331039510048 ) ) ;
#90984=CARTESIAN_POINT ( 'NONE',  ( 0.1144970540559999972, 1419.768045047230089, 184.3728024650980046 ) ) ;
#90985=CARTESIAN_POINT ( 'NONE',  ( -14.03738926715088020, 1486.050909705618778, 185.7519581601395373 ) ) ;
#90989=CARTESIAN_POINT ( 'NONE',  ( 18.64672481350000055, 1416.851343894929869, 209.6839434898159880 ) ) ;
#90990=CARTESIAN_POINT ( 'NONE',  ( -17.33645362950000290, 1414.996442546130083, 207.8511177337479978 ) ) ;
#90991=CARTESIAN_POINT ( 'NONE',  ( -4.619855912889999416, 1417.833749415829971, 234.7627619328980018 ) ) ;
#90994=CARTESIAN_POINT ( 'NONE',  ( 3.932771983779999925, 1448.980696587250122, 184.2693349551980191 ) ) ;
#90996=DIRECTION ( 'NONE',  ( 0.000000000000000000, -1.000000000000000000, 0.000000000000000000 ) ) ;
#90997=CARTESIAN_POINT ( 'NONE',  ( -26.24366108068827685, 1450.757924316903200, 136.5808154326949477 ) ) ;
#90999=ORIENTED_EDGE ( 'NONE', *, *, #7669, .F. ) ;
#91002=ORIENTED_EDGE ( 'NONE', *, *, #6527, .T. ) ;
#91003=CARTESIAN_POINT ( 'NONE',  ( 0.08715897492290000659, 1457.824249707829949, 229.0178643556979807 ) ) ;
#91005=CARTESIAN_POINT ( 'NONE',  ( 24.32474686429999977, 1445.057405757869901, 214.3193390981779771 ) ) ;
#91009=CARTESIAN_POINT ( 'NONE',  ( 3.846235792629999928, 1440.870317293109792, 184.3772602386979997 ) ) ;
#91011=CARTESIAN_POINT ( 'NONE',  ( -19.04818187609999924, 1425.840467097430064, 224.4548499685980119 ) ) ;
#91015=CARTESIAN_POINT ( 'NONE',  ( 18.43597720400000028, 1478.525022087329944, 189.5193842725980176 ) ) ;
#91016=CARTESIAN_POINT ( 'NONE',  ( 0.2256679910384030152, 1409.089073560189945, 232.6561860856899955 ) ) ;
#91017=CARTESIAN_POINT ( 'NONE',  ( -38.47038145532883391, 1453.194700005767572, 269.5842303393881139 ) ) ;
#91021=CARTESIAN_POINT ( 'NONE',  ( -43.73032397436223562, 1431.081481799955782, 269.0283264950530224 ) ) ;
#91025=CARTESIAN_POINT ( 'NONE',  ( -0.02607537583049999996, 1415.758200151029996, 233.4550498395979901 ) ) ;
#91026=CARTESIAN_POINT ( 'NONE',  ( -13.13904713841083272, 1444.767805270108965, 186.4863153449116453 ) ) ;
#91029=CIRCLE ( 'NONE', #89279, 1.999999999999912514 ) ;
#91030=CARTESIAN_POINT ( 'NONE',  ( 11.60004869885203682, 1411.254281879943164, 134.0999999980979851 ) ) ;
#91033=CARTESIAN_POINT ( 'NONE',  ( 24.99158728859999812, 1436.290377140129749, 137.7556578815979833 ) ) ;
#91034=DIRECTION ( 'NONE',  ( -0.9993779840209169318, 0.0009463042317009218206, 0.03525265327019708878 ) ) ;
#91035=CARTESIAN_POINT ( 'NONE',  ( -14.79762023470000187, 1410.816705584730016, 226.7256837507980265 ) ) ;
#91036=ORIENTED_EDGE ( 'NONE', *, *, #21057, .T. ) ;
#91039=ORIENTED_EDGE ( 'NONE', *, *, #27175, .T. ) ;
#91044=CARTESIAN_POINT ( 'NONE',  ( -22.11712025990000186, 1461.968260157729901, 248.4077083967980286 ) ) ;
#91045=CARTESIAN_POINT ( 'NONE',  ( -19.49548631520000086, 1491.251290675329983, 189.4511891077980010 ) ) ;
#91046=CARTESIAN_POINT ( 'NONE',  ( -11.07768414439999916, 1433.779967063539971, 151.7039717618979751 ) ) ;
#91051=CARTESIAN_POINT ( 'NONE',  ( -25.97380345099999843, 1440.631369481410047, 137.9741832456979864 ) ) ;
#91054=CARTESIAN_POINT ( 'NONE',  ( 2.392895678049999919, 1449.650479641829861, 182.2220820520979885 ) ) ;
#91056=CARTESIAN_POINT ( 'NONE',  ( 22.52609270013210008, 1509.699688878029974, 227.6602567939980020 ) ) ;
#91057=CARTESIAN_POINT ( 'NONE',  ( 3.287954922066450199E-10, 1411.119718540189751, 255.8594453057300200 ) ) ;
#91059=ORIENTED_EDGE ( 'NONE', *, *, #105682, .T. ) ;
#91064=CARTESIAN_POINT ( 'NONE',  ( -8.103048356079998626, 1472.070011036030110, 270.3694265424979903 ) ) ;
#91065=CARTESIAN_POINT ( 'NONE',  ( 0.000000000000000000, 1514.413060387330006, 209.1218459616979999 ) ) ;
#91068=CARTESIAN_POINT ( 'NONE',  ( 34.51399565513580114, 1450.846036594779889, 136.1540978105180102 ) ) ;
#91069=CARTESIAN_POINT ( 'NONE',  ( 0.3162628321739870407, 1451.008570913309995, 181.9092865251629973 ) ) ;
#91075=CARTESIAN_POINT ( 'NONE',  ( -37.39809849698710309, 1420.331652018609930, 268.7662396804499849 ) ) ;
#91076=EDGE_LOOP ( 'NONE', ( #23047, #25496, #63048, #67632, #95393, #78120, #45416 ) ) ;
#91077=CARTESIAN_POINT ( 'NONE',  ( -3.533503288940170073, 1491.923507061140072, 181.6243563976589996 ) ) ;
#91079=ORIENTED_EDGE ( 'NONE', *, *, #43333, .T. ) ;
#91082=CARTESIAN_POINT ( 'NONE',  ( 40.97446893530570122, 1444.174879737809988, 136.8850285840350125 ) ) ;
#91085=CARTESIAN_POINT ( 'NONE',  ( -16.81040325900000099, 1455.454303044529979, 189.6281205366979918 ) ) ;
#91086=AXIS2_PLACEMENT_3D ( 'NONE', #57000, #34949, #42809 ) ;
#91087=CARTESIAN_POINT ( 'NONE',  ( -12.53380499169999851, 1442.773887286369927, 181.5854552579979782 ) ) ;
#91090=CARTESIAN_POINT ( 'NONE',  ( -10.79382269979189957, 1414.913060387349788, 196.1395788316550011 ) ) ;
#91091=EDGE_CURVE ( 'NONE', #74077, #104782, #26299, .T. ) ;
#91092=B_SPLINE_CURVE_WITH_KNOTS ( 'NONE', 5,
 ( #21732, #45886, #105790, #54839, #72200, #29604, #56482, #11715, #63791 ),
 .UNSPECIFIED., .F., .F.,
 ( 6, 3, 6 ),
 ( 0.000000000000000000, 0.4491568913793235751, 1.000000000000000000 ),
 .UNSPECIFIED. ) ;
#91096=DIRECTION ( 'NONE',  ( 0.000000000000000000, 0.000000000000000000, -1.000000000000000000 ) ) ;
#91097=EDGE_CURVE ( 'NONE', #104566, #2114, #206, .T. ) ;
#91099=CARTESIAN_POINT ( 'NONE',  ( 0.03232804668210000759, 1407.837594160830122, 195.9367397046979988 ) ) ;
#91100=CARTESIAN_POINT ( 'NONE',  ( -2.664535259099599458E-15, 1405.913060387330006, 209.1218459616979999 ) ) ;
#91104=ORIENTED_EDGE ( 'NONE', *, *, #57754, .T. ) ;
#91105=CARTESIAN_POINT ( 'NONE',  ( 0.2703871436749999968, 1452.337177918929910, 183.2881653520979910 ) ) ;
#91106=ADVANCED_FACE ( 'NONE', ( #103568 ), #95179, .F. ) ;
#91114=CARTESIAN_POINT ( 'NONE',  ( -1.782112605382539794, 1484.239369046139927, 182.8010181983919722 ) ) ;
#91115=CARTESIAN_POINT ( 'NONE',  ( -14.87168878229999969, 1430.147188444230096, 221.8136313627980201 ) ) ;
#91120=CARTESIAN_POINT ( 'NONE',  ( -36.37832872588079169, 1435.767865734240104, 134.7398496865939990 ) ) ;
#91124=CARTESIAN_POINT ( 'NONE',  ( 2.787053946926249637, 1424.897258074847059, 183.3886486283980162 ) ) ;
#91125=CARTESIAN_POINT ( 'NONE',  ( -24.67353296015457076, 1509.777057924631208, 225.1797433603865386 ) ) ;
#91126=CARTESIAN_POINT ( 'NONE',  ( 13.76900370180000088, 1415.553739807329976, 196.8536881224979993 ) ) ;
#91128=CARTESIAN_POINT ( 'NONE',  ( -20.81306254345079765, 1578.884139733799884, 163.1496826969390384 ) ) ;
#91129=CARTESIAN_POINT ( 'NONE',  ( 17.48729376020000004, 1410.446401242629918, 225.6075485739979740 ) ) ;
#91131=CARTESIAN_POINT ( 'NONE',  ( 2.382436964801011303, 1426.901689560120076, 137.0999999980980135 ) ) ;
#91132=CARTESIAN_POINT ( 'NONE',  ( 22.77112932521035304, 1451.090417561717004, 218.6197847536123788 ) ) ;
#91133=CIRCLE ( 'NONE', #3581, 41.12363927708771882 ) ;
#91139=CARTESIAN_POINT ( 'NONE',  ( -26.02835829340000018, 1468.278484548229926, 269.9886483896979712 ) ) ;
#91143=CARTESIAN_POINT ( 'NONE',  ( 6.500314218507900144, 1509.153493339920033, 179.5230332626949803 ) ) ;
#91144=CARTESIAN_POINT ( 'NONE',  ( 11.60004869885203682, 1425.888728951611938, 137.5022903913526591 ) ) ;
#91145=CARTESIAN_POINT ( 'NONE',  ( 2.933420754659926466, 1417.794866989897400, 234.2124010178503113 ) ) ;
#91147=CARTESIAN_POINT ( 'NONE',  ( -2.500000000000000000, 1424.046630307830128, 154.4234530583979961 ) ) ;
#91150=CARTESIAN_POINT ( 'NONE',  ( 28.79543911281049873, 1440.913060387340010, 234.2238028330110069 ) ) ;
#91154=ORIENTED_EDGE ( 'NONE', *, *, #104403, .F. ) ;
#91155=ORIENTED_EDGE ( 'NONE', *, *, #51331, .F. ) ;
#91156=CARTESIAN_POINT ( 'NONE',  ( 13.51610093808350221, 1442.913060377700731, 206.7785865123596807 ) ) ;
#91157=EDGE_CURVE ( 'NONE', #944, #14800, #105708, .T. ) ;
#91158=CARTESIAN_POINT ( 'NONE',  ( -9.840693639790396574, 1506.501081010019561, 228.8468162685099685 ) ) ;
#91168=CARTESIAN_POINT ( 'NONE',  ( -14.46947201719999931, 1471.323284330429715, 193.8233120731979966 ) ) ;
#91174=EDGE_CURVE ( 'NONE', #11504, #79125, #59328, .T. ) ;
#91182=CARTESIAN_POINT ( 'NONE',  ( -0.5621806508122783042, 1416.843574565329845, 227.7683146822559763 ) ) ;
#91188=CARTESIAN_POINT ( 'NONE',  ( 1.642074464903110043, 1408.970402891180129, 194.2161375618219950 ) ) ;
#91189=CARTESIAN_POINT ( 'NONE',  ( 18.80464029359000122, 1425.800308749483975, 225.6068200636500194 ) ) ;
#91190=CARTESIAN_POINT ( 'NONE',  ( 2.412180996239999597, 1419.421713268930034, 185.1536642287979930 ) ) ;
#91194=CARTESIAN_POINT ( 'NONE',  ( -3.365813053994819892, 1449.482398035879896, 184.7700481427870045 ) ) ;
#91197=CARTESIAN_POINT ( 'NONE',  ( -6.232532191338900240, 1398.098440470949981, 197.7132727547819968 ) ) ;
#91198=CARTESIAN_POINT ( 'NONE',  ( 19.38194617106359985, 1456.050539493930046, 227.4026333903129853 ) ) ;
#91199=CARTESIAN_POINT ( 'NONE',  ( -12.70521320840000001, 1434.771930543859980, 150.2289112725980260 ) ) ;
#91200=CARTESIAN_POINT ( 'NONE',  ( -4.034698761822709636E-10, 1466.818507878050013, 244.3811635369520161 ) ) ;
#91201=CARTESIAN_POINT ( 'NONE',  ( -20.47924549841579989, 1503.953507240960107, 190.5028550971699985 ) ) ;
#91202=PLANE ( 'NONE',  #78639 ) ;
#91204=CARTESIAN_POINT ( 'NONE',  ( -0.1801023543370000035, 1476.672953218830116, 182.1974262930980046 ) ) ;
#91206=CARTESIAN_POINT ( 'NONE',  ( -45.84755609590860104, 1440.256076863080125, 268.7565746053210205 ) ) ;
#91207=CARTESIAN_POINT ( 'NONE',  ( -20.86430737430000448, 1507.787508480630095, 191.9680527028979782 ) ) ;
#91208=ADVANCED_FACE ( 'NONE', ( #41275 ), #72534, .T. ) ;
#91210=VECTOR ( 'NONE', #47812, 1000.000000000000000 ) ;
#91211=CARTESIAN_POINT ( 'NONE',  ( 5.683171320879200294, 1409.111521102960069, 222.7165751117499894 ) ) ;
#91214=CARTESIAN_POINT ( 'NONE',  ( 8.963481490043514910, 1426.098811295182031, 225.6675240377605292 ) ) ;
#91218=CARTESIAN_POINT ( 'NONE',  ( 31.69751081770000312, 1436.813883501469945, 244.1892870132980136 ) ) ;
#91220=CARTESIAN_POINT ( 'NONE',  ( -1.525257681609999860, 1486.442310458030079, 181.6794219812979918 ) ) ;
#91224=CARTESIAN_POINT ( 'NONE',  ( -4.104542198569999911, 1419.727281559329867, 225.2064028888979976 ) ) ;
#91226=CARTESIAN_POINT ( 'NONE',  ( -19.56170200118970115, 1452.229950700849940, 143.7718973678339864 ) ) ;
#91231=FACE_OUTER_BOUND ( 'NONE', #32399, .T. ) ;
#91233=ORIENTED_EDGE ( 'NONE', *, *, #23447, .F. ) ;
#91237=CARTESIAN_POINT ( 'NONE',  ( -23.76160520478569893, 1410.154579653240035, 209.1277447343530014 ) ) ;
#91242=CARTESIAN_POINT ( 'NONE',  ( -3.894297052259999781, 1498.349224807129985, 236.2074788674979970 ) ) ;
#91243=CARTESIAN_POINT ( 'NONE',  ( -18.37208795600000144, 1410.877977816430075, 224.1326316794980187 ) ) ;
#91244=CARTESIAN_POINT ( 'NONE',  ( 44.21373685866610259, 1449.831903069469945, 266.2301373114850094 ) ) ;
#91247=( BOUNDED_CURVE ( )  B_SPLINE_CURVE ( 3, ( #48843, #81857, #40959, #100320 ),
 .UNSPECIFIED., .F., .F. ) 
 B_SPLINE_CURVE_WITH_KNOTS ( ( 4, 4 ),
 ( 3.086775739023659870, 3.394672873780574918 ),
 .UNSPECIFIED. ) 
 CURVE ( )  GEOMETRIC_REPRESENTATION_ITEM ( )  RATIONAL_B_SPLINE_CURVE ( ( 1.000000000000000000, 0.9921155365922033065, 0.9921155365922033065, 1.000000000000000000 ) ) 
 REPRESENTATION_ITEM ( '' )  );
#91250=CARTESIAN_POINT ( 'NONE',  ( -0.2331143941452460122, 1408.921200921389982, 231.7611568498559791 ) ) ;
#91252=CARTESIAN_POINT ( 'NONE',  ( 13.49429930720275017, 1443.686343019639480, 188.0286533011901042 ) ) ;
#91257=B_SPLINE_SURFACE_WITH_KNOTS ( 'NONE', 5, 5, ( 
 ( #85278, #2435, #51707, #70747, #104858, #43309 ),
 ( #85847, #9146, #760, #34888, #103178, #60676 ),
 ( #94802, #18077, #52272, #105414, #5145, #88077 ),
 ( #11365, #98646, #28706, #71300, #79675, #30341 ),
 ( #46079, #71858, #4606, #88624, #38740, #80763 ),
 ( #20834, #55576, #3528, #89700, #62911, #11904 ),
 ( #80210, #30889, #105975, #107606, #96462, #98095 ),
 ( #97022, #21368, #29252, #37100, #37653, #12444 ),
 ( #55029, #2980, #72918, #4071, #12981, #38196 ),
 ( #81840, #89156, #39300, #63985, #45536, #47711 ),
 ( #63443, #97561, #46629, #72379, #106507, #29797 ),
 ( #20283, #47164, #54489, #81292, #73473, #107057 ) ),
 .UNSPECIFIED., .F., .F., .F.,
 ( 6, 3, 3, 6 ),
 ( 6, 6 ),
 ( 37.11367623070000121, 43.72652432289999780, 46.71962562659999918, 49.71279531210000613 ),
 ( 0.000000000000000000, 2.000000000000000000 ),
 .UNSPECIFIED. ) ;
#91264=( GEOMETRIC_REPRESENTATION_CONTEXT ( 3 ) GLOBAL_UNCERTAINTY_ASSIGNED_CONTEXT ( ( #89367 ) ) GLOBAL_UNIT_ASSIGNED_CONTEXT ( ( #19752, #88636, #46091 ) ) REPRESENTATION_CONTEXT ( 'NONE', 'WORKASPACE' ) );
#91268=CARTESIAN_POINT ( 'NONE',  ( 16.43752752869999867, 1507.637957906029897, 193.5312328863980156 ) ) ;
#91270=CARTESIAN_POINT ( 'NONE',  ( -24.61162824655679771, 1509.291569965729877, 222.5955736776400045 ) ) ;
#91271=CARTESIAN_POINT ( 'NONE',  ( 11.01124415049999961, 1428.984115384829920, 91.31218443469779800 ) ) ;
#91279=ORIENTED_EDGE ( 'NONE', *, *, #78052, .F. ) ;
#91281=CARTESIAN_POINT ( 'NONE',  ( -2.488082932330000219, 1441.600846913620217, 150.5962877614979902 ) ) ;
#91282=CARTESIAN_POINT ( 'NONE',  ( -14.35446004689999810, 1416.822692864329838, 221.5782750974979933 ) ) ;
#91283=CARTESIAN_POINT ( 'NONE',  ( 11.22261500629999986, 1433.988530975800131, 151.5940001495979743 ) ) ;
#91284=CARTESIAN_POINT ( 'NONE',  ( 5.757839680140000027, 1468.063065669429989, 262.6648722463980334 ) ) ;
#91286=CARTESIAN_POINT ( 'NONE',  ( -11.60004869885203682, 1428.983126981193436, 134.0999999980979851 ) ) ;
#91292=CARTESIAN_POINT ( 'NONE',  ( 0.5697990016583959205, 1450.893162567740092, 181.2939912002310052 ) ) ;
#91293=CARTESIAN_POINT ( 'NONE',  ( -17.92837075459999951, 1410.035885881930199, 224.4980084594979814 ) ) ;
#91295=CARTESIAN_POINT ( 'NONE',  ( 34.33069675793380071, 1442.322945860919845, 137.1732133209670224 ) ) ;
#91297=CARTESIAN_POINT ( 'NONE',  ( 9.726491193908251375E-12, 1408.913060387299993, 194.1220083575990145 ) ) ;
#91300=CARTESIAN_POINT ( 'NONE',  ( -9.959064579650000582, 1415.087818611729972, 222.8661268712980075 ) ) ;
#91301=CARTESIAN_POINT ( 'NONE',  ( 0.2077598587401390251, 1458.608988913009853, 183.0127631382089817 ) ) ;
#91302=CARTESIAN_POINT ( 'NONE',  ( -2.814434489400770012, 1407.025243844600027, 222.1218459754350363 ) ) ;
#91304=CARTESIAN_POINT ( 'NONE',  ( 0.4435022289555869968, 1418.672171135500093, 184.7048927309859891 ) ) ;
#91306=EDGE_CURVE ( 'NONE', #104116, #9907, #69987, .T. ) ;
#91307=CARTESIAN_POINT ( 'NONE',  ( -28.79711193535739966, 1509.835383000219963, 211.3965062070199963 ) ) ;
#91308=CARTESIAN_POINT ( 'NONE',  ( 11.94118163750000150, 1433.615363880359837, 149.1895118235980249 ) ) ;
#91309=CARTESIAN_POINT ( 'NONE',  ( -26.81573373259999826, 1435.593055354309854, 136.1631887211979688 ) ) ;
#91310=CARTESIAN_POINT ( 'NONE',  ( 11.78238822100000149, 1440.882651071759938, 188.1224418543980335 ) ) ;
#91316=CARTESIAN_POINT ( 'NONE',  ( -1.371718781699999834, 1452.291798068730031, 183.7871359344979965 ) ) ;
#91317=B_SPLINE_CURVE_WITH_KNOTS ( 'NONE', 3,
 ( #85724, #44864, #86283, #52150 ),
 .UNSPECIFIED., .F., .F.,
 ( 4, 4 ),
 ( 0.000000000000000000, 1.000000000000000000 ),
 .UNSPECIFIED. ) ;
#91319=CARTESIAN_POINT ( 'NONE',  ( 40.52588777580712076, 1425.188750968595741, 269.1149643231569826 ) ) ;
#91320=CARTESIAN_POINT ( 'NONE',  ( -19.95761699851187387, 1506.164913903586239, 189.0205224701858526 ) ) ;
#91321=CARTESIAN_POINT ( 'NONE',  ( 20.61690388284639042, 1509.299818271619188, 189.0201435835461439 ) ) ;
#91327=CARTESIAN_POINT ( 'NONE',  ( -28.81018896820719988, 1509.453431482950009, 208.7252267088939846 ) ) ;
#91328=CARTESIAN_POINT ( 'NONE',  ( -15.92445961705290003, 1410.432587407550045, 226.6488369890140007 ) ) ;
#91330=ORIENTED_EDGE ( 'NONE', *, *, #5020, .F. ) ;
#91331=CARTESIAN_POINT ( 'NONE',  ( -11.82552473729999853, 1507.579552363830089, 183.2239286378979841 ) ) ;
#91332=CARTESIAN_POINT ( 'NONE',  ( 40.27307890487595898, 1443.616175311578900, 137.1168156925720893 ) ) ;
#91333=CARTESIAN_POINT ( 'NONE',  ( 21.59613673650000010, 1509.442267771630213, 226.5610156191980025 ) ) ;
#91337=CARTESIAN_POINT ( 'NONE',  ( 2.219943772349999733, 1464.863888256930068, 237.3912208446979832 ) ) ;
#91339=CARTESIAN_POINT ( 'NONE',  ( 19.70825520289999844, 1410.962810032930065, 220.5533580383980166 ) ) ;
#91340=B_SPLINE_SURFACE_WITH_KNOTS ( 'NONE', 5, 5, ( 
 ( #85216, #109347, #76838, #109884, #151, #58937, #68454, #17440, #85775, #9076, #43243, #18009, #35379, #10743, #1807, #29186, #86330, #53307, #96954, #69568, #104793 ),
 ( #20220, #70680, #54421, #28636, #77935, #1242, #103687, #20761, #87449, #52748, #2913, #26988, #44916, #46008, #61176, #88553, #105907, #95294, #79608, #37585, #9615 ),
 ( #79063, #18555, #86882, #10176, #44350, #78493, #61715, #35944, #70130, #80138, #43785, #104241, #62841, #37030, #28079, #27532, #95836, #11836, #19104, #2368, #3457 ),
 ( #63377, #71788, #36482, #97493, #62267, #96397, #19672, #53877, #88015, #11299, #45467, #71223, #105347, #81226, #48203, #106444, #72312, #39225, #46559, #72850, #80695 ),
 ( #5074, #4541, #90171, #99669, #4005, #31928, #55504, #14571, #74512, #99119, #29726, #30272, #39792, #38131, #63912, #98581, #21847, #82342, #98026, #47643, #12373 ),
 ( #57167, #13454, #107538, #64465, #14014, #40331, #81771, #21300, #73399, #89632, #56044, #47099, #12920, #5641, #73951, #38675, #30826, #106985, #65002, #108642, #22397 ) ),
 .UNSPECIFIED., .F., .F., .F.,
 ( 6, 6 ),
 ( 6, 3, 3, 3, 3, 3, 6 ),
 ( 1.704359096279999930, 13.41865417910000069 ),
 ( 27.98477882999999977, 34.32981118040000013, 36.68144354599999701, 37.85725972880000256, 39.03307591160000101, 39.85395972119999897, 40.67484353080000403 ),
 .UNSPECIFIED. ) ;
#91341=CARTESIAN_POINT ( 'NONE',  ( -2.923659802470610192, 1410.372349471019788, 186.6137880374459996 ) ) ;
#91343=CARTESIAN_POINT ( 'NONE',  ( -17.85622223500000061, 1424.491927465330036, 227.8867262256979984 ) ) ;
#91345=CARTESIAN_POINT ( 'NONE',  ( 22.01621720475775135, 1506.474306125260682, 208.9595913853024456 ) ) ;
#91346=FACE_OUTER_BOUND ( 'NONE', #48869, .T. ) ;
#91348=EDGE_CURVE ( 'NONE', #75020, #72755, #39537, .T. ) ;
#91349=CARTESIAN_POINT ( 'NONE',  ( 24.50927534411190933, 1509.771934658697091, 192.7779650040213539 ) ) ;
#91350=CARTESIAN_POINT ( 'NONE',  ( -1.392294270230000075, 1415.872631189930189, 233.2008784669980059 ) ) ;
#91352=EDGE_CURVE ( 'NONE', #83528, #33967, #84287, .T. ) ;
#91354=CARTESIAN_POINT ( 'NONE',  ( -5.351895964595500210, 1484.703362324490172, 183.6627706421859898 ) ) ;
#91358=CARTESIAN_POINT ( 'NONE',  ( -4.241168549582178926, 1441.430627509509804, 162.5672745638440233 ) ) ;
#91367=CARTESIAN_POINT ( 'NONE',  ( -20.59685312423998127, 1507.762914175841161, 190.3821643482645811 ) ) ;
#91368=CARTESIAN_POINT ( 'NONE',  ( 16.24165198109999864, 1409.730207214729944, 192.2072427057979951 ) ) ;
#91370=CARTESIAN_POINT ( 'NONE',  ( 40.14987069115329632, 1439.836753192460037, 136.5114502648049779 ) ) ;
#91373=CARTESIAN_POINT ( 'NONE',  ( 17.11398521796633432, 1460.311162561034280, 228.6660193555352407 ) ) ;
#91376=CARTESIAN_POINT ( 'NONE',  ( 1.876675108085915644, 1395.978595326182813, 220.1335329578695621 ) ) ;
#91377=ORIENTED_EDGE ( 'NONE', *, *, #17075, .T. ) ;
#91379=CARTESIAN_POINT ( 'NONE',  ( -19.16952157780000121, 1456.627486491929858, 228.8719534504979833 ) ) ;
#91382=CARTESIAN_POINT ( 'NONE',  ( 13.41947731569904079, 1410.754602942108477, 228.3337818491096414 ) ) ;
#91387=CARTESIAN_POINT ( 'NONE',  ( -2.500000000000280220, 1439.222456145959995, 159.1125091106669913 ) ) ;
#91391=CARTESIAN_POINT ( 'NONE',  ( 42.60628463550120415, 1443.705283444789984, 134.7402669369780028 ) ) ;
#91393=CARTESIAN_POINT ( 'NONE',  ( 26.91754656130000001, 1437.398890514510185, 136.8530043402979857 ) ) ;
#91395=CARTESIAN_POINT ( 'NONE',  ( 3.877170719089999995, 1415.932617989529945, 191.1210336056979884 ) ) ;
#91397=EDGE_LOOP ( 'NONE', ( #37808, #84595, #6737, #54562, #42193 ) ) ;
#91401=CARTESIAN_POINT ( 'NONE',  ( 40.88256439680969834, 1440.913060387330006, 268.3738206050749682 ) ) ;
#91403=CARTESIAN_POINT ( 'NONE',  ( -0.0005080901876549786828, 1451.974260998641057, 153.9770172106709936 ) ) ;
#91404=ORIENTED_EDGE ( 'NONE', *, *, #80321, .T. ) ;
#91410=CARTESIAN_POINT ( 'NONE',  ( 12.84239221398829933, 1435.935692713660046, 150.8114773724069835 ) ) ;
#91411=CARTESIAN_POINT ( 'NONE',  ( 30.02767535379999941, 1414.536195395429786, 266.6069031101980045 ) ) ;
#91412=CARTESIAN_POINT ( 'NONE',  ( -12.40432178540000052, 1434.419968829250138, 147.8552690333980308 ) ) ;
#91414=CARTESIAN_POINT ( 'NONE',  ( 14.78718726039999787, 1460.545059401930075, 230.6966295517979688 ) ) ;
#91415=CARTESIAN_POINT ( 'NONE',  ( -11.60004869885203505, 1422.462482050413655, 137.0350105543709844 ) ) ;
#91418=VERTEX_POINT ( 'NONE', #52372 ) ;
#91419=CIRCLE ( 'NONE', #244, 8.000000000000007105 ) ;
#91422=CARTESIAN_POINT ( 'NONE',  ( -0.06741725946591989316, 1508.620385720349987, 180.1145002095929897 ) ) ;
#91423=CARTESIAN_POINT ( 'NONE',  ( 16.70757379908175722, 1449.396063251830583, 219.0502673354835679 ) ) ;
#91425=CARTESIAN_POINT ( 'NONE',  ( 18.51562415000000072, 1509.322649222929840, 187.7614736601980212 ) ) ;
#91426=CARTESIAN_POINT ( 'NONE',  ( -11.44617051164304833, 1425.796922195610705, 139.1405492985841477 ) ) ;
#91430=CARTESIAN_POINT ( 'NONE',  ( 16.70417082779999873, 1456.998411956430118, 221.6179017295980032 ) ) ;
#91431=CARTESIAN_POINT ( 'NONE',  ( -11.57526502019999981, 1432.244206860189934, 151.1962845448979920 ) ) ;
#91432=CARTESIAN_POINT ( 'NONE',  ( 19.08296562770900096, 1456.929326075580093, 225.1994806392700070 ) ) ;
#91436=CARTESIAN_POINT ( 'NONE',  ( 12.40489012449999962, 1446.137994316120057, 188.0544017187980046 ) ) ;
#91437=CARTESIAN_POINT ( 'NONE',  ( -20.58707005339999796, 1482.729478077029853, 226.3829017035980087 ) ) ;
#91438=FACE_OUTER_BOUND ( 'NONE', #71034, .T. ) ;
#91439=CARTESIAN_POINT ( 'NONE',  ( -1.687592144759999968, 1484.749778137530029, 182.6858646861979878 ) ) ;
#91442=CARTESIAN_POINT ( 'NONE',  ( 7.054183505060000137, 1406.398142208129912, 266.9413180379979735 ) ) ;
#91443=CARTESIAN_POINT ( 'NONE',  ( 38.64637139974560398, 1443.913060387190171, 137.1864063390110005 ) ) ;
#91445=CARTESIAN_POINT ( 'NONE',  ( 22.91305534397972465, 1432.047512284617142, 216.2803340805854475 ) ) ;
#91446=DIRECTION ( 'NONE',  ( 0.000000000000000000, 1.000000000000000000, 0.000000000000000000 ) ) ;
#91450=CARTESIAN_POINT ( 'NONE',  ( -1.459574862452099886, 1450.689303299579933, 154.7904098955449967 ) ) ;
#91451=CARTESIAN_POINT ( 'NONE',  ( -1.561820929657351309, 1450.950381850439953, 183.5281567525138655 ) ) ;
#91452=LINE ( 'NONE', #22550, #49732 ) ;
#91455=CARTESIAN_POINT ( 'NONE',  ( -17.83186622659999898, 1434.542072767570062, 214.3676144203579952 ) ) ;
#91456=CARTESIAN_POINT ( 'NONE',  ( -27.08287658454329971, 1507.996869902240178, 211.2978356732120062 ) ) ;
#91457=CARTESIAN_POINT ( 'NONE',  ( 2.500000002550000211, 1439.653804531360038, 157.1389828242980116 ) ) ;
#91458=AXIS2_PLACEMENT_3D ( 'NONE', #36124, #69184, #1413 ) ;
#91459=CARTESIAN_POINT ( 'NONE',  ( -3.436075876849999933, 1475.886457539630101, 267.2300234903979685 ) ) ;
#91462=CARTESIAN_POINT ( 'NONE',  ( 17.71056690938649680, 1414.273744580000084, 224.2882958007120067 ) ) ;
#91464=CARTESIAN_POINT ( 'NONE',  ( 16.78507865760100159, 1507.483738429089954, 193.5970331257109933 ) ) ;
#91468=CARTESIAN_POINT ( 'NONE',  ( -20.12576653420000028, 1409.615867641330169, 201.4144580155179938 ) ) ;
#91471=CARTESIAN_POINT ( 'NONE',  ( -30.65556899779999966, 1416.265499210330063, 269.9312797238980011 ) ) ;
#91474=CARTESIAN_POINT ( 'NONE',  ( -2.869563509691151371, 1410.390895325194833, 232.5635847210010070 ) ) ;
#91477=CARTESIAN_POINT ( 'NONE',  ( 11.67374344909999984, 1426.737914103830008, 139.6438984324979913 ) ) ;
#91484=CARTESIAN_POINT ( 'NONE',  ( -12.87605230667369405, 1398.294690222690406, 210.9476564090868749 ) ) ;
#91492=VERTEX_POINT ( 'NONE', #54583 ) ;
#91493=CARTESIAN_POINT ( 'NONE',  ( 11.45756101023500051, 1434.780485529720181, 151.4565597636700147 ) ) ;
#91495=CARTESIAN_POINT ( 'NONE',  ( -12.38973388049999969, 1396.865112417229966, 211.4033042261380047 ) ) ;
#91496=CARTESIAN_POINT ( 'NONE',  ( -20.64057905079999955, 1409.633845290530189, 214.6320756031479959 ) ) ;
#91498=CARTESIAN_POINT ( 'NONE',  ( -12.57974774915637717, 1445.046023591448829, 169.4706963785791061 ) ) ;
#91502=CARTESIAN_POINT ( 'NONE',  ( 17.93995879599999910, 1421.703940548830133, 225.5244287617980206 ) ) ;
#91503=CARTESIAN_POINT ( 'NONE',  ( 1.315358370620000050, 1449.240786182220063, 183.5913257811980088 ) ) ;
#91505=EDGE_CURVE ( 'NONE', #6406, #100495, #16291, .T. ) ;
#91507=CARTESIAN_POINT ( 'NONE',  ( 10.75712941972539838, 1396.288707624410108, 206.5173657439860335 ) ) ;
#91508=LINE ( 'NONE', #76361, #26556 ) ;
#91509=CARTESIAN_POINT ( 'NONE',  ( 11.80251472770000021, 1427.996663069729948, 148.7256247452979778 ) ) ;
#91510=CARTESIAN_POINT ( 'NONE',  ( 1.716045945209999868, 1509.007693206030126, 179.5167849949980052 ) ) ;
#91512=CARTESIAN_POINT ( 'NONE',  ( 12.95810389287730047, 1435.988623967140029, 150.7629203163199918 ) ) ;
#91513=VERTEX_POINT ( 'NONE', #89253 ) ;
#91515=CARTESIAN_POINT ( 'NONE',  ( -17.75009271329319915, 1468.179955452010063, 228.4966567787849954 ) ) ;
#91516=CARTESIAN_POINT ( 'NONE',  ( -5.135155612019999261, 1464.351819601929947, 236.1467049461980139 ) ) ;
#91523=CARTESIAN_POINT ( 'NONE',  ( 2.500000000000000000, 1448.210448412289907, 170.5244215879980061 ) ) ;
#91526=ORIENTED_EDGE ( 'NONE', *, *, #80879, .F. ) ;
#91528=ORIENTED_EDGE ( 'NONE', *, *, #71923, .F. ) ;
#91530=CARTESIAN_POINT ( 'NONE',  ( -20.18532072600000049, 1508.602711282829887, 229.1243101363980088 ) ) ;
#91531=CARTESIAN_POINT ( 'NONE',  ( -29.88849338478334161, 1419.495351112958360, 269.4696191733103205 ) ) ;
#91533=CARTESIAN_POINT ( 'NONE',  ( -1.190628175403880107, 1414.913057834419988, 226.0043277146490084 ) ) ;
#91534=ORIENTED_EDGE ( 'NONE', *, *, #80321, .F. ) ;
#91535=CARTESIAN_POINT ( 'NONE',  ( 24.59498516420000058, 1440.913044728469913, 213.3385258196480265 ) ) ;
#91536=CARTESIAN_POINT ( 'NONE',  ( -27.79719865735470208, 1440.913060392109855, 230.3218327024129906 ) ) ;
#91540=CARTESIAN_POINT ( 'NONE',  ( 4.958608739790000719, 1408.764127645530152, 270.4263178542980768 ) ) ;
#91542=CARTESIAN_POINT ( 'NONE',  ( 22.69544225309999774, 1409.705575941829920, 209.0104250642420141 ) ) ;
#91543=CARTESIAN_POINT ( 'NONE',  ( -21.68655196239999938, 1509.722744064730023, 188.6979275785979837 ) ) ;
#91548=CARTESIAN_POINT ( 'NONE',  ( 0.09565136837490001431, 1420.220989488129817, 183.9056119367980102 ) ) ;
#91549=CARTESIAN_POINT ( 'NONE',  ( -11.67160011230928340, 1486.022816546380454, 184.5451946457169186 ) ) ;
#91553=CIRCLE ( 'NONE', #66559, 39.37709583113206691 ) ;
#91554=CARTESIAN_POINT ( 'NONE',  ( 45.31156206859999713, 1446.488581015689988, 266.2044087351980011 ) ) ;
#91556=B_SPLINE_CURVE_WITH_KNOTS ( 'NONE', 3,
 ( #42884, #68651, #9821, #51275, #102752, #15994, #84856, #110079, #110629, #69199, #25500, #51841, #59691, #52404, #94935, #103306, #7613, #349, #93803, #41769, #50196, #8156, #33354, #17080, #67549 ),
 .UNSPECIFIED., .F., .F.,
 ( 4, 1, 1, 2, 2, 2, 1, 2, 2, 2, 2, 2, 2, 4 ),
 ( 0.000000000000000000, 0.1250000000001981193, 0.1875000000002736422, 0.2187500000002864931, 0.2500000000002993716, 0.3750000000003361200, 0.4375000000003544387, 0.4687500000003027578, 0.5000000000002510214, 0.6250000000002813305, 0.6875000000002928768, 0.7500000000003043121, 0.8750000000001521006, 1.000000000000000000 ),
 .UNSPECIFIED. ) ;
#91558=CARTESIAN_POINT ( 'NONE',  ( -5.451409632509999881, 1437.905383012069933, 154.7243395035980029 ) ) ;
#91560=CARTESIAN_POINT ( 'NONE',  ( 0.3987454328862090058, 1452.975505999449979, 183.2778484764669997 ) ) ;
#91569=CARTESIAN_POINT ( 'NONE',  ( -0.1694244116599999961, 1487.208880437030075, 230.4477740473979850 ) ) ;
#91570=CARTESIAN_POINT ( 'NONE',  ( 23.13311796429999845, 1449.197330723620098, 218.1771922301180098 ) ) ;
#91575=CARTESIAN_POINT ( 'NONE',  ( 25.25200551730000242, 1450.804230319249882, 137.6134878989979882 ) ) ;
#91576=CARTESIAN_POINT ( 'NONE',  ( 15.58582549078360380, 1420.996909499524236, 227.6524987713947894 ) ) ;
#91577=CARTESIAN_POINT ( 'NONE',  ( -38.64637139473789773, 1443.913060387190171, 137.1864063576500143 ) ) ;
#91578=CARTESIAN_POINT ( 'NONE',  ( -19.44347141579999771, 1426.034560796430014, 223.5248983639980054 ) ) ;
#91579=CARTESIAN_POINT ( 'NONE',  ( -28.97201236651673995, 1467.320980035921593, 269.3759728919557688 ) ) ;
#91581=CARTESIAN_POINT ( 'NONE',  ( 12.71733191150000053, 1509.357159403529977, 183.2206200378979872 ) ) ;
#91583=CARTESIAN_POINT ( 'NONE',  ( -35.02259794696599471, 1457.750285243617100, 269.5318678299763064 ) ) ;
#91586=CARTESIAN_POINT ( 'NONE',  ( 6.599306557268372231, 1506.776553301877129, 187.7051843307115462 ) ) ;
#91588=CARTESIAN_POINT ( 'NONE',  ( -0.2027342012590000186, 1416.110316472029808, 233.5455375878979964 ) ) ;
#91589=CARTESIAN_POINT ( 'NONE',  ( -13.42860621949387934, 1443.470021403052897, 187.0641147421139578 ) ) ;
#91592=CARTESIAN_POINT ( 'NONE',  ( -3.565261586666695681, 1415.863973584654332, 232.5973463957437843 ) ) ;
#91595=CARTESIAN_POINT ( 'NONE',  ( -12.53380499174499896, 1442.773887286369927, 169.4755105688890069 ) ) ;
#91598=CARTESIAN_POINT ( 'NONE',  ( 0.05152562430226129836, 1416.529254608160045, 190.9681162060270196 ) ) ;
#91599=CARTESIAN_POINT ( 'NONE',  ( 21.94594828856675051, 1509.533994805570501, 226.8419239637491955 ) ) ;
#91600=ORIENTED_EDGE ( 'NONE', *, *, #73887, .F. ) ;
#91601=ORIENTED_EDGE ( 'NONE', *, *, #110159, .T. ) ;
#91602=CARTESIAN_POINT ( 'NONE',  ( 16.93365818059630001, 1414.971717244350202, 209.8484561376429838 ) ) ;
#91604=CARTESIAN_POINT ( 'NONE',  ( 41.26157930654738237, 1435.022522197726857, 269.6335040890825780 ) ) ;
#91605=CARTESIAN_POINT ( 'NONE',  ( -25.74056221470000239, 1442.596569739780080, 220.8687942055980216 ) ) ;
#91607=CARTESIAN_POINT ( 'NONE',  ( -11.88353474240000018, 1433.300648518049911, 150.2496884404980051 ) ) ;
#91609=CARTESIAN_POINT ( 'NONE',  ( 27.15450531368009734, 1482.666413628910050, 209.4389354641179750 ) ) ;
#91610=CARTESIAN_POINT ( 'NONE',  ( -26.84000540299999926, 1441.581970623780080, 137.4710795974980329 ) ) ;
#91611=CARTESIAN_POINT ( 'NONE',  ( -14.40908221889993790, 1429.715078873349512, 222.2182523075439633 ) ) ;
#91613=CARTESIAN_POINT ( 'NONE',  ( 1.940237629179999868, 1450.366509861609757, 181.9011059340980125 ) ) ;
#91615=CARTESIAN_POINT ( 'NONE',  ( -10.85473188425545565, 1509.417389448126414, 237.0896451841293526 ) ) ;
#91616=CARTESIAN_POINT ( 'NONE',  ( 1.565460387769590331E-08, 1407.727994899569921, 263.5611240349619493 ) ) ;
#91620=CARTESIAN_POINT ( 'NONE',  ( -11.82802681128099920, 1429.780949742419807, 149.3576024833930092 ) ) ;
#91622=CARTESIAN_POINT ( 'NONE',  ( -6.437126621210000010, 1473.252205434630241, 270.3863109987980238 ) ) ;
#91626=CARTESIAN_POINT ( 'NONE',  ( 0.000000000000000000, 1405.413060387330006, 209.1218459616979999 ) ) ;
#91627=CARTESIAN_POINT ( 'NONE',  ( 7.105427357599999217E-15, 1405.913060387330006, 137.0999999980979851 ) ) ;
#91628=EDGE_CURVE ( 'NONE', #56546, #11723, #36651, .T. ) ;
#91632=CARTESIAN_POINT ( 'NONE',  ( -28.98944848162919996, 1413.705768742049941, 268.7096924078339839 ) ) ;
#91633=ORIENTED_EDGE ( 'NONE', *, *, #105010, .T. ) ;
#91635=ORIENTED_EDGE ( 'NONE', *, *, #83599, .F. ) ;
#91639=CARTESIAN_POINT ( 'NONE',  ( 41.62830255093239629, 1444.039180007019922, 135.9573986949209825 ) ) ;
#91642=CARTESIAN_POINT ( 'NONE',  ( -9.692726333870000488, 1440.427639384229906, 186.8581189109980301 ) ) ;
#91644=CARTESIAN_POINT ( 'NONE',  ( -18.58720762869999987, 1416.311719779230089, 208.5274638254259969 ) ) ;
#91646=CARTESIAN_POINT ( 'NONE',  ( -26.49726434420000132, 1436.728585065589868, 136.8015681357979929 ) ) ;
#91649=CARTESIAN_POINT ( 'NONE',  ( -41.14893945019565535, 1446.681898757845147, 135.2730607365670608 ) ) ;
#91650=CARTESIAN_POINT ( 'NONE',  ( 0.9227939322070656258, 1508.990480019933557, 238.8126630289496575 ) ) ;
#91651=CARTESIAN_POINT ( 'NONE',  ( -27.35670215475310130, 1417.239247989339901, 269.9340778386260240 ) ) ;
#91653=CARTESIAN_POINT ( 'NONE',  ( -5.033438044520000432, 1397.146222143329851, 197.2622438200980071 ) ) ;
#91657=CARTESIAN_POINT ( 'NONE',  ( 0.3552831700869999998, 1450.900653625639961, 181.9147599137979796 ) ) ;
#91658=CARTESIAN_POINT ( 'NONE',  ( 3.809629103879523804, 1425.717714542633303, 185.2543070201454043 ) ) ;
#91660=CARTESIAN_POINT ( 'NONE',  ( -24.46729980500000323, 1435.535532743930162, 137.3091962579979963 ) ) ;
#91661=CARTESIAN_POINT ( 'NONE',  ( -0.4542904894729999921, 1486.188528289530041, 181.7644461267980205 ) ) ;
#91664=CARTESIAN_POINT ( 'NONE',  ( 5.449707646490000279, 1437.831544062859848, 154.7230940508980268 ) ) ;
#91666=DIRECTION ( 'NONE',  ( -1.000000000000000000, -5.823966869780190178E-19, 4.137698748469999823E-18 ) ) ;
#91670=CARTESIAN_POINT ( 'NONE',  ( -2.745249273916440469, 1451.958939284520056, 184.7272525765399962 ) ) ;
#91672=CARTESIAN_POINT ( 'NONE',  ( -19.60719674227114240, 1457.056223723324820, 225.8784467642674656 ) ) ;
#91675=CARTESIAN_POINT ( 'NONE',  ( -22.66501075923255826, 1509.725766826326435, 228.1954490747540376 ) ) ;
#91676=CARTESIAN_POINT ( 'NONE',  ( -4.148978217093812759, 1439.755697323768118, 185.4934640260758556 ) ) ;
#91678=CARTESIAN_POINT ( 'NONE',  ( 24.13017307760000207, 1452.070412388429986, 136.4016798020979877 ) ) ;
#91679=CARTESIAN_POINT ( 'NONE',  ( 3.472242611860356210, 1450.898212748911419, 184.0506856000464779 ) ) ;
#91681=CARTESIAN_POINT ( 'NONE',  ( 2.387854443607448918, 1426.854124017601634, 138.5187392187245052 ) ) ;
#91682=CARTESIAN_POINT ( 'NONE',  ( 23.07346110646793491, 1450.308246357729104, 217.9087771107495541 ) ) ;
#91683=CARTESIAN_POINT ( 'NONE',  ( -11.94206337009999963, 1438.199233188169956, 150.9847479746979957 ) ) ;
#91686=ORIENTED_EDGE ( 'NONE', *, *, #39244, .F. ) ;
#91688=DIRECTION ( 'NONE',  ( 3.446748568029901836E-05, -0.9328683086395049839, -0.3602175974991528862 ) ) ;
#91691=EDGE_CURVE ( 'NONE', #78256, #46740, #32321, .T. ) ;
#91694=CARTESIAN_POINT ( 'NONE',  ( 11.60004869885203505, 1426.109591897770542, 139.1549358429673759 ) ) ;
#91696=B_SPLINE_CURVE_WITH_KNOTS ( 'NONE', 3,
 ( #110783, #25102, #49789, #34074, #109684, #57654, #50887, #83923, #101810, #59308, #93421, #75549, #42472, #83364, #50353, #108577, #32428, #91766, #68267 ),
 .UNSPECIFIED., .F., .F.,
 ( 4, 3, 3, 3, 3, 3, 4 ),
 ( -1.000000000000000000, -0.7168501403031710684, -0.3505194570518059827, -0.001863983869921592706, 0.3397317646628350563, 0.6718016826570070155, 1.000000000000000000 ),
 .UNSPECIFIED. ) ;
#91697=CARTESIAN_POINT ( 'NONE',  ( 17.14350470404602333, 1422.299115860800157, 226.7520998961785494 ) ) ;
#91701=CARTESIAN_POINT ( 'NONE',  ( 28.40112187179950354, 1440.913060387299993, 232.7382060992320021 ) ) ;
#91705=CARTESIAN_POINT ( 'NONE',  ( 12.90626675129999867, 1419.889181702930046, 222.0924173487979658 ) ) ;
#91706=ORIENTED_EDGE ( 'NONE', *, *, #57560, .T. ) ;
#91707=ORIENTED_EDGE ( 'NONE', *, *, #30538, .F. ) ;
#91709=CARTESIAN_POINT ( 'NONE',  ( -19.67951034195003146, 1485.238740488470739, 190.3370758437304175 ) ) ;
#91710=CARTESIAN_POINT ( 'NONE',  ( -0.3788383082595139784, 1408.926289712549988, 186.6322538385570056 ) ) ;
#91713=CARTESIAN_POINT ( 'NONE',  ( 14.43289921540000087, 1509.539432541030010, 235.4218729623979982 ) ) ;
#91736=CARTESIAN_POINT ( 'NONE',  ( 3.933988272389480123, 1409.050438284940128, 194.6660132622929780 ) ) ;
#91737=CARTESIAN_POINT ( 'NONE',  ( 0.2331197489560000169, 1408.921201108330024, 186.4825419995979985 ) ) ;
#91740=CARTESIAN_POINT ( 'NONE',  ( -3.119435209982429846, 1441.198230638479799, 165.1033167001029938 ) ) ;
#91742=EDGE_LOOP ( 'NONE', ( #4605, #71247, #37651 ) ) ;
#91744=CARTESIAN_POINT ( 'NONE',  ( 19.22912473335630423, 1456.153986460939905, 226.8534579158520046 ) ) ;
#91745=CARTESIAN_POINT ( 'NONE',  ( -12.78772699639999999, 1434.671431919079851, 149.7610961743979772 ) ) ;
#91746=CARTESIAN_POINT ( 'NONE',  ( -8.321770097687579715E-10, 1467.826180283610029, 247.7074370028710177 ) ) ;
#91749=DIRECTION ( 'NONE',  ( 1.000000000000000000, 0.000000000000000000, 0.000000000000000000 ) ) ;
#91751=CARTESIAN_POINT ( 'NONE',  ( -1.466185886320000131, 1484.851694392830041, 182.4600082771979999 ) ) ;
#91753=FACE_OUTER_BOUND ( 'NONE', #95800, .T. ) ;
#91754=CARTESIAN_POINT ( 'NONE',  ( 13.60272764034519888, 1508.889111070959871, 233.6609499386090079 ) ) ;
#91757=CARTESIAN_POINT ( 'NONE',  ( -21.03123196678649975, 1507.789098018889945, 192.1781278620359785 ) ) ;
#91762=CARTESIAN_POINT ( 'NONE',  ( -7.369671095600000695E-09, 1422.147183830129961, 212.8701394402079927 ) ) ;
#91763=CARTESIAN_POINT ( 'NONE',  ( -28.13115138559999906, 1508.134099163530209, 208.1186796399779837 ) ) ;
#91764=CARTESIAN_POINT ( 'NONE',  ( -3.527537870079999749, 1486.454657621929982, 181.8568875002980292 ) ) ;
#91766=CARTESIAN_POINT ( 'NONE',  ( -2.850245122384609697, 1419.522424184869806, 186.1943312919690072 ) ) ;
#91767=CARTESIAN_POINT ( 'NONE',  ( -26.35128651260000154, 1437.443204552669840, 225.2418051465980113 ) ) ;
#91768=CARTESIAN_POINT ( 'NONE',  ( -29.51860354171773082, 1509.963695514703204, 206.5604812588238985 ) ) ;
#91769=CARTESIAN_POINT ( 'NONE',  ( -21.13360565959400006, 1452.175058615539911, 141.7927856989660143 ) ) ;
#91770=CARTESIAN_POINT ( 'NONE',  ( 29.26105829599999808, 1451.435244290330047, 136.0815397235980129 ) ) ;
#91772=CARTESIAN_POINT ( 'NONE',  ( -5.367153005107930142, 1426.308048638930131, 152.5548644906199911 ) ) ;
#91774=CARTESIAN_POINT ( 'NONE',  ( 16.73020750861299888, 1423.490444015980074, 228.1585555744700002 ) ) ;
#91777=EDGE_LOOP ( 'NONE', ( #75024, #56829, #74309, #93016 ) ) ;
#91779=CARTESIAN_POINT ( 'NONE',  ( -23.49170351482609931, 1410.011808632399834, 209.6547519446870069 ) ) ;
#91785=CARTESIAN_POINT ( 'NONE',  ( -4.792740298340000038, 1507.637309065929912, 236.3818457613980115 ) ) ;
#91786=CARTESIAN_POINT ( 'NONE',  ( -18.04342283379999756, 1410.879798814630021, 224.6982261388980078 ) ) ;
#91787=ORIENTED_EDGE ( 'NONE', *, *, #15607, .F. ) ;
#91788=CARTESIAN_POINT ( 'NONE',  ( 41.71199689262579824, 1455.342431078719983, 268.8818206049920150 ) ) ;
#91791=CARTESIAN_POINT ( 'NONE',  ( 0.006268853705600000749, 1420.201965319130068, 183.8994898050980282 ) ) ;
#91797=ORIENTED_EDGE ( 'NONE', *, *, #12860, .F. ) ;
#91804=CARTESIAN_POINT ( 'NONE',  ( 22.63852601520000007, 1409.703615135929795, 209.5818420717589845 ) ) ;
#91807=CARTESIAN_POINT ( 'NONE',  ( 2.005245171522929581, 1408.983085091729890, 186.9291916408829763 ) ) ;
#91809=CARTESIAN_POINT ( 'NONE',  ( 10.20313649189779959, 1171.102791779800100, 156.7234425824970003 ) ) ;
#91813=CARTESIAN_POINT ( 'NONE',  ( 11.84242369139999873, 1431.324257919750153, 147.6543138610979895 ) ) ;
#91815=CARTESIAN_POINT ( 'NONE',  ( 12.70951029399999932, 1416.237488680629895, 222.2791103869979850 ) ) ;
#91816=CARTESIAN_POINT ( 'NONE',  ( -11.63668813159994286, 1425.864839735430678, 144.1681848196939768 ) ) ;
#91819=EDGE_CURVE ( 'NONE', #39980, #45174, #85876, .T. ) ;
#91821=CARTESIAN_POINT ( 'NONE',  ( 4.758677794462281341, 1427.076634120264089, 137.0999999980979567 ) ) ;
#91823=ADVANCED_FACE ( 'NONE', ( #92005 ), #19721, .T. ) ;
#91827=CARTESIAN_POINT ( 'NONE',  ( 11.93819009070000092, 1433.480077612689911, 149.8972056143980183 ) ) ;
#91828=CARTESIAN_POINT ( 'NONE',  ( 34.97756116859999764, 1449.243413927999882, 262.6648722511980054 ) ) ;
#91829=CARTESIAN_POINT ( 'NONE',  ( 1.108081647679679982, 1450.800742795999895, 181.4825116590070024 ) ) ;
#91830=CARTESIAN_POINT ( 'NONE',  ( -11.60004869885205636, 1428.977684734793911, 135.1000015630646089 ) ) ;
#91831=CARTESIAN_POINT ( 'NONE',  ( -5.164876290100000489, 1519.913060387329779, 231.9023197776979828 ) ) ;
#91835=CARTESIAN_POINT ( 'NONE',  ( 22.98253439269999987, 1410.218983183530099, 207.4712557340779995 ) ) ;
#91838=CARTESIAN_POINT ( 'NONE',  ( -17.84188412740000018, 1410.460489672530230, 225.0030837357979863 ) ) ;
#91839=CARTESIAN_POINT ( 'NONE',  ( 20.06299576540000018, 1508.017094725129937, 189.2032669109979963 ) ) ;
#91840=EDGE_CURVE ( 'NONE', #52837, #98127, #44445, .T. ) ;
#91842=CARTESIAN_POINT ( 'NONE',  ( 2.566893074593609807E-08, 1406.911841303630126, 196.1218459607310081 ) ) ;
#91845=B_SPLINE_CURVE_WITH_KNOTS ( 'NONE', 3,
 ( #15433, #16521, #69187, #93257, #883, #84308, #18195, #69752, #60227, #52392, #335, #85394, #85966, #78113, #101635, #59677, #33898, #26599, #35556, #15980, #76462, #33341, #84842, #92702, #50181, #1417, #68093, #102206, #7600, #67536, #110615, #102738, #59135, #86515, #94346, #9808, #25486, #93789, #41754, #103293, #75913, #17623, #26033, #17064, #24925, #68638, #50712, #51261, #103870, #110065, #77575, #8690, #8142, #60796, #35006, #42872 ),
 .UNSPECIFIED., .F., .F.,
 ( 4, 2, 2, 1, 2, 2, 2, 1, 1, 2, 2, 2, 2, 1, 1, 2, 2, 2, 2, 2, 1, 1, 2, 2, 2, 2, 1, 1, 1, 2, 2, 2, 4 ),
 ( 0.000000000000000000, 0.03125000000081699925, 0.04687500000111776560, 0.05468750000126820776, 0.05859375000134336986, 0.06250000000141853196, 0.09375000000176267334, 0.1093750000018305218, 0.1171875000017644497, 0.1210937500016381063, 0.1250000000015117629, 0.1875000000004202749, 0.2187499999998744615, 0.2343749999996015687, 0.2421874999994600985, 0.2460937499993843258, 0.2499999999993085253, 0.3749999999989888644, 0.4374999999987320143, 0.4687499999985955679, 0.4843749999984700016, 0.4921874999984772181, 0.4960937499985410559, 0.4999999999986049493, 0.6250000000006696865, 0.6875000000017634783, 0.7187500000022626345, 0.7343750000025426328, 0.7421875000026716407, 0.7460937500027362557, 0.7500000000028008706, 0.8750000000014004353, 1.000000000000000000 ),
 .UNSPECIFIED. ) ;
#91846=CARTESIAN_POINT ( 'NONE',  ( -6.036595121079999515, 1415.425582719929707, 225.8522314191980058 ) ) ;
#91848=CARTESIAN_POINT ( 'NONE',  ( 0.1723280242880049773, 1478.963607770360113, 182.1389088959510048 ) ) ;
#91849=CARTESIAN_POINT ( 'NONE',  ( -2.803523226207980112, 1407.337701542270224, 222.1242196241450131 ) ) ;
#91851=CARTESIAN_POINT ( 'NONE',  ( -16.90742463042001376, 1444.994950788469623, 162.4348201727408991 ) ) ;
#91853=CARTESIAN_POINT ( 'NONE',  ( 11.87950672170000033, 1433.311310111189869, 147.9453571599980251 ) ) ;
#91854=CARTESIAN_POINT ( 'NONE',  ( -41.46889560185230295, 1441.954934107629924, 134.0999999980859911 ) ) ;
#91856=ORIENTED_EDGE ( 'NONE', *, *, #30249, .F. ) ;
#91863=ADVANCED_FACE ( 'NONE', ( #103143 ), #18782, .T. ) ;
#91865=CARTESIAN_POINT ( 'NONE',  ( -46.15243904500000127, 1440.913037427970266, 268.2044236447979983 ) ) ;
#91868=CARTESIAN_POINT ( 'NONE',  ( 2.500000000000000000, 1439.615672362369878, 182.7715267708979923 ) ) ;
#91872=ORIENTED_EDGE ( 'NONE', *, *, #95259, .F. ) ;
#91874=CARTESIAN_POINT ( 'NONE',  ( -29.31938507799999982, 1451.735856109730094, 135.7220070057980195 ) ) ;
#91875=CARTESIAN_POINT ( 'NONE',  ( -15.82357197924079806, 1409.473877788359914, 225.4813571472639921 ) ) ;
#91877=VERTEX_POINT ( 'NONE', #55538 ) ;
#91880=CARTESIAN_POINT ( 'NONE',  ( 16.93236825731289841, 1416.913057013589878, 210.7966595891460031 ) ) ;
#91882=CARTESIAN_POINT ( 'NONE',  ( -0.07495072822490929376, 1420.236531064540031, 183.6031585757189930 ) ) ;
#91883=CARTESIAN_POINT ( 'NONE',  ( 19.61574826060000021, 1409.598057419529823, 218.7671105721680078 ) ) ;
#91884=CARTESIAN_POINT ( 'NONE',  ( -1.977028453051359991, 1417.217131934150075, 185.9238632041590051 ) ) ;
#91885=CARTESIAN_POINT ( 'NONE',  ( -17.72483192860000045, 1424.402862424130035, 227.6947415401980095 ) ) ;
#91887=CARTESIAN_POINT ( 'NONE',  ( 2.500000000000000000, 1425.929641634319978, 183.3886485707629959 ) ) ;
#91889=CARTESIAN_POINT ( 'NONE',  ( 23.32695134950520099, 1509.740226291735098, 190.9604462070601016 ) ) ;
#91892=CARTESIAN_POINT ( 'NONE',  ( -5.376660071774439942, 1485.139014803799910, 183.5235869889660023 ) ) ;
#91895=CARTESIAN_POINT ( 'NONE',  ( -4.227095715345259741, 1441.558630613729974, 165.7615266881739728 ) ) ;
#91898=CARTESIAN_POINT ( 'NONE',  ( -15.63365311440000127, 1422.686384262629872, 229.4762402829979919 ) ) ;
#91902=CARTESIAN_POINT ( 'NONE',  ( -11.73848972823176062, 1426.695089812134484, 144.2749369092671827 ) ) ;
#91903=CARTESIAN_POINT ( 'NONE',  ( 16.10936821303920041, 1409.855324947380041, 191.9958954789800032 ) ) ;
#91905=EDGE_CURVE ( 'NONE', #92411, #71735, #1836, .T. ) ;
#91907=CARTESIAN_POINT ( 'NONE',  ( 41.10105618305409791, 1442.565812537450029, 136.7947891895450141 ) ) ;
#91908=CARTESIAN_POINT ( 'NONE',  ( 33.91369278643569629, 1437.010534640189690, 136.5611839302279691 ) ) ;
#91912=CARTESIAN_POINT ( 'NONE',  ( 34.05830400097580224, 1451.723718204009856, 134.0999999980979851 ) ) ;
#91913=PLANE ( 'NONE',  #38216 ) ;
#91916=FACE_OUTER_BOUND ( 'NONE', #42365, .T. ) ;
#91917=VERTEX_POINT ( 'NONE', #11869 ) ;
#91920=CYLINDRICAL_SURFACE ( 'NONE', #3789, 1.455175085940000335 ) ;
#91921=FACE_OUTER_BOUND ( 'NONE', #41551, .T. ) ;
#91922=EDGE_CURVE ( 'NONE', #56404, #60533, #46469, .T. ) ;
#91923=CARTESIAN_POINT ( 'NONE',  ( -0.07496883016649999454, 1450.915678356330091, 181.8856722418979928 ) ) ;
#91924=CARTESIAN_POINT ( 'NONE',  ( -3.260695655560000183, 1485.137811735230116, 183.2004311182980132 ) ) ;
#91928=CARTESIAN_POINT ( 'NONE',  ( 11.91277487560000026, 1442.215011169370200, 187.5867736087979836 ) ) ;
#91929=CARTESIAN_POINT ( 'NONE',  ( 40.71747595839759981, 1448.637563203230002, 135.3769927381360105 ) ) ;
#91930=CARTESIAN_POINT ( 'NONE',  ( 4.363122683464830232, 1421.971318488559973, 183.8271341761570170 ) ) ;
#91931=CARTESIAN_POINT ( 'NONE',  ( 26.87614569890000027, 1439.497608261269761, 137.1020444149980051 ) ) ;
#91938=CARTESIAN_POINT ( 'NONE',  ( 39.78035207931749540, 1440.913060387330006, 267.1197271637229278 ) ) ;
#91939=EDGE_CURVE ( 'NONE', #2071, #101781, #7444, .T. ) ;
#91940=CARTESIAN_POINT ( 'NONE',  ( -0.0002562030068480412176, 1452.575673631712561, 153.5027436610795917 ) ) ;
#91942=CARTESIAN_POINT ( 'NONE',  ( -13.36846539809999967, 1415.041103189330215, 220.6286931108980127 ) ) ;
#91946=CARTESIAN_POINT ( 'NONE',  ( 21.74459043622260168, 1409.809204975360217, 206.3233155530909926 ) ) ;
#91951=CARTESIAN_POINT ( 'NONE',  ( 25.71940137246620139, 1482.323570389569795, 206.2243813634200080 ) ) ;
#91952=CARTESIAN_POINT ( 'NONE',  ( 14.85640376749999980, 1461.023002278929880, 230.2637214827979903 ) ) ;
#91954=CARTESIAN_POINT ( 'NONE',  ( -4.363122647530000009, 1414.776585547029981, 163.8086717993979846 ) ) ;
#91958=CARTESIAN_POINT ( 'NONE',  ( -0.1147649368047699986, 1508.126957518789823, 180.5760551733519890 ) ) ;
#91961=EDGE_CURVE ( 'NONE', #86293, #18369, #87054, .T. ) ;
#91962=CARTESIAN_POINT ( 'NONE',  ( 18.49117119079999938, 1508.844092021829965, 188.2543554912979857 ) ) ;
#91963=CARTESIAN_POINT ( 'NONE',  ( -10.92124405496922002, 1424.881793267335979, 138.2645581544207971 ) ) ;
#91965=VERTEX_POINT ( 'NONE', #13485 ) ;
#91967=CARTESIAN_POINT ( 'NONE',  ( 25.89198661300000026, 1442.605201390229922, 221.6500998664980102 ) ) ;
#91969=CARTESIAN_POINT ( 'NONE',  ( -11.85363313409999897, 1431.417378487679798, 150.3276964087979763 ) ) ;
#91970=CARTESIAN_POINT ( 'NONE',  ( 11.73709356400000026, 1426.695943141129874, 144.1748013759980154 ) ) ;
#91972=CARTESIAN_POINT ( 'NONE',  ( 9.267034410570261116, 1423.582047773290014, 146.9531695596949987 ) ) ;
#91974=CARTESIAN_POINT ( 'NONE',  ( 12.65231296470000188, 1445.580367743630177, 187.9555106065979828 ) ) ;
#91975=EDGE_CURVE ( 'NONE', #80209, #67449, #24093, .T. ) ;
#91976=CARTESIAN_POINT ( 'NONE',  ( -22.31028234190000248, 1482.724791558229981, 223.3675453720979931 ) ) ;
#91978=CARTESIAN_POINT ( 'NONE',  ( -33.91369114349999592, 1451.728768196330066, 134.7155300131979914 ) ) ;
#91981=CARTESIAN_POINT ( 'NONE',  ( 4.911197430519999685, 1406.966595134230147, 269.6424802271980070 ) ) ;
#91982=CARTESIAN_POINT ( 'NONE',  ( 0.1980232598670000066, 1409.427787371929981, 185.2209094312979971 ) ) ;
#91983=CARTESIAN_POINT ( 'NONE',  ( 0.1720217706479290065, 1499.798427092860038, 209.5061785884660139 ) ) ;
#91985=CARTESIAN_POINT ( 'NONE',  ( 21.45878957224126538, 1428.925085783155055, 219.0154504687402834 ) ) ;
#91988=CARTESIAN_POINT ( 'NONE',  ( 8.038768963489999919, 1463.606875709430142, 235.5281748529980064 ) ) ;
#91990=CARTESIAN_POINT ( 'NONE',  ( -12.71224440519999987, 1445.116720337619881, 186.6519215034980164 ) ) ;
#91991=CARTESIAN_POINT ( 'NONE',  ( -19.82693296922757753, 1485.723221708761912, 190.4380495410725302 ) ) ;
#91992=CARTESIAN_POINT ( 'NONE',  ( -13.43786151985979949, 1415.007830321470010, 220.3585435133520036 ) ) ;
#91995=EDGE_CURVE ( 'NONE', #5297, #80757, #104509, .T. ) ;
#91996=B_SPLINE_SURFACE_WITH_KNOTS ( 'NONE', 5, 5, ( 
 ( #64110, #61493, #44689, #99319, #95623, #53087, #73047, #90371, #78834 ),
 ( #2145, #13649, #62052, #104576, #96177, #19452, #11079, #45246, #80892 ),
 ( #98231, #103207, #3562, #95390, #62941, #9718, #80243, #69106, #86428 ),
 ( #11933, #11396, #103790, #86980, #95939, #43884, #97052, #69668, #27090 ),
 ( #10269, #52304, #104337, #1906, #71333, #96493, #88107, #19772, #20316 ),
 ( #26513, #35475, #54521, #46113, #18654, #70231, #94832, #88656, #60711 ) ),
 .UNSPECIFIED., .F., .F., .F.,
 ( 6, 6 ),
 ( 6, 3, 6 ),
 ( 1.103913001820000073, 5.464014710059999835 ),
 ( 0.000000000000000000, 1.000000000000000000, 2.000000000000000000 ),
 .UNSPECIFIED. ) ;
#91999=CARTESIAN_POINT ( 'NONE',  ( -2.500000000000000000, 1432.302173844710069, 157.4936352153980010 ) ) ;
#92000=CARTESIAN_POINT ( 'NONE',  ( -4.911878354730000673, 1474.859473121729934, 269.6424781226980372 ) ) ;
#92001=CARTESIAN_POINT ( 'NONE',  ( 0.1681681984989999989, 1405.973120458229914, 146.1721969590979882 ) ) ;
#92005=FACE_OUTER_BOUND ( 'NONE', #54840, .T. ) ;
#92010=B_SPLINE_SURFACE_WITH_KNOTS ( 'NONE', 5, 5, ( 
 ( #57911, #32690, #49511, #47841, #39438, #92583 ),
 ( #24274, #15854, #50059, #84187, #41647, #101521 ),
 ( #13651, #73613, #107742, #99321, #22595, #56798 ),
 ( #90935, #74163, #78003, #51710, #94237, #103760 ),
 ( #85281, #110500, #17512, #25367, #1309, #8580 ),
 ( #67977, #36012, #34344, #43856, #68522, #35449 ) ),
 .UNSPECIFIED., .F., .F., .F.,
 ( 6, 6 ),
 ( 6, 6 ),
 ( 63.41643075169999832, 77.02573483309998892 ),
 ( 0.000000000000000000, 2.000000000000000000 ),
 .UNSPECIFIED. ) ;
#92011=CARTESIAN_POINT ( 'NONE',  ( -24.83894917540860092, 1457.427378167110191, 211.2740613720590090 ) ) ;
#92013=CARTESIAN_POINT ( 'NONE',  ( -13.62133678120479985, 1452.879579795280051, 223.2680741433150047 ) ) ;
#92014=CARTESIAN_POINT ( 'NONE',  ( -18.72568150940000109, 1410.063174156229934, 196.5773035203979759 ) ) ;
#92016=B_SPLINE_CURVE_WITH_KNOTS ( 'NONE', 5,
 ( #105595, #29409, #71474, #70916, #54107, #96072 ),
 .UNSPECIFIED., .F., .F.,
 ( 6, 6 ),
 ( 0.000000000000000000, 1.000000000000000000 ),
 .UNSPECIFIED. ) ;
#92017=CARTESIAN_POINT ( 'NONE',  ( -15.03721467795600120, 1422.461604470153816, 229.1222033841939947 ) ) ;
#92018=CARTESIAN_POINT ( 'NONE',  ( -22.73294892570000059, 1411.115434492829991, 269.4808104911980422 ) ) ;
#92021=CARTESIAN_POINT ( 'NONE',  ( -7.736485947205265390, 1410.556087339033184, 230.7423858731618793 ) ) ;
#92025=CARTESIAN_POINT ( 'NONE',  ( 11.64207462749999955, 1426.343247851129945, 137.4322893907980188 ) ) ;
#92032=CARTESIAN_POINT ( 'NONE',  ( -13.53550618839999942, 1416.067629290630066, 221.7501982114980308 ) ) ;
#92036=CARTESIAN_POINT ( 'NONE',  ( 20.10171151328989936, 1507.852744525929893, 228.9948058528690069 ) ) ;
#92040=CARTESIAN_POINT ( 'NONE',  ( 11.97977764410059898, 1433.676209271590096, 150.1594973095589864 ) ) ;
#92041=CARTESIAN_POINT ( 'NONE',  ( -7.156127822910000269, 1396.223004704730101, 218.8316158439280059 ) ) ;
#92042=CARTESIAN_POINT ( 'NONE',  ( -18.89832309190000004, 1409.737660254029834, 221.9605378414980237 ) ) ;
#92044=CARTESIAN_POINT ( 'NONE',  ( -13.49166848079650016, 1444.154048989462581, 169.3566495046044054 ) ) ;
#92045=CARTESIAN_POINT ( 'NONE',  ( -0.1620860067307069718, 1416.842625005220043, 227.3681785903409889 ) ) ;
#92048=CARTESIAN_POINT ( 'NONE',  ( 17.09785234980000013, 1424.306259183129896, 226.8830076123979893 ) ) ;
#92050=CARTESIAN_POINT ( 'NONE',  ( 14.94681733220000197, 1488.165501005629721, 187.6195381541980112 ) ) ;
#92051=CARTESIAN_POINT ( 'NONE',  ( -11.45334864920000051, 1414.913060387329779, 196.1469376852979849 ) ) ;
#92052=DIRECTION ( 'NONE',  ( 0.000000000000000000, 0.000000000000000000, -1.000000000000000000 ) ) ;
#92053=CARTESIAN_POINT ( 'NONE',  ( 10.99229733427299927, 1396.296919868740133, 207.7930052487479884 ) ) ;
#92054=CARTESIAN_POINT ( 'NONE',  ( -1.366628593397161140, 1414.941152333554328, 226.2919196448577566 ) ) ;
#92055=CARTESIAN_POINT ( 'NONE',  ( 10.96256097240000038, 1431.846305526410106, 151.7537324878979916 ) ) ;
#92056=CARTESIAN_POINT ( 'NONE',  ( 5.486049730215052378, 1509.110800823655609, 180.1874592187983524 ) ) ;
#92058=CARTESIAN_POINT ( 'NONE',  ( 13.00447142352859942, 1434.790086459339818, 149.3565780673969812 ) ) ;
#92061=CARTESIAN_POINT ( 'NONE',  ( -18.24651515909999944, 1497.962091606229933, 229.4161187919980023 ) ) ;
#92062=CARTESIAN_POINT ( 'NONE',  ( -11.01432655910000058, 1463.805739907729958, 231.7836158196980136 ) ) ;
#92063=B_SPLINE_CURVE_WITH_KNOTS ( 'NONE', 5,
 ( #4424, #10613, #87319, #20632, #44782, #12250, #36353, #96831, #46439 ),
 .UNSPECIFIED., .F., .F.,
 ( 6, 3, 6 ),
 ( -167.5214206057449928, -163.5285714420000147, -95.54118695260000038 ),
 .UNSPECIFIED. ) ;
#92067=EDGE_LOOP ( 'NONE', ( #25841, #24825, #869, #57293 ) ) ;
#92076=CARTESIAN_POINT ( 'NONE',  ( -16.41715922884294088, 1412.832312668764416, 269.3709241187901284 ) ) ;
#92077=CARTESIAN_POINT ( 'NONE',  ( -0.9647690717699999308, 1408.946750865729882, 231.5874088180979982 ) ) ;
#92078=CARTESIAN_POINT ( 'NONE',  ( -1.003994675859730012, 1414.971993471370070, 226.2520308800979763 ) ) ;
#92080=CARTESIAN_POINT ( 'NONE',  ( -0.01299678013268519908, 1452.713242787300032, 183.2314067176189667 ) ) ;
#92081=CARTESIAN_POINT ( 'NONE',  ( -27.33609021896520019, 1440.913060404380076, 228.3511589320279995 ) ) ;
#92084=CARTESIAN_POINT ( 'NONE',  ( -0.5359182486523100808, 1465.001494122579970, 237.3401029919169787 ) ) ;
#92085=CARTESIAN_POINT ( 'NONE',  ( 7.932946949084449528, 1410.936298116179842, 269.3426690103589749 ) ) ;
#92087=CARTESIAN_POINT ( 'NONE',  ( 22.81351936760000143, 1409.709713646930140, 209.2743772224270060 ) ) ;
#92088=CARTESIAN_POINT ( 'NONE',  ( -20.85386846230000302, 1509.307898977730019, 189.1594074083980104 ) ) ;
#92092=CARTESIAN_POINT ( 'NONE',  ( -3.484501540619901583, 1447.229515926233262, 154.8508231829048327 ) ) ;
#92094=CARTESIAN_POINT ( 'NONE',  ( -15.43014126019903642, 1486.078120340402620, 186.6022703082439023 ) ) ;
#92096=ORIENTED_EDGE ( 'NONE', *, *, #66097, .F. ) ;
#92100=CARTESIAN_POINT ( 'NONE',  ( 45.67186676709999915, 1443.699405974909951, 266.1886920326980430 ) ) ;
#92103=CARTESIAN_POINT ( 'NONE',  ( -10.37900483499999993, 1419.722126144429922, 232.2032976616980022 ) ) ;
#92105=CARTESIAN_POINT ( 'NONE',  ( -23.86676970839999612, 1446.511384828899963, 213.7383374791680239 ) ) ;
#92107=CARTESIAN_POINT ( 'NONE',  ( 17.60627508980000044, 1410.895669370830092, 224.8086596393980017 ) ) ;
#92110=CARTESIAN_POINT ( 'NONE',  ( 10.85845406881951192, 1424.793774302243946, 138.1921923613813590 ) ) ;
#92111=EDGE_LOOP ( 'NONE', ( #56988, #58859, #47066, #85452 ) ) ;
#92117=CARTESIAN_POINT ( 'NONE',  ( 21.39322610469999830, 1453.000988217330132, 223.2795384177979940 ) ) ;
#92121=DIRECTION ( 'NONE',  ( 0.000000000000000000, 1.000000000000000000, 0.000000000000000000 ) ) ;
#92122=CARTESIAN_POINT ( 'NONE',  ( 27.32003778001789840, 1435.451595106259902, 135.2710127990389992 ) ) ;
#92123=CARTESIAN_POINT ( 'NONE',  ( -38.64678288070560086, 1443.959461592480011, 137.1848748001749811 ) ) ;
#92124=CARTESIAN_POINT ( 'NONE',  ( -21.78955385629999952, 1429.676808758129937, 218.6229220870480106 ) ) ;
#92125=CARTESIAN_POINT ( 'NONE',  ( -23.69366750909999908, 1436.553436369609926, 140.6102976164979736 ) ) ;
#92127=CARTESIAN_POINT ( 'NONE',  ( -16.23351320129999920, 1415.813397303330021, 226.8799459504980121 ) ) ;
#92129=AXIS2_PLACEMENT_3D ( 'NONE', #32020, #57800, #74043 ) ;
#92130=CARTESIAN_POINT ( 'NONE',  ( -33.53568936489296703, 1459.273957448159308, 269.5121044595919670 ) ) ;
#92133=CARTESIAN_POINT ( 'NONE',  ( 1.090037377353519974E-11, 1406.777728848529932, 269.6500679732980075 ) ) ;
#92135=CARTESIAN_POINT ( 'NONE',  ( -13.91344329490000042, 1453.313060387329870, 223.0352892571980021 ) ) ;
#92136=CARTESIAN_POINT ( 'NONE',  ( -15.40184547864896203, 1451.472071962601376, 222.6652460525484685 ) ) ;
#92137=CARTESIAN_POINT ( 'NONE',  ( -29.28982059419999828, 1509.872724137230080, 209.1124962506749796 ) ) ;
#92138=B_SPLINE_SURFACE_WITH_KNOTS ( 'NONE', 5, 5, ( 
 ( #103033, #86246, #76202, #33084, #42598, #7340 ),
 ( #41505, #26331, #77315, #59973, #94089, #33623 ),
 ( #8427, #76752, #67273, #101367, #94648, #16804 ),
 ( #62, #8988, #51007, #17920, #101931, #25218 ),
 ( #17360, #93534, #9537, #24116, #92988, #68377 ),
 ( #43705, #43159, #102485, #15706, #60526, #109265 ),
 ( #613, #85140, #92430, #34744, #32550, #66725 ),
 ( #59422, #84590, #100828, #7881, #75663, #58308 ),
 ( #49908, #84042, #24657, #58858, #16263, #50466 ) ),
 .UNSPECIFIED., .F., .F., .F.,
 ( 6, 3, 6 ),
 ( 6, 6 ),
 ( 8.507271964660001018, 19.64990296329999708, 30.22064862610000091 ),
 ( -8.673617379890000077E-19, 2.000000000000000000 ),
 .UNSPECIFIED. ) ;
#92142=CARTESIAN_POINT ( 'NONE',  ( -3.722981371187852773, 1415.895496273001299, 232.5493218368858663 ) ) ;
#92143=CARTESIAN_POINT ( 'NONE',  ( -38.22966134359450763, 1444.824641043700012, 137.0630644298269942 ) ) ;
#92144=CARTESIAN_POINT ( 'NONE',  ( 18.80585470380003699, 1425.655286308133100, 226.1606062853977903 ) ) ;
#92147=CARTESIAN_POINT ( 'NONE',  ( -14.24542985449999932, 1409.914296747629805, 226.6445893585980116 ) ) ;
#92149=CARTESIAN_POINT ( 'NONE',  ( -0.08492873674538491124, 1416.830086716310007, 191.0182577611500108 ) ) ;
#92150=CARTESIAN_POINT ( 'NONE',  ( 21.46972926610340338, 1509.114287161091397, 226.4513171853454878 ) ) ;
#92153=CARTESIAN_POINT ( 'NONE',  ( 16.96258009527109678, 1415.088012641449950, 208.8510795922890111 ) ) ;
#92156=CARTESIAN_POINT ( 'NONE',  ( 4.556270434109999981E-09, 1462.105318172430088, 225.2361590696979761 ) ) ;
#92158=CARTESIAN_POINT ( 'NONE',  ( -11.86100656449999846, 1433.089193586070223, 150.2744710860979751 ) ) ;
#92162=CARTESIAN_POINT ( 'NONE',  ( -24.74889967529999879, 1438.379598184860015, 210.4710876470479946 ) ) ;
#92164=CARTESIAN_POINT ( 'NONE',  ( 2.701075187949999901, 1449.975605856229777, 183.4649351312980059 ) ) ;
#92166=B_SPLINE_CURVE_WITH_KNOTS ( 'NONE', 3,
 ( #89430, #35859, #86244, #27441 ),
 .UNSPECIFIED., .F., .F.,
 ( 4, 4 ),
 ( 0.9448711999806849171, 1.000000000000000000 ),
 .UNSPECIFIED. ) ;
#92168=CARTESIAN_POINT ( 'NONE',  ( -27.67602665774289861, 1509.991482826411129, 197.5435719732463156 ) ) ;
#92171=VERTEX_POINT ( 'NONE', #77292 ) ;
#92172=CARTESIAN_POINT ( 'NONE',  ( -11.84382825295330122, 1430.801220114690068, 149.7666669350089990 ) ) ;
#92175=CARTESIAN_POINT ( 'NONE',  ( -5.012278527039999432, 1473.692053561029752, 270.2879168812979742 ) ) ;
#92176=CARTESIAN_POINT ( 'NONE',  ( -1.556584322539999787, 1415.163755998629995, 226.9904013962980116 ) ) ;
#92178=CARTESIAN_POINT ( 'NONE',  ( 40.43717099943859949, 1446.119067000189943, 136.7611679657780144 ) ) ;
#92179=CARTESIAN_POINT ( 'NONE',  ( 16.66821264700000071, 1497.713060387329961, 193.8376437397980112 ) ) ;
#92182=CARTESIAN_POINT ( 'NONE',  ( -18.04400385319999955, 1497.713060387329961, 196.8245703038979855 ) ) ;
#92184=CARTESIAN_POINT ( 'NONE',  ( -39.66812107539500687, 1422.901596644940128, 268.6990807517719304 ) ) ;
#92185=EDGE_LOOP ( 'NONE', ( #36287, #88336, #11435, #18906 ) ) ;
#92187=ORIENTED_EDGE ( 'NONE', *, *, #29727, .F. ) ;
#92188=ORIENTED_EDGE ( 'NONE', *, *, #82507, .T. ) ;
#92190=CARTESIAN_POINT ( 'NONE',  ( 4.363119589138680254, 1423.854801764450031, 183.5697712894070150 ) ) ;
#92193=CARTESIAN_POINT ( 'NONE',  ( -2.500000000000000000, 1439.615672362369878, 170.5246407198980023 ) ) ;
#92194=CARTESIAN_POINT ( 'NONE',  ( -4.582611926280000247, 1470.461621793529957, 184.1408639795980093 ) ) ;
#92197=CARTESIAN_POINT ( 'NONE',  ( -26.54855949080000244, 1435.424486255840065, 135.3738653627980000 ) ) ;
#92200=CARTESIAN_POINT ( 'NONE',  ( 1.546896728100281004, 1416.831922880601041, 190.2226035042538683 ) ) ;
#92203=CARTESIAN_POINT ( 'NONE',  ( -33.93501299241329860, 1421.187233221759925, 270.1375433979869740 ) ) ;
#92205=CARTESIAN_POINT ( 'NONE',  ( -15.74154698502330163, 1459.394320999469983, 230.7248352790539911 ) ) ;
#92211=CARTESIAN_POINT ( 'NONE',  ( -24.86449449159999858, 1436.143114817140031, 137.8606781676980120 ) ) ;
#92212=CARTESIAN_POINT ( 'NONE',  ( -24.44980076159999882, 1442.538154569769858, 211.0821171723179930 ) ) ;
#92215=CARTESIAN_POINT ( 'NONE',  ( -2.684419367044589944, 1484.261477463810024, 183.2784813993209809 ) ) ;
#92226=CARTESIAN_POINT ( 'NONE',  ( -23.32592407598632533, 1509.740261108241157, 227.2847643979908980 ) ) ;
#92227=CARTESIAN_POINT ( 'NONE',  ( 15.76891116102829926, 1459.304365935679925, 229.4386636210950030 ) ) ;
#92229=CARTESIAN_POINT ( 'NONE',  ( 12.00387303569999986, 1415.296882282229944, 222.4718873070980294 ) ) ;
#92231=CARTESIAN_POINT ( 'NONE',  ( 0.2751658889820000065, 1506.798305107329952, 186.8348836488979998 ) ) ;
#92232=CARTESIAN_POINT ( 'NONE',  ( 23.29879903081510761, 1449.672675653727538, 217.3473003333802751 ) ) ;
#92234=CARTESIAN_POINT ( 'NONE',  ( -11.98951922200000020, 1442.759074889710064, 150.6922381223979812 ) ) ;
#92235=CARTESIAN_POINT ( 'NONE',  ( 33.91369968912619726, 1451.728767897860052, 134.7155302171979940 ) ) ;
#92238=CARTESIAN_POINT ( 'NONE',  ( -12.61640448640000045, 1416.837080243330092, 194.9197993102980035 ) ) ;
#92239=CARTESIAN_POINT ( 'NONE',  ( 16.14455737950000724, 1409.476838739224604, 193.1641866934976406 ) ) ;
#92240=CARTESIAN_POINT ( 'NONE',  ( 2.226504434969999835, 1420.543949298730013, 184.8375689860979776 ) ) ;
#92241=VECTOR ( 'NONE', #3146, 1000.000000000000000 ) ;
#92249=CARTESIAN_POINT ( 'NONE',  ( 17.36345563492336197, 1422.678662251234528, 226.5855745038400073 ) ) ;
#92253=CARTESIAN_POINT ( 'NONE',  ( 38.29114240145940329, 1440.913060381290052, 256.7438938512759705 ) ) ;
#92259=CARTESIAN_POINT ( 'NONE',  ( -14.30333153811707447, 1506.380977071295547, 225.8074781016927943 ) ) ;
#92263=CARTESIAN_POINT ( 'NONE',  ( 17.56614062935820542, 1509.646347970504848, 233.5045441439745559 ) ) ;
#92269=CARTESIAN_POINT ( 'NONE',  ( -15.59042067090000039, 1507.631725798030175, 192.4853000667980041 ) ) ;
#92280=CARTESIAN_POINT ( 'NONE',  ( 34.26962912923569604, 1437.033889869800078, 136.5514234110600000 ) ) ;
#92284=DIRECTION ( 'NONE',  ( 0.000000000000000000, -1.000000000000000000, 0.000000000000000000 ) ) ;
#92288=CARTESIAN_POINT ( 'NONE',  ( 0.8274403209489998856, 1409.880679658830104, 185.1639250197980004 ) ) ;
#92291=CARTESIAN_POINT ( 'NONE',  ( -3.116026071596179836, 1441.256293133330018, 168.7233834905880201 ) ) ;
#92293=EDGE_LOOP ( 'NONE', ( #24687, #95554, #106406, #100207 ) ) ;
#92297=CARTESIAN_POINT ( 'NONE',  ( -2.207267873112999722E-10, 1469.464448464210136, 252.5672569689040188 ) ) ;
#92303=CARTESIAN_POINT ( 'NONE',  ( -45.67167540701009898, 1440.701191047660132, 266.1885089217859672 ) ) ;
#92307=CARTESIAN_POINT ( 'NONE',  ( 5.091542648593849307, 1407.116995818669920, 221.1537445908610096 ) ) ;
#92308=CARTESIAN_POINT ( 'NONE',  ( 5.035044309065482615, 1424.909721106467032, 226.7892474147294308 ) ) ;
#92310=CARTESIAN_POINT ( 'NONE',  ( -26.61818857643220326, 1451.071572817590095, 136.3881969644360197 ) ) ;
#92311=ORIENTED_EDGE ( 'NONE', *, *, #68464, .T. ) ;
#92312=CARTESIAN_POINT ( 'NONE',  ( 21.37677629770000109, 1428.055008772630117, 225.6922921337979915 ) ) ;
#92313=CARTESIAN_POINT ( 'NONE',  ( -1.477410530420000034, 1458.407133990929879, 182.8647753367980044 ) ) ;
#92314=DIRECTION ( 'NONE',  ( 0.000000000000000000, -0.7071067811865474617, -0.7071067811865474617 ) ) ;
#92316=CARTESIAN_POINT ( 'NONE',  ( -20.99439929906685975, 1454.025623455535424, 225.3869460591365623 ) ) ;
#92317=CARTESIAN_POINT ( 'NONE',  ( -28.15442856212169787, 1509.896234822020006, 200.8410265843269826 ) ) ;
#92318=CARTESIAN_POINT ( 'NONE',  ( -15.88438700284329919, 1452.358365370260117, 147.2139129419049937 ) ) ;
#92319=CARTESIAN_POINT ( 'NONE',  ( -25.73472869180000089, 1440.328566752500137, 138.3426558852979724 ) ) ;
#92321=CARTESIAN_POINT ( 'NONE',  ( -5.359994163131460709, 1422.229041729120127, 144.9878932283519930 ) ) ;
#92323=CARTESIAN_POINT ( 'NONE',  ( 16.22918548398149952, 1421.473783082869886, 227.2926025833970129 ) ) ;
#92325=ORIENTED_EDGE ( 'NONE', *, *, #41428, .F. ) ;
#92328=CARTESIAN_POINT ( 'NONE',  ( -24.06092262379999980, 1410.732887028930008, 209.4001518044459829 ) ) ;
#92329=CARTESIAN_POINT ( 'NONE',  ( -4.095484028299999579, 1423.950387520030063, 184.1987660818980146 ) ) ;
#92331=CARTESIAN_POINT ( 'NONE',  ( -8.828869558830000130, 1428.756629641229893, 91.31218443469779800 ) ) ;
#92332=CARTESIAN_POINT ( 'NONE',  ( -2.316151605259999968, 1498.351462479429983, 236.5782940619979797 ) ) ;
#92333=CARTESIAN_POINT ( 'NONE',  ( -20.46972343990000098, 1415.849044050329894, 220.3380584269980034 ) ) ;
#92335=ORIENTED_EDGE ( 'NONE', *, *, #50002, .T. ) ;
#92336=CARTESIAN_POINT ( 'NONE',  ( 45.72863391218620421, 1443.707261214470009, 268.7602522196279438 ) ) ;
#92338=CARTESIAN_POINT ( 'NONE',  ( -0.006904034787109999440, 1420.198046511930215, 183.9035050854979829 ) ) ;
#92341=CARTESIAN_POINT ( 'NONE',  ( 18.71873819915595405, 1458.256924698515377, 227.3233249423684015 ) ) ;
#92343=DIRECTION ( 'NONE',  ( 0.000000000000000000, 0.000000000000000000, 1.000000000000000000 ) ) ;
#92346=CARTESIAN_POINT ( 'NONE',  ( 26.69869368971990298, 1451.980701177230003, 134.9228189439619996 ) ) ;
#92348=CIRCLE ( 'NONE', #88779, 2.000000000000000000 ) ;
#92353=CARTESIAN_POINT ( 'NONE',  ( 2.021802345552520030, 1408.983663280989958, 186.9337625968530006 ) ) ;
#92355=CARTESIAN_POINT ( 'NONE',  ( -18.56260928087826656, 1424.353331803792344, 224.9312564898113749 ) ) ;
#92358=CARTESIAN_POINT ( 'NONE',  ( 9.584198994920001269, 1428.531551829730233, 147.0197059986979866 ) ) ;
#92359=ORIENTED_EDGE ( 'NONE', *, *, #62608, .F. ) ;
#92360=CARTESIAN_POINT ( 'NONE',  ( 11.96392952312509905, 1414.971349104630008, 220.7371169548410137 ) ) ;
#92361=CARTESIAN_POINT ( 'NONE',  ( 11.04095755852680050, 1432.346658633729930, 151.7150567104229992 ) ) ;
#92367=CARTESIAN_POINT ( 'NONE',  ( 1.532107773980000135E-14, 1465.000168611230038, 255.3819207742980097 ) ) ;
#92368=CARTESIAN_POINT ( 'NONE',  ( -22.01759379845357500, 1509.573295812402421, 191.3436680351161669 ) ) ;
#92369=CARTESIAN_POINT ( 'NONE',  ( -20.59664500270120158, 1507.763472350329948, 190.3621299389660066 ) ) ;
#92371=CARTESIAN_POINT ( 'NONE',  ( 30.40113727430000168, 1448.202175313850148, 255.3819207682979595 ) ) ;
#92373=CARTESIAN_POINT ( 'NONE',  ( -16.87240959569610155, 1409.502257913620042, 196.1298155364530089 ) ) ;
#92376=CARTESIAN_POINT ( 'NONE',  ( -17.51176841079999846, 1485.959496867730195, 188.3680485027980183 ) ) ;
#92378=CARTESIAN_POINT ( 'NONE',  ( -18.09437733770000278, 1410.908168226329963, 224.6134321192979826 ) ) ;
#92379=CARTESIAN_POINT ( 'NONE',  ( 23.79684662030000197, 1410.916736074229902, 210.7771579475879946 ) ) ;
#92380=AXIS2_PLACEMENT_3D ( 'NONE', #46166, #3611, #63526 ) ;
#92382=CARTESIAN_POINT ( 'NONE',  ( -17.41349417983979819, 1410.020399789049861, 193.4350316837939943 ) ) ;
#92383=CARTESIAN_POINT ( 'NONE',  ( 1.098845374075520025E-07, 1407.083025879190018, 196.1147840738369723 ) ) ;
#92386=CARTESIAN_POINT ( 'NONE',  ( -12.50239388149999975, 1416.520646107730045, 222.1348954077979840 ) ) ;
#92388=CARTESIAN_POINT ( 'NONE',  ( 0.2071197430525490157, 1458.969830049299844, 182.9972804725040021 ) ) ;
#92389=DIRECTION ( 'NONE',  ( -1.000000000000000000, 0.000000000000000000, 0.000000000000000000 ) ) ;
#92390=VERTEX_POINT ( 'NONE', #16238 ) ;
#92391=CARTESIAN_POINT ( 'NONE',  ( -18.64337105059427913, 1443.913060387330233, 162.1710875046049694 ) ) ;
#92393=CARTESIAN_POINT ( 'NONE',  ( 12.40399033819999985, 1434.420133248469938, 149.8851994706980122 ) ) ;
#92394=CARTESIAN_POINT ( 'NONE',  ( -41.65423399716719643, 1444.110307754890073, 134.0999999982789745 ) ) ;
#92395=DIRECTION ( 'NONE',  ( 0.000000000000000000, 0.000000000000000000, -1.000000000000000000 ) ) ;
#92400=CARTESIAN_POINT ( 'NONE',  ( -6.232532001854649728, 1405.413060387330006, 197.7132726571231558 ) ) ;
#92401=EDGE_CURVE ( 'NONE', #11383, #575, #50984, .T. ) ;
#92405=VECTOR ( 'NONE', #69819, 1000.000000000000000 ) ;
#92407=CARTESIAN_POINT ( 'NONE',  ( 2.500000007239999711, 1434.165708943269919, 183.5270322547980015 ) ) ;
#92411=VERTEX_POINT ( 'NONE', #85113 ) ;
#92412=CARTESIAN_POINT ( 'NONE',  ( 11.87713710604131379, 1433.166847837657770, 149.9793738463967259 ) ) ;
#92413=CARTESIAN_POINT ( 'NONE',  ( -16.12920693297470009, 1409.501579173550226, 225.4780555564630049 ) ) ;
#92414=CARTESIAN_POINT ( 'NONE',  ( 2.500000000000000000, 1418.913060387330006, 172.2701767054979882 ) ) ;
#92415=EDGE_LOOP ( 'NONE', ( #57387, #37955, #67908, #6088 ) ) ;
#92417=CARTESIAN_POINT ( 'NONE',  ( -19.85273216998108126, 1410.967088625417546, 221.2148261137424754 ) ) ;
#92418=CARTESIAN_POINT ( 'NONE',  ( 15.81201445386249915, 1506.433683730510211, 224.3933755863170063 ) ) ;
#92419=CARTESIAN_POINT ( 'NONE',  ( -0.08981465318181031110, 1420.356465652879933, 183.3314806077030141 ) ) ;
#92422=CARTESIAN_POINT ( 'NONE',  ( -15.96680046119999830, 1422.914845696529937, 228.4252575972979855 ) ) ;
#92426=CARTESIAN_POINT ( 'NONE',  ( 6.553899686920000356, 1408.913060387329779, 225.8798606464979741 ) ) ;
#92430=CARTESIAN_POINT ( 'NONE',  ( 3.116049927029999722, 1446.579647245350088, 167.4613963303980029 ) ) ;
#92431=ORIENTED_EDGE ( 'NONE', *, *, #65688, .T. ) ;
#92432=CARTESIAN_POINT ( 'NONE',  ( -4.363122647530000009, 1416.108409730630001, 162.4768476156980057 ) ) ;
#92433=CARTESIAN_POINT ( 'NONE',  ( -7.105427357599999217E-15, 1420.413060387330006, 188.2701767054980166 ) ) ;
#92437=ORIENTED_EDGE ( 'NONE', *, *, #6044, .F. ) ;
#92439=EDGE_CURVE ( 'NONE', #35481, #100091, #93772, .T. ) ;
#92441=CARTESIAN_POINT ( 'NONE',  ( -11.13193939202500005, 1425.173970145079920, 142.6750931195440160 ) ) ;
#92442=CARTESIAN_POINT ( 'NONE',  ( 16.40909233880620022, 1410.440661368950032, 191.7158404879280056 ) ) ;
#92445=CARTESIAN_POINT ( 'NONE',  ( 40.27241789890000234, 1443.136959010180135, 137.0603092562980123 ) ) ;
#92446=ADVANCED_FACE ( 'NONE', ( #98480 ), #90072, .T. ) ;
#92447=CARTESIAN_POINT ( 'NONE',  ( -45.31147080460000609, 1435.337549144299828, 266.2043115811979987 ) ) ;
#92450=CARTESIAN_POINT ( 'NONE',  ( 14.99814013759614539, 1461.964485411068381, 230.0038671489789976 ) ) ;
#92452=EDGE_CURVE ( 'NONE', #5500, #44794, #40454, .T. ) ;
#92453=CARTESIAN_POINT ( 'NONE',  ( 36.14177852621219955, 1451.331926750559887, 134.0999999986410103 ) ) ;
#92454=CARTESIAN_POINT ( 'NONE',  ( -40.20798285448640286, 1442.677115920979986, 137.0083301852329782 ) ) ;
#92457=CARTESIAN_POINT ( 'NONE',  ( 2.921131820879320440, 1415.930151663460038, 231.8786077272699799 ) ) ;
#92459=ORIENTED_EDGE ( 'NONE', *, *, #91157, .F. ) ;
#92460=CARTESIAN_POINT ( 'NONE',  ( -29.41270317694913672, 1509.945394547169371, 211.3255468430687927 ) ) ;
#92463=CARTESIAN_POINT ( 'NONE',  ( 4.500000000000000000, 1425.929641636930000, 126.8043280305979863 ) ) ;
#92467=CARTESIAN_POINT ( 'NONE',  ( 42.60628463180059811, 1443.705283475309898, 134.4205488470810224 ) ) ;
#92468=CARTESIAN_POINT ( 'NONE',  ( 12.78723757108998704, 1416.835806623466169, 222.7043020517274670 ) ) ;
#92469=CARTESIAN_POINT ( 'NONE',  ( 25.20424027759999674, 1437.598577823609958, 138.0428463375980073 ) ) ;
#92471=EDGE_CURVE ( 'NONE', #6406, #14678, #2124, .T. ) ;
#92473=ORIENTED_EDGE ( 'NONE', *, *, #58529, .F. ) ;
#92476=VERTEX_POINT ( 'NONE', #67116 ) ;
#92477=CARTESIAN_POINT ( 'NONE',  ( 11.75840501554399964, 1426.865784514229972, 145.6544800655120184 ) ) ;
#92480=CARTESIAN_POINT ( 'NONE',  ( -13.72467564589999967, 1416.021639796329964, 221.7306982637980184 ) ) ;
#92481=CARTESIAN_POINT ( 'NONE',  ( -11.86607447778760083, 1432.335962723229841, 150.0622432091620055 ) ) ;
#92485=CARTESIAN_POINT ( 'NONE',  ( 21.69166379610710038, 1409.783307410840052, 206.3313277539500348 ) ) ;
#92489=CARTESIAN_POINT ( 'NONE',  ( -10.06780437910142645, 1410.639284901293877, 188.4524536534676429 ) ) ;
#92491=CARTESIAN_POINT ( 'NONE',  ( -15.97096329820000093, 1473.842985808030107, 223.5132954784979802 ) ) ;
#92492=CARTESIAN_POINT ( 'NONE',  ( 15.26419385149999997, 1460.025905744229931, 232.1043486749979934 ) ) ;
#92493=LINE ( 'NONE', #57827, #90438 ) ;
#92494=CARTESIAN_POINT ( 'NONE',  ( -4.802294408477028043, 1422.281227809200118, 184.7525987295207415 ) ) ;
#92499=CARTESIAN_POINT ( 'NONE',  ( -22.62008889866104866, 1409.702957286100855, 209.3923290094326148 ) ) ;
#92504=CARTESIAN_POINT ( 'NONE',  ( -11.60004869884644485, 1425.874190438160667, 138.5974276262502940 ) ) ;
#92506=ORIENTED_EDGE ( 'NONE', *, *, #14782, .T. ) ;
#92507=CARTESIAN_POINT ( 'NONE',  ( 0.5710642426230000401, 1435.008643400159826, 189.6733896163979978 ) ) ;
#92509=CARTESIAN_POINT ( 'NONE',  ( -11.68915241180000031, 1426.973230569230054, 148.0825247161979803 ) ) ;
#92512=CARTESIAN_POINT ( 'NONE',  ( 11.86590152282269983, 1432.348277341620133, 151.0567667683120021 ) ) ;
#92514=LINE ( 'NONE', #26416, #99819 ) ;
#92515=CARTESIAN_POINT ( 'NONE',  ( -26.09377909390000028, 1495.363898751129909, 213.7758989565080014 ) ) ;
#92518=FACE_OUTER_BOUND ( 'NONE', #63278, .T. ) ;
#92521=CARTESIAN_POINT ( 'NONE',  ( 4.933164704560000224, 1406.696844280630103, 269.4903318383980491 ) ) ;
#92522=CARTESIAN_POINT ( 'NONE',  ( 0.1880691449870000032, 1408.919627906630012, 186.4705829950979989 ) ) ;
#92523=CARTESIAN_POINT ( 'NONE',  ( 18.55657787220000188, 1449.736067588349897, 191.3116986559980148 ) ) ;
#92524=CARTESIAN_POINT ( 'NONE',  ( 8.065173493921880876, 1506.579904882062237, 229.7035030383271419 ) ) ;
#92527=CARTESIAN_POINT ( 'NONE',  ( 11.87275636863970085, 1432.783179063080070, 147.6501916617970096 ) ) ;
#92528=CARTESIAN_POINT ( 'NONE',  ( -18.72407526530000155, 1458.246115540929850, 227.3156487912980026 ) ) ;
#92530=CARTESIAN_POINT ( 'NONE',  ( -13.22933013659999979, 1444.724273266610226, 186.9257294308980022 ) ) ;
#92533=CARTESIAN_POINT ( 'NONE',  ( 29.18127911709999722, 1415.346630214729885, 269.9487154676979799 ) ) ;
#92534=CARTESIAN_POINT ( 'NONE',  ( 1.463768699429939923, 1492.321606822109970, 181.7584585652749922 ) ) ;
#92535=CARTESIAN_POINT ( 'NONE',  ( -2.984513020910000147, 1427.913060387330006, 209.1218459616979999 ) ) ;
#92540=CARTESIAN_POINT ( 'NONE',  ( -2.111106103540000056, 1476.041150137029945, 267.5352996838980175 ) ) ;
#92541=CARTESIAN_POINT ( 'NONE',  ( -6.754078978114156584, 1512.913060387330006, 184.4732361498326156 ) ) ;
#92543=CARTESIAN_POINT ( 'NONE',  ( -5.050714599155177176, 1486.518763338962117, 182.0512026800892045 ) ) ;
#92546=CARTESIAN_POINT ( 'NONE',  ( -6.558760908210000906, 1438.201672707379885, 154.7769642619979891 ) ) ;
#92549=CARTESIAN_POINT ( 'NONE',  ( -13.95127756348659886, 1463.590397533409941, 223.6014887471609995 ) ) ;
#92552=CARTESIAN_POINT ( 'NONE',  ( 0.000000000000000000, 1519.913060387329779, 209.1218459616979999 ) ) ;
#92553=CARTESIAN_POINT ( 'NONE',  ( -15.04132722364800046, 1422.464884556249899, 228.7611645815219958 ) ) ;
#92557=CARTESIAN_POINT ( 'NONE',  ( -1.600048698852036821, 1401.254281879943164, 135.5999999980979851 ) ) ;
#92562=CARTESIAN_POINT ( 'NONE',  ( 13.89869200000000049, 1452.835253893030085, 223.8385666725980059 ) ) ;
#92566=CARTESIAN_POINT ( 'NONE',  ( -0.07943192025475609430, 1419.763154935769990, 184.3780508227239920 ) ) ;
#92570=CARTESIAN_POINT ( 'NONE',  ( -13.45946769660000086, 1415.628674266529742, 221.4934452861980105 ) ) ;
#92574=CARTESIAN_POINT ( 'NONE',  ( 21.53212336100769875, 1509.608430946529779, 228.7663254442010157 ) ) ;
#92578=CARTESIAN_POINT ( 'NONE',  ( 11.79580364919999980, 1433.901673931670075, 150.9072373718979918 ) ) ;
#92579=CARTESIAN_POINT ( 'NONE',  ( -2.678904600480000120, 1397.368089890330111, 222.0733538051979963 ) ) ;
#92583=CARTESIAN_POINT ( 'NONE',  ( -26.35475707739999862, 1507.985742211030129, 201.5462075370979846 ) ) ;
#92586=CARTESIAN_POINT ( 'NONE',  ( -13.78816838342430096, 1508.464041683439973, 184.0619282346299883 ) ) ;
#92587=CARTESIAN_POINT ( 'NONE',  ( 8.417993523019999813, 1507.806286985430006, 234.9608247068980234 ) ) ;
#92588=CARTESIAN_POINT ( 'NONE',  ( 4.283104481010000519, 1468.702552713330078, 183.4792885116980017 ) ) ;
#92590=CARTESIAN_POINT ( 'NONE',  ( -9.257693745890000159, 1414.913060387329779, 195.2866393220980115 ) ) ;
#92591=CARTESIAN_POINT ( 'NONE',  ( -22.12673812478050195, 1409.685743108969973, 209.8966867368829980 ) ) ;
#92593=CARTESIAN_POINT ( 'NONE',  ( 2.500000000000000000, 1419.419920435030008, 142.4063544201979994 ) ) ;
#92594=CARTESIAN_POINT ( 'NONE',  ( 11.57711677559999863, 1432.386434236500008, 151.1965308031980157 ) ) ;
#92596=ORIENTED_EDGE ( 'NONE', *, *, #4413, .F. ) ;
#92597=CARTESIAN_POINT ( 'NONE',  ( 13.17364486784780020, 1435.644391491809984, 150.5032994553720300 ) ) ;
#92598=ORIENTED_EDGE ( 'NONE', *, *, #86562, .F. ) ;
#92599=ORIENTED_EDGE ( 'NONE', *, *, #9971, .F. ) ;
#92601=CARTESIAN_POINT ( 'NONE',  ( -19.29276911551260199, 1507.866073106370095, 229.6337110716330017 ) ) ;
#92602=CARTESIAN_POINT ( 'NONE',  ( -9.181565401679998573, 1464.648192115530037, 232.7317226279979820 ) ) ;
#92607=EDGE_CURVE ( 'NONE', #39656, #9799, #77741, .T. ) ;
#92610=CARTESIAN_POINT ( 'NONE',  ( 2.500000000000000000, 1448.203471567069982, 169.7709218380130096 ) ) ;
#92612=ORIENTED_EDGE ( 'NONE', *, *, #71307, .F. ) ;
#92614=ORIENTED_EDGE ( 'NONE', *, *, #38357, .F. ) ;
#92616=CARTESIAN_POINT ( 'NONE',  ( -19.21159046289999850, 1509.355098188429793, 230.6178137211979902 ) ) ;
#92617=CARTESIAN_POINT ( 'NONE',  ( -12.40163225230000066, 1409.346134928529864, 191.0060158467980216 ) ) ;
#92619=CARTESIAN_POINT ( 'NONE',  ( -0.5081859946160119934, 1415.431750870129918, 226.9099371985450091 ) ) ;
#92621=CARTESIAN_POINT ( 'NONE',  ( 22.84395564920000155, 1432.441498076889957, 216.6658011494079972 ) ) ;
#92623=EDGE_CURVE ( 'NONE', #100575, #43125, #52378, .T. ) ;
#92628=CARTESIAN_POINT ( 'NONE',  ( 8.283412044549999464, 1408.491064663830002, 270.2796699746979812 ) ) ;
#92629=ADVANCED_FACE ( 'NONE', ( #11475 ), #30462, .F. ) ;
#92632=CARTESIAN_POINT ( 'NONE',  ( 23.56944756660000095, 1409.993291288429873, 208.9546729833109850 ) ) ;
#92644=CARTESIAN_POINT ( 'NONE',  ( 34.48978216789999607, 1443.099005942970052, 250.0021841735980388 ) ) ;
#92647=CARTESIAN_POINT ( 'NONE',  ( -5.397648344820000332, 1433.838088735599968, 154.6405597680980009 ) ) ;
#92648=FACE_OUTER_BOUND ( 'NONE', #31473, .T. ) ;
#92654=AXIS2_PLACEMENT_3D ( 'NONE', #5403, #11610, #106754 ) ;
#92655=ORIENTED_EDGE ( 'NONE', *, *, #11965, .T. ) ;
#92658=CARTESIAN_POINT ( 'NONE',  ( 24.59498549419999947, 1440.913060393719888, 213.3385281389880106 ) ) ;
#92662=CARTESIAN_POINT ( 'NONE',  ( 12.09220637906934037, 1418.812808926449861, 229.3497755446491624 ) ) ;
#92664=CARTESIAN_POINT ( 'NONE',  ( 28.38544967506950201, 1436.384351133610153, 136.6812180996950019 ) ) ;
#92665=CARTESIAN_POINT ( 'NONE',  ( 37.86953476771359561, 1448.932043378939852, 136.3660121938399925 ) ) ;
#92666=CARTESIAN_POINT ( 'NONE',  ( -23.64337581500000240, 1435.765689707139700, 212.0349968343079752 ) ) ;
#92669=CARTESIAN_POINT ( 'NONE',  ( -17.37855975720000146, 1418.344423645829920, 226.3668775949979874 ) ) ;
#92671=CARTESIAN_POINT ( 'NONE',  ( -37.69191876346824444, 1454.405435348816582, 269.5715054350180822 ) ) ;
#92672=VERTEX_POINT ( 'NONE', #105535 ) ;
#92673=CARTESIAN_POINT ( 'NONE',  ( -27.06019685167559885, 1499.595773131199849, 210.8334130608849932 ) ) ;
#92674=CARTESIAN_POINT ( 'NONE',  ( -44.80680645038494703, 1434.320850119760053, 268.9981820606464566 ) ) ;
#92677=CARTESIAN_POINT ( 'NONE',  ( 10.82822666301168546, 1452.534930380026481, 150.8032249175824973 ) ) ;
#92678=CARTESIAN_POINT ( 'NONE',  ( 14.46096030374320129, 1429.566239157359860, 190.5376751034600034 ) ) ;
#92679=CARTESIAN_POINT ( 'NONE',  ( 11.60004869885203327, 1427.311649295585767, 134.3124698398398493 ) ) ;
#92681=CARTESIAN_POINT ( 'NONE',  ( -12.60265035039207504, 1445.042479274662128, 185.7580730998129184 ) ) ;
#92684=CARTESIAN_POINT ( 'NONE',  ( -7.687944582605556576, 1417.018756110837558, 231.0788709786680784 ) ) ;
#92685=CARTESIAN_POINT ( 'NONE',  ( -1.816375554928643776, 1451.599121610970769, 154.0952112748995830 ) ) ;
#92686=CARTESIAN_POINT ( 'NONE',  ( -17.85664671351639754, 1415.933499560010205, 209.2963377197989985 ) ) ;
#92687=CARTESIAN_POINT ( 'NONE',  ( 25.18454231669999999, 1435.453564675389771, 136.2348277442980020 ) ) ;
#92688=CARTESIAN_POINT ( 'NONE',  ( -12.95684771466127216, 1442.923466797464471, 169.4279956361965560 ) ) ;
#92689=FACE_OUTER_BOUND ( 'NONE', #19811, .T. ) ;
#92692=CARTESIAN_POINT ( 'NONE',  ( 0.1620860067197200105, 1416.842625005220043, 190.8755133330550109 ) ) ;
#92694=EDGE_LOOP ( 'NONE', ( #73990, #30888, #83237, #7775 ) ) ;
#92695=EDGE_LOOP ( 'NONE', ( #78195, #45827, #305, #103581 ) ) ;
#92696=CARTESIAN_POINT ( 'NONE',  ( 17.55992563626299940, 1415.427621830080170, 209.2440911636060150 ) ) ;
#92697=CARTESIAN_POINT ( 'NONE',  ( 42.06232341934592966, 1438.972018477124266, 269.6487565939506794 ) ) ;
#92698=CARTESIAN_POINT ( 'NONE',  ( -25.06556152449999786, 1445.939394628079981, 220.8709965880979951 ) ) ;
#92700=CARTESIAN_POINT ( 'NONE',  ( -11.71548584529999992, 1433.111737081540014, 150.8480738170979976 ) ) ;
#92702=CARTESIAN_POINT ( 'NONE',  ( -2.720407840123674426, 1420.142528854944203, 186.0334220698562149 ) ) ;
#92705=CARTESIAN_POINT ( 'NONE',  ( -13.97867491850210087, 1429.402194067919709, 222.2970902837259928 ) ) ;
#92707=CARTESIAN_POINT ( 'NONE',  ( 2.893622070869999785, 1451.002760034029734, 183.8359331502979614 ) ) ;
#92712=VERTEX_POINT ( 'NONE', #90357 ) ;
#92714=CARTESIAN_POINT ( 'NONE',  ( -11.84158678921130026, 1430.652403269130218, 149.7191781297279931 ) ) ;
#92717=CARTESIAN_POINT ( 'NONE',  ( -4.958608741100000827, 1473.061993129130087, 270.4263178540980448 ) ) ;
#92720=CARTESIAN_POINT ( 'NONE',  ( -13.84676392108729992, 1425.218576473590019, 222.1679296936039805 ) ) ;
#92727=CARTESIAN_POINT ( 'NONE',  ( -10.57232560421230083, 1407.157108062349835, 269.2531376779569996 ) ) ;
#92728=EDGE_CURVE ( 'NONE', #98935, #36118, #3880, .T. ) ;
#92729=CARTESIAN_POINT ( 'NONE',  ( -13.69536319195090002, 1435.838696954500165, 150.2679701917390105 ) ) ;
#92733=ORIENTED_EDGE ( 'NONE', *, *, #54473, .T. ) ;
#92734=EDGE_CURVE ( 'NONE', #7082, #57816, #54012, .T. ) ;
#92743=VERTEX_POINT ( 'NONE', #20396 ) ;
#92751=ORIENTED_EDGE ( 'NONE', *, *, #106537, .F. ) ;
#92752=CARTESIAN_POINT ( 'NONE',  ( -25.74606116824569924, 1449.914928412390054, 208.7281950135569843 ) ) ;
#92753=CARTESIAN_POINT ( 'NONE',  ( 27.46043822030000214, 1488.693027617030111, 209.1483437815799675 ) ) ;
#92756=CARTESIAN_POINT ( 'NONE',  ( -23.99259057559999775, 1435.335336374720100, 136.7764849531980076 ) ) ;
#92757=CARTESIAN_POINT ( 'NONE',  ( -24.91076472390000163, 1442.007094529510141, 210.4668357637779934 ) ) ;
#92758=ADVANCED_FACE ( 'NONE', ( #46747 ), #65101, .T. ) ;
#92761=CARTESIAN_POINT ( 'NONE',  ( 5.414082080120000917, 1435.477060051989838, 154.6761060569980089 ) ) ;
#92768=CARTESIAN_POINT ( 'NONE',  ( -33.91369120209999721, 1435.681798817159915, 134.0999984767980209 ) ) ;
#92771=ORIENTED_EDGE ( 'NONE', *, *, #70316, .F. ) ;
#92773=CARTESIAN_POINT ( 'NONE',  ( 12.71462359147169963, 1434.614816316360020, 149.3386743435430049 ) ) ;
#92774=B_SPLINE_SURFACE_WITH_KNOTS ( 'NONE', 5, 4, ( 
 ( #60943, #9956, #1033, #35156, #61491 ),
 ( #95072, #79933, #35711, #70453, #53085 ),
 ( #104574, #103449, #20545, #54204, #18338 ),
 ( #62622, #43570, #87793, #20011, #97270 ),
 ( #28423, #79382, #27868, #11076, #45244 ),
 ( #96739, #78263, #2697, #27310, #86115 ) ),
 .UNSPECIFIED., .F., .F., .F.,
 ( 6, 6 ),
 ( 5, 5 ),
 ( 0.000000000000000000, 111.1101480259999903 ),
 ( 25.81581217359999769, 39.03307591160000101 ),
 .UNSPECIFIED. ) ;
#92775=CARTESIAN_POINT ( 'NONE',  ( 17.94638693882010116, 1459.309748162179858, 228.0675985784120314 ) ) ;
#92777=CARTESIAN_POINT ( 'NONE',  ( 25.32264566339999945, 1452.028773922830169, 135.3109774066980151 ) ) ;
#92779=CARTESIAN_POINT ( 'NONE',  ( -1.356522590139999984, 1410.335674019929911, 185.6037846922979782 ) ) ;
#92788=B_SPLINE_SURFACE_WITH_KNOTS ( 'NONE', 5, 5, ( 
 ( #43473, #110655, #93841, #77618, #51301, #60844 ),
 ( #42919, #75958, #69235, #103344, #26646, #18238 ),
 ( #28873, #54102, #38358, #88231, #46250, #19340 ),
 ( #3142, #87116, #54650, #89322, #70354, #97169 ),
 ( #70909, #29401, #96630, #28318, #64149, #19901 ),
 ( #10968, #44577, #10407, #37275, #45698, #53540 ),
 ( #72536, #78721, #61951, #2037, #36170, #105025 ),
 ( #106667, #20991, #11522, #62509, #36717, #63069 ),
 ( #79836, #104466, #71469, #105588, #27761, #96067 ),
 ( #29956, #87686, #20441, #88780, #18787, #12061 ),
 ( #80380, #3696, #37824, #72010, #45141, #79282 ),
 ( #2591, #106128, #63604, #97721, #55196, #12618 ),
 ( #46797, #80927, #52984, #4225, #73646, #15351 ),
 ( #73084, #108330, #22629, #6967, #56835, #14810 ),
 ( #49545, #82585, #55751, #23207, #57945, #38902 ),
 ( #92077, #39476, #108880, #65243, #107777, #32724 ),
 ( #14257, #90409, #13139, #89870, #5876, #48447 ),
 ( #83670, #41121, #47323, #30514, #81453, #4758 ) ),
 .UNSPECIFIED., .F., .F., .F.,
 ( 6, 3, 3, 3, 3, 6 ),
 ( 6, 6 ),
 ( 30.30137858949999696, 39.81263101060000054, 43.27628380800000230, 45.00811020669999607, 46.73993660539999695, 49.32388343160000233 ),
 ( 0.000000000000000000, 1.452596962060000108 ),
 .UNSPECIFIED. ) ;
#92791=CARTESIAN_POINT ( 'NONE',  ( 1.611684368509999965, 1420.766153637229991, 184.2335115979979889 ) ) ;
#92792=CONICAL_SURFACE ( 'NONE', #58841, 1.499999999999955369, 0.3430239404209998177 ) ;
#92797=CARTESIAN_POINT ( 'NONE',  ( 11.60004869885177925, 1426.116582408723389, 139.0978670934243553 ) ) ;
#92799=CARTESIAN_POINT ( 'NONE',  ( 18.95816141779999953, 1416.822690122629865, 210.4639565196879971 ) ) ;
#92800=CARTESIAN_POINT ( 'NONE',  ( 16.84932835999988754, 1507.643874508232784, 231.2344471367978826 ) ) ;
#92801=CARTESIAN_POINT ( 'NONE',  ( 15.02262665340000147, 1434.992946305229907, 196.2760509299980072 ) ) ;
#92802=CARTESIAN_POINT ( 'NONE',  ( 39.17967913610949893, 1440.913060373489770, 258.0998150948020111 ) ) ;
#92805=CARTESIAN_POINT ( 'NONE',  ( 12.97602761339999944, 1422.949401640830047, 222.4689737549979895 ) ) ;
#92810=CARTESIAN_POINT ( 'NONE',  ( -27.79064046509999741, 1508.605033444930086, 210.4916514804280041 ) ) ;
#92815=CARTESIAN_POINT ( 'NONE',  ( -1.514738108749209999, 1507.606285622480073, 232.0384771855580084 ) ) ;
#92818=CARTESIAN_POINT ( 'NONE',  ( 23.58949756300000189, 1451.946940865630040, 139.7425502278979934 ) ) ;
#92825=CARTESIAN_POINT ( 'NONE',  ( 19.81748036228530196, 1508.389368817880040, 229.3831171527509980 ) ) ;
#92829=CARTESIAN_POINT ( 'NONE',  ( 37.16250662717590103, 1438.008325804049946, 136.5646560650300216 ) ) ;
#92831=CARTESIAN_POINT ( 'NONE',  ( -22.59589169820000265, 1507.700907224229923, 208.9176257130850161 ) ) ;
#92835=CARTESIAN_POINT ( 'NONE',  ( 41.66090683250000382, 1443.836063800979900, 135.6920700532980106 ) ) ;
#92836=CARTESIAN_POINT ( 'NONE',  ( 14.38276615811350645, 1518.913060387330006, 235.4493228183861504 ) ) ;
#92838=CARTESIAN_POINT ( 'NONE',  ( 1.236505811250000031, 1408.956240125730119, 186.2695617811980071 ) ) ;
#92839=CARTESIAN_POINT ( 'NONE',  ( 4.585187189710000055, 1425.138335953130081, 185.5538527434979983 ) ) ;
#92840=CARTESIAN_POINT ( 'NONE',  ( -11.54436755831595995, 1432.352357148824467, 151.3410661337507008 ) ) ;
#92841=CARTESIAN_POINT ( 'NONE',  ( -2.705111913362410192, 1440.761320489169975, 170.5389615272939920 ) ) ;
#92843=CARTESIAN_POINT ( 'NONE',  ( 11.81707102253409936, 1430.266227662830033, 147.2485957573000235 ) ) ;
#92845=CARTESIAN_POINT ( 'NONE',  ( 3.813082683120000433E-15, 1426.500992774829911, 146.0666368882980066 ) ) ;
#92846=CARTESIAN_POINT ( 'NONE',  ( 18.93827134509360022, 1456.920588905010163, 229.2656879365239888 ) ) ;
#92847=CARTESIAN_POINT ( 'NONE',  ( 15.91888908530000180, 1468.833198747830011, 189.4696677705980221 ) ) ;
#92851=CARTESIAN_POINT ( 'NONE',  ( 20.50381857201226765, 1436.445248144109883, 144.8890132701617404 ) ) ;
#92852=CARTESIAN_POINT ( 'NONE',  ( -0.9044596846589999517, 1416.819756528429934, 228.0287516232980067 ) ) ;
#92857=CARTESIAN_POINT ( 'NONE',  ( -45.97693700823750618, 1439.231401605989959, 268.4976759586160142 ) ) ;
#92865=CARTESIAN_POINT ( 'NONE',  ( -27.01904753585120034, 1451.963896065450172, 135.0863428763389891 ) ) ;
#92867=EDGE_CURVE ( 'NONE', #4207, #36154, #89755, .T. ) ;
#92868=CARTESIAN_POINT ( 'NONE',  ( 9.325404832400000288, 1417.437270712429836, 238.2842636990980054 ) ) ;
#92876=CARTESIAN_POINT ( 'NONE',  ( -6.754078978114156584, 1519.913060387329779, 184.4732361498326156 ) ) ;
#92878=ORIENTED_EDGE ( 'NONE', *, *, #49516, .F. ) ;
#92884=CARTESIAN_POINT ( 'NONE',  ( -23.97223816435240096, 1410.985435140949903, 209.8860510689419812 ) ) ;
#92885=ORIENTED_EDGE ( 'NONE', *, *, #30453, .F. ) ;
#92888=CARTESIAN_POINT ( 'NONE',  ( -6.984406781949999754, 1427.831049039629988, 123.0297916884979941 ) ) ;
#92890=CARTESIAN_POINT ( 'NONE',  ( -12.15081611480000134, 1498.343186948530047, 232.9523657193980171 ) ) ;
#92891=CARTESIAN_POINT ( 'NONE',  ( -19.73144153160000158, 1410.871738074529958, 221.4848234238980069 ) ) ;
#92893=CARTESIAN_POINT ( 'NONE',  ( 45.44632409768470183, 1446.108118615839885, 266.4255912768500139 ) ) ;
#92894=CARTESIAN_POINT ( 'NONE',  ( -0.7134561372089449627, 1424.170322885679980, 228.2193000291970293 ) ) ;
#92895=PLANE ( 'NONE',  #100769 ) ;
#92899=CARTESIAN_POINT ( 'NONE',  ( -11.23615794200000018, 1433.983026149579928, 151.5834757130979824 ) ) ;
#92901=CARTESIAN_POINT ( 'NONE',  ( 22.57319362359999815, 1409.701316935530031, 208.7927549349429910 ) ) ;
#92905=CARTESIAN_POINT ( 'NONE',  ( 26.73360441909009921, 1451.227420629079916, 136.2859150302269882 ) ) ;
#92907=CARTESIAN_POINT ( 'NONE',  ( 5.220070305037049607, 1452.730771515490005, 152.0329402684909894 ) ) ;
#92909=CARTESIAN_POINT ( 'NONE',  ( 17.72062905389999798, 1409.531878389729854, 220.9701597516980200 ) ) ;
#92910=B_SPLINE_SURFACE_WITH_KNOTS ( 'NONE', 5, 5, ( 
 ( #97853, #89467, #62657, #3287, #22229, #39042 ),
 ( #72682, #46941, #45835, #55889, #96779, #13285 ),
 ( #73223, #106806, #107366, #21683, #88370, #38504 ),
 ( #37418, #64291, #97313, #4903, #11660, #12761 ),
 ( #105736, #71051, #20582, #48023, #29020, #30662 ),
 ( #47476, #81060, #29555, #98956, #81599, #30096 ),
 ( #4373, #90558, #98411, #54782, #3842, #63206 ),
 ( #105173, #20050, #88914, #12200, #46395, #80526 ),
 ( #37969, #72150, #63740, #73788, #33396, #57543 ) ),
 .UNSPECIFIED., .F., .F., .F.,
 ( 6, 3, 6 ),
 ( 6, 6 ),
 ( 0.7655572723410000169, 2.316155491860000026, 3.835724788439999866 ),
 ( 0.000000000000000000, 1.000000000000000000 ),
 .UNSPECIFIED. ) ;
#92912=CARTESIAN_POINT ( 'NONE',  ( 1.928639190254139990, 1408.980409951920137, 186.9081713113440060 ) ) ;
#92913=CARTESIAN_POINT ( 'NONE',  ( 2.041787225690000263, 1417.577345369830027, 234.8566030110980023 ) ) ;
#92916=B_SPLINE_CURVE_WITH_KNOTS ( 'NONE', 3,
 ( #1978, #36113, #59664, #868, #52379, #51814, #87623, #27158, #53480, #77564, #33884, #94909, #76447, #10341, #104410, #18183, #17612, #26019, #60784, #103280, #93773, #85954, #9793, #44514, #43959, #17051, #60216, #1403, #51248, #35544, #85381, #95462, #69739, #61890, #19276, #42295, #110601, #8676, #77016, #322, #68623, #102725, #94334, #9255, #10910, #71408, #46734, #89260, #13078, #20386, #28253, #3635, #70853, #37212, #107160, #3085, #80867, #38843, #72477, #12555, #21475, #47265, #96569, #98205, #63547, #29347, #98757, #105522, #104963, #81388, #11465, #97662, #46187, #64085, #106067, #29891, #64636, #36657, #12006, #55685, #89808, #45084, #28811, #79226, #63010, #62444, #37763, #30452, #4166, #38296, #106607, #80318, #4701, #20934, #97117, #2535, #54589, #88173, #55140, #79778, #45640, #19841, #54046, #73021, #88724, #71956, #22018, #56215, #82522, #32660, #74682, #7455, #14749, #49477, #108262 ),
 .UNSPECIFIED., .F., .F.,
 ( 4, 3, 3, 3, 3, 3, 3, 3, 3, 3, 3, 3, 3, 3, 3, 3, 3, 3, 3, 3, 3, 3, 3, 3, 3, 3, 3, 3, 3, 3, 3, 3, 3, 3, 3, 3, 3, 3, 4 ),
 ( 12.74698783810000080, 13.96492021158590013, 15.19021758214300100, 16.42218468397550168, 17.66253057083640243, 18.90660447896850016, 20.15461610509670010, 20.77312021709999712, 22.02323751836510013, 23.27242081405690044, 24.51932165410020303, 25.76266663883209773, 26.99840962570149827, 28.22887374697500107, 29.44992649507029725, 30.29491413010000045, 31.53003531328260323, 32.76773977463359699, 34.00715209279349693, 35.24735736430879740, 36.48697184716329645, 37.72530858092299866, 38.96034359410540304, 39.81482060289999936, 41.03520056654750192, 42.26691267544130426, 43.50464977309270154, 44.74750943314289486, 45.99445407601399438, 47.24535532816859984, 48.49720425972940063, 49.74861903010859976, 50.51404411539999728, 51.76209235851399626, 53.00622896957969488, 54.24216509689028953, 55.47265940268459872, 56.69304412978929975, 57.85069212525870341 ),
 .UNSPECIFIED. ) ;
#92921=CYLINDRICAL_SURFACE ( 'NONE', #71358, 2.000000000000002220 ) ;
#92928=CARTESIAN_POINT ( 'NONE',  ( -5.757839680740000077, 1468.063065667029832, 262.6648722463980334 ) ) ;
#92930=CARTESIAN_POINT ( 'NONE',  ( 11.00807055750000174, 1433.414002013319987, 151.7532352853980058 ) ) ;
#92931=CARTESIAN_POINT ( 'NONE',  ( 16.86383896579999941, 1465.456048507830019, 262.6648722511980054 ) ) ;
#92938=CARTESIAN_POINT ( 'NONE',  ( 12.78776258891489981, 1416.851343896290018, 222.2791104166909975 ) ) ;
#92939=CARTESIAN_POINT ( 'NONE',  ( -14.10814497719999849, 1418.505680634830014, 227.3595528058979767 ) ) ;
#92940=CARTESIAN_POINT ( 'NONE',  ( -16.88043746970000214, 1409.502538253129842, 223.8714129622979954 ) ) ;
#92944=CARTESIAN_POINT ( 'NONE',  ( -16.19056346127430146, 1409.478447324650006, 193.3259909677289841 ) ) ;
#92949=CARTESIAN_POINT ( 'NONE',  ( 0.1721355080774560065, 1479.076444530880053, 182.1340621069099939 ) ) ;
#92950=CARTESIAN_POINT ( 'NONE',  ( 0.06979892568819999477, 1408.910622955130066, 223.8076866983980153 ) ) ;
#92951=ORIENTED_EDGE ( 'NONE', *, *, #106730, .F. ) ;
#92952=CARTESIAN_POINT ( 'NONE',  ( -13.14421740897469704, 1444.740067931810472, 164.8757063741590230 ) ) ;
#92953=DIRECTION ( 'NONE',  ( -0.000000000000000000, 1.000000000000000000, 0.000000000000000000 ) ) ;
#92954=CARTESIAN_POINT ( 'NONE',  ( 13.80507509150000089, 1434.979586913100093, 149.8855771064980047 ) ) ;
#92955=CARTESIAN_POINT ( 'NONE',  ( -41.40218316859470349, 1445.741963847249963, 134.0999999985380100 ) ) ;
#92961=DIRECTION ( 'NONE',  ( 1.000000000000000000, 0.000000000000000000, 0.000000000000000000 ) ) ;
#92964=VECTOR ( 'NONE', #58523, 1000.000000000000000 ) ;
#92965=CARTESIAN_POINT ( 'NONE',  ( 22.09712912739999879, 1489.469559537729992, 210.0355320487269921 ) ) ;
#92967=CARTESIAN_POINT ( 'NONE',  ( 3.424114012090000436, 1431.484821031499905, 184.9008735491980246 ) ) ;
#92971=CARTESIAN_POINT ( 'NONE',  ( -28.55009427459999927, 1451.055185256330105, 136.3289724744979878 ) ) ;
#92972=CARTESIAN_POINT ( 'NONE',  ( 16.90776107416510143, 1442.831169986189479, 162.4346387413914385 ) ) ;
#92980=CARTESIAN_POINT ( 'NONE',  ( 39.14117453815377701, 1452.031574234373693, 269.5953450738427932 ) ) ;
#92982=CARTESIAN_POINT ( 'NONE',  ( 14.97515213747811380, 1430.621276459560022, 220.1205205015936031 ) ) ;
#92985=DIRECTION ( 'NONE',  ( -0.3390050494208924348, 0.7071067811868634312, -0.6205445805634688394 ) ) ;
#92986=CARTESIAN_POINT ( 'NONE',  ( 24.16067383110895506, 1509.761787560979656, 192.2118785171494721 ) ) ;
#92988=CARTESIAN_POINT ( 'NONE',  ( 2.500000010130000394, 1447.770735655929911, 162.7884763477979959 ) ) ;
#92991=CARTESIAN_POINT ( 'NONE',  ( -7.027906745119999823E-11, 1474.175172799329857, 270.1377427386980230 ) ) ;
#92995=ORIENTED_EDGE ( 'NONE', *, *, #76825, .F. ) ;
#92997=CARTESIAN_POINT ( 'NONE',  ( -23.86310425759999987, 1449.793994890560043, 202.1964979560380016 ) ) ;
#92998=CARTESIAN_POINT ( 'NONE',  ( -10.84109190673120082, 1425.665916405870121, 103.8959551503590006 ) ) ;
#92999=CARTESIAN_POINT ( 'NONE',  ( 16.07520829236349869, 1409.725530412830039, 192.1484554476330118 ) ) ;
#93001=CARTESIAN_POINT ( 'NONE',  ( 34.99705909933560122, 1436.617605928890043, 136.4767353441200157 ) ) ;
#93003=CARTESIAN_POINT ( 'NONE',  ( 2.477004153399889219, 1449.252234172512999, 182.3064460912110576 ) ) ;
#93004=B_SPLINE_SURFACE_WITH_KNOTS ( 'NONE', 5, 5, ( 
 ( #5287, #92051, #73619, #65214, #30484, #24280, #14784, #58462, #22600 ),
 ( #92590, #15861, #6936, #50066, #100448, #7492, #31032, #90378, #48969 ),
 ( #22052, #40542, #83103, #56249, #108848, #107748, #90941, #57918, #14227 ),
 ( #82559, #42207, #86957, #9157, #27069, #24816, #84740, #9695, #68528 ),
 ( #86407, #52282, #93679, #76358, #8038, #77468, #101528, #85856, #43863 ),
 ( #110507, #60687, #61253, #43322, #34353, #75810, #76919, #102627, #42758 ) ),
 .UNSPECIFIED., .F., .F., .F.,
 ( 6, 6 ),
 ( 6, 3, 6 ),
 ( 25.26539769200000052, 42.22154018949999710 ),
 ( 0.000000000000000000, 1.000000000000000000, 2.000000000000000000 ),
 .UNSPECIFIED. ) ;
#93005=CARTESIAN_POINT ( 'NONE',  ( -35.51625343300000281, 1423.702337785729924, 261.8360441569980139 ) ) ;
#93007=CARTESIAN_POINT ( 'NONE',  ( 17.08853468078067550, 1460.333142299152769, 228.6834606794553792 ) ) ;
#93010=CARTESIAN_POINT ( 'NONE',  ( -36.07989623025710557, 1437.464731524360104, 136.5385958873009997 ) ) ;
#93014=CARTESIAN_POINT ( 'NONE',  ( -18.92249268369999982, 1456.941604937630018, 229.2980728310979828 ) ) ;
#93016=ORIENTED_EDGE ( 'NONE', *, *, #61940, .T. ) ;
#93024=CARTESIAN_POINT ( 'NONE',  ( 38.81202645930000017, 1450.612734574179967, 134.0999998922980012 ) ) ;
#93026=CARTESIAN_POINT ( 'NONE',  ( -9.849896899200842881, 1512.913060387330006, 185.5490084180013923 ) ) ;
#93027=CARTESIAN_POINT ( 'NONE',  ( 17.22592475669953416, 1443.913060387330688, 162.9227486557969655 ) ) ;
#93033=EDGE_LOOP ( 'NONE', ( #8254, #41273, #6552, #5298 ) ) ;
#93034=CARTESIAN_POINT ( 'NONE',  ( 10.79382126600000014, 1414.913060387329779, 222.1041115775979904 ) ) ;
#93036=ORIENTED_EDGE ( 'NONE', *, *, #74475, .T. ) ;
#93037=CARTESIAN_POINT ( 'NONE',  ( -13.47470376080000065, 1415.128105756529976, 220.8293656388979969 ) ) ;
#93044=B_SPLINE_CURVE_WITH_KNOTS ( 'NONE', 3,
 ( #73431, #5101, #20789, #55533, #47125, #81252, #21327, #7720, #56071, #54989 ),
 .UNSPECIFIED., .F., .F.,
 ( 4, 3, 3, 4 ),
 ( -157.4228417709999803, -134.4932994732330087, -78.88177757080619301, -29.50720979954130030 ),
 .UNSPECIFIED. ) ;
#93045=CARTESIAN_POINT ( 'NONE',  ( -14.97640067789438056, 1410.808495669646845, 190.7346035218114082 ) ) ;
#93047=CARTESIAN_POINT ( 'NONE',  ( 24.49219634299049986, 1454.783420082590055, 206.2155678165669883 ) ) ;
#93050=FACE_OUTER_BOUND ( 'NONE', #55270, .T. ) ;
#93058=CARTESIAN_POINT ( 'NONE',  ( -11.60004869885203682, 1425.894669204696356, 137.5118601392097730 ) ) ;
#93060=ORIENTED_EDGE ( 'NONE', *, *, #82851, .F. ) ;
#93062=AXIS2_PLACEMENT_3D ( 'NONE', #44772, #20621, #88948 ) ;
#93064=CARTESIAN_POINT ( 'NONE',  ( -11.73709484269999948, 1429.894488352029839, 150.3345969089980088 ) ) ;
#93065=CARTESIAN_POINT ( 'NONE',  ( 19.15249185863720172, 1456.934575639789955, 224.9730113979510122 ) ) ;
#93069=CARTESIAN_POINT ( 'NONE',  ( 0.2612772751870610088, 1416.851343895820037, 190.7759414009450154 ) ) ;
#93070=CARTESIAN_POINT ( 'NONE',  ( -22.07223515240000111, 1495.368308318629943, 224.9714801519980085 ) ) ;
#93072=CARTESIAN_POINT ( 'NONE',  ( -17.15288881900699991, 1460.895685894954113, 228.2717695460779908 ) ) ;
#93073=ORIENTED_EDGE ( 'NONE', *, *, #62468, .T. ) ;
#93075=CARTESIAN_POINT ( 'NONE',  ( 21.97873717970000129, 1409.919016783729830, 268.2775909820980473 ) ) ;
#93077=CARTESIAN_POINT ( 'NONE',  ( 18.62522279299999894, 1430.306151902329930, 192.9288626887980058 ) ) ;
#93079=CARTESIAN_POINT ( 'NONE',  ( -0.3859486939953010176, 1508.980285656380147, 238.8607942401669959 ) ) ;
#93082=CARTESIAN_POINT ( 'NONE',  ( -1.695277381189999932, 1451.989423603729847, 184.1238975007979946 ) ) ;
#93085=CARTESIAN_POINT ( 'NONE',  ( -13.55686268810000072, 1443.939294377719989, 187.3937464511979840 ) ) ;
#93086=ADVANCED_FACE ( 'NONE', ( #65737 ), #41629, .F. ) ;
#93087=CARTESIAN_POINT ( 'NONE',  ( 18.89905511659999959, 1416.828040475729949, 210.6687957193779823 ) ) ;
#93090=CARTESIAN_POINT ( 'NONE',  ( 43.83783108890263946, 1431.613812174279474, 269.7043230926977344 ) ) ;
#93091=CARTESIAN_POINT ( 'NONE',  ( 1.465471608279500071, 1490.706886906569935, 181.8288697470349859 ) ) ;
#93095=CARTESIAN_POINT ( 'NONE',  ( -9.814534880020000074, 1474.572486408329951, 269.4661027754979727 ) ) ;
#93098=CARTESIAN_POINT ( 'NONE',  ( -24.15580053757905787, 1444.499259447567738, 211.6244612293730825 ) ) ;
#93102=CARTESIAN_POINT ( 'NONE',  ( 11.66418951319000108, 1415.301705644340018, 222.9857275129059815 ) ) ;
#93106=CARTESIAN_POINT ( 'NONE',  ( -22.20360156850000166, 1409.688427239630073, 206.9744876511380198 ) ) ;
#93111=CARTESIAN_POINT ( 'NONE',  ( 2.482344662330000062, 1440.444625599219989, 150.5580151863979950 ) ) ;
#93115=CARTESIAN_POINT ( 'NONE',  ( -34.33069563939339730, 1442.322945709279793, 137.1732133424210360 ) ) ;
#93121=CARTESIAN_POINT ( 'NONE',  ( 15.73570983720359884, 1409.462563483369877, 192.9527024472970140 ) ) ;
#93124=CARTESIAN_POINT ( 'NONE',  ( 1.299941910205479889, 1406.964220106440052, 222.1218459604740190 ) ) ;
#93128=CARTESIAN_POINT ( 'NONE',  ( -11.17497852669747793, 1398.244341017566740, 202.4708927046083886 ) ) ;
#93132=CARTESIAN_POINT ( 'NONE',  ( 20.77675428743160069, 1508.900241235260182, 228.2412293500289877 ) ) ;
#93136=CARTESIAN_POINT ( 'NONE',  ( 11.33665491360190103, 1434.299677755099992, 151.5166025912550083 ) ) ;
#93137=CARTESIAN_POINT ( 'NONE',  ( -10.98878578539999928, 1396.296797242730008, 211.1406780321979966 ) ) ;
#93143=CARTESIAN_POINT ( 'NONE',  ( -13.99352145463339880, 1509.057321564920130, 183.6517433629080074 ) ) ;
#93144=CARTESIAN_POINT ( 'NONE',  ( 19.52954207340370019, 1507.817373360699776, 229.4580641922199788 ) ) ;
#93146=CARTESIAN_POINT ( 'NONE',  ( 2.177068321099999704, 1449.238783986130102, 183.7865808134980057 ) ) ;
#93150=CARTESIAN_POINT ( 'NONE',  ( 1.455250893800000167, 1415.140114704729967, 191.2687284723980099 ) ) ;
#93151=CARTESIAN_POINT ( 'NONE',  ( 11.30046002139999928, 1432.242744379899932, 151.5215588119980339 ) ) ;
#93154=CARTESIAN_POINT ( 'NONE',  ( 13.27755285367060090, 1435.679892222259923, 150.4537440835390214 ) ) ;
#93156=ORIENTED_EDGE ( 'NONE', *, *, #4212, .T. ) ;
#93157=CARTESIAN_POINT ( 'NONE',  ( 13.50124191877204716, 1444.098444817566815, 169.3544818395477591 ) ) ;
#93158=CARTESIAN_POINT ( 'NONE',  ( -5.054744702799999878, 1466.411211125930095, 234.4407030224980133 ) ) ;
#93163=CARTESIAN_POINT ( 'NONE',  ( 2.500000000000000000, 1448.322079714279880, 163.7894488454339808 ) ) ;
#93165=ORIENTED_EDGE ( 'NONE', *, *, #45955, .F. ) ;
#93169=CARTESIAN_POINT ( 'NONE',  ( -18.84890028649999749, 1508.241238781830134, 229.7780645497980174 ) ) ;
#93170=CARTESIAN_POINT ( 'NONE',  ( -12.98830284870000185, 1410.299474438730158, 189.7180828017980048 ) ) ;
#93174=CARTESIAN_POINT ( 'NONE',  ( 19.78185562140000187, 1426.701755847230061, 221.7132604633979724 ) ) ;
#93184=CARTESIAN_POINT ( 'NONE',  ( 23.54053215893118534, 1409.992431867414780, 209.4961292702789422 ) ) ;
#93187=CARTESIAN_POINT ( 'NONE',  ( 39.47393889809999479, 1426.323565199129916, 271.1218459616979999 ) ) ;
#93188=CARTESIAN_POINT ( 'NONE',  ( 13.79686514299999978, 1409.394857534729908, 192.7614752862980083 ) ) ;
#93190=CARTESIAN_POINT ( 'NONE',  ( -11.14267526204083403, 1486.018413702905264, 184.3103354489751382 ) ) ;
#93195=CARTESIAN_POINT ( 'NONE',  ( 15.89627787829999939, 1466.157227575730076, 250.4785789420980109 ) ) ;
#93197=CARTESIAN_POINT ( 'NONE',  ( -16.68599179859999992, 1461.161699058329987, 228.2799821568980008 ) ) ;
#93199=CARTESIAN_POINT ( 'NONE',  ( 1.354493917142649995, 1452.777995751539947, 183.4488450902570094 ) ) ;
#93203=PLANE ( 'NONE',  #29961 ) ;
#93205=ORIENTED_EDGE ( 'NONE', *, *, #73249, .F. ) ;
#93208=CARTESIAN_POINT ( 'NONE',  ( 14.13195592840999915, 1452.421092199690065, 222.7290593210850034 ) ) ;
#93210=CARTESIAN_POINT ( 'NONE',  ( 13.06198372480000103, 1425.733590216230141, 223.1966135260979911 ) ) ;
#93214=CARTESIAN_POINT ( 'NONE',  ( 27.01381218759999925, 1450.681579806120226, 136.4483250053980044 ) ) ;
#93215=CARTESIAN_POINT ( 'NONE',  ( 4.276238399013360336, 1416.103362730192430, 231.6875764602628465 ) ) ;
#93218=CARTESIAN_POINT ( 'NONE',  ( 30.86937158395179992, 1435.735953314200060, 136.0385399056279994 ) ) ;
#93219=CARTESIAN_POINT ( 'NONE',  ( 39.15545969614949229, 1447.513155944669961, 136.5656658507510031 ) ) ;
#93220=CARTESIAN_POINT ( 'NONE',  ( 2.531940903048510086E-08, 1457.850589566970029, 229.0733431205499926 ) ) ;
#93222=CARTESIAN_POINT ( 'NONE',  ( 10.18862200870000123, 1507.986924515629880, 183.7493071292980176 ) ) ;
#93231=FACE_OUTER_BOUND ( 'NONE', #56166, .T. ) ;
#93232=CARTESIAN_POINT ( 'NONE',  ( 11.27587417618524057, 1425.429644209827529, 138.6751927835265121 ) ) ;
#93234=CARTESIAN_POINT ( 'NONE',  ( -12.53380652166779896, 1445.052232296300190, 185.6742736269380032 ) ) ;
#93239=CARTESIAN_POINT ( 'NONE',  ( 44.70563250888439910, 1440.913044414219939, 269.9105896417649433 ) ) ;
#93240=CARTESIAN_POINT ( 'NONE',  ( -20.21907573023804261, 1450.974930438806950, 145.3432850838296133 ) ) ;
#93241=CARTESIAN_POINT ( 'NONE',  ( 25.85268144089999964, 1436.351425001499820, 136.9215235935979820 ) ) ;
#93242=CARTESIAN_POINT ( 'NONE',  ( -13.10805326783636282, 1443.031241081782355, 169.4048015275553780 ) ) ;
#93245=CARTESIAN_POINT ( 'NONE',  ( 21.44621485940070471, 1509.083181763402308, 226.4317593619785782 ) ) ;
#93246=EDGE_LOOP ( 'NONE', ( #60955, #104857, #63999, #100627, #47165 ) ) ;
#93247=ORIENTED_EDGE ( 'NONE', *, *, #75427, .F. ) ;
#93250=EDGE_CURVE ( 'NONE', #22625, #93667, #61836, .T. ) ;
#93252=CARTESIAN_POINT ( 'NONE',  ( -20.43149705680000139, 1451.305676987330116, 211.9821049860279913 ) ) ;
#93255=CARTESIAN_POINT ( 'NONE',  ( -11.25211100100000117, 1433.083168801150123, 151.5369127784980208 ) ) ;
#93257=CARTESIAN_POINT ( 'NONE',  ( -2.887076735410655015, 1419.617858305948175, 186.1929011117634900 ) ) ;
#93259=CARTESIAN_POINT ( 'NONE',  ( -24.48419039099999850, 1440.340129069209979, 210.9825192850280189 ) ) ;
#93261=CARTESIAN_POINT ( 'NONE',  ( 2.874932676220000261, 1451.924210125230047, 183.8349795613980007 ) ) ;
#93264=CARTESIAN_POINT ( 'NONE',  ( -29.03599522121404419, 1510.037923944993963, 216.6658193178216436 ) ) ;
#93269=CARTESIAN_POINT ( 'NONE',  ( -19.88572122277579979, 1484.728771715989751, 191.0592865161910083 ) ) ;
#93270=CARTESIAN_POINT ( 'NONE',  ( -4.854328638709999311, 1471.845299823429968, 270.0724596863979627 ) ) ;
#93273=CARTESIAN_POINT ( 'NONE',  ( 21.61512607259999896, 1497.713060387329961, 209.1218459615069776 ) ) ;
#93275=CARTESIAN_POINT ( 'NONE',  ( -13.91344329550000047, 1453.313060387329870, 195.2084026667980083 ) ) ;
#93278=CARTESIAN_POINT ( 'NONE',  ( -15.29008408311359979, 1408.674945077619896, 269.5757537869589555 ) ) ;
#93279=CARTESIAN_POINT ( 'NONE',  ( -13.72009304850000078, 1435.216353071280082, 149.6398781814980055 ) ) ;
#93282=CARTESIAN_POINT ( 'NONE',  ( 13.69653208179999915, 1445.056976842780159, 189.0353891572979990 ) ) ;
#93283=EDGE_LOOP ( 'NONE', ( #98530, #19762, #14005, #78103 ) ) ;
#93286=CARTESIAN_POINT ( 'NONE',  ( 5.023595874863397093, 1422.819015197833551, 184.4347302699305260 ) ) ;
#93289=CARTESIAN_POINT ( 'NONE',  ( -14.88092153600000067, 1470.466294572129755, 187.7539579896979944 ) ) ;
#93296=CARTESIAN_POINT ( 'NONE',  ( -28.13569435490000004, 1509.875538910929890, 202.7428287808179732 ) ) ;
#93297=CARTESIAN_POINT ( 'NONE',  ( 4.026786250540000722, 1408.413060387330006, 137.0999999980979851 ) ) ;
#93299=CARTESIAN_POINT ( 'NONE',  ( -5.451927469500000178, 1408.921438759329931, 196.0890200002980066 ) ) ;
#93301=CARTESIAN_POINT ( 'NONE',  ( 15.58634593796259082, 1506.535970899979247, 193.4985844669198514 ) ) ;
#93302=ORIENTED_EDGE ( 'NONE', *, *, #98759, .F. ) ;
#93303=CARTESIAN_POINT ( 'NONE',  ( -26.02644626588410048, 1469.349415895499760, 210.5465789334240299 ) ) ;
#93304=CARTESIAN_POINT ( 'NONE',  ( 22.23102602810000405, 1508.124938944730047, 224.5788317314980134 ) ) ;
#93315=VERTEX_POINT ( 'NONE', #10794 ) ;
#93317=CARTESIAN_POINT ( 'NONE',  ( -19.96907025085698351, 1456.518973795319653, 225.2441494129984676 ) ) ;
#93320=EDGE_CURVE ( 'NONE', #36772, #39681, #46644, .T. ) ;
#93321=CARTESIAN_POINT ( 'NONE',  ( -22.98628035409431192, 1509.732561025907899, 227.7597765635970859 ) ) ;
#93322=CARTESIAN_POINT ( 'NONE',  ( -4.070572111042093155, 1440.961967058545042, 184.9442369547908243 ) ) ;
#93324=CARTESIAN_POINT ( 'NONE',  ( 2.482344662330000062, 1440.444625599219989, 150.5580151863979950 ) ) ;
#93330=CARTESIAN_POINT ( 'NONE',  ( 35.14729775950531376, 1435.724875876663646, 135.0317234473804433 ) ) ;
#93331=CARTESIAN_POINT ( 'NONE',  ( 20.25110058739999985, 1509.046039775230156, 188.8042360712979928 ) ) ;
#93333=ORIENTED_EDGE ( 'NONE', *, *, #80813, .F. ) ;
#93334=CARTESIAN_POINT ( 'NONE',  ( -17.14943674877569890, 1460.897686246159992, 228.2718295297070199 ) ) ;
#93335=CARTESIAN_POINT ( 'NONE',  ( -11.60004869885204215, 1426.273944179774844, 138.2686100621498326 ) ) ;
#93336=VERTEX_POINT ( 'NONE', #59969 ) ;
#93337=CARTESIAN_POINT ( 'NONE',  ( 1.654267213550000060, 1420.334206264930117, 184.6982689316979815 ) ) ;
#93342=CARTESIAN_POINT ( 'NONE',  ( 17.57597226803159529, 1423.079937563883959, 226.3733900275827580 ) ) ;
#93344=EDGE_CURVE ( 'NONE', #102960, #7082, #16799, .T. ) ;
#93345=SPHERICAL_SURFACE ( 'NONE', #103859, 2.000000000510000042 ) ;
#93346=CARTESIAN_POINT ( 'NONE',  ( -9.709302419510001059, 1435.943783413959864, 148.7752736812980174 ) ) ;
#93347=CARTESIAN_POINT ( 'NONE',  ( 42.05112052806060063, 1440.913060353040009, 262.0200795381490479 ) ) ;
#93352=EDGE_CURVE ( 'NONE', #8198, #61380, #57267, .T. ) ;
#93354=CARTESIAN_POINT ( 'NONE',  ( 1.548840712014900145, 1416.196255291370107, 190.3585702930099899 ) ) ;
#93355=EDGE_CURVE ( 'NONE', #101350, #29004, #14963, .T. ) ;
#93358=CARTESIAN_POINT ( 'NONE',  ( 3.920879176457659820, 1439.701872010520219, 184.6839060028229937 ) ) ;
#93359=CARTESIAN_POINT ( 'NONE',  ( 2.500000000000000000, 1448.894380913990062, 168.9807461826979704 ) ) ;
#93360=EDGE_CURVE ( 'NONE', #6969, #101078, #77242, .T. ) ;
#93364=CARTESIAN_POINT ( 'NONE',  ( 22.54437430309999968, 1451.697077564529991, 142.2380798234979977 ) ) ;
#93369=CARTESIAN_POINT ( 'NONE',  ( -1.359627476360000031, 1451.982671778829854, 183.7885425899980305 ) ) ;
#93372=VERTEX_POINT ( 'NONE', #58853 ) ;
#93373=ORIENTED_EDGE ( 'NONE', *, *, #44989, .F. ) ;
#93374=DIRECTION ( 'NONE',  ( 0.000000000000000000, 1.000000000000000000, 0.000000000000000000 ) ) ;
#93376=CARTESIAN_POINT ( 'NONE',  ( 39.78919856916219544, 1441.136557108880197, 136.8413242771979981 ) ) ;
#93378=CARTESIAN_POINT ( 'NONE',  ( 18.34590456075850184, 1416.851343895820037, 209.3831232368769975 ) ) ;
#93383=CARTESIAN_POINT ( 'NONE',  ( -0.3594932246804328768, 1451.468209969438931, 182.7573421932325459 ) ) ;
#93385=CARTESIAN_POINT ( 'NONE',  ( 4.243919250670000309, 1409.061261313129990, 187.1626498370980016 ) ) ;
#93386=CARTESIAN_POINT ( 'NONE',  ( 4.187037607680000662, 1423.917686004630013, 184.1424184849980179 ) ) ;
#93389=CARTESIAN_POINT ( 'NONE',  ( -4.277751951706020073, 1441.052902712039895, 157.0207293387669836 ) ) ;
#93391=CARTESIAN_POINT ( 'NONE',  ( 11.78818133093700027, 1426.417832666100139, 148.5075478569980021 ) ) ;
#93392=CARTESIAN_POINT ( 'NONE',  ( 0.7979415355729999604, 1465.377788775429963, 236.2027333408979928 ) ) ;
#93396=CARTESIAN_POINT ( 'NONE',  ( -26.04901691849709877, 1446.564900598870054, 138.1454006445720211 ) ) ;
#93398=CARTESIAN_POINT ( 'NONE',  ( 18.18137294690000161, 1507.608465325429734, 188.5297611294979845 ) ) ;
#93400=CARTESIAN_POINT ( 'NONE',  ( -2.040094528446590223E-09, 1471.382348965860047, 257.5322757312809472 ) ) ;
#93401=CARTESIAN_POINT ( 'NONE',  ( 14.59277107062129986, 1436.244837967300100, 149.8707660814949918 ) ) ;
#93402=CARTESIAN_POINT ( 'NONE',  ( -0.7890062529830000893, 1416.021639796329964, 227.7424621462980099 ) ) ;
#93403=CARTESIAN_POINT ( 'NONE',  ( -23.80546598920000179, 1430.806027415329936, 211.0847187605880038 ) ) ;
#93408=CARTESIAN_POINT ( 'NONE',  ( -46.25879973035969783, 1439.825279062879872, 267.5901298074010128 ) ) ;
#93411=EDGE_LOOP ( 'NONE', ( #59573, #84489, #10805, #103649 ) ) ;
#93414=CARTESIAN_POINT ( 'NONE',  ( 19.26228722078564459, 1456.171679175456120, 225.0188521063314511 ) ) ;
#93416=CARTESIAN_POINT ( 'NONE',  ( -26.58673239743909633, 1451.978834094609965, 135.0959505759149977 ) ) ;
#93417=VERTEX_POINT ( 'NONE', #26899 ) ;
#93418=CARTESIAN_POINT ( 'NONE',  ( -2.138097991060000180E-08, 1420.509147084929964, 221.4103263195979707 ) ) ;
#93420=CARTESIAN_POINT ( 'NONE',  ( 15.24905281719999905, 1488.805759879029893, 194.1126383535979869 ) ) ;
#93421=CARTESIAN_POINT ( 'NONE',  ( -2.374774714134009646, 1419.515052570159924, 186.0454628696550117 ) ) ;
#93425=EDGE_LOOP ( 'NONE', ( #65847, #57664, #1373, #18513 ) ) ;
#93426=CARTESIAN_POINT ( 'NONE',  ( -4.976825802775040053, 1408.127936775080116, 270.2880426513530097 ) ) ;
#93427=CARTESIAN_POINT ( 'NONE',  ( 6.488431865357080497, 1418.472541117210085, 233.3050633955320166 ) ) ;
#93429=ORIENTED_EDGE ( 'NONE', *, *, #13099, .T. ) ;
#93431=CARTESIAN_POINT ( 'NONE',  ( -23.26431872588840122, 1410.005238423490027, 210.0136070511539970 ) ) ;
#93432=CARTESIAN_POINT ( 'NONE',  ( -1.356543646279819937, 1410.335726175669834, 185.6038078910299873 ) ) ;
#93433=CARTESIAN_POINT ( 'NONE',  ( -3.955028505459999653E-16, 1420.349145488430167, 170.8340916043979973 ) ) ;
#93434=CARTESIAN_POINT ( 'NONE',  ( -2.286265947080000416, 1427.727383903629971, 112.4493539157979995 ) ) ;
#93435=CARTESIAN_POINT ( 'NONE',  ( -19.84697927394439887, 1469.911627675270211, 193.3779138725080031 ) ) ;
#93437=CARTESIAN_POINT ( 'NONE',  ( 36.83564954605069630, 1461.809058848290078, 268.7794616686949780 ) ) ;
#93441=ORIENTED_EDGE ( 'NONE', *, *, #29677, .T. ) ;
#93442=CARTESIAN_POINT ( 'NONE',  ( 18.80856254815538975, 1458.020595720538040, 227.1643417640127041 ) ) ;
#93453=CARTESIAN_POINT ( 'NONE',  ( 1.909580902767660016, 1408.979744421860232, 186.9029660347310084 ) ) ;
#93454=CARTESIAN_POINT ( 'NONE',  ( 1.492583962270000120, 1417.432316503030052, 234.4047366681980122 ) ) ;
#93460=CARTESIAN_POINT ( 'NONE',  ( 11.69495607182030028, 1415.089948427370018, 221.9856941327800257 ) ) ;
#93462=CARTESIAN_POINT ( 'NONE',  ( 20.28288303839970297, 1497.593166955129846, 226.9817472065090271 ) ) ;
#93465=CARTESIAN_POINT ( 'NONE',  ( -35.74233958356999352, 1450.108979485610007, 136.2379703606449937 ) ) ;
#93466=CARTESIAN_POINT ( 'NONE',  ( 13.29158107345610063, 1425.436905002130061, 221.8979834808779970 ) ) ;
#93468=CARTESIAN_POINT ( 'NONE',  ( -11.47403709369999980, 1467.186912539730201, 262.6648722463980334 ) ) ;
#93469=CARTESIAN_POINT ( 'NONE',  ( -16.87240959569610155, 1409.502257913620042, 196.1298155364530089 ) ) ;
#93470=CARTESIAN_POINT ( 'NONE',  ( 11.92576087849999844, 1433.460360144529886, 150.1385202855979912 ) ) ;
#93472=CARTESIAN_POINT ( 'NONE',  ( 17.26713005559999914, 1453.798585003029984, 234.3916895593979746 ) ) ;
#93478=CARTESIAN_POINT ( 'NONE',  ( -19.52953025160000067, 1486.085187770929906, 189.9534856570979855 ) ) ;
#93480=CARTESIAN_POINT ( 'NONE',  ( 12.92120458945395178, 1398.295995395735417, 207.6489814522168160 ) ) ;
#93481=CARTESIAN_POINT ( 'NONE',  ( 2.902343810100000088, 1466.632250239430050, 234.1422825223980340 ) ) ;
#93482=B_SPLINE_CURVE_WITH_KNOTS ( 'NONE', 3,
 ( #23266, #108392, #80987, #65854, #47393, #31123, #55811, #6480, #73141, #4818, #40080, #4293, #90477, #106725, #38963, #99973, #5934, #73710, #31673, #74260, #89928, #48504, #74803, #23812, #57463, #38420, #30578, #83191, #98328, #107284, #46858, #72596, #32235, #13203, #99417, #91589, #14864, #56345, #107835, #49055, #40632, #30015, #108946, #21606, #82643, #66415, #100532, #64769, #65305, #98879, #13753, #22145, #82073, #47938, #22696, #58003, #64205, #12678, #5378, #81514, #39536, #56895, #91026, #14313, #7030, #68070, #110044, #77008, #102182, #85946, #314, #66960, #41188, #109500, #51805, #24902, #7579, #75360, #84286, #32776, #42846, #8121, #92681, #93234 ),
 .UNSPECIFIED., .F., .F.,
 ( 4, 2, 2, 2, 2, 2, 1, 1, 2, 2, 2, 1, 2, 2, 2, 1, 2, 2, 2, 2, 2, 2, 2, 2, 2, 1, 2, 2, 2, 2, 1, 2, 2, 2, 1, 1, 2, 2, 2, 2, 2, 2, 2, 2, 2, 4 ),
 ( 0.000000000000000000, 0.03125000000032555209, 0.04687500000049735216, 0.06250000000066914529, 0.09375000000098251962, 0.1093750000011391998, 0.1171875000012245205, 0.1210937500012671947, 0.1230468750012885248, 0.1250000000013098411, 0.1562500000012651546, 0.1718750000012148615, 0.1796875000011508294, 0.1875000000010867973, 0.2187500000008300860, 0.2343750000007013834, 0.2421875000006821210, 0.2500000000006628031, 0.3125000000008504308, 0.3437500000008782974, 0.3750000000009061085, 0.4375000000009540146, 0.5000000000010018653, 0.5625000000010497159, 0.5937500000010736967, 0.6093750000010144108, 0.6171875000009849899, 0.6250000000009555690, 0.6875000000012977397, 0.7187500000014160895, 0.7343750000015131230, 0.7421875000015614177, 0.7500000000016097124, 0.7812500000016466828, 0.7968750000016586732, 0.8046875000017007507, 0.8085937500016995294, 0.8125000000016981971, 0.8437500000015355495, 0.8593750000014233059, 0.8671875000013464785, 0.8750000000012696511, 0.9062500000009766632, 0.9218750000008136825, 0.9375000000006507017, 1.000000000000000000 ),
 .UNSPECIFIED. ) ;
#93483=CARTESIAN_POINT ( 'NONE',  ( 22.14280420710000286, 1430.347761818229856, 217.9176945388080071 ) ) ;
#93492=CARTESIAN_POINT ( 'NONE',  ( 0.1688278169330330314, 1481.018758052769954, 182.0506284089370013 ) ) ;
#93496=CARTESIAN_POINT ( 'NONE',  ( -17.11714618744286653, 1444.740067931808881, 162.7561046190442369 ) ) ;
#93497=CARTESIAN_POINT ( 'NONE',  ( 13.50074992389999906, 1434.968959668390198, 149.7892634259980298 ) ) ;
#93498=CARTESIAN_POINT ( 'NONE',  ( -39.62133910739139964, 1449.056109088350013, 134.0999999980940061 ) ) ;
#93501=CARTESIAN_POINT ( 'NONE',  ( -38.62063634653199529, 1443.662372644130073, 137.1803698382369987 ) ) ;
#93504=FACE_OUTER_BOUND ( 'NONE', #26631, .T. ) ;
#93514=ORIENTED_EDGE ( 'NONE', *, *, #6278, .F. ) ;
#93515=CARTESIAN_POINT ( 'NONE',  ( -33.31574679630000446, 1451.295103689730240, 135.9631183953979985 ) ) ;
#93516=CARTESIAN_POINT ( 'NONE',  ( 17.22654844235838567, 1443.913060387328869, 162.9224179604370590 ) ) ;
#93518=VERTEX_POINT ( 'NONE', #46477 ) ;
#93520=( BOUNDED_CURVE ( )  B_SPLINE_CURVE ( 3, ( #25192, #17892, #67789, #34 ),
 .UNSPECIFIED., .F., .T. ) 
 B_SPLINE_CURVE_WITH_KNOTS ( ( 4, 4 ),
 ( 0.9324631327127209657, 1.578300326584209934 ),
 .UNSPECIFIED. ) 
 CURVE ( )  GEOMETRIC_REPRESENTATION_ITEM ( )  RATIONAL_B_SPLINE_CURVE ( ( 1.000000000000000000, 0.9655421889976167904, 0.9655421889976167904, 1.000000000000000000 ) ) 
 REPRESENTATION_ITEM ( '' )  );
#93521=EDGE_CURVE ( 'NONE', #109101, #13629, #56319, .T. ) ;
#93525=DIRECTION ( 'NONE',  ( 0.9999982561604894293, 0.0004617740651251722099, 0.001809541569896410676 ) ) ;
#93527=CARTESIAN_POINT ( 'NONE',  ( 19.05403812430366628, 1437.962009608390417, 213.1328251454357314 ) ) ;
#93531=CARTESIAN_POINT ( 'NONE',  ( 12.45610846519999981, 1519.913060387329779, 228.8821925242980058 ) ) ;
#93534=CARTESIAN_POINT ( 'NONE',  ( 3.667960006519999983, 1446.440575811169992, 162.7182762402979961 ) ) ;
#93535=CARTESIAN_POINT ( 'NONE',  ( -2.500000000000000000, 1433.766566658040119, 157.5373253330980106 ) ) ;
#93542=CARTESIAN_POINT ( 'NONE',  ( -22.97761739119999902, 1449.791915370539982, 200.0590113766180025 ) ) ;
#93543=CARTESIAN_POINT ( 'NONE',  ( -11.24352777690759808, 1426.459969836569826, 108.4497583346609986 ) ) ;
#93544=CARTESIAN_POINT ( 'NONE',  ( 17.36313619760800009, 1410.599962583540218, 192.4802441439230165 ) ) ;
#93546=CARTESIAN_POINT ( 'NONE',  ( 29.52087390520885890, 1510.054509514609435, 214.7123836248202338 ) ) ;
#93547=CARTESIAN_POINT ( 'NONE',  ( 1.228114002177200126, 1450.757138880049979, 181.5372592238319953 ) ) ;
#93553=CARTESIAN_POINT ( 'NONE',  ( -37.59663830446049815, 1438.304367445970001, 136.5843146558879937 ) ) ;
#93555=CARTESIAN_POINT ( 'NONE',  ( 10.63633553050959968, 1397.322975409730134, 200.4736743436469908 ) ) ;
#93557=CARTESIAN_POINT ( 'NONE',  ( -18.44235347220000065, 1458.914805433830225, 227.7103923031980059 ) ) ;
#93559=ORIENTED_EDGE ( 'NONE', *, *, #10545, .T. ) ;
#93560=DIRECTION ( 'NONE',  ( 0.7074300732568278294, -0.02470400251969398497, 0.7063514732138287400 ) ) ;
#93561=CARTESIAN_POINT ( 'NONE',  ( -6.446325850290750559, 1432.345402019870107, 154.6647260408460056 ) ) ;
#93566=CARTESIAN_POINT ( 'NONE',  ( -3.218186458279999940, 1461.193909496529841, 234.7217908393980110 ) ) ;
#93567=PLANE ( 'NONE',  #9960 ) ;
#93569=CARTESIAN_POINT ( 'NONE',  ( 16.90742456144603523, 1442.831169986190389, 162.4348202098863396 ) ) ;
#93571=ORIENTED_EDGE ( 'NONE', *, *, #23472, .T. ) ;
#93574=ORIENTED_EDGE ( 'NONE', *, *, #100590, .F. ) ;
#93578=CARTESIAN_POINT ( 'NONE',  ( -14.44947381900000138, 1416.568813549730066, 221.3833631277979919 ) ) ;
#93582=CARTESIAN_POINT ( 'NONE',  ( -4.629727834550000587, 1424.354173624029954, 185.7675860119980200 ) ) ;
#93583=CARTESIAN_POINT ( 'NONE',  ( -7.667845439150741349, 1446.704503592666470, 154.1274023243013005 ) ) ;
#93588=CARTESIAN_POINT ( 'NONE',  ( -17.27619074209999894, 1507.625766698130064, 224.2558816620979769 ) ) ;
#93589=CARTESIAN_POINT ( 'NONE',  ( 17.96268052179999941, 1457.880256331229930, 230.1796192676980013 ) ) ;
#93591=CARTESIAN_POINT ( 'NONE',  ( -4.863986520837263683, 1423.459995654392742, 184.6347918575768858 ) ) ;
#93592=CARTESIAN_POINT ( 'NONE',  ( -2.499957339907119991, 1419.383080839190143, 144.1003724646560045 ) ) ;
#93594=CARTESIAN_POINT ( 'NONE',  ( 18.19680845026800142, 1424.503018947390046, 223.8103149804830139 ) ) ;
#93596=CARTESIAN_POINT ( 'NONE',  ( -2.901263397339155503, 1484.476379004488081, 183.2956404250009541 ) ) ;
#93599=VERTEX_POINT ( 'NONE', #63828 ) ;
#93600=CARTESIAN_POINT ( 'NONE',  ( 1.116994350369999944, 1471.309462467129833, 187.7634697624980049 ) ) ;
#93602=CARTESIAN_POINT ( 'NONE',  ( -11.78791146169999848, 1427.317704561630080, 147.8403236071979734 ) ) ;
#93605=CARTESIAN_POINT ( 'NONE',  ( 14.44412038922260066, 1509.548839689010038, 235.4430145295710020 ) ) ;
#93607=CARTESIAN_POINT ( 'NONE',  ( -2.482344662330000062, 1440.444625599219989, 150.5580151863979950 ) ) ;
#93608=CARTESIAN_POINT ( 'NONE',  ( -21.80579869879999677, 1495.368972219230045, 225.4358925196980010 ) ) ;
#93613=CARTESIAN_POINT ( 'NONE',  ( 23.55040952570000101, 1411.064796383629982, 269.0842170185980535 ) ) ;
#93614=CARTESIAN_POINT ( 'NONE',  ( 0.8662106067031465351, 1465.087948376955410, 238.0466371020243059 ) ) ;
#93615=CARTESIAN_POINT ( 'NONE',  ( 24.17852980030000154, 1469.149352981230095, 201.1913038658580035 ) ) ;
#93616=ADVANCED_FACE ( 'NONE', ( #2281 ), #104649, .T. ) ;
#93617=CARTESIAN_POINT ( 'NONE',  ( 0.05134268663526449922, 1508.133705146910188, 237.5625132777319948 ) ) ;
#93619=CARTESIAN_POINT ( 'NONE',  ( -1.370024040769999951, 1450.924184932629942, 183.2893338627980029 ) ) ;
#93620=CARTESIAN_POINT ( 'NONE',  ( 17.41280537782821369, 1458.364529780870271, 230.6041477805117665 ) ) ;
#93622=CARTESIAN_POINT ( 'NONE',  ( -13.74969930740000024, 1443.369189997270041, 188.1932585784979892 ) ) ;
#93624=CARTESIAN_POINT ( 'NONE',  ( -21.61512607259999896, 1497.713060387329961, 209.1218459618889938 ) ) ;
#93626=CARTESIAN_POINT ( 'NONE',  ( 1.861700016370000164E-09, 1407.650947845630071, 270.1377426662980383 ) ) ;
#93628=CARTESIAN_POINT ( 'NONE',  ( 1.466447836938430171, 1489.784574236090066, 181.8690865221339834 ) ) ;
#93629=CARTESIAN_POINT ( 'NONE',  ( -12.69333308194260113, 1409.356321345949937, 201.2342037859239952 ) ) ;
#93632=CARTESIAN_POINT ( 'NONE',  ( -18.25597770279999921, 1472.821217557230057, 269.1701651182979731 ) ) ;
#93635=CARTESIAN_POINT ( 'NONE',  ( 18.15041076583969826, 1424.504405689699979, 223.8575062216150116 ) ) ;
#93638=CARTESIAN_POINT ( 'NONE',  ( 11.44693299035330192, 1415.124054205850143, 222.7699361616149929 ) ) ;
#93639=CARTESIAN_POINT ( 'NONE',  ( 3.439855069772169809E-11, 1452.913060387330006, 150.8032249182200246 ) ) ;
#93640=DIRECTION ( 'NONE',  ( 0.001027118858036968341, 0.9999913661844073154, 0.004026485253184815781 ) ) ;
#93642=CARTESIAN_POINT ( 'NONE',  ( -22.04343844010000097, 1409.682834220629957, 204.9962922481880128 ) ) ;
#93646=CARTESIAN_POINT ( 'NONE',  ( 2.927701378049999713E-15, 1442.756953654919926, 150.7628527808980152 ) ) ;
#93650=( BOUNDED_SURFACE ( )  B_SPLINE_SURFACE ( 4, 2, ( 
 ( #25810, #74602, #33667 ),
 ( #93569, #16844, #33123 ),
 ( #107, #51596, #94129 ),
 ( #59459, #42638, #75699 ),
 ( #93027, #40426, #49942 ) ),
 .UNSPECIFIED., .F., .F., .F. ) 
 B_SPLINE_SURFACE_WITH_KNOTS ( ( 5, 5 ),
 ( 3, 3 ),
 ( 1.967616199060000071, 3.613988937050000239 ),
 ( 5.300753508050029872, 6.148936695274129782 ),
 .UNSPECIFIED. ) 
 GEOMETRIC_REPRESENTATION_ITEM ( )  RATIONAL_B_SPLINE_SURFACE ( (
 ( 0.8627701935039280290, 0.8230940375028089617, 0.9542143464239759565),
 ( 0.8627701935039280290, 0.8230940375028089617, 0.9542143464239759565),
 ( 0.8627701935039280290, 0.8230940375028089617, 0.9542143464239759565),
 ( 0.8627701935039280290, 0.8230940375028089617, 0.9542143464239759565),
 ( 0.8627701935039280290, 0.8230940375028089617, 0.9542143464239759565) ) ) 
 REPRESENTATION_ITEM ( '' )  SURFACE ( )  );
#93653=CARTESIAN_POINT ( 'NONE',  ( 11.71967320325980211, 1426.707059066819966, 142.9268082951259942 ) ) ;
#93654=CARTESIAN_POINT ( 'NONE',  ( -3.171072485709999889, 1451.871858332230204, 182.7750508701979868 ) ) ;
#93655=CARTESIAN_POINT ( 'NONE',  ( -6.754078978114156584, 1512.913060387330006, 184.4732361498326156 ) ) ;
#93658=CARTESIAN_POINT ( 'NONE',  ( -17.01536243937009729, 1507.593738226439882, 224.5318899074820251 ) ) ;
#93660=CARTESIAN_POINT ( 'NONE',  ( -8.492040095572983560, 1398.165184799730923, 218.9680983094823148 ) ) ;
#93661=CARTESIAN_POINT ( 'NONE',  ( -3.406513463655362894, 1440.721058893708914, 156.8280215876527848 ) ) ;
#93663=FACE_OUTER_BOUND ( 'NONE', #28209, .T. ) ;
#93667=VERTEX_POINT ( 'NONE', #30744 ) ;
#93669=CARTESIAN_POINT ( 'NONE',  ( 11.97438681890969825, 1433.814205175160168, 150.4339170446530147 ) ) ;
#93670=CARTESIAN_POINT ( 'NONE',  ( -12.55642688110000016, 1397.977875496030038, 212.9353772083979948 ) ) ;
#93676=CARTESIAN_POINT ( 'NONE',  ( -13.85731421134180152, 1508.722096842320070, 183.9202016419540087 ) ) ;
#93678=CARTESIAN_POINT ( 'NONE',  ( 9.322640526599998978, 1468.697217342230033, 185.3328853447980009 ) ) ;
#93679=CARTESIAN_POINT ( 'NONE',  ( -2.628012640819999746, 1414.971287085330005, 192.6484313466980041 ) ) ;
#93684=CARTESIAN_POINT ( 'NONE',  ( 14.30082345506829888, 1416.007771869970156, 197.0130041503479958 ) ) ;
#93685=CARTESIAN_POINT ( 'NONE',  ( 11.86332839419999985, 1432.142273804659908, 149.9796868945980179 ) ) ;
#93687=VERTEX_POINT ( 'NONE', #48678 ) ;
#93688=CARTESIAN_POINT ( 'NONE',  ( 13.42930060380339974, 1434.933243636549832, 148.8496443608690072 ) ) ;
#93690=ORIENTED_EDGE ( 'NONE', *, *, #71836, .T. ) ;
#93691=CARTESIAN_POINT ( 'NONE',  ( 13.51303151820626169, 1443.998943487957831, 169.3513894483426157 ) ) ;
#93692=CARTESIAN_POINT ( 'NONE',  ( -4.353746609069999884, 1464.535296998829836, 236.7958744120979873 ) ) ;
#93696=B_SPLINE_SURFACE_WITH_KNOTS ( 'NONE', 5, 5, ( 
 ( #32681, #24799, #5838, #82544, #83086, #65748 ),
 ( #99865, #66860, #23163, #67413, #100970, #109405 ),
 ( #14769, #24266, #75794, #49500, #39978, #33771 ),
 ( #6379, #109946, #83625, #57902, #58446, #92036 ),
 ( #84179, #74154, #6922, #108284, #33225, #67968 ),
 ( #41079, #92574, #50051, #101513, #42191, #14214 ),
 ( #31571, #66316, #59005, #93132, #57364, #16400 ),
 ( #50594, #84725, #76342, #102076, #25359, #32131 ),
 ( #100434, #90927, #48955, #40525, #74703, #108834 ) ),
 .UNSPECIFIED., .F., .F., .F.,
 ( 6, 3, 6 ),
 ( 6, 6 ),
 ( 1.126366143519770047, 3.287928953729999826, 6.228946179000230288 ),
 ( 0.000000000000000000, 2.000010957310230264 ),
 .UNSPECIFIED. ) ;
#93698=CARTESIAN_POINT ( 'NONE',  ( -19.07453550630248174, 1442.252090472558848, 210.5365316514335916 ) ) ;
#93699=CARTESIAN_POINT ( 'NONE',  ( 2.500000000000000000, 1448.365115610690054, 162.8856519708890005 ) ) ;
#93704=ORIENTED_EDGE ( 'NONE', *, *, #84481, .F. ) ;
#93707=CARTESIAN_POINT ( 'NONE',  ( 5.451195050909999503E-14, 1410.389826760030019, 269.3346704430979912 ) ) ;
#93708=EDGE_CURVE ( 'NONE', #80584, #86711, #51979, .T. ) ;
#93710=CARTESIAN_POINT ( 'NONE',  ( -0.2892576526283990312, 1415.943166310999914, 227.2001892735609943 ) ) ;
#93711=ORIENTED_EDGE ( 'NONE', *, *, #24808, .T. ) ;
#93712=CARTESIAN_POINT ( 'NONE',  ( 19.54815321029999708, 1426.815511739029944, 223.9912215281979968 ) ) ;
#93714=CARTESIAN_POINT ( 'NONE',  ( -11.60004869885203860, 1428.965959225140750, 137.0999999980979851 ) ) ;
#93720=CARTESIAN_POINT ( 'NONE',  ( -20.58397420629999885, 1508.353852242129960, 189.9891704665979830 ) ) ;
#93724=CARTESIAN_POINT ( 'NONE',  ( -18.09477754449768838, 1486.177057533957395, 188.5520870720846176 ) ) ;
#93728=CARTESIAN_POINT ( 'NONE',  ( 31.20802388370000102, 1451.456139920330088, 248.1710554673980198 ) ) ;
#93731=CARTESIAN_POINT ( 'NONE',  ( -7.140946062075090417, 1508.970007424190044, 236.7165944161500022 ) ) ;
#93732=CARTESIAN_POINT ( 'NONE',  ( -23.29298009400000069, 1448.643654431140021, 216.8814030764980032 ) ) ;
#93736=CARTESIAN_POINT ( 'NONE',  ( 19.47214361940000060, 1455.728784677129852, 226.5116728881979782 ) ) ;
#93741=CARTESIAN_POINT ( 'NONE',  ( 2.779481089730000180E-10, 1406.506670174130022, 269.4986873273979882 ) ) ;
#93742=CARTESIAN_POINT ( 'NONE',  ( 27.77037800339999762, 1508.603156330129877, 207.7292936111279857 ) ) ;
#93744=CARTESIAN_POINT ( 'NONE',  ( 24.61702284729999946, 1442.198266432479841, 213.4925807370779864 ) ) ;
#93747=CARTESIAN_POINT ( 'NONE',  ( 26.35137190500821092, 1450.746515883685333, 136.5686529940089713 ) ) ;
#93749=CARTESIAN_POINT ( 'NONE',  ( 26.81567905896629966, 1435.593051660359833, 136.1631590423840237 ) ) ;
#93750=CARTESIAN_POINT ( 'NONE',  ( 40.16194930853830414, 1445.050329818410091, 136.9555904954470122 ) ) ;
#93751=DIRECTION ( 'NONE',  ( 0.7067700363771036720, 0.03085824620770448445, 0.7067700363771035610 ) ) ;
#93753=CARTESIAN_POINT ( 'NONE',  ( -17.38342248510000232, 1410.833857452530083, 225.7816926272979856 ) ) ;
#93756=CARTESIAN_POINT ( 'NONE',  ( 2.923521462801879967, 1410.394928839790055, 231.6309329194170061 ) ) ;
#93759=CARTESIAN_POINT ( 'NONE',  ( 2.660639375520162719, 1425.975332079923646, 184.4015672484581785 ) ) ;
#93762=CARTESIAN_POINT ( 'NONE',  ( 10.85919384568302526, 1424.796381347971874, 138.1955824056398399 ) ) ;
#93765=CARTESIAN_POINT ( 'NONE',  ( -28.30178298279999893, 1508.659383665829864, 209.2808554955639977 ) ) ;
#93769=CARTESIAN_POINT ( 'NONE',  ( -38.60438541162910298, 1444.259423794019995, 137.1474472167009822 ) ) ;
#93770=CARTESIAN_POINT ( 'NONE',  ( -18.10358820054819873, 1416.830086716310007, 209.2067746984330086 ) ) ;
#93771=CARTESIAN_POINT ( 'NONE',  ( 25.87716807187569756, 1435.480308988900106, 135.9284055610729922 ) ) ;
#93772=B_SPLINE_CURVE_WITH_KNOTS ( 'NONE', 3,
 ( #24632, #76175, #84016, #50442, #7857, #33597, #25194, #34168, #68354, #62162, #79499, #11733, #63272, #54314, #46460, #36376, #96288, #2806, #28533, #18443, #27977, #10634, #19565, #44802, #87907, #78955, #105242, #97382, #70018, #37485, #53771, #61601, #29087, #105807, #11196, #36924, #71121, #86779, #20121, #71689, #12268, #80593, #3359, #104132, #44242, #35835, #88980, #45360, #3907, #70565, #88442, #62732, #20654, #87338, #38036, #96853, #106338, #29624, #72216, #10068, #78386, #45902, #27418, #1694, #63808, #53198, #52642, #54856, #95734, #18998, #80038, #2262, #104683, #31280, #39116, #64358, #40787, #65464, #99022, #73856, #6632, #4444, #31832, #49208, #81666, #21748, #47003, #107983, #108542, #39688, #74963, #82786, #23427, #73296, #109113, #82236, #83336, #22298, #99571, #32393, #57620, #66018, #97925, #4972, #55950, #81126, #22857, #100141, #57063, #21192, #6081, #91736, #107431, #55402, #5537, #89534, #12823, #30726, #91188, #64911, #56500, #14469, #30168, #15010 ),
 .UNSPECIFIED., .F., .F.,
 ( 4, 3, 3, 3, 3, 3, 3, 3, 3, 3, 3, 3, 3, 3, 3, 3, 3, 3, 3, 3, 3, 3, 3, 3, 3, 3, 3, 3, 3, 3, 3, 3, 3, 3, 3, 3, 3, 3, 3, 3, 3, 4 ),
 ( -74.85727727459999414, -74.48123371302079931, -73.19548303872750239, -71.89858627928869339, -70.59406779746200300, -69.27706090161748875, -67.95207998846730391, -66.61972111345330916, -65.28071632980000061, -65.07820501495520205, -63.73244012951310111, -62.38233361708310554, -61.03011531218779595, -59.61324830631710370, -58.26014992637010437, -56.90891767115380162, -55.56075881110690062, -54.17219345129359453, -52.83759983287470163, -51.51014382337439201, -50.19057675987170342, -48.87949243769620011, -47.57733876788930161, -46.28443321930000565, -45.15800308885260250, -43.85412093733170025, -42.53885251026929382, -41.21701627981990157, -39.88454573359799582, -38.54622334132480432, -37.20301750951840347, -35.85601880476590253, -34.50543421572560732, -33.15433547973400863, -31.80422057938690017, -30.45655169721700872, -29.11270829773580004, -27.77394855399130336, -26.44138195807519764, -25.11595400857649452, -23.80322223705459805, -22.49960185790659750 ),
 .UNSPECIFIED. ) ;
#93773=CARTESIAN_POINT ( 'NONE',  ( -9.075617034181210130, 1396.229987919329915, 202.8041746642439875 ) ) ;
#93774=ORIENTED_EDGE ( 'NONE', *, *, #29645, .T. ) ;
#93776=CARTESIAN_POINT ( 'NONE',  ( -24.02854066789229748, 1507.902906607559999, 222.3115874531950169 ) ) ;
#93777=CARTESIAN_POINT ( 'NONE',  ( 21.87285660853828162, 1509.490619970689522, 226.7826239887661757 ) ) ;
#93782=CARTESIAN_POINT ( 'NONE',  ( 10.04590426459999897, 1425.199081096129930, 97.30533624469789800 ) ) ;
#93783=CARTESIAN_POINT ( 'NONE',  ( -11.10358245799999999, 1458.675538803330028, 216.3235414262480276 ) ) ;
#93784=B_SPLINE_CURVE_WITH_KNOTS ( 'NONE', 3,
 ( #74690, #13632, #14755, #6908 ),
 .UNSPECIFIED., .F., .F.,
 ( 4, 4 ),
 ( 0.000000000000000000, 1.000000000000000000 ),
 .UNSPECIFIED. ) ;
#93785=CARTESIAN_POINT ( 'NONE',  ( -20.55914306749999909, 1506.541454689430111, 190.4276830417979909 ) ) ;
#93786=CARTESIAN_POINT ( 'NONE',  ( 4.259251705083289430, 1425.302291051229759, 185.3604417148609969 ) ) ;
#93787=EDGE_CURVE ( 'NONE', #61056, #43369, #25673, .T. ) ;
#93789=CARTESIAN_POINT ( 'NONE',  ( -2.559527845430900950, 1420.757063664457291, 185.5806755108912967 ) ) ;
#93793=CARTESIAN_POINT ( 'NONE',  ( 2.500000780830000213, 1448.894380426520001, 182.3534016871979873 ) ) ;
#93796=CARTESIAN_POINT ( 'NONE',  ( -28.29825159847881011, 1510.012726057827649, 199.1527708751072794 ) ) ;
#93797=CARTESIAN_POINT ( 'NONE',  ( -1.719768424131510052E-09, 1416.259762861719992, 239.8605997301720265 ) ) ;
#93800=CARTESIAN_POINT ( 'NONE',  ( -11.84918753543019854, 1431.164029985320212, 149.8564009815129907 ) ) ;
#93802=CARTESIAN_POINT ( 'NONE',  ( -1.423698823499999877, 1472.030635481829904, 270.0714644396979907 ) ) ;
#93803=CARTESIAN_POINT ( 'NONE',  ( 12.11072210459613885, 1433.924378751797121, 147.5235493649816192 ) ) ;
#93811=CARTESIAN_POINT ( 'NONE',  ( -18.81371465716550162, 1408.757176060300026, 267.3868151054060149 ) ) ;
#93812=CARTESIAN_POINT ( 'NONE',  ( -14.42244451974389996, 1436.256339167430042, 149.9811569559620068 ) ) ;
#93815=CARTESIAN_POINT ( 'NONE',  ( 14.11808846290000119, 1443.215913278590051, 189.5356027256979985 ) ) ;
#93818=EDGE_LOOP ( 'NONE', ( #29463, #30930, #81491, #48290 ) ) ;
#93822=CIRCLE ( 'NONE', #33004, 1.999999592264639414 ) ;
#93824=CARTESIAN_POINT ( 'NONE',  ( -15.32559775480000042, 1485.482973650830218, 187.2514416256980212 ) ) ;
#93825=CARTESIAN_POINT ( 'NONE',  ( -17.61615199279099997, 1498.327676081939899, 229.4274054627400119 ) ) ;
#93829=ADVANCED_FACE ( 'NONE', ( #78267 ), #37912, .T. ) ;
#93834=CARTESIAN_POINT ( 'NONE',  ( -26.94883404700000185, 1508.590872208830206, 203.1439566689379888 ) ) ;
#93835=EDGE_CURVE ( 'NONE', #36566, #67278, #32279, .T. ) ;
#93836=B_SPLINE_SURFACE_WITH_KNOTS ( 'NONE', 5, 5, ( 
 ( #58894, #67857, #48301, #66217, #84624, #100864 ),
 ( #23623, #101969, #65651, #109844, #57807, #23057 ),
 ( #67309, #91931, #109302, #58345, #101406, #14671 ),
 ( #7377, #99767, #57266, #108179, #24155, #7921 ),
 ( #91393, #42091, #39883, #15205, #49394, #92469 ),
 ( #6816, #33122, #48859, #24697, #25255, #75155 ) ),
 .UNSPECIFIED., .F., .F., .F.,
 ( 6, 6 ),
 ( 6, 6 ),
 ( 7.312299096829999456, 16.26600630569999950 ),
 ( -3.330669073880000148E-16, 2.000000000000000000 ),
 .UNSPECIFIED. ) ;
#93837=CARTESIAN_POINT ( 'NONE',  ( -0.9123187539339999708, 1477.817894300629860, 230.7076694989980012 ) ) ;
#93838=ADVANCED_FACE ( 'NONE', ( #72645 ), #63602, .T. ) ;
#93840=CARTESIAN_POINT ( 'NONE',  ( -6.224176958410000182, 1407.473636847229955, 197.7087082664980073 ) ) ;
#93841=CARTESIAN_POINT ( 'NONE',  ( -13.55936951270000002, 1409.552479637329952, 226.6517338397979984 ) ) ;
#93845=CARTESIAN_POINT ( 'NONE',  ( 24.64286055050000002, 1488.680273900929933, 218.7263997298479694 ) ) ;
#93849=CARTESIAN_POINT ( 'NONE',  ( -23.69915799640000031, 1435.325095724740095, 137.0907082570979867 ) ) ;
#93852=CARTESIAN_POINT ( 'NONE',  ( -14.29797315729999951, 1418.019966737229879, 227.1912819175979905 ) ) ;
#93854=CIRCLE ( 'NONE', #79592, 2.000000000000068390 ) ;
#93859=EDGE_CURVE ( 'NONE', #94676, #54104, #97874, .T. ) ;
#93865=CARTESIAN_POINT ( 'NONE',  ( 11.97008865472790085, 1434.984363622560068, 151.1079544380379787 ) ) ;
#93866=CARTESIAN_POINT ( 'NONE',  ( -4.078748368091082988, 1441.172350307923807, 184.7183383138763588 ) ) ;
#93869=CARTESIAN_POINT ( 'NONE',  ( -0.8378199854720000950, 1507.147729960229753, 180.8463070743979983 ) ) ;
#93871=CARTESIAN_POINT ( 'NONE',  ( -1.137524366430000100, 1408.952783613529846, 187.3908199154979854 ) ) ;
#93872=EDGE_CURVE ( 'NONE', #67049, #105289, #11031, .T. ) ;
#93876=CARTESIAN_POINT ( 'NONE',  ( 13.58268853708210067, 1416.851343896850040, 196.3340833727469885 ) ) ;
#93877=CARTESIAN_POINT ( 'NONE',  ( 19.97699626480000035, 1508.102459361230103, 189.1029257653979982 ) ) ;
#93880=CARTESIAN_POINT ( 'NONE',  ( -12.27023112300000030, 1416.839692131129823, 194.6640134917980163 ) ) ;
#93882=ORIENTED_EDGE ( 'NONE', *, *, #86258, .T. ) ;
#93884=CARTESIAN_POINT ( 'NONE',  ( 0.1674543970350000077, 1419.793577484730122, 184.3767484295979955 ) ) ;
#93891=CARTESIAN_POINT ( 'NONE',  ( 18.64588652299999794, 1416.828040475229955, 209.6843149956849857 ) ) ;
#93892=CARTESIAN_POINT ( 'NONE',  ( 18.69800617379813801, 1425.875008635436643, 224.9978991839990954 ) ) ;
#93893=DIRECTION ( 'NONE',  ( 0.000000000000000000, 1.000000000000000000, 0.000000000000000000 ) ) ;
#93895=CARTESIAN_POINT ( 'NONE',  ( -2.265645423020000049, 1414.246892558129957, 164.3383647881979925 ) ) ;
#93899=ORIENTED_EDGE ( 'NONE', *, *, #95927, .T. ) ;
#93902=CARTESIAN_POINT ( 'NONE',  ( -24.41204057910000103, 1440.938895779720042, 212.0297384891179888 ) ) ;
#93906=EDGE_CURVE ( 'NONE', #48999, #101369, #61201, .T. ) ;
#93908=CARTESIAN_POINT ( 'NONE',  ( 13.20846944180000015, 1414.988015876730060, 197.7899243527979820 ) ) ;
#93910=CARTESIAN_POINT ( 'NONE',  ( 23.90214117500000057, 1451.650320089529941, 139.9216469008979971 ) ) ;
#93912=CARTESIAN_POINT ( 'NONE',  ( -29.75012120250000081, 1509.993914124430148, 208.5595671623779879 ) ) ;
#93915=VERTEX_POINT ( 'NONE', #103890 ) ;
#93916=CARTESIAN_POINT ( 'NONE',  ( -17.62491468606772926, 1460.289161246174444, 228.1912235019598540 ) ) ;
#93920=EDGE_LOOP ( 'NONE', ( #81621, #17405, #66864, #80764 ) ) ;
#93921=CARTESIAN_POINT ( 'NONE',  ( 17.33159214698790151, 1507.668127079400165, 230.9408589578669933 ) ) ;
#93923=CARTESIAN_POINT ( 'NONE',  ( 37.05187274396420349, 1437.940711956549876, 136.5605698765780005 ) ) ;
#93924=CARTESIAN_POINT ( 'NONE',  ( 20.71063674850000069, 1470.804162803530062, 209.3922244785459839 ) ) ;
#93930=CARTESIAN_POINT ( 'NONE',  ( -12.83448315710464094, 1435.932405785817082, 150.8148811484861085 ) ) ;
#93932=CARTESIAN_POINT ( 'NONE',  ( 1.843841672930000009, 1409.915254994430143, 185.4154735675980135 ) ) ;
#93934=CARTESIAN_POINT ( 'NONE',  ( 40.27308693906149273, 1443.611999474700042, 137.1163322506119755 ) ) ;
#93935=CARTESIAN_POINT ( 'NONE',  ( 10.83341016640000021, 1434.513252767399763, 151.9041015218980135 ) ) ;
#93936=CARTESIAN_POINT ( 'NONE',  ( -3.117233513421850066, 1441.234898769120036, 170.5448813734479927 ) ) ;
#93937=CARTESIAN_POINT ( 'NONE',  ( 11.76196284288320015, 1425.587143582329873, 146.3421855601949915 ) ) ;
#93938=CARTESIAN_POINT ( 'NONE',  ( 1.430284437999999936, 1465.025931307530072, 237.8691342077979982 ) ) ;
#93939=VERTEX_POINT ( 'NONE', #104999 ) ;
#93942=CARTESIAN_POINT ( 'NONE',  ( -42.15579669299999921, 1443.896589930619939, 269.8789809301979403 ) ) ;
#93943=CARTESIAN_POINT ( 'NONE',  ( -23.72545963659144874, 1436.118670184939447, 211.8535580904316191 ) ) ;
#93944=FACE_OUTER_BOUND ( 'NONE', #93920, .T. ) ;
#93945=CARTESIAN_POINT ( 'NONE',  ( 14.54088607839999980, 1410.754219483329962, 191.4792867801979810 ) ) ;
#93946=EDGE_CURVE ( 'NONE', #98935, #77078, #1723, .T. ) ;
#93950=CARTESIAN_POINT ( 'NONE',  ( -8.352280533070000956, 1418.964256225429835, 232.1493934695980101 ) ) ;
#93954=CARTESIAN_POINT ( 'NONE',  ( 0.01072155311641910871, 1486.299748484872907, 181.8129703845364133 ) ) ;
#93957=CARTESIAN_POINT ( 'NONE',  ( -45.75507445926909611, 1438.283494741970117, 266.4162312795270395 ) ) ;
#93958=CARTESIAN_POINT ( 'NONE',  ( 13.58148582911039881, 1508.837191255689959, 233.6100809729150001 ) ) ;
#93959=ADVANCED_FACE ( 'NONE', ( #61372 ), #12616, .T. ) ;
#93960=CARTESIAN_POINT ( 'NONE',  ( -12.98226713004480004, 1414.913060387349788, 219.9156686614909972 ) ) ;
#93961=ORIENTED_EDGE ( 'NONE', *, *, #53441, .T. ) ;
#93963=CARTESIAN_POINT ( 'NONE',  ( -2.478930769269999779, 1432.582979956780036, 157.5229504622980130 ) ) ;
#93965=CARTESIAN_POINT ( 'NONE',  ( -26.31343033946440002, 1441.279830965969950, 137.8584457592320121 ) ) ;
#93967=CARTESIAN_POINT ( 'NONE',  ( -26.37095841104669702, 1451.986996602540103, 135.1286765312639773 ) ) ;
#93969=CARTESIAN_POINT ( 'NONE',  ( 22.58796458730000012, 1427.336410677830145, 231.9597913024979903 ) ) ;
#93971=CARTESIAN_POINT ( 'NONE',  ( 13.85241133699999949, 1452.817890303829927, 195.1465048085980243 ) ) ;
#93973=CARTESIAN_POINT ( 'NONE',  ( 1.801533744329999909, 1412.572206465630188, 232.2925451922980074 ) ) ;
#93980=CARTESIAN_POINT ( 'NONE',  ( -6.563901503888989630, 1410.596044972080108, 269.6193547258999956 ) ) ;
#93981=CARTESIAN_POINT ( 'NONE',  ( 4.104804799730410458, 1416.793721508729732, 231.8084991735399853 ) ) ;
#93983=CARTESIAN_POINT ( 'NONE',  ( -2.500000000000000000, 1439.509563876250013, 163.9071501952790300 ) ) ;
#93987=EDGE_CURVE ( 'NONE', #32165, #44736, #76465, .T. ) ;
#93988=CARTESIAN_POINT ( 'NONE',  ( -0.08584137263299880527, 1408.916058034080152, 186.4688618524710080 ) ) ;
#93990=CARTESIAN_POINT ( 'NONE',  ( -39.51550670970809165, 1423.010682514669952, 266.3652739410081836 ) ) ;
#93991=EDGE_CURVE ( 'NONE', #9014, #17632, #96492, .T. ) ;
#93992=CARTESIAN_POINT ( 'NONE',  ( -20.83970284856240340, 1501.660516804690133, 192.3719794906700145 ) ) ;
#93994=CARTESIAN_POINT ( 'NONE',  ( -17.72560687289999848, 1420.841998356029990, 226.0101997189979954 ) ) ;
#93995=CARTESIAN_POINT ( 'NONE',  ( 35.78853434691840363, 1463.243804785920020, 267.3096158296730209 ) ) ;
#93996=AXIS2_PLACEMENT_3D ( 'NONE', #5569, #23457, #31308 ) ;
#93997=CARTESIAN_POINT ( 'NONE',  ( -3.481252530716044458, 1466.728071799404233, 234.8984253771955935 ) ) ;
#93998=CARTESIAN_POINT ( 'NONE',  ( -17.33992335449591238, 1422.584892946659920, 226.5971582259074637 ) ) ;
#94000=VERTEX_POINT ( 'NONE', #83862 ) ;
#94001=CARTESIAN_POINT ( 'NONE',  ( -11.94180849701186631, 1433.516162581537174, 150.0911432144437470 ) ) ;
#94005=CARTESIAN_POINT ( 'NONE',  ( -1.123912433469769878, 1458.003495002930094, 229.8665499421440188 ) ) ;
#94006=CARTESIAN_POINT ( 'NONE',  ( 26.70809291654819972, 1451.980330768489921, 135.0059442101320144 ) ) ;
#94008=CARTESIAN_POINT ( 'NONE',  ( -1.543833121739990100, 1424.175334750540060, 228.3471663839470125 ) ) ;
#94010=EDGE_CURVE ( 'NONE', #56530, #11508, #23936, .T. ) ;
#94011=CARTESIAN_POINT ( 'NONE',  ( 18.50818375480000100, 1409.559380405929915, 219.7813082434980174 ) ) ;
#94013=CARTESIAN_POINT ( 'NONE',  ( 8.043739714546198627, 1409.193953967760081, 189.2334580016899963 ) ) ;
#94014=CARTESIAN_POINT ( 'NONE',  ( 1.379877562750000175, 1416.709753722929918, 233.1857291387979956 ) ) ;
#94015=CARTESIAN_POINT ( 'NONE',  ( -18.07895559939639796, 1423.750420671800157, 225.6737883517463672 ) ) ;
#94016=CARTESIAN_POINT ( 'NONE',  ( 10.56558922819999857, 1409.282018893330132, 228.0601045111980056 ) ) ;
#94018=EDGE_CURVE ( 'NONE', #98127, #73912, #34134, .T. ) ;
#94022=CARTESIAN_POINT ( 'NONE',  ( 11.74913122504709939, 1432.337153681070049, 150.6947002683050130 ) ) ;
#94023=DIRECTION ( 'NONE',  ( 1.025155669219414347E-18, -1.000000000000000000, 0.000000000000000000 ) ) ;
#94029=CARTESIAN_POINT ( 'NONE',  ( -13.66603629819999810, 1471.441739209529942, 271.1218459616979999 ) ) ;
#94030=CARTESIAN_POINT ( 'NONE',  ( -21.91509347160294396, 1509.516311833964437, 191.4267936841458493 ) ) ;
#94031=CARTESIAN_POINT ( 'NONE',  ( 11.89524296629999967, 1433.269816950409904, 149.9550912523980060 ) ) ;
#94032=CARTESIAN_POINT ( 'NONE',  ( 19.47651264659999626, 1455.559577376729976, 243.9198229517980110 ) ) ;
#94033=CARTESIAN_POINT ( 'NONE',  ( 12.50317167496160131, 1415.933499560010205, 196.3719056758750128 ) ) ;
#94038=CARTESIAN_POINT ( 'NONE',  ( -17.59109303050000150, 1486.013267125129914, 188.2745623029979924 ) ) ;
#94039=CARTESIAN_POINT ( 'NONE',  ( 11.80540162446047603, 1398.263086677583033, 214.5664719749284473 ) ) ;
#94040=CARTESIAN_POINT ( 'NONE',  ( 2.385953148540000068, 1466.626847306429909, 234.2518259445980107 ) ) ;
#94041=CARTESIAN_POINT ( 'NONE',  ( 23.75028666869999938, 1410.916158841730066, 210.9577920301479992 ) ) ;
#94042=CARTESIAN_POINT ( 'NONE',  ( 12.26979804483799974, 1416.828039243390094, 223.5793509210460002 ) ) ;
#94043=CARTESIAN_POINT ( 'NONE',  ( 26.51057051087156680, 1436.730213643903198, 136.8073690796935011 ) ) ;
#94045=CARTESIAN_POINT ( 'NONE',  ( 11.40809304261581403, 1434.668754042350429, 151.4869022581049194 ) ) ;
#94049=CARTESIAN_POINT ( 'NONE',  ( 0.2057925133900349868, 1459.718704435009840, 182.9651470494519856 ) ) ;
#94054=CARTESIAN_POINT ( 'NONE',  ( 12.06086588840000040, 1433.903735958359903, 149.7888706136980090 ) ) ;
#94055=CARTESIAN_POINT ( 'NONE',  ( -41.50828902776399332, 1442.131284357510140, 134.0999999980909934 ) ) ;
#94057=ORIENTED_EDGE ( 'NONE', *, *, #17863, .T. ) ;
#94060=CARTESIAN_POINT ( 'NONE',  ( -14.39499459219999977, 1414.971339025629959, 218.6292155375679727 ) ) ;
#94071=EDGE_LOOP ( 'NONE', ( #63243, #49909, #99177, #64129, #20568, #107865, #76453 ) ) ;
#94072=CARTESIAN_POINT ( 'NONE',  ( -33.31575678469999247, 1451.596268149030038, 135.6057732153979885 ) ) ;
#94073=CARTESIAN_POINT ( 'NONE',  ( 11.60004869885203682, 1428.983126981193436, 134.0999999980966777 ) ) ;
#94074=EDGE_LOOP ( 'NONE', ( #91797, #110712, #38229, #61377 ) ) ;
#94079=EDGE_CURVE ( 'NONE', #75001, #44739, #105700, .T. ) ;
#94081=CARTESIAN_POINT ( 'NONE',  ( 16.33922116421775428, 1432.268274340457310, 218.1941633188057779 ) ) ;
#94082=CARTESIAN_POINT ( 'NONE',  ( 1.808028501710000180, 1417.177841219630182, 232.8705156747979856 ) ) ;
#94089=CARTESIAN_POINT ( 'NONE',  ( 2.499999999749999979, 1448.248598671410036, 156.2048689938979749 ) ) ;
#94091=CARTESIAN_POINT ( 'NONE',  ( 40.34922463040000196, 1457.054874283830031, 269.7804020139980139 ) ) ;
#94093=VERTEX_POINT ( 'NONE', #49731 ) ;
#94095=CARTESIAN_POINT ( 'NONE',  ( 1.804213551060599885, 1410.351307734219972, 232.1928989352460064 ) ) ;
#94099=CARTESIAN_POINT ( 'NONE',  ( -21.05081438890000101, 1449.791259199039814, 196.5491838007980050 ) ) ;
#94100=CARTESIAN_POINT ( 'NONE',  ( -11.12709171348789994, 1426.472547912719847, 99.91404471913999430 ) ) ;
#94101=CARTESIAN_POINT ( 'NONE',  ( 17.14529549334500302, 1410.143790924649920, 192.4629487703649886 ) ) ;
#94104=CARTESIAN_POINT ( 'NONE',  ( 1.758988666023477698, 1450.448601557000757, 181.8112131745612885 ) ) ;
#94105=CARTESIAN_POINT ( 'NONE',  ( -37.17587469459999738, 1423.049458637629868, 264.1764750911980286 ) ) ;
#94107=CARTESIAN_POINT ( 'NONE',  ( 28.66375039995369889, 1509.283859617730059, 209.4897258303710146 ) ) ;
#94108=EDGE_CURVE ( 'NONE', #36324, #73043, #24491, .T. ) ;
#94110=CARTESIAN_POINT ( 'NONE',  ( -39.25138508177120400, 1440.085603367899921, 136.7362581835410253 ) ) ;
#94112=CARTESIAN_POINT ( 'NONE',  ( 8.792868328939640321, 1397.264807581909963, 218.9196783556029970 ) ) ;
#94115=CARTESIAN_POINT ( 'NONE',  ( -17.79268936480000107, 1459.536118998330039, 228.1430453449980007 ) ) ;
#94116=VERTEX_POINT ( 'NONE', #7163 ) ;
#94119=CARTESIAN_POINT ( 'NONE',  ( -3.165116544085609718, 1422.680544489370277, 151.1405016111839927 ) ) ;
#94123=CARTESIAN_POINT ( 'NONE',  ( -0.4967073565345429542, 1415.438070636819930, 233.3911243540180180 ) ) ;
#94124=CARTESIAN_POINT ( 'NONE',  ( 13.69373227756942057, 1507.296992741110671, 227.3135802372769092 ) ) ;
#94126=CARTESIAN_POINT ( 'NONE',  ( -2.573686490390000081, 1461.195040433729901, 234.8853213935979909 ) ) ;
#94127=CARTESIAN_POINT ( 'NONE',  ( 2.161235707085400026, 1421.184930282719961, 183.1997352710330063 ) ) ;
#94129=CARTESIAN_POINT ( 'NONE',  ( 38.50397186617925627, 1443.086052842850904, 136.9545993544632552 ) ) ;
#94135=CARTESIAN_POINT ( 'NONE',  ( 11.79631778455750002, 1428.064473684170025, 147.9895841176879685 ) ) ;
#94138=CARTESIAN_POINT ( 'NONE',  ( -13.73564804769999981, 1415.163755998629995, 220.6561513494980034 ) ) ;
#94139=CARTESIAN_POINT ( 'NONE',  ( -11.58617079055879806, 1432.339219433009930, 151.0669314679269917 ) ) ;
#94140=CARTESIAN_POINT ( 'NONE',  ( 4.966585816180000279, 1508.577461573030178, 236.2865006180979890 ) ) ;
#94142=CARTESIAN_POINT ( 'NONE',  ( -4.895323701719999754, 1423.483672866529787, 184.9472429021979849 ) ) ;
#94145=CARTESIAN_POINT ( 'NONE',  ( -9.840626851222889826, 1410.631480589668854, 188.3682688390927638 ) ) ;
#94147=CARTESIAN_POINT ( 'NONE',  ( 23.05067725217429953, 1422.501892093690003, 206.2034611426070114 ) ) ;
#94150=CARTESIAN_POINT ( 'NONE',  ( -5.007627065198849259, 1423.109407737726542, 184.7889011730115669 ) ) ;
#94154=CARTESIAN_POINT ( 'NONE',  ( 5.360207926212690488, 1422.242713656610022, 144.1549664376839814 ) ) ;
#94157=CARTESIAN_POINT ( 'NONE',  ( -2.899874285569436161, 1484.420918474829932, 183.3032565327546592 ) ) ;
#94161=ORIENTED_EDGE ( 'NONE', *, *, #109775, .F. ) ;
#94162=CARTESIAN_POINT ( 'NONE',  ( 1.514732344039999790, 1507.625766668030110, 186.2043550924979911 ) ) ;
#94163=CARTESIAN_POINT ( 'NONE',  ( -12.78690713350000152, 1416.828040475229955, 195.5394874918979724 ) ) ;
#94164=CARTESIAN_POINT ( 'NONE',  ( -11.24637745149999901, 1428.358274944230061, 150.3272095878980110 ) ) ;
#94166=CARTESIAN_POINT ( 'NONE',  ( -4.219439073160000220, 1441.595895977600094, 183.5288107362979702 ) ) ;
#94170=CARTESIAN_POINT ( 'NONE',  ( -2.461716435160000049, 1435.943783413959864, 150.4083956814980070 ) ) ;
#94173=LINE ( 'NONE', #109350, #74668 ) ;
#94174=VERTEX_POINT ( 'NONE', #87181 ) ;
#94176=CARTESIAN_POINT ( 'NONE',  ( 26.99677755089999920, 1412.522578206929893, 268.7553209094979820 ) ) ;
#94178=CARTESIAN_POINT ( 'NONE',  ( 22.65318487140000059, 1449.722345962300096, 199.2838700365680040 ) ) ;
#94179=B_SPLINE_CURVE_WITH_KNOTS ( 'NONE', 5,
 ( #61753, #105950, #10780, #21342, #55005, #89131 ),
 .UNSPECIFIED., .F., .F.,
 ( 6, 6 ),
 ( -74.90934616261959889, -17.77505807049999476 ),
 .UNSPECIFIED. ) ;
#94180=CARTESIAN_POINT ( 'NONE',  ( -0.2086532769659229791, 1507.120225578089958, 237.3378754264870167 ) ) ;
#94183=CARTESIAN_POINT ( 'NONE',  ( -1.271867598320000292, 1450.975052773130074, 183.1634528037979806 ) ) ;
#94184=CARTESIAN_POINT ( 'NONE',  ( 14.92875414504869980, 1473.796938403280137, 194.5760049489949779 ) ) ;
#94186=CARTESIAN_POINT ( 'NONE',  ( -14.12261623989999926, 1444.009911080699794, 188.5535776405979789 ) ) ;
#94189=CARTESIAN_POINT ( 'NONE',  ( -1.530900592538410043, 1457.980095062469900, 229.8454460011110143 ) ) ;
#94192=CARTESIAN_POINT ( 'NONE',  ( -13.46159057049859875, 1409.383149488619893, 202.6401911298929974 ) ) ;
#94195=CARTESIAN_POINT ( 'NONE',  ( -14.64149520810000027, 1474.304963572530141, 268.3932719582979871 ) ) ;
#94198=CARTESIAN_POINT ( 'NONE',  ( -24.06860914254439621, 1444.374860723432676, 212.0637649108989251 ) ) ;
#94201=CARTESIAN_POINT ( 'NONE',  ( 11.82816149694599872, 1415.492117401570113, 223.1475517754469990 ) ) ;
#94203=LINE ( 'NONE', #67389, #1898 ) ;
#94204=CARTESIAN_POINT ( 'NONE',  ( -46.05259875475182696, 1440.913026109461498, 266.6770514725025691 ) ) ;
#94205=CARTESIAN_POINT ( 'NONE',  ( -22.53916331800000350, 1409.864589572430077, 205.1045926694380057 ) ) ;
#94206=CARTESIAN_POINT ( 'NONE',  ( 15.72677903779999831, 1414.913060387329779, 204.2094322949480159 ) ) ;
#94208=DIRECTION ( 'NONE',  ( 0.08077839049150441209, -0.9967320861844480850, 0.000000000000000000 ) ) ;
#94209=CARTESIAN_POINT ( 'NONE',  ( 24.18363701780000241, 1464.258769156330118, 206.0765659417580196 ) ) ;
#94210=VECTOR ( 'NONE', #57561, 1000.000000000000114 ) ;
#94214=CARTESIAN_POINT ( 'NONE',  ( -22.77127499929999743, 1411.073674604029975, 211.3149786677880115 ) ) ;
#94216=CARTESIAN_POINT ( 'NONE',  ( 11.72356565703490006, 1426.704528874140124, 143.2054359492850040 ) ) ;
#94219=B_SPLINE_CURVE_WITH_KNOTS ( 'NONE', 3,
 ( #44396, #46612, #95885, #97002 ),
 .UNSPECIFIED., .F., .F.,
 ( 4, 4 ),
 ( 123.8981301339999987, 143.2822930380000059 ),
 .UNSPECIFIED. ) ;
#94221=CARTESIAN_POINT ( 'NONE',  ( -17.27558692971449972, 1507.606285623229951, 224.2552697136770234 ) ) ;
#94223=CARTESIAN_POINT ( 'NONE',  ( -8.039183776086851196, 1398.151822053308933, 219.3381333954307593 ) ) ;
#94233=CARTESIAN_POINT ( 'NONE',  ( 11.90939254660839985, 1433.635556608139950, 150.4772598317650250 ) ) ;
#94236=CARTESIAN_POINT ( 'NONE',  ( -0.0003153230261271207065, 1396.811848177620050, 221.8113320389208809 ) ) ;
#94237=CARTESIAN_POINT ( 'NONE',  ( -23.61138782050000273, 1508.482532590330038, 195.6450445675980063 ) ) ;
#94240=FACE_OUTER_BOUND ( 'NONE', #49085, .T. ) ;
#94241=CARTESIAN_POINT ( 'NONE',  ( 19.49173981795879840, 1498.116573650230066, 228.9790417235219877 ) ) ;
#94242=CARTESIAN_POINT ( 'NONE',  ( 1.210143529950000074, 1488.175041650030153, 181.8896941532979952 ) ) ;
#94245=EDGE_CURVE ( 'NONE', #41855, #10827, #103010, .T. ) ;
#94248=CARTESIAN_POINT ( 'NONE',  ( 34.92262156983900212, 1435.778361306969828, 134.0999999978019730 ) ) ;
#94249=CARTESIAN_POINT ( 'NONE',  ( 11.86558108900000086, 1432.299711256910086, 149.9824918235980249 ) ) ;
#94251=VERTEX_POINT ( 'NONE', #1533 ) ;
#94252=CARTESIAN_POINT ( 'NONE',  ( 13.74692504272130122, 1435.515273018320158, 150.0128078956250306 ) ) ;
#94253=EDGE_LOOP ( 'NONE', ( #101120, #103791, #86089, #55860, #68383 ) ) ;
#94255=CARTESIAN_POINT ( 'NONE',  ( 13.14995078890901681, 1444.757455661086169, 169.3984255879898626 ) ) ;
#94256=CARTESIAN_POINT ( 'NONE',  ( -0.7477858788270000945, 1465.398313615129837, 236.2223280954979998 ) ) ;
#94264=EDGE_CURVE ( 'NONE', #22920, #25299, #19943, .T. ) ;
#94269=VERTEX_POINT ( 'NONE', #96129 ) ;
#94270=ADVANCED_FACE ( 'NONE', ( #26143 ), #103404, .T. ) ;
#94271=CARTESIAN_POINT ( 'NONE',  ( -13.15560506839999988, 1409.874636222130221, 190.0057851175980090 ) ) ;
#94275=CARTESIAN_POINT ( 'NONE',  ( 24.22543016360000223, 1436.719751587260134, 213.3442258677480083 ) ) ;
#94278=CARTESIAN_POINT ( 'NONE',  ( 0.003825492543937429601, 1466.393772595959945, 235.6965109011690060 ) ) ;
#94279=LINE ( 'NONE', #17556, #39599 ) ;
#94280=AXIS2_PLACEMENT_3D ( 'NONE', #91128, #14405, #11962 ) ;
#94283=CARTESIAN_POINT ( 'NONE',  ( -21.06166912470000341, 1509.324064458830208, 189.5257785579979952 ) ) ;
#94286=CARTESIAN_POINT ( 'NONE',  ( 13.85929690100000045, 1410.325638471030061, 191.1496520999980078 ) ) ;
#94292=CARTESIAN_POINT ( 'NONE',  ( 26.19684153890000289, 1465.282679496030141, 259.6167425913980082 ) ) ;
#94293=CARTESIAN_POINT ( 'NONE',  ( 2.479191938638227732, 1452.138930638437387, 183.7341620333366166 ) ) ;
#94294=CARTESIAN_POINT ( 'NONE',  ( -11.86716023049999968, 1432.353341358199941, 147.6509521729980179 ) ) ;
#94295=CARTESIAN_POINT ( 'NONE',  ( -7.652862273441430219, 1508.994713535709934, 236.5479620134960044 ) ) ;
#94299=CARTESIAN_POINT ( 'NONE',  ( 19.47028325960000217, 1455.696635970729858, 226.3889713599980098 ) ) ;
#94304=CARTESIAN_POINT ( 'NONE',  ( 0.3396529269219999980, 1405.776763257430048, 268.4837298631979934 ) ) ;
#94305=CARTESIAN_POINT ( 'NONE',  ( 28.17856933310000045, 1509.667335739130067, 207.1106752990980056 ) ) ;
#94307=CARTESIAN_POINT ( 'NONE',  ( 24.50134868650000186, 1443.648489106190027, 213.6791898706979964 ) ) ;
#94311=CARTESIAN_POINT ( 'NONE',  ( 28.37195397669790253, 1435.488266588540000, 135.2384698397310103 ) ) ;
#94312=CARTESIAN_POINT ( 'NONE',  ( 35.84500107954239922, 1450.075251917649894, 136.2401620429770048 ) ) ;
#94313=CARTESIAN_POINT ( 'NONE',  ( 3.360259919131120113E-15, 1458.663800951910162, 232.7180369472359871 ) ) ;
#94320=CARTESIAN_POINT ( 'NONE',  ( 0.2331202188386839735, 1408.921201124740037, 186.4825399812679905 ) ) ;
#94321=CARTESIAN_POINT ( 'NONE',  ( 12.40450132490000179, 1434.419879851630185, 146.7589221149980006 ) ) ;
#94323=CARTESIAN_POINT ( 'NONE',  ( 15.25323211731929973, 1454.458797326860122, 189.7583580193819728 ) ) ;
#94324=CARTESIAN_POINT ( 'NONE',  ( -0.7333927689999999444, 1417.382029894330117, 235.1308572242979835 ) ) ;
#94327=CARTESIAN_POINT ( 'NONE',  ( -29.77420895410000057, 1509.998730836529830, 208.8314797160269904 ) ) ;
#94330=CARTESIAN_POINT ( 'NONE',  ( -9.338711182531437061, 1417.673218423038179, 230.3173475666119998 ) ) ;
#94331=CARTESIAN_POINT ( 'NONE',  ( -21.03297590181131582, 1450.947314460161351, 144.4212294945661768 ) ) ;
#94333=CARTESIAN_POINT ( 'NONE',  ( 23.99831809630000024, 1435.341613007889919, 136.9207814653979938 ) ) ;
#94334=CARTESIAN_POINT ( 'NONE',  ( -11.02512559413370141, 1396.298066256809761, 208.1314111368130000 ) ) ;
#94336=CARTESIAN_POINT ( 'NONE',  ( -17.36307779888920066, 1410.600141639559979, 225.7635892599339797 ) ) ;
#94337=CARTESIAN_POINT ( 'NONE',  ( 7.346057189749999772, 1434.541746329560056, 149.5958201245979922 ) ) ;
#94339=ORIENTED_EDGE ( 'NONE', *, *, #91348, .T. ) ;
#94344=CARTESIAN_POINT ( 'NONE',  ( 4.383945358651920365, 1425.749019032469960, 185.4609551595589778 ) ) ;
#94346=CARTESIAN_POINT ( 'NONE',  ( -2.571138338408573532, 1420.704546681525699, 185.6354774934253840 ) ) ;
#94350=CARTESIAN_POINT ( 'NONE',  ( 2.864767215090000096, 1448.949360505710047, 183.5737851087979777 ) ) ;
#94355=CARTESIAN_POINT ( 'NONE',  ( -41.14440994790000161, 1444.077640937079877, 136.9184649836980157 ) ) ;
#94358=CARTESIAN_POINT ( 'NONE',  ( -7.875528793950000407E-10, 1472.619496933430128, 270.3713665234980112 ) ) ;
#94360=CARTESIAN_POINT ( 'NONE',  ( 0.1141191476639999841, 1485.968486491729891, 182.2121106956980157 ) ) ;
#94363=CARTESIAN_POINT ( 'NONE',  ( -33.91368313123930278, 1450.440614192689964, 136.2454513106639808 ) ) ;
#94365=CARTESIAN_POINT ( 'NONE',  ( -13.22806383200000013, 1431.113060387329824, 195.8937821299979873 ) ) ;
#94367=CARTESIAN_POINT ( 'NONE',  ( 9.106334930605640920, 1408.186707947460036, 198.7849738689709795 ) ) ;
#94368=CARTESIAN_POINT ( 'NONE',  ( -18.83033903852280133, 1408.714486736299932, 267.7018036114649817 ) ) ;
#94369=B_SPLINE_CURVE_WITH_KNOTS ( 'NONE', 3,
 ( #61788, #95910, #44421, #53377, #68524, #8033, #10245, #43858, #78005, #76914, #69639, #60681, #25924, #76353, #60121, #77463, #27063, #110502, #765, #61249, #69082, #103183, #29256, #44982, #79131, #62341, #38200, #12449, #38744, #98651, #98100, #2439, #105418, #47168, #96466, #2985, #10813, #36554, #107061, #81296, #106512, #20287, #71304, #21372, #64536, #4610, #55581, #4075, #3532, #54493, #46633, #72922, #30345, #37105, #63447 ),
 .UNSPECIFIED., .F., .F.,
 ( 4, 3, 3, 3, 3, 3, 3, 3, 3, 3, 3, 3, 3, 3, 3, 3, 3, 3, 4 ),
 ( -169.6276195580000206, -126.5933223886119947, -88.68156620233840215, -52.61810133791399835, -51.73140211568609459, -50.56540007835791073, -49.37793206528289147, -48.17557270853839668, -46.94365568215079065, -45.68967734683630511, -44.41100891884349267, -43.10437972021219366, -41.74527663196900562, -40.34034550197179669, -38.87942175190678995, -37.34527141349130375, -35.70714590379060382, -33.89535962364968213, -31.55396706740000923 ),
 .UNSPECIFIED. ) ;
#94371=VERTEX_POINT ( 'NONE', #9913 ) ;
#94372=CARTESIAN_POINT ( 'NONE',  ( -11.86538722380000088, 1432.286166193919826, 149.9824190662980072 ) ) ;
#94373=CARTESIAN_POINT ( 'NONE',  ( 13.47846152179999990, 1444.303430095470048, 188.1230873751979686 ) ) ;
#94374=ORIENTED_EDGE ( 'NONE', *, *, #92623, .F. ) ;
#94377=CARTESIAN_POINT ( 'NONE',  ( 4.939111363942668476, 1423.323286052371714, 184.2638540454798886 ) ) ;
#94380=CARTESIAN_POINT ( 'NONE',  ( -18.39416877649999904, 1470.473699348829996, 189.9134802429980198 ) ) ;
#94385=FACE_OUTER_BOUND ( 'NONE', #73325, .T. ) ;
#94387=CARTESIAN_POINT ( 'NONE',  ( -28.44576460359999714, 1509.873577826230076, 203.8870703132379845 ) ) ;
#94388=DIRECTION ( 'NONE',  ( -0.000000000000000000, -0.000000000000000000, 1.000000000000000000 ) ) ;
#94391=CARTESIAN_POINT ( 'NONE',  ( -1.288987972930000003, 1407.277489897129954, 196.1207496164979887 ) ) ;
#94393=CARTESIAN_POINT ( 'NONE',  ( -5.705323726350000513, 1447.426426495140049, 185.3480178495979658 ) ) ;
#94395=CARTESIAN_POINT ( 'NONE',  ( -24.65352725776519804, 1430.511890270439835, 210.2240530382869963 ) ) ;
#94396=CARTESIAN_POINT ( 'NONE',  ( 25.47381561340000289, 1508.124471600029892, 219.0002699717279881 ) ) ;
#94398=CARTESIAN_POINT ( 'NONE',  ( -25.10800663690000079, 1436.295742790639906, 137.5680277278979986 ) ) ;
#94403=CARTESIAN_POINT ( 'NONE',  ( -14.60531145299999878, 1420.435034123629976, 227.1460274248979943 ) ) ;
#94404=DIRECTION ( 'NONE',  ( 0.000000000000000000, 0.000000000000000000, 1.000000000000000000 ) ) ;
#94407=CARTESIAN_POINT ( 'NONE',  ( 2.500000000000000000, 1435.404599731399912, 157.5892871108979989 ) ) ;
#94408=CARTESIAN_POINT ( 'NONE',  ( -2.365925665009999790, 1412.840979806830092, 232.8160838550979861 ) ) ;
#94413=CARTESIAN_POINT ( 'NONE',  ( 12.23060000949119974, 1434.169197542179973, 149.9832296201709880 ) ) ;
#94414=CARTESIAN_POINT ( 'NONE',  ( 16.77391199951920342, 1459.306422992139915, 228.8325835937480122 ) ) ;
#94415=CARTESIAN_POINT ( 'NONE',  ( -21.33188221090540182, 1507.840646589619837, 227.2305681273250002 ) ) ;
#94417=CARTESIAN_POINT ( 'NONE',  ( -2.760778490449999900, 1409.009468896630096, 188.0459414135980012 ) ) ;
#94418=B_SPLINE_CURVE_WITH_KNOTS ( 'NONE', 5,
 ( #6807, #51035, #109834, #49933, #58885, #24146 ),
 .UNSPECIFIED., .F., .F.,
 ( 6, 6 ),
 ( -93.91916526269999110, -17.09700588378190389 ),
 .UNSPECIFIED. ) ;
#94420=LINE ( 'NONE', #17140, #16477 ) ;
#94421=EDGE_CURVE ( 'NONE', #62944, #41530, #61514, .T. ) ;
#94425=CARTESIAN_POINT ( 'NONE',  ( -2.500000000000000000, 1419.383100980419840, 144.1003751433630100 ) ) ;
#94426=ORIENTED_EDGE ( 'NONE', *, *, #68016, .F. ) ;
#94427=CARTESIAN_POINT ( 'NONE',  ( -12.26979143229999991, 1416.828042640230024, 194.6643372026980217 ) ) ;
#94428=CARTESIAN_POINT ( 'NONE',  ( -11.60004869885203682, 1426.043662085331562, 137.7527993286476544 ) ) ;
#94430=CARTESIAN_POINT ( 'NONE',  ( 3.571721340409999890, 1420.465157505230081, 185.4391698450980073 ) ) ;
#94434=CARTESIAN_POINT ( 'NONE',  ( -26.35977987659270028, 1508.073080378489749, 201.5431538711860071 ) ) ;
#94435=CARTESIAN_POINT ( 'NONE',  ( -16.38947255413719617, 1409.756821326547652, 192.2387554727406496 ) ) ;
#94436=CARTESIAN_POINT ( 'NONE',  ( 18.46483594369999892, 1415.628674276829770, 210.6745050120780149 ) ) ;
#94440=CARTESIAN_POINT ( 'NONE',  ( 26.92291421019269748, 1446.493256787829978, 137.3410761307699772 ) ) ;
#94442=CARTESIAN_POINT ( 'NONE',  ( -2.506807337198010188, 1509.132703289729989, 179.1218463405919863 ) ) ;
#94444=VERTEX_POINT ( 'NONE', #78785 ) ;
#94445=CARTESIAN_POINT ( 'NONE',  ( 1.550759356559749946, 1415.890045858090161, 190.5138187982429940 ) ) ;
#94446=CARTESIAN_POINT ( 'NONE',  ( 26.22432434920000333, 1488.572867069630092, 206.9931121771180074 ) ) ;
#94448=CARTESIAN_POINT ( 'NONE',  ( 5.066731847092691865, 1410.465363966433870, 186.3980185437680177 ) ) ;
#94451=CARTESIAN_POINT ( 'NONE',  ( 12.15678282470000049, 1407.401676941830146, 215.7644370117779999 ) ) ;
#94452=CARTESIAN_POINT ( 'NONE',  ( -18.49885826511389908, 1509.559054752839984, 185.8253364393310108 ) ) ;
#94454=CARTESIAN_POINT ( 'NONE',  ( -1.520740653450000091, 1487.755788924029957, 231.1622291657979815 ) ) ;
#94455=FACE_OUTER_BOUND ( 'NONE', #38602, .T. ) ;
#94458=EDGE_CURVE ( 'NONE', #11723, #79464, #37592, .T. ) ;
#94459=EDGE_CURVE ( 'NONE', #27091, #20305, #52298, .T. ) ;
#94460=CARTESIAN_POINT ( 'NONE',  ( 22.25038035520000079, 1451.993487009829778, 142.0274306324980103 ) ) ;
#94462=CARTESIAN_POINT ( 'NONE',  ( -23.52438668707183211, 1410.744642857871213, 210.4400693876917217 ) ) ;
#94463=EDGE_CURVE ( 'NONE', #77650, #66906, #65562, .T. ) ;
#94464=CARTESIAN_POINT ( 'NONE',  ( 23.97351809889999785, 1509.497062395329976, 194.1275154229979876 ) ) ;
#94465=ORIENTED_EDGE ( 'NONE', *, *, #41858, .T. ) ;
#94467=CARTESIAN_POINT ( 'NONE',  ( -18.29272317556928940, 1459.191059311327763, 227.8243320175402573 ) ) ;
#94469=ADVANCED_FACE ( 'NONE', ( #45758 ), #99353, .F. ) ;
#94470=CARTESIAN_POINT ( 'NONE',  ( -0.5929201156298425923, 1417.119756057481027, 234.4154478403977180 ) ) ;
#94473=CARTESIAN_POINT ( 'NONE',  ( 18.66884402514269681, 1509.506581848020005, 231.4335292741830017 ) ) ;
#94474=DIRECTION ( 'NONE',  ( -0.3081687959821756695, 0.7660444431188054848, -0.5640991972602826809 ) ) ;
#94475=CARTESIAN_POINT ( 'NONE',  ( 40.20118103687880051, 1442.631303985449904, 137.0031652087610041 ) ) ;
#94476=CARTESIAN_POINT ( 'NONE',  ( 5.510800338187703318, 1410.588349387585595, 269.3375996105341983 ) ) ;
#94477=CARTESIAN_POINT ( 'NONE',  ( -8.081131085970000546E-10, 1475.995192538530091, 267.2558860777979817 ) ) ;
#94480=CARTESIAN_POINT ( 'NONE',  ( -11.87299952773408762, 1435.287980174489348, 151.2457144668333910 ) ) ;
#94481=CARTESIAN_POINT ( 'NONE',  ( -20.02256639929999693, 1485.317074534930043, 191.1140876134980147 ) ) ;
#94483=CARTESIAN_POINT ( 'NONE',  ( 2.894471309390000080, 1409.014137552730062, 187.1861089909980080 ) ) ;
#94485=CARTESIAN_POINT ( 'NONE',  ( -12.15187876699999947, 1435.108173511759787, 151.0159321440980023 ) ) ;
#94489=CARTESIAN_POINT ( 'NONE',  ( 0.2811493428090000024, 1466.033507498329982, 235.8442874365980231 ) ) ;
#94490=VERTEX_POINT ( 'NONE', #4819 ) ;
#94493=CARTESIAN_POINT ( 'NONE',  ( -37.00343483889999874, 1455.724349294930107, 269.5585655813979997 ) ) ;
#94496=CARTESIAN_POINT ( 'NONE',  ( 17.41346973679999977, 1410.020394403929913, 224.1775087769979962 ) ) ;
#94498=CARTESIAN_POINT ( 'NONE',  ( -1.076288783000059918E-08, 1474.539729485439921, 264.4539261149100184 ) ) ;
#94500=CARTESIAN_POINT ( 'NONE',  ( -1.061258286910000015, 1415.553739807329976, 227.5328994501979878 ) ) ;
#94501=CARTESIAN_POINT ( 'NONE',  ( -6.733539913119999554, 1418.366792801529982, 233.9669031324980040 ) ) ;
#94506=CARTESIAN_POINT ( 'NONE',  ( -45.98858655093319925, 1439.424532750870185, 268.4973034418130169 ) ) ;
#94507=CARTESIAN_POINT ( 'NONE',  ( -2.694622903610000009, 1431.454301131900138, 185.0137053526979969 ) ) ;
#94512=CARTESIAN_POINT ( 'NONE',  ( -5.455807433810000440, 1438.116814840910138, 154.7280903985979990 ) ) ;
#94515=CARTESIAN_POINT ( 'NONE',  ( -26.88702675072890003, 1451.212428032629987, 136.2751528734569888 ) ) ;
#94516=ORIENTED_EDGE ( 'NONE', *, *, #50285, .T. ) ;
#94517=CARTESIAN_POINT ( 'NONE',  ( 10.80267214090000039, 1423.683922205029830, 212.9172522967979830 ) ) ;
#94520=( BOUNDED_CURVE ( )  B_SPLINE_CURVE ( 3, ( #66116, #107531, #74507, #90726 ),
 .UNSPECIFIED., .F., .T. ) 
 B_SPLINE_CURVE_WITH_KNOTS ( ( 4, 4 ),
 ( 4.409610424194855050, 5.070003779556289558 ),
 .UNSPECIFIED. ) 
 CURVE ( )  GEOMETRIC_REPRESENTATION_ITEM ( )  RATIONAL_B_SPLINE_CURVE ( ( 1.000000000000000000, 0.9639857288000422963, 0.9639857288000422963, 1.000000000000000000 ) ) 
 REPRESENTATION_ITEM ( '' )  );
#94521=CARTESIAN_POINT ( 'NONE',  ( 11.60004869885203682, 1425.691286098748606, 137.2109839355661904 ) ) ;
#94522=CARTESIAN_POINT ( 'NONE',  ( 13.43167025587599817, 1509.382104656720003, 235.1752264429409820 ) ) ;
#94526=CARTESIAN_POINT ( 'NONE',  ( -1.249564655339530095, 1407.936288853909900, 270.2925089982160216 ) ) ;
#94528=CARTESIAN_POINT ( 'NONE',  ( 10.72383926760000072, 1418.448279815129808, 229.9424527573980015 ) ) ;
#94529=CARTESIAN_POINT ( 'NONE',  ( -2.500000000000000000, 1448.894380913990062, 183.1110264324979937 ) ) ;
#94530=CARTESIAN_POINT ( 'NONE',  ( -2.500000000000000000, 1439.390253060799978, 161.6061717842659959 ) ) ;
#94533=CARTESIAN_POINT ( 'NONE',  ( -22.76136400371149904, 1409.717529452729877, 209.5657493702119893 ) ) ;
#94534=CARTESIAN_POINT ( 'NONE',  ( -4.249337494120000613, 1423.895439858529926, 184.8620138466980052 ) ) ;
#94535=CARTESIAN_POINT ( 'NONE',  ( -12.13574144734536375, 1436.932434855902784, 151.4274810089637526 ) ) ;
#94536=CARTESIAN_POINT ( 'NONE',  ( -4.579624579470000789, 1427.832655172230034, 112.4493539157979995 ) ) ;
#94538=AXIS2_PLACEMENT_3D ( 'NONE', #58162, #101222, #76054 ) ;
#94539=CARTESIAN_POINT ( 'NONE',  ( -20.57759663809800088, 1493.275265424210147, 192.6373786097109928 ) ) ;
#94540=CARTESIAN_POINT ( 'NONE',  ( -17.98568901069999981, 1415.860170671229980, 225.2002861224979995 ) ) ;
#94542=CARTESIAN_POINT ( 'NONE',  ( 39.10679733682070491, 1459.373169423960007, 268.7147505820800006 ) ) ;
#94543=CARTESIAN_POINT ( 'NONE',  ( -2.201151872242963492, 1466.932782758140092, 235.2250472885538670 ) ) ;
#94544=CARTESIAN_POINT ( 'NONE',  ( -16.94111210471653450, 1421.944315043240977, 226.8380784755184152 ) ) ;
#94547=CARTESIAN_POINT ( 'NONE',  ( 18.89223017036711738, 1457.760250004050249, 226.9657477437493185 ) ) ;
#94548=CARTESIAN_POINT ( 'NONE',  ( 1.523969922190620219, 1455.113528485800089, 183.3838728237819851 ) ) ;
#94549=CARTESIAN_POINT ( 'NONE',  ( 22.65292971370000075, 1409.704085498430004, 208.9051947466459751 ) ) ;
#94550=VERTEX_POINT ( 'NONE', #97230 ) ;
#94551=DIRECTION ( 'NONE',  ( 0.000000000000000000, 0.000000000000000000, 1.000000000000000000 ) ) ;
#94552=CARTESIAN_POINT ( 'NONE',  ( 24.77492596718960272, 1452.047903808549790, 135.6621443109009988 ) ) ;
#94556=CARTESIAN_POINT ( 'NONE',  ( 17.69145655820000229, 1410.027806010230051, 193.3443910425980050 ) ) ;
#94557=CARTESIAN_POINT ( 'NONE',  ( 20.75326766870000128, 1444.324653571829913, 176.0807405191980024 ) ) ;
#94558=CARTESIAN_POINT ( 'NONE',  ( 3.400285785609643785, 1439.690925502392702, 184.4405085457196662 ) ) ;
#94560=CARTESIAN_POINT ( 'NONE',  ( -22.76204189940434830, 1432.230029621326366, 215.7233072855924831 ) ) ;
#94561=CARTESIAN_POINT ( 'NONE',  ( 1.131322572361280088, 1452.208024494899746, 183.3657943293449932 ) ) ;
#94563=CARTESIAN_POINT ( 'NONE',  ( -0.01940215194334939802, 1508.902653225929953, 179.5976350532890251 ) ) ;
#94565=CARTESIAN_POINT ( 'NONE',  ( 1.363639811660000145, 1415.765555525229956, 232.8698637559979829 ) ) ;
#94567=CARTESIAN_POINT ( 'NONE',  ( 17.22592475670000312, 1443.913060387330006, 162.9227486557980171 ) ) ;
#94569=CARTESIAN_POINT ( 'NONE',  ( 11.40293847519150106, 1414.971993471370070, 221.9446473240219859 ) ) ;
#94571=CARTESIAN_POINT ( 'NONE',  ( -0.3563141984344909696, 1409.037191904199972, 232.3070811437949885 ) ) ;
#94574=CARTESIAN_POINT ( 'NONE',  ( 0.2545641544693758029, 1506.446781329472969, 231.1141566264156779 ) ) ;
#94575=CARTESIAN_POINT ( 'NONE',  ( -19.62446893450000118, 1443.054186837209954, 214.3676144197979738 ) ) ;
#94576=ADVANCED_FACE ( 'NONE', ( #12123 ), #12723, .F. ) ;
#94577=CARTESIAN_POINT ( 'NONE',  ( -21.41430812654454385, 1509.039033548261386, 191.8384994702369966 ) ) ;
#94578=CARTESIAN_POINT ( 'NONE',  ( 11.62685186760000100, 1433.421535312869764, 151.0711183502979793 ) ) ;
#94579=CARTESIAN_POINT ( 'NONE',  ( 21.37693748330000076, 1443.303628179369980, 224.8635562210979799 ) ) ;
#94580=CARTESIAN_POINT ( 'NONE',  ( 12.71641934408430075, 1415.429375168349907, 196.8674432429739909 ) ) ;
#94582=CARTESIAN_POINT ( 'NONE',  ( 22.91663120903140083, 1507.606285602550088, 210.6365840681099826 ) ) ;
#94583=CARTESIAN_POINT ( 'NONE',  ( 24.86520269990570142, 1436.144666160072575, 137.8610266872903196 ) ) ;
#94584=CARTESIAN_POINT ( 'NONE',  ( 22.58840255639999839, 1409.701846760530088, 208.8102578915460015 ) ) ;
#94585=CARTESIAN_POINT ( 'NONE',  ( 10.57127173870284054, 1398.226368140626164, 201.5218381721108756 ) ) ;
#94586=CARTESIAN_POINT ( 'NONE',  ( -21.61785201490240027, 1509.681104934679979, 231.5207931856990058 ) ) ;
#94589=B_SPLINE_CURVE_WITH_KNOTS ( 'NONE', 3,
 ( #36094, #70280, #45619, #62991, #18706, #70834, #28235, #96548, #79759, #104389, #37740, #27686, #62422, #87604, #61870, #105501, #46170, #95988, #88156, #71389, #53459, #10892, #45065 ),
 .UNSPECIFIED., .F., .F.,
 ( 4, 2, 2, 1, 2, 2, 2, 2, 2, 2, 2, 4 ),
 ( 0.000000000000000000, 0.1249999999998680222, 0.1874999999999092115, 0.2187499999998207545, 0.2343749999997765676, 0.2499999999997324085, 0.3749999999997780109, 0.4999999999998235856, 0.6249999999998692157, 0.6874999999998908651, 0.7499999999999124034, 1.000000000000000000 ),
 .UNSPECIFIED. ) ;
#94591=CARTESIAN_POINT ( 'NONE',  ( -8.664500300950001233, 1509.043687291729839, 236.1803262411980029 ) ) ;
#94597=CARTESIAN_POINT ( 'NONE',  ( 0.1603187917380029803, 1486.074899099739923, 181.8333893279200026 ) ) ;
#94600=VERTEX_POINT ( 'NONE', #51912 ) ;
#94601=CARTESIAN_POINT ( 'NONE',  ( -0.9044596104409999837, 1416.819760301830001, 228.0287517993979804 ) ) ;
#94602=AXIS2_PLACEMENT_3D ( 'NONE', #23011, #99164, #82933 ) ;
#94605=CARTESIAN_POINT ( 'NONE',  ( 13.50077136620000040, 1434.968960439809962, 149.6996353846979844 ) ) ;
#94610=DIRECTION ( 'NONE',  ( 0.000000000000000000, 2.960594732333748082E-13, -1.000000000000000000 ) ) ;
#94617=B_SPLINE_CURVE_WITH_KNOTS ( 'NONE', 3,
 ( #63211, #14398, #48592, #48028, #38509, #89472, #82726, #72688, #81065, #73228, #5465, #31216, #20588, #73794, #82166, #63745, #88919, #30102, #12205, #65398, #39048, #6016, #64852, #30667, #39626, #107921, #90013, #81605, #98962, #97318, #12768, #54787, #90564, #3847, #64297, #13290, #46400, #80532, #37974, #72156, #106274, #23358, #101155, #16046, #49142, #109586, #108479, #8201, #23896, #31762, #102269, #25548, #93317, #83821, #100612, #59740, #7121, #49692, #41820, #84909, #110673, #42368, #50776, #109043, #57549, #41276, #91672, #33966, #84377, #32856, #74352, #24449, #67048, #75451, #40170, #50247, #58091, #24996 ),
 .UNSPECIFIED., .F., .F.,
 ( 4, 2, 2, 1, 1, 1, 1, 2, 2, 2, 1, 1, 1, 1, 1, 2, 2, 2, 2, 1, 1, 1, 2, 2, 2, 1, 1, 1, 1, 1, 2, 2, 2, 2, 2, 1, 1, 1, 1, 2, 2, 2, 2, 1, 1, 1, 2, 2, 2, 2, 4 ),
 ( 0.000000000000000000, 0.06249999999905236914, 0.09374999999857999700, 0.1093749999983438387, 0.1171874999982358140, 0.1210937499981719484, 0.1230468749981302318, 0.1240234374981080828, 0.1249999999980859339, 0.1874999999981248888, 0.2187499999981443732, 0.2343749999981540599, 0.2421874999981687426, 0.2460937499981760701, 0.2480468749981797338, 0.2490234374981733778, 0.2499999999981670773, 0.3749999999993307576, 0.4374999999999126810, 0.4687500000002036704, 0.4843750000003492207, 0.4921875000004325429, 0.4960937500004755085, 0.5000000000005184742, 0.6250000000021559421, 0.6875000000029746205, 0.7187500000033728575, 0.7343750000035703662, 0.7421875000036677328, 0.7460937500037260195, 0.7480468750037470027, 0.7500000000037678749, 0.8125000000041449066, 0.8437500000043415271, 0.8593750000044494408, 0.8671875000045020654, 0.8710937500045184967, 0.8730468750045379256, 0.8740234375045391468, 0.8745117187545383697, 0.8750000000045374815, 0.8906250000045405901, 0.8984375000045421444, 0.9023437500045430326, 0.9042968750045285997, 0.9052734375045072834, 0.9057617187544817483, 0.9062500000044562132, 0.9218750000037139181, 0.9375000000029716229, 1.000000000000000000 ),
 .UNSPECIFIED. ) ;
#94621=B_SPLINE_SURFACE_WITH_KNOTS ( 'NONE', 5, 5, ( 
 ( #44149, #34626, #68810, #41931, #102912, #26211 ),
 ( #67700, #93420, #17794, #76087, #42471, #1053 ),
 ( #35178, #18909, #76629, #27328, #78284, #1597 ),
 ( #59847, #51994, #9428, #93971, #43592, #35734 ),
 ( #77740, #69922, #61513, #89857, #70474, #99340 ),
 ( #45264, #107211, #87814, #44707, #47311, #13127 ) ),
 .UNSPECIFIED., .F., .F., .F.,
 ( 6, 6 ),
 ( 6, 6 ),
 ( 30.40177460640000007, 157.7844419379999863 ),
 ( -6.938893903909999252E-17, 1.000000000000000000 ),
 .UNSPECIFIED. ) ;
#94623=CARTESIAN_POINT ( 'NONE',  ( -17.53497677579999703, 1411.915013305630055, 192.5944228452979985 ) ) ;
#94627=CARTESIAN_POINT ( 'NONE',  ( 12.93811130839999812, 1442.831169986189934, 169.4238961894979809 ) ) ;
#94628=DIRECTION ( 'NONE',  ( -0.05876148091703057436, 0.002052003564324334384, 0.9982699422710319404 ) ) ;
#94632=EDGE_LOOP ( 'NONE', ( #106547, #100909, #3973, #89853 ) ) ;
#94636=CARTESIAN_POINT ( 'NONE',  ( 1.114882633370010031E-09, 1467.056812769279986, 237.6398032221420067 ) ) ;
#94638=CARTESIAN_POINT ( 'NONE',  ( 19.02416918379194044, 1437.840865032662805, 213.1984861927293480 ) ) ;
#94641=CARTESIAN_POINT ( 'NONE',  ( -4.155669664704369382, 1439.704322410719897, 185.4969487652249995 ) ) ;
#94644=EDGE_CURVE ( 'NONE', #76907, #51033, #25161, .T. ) ;
#94647=AXIS2_PLACEMENT_3D ( 'NONE', #77629, #59193, #26656 ) ;
#94648=CARTESIAN_POINT ( 'NONE',  ( 2.500000005440000006, 1448.104721459739949, 157.8850530793979772 ) ) ;
#94649=EDGE_CURVE ( 'NONE', #22078, #12048, #76518, .T. ) ;
#94651=LINE ( 'NONE', #70048, #28312 ) ;
#94658=CARTESIAN_POINT ( 'NONE',  ( -23.88743783630000195, 1410.917949452529911, 207.8246455712279896 ) ) ;
#94659=CARTESIAN_POINT ( 'NONE',  ( -10.35833152844089966, 1425.137813717620020, 115.9780672966650030 ) ) ;
#94660=CARTESIAN_POINT ( 'NONE',  ( 16.21964127711080295, 1409.479387927570087, 193.0992798958739911 ) ) ;
#94662=CARTESIAN_POINT ( 'NONE',  ( 28.80933051664284861, 1510.030156971867427, 200.7517252896445257 ) ) ;
#94665=CARTESIAN_POINT ( 'NONE',  ( -30.10636673460000168, 1413.645518868930139, 266.8104471709979748 ) ) ;
#94667=CARTESIAN_POINT ( 'NONE',  ( 17.47747713618334942, 1459.994120045239242, 228.4137988842376217 ) ) ;
#94670=CARTESIAN_POINT ( 'NONE',  ( -35.83369766294850223, 1437.372084409380022, 136.5363233108159875 ) ) ;
#94672=CARTESIAN_POINT ( 'NONE',  ( 6.700735663969999756, 1396.147055234629988, 199.0043882911979836 ) ) ;
#94674=CARTESIAN_POINT ( 'NONE',  ( -17.12355492049999839, 1460.407125116229736, 228.2713570448979965 ) ) ;
#94675=VERTEX_POINT ( 'NONE', #9893 ) ;
#94676=VERTEX_POINT ( 'NONE', #54689 ) ;
#94677=CARTESIAN_POINT ( 'NONE',  ( -2.431412526649999961, 1428.647745098929818, 149.4227846719979880 ) ) ;
#94678=CARTESIAN_POINT ( 'NONE',  ( -11.76196305498579875, 1425.587148902949821, 146.3422030814200241 ) ) ;
#94682=CARTESIAN_POINT ( 'NONE',  ( -11.87239127897699831, 1432.808531436009844, 149.9811485733590075 ) ) ;
#94683=CIRCLE ( 'NONE', #101778, 10.00000000000000000 ) ;
#94687=FACE_OUTER_BOUND ( 'NONE', #84393, .T. ) ;
#94693=CARTESIAN_POINT ( 'NONE',  ( 11.80334487768269902, 1428.396969778590119, 148.3489976931730041 ) ) ;
#94697=CARTESIAN_POINT ( 'NONE',  ( -13.31869796660000027, 1443.086052842849995, 169.3753098992980028 ) ) ;
#94698=CARTESIAN_POINT ( 'NONE',  ( 11.34707687579999913, 1509.309309043230087, 235.7409118476979870 ) ) ;
#94700=CARTESIAN_POINT ( 'NONE',  ( -6.205088089679999364, 1421.916341492230003, 186.7344349734979971 ) ) ;
#94702=CARTESIAN_POINT ( 'NONE',  ( 4.235651746019999386, 1408.707576597030084, 270.4270856384979993 ) ) ;
#94706=CARTESIAN_POINT ( 'NONE',  ( 24.33627900605520011, 1451.288492182929986, 206.2143456058219897 ) ) ;
#94709=CARTESIAN_POINT ( 'NONE',  ( -4.636078765298575100, 1423.706159026812657, 184.4443473542607990 ) ) ;
#94712=CARTESIAN_POINT ( 'NONE',  ( -2.152516339165368109, 1506.379860764218165, 187.2722548778648104 ) ) ;
#94717=CARTESIAN_POINT ( 'NONE',  ( -2.913081468028484000, 1484.790404518151718, 183.2223388818480316 ) ) ;
#94718=CARTESIAN_POINT ( 'NONE',  ( -17.60616670766113856, 1410.892144164382898, 193.1022257080302893 ) ) ;
#94721=CARTESIAN_POINT ( 'NONE',  ( 0.5928098971900001013, 1489.480617679929765, 187.2733462026980078 ) ) ;
#94724=CARTESIAN_POINT ( 'NONE',  ( -11.82919182880000086, 1429.685437959029969, 149.7801030883980218 ) ) ;
#94725=CARTESIAN_POINT ( 'NONE',  ( -10.83059686145892186, 1424.984354290685587, 145.3974420532384499 ) ) ;
#94733=CARTESIAN_POINT ( 'NONE',  ( -15.80613827389999670, 1459.265199882230036, 230.3675922840980093 ) ) ;
#94734=AXIS2_PLACEMENT_3D ( 'NONE', #66437, #64792, #100553 ) ;
#94736=CARTESIAN_POINT ( 'NONE',  ( 18.38362700379999737, 1408.577091670229947, 267.3950545271980559 ) ) ;
#94737=CARTESIAN_POINT ( 'NONE',  ( 2.219943740554563227, 1464.863888248525654, 237.3912208037882294 ) ) ;
#94738=CARTESIAN_POINT ( 'NONE',  ( 20.68393032789999708, 1449.727573619960140, 194.8750444304980078 ) ) ;
#94739=CARTESIAN_POINT ( 'NONE',  ( -23.01365769190000066, 1432.948698623059954, 214.9133548742180153 ) ) ;
#94740=CARTESIAN_POINT ( 'NONE',  ( -0.09392903680032700653, 1507.117918406099989, 237.3493018655460105 ) ) ;
#94742=CARTESIAN_POINT ( 'NONE',  ( 20.59269117493390056, 1507.766073655780019, 227.7908423917359926 ) ) ;
#94743=CARTESIAN_POINT ( 'NONE',  ( -6.294750357631860638, 1408.079328830519898, 197.5408074016749822 ) ) ;
#94744=CARTESIAN_POINT ( 'NONE',  ( -18.88659680459999990, 1416.522662136229883, 207.5785872533780037 ) ) ;
#94745=CIRCLE ( 'NONE', #16070, 1.000002395586160775 ) ;
#94746=CARTESIAN_POINT ( 'NONE',  ( -12.54789821530000005, 1442.763165783939940, 186.3817407933979950 ) ) ;
#94750=CARTESIAN_POINT ( 'NONE',  ( 26.02835829290000191, 1413.547636220630011, 269.9886483863980402 ) ) ;
#94751=VERTEX_POINT ( 'NONE', #107264 ) ;
#94754=CARTESIAN_POINT ( 'NONE',  ( -10.61798429165910029, 1409.283848569250040, 198.5915965930109905 ) ) ;
#94759=CARTESIAN_POINT ( 'NONE',  ( -7.085472565520000821, 1475.647693041629964, 268.4624854401979519 ) ) ;
#94761=CARTESIAN_POINT ( 'NONE',  ( 0.3192358074811350033, 1419.260587148479772, 184.5597205914540098 ) ) ;
#94762=CARTESIAN_POINT ( 'NONE',  ( 18.02577102991580205, 1424.483463156160042, 224.6203623841139745 ) ) ;
#94765=CARTESIAN_POINT ( 'NONE',  ( 11.74953517310929918, 1415.393085341090000, 223.0700735755810058 ) ) ;
#94770=CARTESIAN_POINT ( 'NONE',  ( -22.93992789289999834, 1409.878607768230040, 206.3744506774879994 ) ) ;
#94771=CARTESIAN_POINT ( 'NONE',  ( 17.76192431929999671, 1416.216739748630062, 206.2762435944279957 ) ) ;
#94776=CARTESIAN_POINT ( 'NONE',  ( 1.650293394300000216, 1438.194204504490017, 150.5634062101979964 ) ) ;
#94780=CARTESIAN_POINT ( 'NONE',  ( -23.10442739089999975, 1411.095127590530183, 210.9251608893080174 ) ) ;
#94782=CARTESIAN_POINT ( 'NONE',  ( 11.71397520463430020, 1426.710800257239953, 142.5191138725960229 ) ) ;
#94788=CARTESIAN_POINT ( 'NONE',  ( -16.49511036701739997, 1507.275788732180217, 224.7012778065829934 ) ) ;
#94790=CARTESIAN_POINT ( 'NONE',  ( -4.672678730482617837, 1398.052343473715382, 221.2534302702293019 ) ) ;
#94791=DIRECTION ( 'NONE',  ( 0.4794255386042040601, 0.000000000000000000, 0.8775825618903722036 ) ) ;
#94793=CARTESIAN_POINT ( 'NONE',  ( -19.21352096260000053, 1449.658915334390258, 194.0202163047979980 ) ) ;
#94800=ORIENTED_EDGE ( 'NONE', *, *, #14548, .T. ) ;
#94801=CARTESIAN_POINT ( 'NONE',  ( 11.25336247954099989, 1434.059297280159853, 151.5716172890120106 ) ) ;
#94802=CARTESIAN_POINT ( 'NONE',  ( 28.65660564130000054, 1509.914370929529923, 215.8254011786380033 ) ) ;
#94809=CARTESIAN_POINT ( 'NONE',  ( 4.677877709162899578, 1498.105331289570131, 235.3354212934999907 ) ) ;
#94810=CARTESIAN_POINT ( 'NONE',  ( -0.1852737114690000131, 1488.178506539929913, 181.6492668772979755 ) ) ;
#94812=CARTESIAN_POINT ( 'NONE',  ( 16.05825058989999832, 1409.640465031130134, 226.2302501376979933 ) ) ;
#94814=CARTESIAN_POINT ( 'NONE',  ( 14.13596061226570022, 1415.658863692649902, 197.1814981948540151 ) ) ;
#94818=CARTESIAN_POINT ( 'NONE',  ( 14.36046478289659944, 1436.108318026239886, 149.9810154171919976 ) ) ;
#94830=CARTESIAN_POINT ( 'NONE',  ( 13.55937018769710001, 1409.552481286539887, 191.5919570012989936 ) ) ;
#94832=CARTESIAN_POINT ( 'NONE',  ( 0.001298364960140000043, 1507.624704233530110, 237.4156383742980267 ) ) ;
#94833=ORIENTED_EDGE ( 'NONE', *, *, #83607, .T. ) ;
#94838=CARTESIAN_POINT ( 'NONE',  ( -18.67054469629999858, 1509.506033879029928, 231.0930226666980047 ) ) ;
#94839=EDGE_LOOP ( 'NONE', ( #641, #45731, #107605 ) ) ;
#94840=CARTESIAN_POINT ( 'NONE',  ( 25.89699081781530055, 1448.079192754820042, 137.6508162902210017 ) ) ;
#94841=CARTESIAN_POINT ( 'NONE',  ( -7.284723200410000210, 1410.103078541930017, 187.5144291113979875 ) ) ;
#94842=CARTESIAN_POINT ( 'NONE',  ( -24.35760538859999969, 1442.387172495660025, 212.1777658713180017 ) ) ;
#94850=CARTESIAN_POINT ( 'NONE',  ( -1.753571105566960053, 1484.238156075060033, 182.7741811579140006 ) ) ;
#94853=CARTESIAN_POINT ( 'NONE',  ( 24.05887429810000100, 1410.845155071830277, 209.6244263713389842 ) ) ;
#94854=CARTESIAN_POINT ( 'NONE',  ( 24.05887576171189579, 1410.845155067154792, 209.6244200405261324 ) ) ;
#94855=CARTESIAN_POINT ( 'NONE',  ( 28.28208337139999884, 1508.151294399930066, 209.1094497554269935 ) ) ;
#94858=( BOUNDED_SURFACE ( )  B_SPLINE_SURFACE ( 4, 2, ( 
 ( #32511, #85097, #51514, #101888, #75077, #109762, #41468, #7302, #33042, #92391, #16224 ),
 ( #6738, #100786, #101327, #67231, #24079, #57732, #84002, #17319, #15664, #24617, #58812 ),
 ( #25180, #92952, #42011, #16766, #50429, #102447, #49317, #83443, #40896, #42557, #108657 ),
 ( #91851, #84554, #6193, #7843, #50969, #76160, #100260, #74526, #31944, #23540, #66139 ),
 ( #87892, #45345, #18428, #10620, #61049, #11183, #19551, #53182, #96274, #69443, #79484 ) ),
 .UNSPECIFIED., .F., .T., .F. ) 
 B_SPLINE_SURFACE_WITH_KNOTS ( ( 5, 5 ),
 ( 3, 2, 2, 2, 2, 3 ),
 ( 3.613988937050000239, 5.260361675040000407 ),
 ( 5.178099995975929737, 6.283185307179590673, 7.853981633974480125, 9.424777960769379348, 10.99557428756429900, 11.46128530315550087 ),
 .UNSPECIFIED. ) 
 GEOMETRIC_REPRESENTATION_ITEM ( )  RATIONAL_B_SPLINE_SURFACE ( (
 ( 0.8778166930676719604, 0.7939440089458740246, 1.000000000000000000, 0.7071067811865480168, 1.000000000000000000, 0.7071067811865480168, 1.000000000000000000, 0.7071067811865480168, 1.000000000000000000, 0.9131627722406739922, 0.8778166930676719604),
 ( 0.8778166930676719604, 0.7939440089458740246, 1.000000000000000000, 0.7071067811865480168, 1.000000000000000000, 0.7071067811865480168, 1.000000000000000000, 0.7071067811865480168, 1.000000000000000000, 0.9131627722406739922, 0.8778166930676719604),
 ( 0.8778166930676719604, 0.7939440089458740246, 1.000000000000000000, 0.7071067811865480168, 1.000000000000000000, 0.7071067811865480168, 1.000000000000000000, 0.7071067811865480168, 1.000000000000000000, 0.9131627722406739922, 0.8778166930676719604),
 ( 0.8778166930676719604, 0.7939440089458740246, 1.000000000000000000, 0.7071067811865480168, 1.000000000000000000, 0.7071067811865480168, 1.000000000000000000, 0.7071067811865480168, 1.000000000000000000, 0.9131627722406739922, 0.8778166930676719604),
 ( 0.8778166930676719604, 0.7939440089458740246, 1.000000000000000000, 0.7071067811865480168, 1.000000000000000000, 0.7071067811865480168, 1.000000000000000000, 0.7071067811865480168, 1.000000000000000000, 0.9131627722406739922, 0.8778166930676719604) ) ) 
 REPRESENTATION_ITEM ( '' )  SURFACE ( )  );
#94863=CARTESIAN_POINT ( 'NONE',  ( 24.26836866860000086, 1463.758695672930116, 255.0044592737980054 ) ) ;
#94864=CARTESIAN_POINT ( 'NONE',  ( 3.479472432754871392, 1450.884102103086661, 184.0533424794217581 ) ) ;
#94866=CARTESIAN_POINT ( 'NONE',  ( -8.309204053089999320, 1507.619019172929939, 235.1728781061979987 ) ) ;
#94867=CARTESIAN_POINT ( 'NONE',  ( -20.73227332440000126, 1454.210575483330103, 225.1076712988979978 ) ) ;
#94869=CARTESIAN_POINT ( 'NONE',  ( -19.43886440797159665, 1410.953638617170554, 197.3090217047405304 ) ) ;
#94870=CARTESIAN_POINT ( 'NONE',  ( 17.84735382287039585, 1410.225448354170112, 222.8565957718949733 ) ) ;
#94873=VERTEX_POINT ( 'NONE', #25991 ) ;
#94875=CARTESIAN_POINT ( 'NONE',  ( 0.3398959847620000030, 1405.717602100329941, 267.8539949327980025 ) ) ;
#94876=AXIS2_PLACEMENT_3D ( 'NONE', #28859, #13668, #14238 ) ;
#94878=CARTESIAN_POINT ( 'NONE',  ( -18.87576674860000026, 1410.495261148229929, 223.1730055151980139 ) ) ;
#94883=CARTESIAN_POINT ( 'NONE',  ( -37.65027717969969245, 1440.913060388920030, 255.7160772220900071 ) ) ;
#94884=CARTESIAN_POINT ( 'NONE',  ( -27.00037440250000031, 1448.139615625060060, 136.8881630574980193 ) ) ;
#94885=CARTESIAN_POINT ( 'NONE',  ( 3.127068336719009611E-15, 1468.922471155709900, 264.4545146619439606 ) ) ;
#94887=EDGE_CURVE ( 'NONE', #92743, #105306, #20122, .T. ) ;
#94892=ORIENTED_EDGE ( 'NONE', *, *, #72894, .T. ) ;
#94893=CARTESIAN_POINT ( 'NONE',  ( -3.996802888650000299E-15, 1409.413060387330006, 271.1218459616979999 ) ) ;
#94894=CARTESIAN_POINT ( 'NONE',  ( 11.94168174870000065, 1433.614859990550030, 146.5967844433980076 ) ) ;
#94896=CARTESIAN_POINT ( 'NONE',  ( 16.54279911444290008, 1495.117735635360077, 188.4866523640159812 ) ) ;
#94898=CARTESIAN_POINT ( 'NONE',  ( -0.6608933561119999522, 1417.306151990130047, 234.7827825253980052 ) ) ;
#94904=CARTESIAN_POINT ( 'NONE',  ( -11.86722885316952691, 1418.961735472639475, 228.9247715664120051 ) ) ;
#94905=CARTESIAN_POINT ( 'NONE',  ( -18.82708389389999581, 1416.254459046630018, 208.1920681675479727 ) ) ;
#94908=CARTESIAN_POINT ( 'NONE',  ( 25.53921057650000037, 1435.901306799000167, 136.7951300741979992 ) ) ;
#94909=CARTESIAN_POINT ( 'NONE',  ( -7.684237820892370507, 1396.181399885199880, 201.1787653736790276 ) ) ;
#94910=ORIENTED_EDGE ( 'NONE', *, *, #37285, .F. ) ;
#94912=CARTESIAN_POINT ( 'NONE',  ( -16.95064093090770285, 1409.878458079239863, 225.6674120715180152 ) ) ;
#94913=CARTESIAN_POINT ( 'NONE',  ( 2.451271202390000070, 1433.447543843880112, 150.3250444719979839 ) ) ;
#94914=ORIENTED_EDGE ( 'NONE', *, *, #44571, .T. ) ;
#94915=EDGE_LOOP ( 'NONE', ( #55878, #12980, #63625, #93302 ) ) ;
#94921=CARTESIAN_POINT ( 'NONE',  ( 4.172408078941279186, 1424.841910750820034, 185.1366873668810058 ) ) ;
#94932=DIRECTION ( 'NONE',  ( 0.000000000000000000, 1.000000000000000000, 0.000000000000000000 ) ) ;
#94934=CARTESIAN_POINT ( 'NONE',  ( -3.048592212130000423, 1471.356831017029890, 269.3358345869979757 ) ) ;
#94935=CARTESIAN_POINT ( 'NONE',  ( 12.41107674216090828, 1434.349308524667094, 147.3453250864402264 ) ) ;
#94936=CARTESIAN_POINT ( 'NONE',  ( -0.03226023477341029982, 1410.297896964309984, 185.0217421575940193 ) ) ;
#94941=B_SPLINE_SURFACE_WITH_KNOTS ( 'NONE', 5, 4, ( 
 ( #63561, #20949, #88187, #79794, #3100 ),
 ( #89275, #71425, #12572, #105541, #72491 ),
 ( #64099, #29907, #98220, #13095, #47279 ),
 ( #28828, #65195, #48951, #108280, #15304 ),
 ( #31567, #49496, #75790, #41635, #101509 ),
 ( #90923, #100429, #41074, #40521, #76337 ) ),
 .UNSPECIFIED., .F., .F., .F.,
 ( 6, 6 ),
 ( 5, 5 ),
 ( 0.000000000000000000, 11.48858425020000062 ),
 ( 40.20365518519999881, 50.26548245740000453 ),
 .UNSPECIFIED. ) ;
#94943=CARTESIAN_POINT ( 'NONE',  ( -2.500000000000000000, 1448.308233332059899, 164.1021382917789992 ) ) ;
#94945=CARTESIAN_POINT ( 'NONE',  ( 6.311810463515059588, 1408.080013037259960, 196.8766857931779839 ) ) ;
#94946=CARTESIAN_POINT ( 'NONE',  ( -12.14058727293699924, 1406.960395450699934, 267.4746583413689791 ) ) ;
#94947=CARTESIAN_POINT ( 'NONE',  ( 18.02574679518840028, 1424.482682570480165, 224.6196048480980210 ) ) ;
#94948=VERTEX_POINT ( 'NONE', #84264 ) ;
#94949=CARTESIAN_POINT ( 'NONE',  ( -10.96867220919999930, 1432.296152601269796, 151.7700998140979891 ) ) ;
#94950=CARTESIAN_POINT ( 'NONE',  ( 13.87374158799999968, 1442.959733380379930, 189.3447062249979922 ) ) ;
#94951=ORIENTED_EDGE ( 'NONE', *, *, #39126, .F. ) ;
#94957=CIRCLE ( 'NONE', #46708, 2.000057822092189408 ) ;
#94964=CARTESIAN_POINT ( 'NONE',  ( -27.24055943209999953, 1509.630994782629841, 201.8111112392580253 ) ) ;
#94971=CARTESIAN_POINT ( 'NONE',  ( -7.548561889089999255, 1445.758549893310146, 184.1610481276980238 ) ) ;
#94972=EDGE_LOOP ( 'NONE', ( #10585, #46761, #15825, #104121 ) ) ;
#94974=CARTESIAN_POINT ( 'NONE',  ( 27.95183976710000096, 1508.132394785230190, 211.1111938569680149 ) ) ;
#94976=CARTESIAN_POINT ( 'NONE',  ( -25.57615594259999980, 1435.901898142059963, 136.7757793872980017 ) ) ;
#94980=CARTESIAN_POINT ( 'NONE',  ( -15.05055458040000005, 1410.738883427430210, 226.7232811513979982 ) ) ;
#94982=CARTESIAN_POINT ( 'NONE',  ( 17.56829117542830332, 1410.890577958010226, 192.7553912862538255 ) ) ;
#94985=CARTESIAN_POINT ( 'NONE',  ( -43.51386627571789489, 1440.913030677579854, 268.2728861700509810 ) ) ;
#94986=CARTESIAN_POINT ( 'NONE',  ( -0.6856103501910000286, 1410.310356903130014, 233.1312677497980133 ) ) ;
#94988=B_SPLINE_CURVE_WITH_KNOTS ( 'NONE', 3,
 ( #66328, #15320, #83098, #14781, #48967, #32142, #100446, #59016, #84190, #84737, #24812, #99876, #6392, #31582, #92586, #23729, #23175, #100982, #93676, #74715, #59562, #16956, #25370, #57915, #93143, #75268, #109417, #32693, #42204, #76354, #83638, #65760, #66873, #57375, #33783, #41650, #109958 ),
 .UNSPECIFIED., .F., .F.,
 ( 4, 3, 3, 3, 3, 3, 3, 3, 3, 3, 3, 3, 4 ),
 ( -1.999999927956309875, -1.972989624484049909, -1.798098438852570036, -1.621156865559949978, -1.442904648552300051, -1.257206222084299885, -1.076442897241259855, -0.8953608614236658880, -0.7144086979874439969, -0.5307528079918921726, -0.3521692608878350672, -0.1751745349638540450, -6.152018885430265982E-07 ),
 .UNSPECIFIED. ) ;
#94989=VERTEX_POINT ( 'NONE', #59090 ) ;
#94993=CARTESIAN_POINT ( 'NONE',  ( 12.43286703105460056, 1435.614820761110195, 150.9635431477080090 ) ) ;
#94994=CARTESIAN_POINT ( 'NONE',  ( 18.58484988559350271, 1469.012271477369950, 228.1231286946100170 ) ) ;
#94995=AXIS2_PLACEMENT_3D ( 'NONE', #38945, #5361, #22128 ) ;
#94996=FACE_OUTER_BOUND ( 'NONE', #92694, .T. ) ;
#94997=CARTESIAN_POINT ( 'NONE',  ( -2.325358437519999821, 1408.994263693330140, 187.9843026324979860 ) ) ;
#94998=CARTESIAN_POINT ( 'NONE',  ( -0.3096201624669999708, 1409.092176881229989, 232.6500405377979916 ) ) ;
#94999=CARTESIAN_POINT ( 'NONE',  ( 4.227028548029660548, 1441.559244791980063, 165.7750707031279944 ) ) ;
#95001=CARTESIAN_POINT ( 'NONE',  ( -4.304697625840000264, 1420.046328294529985, 186.4088000267980192 ) ) ;
#95002=CARTESIAN_POINT ( 'NONE',  ( 20.81915283020000018, 1509.403205473429807, 188.8735477223980013 ) ) ;
#95005=CARTESIAN_POINT ( 'NONE',  ( -12.80019129569859970, 1416.529254608160045, 196.2487864292310178 ) ) ;
#95006=CARTESIAN_POINT ( 'NONE',  ( -11.79695136760000018, 1504.313428625830056, 182.6247401251980023 ) ) ;
#95007=ORIENTED_EDGE ( 'NONE', *, *, #3739, .T. ) ;
#95009=CARTESIAN_POINT ( 'NONE',  ( 2.793917634100000047, 1420.174898411929917, 185.2234237461979944 ) ) ;
#95010=CARTESIAN_POINT ( 'NONE',  ( 18.64588652299999794, 1416.828040475229955, 209.6843149956849857 ) ) ;
#95015=CARTESIAN_POINT ( 'NONE',  ( 18.71036172829999700, 1415.996778984329922, 210.0886326743409995 ) ) ;
#95018=CARTESIAN_POINT ( 'NONE',  ( 17.45848092850000199, 1413.521836630329972, 192.3744159994980123 ) ) ;
#95020=CARTESIAN_POINT ( 'NONE',  ( 0.5730919830699721107, 1440.103938664269890, 189.4488964803610145 ) ) ;
#95022=ORIENTED_EDGE ( 'NONE', *, *, #83173, .F. ) ;
#95023=CARTESIAN_POINT ( 'NONE',  ( 1.552414559603289890, 1415.673583080789967, 190.6708713369849875 ) ) ;
#95024=CARTESIAN_POINT ( 'NONE',  ( 26.37684233794689348, 1508.582724258994403, 216.7137066027032404 ) ) ;
#95026=CARTESIAN_POINT ( 'NONE',  ( 7.548436927367426996, 1410.549687724076421, 187.4153570461994605 ) ) ;
#95027=CARTESIAN_POINT ( 'NONE',  ( 0.3621993315900440269, 1416.825784014750070, 227.1772709241249970 ) ) ;
#95034=EDGE_CURVE ( 'NONE', #100575, #33927, #7009, .T. ) ;
#95035=CARTESIAN_POINT ( 'NONE',  ( 3.484702367460000172, 1452.791371899229944, 152.5519604361979873 ) ) ;
#95037=CARTESIAN_POINT ( 'NONE',  ( -23.06762233478933055, 1409.889827747422032, 209.9527113325115408 ) ) ;
#95041=CARTESIAN_POINT ( 'NONE',  ( -17.78552240860015488, 1460.054203228820370, 228.1338144972297926 ) ) ;
#95045=VERTEX_POINT ( 'NONE', #10316 ) ;
#95047=CARTESIAN_POINT ( 'NONE',  ( 19.56213531549639839, 1508.835144824000054, 229.7005312132949939 ) ) ;
#95049=CARTESIAN_POINT ( 'NONE',  ( 40.27308693906149273, 1443.611999474700042, 137.1163322506119755 ) ) ;
#95050=CARTESIAN_POINT ( 'NONE',  ( 14.55570725811163157, 1412.291795584168312, 269.3628599515130873 ) ) ;
#95051=CARTESIAN_POINT ( 'NONE',  ( -37.17588026959999326, 1458.776664316129882, 264.1764829737979881 ) ) ;
#95056=CARTESIAN_POINT ( 'NONE',  ( -19.85891451210000014, 1485.179989725129872, 190.7502780007980050 ) ) ;
#95057=CARTESIAN_POINT ( 'NONE',  ( 1.441735424540000032, 1409.901586897629841, 185.3129409531979945 ) ) ;
#95059=CARTESIAN_POINT ( 'NONE',  ( -7.036086178909999767, 1439.758762051160147, 154.1890771745979691 ) ) ;
#95062=CARTESIAN_POINT ( 'NONE',  ( -3.146029458580000160, 1451.975600841429923, 154.0166248088980012 ) ) ;
#95067=CARTESIAN_POINT ( 'NONE',  ( -44.93135410500000404, 1442.582777215279975, 269.6838066175980089 ) ) ;
#95069=CARTESIAN_POINT ( 'NONE',  ( 11.98951922200000020, 1442.759074889710064, 150.6922381223979812 ) ) ;
#95072=CARTESIAN_POINT ( 'NONE',  ( 13.22806383169999833, 1431.113060387329824, 195.8937821296979962 ) ) ;
#95073=CARTESIAN_POINT ( 'NONE',  ( 2.793203188579529872, 1409.027311659480119, 230.4220898241179896 ) ) ;
#95074=CARTESIAN_POINT ( 'NONE',  ( -0.7440358369610000633, 1416.274718422629803, 227.8470358584980033 ) ) ;
#95075=CARTESIAN_POINT ( 'NONE',  ( -2.256759385399999651, 1417.436677706029968, 235.4758680199980176 ) ) ;
#95076=CARTESIAN_POINT ( 'NONE',  ( -0.6733940044856625562, 1485.373885326774371, 181.9506766061667804 ) ) ;
#95078=CARTESIAN_POINT ( 'NONE',  ( -45.50576722784600037, 1438.311143129649963, 268.9784717228729960 ) ) ;
#95079=CARTESIAN_POINT ( 'NONE',  ( -2.500000000000000000, 1425.929641636930000, 184.1455913746980002 ) ) ;
#95088=EDGE_LOOP ( 'NONE', ( #51940, #49812, #110057, #56125 ) ) ;
#95089=CYLINDRICAL_SURFACE ( 'NONE', #68901, 2.000000000000000000 ) ;
#95093=CARTESIAN_POINT ( 'NONE',  ( -11.59871332934921639, 1426.255604624567468, 138.4425913800236287 ) ) ;
#95096=VERTEX_POINT ( 'NONE', #95437 ) ;
#95097=CARTESIAN_POINT ( 'NONE',  ( -3.098696616388379788, 1408.307991063760255, 270.3912379415129976 ) ) ;
#95099=CARTESIAN_POINT ( 'NONE',  ( 12.42248214874839896, 1420.733284265709926, 230.8418435108919766 ) ) ;
#95100=CARTESIAN_POINT ( 'NONE',  ( -20.59684415639999955, 1507.762623717429960, 190.9355247910979756 ) ) ;
#95104=CARTESIAN_POINT ( 'NONE',  ( -23.73673603223410211, 1411.112104334589958, 210.2769570570919768 ) ) ;
#95106=CARTESIAN_POINT ( 'NONE',  ( 3.653292041488962916, 1424.985912203865610, 184.9355336758895874 ) ) ;
#95109=CARTESIAN_POINT ( 'NONE',  ( -20.53774147538043238, 1436.446361497854241, 144.8508540958611093 ) ) ;
#95110=CARTESIAN_POINT ( 'NONE',  ( -22.98589895030000108, 1420.827177425029959, 211.9705801624280070 ) ) ;
#95111=CARTESIAN_POINT ( 'NONE',  ( 38.96315770833140135, 1459.274076524980046, 266.3799300039799505 ) ) ;
#95112=EDGE_CURVE ( 'NONE', #19532, #21233, #85555, .T. ) ;
#95114=CARTESIAN_POINT ( 'NONE',  ( 14.25613302710000063, 1464.413060387330006, 224.0689215379980226 ) ) ;
#95117=CARTESIAN_POINT ( 'NONE',  ( 23.51028611932632018, 1411.094384488653986, 211.8659750899354037 ) ) ;
#95118=CARTESIAN_POINT ( 'NONE',  ( 1.486105993495000277, 1473.851208882719902, 182.5641111719070295 ) ) ;
#95119=CARTESIAN_POINT ( 'NONE',  ( 22.69620822199999921, 1409.705526811329946, 208.7849502228380345 ) ) ;
#95120=ORIENTED_EDGE ( 'NONE', *, *, #36144, .F. ) ;
#95123=CARTESIAN_POINT ( 'NONE',  ( 24.99678597100239585, 1451.803817917760171, 136.6927953316869946 ) ) ;
#95128=CARTESIAN_POINT ( 'NONE',  ( 18.03578411879999877, 1409.707763031429749, 194.6290428685979919 ) ) ;
#95129=CARTESIAN_POINT ( 'NONE',  ( 13.35741048202589809, 1444.324653571830822, 164.9741927960640453 ) ) ;
#95130=CARTESIAN_POINT ( 'NONE',  ( 3.573960252902736556, 1439.695850415500217, 184.5435116089865915 ) ) ;
#95131=CARTESIAN_POINT ( 'NONE',  ( 0.1707430212980000084, 1416.982709795129949, 234.1884028855980091 ) ) ;
#95132=CARTESIAN_POINT ( 'NONE',  ( -22.83130780170417395, 1432.445202165297133, 215.4846681824749908 ) ) ;
#95133=DIRECTION ( 'NONE',  ( -0.8960382015506694886, 0.4437655256578362795, 0.01370035034099489381 ) ) ;
#95138=CARTESIAN_POINT ( 'NONE',  ( 10.63675272238868885, 1419.812825537269873, 232.2865147438434690 ) ) ;
#95142=CARTESIAN_POINT ( 'NONE',  ( -0.4930154003685739972, 1409.658068983249905, 232.9865684859400119 ) ) ;
#95147=CARTESIAN_POINT ( 'NONE',  ( -20.74408966469999882, 1445.748654444849990, 224.8635561966979708 ) ) ;
#95149=CARTESIAN_POINT ( 'NONE',  ( 11.88679881449999876, 1433.350353069249877, 150.2822412956980145 ) ) ;
#95150=CARTESIAN_POINT ( 'NONE',  ( 19.46212511719999938, 1448.109899942129914, 224.8635562210979799 ) ) ;
#95152=ADVANCED_FACE ( 'NONE', ( #18156 ), #55555, .F. ) ;
#95155=CARTESIAN_POINT ( 'NONE',  ( 23.77649893510000112, 1435.334014145809988, 137.3596790345980025 ) ) ;
#95156=CARTESIAN_POINT ( 'NONE',  ( 22.60265952820000024, 1409.702346025430188, 208.8284293190110077 ) ) ;
#95157=CARTESIAN_POINT ( 'NONE',  ( 11.91243657443186699, 1398.266254915216905, 214.3270314564130103 ) ) ;
#95158=CARTESIAN_POINT ( 'NONE',  ( -29.74692510567269821, 1509.964815989430008, 211.8522445133610290 ) ) ;
#95159=TOROIDAL_SURFACE ( 'NONE', #9319, 4.000000000000000000, 1.000000000000000000 ) ;
#95160=CARTESIAN_POINT ( 'NONE',  ( 25.27895407529999972, 1469.239702721330104, 214.6649670560380230 ) ) ;
#95161=B_SPLINE_CURVE_WITH_KNOTS ( 'NONE', 3,
 ( #107994, #22311, #31291, #23438, #38050, #90641, #22867, #65475, #74427, #40245, #63823, #97936, #83346, #73308, #66030, #12836, #91200, #82797, #107444, #106351, #55413, #57076, #100153, #89547, #57632, #91746, #72227, #4985, #47016, #81141, #72763, #38584, #106890, #47557, #90085, #92297, #480, #67127, #101789, #84458, #101227, #110761, #59282, #42449, #76609, #7745, #76063, #102351, #32406, #8837, #34051, #50863, #66587, #93400, #83900, #34604, #110205, #17214, #43020, #77178, #25078, #7206, #67681, #68790, #58168, #109664, #50332, #102890, #26189, #25634, #58715, #15567, #100690, #85540, #6644, #16665, #23973, #60377, #94498, #41909, #49768, #68242, #24527, #84992, #109125, #41362, #33479, #8287 ),
 .UNSPECIFIED., .F., .F.,
 ( 4, 3, 3, 3, 3, 3, 3, 3, 3, 3, 3, 3, 3, 3, 3, 3, 3, 3, 3, 3, 3, 3, 3, 3, 3, 3, 3, 3, 3, 4 ),
 ( -2.608805242767630261, -1.335759665544890007, -0.03842482041208983290, 1.300439966035479955, 2.667507357936759860, 4.080875363370900288, 4.341750878185000495, 5.839428055071511636, 7.370373697392469836, 8.938676201850199732, 10.62243765222589964, 12.30567332129900038, 14.04213788646359973, 15.10556603929509834, 15.67372200335319832, 16.64339347143850034, 17.60617660898700265, 18.59539778760229822, 19.57499817531500241, 20.56364872257519849, 21.56169445605650026, 22.52530327033359825, 23.60819854813160035, 24.64216807509990304, 25.68594691940390007, 26.73955916627750184, 27.85178574788760386, 28.92923767607740260, 30.05885158439770066, 31.18846549271799518 ),
 .UNSPECIFIED. ) ;
#95163=CARTESIAN_POINT ( 'NONE',  ( 26.47820321154927470, 1436.726665921244148, 136.8127344866470025 ) ) ;
#95165=( BOUNDED_CURVE ( )  B_SPLINE_CURVE ( 3, ( #41601, #103703, #26431, #93087 ),
 .UNSPECIFIED., .F., .F. ) 
 B_SPLINE_CURVE_WITH_KNOTS ( ( 4, 4 ),
 ( 6.248344042517810948, 6.260122023476537123 ),
 .UNSPECIFIED. ) 
 CURVE ( )  GEOMETRIC_REPRESENTATION_ITEM ( )  RATIONAL_B_SPLINE_CURVE ( ( 1.000000000000000000, 0.9999884399637866128, 0.9999884399637866128, 1.000000000000000000 ) ) 
 REPRESENTATION_ITEM ( '' )  );
#95169=CARTESIAN_POINT ( 'NONE',  ( 0.1596977958884080173, 1486.448930399509891, 181.8173153803849971 ) ) ;
#95171=EDGE_LOOP ( 'NONE', ( #64565, #79267, #96523, #48328, #74816 ) ) ;
#95172=CARTESIAN_POINT ( 'NONE',  ( -0.7133823615420000763, 1416.822694282129987, 227.9183241380980007 ) ) ;
#95174=CARTESIAN_POINT ( 'NONE',  ( -20.59664500270120158, 1507.763472350329948, 190.3621299389660066 ) ) ;
#95179=SPHERICAL_SURFACE ( 'NONE', #82509, 2.000000000730000060 ) ;
#95181=CARTESIAN_POINT ( 'NONE',  ( -12.70717216449999931, 1414.913060387329779, 220.4277423101980276 ) ) ;
#95195=CARTESIAN_POINT ( 'NONE',  ( 24.66759386739999727, 1507.924354362629856, 220.6865237209979966 ) ) ;
#95198=CARTESIAN_POINT ( 'NONE',  ( 29.14946092887392481, 1509.937924658664770, 213.7557683796928814 ) ) ;
#95200=CARTESIAN_POINT ( 'NONE',  ( 19.15376622239216076, 1438.408328458145661, 212.9158144853951740 ) ) ;
#95201=CARTESIAN_POINT ( 'NONE',  ( 1.723041758439999960, 1417.151714778930000, 232.9552265120979939 ) ) ;
#95207=EDGE_CURVE ( 'NONE', #43746, #60804, #73486, .T. ) ;
#95211=CARTESIAN_POINT ( 'NONE',  ( -2.500000000000000000, 1438.683324620350049, 157.7083961265980179 ) ) ;
#95212=CARTESIAN_POINT ( 'NONE',  ( 14.20177175210000087, 1416.825532216630108, 196.5059038677979686 ) ) ;
#95214=ORIENTED_EDGE ( 'NONE', *, *, #55537, .T. ) ;
#95216=ORIENTED_EDGE ( 'NONE', *, *, #23342, .T. ) ;
#95218=CARTESIAN_POINT ( 'NONE',  ( -23.18005802010000238, 1410.911243146729930, 205.3224337777979827 ) ) ;
#95219=CARTESIAN_POINT ( 'NONE',  ( -10.90887219343169967, 1425.661441503749757, 108.4510460995380043 ) ) ;
#95220=CARTESIAN_POINT ( 'NONE',  ( 17.28255409390969888, 1410.597227212849930, 192.3502816095650019 ) ) ;
#95222=CARTESIAN_POINT ( 'NONE',  ( 28.69212989171126083, 1510.026194129199666, 217.9223110541325923 ) ) ;
#95223=CARTESIAN_POINT ( 'NONE',  ( -22.95908931529999819, 1507.624001450029937, 207.8018278714380074 ) ) ;
#95224=CARTESIAN_POINT ( 'NONE',  ( -36.52133751200000233, 1436.268775032720214, 254.5789788204980084 ) ) ;
#95226=CARTESIAN_POINT ( 'NONE',  ( 28.32839678142520157, 1508.625224770790055, 209.4146328292849830 ) ) ;
#95228=CARTESIAN_POINT ( 'NONE',  ( -36.89672635344380325, 1437.851014151270192, 136.5554436358479791 ) ) ;
#95229=ORIENTED_EDGE ( 'NONE', *, *, #80952, .T. ) ;
#95230=CARTESIAN_POINT ( 'NONE',  ( 10.70562411493910027, 1396.809431658850144, 216.5037525343219897 ) ) ;
#95232=CARTESIAN_POINT ( 'NONE',  ( -17.43039599940000173, 1458.275712043530120, 229.4620914164979979 ) ) ;
#95234=ORIENTED_EDGE ( 'NONE', *, *, #70945, .F. ) ;
#95237=ORIENTED_EDGE ( 'NONE', *, *, #69676, .T. ) ;
#95238=CARTESIAN_POINT ( 'NONE',  ( 0.1180531581219999987, 1410.296228957430003, 184.9798896325980024 ) ) ;
#95239=DIRECTION ( 'NONE',  ( -0.8564730265368828421, -0.5161917810414575758, 0.000000000000000000 ) ) ;
#95241=CARTESIAN_POINT ( 'NONE',  ( 27.43651637349223193, 1509.328400154276551, 206.1603289671332107 ) ) ;
#95243=EDGE_CURVE ( 'NONE', #81651, #102101, #38579, .T. ) ;
#95251=CARTESIAN_POINT ( 'NONE',  ( 11.85930646257130050, 1431.861885083070092, 149.9617303242330308 ) ) ;
#95252=EDGE_CURVE ( 'NONE', #80530, #100437, #86974, .T. ) ;
#95255=ORIENTED_EDGE ( 'NONE', *, *, #76298, .T. ) ;
#95256=CARTESIAN_POINT ( 'NONE',  ( 7.254034580837151580, 1423.037804158368544, 139.1419882753651791 ) ) ;
#95258=CARTESIAN_POINT ( 'NONE',  ( 9.157527028969999705, 1509.060285975029956, 235.8715647223980056 ) ) ;
#95259=EDGE_CURVE ( 'NONE', #67251, #76272, #62065, .T. ) ;
#95261=CARTESIAN_POINT ( 'NONE',  ( -4.605225103679999599, 1422.042318833529862, 184.9396219054979724 ) ) ;
#95262=CARTESIAN_POINT ( 'NONE',  ( 1.462222899693720102, 1408.251425098729896, 270.3922974192450397 ) ) ;
#95263=CARTESIAN_POINT ( 'NONE',  ( -4.738498500012391368, 1427.169020172040746, 137.0999999980979851 ) ) ;
#95270=CARTESIAN_POINT ( 'NONE',  ( 15.29853388839999973, 1471.323284329529770, 194.6523739445979970 ) ) ;
#95272=CARTESIAN_POINT ( 'NONE',  ( 17.61568774148620165, 1411.200535208959991, 224.8174967984410273 ) ) ;
#95273=CARTESIAN_POINT ( 'NONE',  ( -5.735709145435179401, 1423.321980822750220, 94.86005652877258854 ) ) ;
#95275=CARTESIAN_POINT ( 'NONE',  ( 43.50000000000000000, 1440.913060387330006, 271.1218459616979999 ) ) ;
#95277=CARTESIAN_POINT ( 'NONE',  ( 18.02694236555139895, 1424.485126976410129, 224.5424481119590041 ) ) ;
#95279=CARTESIAN_POINT ( 'NONE',  ( -2.910649417096987435, 1484.739743472488044, 183.2378289904456210 ) ) ;
#95283=VERTEX_POINT ( 'NONE', #110444 ) ;
#95284=CARTESIAN_POINT ( 'NONE',  ( 17.09817538404499970, 1414.913526854310021, 210.5930684982130003 ) ) ;
#95287=DIRECTION ( 'NONE',  ( 0.4794255386042038380, 0.000000000000000000, 0.8775825618903722036 ) ) ;
#95291=DIRECTION ( 'NONE',  ( -1.000000000000000000, 0.000000000000000000, 0.000000000000000000 ) ) ;
#95294=CARTESIAN_POINT ( 'NONE',  ( 16.27592940589999770, 1412.749584434430062, 226.8352020966980263 ) ) ;
#95296=CARTESIAN_POINT ( 'NONE',  ( -16.33051720469999779, 1460.522939258030192, 228.3433114430980027 ) ) ;
#95298=CARTESIAN_POINT ( 'NONE',  ( 14.52947405539999970, 1407.976345905729886, 269.2157512787979954 ) ) ;
#95299=CARTESIAN_POINT ( 'NONE',  ( 24.02336744349999620, 1436.564838698800031, 139.9832055672980005 ) ) ;
#95301=CARTESIAN_POINT ( 'NONE',  ( 20.93632175249999960, 1469.156076992429917, 193.5744950039980097 ) ) ;
#95302=CARTESIAN_POINT ( 'NONE',  ( -23.24680097320000272, 1434.020615140939981, 214.0512479341779795 ) ) ;
#95305=CARTESIAN_POINT ( 'NONE',  ( -1.568427187249999966, 1452.094535719030091, 183.9924580127980107 ) ) ;
#95306=CARTESIAN_POINT ( 'NONE',  ( -6.825986752669999547, 1409.091027441130109, 196.5037156953979718 ) ) ;
#95308=CARTESIAN_POINT ( 'NONE',  ( -13.58597427780000011, 1441.854506128520143, 188.4823871297980133 ) ) ;
#95314=CARTESIAN_POINT ( 'NONE',  ( -14.73919588483700061, 1409.427764449309734, 211.5316301116640147 ) ) ;
#95315=FACE_OUTER_BOUND ( 'NONE', #104188, .T. ) ;
#95317=CARTESIAN_POINT ( 'NONE',  ( -26.93323766929999863, 1469.218382335129945, 266.6753116650979791 ) ) ;
#95318=CARTESIAN_POINT ( 'NONE',  ( -17.27558692971449972, 1507.606285623229951, 224.2552697136770234 ) ) ;
#95319=CARTESIAN_POINT ( 'NONE',  ( 0.1904623309857999824, 1420.430684221689944, 183.1881945191479986 ) ) ;
#95320=CARTESIAN_POINT ( 'NONE',  ( -24.17806289182839663, 1444.519329898075512, 211.5601904552849533 ) ) ;
#95323=CARTESIAN_POINT ( 'NONE',  ( 17.04561243864089803, 1423.674420110669871, 228.9411243753750114 ) ) ;
#95324=CARTESIAN_POINT ( 'NONE',  ( 20.59269117889999734, 1507.766073656829803, 227.7908422914979951 ) ) ;
#95325=CARTESIAN_POINT ( 'NONE',  ( -28.25247054546100145, 1508.179583162469953, 208.8562385362949954 ) ) ;
#95326=ADVANCED_FACE ( 'NONE', ( #34284 ), #22674, .F. ) ;
#95329=CARTESIAN_POINT ( 'NONE',  ( -5.818429214160000029, 1509.055275519029919, 180.2714693110980022 ) ) ;
#95330=CARTESIAN_POINT ( 'NONE',  ( -23.26696311050000077, 1409.890070742030048, 207.5628654440679952 ) ) ;
#95332=CARTESIAN_POINT ( 'NONE',  ( 17.48265376240000180, 1415.426210663629945, 208.8075711781490043 ) ) ;
#95338=CARTESIAN_POINT ( 'NONE',  ( -27.69925886641940238, 1441.434395751479997, 137.3015763626259798 ) ) ;
#95339=CARTESIAN_POINT ( 'NONE',  ( -22.33897372919999924, 1410.187224172929746, 212.0108092242280122 ) ) ;
#95340=CARTESIAN_POINT ( 'NONE',  ( -44.93136608500000051, 1440.913060387330006, 269.6838062106980374 ) ) ;
#95341=CARTESIAN_POINT ( 'NONE',  ( -0.5089086897610000104, 1411.661826841030006, 233.2294965383979957 ) ) ;
#95344=CARTESIAN_POINT ( 'NONE',  ( -23.54487295850000095, 1420.914744205530042, 210.9134490421280077 ) ) ;
#95345=CARTESIAN_POINT ( 'NONE',  ( -0.9591724243577970377, 1420.560689427859870, 184.1653156966539768 ) ) ;
#95349=CARTESIAN_POINT ( 'NONE',  ( -3.356147517029587579, 1440.691650900622562, 156.8829035650872186 ) ) ;
#95350=CARTESIAN_POINT ( 'NONE',  ( -17.42709856749150177, 1485.949155400869813, 188.1984452550049980 ) ) ;
#95351=CARTESIAN_POINT ( 'NONE',  ( -17.72806394670000074, 1410.889176615030010, 194.8230026513979851 ) ) ;
#95353=CARTESIAN_POINT ( 'NONE',  ( 39.23020515599449709, 1448.346468128479955, 136.4190043813750037 ) ) ;
#95355=ORIENTED_EDGE ( 'NONE', *, *, #41982, .T. ) ;
#95356=ORIENTED_EDGE ( 'NONE', *, *, #43968, .T. ) ;
#95357=CARTESIAN_POINT ( 'NONE',  ( 11.95021264318459941, 1433.547364810169938, 150.0873180042360104 ) ) ;
#95358=CARTESIAN_POINT ( 'NONE',  ( 0.06016801242969999769, 1397.283812744030001, 222.0600360843979786 ) ) ;
#95359=ORIENTED_EDGE ( 'NONE', *, *, #103486, .F. ) ;
#95364=CARTESIAN_POINT ( 'NONE',  ( 13.89896040166999924, 1452.843947645199933, 223.8762708690549914 ) ) ;
#95365=CARTESIAN_POINT ( 'NONE',  ( 11.94206337009999963, 1438.199233188169956, 150.9847479746979957 ) ) ;
#95367=CARTESIAN_POINT ( 'NONE',  ( 1.580841669900000079, 1507.641628515030106, 181.1142457626980331 ) ) ;
#95369=CARTESIAN_POINT ( 'NONE',  ( 14.91703010720000044, 1409.433974557229931, 225.8933006754979829 ) ) ;
#95371=CARTESIAN_POINT ( 'NONE',  ( 34.11564357267010195, 1435.688851149350285, 134.0999999980979851 ) ) ;
#95374=ORIENTED_EDGE ( 'NONE', *, *, #41280, .T. ) ;
#95375=CARTESIAN_POINT ( 'NONE',  ( 13.59790036228669940, 1434.964892464889999, 148.8305582646289906 ) ) ;
#95382=CARTESIAN_POINT ( 'NONE',  ( -1.139293766549999809, 1467.057741776030070, 235.4579552793979929 ) ) ;
#95383=CARTESIAN_POINT ( 'NONE',  ( 28.86644038478740626, 1509.921098698501737, 202.4756158416115852 ) ) ;
#95386=CARTESIAN_POINT ( 'NONE',  ( -19.08809138029046082, 1441.859548814234131, 210.2413154080126674 ) ) ;
#95388=CARTESIAN_POINT ( 'NONE',  ( 4.225121941997549868, 1446.251017732170112, 166.4055522513860126 ) ) ;
#95390=CARTESIAN_POINT ( 'NONE',  ( 1.304108710279999972, 1508.717026135230071, 238.0028103276980289 ) ) ;
#95391=ORIENTED_EDGE ( 'NONE', *, *, #106664, .F. ) ;
#95393=ORIENTED_EDGE ( 'NONE', *, *, #47972, .F. ) ;
#95394=CARTESIAN_POINT ( 'NONE',  ( 21.50585395376209874, 1440.913060387330006, 224.9641782112639987 ) ) ;
#95395=CARTESIAN_POINT ( 'NONE',  ( -16.51373361550000141, 1508.736179495329907, 185.6988723191980171 ) ) ;
#95396=EDGE_CURVE ( 'NONE', #48130, #31461, #62818, .T. ) ;
#95399=CARTESIAN_POINT ( 'NONE',  ( -13.50724518150000009, 1409.886837265230042, 190.1809790390979913 ) ) ;
#95400=CARTESIAN_POINT ( 'NONE',  ( -24.90968947180000015, 1441.637783390069899, 210.4505011253679925 ) ) ;
#95401=CARTESIAN_POINT ( 'NONE',  ( -11.08206323070000110, 1414.913528139129994, 196.0394634478979867 ) ) ;
#95402=CARTESIAN_POINT ( 'NONE',  ( -11.73701141503820011, 1426.696005490819971, 144.1689084034089774 ) ) ;
#95403=CARTESIAN_POINT ( 'NONE',  ( -11.95702896124850945, 1433.550299325597734, 147.6125996980034927 ) ) ;
#95404=CARTESIAN_POINT ( 'NONE',  ( -27.37591788248279911, 1439.764921109970146, 137.1160056607250226 ) ) ;
#95405=CARTESIAN_POINT ( 'NONE',  ( -12.27023110815660090, 1416.839692126590080, 194.6640136892829958 ) ) ;
#95406=EDGE_CURVE ( 'NONE', #73277, #102562, #78506, .T. ) ;
#95407=CARTESIAN_POINT ( 'NONE',  ( -26.86204968941349946, 1508.007394745769943, 212.0120970035400205 ) ) ;
#95413=CARTESIAN_POINT ( 'NONE',  ( 28.22027450670000093, 1509.158030589630016, 207.9424314675380003 ) ) ;
#95419=ORIENTED_EDGE ( 'NONE', *, *, #106151, .F. ) ;
#95420=CARTESIAN_POINT ( 'NONE',  ( 6.121216816089999737E-10, 1465.143864797330025, 238.2947585024979844 ) ) ;
#95422=CARTESIAN_POINT ( 'NONE',  ( -28.07099224718820096, 1509.893321036980069, 217.6805618164050031 ) ) ;
#95423=CARTESIAN_POINT ( 'NONE',  ( -7.384241671499998994, 1508.154784625329967, 235.7410849829979895 ) ) ;
#95426=CARTESIAN_POINT ( 'NONE',  ( -20.40418802339999615, 1454.957320663730115, 226.6330256287980092 ) ) ;
#95427=CARTESIAN_POINT ( 'NONE',  ( 11.77090819340000039, 1432.440121525590030, 150.8116842255979861 ) ) ;
#95435=FACE_OUTER_BOUND ( 'NONE', #37674, .T. ) ;
#95436=CARTESIAN_POINT ( 'NONE',  ( 19.66827358063540032, 1471.163942014939948, 270.2287850334790278 ) ) ;
#95437=CARTESIAN_POINT ( 'NONE',  ( -12.87561223598270033, 1428.667272998819954, 222.5140706137790119 ) ) ;
#95438=CARTESIAN_POINT ( 'NONE',  ( -39.89556624698280274, 1446.848291182909861, 136.6543435533029935 ) ) ;
#95441=FACE_OUTER_BOUND ( 'NONE', #68235, .T. ) ;
#95442=CARTESIAN_POINT ( 'NONE',  ( -2.303292313784549794, 1449.840026941649967, 154.2474790842049970 ) ) ;
#95448=CARTESIAN_POINT ( 'NONE',  ( 3.237924447490000190, 1448.965650011070238, 183.9353614378979955 ) ) ;
#95450=CARTESIAN_POINT ( 'NONE',  ( -1.676215897828090107, 1450.511945644329899, 182.4451613505460159 ) ) ;
#95452=CARTESIAN_POINT ( 'NONE',  ( -2.531216514170000106E-09, 1476.109324709230123, 267.8540375962979851 ) ) ;
#95454=CARTESIAN_POINT ( 'NONE',  ( -28.45104125860000011, 1509.631525670130031, 210.7633834292879840 ) ) ;
#95458=B_SPLINE_SURFACE_WITH_KNOTS ( 'NONE', 5, 5, ( 
 ( #38683, #37039, #98036, #105356, #62850, #96963 ),
 ( #97501, #12383, #20770, #20228, #46569, #21309 ),
 ( #4549, #57723, #23531, #39799, #107546, #57174 ),
 ( #101319, #75068, #75619, #109217, #22967, #6731 ),
 ( #92944, #48212, #40887, #40337, #31935, #41456 ),
 ( #49859, #65565, #58261, #92382, #32503, #73410 ) ),
 .UNSPECIFIED., .F., .F., .F.,
 ( 6, 6 ),
 ( 6, 6 ),
 ( 6.286300432643599834, 8.359473755869998968 ),
 ( -6.051085639767849584E-05, 1.449160878988990042 ),
 .UNSPECIFIED. ) ;
#95459=CARTESIAN_POINT ( 'NONE',  ( -18.94485037129999583, 1416.547221147930031, 207.7783220669780064 ) ) ;
#95461=CARTESIAN_POINT ( 'NONE',  ( 26.68817439343250086, 1436.428552520020048, 136.7217815448680085 ) ) ;
#95462=CARTESIAN_POINT ( 'NONE',  ( -10.38565289721849894, 1396.275735379490015, 205.2936222502430041 ) ) ;
#95464=B_SPLINE_CURVE_WITH_KNOTS ( 'NONE', 3,
 ( #64299, #98418, #89474, #12770, #13292, #45843, #30669, #21690, #72690, #79976, #81067, #105743, #47484, #46948, #56435, #90566, #3294, #37426, #28472, #4382, #13845, #38511, #81607, #4912, #39628, #39051, #82168, #71623, #29027, #63213, #97320, #20590, #54789, #88921, #12207, #46402, #80534 ),
 .UNSPECIFIED., .F., .F.,
 ( 4, 2, 2, 1, 1, 2, 2, 2, 2, 1, 1, 1, 2, 2, 2, 2, 1, 1, 1, 1, 2, 2, 4 ),
 ( 0.000000000000000000, 0.1249999999997495059, 0.1874999999996246336, 0.2187499999995654310, 0.2343749999995357880, 0.2421874999995215216, 0.2499999999995072830, 0.3749999999993752775, 0.4374999999993093858, 0.4687499999992708610, 0.4843749999992515987, 0.4921874999992420507, 0.4960937499992379984, 0.4999999999992339461, 0.6249999999992830180, 0.6874999999993065547, 0.7187499999993083311, 0.7343749999993101074, 0.7421874999993202104, 0.7460937499993262056, 0.7480468749993290922, 0.7499999999993318678, 1.000000000000000000 ),
 .UNSPECIFIED. ) ;
#95465=CARTESIAN_POINT ( 'NONE',  ( -16.78826593861180072, 1409.746375843580154, 225.6242863346600132 ) ) ;
#95466=CARTESIAN_POINT ( 'NONE',  ( 7.390160694869999602, 1438.194204504490017, 149.6789596403979772 ) ) ;
#95469=FACE_OUTER_BOUND ( 'NONE', #72733, .T. ) ;
#95473=CARTESIAN_POINT ( 'NONE',  ( 4.145890503519879644, 1424.386680318709978, 184.7442299159029915 ) ) ;
#95481=EDGE_LOOP ( 'NONE', ( #31494, #4741, #88450, #8280, #55978, #37960 ) ) ;
#95483=CARTESIAN_POINT ( 'NONE',  ( -41.66135440509999910, 1443.796918820770088, 135.6885369501979994 ) ) ;
#95485=CARTESIAN_POINT ( 'NONE',  ( 10.78871504700000017, 1416.913060387330006, 209.1218460627730167 ) ) ;
#95487=CARTESIAN_POINT ( 'NONE',  ( -3.509122693450000163, 1486.112957707730175, 181.9976544228979662 ) ) ;
#95490=CARTESIAN_POINT ( 'NONE',  ( -33.92643878696880222, 1450.868569007310043, 136.1710250821759871 ) ) ;
#95491=CARTESIAN_POINT ( 'NONE',  ( -2.500000000000000000, 1448.322085267190005, 163.7893231724509917 ) ) ;
#95493=CARTESIAN_POINT ( 'NONE',  ( -0.06764688652389970469, 1408.848989328409971, 194.7501694707590048 ) ) ;
#95494=CARTESIAN_POINT ( 'NONE',  ( -2.306328001459209798, 1405.753257883129891, 267.8520456273699892 ) ) ;
#95495=CARTESIAN_POINT ( 'NONE',  ( -14.25060731567010031, 1435.219473732530105, 149.2644110217260334 ) ) ;
#95497=CARTESIAN_POINT ( 'NONE',  ( -11.76945428679999850, 1432.334073391449920, 150.8119095936980045 ) ) ;
#95498=CARTESIAN_POINT ( 'NONE',  ( 13.61829878390000026, 1442.132340210329858, 189.2393822471979945 ) ) ;
#95500=ORIENTED_EDGE ( 'NONE', *, *, #5277, .T. ) ;
#95507=( BOUNDED_CURVE ( )  B_SPLINE_CURVE ( 3, ( #86209, #43667, #70002, #86765 ),
 .UNSPECIFIED., .F., .T. ) 
 B_SPLINE_CURVE_WITH_KNOTS ( ( 4, 4 ),
 ( 4.409610686089010301, 5.070003787395050310 ),
 .UNSPECIFIED. ) 
 CURVE ( )  GEOMETRIC_REPRESENTATION_ITEM ( )  RATIONAL_B_SPLINE_CURVE ( ( 1.000000000000000000, 0.9639857562574201122, 0.9639857562574201122, 1.000000000000000000 ) ) 
 REPRESENTATION_ITEM ( '' )  );
#95511=CARTESIAN_POINT ( 'NONE',  ( -27.79260863660000069, 1509.155959128430140, 205.2888991007580159 ) ) ;
#95516=DIRECTION ( 'NONE',  ( 0.03489949670250328678, -0.9993908270190956511, 0.000000000000000000 ) ) ;
#95518=FACE_OUTER_BOUND ( 'NONE', #16577, .T. ) ;
#95519=ORIENTED_EDGE ( 'NONE', *, *, #26905, .F. ) ;
#95520=CARTESIAN_POINT ( 'NONE',  ( -14.33372314578957685, 1435.338670000912771, 149.4045306351138152 ) ) ;
#95522=AXIS2_PLACEMENT_3D ( 'NONE', #19373, #20471, #12651 ) ;
#95524=CARTESIAN_POINT ( 'NONE',  ( -24.14015075980000091, 1435.359055859420096, 136.8785243455980094 ) ) ;
#95528=CARTESIAN_POINT ( 'NONE',  ( -9.528680398390617867, 1426.561164775804173, 224.8846064741542818 ) ) ;
#95530=CARTESIAN_POINT ( 'NONE',  ( 18.24616163292674997, 1410.913102185548269, 193.8889752366858374 ) ) ;
#95532=ORIENTED_EDGE ( 'NONE', *, *, #22963, .F. ) ;
#95534=CARTESIAN_POINT ( 'NONE',  ( -5.188689607679999760, 1410.298383163330072, 231.7973492358979968 ) ) ;
#95539=CARTESIAN_POINT ( 'NONE',  ( 11.77252734353980124, 1435.203425911839986, 151.2926090376209913 ) ) ;
#95541=CARTESIAN_POINT ( 'NONE',  ( 13.45295784994999977, 1488.405218237079907, 232.0949692908260147 ) ) ;
#95542=CARTESIAN_POINT ( 'NONE',  ( -24.20915078813088073, 1443.685751309060606, 212.4183354952696448 ) ) ;
#95544=CARTESIAN_POINT ( 'NONE',  ( 0.001557819129550000068, 1408.913005912429981, 232.2224884858979976 ) ) ;
#95545=CARTESIAN_POINT ( 'NONE',  ( 0.01215979767472630084, 1420.444058567659795, 182.6726269972920136 ) ) ;
#95547=CARTESIAN_POINT ( 'NONE',  ( -3.267314805130000277, 1421.579958532029877, 184.3265788884979770 ) ) ;
#95548=CARTESIAN_POINT ( 'NONE',  ( 19.75308522730000149, 1509.626197197730107, 187.0190083296980106 ) ) ;
#95549=DIRECTION ( 'NONE',  ( 0.000000000000000000, 0.000000000000000000, -1.000000000000000000 ) ) ;
#95552=EDGE_CURVE ( 'NONE', #38397, #23724, #26206, .T. ) ;
#95553=CARTESIAN_POINT ( 'NONE',  ( -16.44126801270000016, 1495.113783635430082, 185.9757610618979697 ) ) ;
#95554=ORIENTED_EDGE ( 'NONE', *, *, #74972, .F. ) ;
#95555=CARTESIAN_POINT ( 'NONE',  ( 3.741709429870000214, 1419.924742150030170, 185.5167356432980057 ) ) ;
#95559=CARTESIAN_POINT ( 'NONE',  ( 18.89905511659999959, 1416.828040475729949, 210.6687957193779823 ) ) ;
#95562=CARTESIAN_POINT ( 'NONE',  ( -16.52123881059080190, 1410.013485281883277, 192.0114425483922673 ) ) ;
#95563=CARTESIAN_POINT ( 'NONE',  ( 17.39559652730000039, 1414.988017874730076, 210.6209831520479838 ) ) ;
#95564=CARTESIAN_POINT ( 'NONE',  ( -17.96561697639999977, 1423.613351837929940, 225.8447415086979788 ) ) ;
#95568=CARTESIAN_POINT ( 'NONE',  ( 0.3188683952948129785, 1408.924195517089856, 231.6706331693599736 ) ) ;
#95570=CARTESIAN_POINT ( 'NONE',  ( 0.5621804143070269211, 1416.843574548494644, 190.4753774787342593 ) ) ;
#95571=ORIENTED_EDGE ( 'NONE', *, *, #58846, .T. ) ;
#95572=CARTESIAN_POINT ( 'NONE',  ( 1.553043158554480163, 1415.595619977640126, 190.7368536681399860 ) ) ;
#95573=CARTESIAN_POINT ( 'NONE',  ( 27.43355929049999986, 1507.980920699130138, 207.4175378521480013 ) ) ;
#95575=CARTESIAN_POINT ( 'NONE',  ( 2.564108462820033907, 1410.380577510105013, 185.5928496559870666 ) ) ;
#95576=CARTESIAN_POINT ( 'NONE',  ( -3.718627449938214813, 1426.012647860741481, 185.9856829451767908 ) ) ;
#95581=B_SPLINE_CURVE_WITH_KNOTS ( 'NONE', 5,
 ( #97605, #20875, #80805, #47750, #4111, #55071 ),
 .UNSPECIFIED., .F., .F.,
 ( 6, 6 ),
 ( -65.26194322900001055, -30.28564970649999566 ),
 .UNSPECIFIED. ) ;
#95585=CARTESIAN_POINT ( 'NONE',  ( -15.53981990976190986, 1506.512156827502622, 224.7632318306688148 ) ) ;
#95587=CARTESIAN_POINT ( 'NONE',  ( 23.72452558869999706, 1509.749085157929812, 191.5066069952979717 ) ) ;
#95589=CARTESIAN_POINT ( 'NONE',  ( 17.27558691658489920, 1507.606285602530079, 193.9884222186300065 ) ) ;
#95591=CARTESIAN_POINT ( 'NONE',  ( 20.12062199643419902, 1509.247360226100000, 229.8833160286590100 ) ) ;
#95594=SPHERICAL_SURFACE ( 'NONE', #11612, 2.000000000000000000 ) ;
#95595=CARTESIAN_POINT ( 'NONE',  ( -8.921631616102883910, 1502.413060387330006, 192.7909088307800403 ) ) ;
#95596=CARTESIAN_POINT ( 'NONE',  ( 12.80703219148647065, 1442.847939688957922, 169.4486344618227918 ) ) ;
#95597=CARTESIAN_POINT ( 'NONE',  ( 4.613723315850000479E-06, 1474.175172091230024, 270.1377426632980132 ) ) ;
#95598=CARTESIAN_POINT ( 'NONE',  ( -39.02581886140000478, 1459.481847435529971, 266.4771544807979922 ) ) ;
#95602=CARTESIAN_POINT ( 'NONE',  ( 25.16176845089999858, 1509.119669543930058, 197.7765890071979982 ) ) ;
#95604=CARTESIAN_POINT ( 'NONE',  ( 7.960762779720000459, 1409.191056350230156, 188.6635358462980037 ) ) ;
#95605=CARTESIAN_POINT ( 'NONE',  ( 4.401092417150000102, 1420.174153566729956, 185.7217845719979721 ) ) ;
#95607=CARTESIAN_POINT ( 'NONE',  ( -11.23219810570000021, 1436.456444669380062, 151.7916771637979991 ) ) ;
#95608=CARTESIAN_POINT ( 'NONE',  ( 12.38112414749999957, 1436.607677747480011, 151.2275680718979913 ) ) ;
#95610=CIRCLE ( 'NONE', #70622, 2.000000000027019720 ) ;
#95611=CARTESIAN_POINT ( 'NONE',  ( -20.13596110940000017, 1451.396157091630130, 145.7046208320979872 ) ) ;
#95612=DIRECTION ( 'NONE',  ( 0.000000000000000000, -1.000000000000000000, 0.000000000000000000 ) ) ;
#95616=CARTESIAN_POINT ( 'NONE',  ( -41.90242663730000316, 1445.386761933250000, 269.8748730912980136 ) ) ;
#95618=CARTESIAN_POINT ( 'NONE',  ( 16.40067670619999873, 1409.485784638129871, 222.8653037321979866 ) ) ;
#95619=CARTESIAN_POINT ( 'NONE',  ( -14.27723474240000101, 1474.170145399029934, 223.9306864886980009 ) ) ;
#95620=B_SPLINE_CURVE_WITH_KNOTS ( 'NONE', 3,
 ( #47614, #56017, #80107, #29155, #89601, #45431, #3426, #81738, #70644, #63881, #5046, #79575, #97996, #37557, #2879, #63341, #20730, #62805, #30239, #20188, #12339, #46529, #11804, #13424, #104761, #62236, #36998, #87981, #19640, #80664, #3978, #38102, #55475, #12894, #47071, #4513, #72821, #106954, #64432, #98549, #66086, #99089, #90697, #32465, #50382, #39191, #82310, #22367, #108050, #56568, #100213, #92907, #5608, #58770, #15080, #40301, #32992, #41419, #39761, #64974, #74484, #6143, #67181, #66640, #13984, #23495, #48172 ),
 .UNSPECIFIED., .F., .F.,
 ( 4, 3, 3, 3, 3, 3, 3, 3, 3, 3, 3, 3, 3, 3, 3, 3, 3, 3, 3, 3, 3, 3, 4 ),
 ( 17.98526104458165165, 20.20158955684989976, 22.42882872137870010, 24.66064011719250004, 26.89515503936650020, 29.13043065886330041, 31.36321373294149950, 33.59263454627130585, 35.81471763752789883, 36.72584873329999766, 38.94364518594499458, 41.26471793637690411, 43.50295931855809783, 45.74609346697479850, 47.99249668729089535, 50.24046781578599052, 52.48759803034639049, 54.73251631032059095, 56.97222553069789797, 57.51222718939999368, 59.74002163354938943, 61.95813442111268898, 62.49779105520408962 ),
 .UNSPECIFIED. ) ;
#95622=FACE_OUTER_BOUND ( 'NONE', #1444, .T. ) ;
#95623=CARTESIAN_POINT ( 'NONE',  ( 1.747240526799999971, 1508.468491276929853, 237.2463171569980034 ) ) ;
#95624=CARTESIAN_POINT ( 'NONE',  ( -4.890835732880000286, 1416.493263303829963, 232.1969941459979907 ) ) ;
#95627=CARTESIAN_POINT ( 'NONE',  ( -44.87017001119260584, 1433.746480055119946, 268.7864504627750080 ) ) ;
#95628=DIRECTION ( 'NONE',  ( 0.000000000000000000, -1.000000000000000000, 0.000000000000000000 ) ) ;
#95635=CARTESIAN_POINT ( 'NONE',  ( -11.52403648599999997, 1410.397193419830046, 189.0409863546979921 ) ) ;
#95638=DIRECTION ( 'NONE',  ( 0.000000000000000000, 0.000000000000000000, 1.000000000000000000 ) ) ;
#95639=CARTESIAN_POINT ( 'NONE',  ( -14.45783243223209880, 1416.839692136300073, 221.3920770721769884 ) ) ;
#95646=AXIS2_PLACEMENT_3D ( 'NONE', #75565, #83938, #59321 ) ;
#95648=CARTESIAN_POINT ( 'NONE',  ( -4.261227898591590346, 1409.354790215370031, 270.3708393906289302 ) ) ;
#95650=CARTESIAN_POINT ( 'NONE',  ( 10.58452527300000057, 1419.025207297029965, 230.2384250536979948 ) ) ;
#95656=CARTESIAN_POINT ( 'NONE',  ( -0.1698155278098549825, 1408.918990476199951, 186.4893999992370084 ) ) ;
#95657=CARTESIAN_POINT ( 'NONE',  ( 3.682239659044672209, 1424.213547858993707, 184.0104720422797300 ) ) ;
#95658=CARTESIAN_POINT ( 'NONE',  ( -0.02314905646560709920, 1409.040033148099837, 185.8702696072230083 ) ) ;
#95660=CARTESIAN_POINT ( 'NONE',  ( -18.84390879411339981, 1416.449138223469845, 207.5741054101650036 ) ) ;
#95661=CARTESIAN_POINT ( 'NONE',  ( -18.65840353449999967, 1420.836464136229779, 224.4798604198980172 ) ) ;
#95663=CARTESIAN_POINT ( 'NONE',  ( 30.10075563091589856, 1467.602242830489786, 267.1542540607859451 ) ) ;
#95664=CARTESIAN_POINT ( 'NONE',  ( -2.672061128083995207, 1466.864270888973124, 235.1107451349035955 ) ) ;
#95665=CARTESIAN_POINT ( 'NONE',  ( 10.57001467410000117, 1445.512273588180051, 185.9502834991980080 ) ) ;
#95670=CARTESIAN_POINT ( 'NONE',  ( 22.58840255639999839, 1409.701846760530088, 208.8102578915460015 ) ) ;
#95673=CARTESIAN_POINT ( 'NONE',  ( 25.76476011969039703, 1450.791939427479974, 136.8860263216379849 ) ) ;
#95675=CARTESIAN_POINT ( 'NONE',  ( -13.58268883541719951, 1416.851343898680170, 221.9096085506480165 ) ) ;
#95678=CARTESIAN_POINT ( 'NONE',  ( 18.58065462780000132, 1409.726647492329903, 195.6460095527979774 ) ) ;
#95680=CARTESIAN_POINT ( 'NONE',  ( 27.40283359139997543, 1444.740067931808653, 161.6370709818978639 ) ) ;
#95682=SPHERICAL_SURFACE ( 'NONE', #37460, 2.000000000000000000 ) ;
#95684=CARTESIAN_POINT ( 'NONE',  ( -19.31676357336673533, 1425.378157214008525, 223.6971631259767719 ) ) ;
#95685=CARTESIAN_POINT ( 'NONE',  ( 0.5746359205532659553, 1452.648651194650029, 183.3151952156349864 ) ) ;
#95687=CARTESIAN_POINT ( 'NONE',  ( 28.17856934087275889, 1509.667335739465443, 207.1106753066228237 ) ) ;
#95693=CARTESIAN_POINT ( 'NONE',  ( -0.4973741856806139783, 1409.710427932380071, 233.0131125714380005 ) ) ;
#95696=DIRECTION ( 'NONE',  ( 0.000000000000000000, 1.000000000000000000, 0.000000000000000000 ) ) ;
#95697=CARTESIAN_POINT ( 'NONE',  ( -19.02913997099999932, 1445.216574189620133, 214.3676144198679765 ) ) ;
#95700=CARTESIAN_POINT ( 'NONE',  ( 6.850948855039999508, 1456.378850165029917, 224.8635561905979898 ) ) ;
#95702=CARTESIAN_POINT ( 'NONE',  ( -16.87240959569610155, 1409.502257913620042, 196.1298155364530089 ) ) ;
#95708=CARTESIAN_POINT ( 'NONE',  ( -7.613477210479999258, 1509.311637010430104, 239.1480524702979835 ) ) ;
#95709=CARTESIAN_POINT ( 'NONE',  ( 25.44333967330000235, 1449.802117268759957, 210.9399225570080034 ) ) ;
#95711=CARTESIAN_POINT ( 'NONE',  ( 26.41054897472661978, 1436.719299170789100, 136.8255246990474348 ) ) ;
#95717=CARTESIAN_POINT ( 'NONE',  ( 0.1612883661501749999, 1485.492233344150009, 181.8584284546379877 ) ) ;
#95720=CARTESIAN_POINT ( 'NONE',  ( -0.7132217361829999991, 1416.830001031129996, 227.9186326107979994 ) ) ;
#95723=CARTESIAN_POINT ( 'NONE',  ( -39.03583412959209653, 1449.647124672839936, 134.0999999981079895 ) ) ;
#95729=CARTESIAN_POINT ( 'NONE',  ( -15.72677893080000011, 1414.913060387329779, 214.0342601902979993 ) ) ;
#95734=CARTESIAN_POINT ( 'NONE',  ( 14.04090786536569979, 1409.403379694359955, 204.0234149207160215 ) ) ;
#95740=CARTESIAN_POINT ( 'NONE',  ( 13.51812398686129590, 1443.913060387330006, 169.4008117781763190 ) ) ;
#95743=CARTESIAN_POINT ( 'NONE',  ( 26.79413740735880367, 1436.761939593030093, 136.7822073642480234 ) ) ;
#95747=CARTESIAN_POINT ( 'NONE',  ( 2.500000000000000000, 1432.413060387330006, 146.1721969590979882 ) ) ;
#95748=CARTESIAN_POINT ( 'NONE',  ( 29.34286956283065351, 1509.949564053853237, 212.7810611423796274 ) ) ;
#95750=CARTESIAN_POINT ( 'NONE',  ( 3.730133759040000108, 1396.578896005830075, 221.1163315688980049 ) ) ;
#95753=CARTESIAN_POINT ( 'NONE',  ( -0.1410079938730000038, 1452.166108153929827, 183.2447143824980174 ) ) ;
#95758=CARTESIAN_POINT ( 'NONE',  ( -12.93890803109800025, 1435.979775554859998, 150.7709582610100085 ) ) ;
#95759=CARTESIAN_POINT ( 'NONE',  ( -2.500000000000000000, 1432.399285533179864, 157.4964730843979908 ) ) ;
#95760=CARTESIAN_POINT ( 'NONE',  ( 20.59684415428669979, 1507.762623717989982, 227.6602567528719874 ) ) ;
#95763=CARTESIAN_POINT ( 'NONE',  ( 10.98592888559996261, 1414.913372219064513, 222.1709358777573300 ) ) ;
#95764=ORIENTED_EDGE ( 'NONE', *, *, #68472, .T. ) ;
#95765=CARTESIAN_POINT ( 'NONE',  ( 40.44435966889999889, 1427.769452941630107, 264.0385845990979874 ) ) ;
#95766=CARTESIAN_POINT ( 'NONE',  ( -25.80166435900000010, 1469.242112534130229, 205.3110786689379950 ) ) ;
#95767=CARTESIAN_POINT ( 'NONE',  ( -11.09416012139399932, 1426.481981508449962, 97.52552186591471184 ) ) ;
#95769=CARTESIAN_POINT ( 'NONE',  ( 16.54156502434519993, 1409.738807616770146, 192.3741591556930075 ) ) ;
#95771=CARTESIAN_POINT ( 'NONE',  ( -20.56075711880000156, 1453.152003547930008, 208.0036112637379802 ) ) ;
#95772=CARTESIAN_POINT ( 'NONE',  ( -30.53571888319999772, 1440.913060383969878, 240.1260121746980190 ) ) ;
#95774=CARTESIAN_POINT ( 'NONE',  ( 28.26734827506700043, 1508.339354035630095, 209.3952658968800051 ) ) ;
#95776=CARTESIAN_POINT ( 'NONE',  ( 30.81588140580000257, 1450.976146373729762, 136.2622935297980007 ) ) ;
#95778=CARTESIAN_POINT ( 'NONE',  ( 13.97631160088559987, 1398.327271670460050, 206.9408228097399842 ) ) ;
#95780=CARTESIAN_POINT ( 'NONE',  ( -16.96621030040000022, 1460.582762785830027, 228.2621070505979901 ) ) ;
#95781=ORIENTED_EDGE ( 'NONE', *, *, #17357, .T. ) ;
#95786=CARTESIAN_POINT ( 'NONE',  ( -0.3007994230680000602, 1410.295996030029983, 184.9875845314979870 ) ) ;
#95788=CARTESIAN_POINT ( 'NONE',  ( -17.13440814833080239, 1415.954755713489931, 207.6490729647759963 ) ) ;
#95789=CARTESIAN_POINT ( 'NONE',  ( 27.73009239421291738, 1509.592381426173688, 206.1248223153826018 ) ) ;
#95793=CARTESIAN_POINT ( 'NONE',  ( 14.61618271530000079, 1485.702860713229938, 225.6110866044979844 ) ) ;
#95798=CARTESIAN_POINT ( 'NONE',  ( 11.86596557949130037, 1432.326593078920041, 149.9824129838200122 ) ) ;
#95799=CARTESIAN_POINT ( 'NONE',  ( 12.97442686480655105, 1444.894871287640854, 186.8703375745810433 ) ) ;
#95800=EDGE_LOOP ( 'NONE', ( #46384, #101975, #101665, #9064 ) ) ;
#95801=CARTESIAN_POINT ( 'NONE',  ( -15.64138586705021439, 1506.512156834081452, 193.5820260421716341 ) ) ;
#95802=CARTESIAN_POINT ( 'NONE',  ( -17.22654844235838567, 1443.501467202828508, 162.9224179604370590 ) ) ;
#95803=CARTESIAN_POINT ( 'NONE',  ( 9.320231801240000280, 1509.238530053529985, 236.4405149249979843 ) ) ;
#95806=CARTESIAN_POINT ( 'NONE',  ( -4.917472706919999936, 1423.551379642630081, 185.2203775299980180 ) ) ;
#95807=CARTESIAN_POINT ( 'NONE',  ( 1.408315213735060079, 1410.404276229229936, 269.3348398410649907 ) ) ;
#95812=CARTESIAN_POINT ( 'NONE',  ( 0.02397233824938014776, 1410.267331098299337, 233.2206758637736641 ) ) ;
#95813=CARTESIAN_POINT ( 'NONE',  ( -17.66977881397309957, 1441.975104135429774, 190.8615125109639905 ) ) ;
#95815=CARTESIAN_POINT ( 'NONE',  ( -4.659955688642280158, 1423.687082602238888, 184.4627326681991519 ) ) ;
#95816=CARTESIAN_POINT ( 'NONE',  ( 17.83380995714600203, 1418.265691733389986, 225.0226617803320153 ) ) ;
#95818=ORIENTED_EDGE ( 'NONE', *, *, #60246, .T. ) ;
#95819=CARTESIAN_POINT ( 'NONE',  ( 13.21926162809999994, 1421.359897795430015, 248.0989693021979861 ) ) ;
#95820=CARTESIAN_POINT ( 'NONE',  ( 12.89607781515299934, 1434.724834403989917, 149.2206011272099886 ) ) ;
#95821=CARTESIAN_POINT ( 'NONE',  ( 41.61761706904538016, 1445.085543264303851, 135.5084622535695189 ) ) ;
#95835=CARTESIAN_POINT ( 'NONE',  ( -3.462069005146249712, 1432.317263652611473, 156.5316857334014742 ) ) ;
#95836=CARTESIAN_POINT ( 'NONE',  ( 16.05001174970000122, 1415.088660905229972, 227.0871310919980033 ) ) ;
#95841=CARTESIAN_POINT ( 'NONE',  ( 45.88373594299999780, 1440.913082249800027, 266.4124089362979930 ) ) ;
#95843=CARTESIAN_POINT ( 'NONE',  ( 22.52657835689999644, 1435.284668822589992, 140.3430705305979984 ) ) ;
#95844=CARTESIAN_POINT ( 'NONE',  ( 18.82137020720000109, 1469.164158803430155, 190.2666150881979945 ) ) ;
#95845=CARTESIAN_POINT ( 'NONE',  ( -22.44438185779999984, 1431.713525257879837, 217.1040214957579906 ) ) ;
#95848=CIRCLE ( 'NONE', #26044, 95.87906523535615122 ) ;
#95849=CARTESIAN_POINT ( 'NONE',  ( -30.02861084270000092, 1467.289302230230078, 266.6068817451980522 ) ) ;
#95851=CARTESIAN_POINT ( 'NONE',  ( -41.62602271621380368, 1442.681057008499920, 135.5698544226029867 ) ) ;
#95852=CARTESIAN_POINT ( 'NONE',  ( -13.30361715113500054, 1409.377633542329932, 226.2974599518520336 ) ) ;
#95854=CARTESIAN_POINT ( 'NONE',  ( -12.24704195820000052, 1441.485080693249984, 187.8203993633979962 ) ) ;
#95860=CARTESIAN_POINT ( 'NONE',  ( -14.05364299196800104, 1409.403824414780047, 214.1745042107170036 ) ) ;
#95861=FACE_OUTER_BOUND ( 'NONE', #101119, .T. ) ;
#95862=CARTESIAN_POINT ( 'NONE',  ( -22.12673812478050195, 1409.685743108969973, 209.8966867368829980 ) ) ;
#95863=CARTESIAN_POINT ( 'NONE',  ( -42.07525187489999752, 1455.849900366930115, 266.2935987290980506 ) ) ;
#95865=CARTESIAN_POINT ( 'NONE',  ( 0.1666873299777550110, 1420.332927348350040, 183.4666007823460063 ) ) ;
#95866=CARTESIAN_POINT ( 'NONE',  ( -28.08612064899999794, 1509.893849332430136, 216.7264453898779948 ) ) ;
#95869=CARTESIAN_POINT ( 'NONE',  ( 17.18900436376040020, 1422.349201594700162, 226.7290623181470153 ) ) ;
#95870=CARTESIAN_POINT ( 'NONE',  ( 13.02322702420000056, 1416.825784011830137, 221.6328457789979893 ) ) ;
#95871=CARTESIAN_POINT ( 'NONE',  ( 14.97303230589999856, 1485.053194597530137, 223.9694979347979711 ) ) ;
#95877=CARTESIAN_POINT ( 'NONE',  ( -9.767576865947649623, 1416.948096802409964, 202.3623712837820108 ) ) ;
#95878=EDGE_CURVE ( 'NONE', #33349, #90510, #53101, .T. ) ;
#95879=EDGE_CURVE ( 'NONE', #21200, #22768, #53472, .T. ) ;
#95880=CARTESIAN_POINT ( 'NONE',  ( 15.58852162090000171, 1416.217772597929979, 199.0820666858980132 ) ) ;
#95881=CARTESIAN_POINT ( 'NONE',  ( -12.78690713350000152, 1416.828040475229955, 195.5394874918979724 ) ) ;
#95883=ADVANCED_FACE ( 'NONE', ( #68886 ), #53734, .T. ) ;
#95884=CARTESIAN_POINT ( 'NONE',  ( 23.75354970140000432, 1410.237980908829968, 210.1586681567179937 ) ) ;
#95885=CARTESIAN_POINT ( 'NONE',  ( 3.908823033620000498, 1430.579202973829979, 185.0915024236979889 ) ) ;
#95888=CARTESIAN_POINT ( 'NONE',  ( -5.359920746595229879, 1422.532334412899900, 146.8567192038190115 ) ) ;
#95889=CARTESIAN_POINT ( 'NONE',  ( -11.77480480780000072, 1432.721983468549979, 150.8108403777980016 ) ) ;
#95890=LINE ( 'NONE', #95340, #73693 ) ;
#95891=CARTESIAN_POINT ( 'NONE',  ( 1.073626246609999724, 1413.031385993829872, 233.0405009011980155 ) ) ;
#95894=DIRECTION ( 'NONE',  ( 1.000000000000000000, 0.000000000000000000, 0.000000000000000000 ) ) ;
#95895=CARTESIAN_POINT ( 'NONE',  ( -1.018590187505569844, 1419.107239897679847, 184.9305502371729801 ) ) ;
#95898=CARTESIAN_POINT ( 'NONE',  ( -14.13418362532219952, 1485.258468063590044, 186.5543704135239977 ) ) ;
#95899=CARTESIAN_POINT ( 'NONE',  ( 2.370878939379999828, 1508.995853304430057, 237.7496061722980016 ) ) ;
#95901=CARTESIAN_POINT ( 'NONE',  ( 40.26396674155190425, 1444.186481489339940, 137.1012378630869932 ) ) ;
#95903=ORIENTED_EDGE ( 'NONE', *, *, #18621, .F. ) ;
#95905=CARTESIAN_POINT ( 'NONE',  ( 11.93812031068550006, 1433.479819799799998, 149.8964887876289822 ) ) ;
#95910=CARTESIAN_POINT ( 'NONE',  ( 18.23239277690950289, 1497.487356725759810, 188.8422295970860034 ) ) ;
#95911=CARTESIAN_POINT ( 'NONE',  ( -0.1670782863309999977, 1507.623008746229971, 180.8803229349979915 ) ) ;
#95913=EDGE_CURVE ( 'NONE', #84894, #25549, #11998, .T. ) ;
#95914=CARTESIAN_POINT ( 'NONE',  ( 0.1008259851559999976, 1507.644663146129915, 180.8662990920980178 ) ) ;
#95916=CARTESIAN_POINT ( 'NONE',  ( 16.31714699009999947, 1410.414996249630121, 226.6977280599979849 ) ) ;
#95919=CARTESIAN_POINT ( 'NONE',  ( 13.90692152919330127, 1415.348334734199852, 197.4141063975939971 ) ) ;
#95923=CARTESIAN_POINT ( 'NONE',  ( 14.13836065253160079, 1435.304170572160047, 149.4741414661730232 ) ) ;
#95927=EDGE_CURVE ( 'NONE', #54399, #54705, #93482, .T. ) ;
#95930=CARTESIAN_POINT ( 'NONE',  ( -0.3157389373359999474, 1466.373614209230027, 235.6705073726980117 ) ) ;
#95931=CARTESIAN_POINT ( 'NONE',  ( 7.943111102253434197, 1451.391306100884776, 152.9620345468942162 ) ) ;
#95939=CARTESIAN_POINT ( 'NONE',  ( 0.7447930487909999453, 1508.354245354229988, 237.7262685846980048 ) ) ;
#95943=CARTESIAN_POINT ( 'NONE',  ( 24.41278939130150150, 1440.913060387330006, 237.1198172069220220 ) ) ;
#95945=ORIENTED_EDGE ( 'NONE', *, *, #6296, .T. ) ;
#95947=CARTESIAN_POINT ( 'NONE',  ( -14.70848724120000028, 1409.928546724029957, 190.8190897573979896 ) ) ;
#95949=CARTESIAN_POINT ( 'NONE',  ( -24.23995371788353026, 1438.560025134897842, 212.1200462699911213 ) ) ;
#95951=CARTESIAN_POINT ( 'NONE',  ( 0.0003311604216102360292, 1396.810862911885124, 196.4330027040883238 ) ) ;
#95952=CARTESIAN_POINT ( 'NONE',  ( -12.59821692533909498, 1434.524816250457661, 147.2310560251989671 ) ) ;
#95955=CARTESIAN_POINT ( 'NONE',  ( -0.4537870827523895478, 1465.110980022260946, 238.1114895919644994 ) ) ;
#95961=CARTESIAN_POINT ( 'NONE',  ( -17.11714618750000128, 1443.086052842849995, 162.7561046190980107 ) ) ;
#95963=CARTESIAN_POINT ( 'NONE',  ( -21.20812184460000083, 1488.814055421829835, 209.5007742268749951 ) ) ;
#95964=CARTESIAN_POINT ( 'NONE',  ( -17.82472165217326321, 1486.162070320810017, 188.3324638760118717 ) ) ;
#95966=ORIENTED_EDGE ( 'NONE', *, *, #81590, .T. ) ;
#95967=CARTESIAN_POINT ( 'NONE',  ( -18.53418666356940037, 1507.620785846770104, 229.7143111648900060 ) ) ;
#95968=CARTESIAN_POINT ( 'NONE',  ( 27.39151915920000135, 1446.363612851640255, 231.9651322872979904 ) ) ;
#95971=CARTESIAN_POINT ( 'NONE',  ( -7.824074142530000664, 1507.599096865930051, 235.3676831994980034 ) ) ;
#95972=CARTESIAN_POINT ( 'NONE',  ( -18.93166004669999936, 1457.983850899830031, 226.9910905844980107 ) ) ;
#95973=EDGE_CURVE ( 'NONE', #25318, #27899, #80237, .T. ) ;
#95974=CARTESIAN_POINT ( 'NONE',  ( -20.37974553509161524, 1410.985820951756523, 198.9094803766706718 ) ) ;
#95975=CARTESIAN_POINT ( 'NONE',  ( 19.01929472089999962, 1456.664510428530093, 226.1307736208979975 ) ) ;
#95976=CARTESIAN_POINT ( 'NONE',  ( -0.08692450656670000497, 1452.817890303729882, 189.4446534707980163 ) ) ;
#95978=VERTEX_POINT ( 'NONE', #41734 ) ;
#95980=CARTESIAN_POINT ( 'NONE',  ( 0.1080863654920000139, 1405.716796065530161, 267.8540375961979407 ) ) ;
#95982=CARTESIAN_POINT ( 'NONE',  ( 42.60984463329660343, 1451.659711123250190, 270.2297449080399474 ) ) ;
#95983=CARTESIAN_POINT ( 'NONE',  ( 5.426920751279999955, 1436.492768174659886, 154.6973185947979914 ) ) ;
#95984=CARTESIAN_POINT ( 'NONE',  ( -40.35744760560000088, 1444.177753733350073, 137.0994330816980096 ) ) ;
#95985=CARTESIAN_POINT ( 'NONE',  ( -40.15144253337770408, 1440.913060403469899, 259.4983307252720124 ) ) ;
#95986=EDGE_CURVE ( 'NONE', #104164, #92476, #77448, .T. ) ;
#95987=CARTESIAN_POINT ( 'NONE',  ( -27.43419230599999992, 1448.208631761229981, 136.8608613106979988 ) ) ;
#95988=CARTESIAN_POINT ( 'NONE',  ( 1.536514403073885315, 1450.607110032781748, 154.2727822066727299 ) ) ;
#95990=CARTESIAN_POINT ( 'NONE',  ( -1.271867600325184311, 1450.975052772127356, 183.1634528063702305 ) ) ;
#95991=CARTESIAN_POINT ( 'NONE',  ( 25.31189446751989891, 1438.152406002519911, 138.1036420975650003 ) ) ;
#95992=FACE_OUTER_BOUND ( 'NONE', #800, .T. ) ;
#95993=ORIENTED_EDGE ( 'NONE', *, *, #7519, .T. ) ;
#95994=CARTESIAN_POINT ( 'NONE',  ( -38.34143788450000301, 1440.913060387330006, 265.6112250856980381 ) ) ;
#95995=CARTESIAN_POINT ( 'NONE',  ( -1.545976657695036005, 1450.600942636307991, 182.1937731406511034 ) ) ;
#95997=CARTESIAN_POINT ( 'NONE',  ( -0.7781779465670000118, 1476.071789383429859, 267.5369107683980019 ) ) ;
#96000=CARTESIAN_POINT ( 'NONE',  ( -3.885048638823741740, 1448.296104563261451, 185.0431407441832334 ) ) ;
#96003=CARTESIAN_POINT ( 'NONE',  ( -18.01569507700000017, 1415.245980409429876, 207.9371297658080096 ) ) ;
#96005=CARTESIAN_POINT ( 'NONE',  ( 26.08096834208760129, 1435.935456896660071, 136.5582649592650171 ) ) ;
#96006=ADVANCED_FACE ( 'NONE', ( #85374 ), #96627, .F. ) ;
#96007=CARTESIAN_POINT ( 'NONE',  ( -13.35899836846294875, 1443.328976958492376, 169.3723828192563587 ) ) ;
#96008=CARTESIAN_POINT ( 'NONE',  ( -16.16218761038539853, 1409.477383793439913, 225.2079466252519921 ) ) ;
#96013=CARTESIAN_POINT ( 'NONE',  ( 2.883409987159999854, 1409.181735908430028, 231.0710517162980011 ) ) ;
#96015=CARTESIAN_POINT ( 'NONE',  ( 26.57484134623869920, 1440.913038224569846, 213.0553080370949885 ) ) ;
#96017=CARTESIAN_POINT ( 'NONE',  ( -0.1613635714646410035, 1507.107001889669846, 180.9028745560509890 ) ) ;
#96018=CARTESIAN_POINT ( 'NONE',  ( 4.198017029517449927, 1424.053073258670111, 184.2502146191590100 ) ) ;
#96026=CARTESIAN_POINT ( 'NONE',  ( 2.476654626830000261, 1449.226390938449867, 182.5716736920980168 ) ) ;
#96028=EDGE_CURVE ( 'NONE', #22743, #59443, #19269, .T. ) ;
#96030=VERTEX_POINT ( 'NONE', #98748 ) ;
#96031=ORIENTED_EDGE ( 'NONE', *, *, #43271, .F. ) ;
#96033=CARTESIAN_POINT ( 'NONE',  ( 1.448807010176029975, 1499.064327800129831, 236.4215994981330198 ) ) ;
#96034=CARTESIAN_POINT ( 'NONE',  ( -1.566309006410000032E-09, 1473.264972808529819, 270.4290818598980195 ) ) ;
#96037=CARTESIAN_POINT ( 'NONE',  ( 24.02863916850529691, 1507.902931906480035, 195.9323055859989893 ) ) ;
#96039=CARTESIAN_POINT ( 'NONE',  ( 22.76038310810000098, 1410.633847097429907, 206.9447164962780334 ) ) ;
#96041=CARTESIAN_POINT ( 'NONE',  ( 33.91368447396819619, 1437.010588082029926, 136.5611905281099894 ) ) ;
#96042=CARTESIAN_POINT ( 'NONE',  ( 27.58305910952065432, 1435.460669043382723, 135.2629866813300623 ) ) ;
#96043=CARTESIAN_POINT ( 'NONE',  ( 3.137687880864949985, 1407.958752388860148, 195.9309462285740153 ) ) ;
#96044=CARTESIAN_POINT ( 'NONE',  ( -0.7722441410959061114, 1405.989132518979886, 266.9610481760290099 ) ) ;
#96045=CARTESIAN_POINT ( 'NONE',  ( 41.66021864449999867, 1443.875655612860101, 135.6929158170979974 ) ) ;
#96046=ORIENTED_EDGE ( 'NONE', *, *, #32935, .F. ) ;
#96048=CARTESIAN_POINT ( 'NONE',  ( 13.74650104269999851, 1441.983649238280123, 189.3366583681979876 ) ) ;
#96049=B_SPLINE_CURVE_WITH_KNOTS ( 'NONE', 3,
 ( #18444, #52643, #104684, #19566, #36925, #21749 ),
 .UNSPECIFIED., .F., .F.,
 ( 4, 2, 4 ),
 ( 0.002076474971749801314, 0.005958898312071419720, 0.009841321652393038993 ),
 .UNSPECIFIED. ) ;
#96050=ORIENTED_EDGE ( 'NONE', *, *, #102051, .F. ) ;
#96059=ORIENTED_EDGE ( 'NONE', *, *, #3506, .T. ) ;
#96062=CARTESIAN_POINT ( 'NONE',  ( 9.507369708760000648, 1414.971339025629959, 223.5168404978979879 ) ) ;
#96067=CARTESIAN_POINT ( 'NONE',  ( -4.474334996270000531, 1410.445275992929965, 232.0547894430980023 ) ) ;
#96068=CARTESIAN_POINT ( 'NONE',  ( -5.689439854299999766, 1447.123656070790048, 185.2293832585979771 ) ) ;
#96070=CARTESIAN_POINT ( 'NONE',  ( 11.86716023049999968, 1432.353341358199941, 147.6509521729980179 ) ) ;
#96071=CARTESIAN_POINT ( 'NONE',  ( -25.49263425876450029, 1440.913060497309971, 219.0479588355970009 ) ) ;
#96072=CARTESIAN_POINT ( 'NONE',  ( -2.793439186891359949, 1486.025328193850100, 182.0741020391329812 ) ) ;
#96073=CARTESIAN_POINT ( 'NONE',  ( 15.62937150409696940, 1506.527232284255660, 224.6916783686666008 ) ) ;
#96074=CARTESIAN_POINT ( 'NONE',  ( -25.57374439069999994, 1436.479224125469955, 137.1536659212979998 ) ) ;
#96078=CARTESIAN_POINT ( 'NONE',  ( -12.98226561589999939, 1414.913060387329779, 219.9156672276980089 ) ) ;
#96079=CARTESIAN_POINT ( 'NONE',  ( 19.23929248577682927, 1410.946498287256873, 195.7385929941525546 ) ) ;
#96081=ORIENTED_EDGE ( 'NONE', *, *, #74749, .F. ) ;
#96083=CARTESIAN_POINT ( 'NONE',  ( -4.407453029090000030, 1410.299935115230028, 232.0713108462980188 ) ) ;
#96088=CARTESIAN_POINT ( 'NONE',  ( 17.40247493689940228, 1469.008714942930055, 228.9206246928509927 ) ) ;
#96092=CARTESIAN_POINT ( 'NONE',  ( -13.95592190008845179, 1416.839570625314309, 221.9092780320571023 ) ) ;
#96095=CARTESIAN_POINT ( 'NONE',  ( -3.189739596009999456, 1421.552253087029840, 184.9104270198979805 ) ) ;
#96097=CARTESIAN_POINT ( 'NONE',  ( -11.03930834155172747, 1425.182627338753264, 139.1363278504886125 ) ) ;
#96102=CARTESIAN_POINT ( 'NONE',  ( -16.55737386589999716, 1499.713794654230014, 185.8142580502980081 ) ) ;
#96104=CARTESIAN_POINT ( 'NONE',  ( 3.104086163079999849, 1421.303663037730075, 184.6144243675980192 ) ) ;
#96105=CARTESIAN_POINT ( 'NONE',  ( 10.46157297396847952, 1435.041345384508304, 152.1695804010182655 ) ) ;
#96112=CARTESIAN_POINT ( 'NONE',  ( 17.74184486700000107, 1415.163755984130148, 210.1742778932080000 ) ) ;
#96113=CARTESIAN_POINT ( 'NONE',  ( -18.65358896220000062, 1425.523870256030023, 225.5826184276980086 ) ) ;
#96114=CARTESIAN_POINT ( 'NONE',  ( -14.51975326280000012, 1434.998496940630048, 148.5999626668979943 ) ) ;
#96116=CARTESIAN_POINT ( 'NONE',  ( -1.725662463192670248, 1484.236887848700007, 182.7463278875050037 ) ) ;
#96117=CARTESIAN_POINT ( 'NONE',  ( 1.159637561179999832, 1415.063410489729904, 191.5788536471979739 ) ) ;
#96119=CARTESIAN_POINT ( 'NONE',  ( 10.88722667122907239, 1426.866889159644870, 149.3503661776646538 ) ) ;
#96120=VERTEX_POINT ( 'NONE', #46727 ) ;
#96121=CARTESIAN_POINT ( 'NONE',  ( 15.27152964737910068, 1506.433683733550197, 193.3098315259690025 ) ) ;
#96122=CARTESIAN_POINT ( 'NONE',  ( 22.92154238690000057, 1411.040135702729913, 207.1380470637979840 ) ) ;
#96124=CARTESIAN_POINT ( 'NONE',  ( -11.90000415720300175, 1434.913060496859998, 147.6452464505769910 ) ) ;
#96128=CARTESIAN_POINT ( 'NONE',  ( 14.69722372230000040, 1408.913060387329779, 219.1592431274980299 ) ) ;
#96129=CARTESIAN_POINT ( 'NONE',  ( 19.02704169900689735, 1456.915441405320053, 225.6706379604710264 ) ) ;
#96137=CARTESIAN_POINT ( 'NONE',  ( 24.57377048660000085, 1509.773436695229975, 192.8657111338980030 ) ) ;
#96138=EDGE_LOOP ( 'NONE', ( #106716, #8575, #99886, #62429 ) ) ;
#96139=CARTESIAN_POINT ( 'NONE',  ( -18.35253423818827301, 1459.074742763881659, 227.7717061293672316 ) ) ;
#96141=EDGE_CURVE ( 'NONE', #93417, #52697, #86754, .T. ) ;
#96145=CARTESIAN_POINT ( 'NONE',  ( 18.23773974694429967, 1416.535698381769862, 209.2906403974349985 ) ) ;
#96147=CARTESIAN_POINT ( 'NONE',  ( 13.20333953265802585, 1443.120703127549177, 169.3908102670497442 ) ) ;
#96148=CARTESIAN_POINT ( 'NONE',  ( 21.21614429629999776, 1488.813684182329780, 208.8886841255019817 ) ) ;
#96149=CARTESIAN_POINT ( 'NONE',  ( -21.01922260210000104, 1472.811049260129948, 267.0603657249980074 ) ) ;
#96153=CARTESIAN_POINT ( 'NONE',  ( -11.72697064220000129, 1433.670490598739889, 150.9444907361979915 ) ) ;
#96156=CARTESIAN_POINT ( 'NONE',  ( -19.92213080605079867, 1499.851339543129825, 228.6477981121460061 ) ) ;
#96157=CARTESIAN_POINT ( 'NONE',  ( 8.147242326480000685, 1409.364186213629864, 188.2664186143980203 ) ) ;
#96158=CARTESIAN_POINT ( 'NONE',  ( 4.123035104040000398, 1421.670591005329925, 184.9173806230979835 ) ) ;
#96159=CARTESIAN_POINT ( 'NONE',  ( -10.43358988419999989, 1436.699218663759893, 152.2773048742980109 ) ) ;
#96160=CARTESIAN_POINT ( 'NONE',  ( 9.012266058079999809, 1437.710537269130100, 153.1651548905980178 ) ) ;
#96163=EDGE_CURVE ( 'NONE', #5297, #9014, #73499, .T. ) ;
#96170=CARTESIAN_POINT ( 'NONE',  ( -41.12099125829999480, 1454.819569115930108, 269.7572481037980197 ) ) ;
#96173=CARTESIAN_POINT ( 'NONE',  ( 17.64684481400000138, 1410.891992924130136, 223.6671000665980102 ) ) ;
#96176=CARTESIAN_POINT ( 'NONE',  ( 2.912741334778549795, 1409.643588917339912, 231.3796457533279920 ) ) ;
#96177=CARTESIAN_POINT ( 'NONE',  ( 1.456020689590000083, 1508.396344578629851, 237.4407949434980196 ) ) ;
#96178=CARTESIAN_POINT ( 'NONE',  ( -8.272300520779998223, 1417.569710766430035, 230.8453573205979978 ) ) ;
#96179=CARTESIAN_POINT ( 'NONE',  ( -1.082042371095176314, 1484.833744122492590, 182.1605000476520786 ) ) ;
#96181=CARTESIAN_POINT ( 'NONE',  ( -43.62459105522109581, 1430.012141993600153, 266.4825913953999930 ) ) ;
#96183=ORIENTED_EDGE ( 'NONE', *, *, #34944, .T. ) ;
#96190=CARTESIAN_POINT ( 'NONE',  ( 13.15366522099999891, 1428.703228679929907, 223.0784815109979888 ) ) ;
#96191=CARTESIAN_POINT ( 'NONE',  ( -16.64352143049999810, 1410.411353541330072, 191.7486415517980163 ) ) ;
#96194=CARTESIAN_POINT ( 'NONE',  ( -17.38483621660000011, 1410.884422118429939, 225.7833436061980024 ) ) ;
#96195=CARTESIAN_POINT ( 'NONE',  ( -14.45771159784271376, 1416.835807144213277, 221.3919539079676611 ) ) ;
#96203=CARTESIAN_POINT ( 'NONE',  ( -9.846959627583329322, 1409.027766033789931, 270.3779765466370577 ) ) ;
#96205=CARTESIAN_POINT ( 'NONE',  ( -1.580871945720000005, 1426.963505220229990, 133.6118001900980232 ) ) ;
#96210=CARTESIAN_POINT ( 'NONE',  ( 43.34298913515119978, 1451.640137698500439, 269.0390372527960494 ) ) ;
#96214=CARTESIAN_POINT ( 'NONE',  ( -0.004275337162772009994, 1408.915998917759907, 186.3744338923069961 ) ) ;
#96215=CARTESIAN_POINT ( 'NONE',  ( -18.17106232659159915, 1415.393085339859908, 207.5671356270640047 ) ) ;
#96216=CARTESIAN_POINT ( 'NONE',  ( -18.45191180620000182, 1425.817450471429993, 225.2353046319980194 ) ) ;
#96217=CARTESIAN_POINT ( 'NONE',  ( 5.256383990386860106, 1475.048120302939878, 269.6502184949890193 ) ) ;
#96219=CARTESIAN_POINT ( 'NONE',  ( -17.35007289223692695, 1422.602586090401246, 226.5892681115564642 ) ) ;
#96221=ORIENTED_EDGE ( 'NONE', *, *, #99936, .T. ) ;
#96223=CARTESIAN_POINT ( 'NONE',  ( 1.471676140451410042, 1484.933433129259811, 182.0806043343100100 ) ) ;
#96226=CARTESIAN_POINT ( 'NONE',  ( 25.51839591191980006, 1450.803344685250295, 137.1473335183449933 ) ) ;
#96227=LINE ( 'NONE', #27362, #109751 ) ;
#96230=CARTESIAN_POINT ( 'NONE',  ( 17.08762417599999850, 1409.674908758129959, 193.0190955581979892 ) ) ;
#96231=CARTESIAN_POINT ( 'NONE',  ( 20.82705473220000059, 1444.994950788469851, 176.6587301488980017 ) ) ;
#96232=DIRECTION ( 'NONE',  ( 0.000000000000000000, 1.000000000000000000, 0.000000000000000000 ) ) ;
#96234=CARTESIAN_POINT ( 'NONE',  ( -20.94045403861742827, 1428.001502734700580, 220.5823066705793565 ) ) ;
#96235=AXIS2_PLACEMENT_3D ( 'NONE', #105057, #34533, #78753 ) ;
#96236=CARTESIAN_POINT ( 'NONE',  ( 0.7101137637400629643, 1451.084754322919935, 182.2944934625020039 ) ) ;
#96240=CARTESIAN_POINT ( 'NONE',  ( 26.72687756924920066, 1447.183547681790060, 137.1848390478849922 ) ) ;
#96241=ORIENTED_EDGE ( 'NONE', *, *, #6203, .F. ) ;
#96246=CARTESIAN_POINT ( 'NONE',  ( -0.3676572738806710428, 1409.061418105000030, 232.3593742318309978 ) ) ;
#96250=CARTESIAN_POINT ( 'NONE',  ( -26.42714720800000094, 1443.942861155959918, 243.9198229428980085 ) ) ;
#96251=CARTESIAN_POINT ( 'NONE',  ( -2.395580532111799776, 1451.953014703720100, 184.6449581330110163 ) ) ;
#96252=CARTESIAN_POINT ( 'NONE',  ( 10.98083629090000102, 1433.016921068679949, 151.7694307944979926 ) ) ;
#96253=CARTESIAN_POINT ( 'NONE',  ( 9.061802757597490208E-06, 1475.058218891730121, 269.6445798169980321 ) ) ;
#96254=CARTESIAN_POINT ( 'NONE',  ( 27.35810488257520134, 1440.913060388870008, 228.4442125759339888 ) ) ;
#96255=CARTESIAN_POINT ( 'NONE',  ( -23.99877502900000081, 1508.007102827230256, 222.4169432911980095 ) ) ;
#96259=CARTESIAN_POINT ( 'NONE',  ( 22.91663120903140083, 1507.606285602550088, 210.6365840681099826 ) ) ;
#96260=CARTESIAN_POINT ( 'NONE',  ( -15.78519159560000062, 1486.362372667630098, 186.5259617109979899 ) ) ;
#96261=CARTESIAN_POINT ( 'NONE',  ( 4.200862373802610072, 1398.037452366075058, 196.7985206626544539 ) ) ;
#96262=CARTESIAN_POINT ( 'NONE',  ( 2.133183460910000218, 1482.812097613729975, 235.0898365658979969 ) ) ;
#96264=CARTESIAN_POINT ( 'NONE',  ( 24.55148953060000139, 1430.358502415830117, 211.1312658929579982 ) ) ;
#96266=CARTESIAN_POINT ( 'NONE',  ( -10.82593705289999875, 1509.291110439329941, 235.9458924929979844 ) ) ;
#96269=CARTESIAN_POINT ( 'NONE',  ( 6.232532001850000114, 1407.162969929529936, 220.5304192662980256 ) ) ;
#96270=CARTESIAN_POINT ( 'NONE',  ( -27.01473127741192570, 1509.856435591600302, 196.9755962829802343 ) ) ;
#96271=CARTESIAN_POINT ( 'NONE',  ( 0.1605139477524830105, 1485.957458676359920, 181.8384362477690104 ) ) ;
#96273=ORIENTED_EDGE ( 'NONE', *, *, #50285, .F. ) ;
#96274=CARTESIAN_POINT ( 'NONE',  ( -20.12133088869999753, 1445.052233488290085, 161.1306464489979930 ) ) ;
#96276=EDGE_CURVE ( 'NONE', #74738, #96843, #109575, .T. ) ;
#96278=CARTESIAN_POINT ( 'NONE',  ( -36.33941889825980809, 1451.266910394130036, 134.0999999986779869 ) ) ;
#96279=ORIENTED_EDGE ( 'NONE', *, *, #88850, .F. ) ;
#96285=DIRECTION ( 'NONE',  ( -0.09978697244513583253, 0.9945729288003561930, -0.02944909892875140905 ) ) ;
#96288=CARTESIAN_POINT ( 'NONE',  ( 10.72705856214020059, 1409.287657520459788, 219.5401174626420016 ) ) ;
#96291=CARTESIAN_POINT ( 'NONE',  ( -17.71575766480000169, 1417.732977527630055, 192.4301206783980263 ) ) ;
#96297=ORIENTED_EDGE ( 'NONE', *, *, #4232, .T. ) ;
#96299=CARTESIAN_POINT ( 'NONE',  ( -12.08615242673420020, 1415.948038442749976, 194.8431646156840031 ) ) ;
#96301=CARTESIAN_POINT ( 'NONE',  ( -11.77299894129999913, 1433.946611324799960, 151.0520174426980020 ) ) ;
#96303=CARTESIAN_POINT ( 'NONE',  ( 2.753149778868899666, 1471.436294210167489, 269.3346708043688409 ) ) ;
#96305=CARTESIAN_POINT ( 'NONE',  ( 2.562074494179999995, 1397.677066227130126, 221.9695021218980173 ) ) ;
#96307=CARTESIAN_POINT ( 'NONE',  ( -0.8670487806669999742, 1452.172290198730025, 183.4042211072979853 ) ) ;
#96309=CARTESIAN_POINT ( 'NONE',  ( -25.41904847911940735, 1436.620868978935960, 137.2922833411249144 ) ) ;
#96311=AXIS2_PLACEMENT_3D ( 'NONE', #50060, #103182, #42751 ) ;
#96312=CARTESIAN_POINT ( 'NONE',  ( -13.01880433582340046, 1435.354293861170163, 150.4303184084199927 ) ) ;
#96313=CARTESIAN_POINT ( 'NONE',  ( 21.13431379670319998, 1409.651086887829933, 206.4149708788170301 ) ) ;
#96314=DIRECTION ( 'NONE',  ( 1.000000000000000000, 0.000000000000000000, -0.000000000000000000 ) ) ;
#96317=CARTESIAN_POINT ( 'NONE',  ( 41.65274031657839515, 1444.011424526299834, 135.7904737122629797 ) ) ;
#96320=CARTESIAN_POINT ( 'NONE',  ( 35.25149216619999493, 1420.828141007130171, 264.2529782732980266 ) ) ;
#96321=CARTESIAN_POINT ( 'NONE',  ( -26.83695571260000179, 1488.686901730929776, 205.9593982892680231 ) ) ;
#96322=CARTESIAN_POINT ( 'NONE',  ( -10.71072610778340106, 1425.695308460959950, 95.13476052875000732 ) ) ;
#96323=CARTESIAN_POINT ( 'NONE',  ( 13.22475641109999955, 1415.063410489729904, 197.5370647170979623 ) ) ;
#96325=EDGE_CURVE ( 'NONE', #100339, #86845, #108547, .T. ) ;
#96326=DIRECTION ( 'NONE',  ( 2.473221764039894783E-17, 0.000000000000000000, 1.000000000000000000 ) ) ;
#96327=CARTESIAN_POINT ( 'NONE',  ( -10.82132307030000007, 1413.960774651630118, 250.5360043753979653 ) ) ;
#96329=CARTESIAN_POINT ( 'NONE',  ( 29.27865644803159739, 1509.812245387229950, 209.6041006200670154 ) ) ;
#96330=CARTESIAN_POINT ( 'NONE',  ( 2.684965486993618811, 1448.122735116655349, 154.7390415180112200 ) ) ;
#96331=DIRECTION ( 'NONE',  ( -0.7071067576156506718, 3.866377236683057960E-11, 0.7071068047574436966 ) ) ;
#96333=CARTESIAN_POINT ( 'NONE',  ( -1.546949757679999760, 1416.828040475729949, 228.0209010782980101 ) ) ;
#96335=CARTESIAN_POINT ( 'NONE',  ( 14.31461351079999922, 1509.452791170529963, 235.1998141392979846 ) ) ;
#96336=ORIENTED_EDGE ( 'NONE', *, *, #109314, .T. ) ;
#96338=CARTESIAN_POINT ( 'NONE',  ( -2.424063131930000115, 1427.257651041929876, 147.9020499575979954 ) ) ;
#96339=CARTESIAN_POINT ( 'NONE',  ( -3.149355042448929609, 1421.363409048820131, 147.6430095841799925 ) ) ;
#96340=ORIENTED_EDGE ( 'NONE', *, *, #48707, .F. ) ;
#96341=CARTESIAN_POINT ( 'NONE',  ( -0.1629132599120000080, 1424.309591313030069, 227.6950206218980099 ) ) ;
#96342=AXIS2_PLACEMENT_3D ( 'NONE', #23332, #30079, #22760 ) ;
#96343=CARTESIAN_POINT ( 'NONE',  ( 7.735000377495650170, 1446.700284064708057, 154.1094615265521384 ) ) ;
#96345=B_SPLINE_CURVE_WITH_KNOTS ( 'NONE', 3,
 ( #89356, #81487, #96097, #2624 ),
 .UNSPECIFIED., .F., .F.,
 ( 4, 4 ),
 ( 0.0004474573906021131627, 0.001555588287050983787 ),
 .UNSPECIFIED. ) ;
#96346=CARTESIAN_POINT ( 'NONE',  ( -2.338091437230000125, 1489.062396073530181, 236.1656132279979943 ) ) ;
#96348=DIRECTION ( 'NONE',  ( 0.9955685427536684617, -0.04363816682463440150, -0.08330058268416962175 ) ) ;
#96350=CARTESIAN_POINT ( 'NONE',  ( 0.07204350251990000731, 1420.438792470029966, 183.3235075831980225 ) ) ;
#96351=ORIENTED_EDGE ( 'NONE', *, *, #73055, .T. ) ;
#96354=VERTEX_POINT ( 'NONE', #70160 ) ;
#96355=CARTESIAN_POINT ( 'NONE',  ( 11.86000693848920129, 1431.910640742250052, 149.9657772557100088 ) ) ;
#96356=DIRECTION ( 'NONE',  ( 0.3363363969979655810, -0.9417419115949056119, 0.000000000000000000 ) ) ;
#96362=CARTESIAN_POINT ( 'NONE',  ( -1.514738108749209999, 1507.606285622480073, 232.0384771855580084 ) ) ;
#96363=CARTESIAN_POINT ( 'NONE',  ( 0.9912764913912639475, 1407.655978583209844, 270.1376065755259788 ) ) ;
#96372=CARTESIAN_POINT ( 'NONE',  ( 17.67562304467840306, 1413.141888578579938, 224.8738151114190202 ) ) ;
#96375=CARTESIAN_POINT ( 'NONE',  ( 29.75208676439999778, 1419.160608152629948, 268.3665355202980436 ) ) ;
#96377=CARTESIAN_POINT ( 'NONE',  ( 19.75084982879439721, 1455.504334177440114, 226.5702129464319796 ) ) ;
#96379=B_SPLINE_SURFACE_WITH_KNOTS ( 'NONE', 5, 4, ( 
 ( #63104, #19376, #71506, #104505, #44615 ),
 ( #9347, #27800, #88263, #9889, #11004 ),
 ( #35090, #61429, #44057, #95553, #105063 ),
 ( #11556, #26681, #45176, #96102, #69272 ),
 ( #78197, #97201, #95006, #28352, #1509 ),
 ( #45733, #18274, #79317, #79869, #103950 ) ),
 .UNSPECIFIED., .F., .F., .F.,
 ( 6, 6 ),
 ( 5, 5 ),
 ( -1.065814103640000080E-14, 23.05527389429999729 ),
 ( 130.1608902480000154, 151.7353186150000113 ),
 .UNSPECIFIED. ) ;
#96384=ORIENTED_EDGE ( 'NONE', *, *, #59616, .F. ) ;
#96387=CARTESIAN_POINT ( 'NONE',  ( -24.75614383750000158, 1444.003657534250124, 210.7102618898479705 ) ) ;
#96389=CARTESIAN_POINT ( 'NONE',  ( -2.299601840677758968, 1449.771133279514743, 154.4058190498332976 ) ) ;
#96392=CARTESIAN_POINT ( 'NONE',  ( -10.44063514870000020, 1441.240651982340069, 187.1052350852980055 ) ) ;
#96393=CARTESIAN_POINT ( 'NONE',  ( 13.23644882699999847, 1509.506897669330101, 180.9128671145980150 ) ) ;
#96396=CARTESIAN_POINT ( 'NONE',  ( -0.9746356023110001043, 1408.913060387329779, 227.8345159065979715 ) ) ;
#96397=CARTESIAN_POINT ( 'NONE',  ( 11.29156966579999910, 1417.418038064730126, 229.6347434530979967 ) ) ;
#96399=CARTESIAN_POINT ( 'NONE',  ( -16.13220469984199923, 1459.078176189990018, 230.3616190125399896 ) ) ;
#96401=CARTESIAN_POINT ( 'NONE',  ( 39.60334749029999557, 1422.313230794130277, 267.8221855244979679 ) ) ;
#96403=CARTESIAN_POINT ( 'NONE',  ( 20.70415920599999637, 1436.034498798209825, 144.5456087543980175 ) ) ;
#96405=CARTESIAN_POINT ( 'NONE',  ( 26.29659629110000196, 1508.005140778730038, 202.4501866991980137 ) ) ;
#96406=CARTESIAN_POINT ( 'NONE',  ( 5.359760538142340103, 1422.219520672319959, 145.5218257772459935 ) ) ;
#96409=CARTESIAN_POINT ( 'NONE',  ( 12.45665488799999920, 1416.827520120730014, 223.4764148226980183 ) ) ;
#96411=CARTESIAN_POINT ( 'NONE',  ( -39.99259053121770080, 1438.670161830759753, 135.1922219426939762 ) ) ;
#96412=CARTESIAN_POINT ( 'NONE',  ( -13.55937006006110046, 1409.552480571150227, 226.6517346244539794 ) ) ;
#96413=CARTESIAN_POINT ( 'NONE',  ( -17.66282533229999885, 1415.426091369230107, 205.3741255001079935 ) ) ;
#96414=CARTESIAN_POINT ( 'NONE',  ( -12.33746580920000113, 1440.929426004120160, 187.9427475994980057 ) ) ;
#96416=CARTESIAN_POINT ( 'NONE',  ( -33.15526401089999808, 1436.131197805709917, 136.3224491675979948 ) ) ;
#96420=CARTESIAN_POINT ( 'NONE',  ( -7.298806753422620197, 1409.167940335549929, 222.1915275659999907 ) ) ;
#96421=DIRECTION ( 'NONE',  ( 0.000000000000000000, -1.000000000000000000, 0.000000000000000000 ) ) ;
#96422=CARTESIAN_POINT ( 'NONE',  ( -2.745154014197499937, 1419.769956470485113, 137.0999999980979851 ) ) ;
#96423=CARTESIAN_POINT ( 'NONE',  ( -46.05258988370000139, 1440.913037442780023, 266.6770556630980309 ) ) ;
#96424=CARTESIAN_POINT ( 'NONE',  ( -16.09266893903710383, 1469.459467177870010, 223.0552979758230094 ) ) ;
#96426=CARTESIAN_POINT ( 'NONE',  ( 0.2286803964500180031, 1420.490562101879959, 182.9054483574730057 ) ) ;
#96430=CARTESIAN_POINT ( 'NONE',  ( 17.10099828737380179, 1423.827771296450010, 227.6321784446419940 ) ) ;
#96431=FACE_OUTER_BOUND ( 'NONE', #67007, .T. ) ;
#96432=CARTESIAN_POINT ( 'NONE',  ( 15.25592359020000011, 1495.928552999029989, 224.4451643109979955 ) ) ;
#96433=CARTESIAN_POINT ( 'NONE',  ( -26.29993148601639774, 1495.365167192059971, 212.0160643654880062 ) ) ;
#96434=EDGE_CURVE ( 'NONE', #24399, #38170, #58801, .T. ) ;
#96438=CARTESIAN_POINT ( 'NONE',  ( 13.95470622120000037, 1415.426952350729835, 197.1288800259980292 ) ) ;
#96439=CARTESIAN_POINT ( 'NONE',  ( -12.71684466930000035, 1416.535385209229844, 195.1197337799980005 ) ) ;
#96442=CARTESIAN_POINT ( 'NONE',  ( 23.42036295790000366, 1410.652421255329955, 212.1072478527780163 ) ) ;
#96443=CARTESIAN_POINT ( 'NONE',  ( 13.89554995500000167, 1452.733480491630189, 223.3956528723979886 ) ) ;
#96445=CARTESIAN_POINT ( 'NONE',  ( -5.374474455745339441, 1429.012600464609932, 154.0236767292889795 ) ) ;
#96446=CARTESIAN_POINT ( 'NONE',  ( -11.58007427770000142, 1432.582736770090150, 151.1961013139979855 ) ) ;
#96449=CARTESIAN_POINT ( 'NONE',  ( 0.3744602044770000138, 1467.547738470929971, 229.3988225936980143 ) ) ;
#96455=CARTESIAN_POINT ( 'NONE',  ( -15.64556917516660128, 1486.082452306300183, 186.7299835657600227 ) ) ;
#96458=CARTESIAN_POINT ( 'NONE',  ( -4.272053644645270154, 1441.099711618939864, 157.6237339584640154 ) ) ;
#96461=VERTEX_POINT ( 'NONE', #79639 ) ;
#96462=CARTESIAN_POINT ( 'NONE',  ( 27.80989915279999991, 1508.614438783829883, 211.9044001959479999 ) ) ;
#96463=ORIENTED_EDGE ( 'NONE', *, *, #3499, .F. ) ;
#96466=CARTESIAN_POINT ( 'NONE',  ( 15.89484604643729959, 1418.061013547770017, 191.2943550237069985 ) ) ;
#96468=CARTESIAN_POINT ( 'NONE',  ( 12.00000000000000000, 1443.913060387330006, 147.5878346084980137 ) ) ;
#96470=CARTESIAN_POINT ( 'NONE',  ( -24.64113440033070290, 1451.811919332890056, 137.3348792521310031 ) ) ;
#96472=CARTESIAN_POINT ( 'NONE',  ( 11.37232255049999807, 1409.477095359130089, 228.6758770766980149 ) ) ;
#96474=CARTESIAN_POINT ( 'NONE',  ( 40.11569180289929903, 1438.966375984099841, 134.0999999981379744 ) ) ;
#96476=CARTESIAN_POINT ( 'NONE',  ( -10603.70820142147204, 2837.742859910728839, -4739.672918702562129 ) ) ;
#96481=VERTEX_POINT ( 'NONE', #2942 ) ;
#96483=CARTESIAN_POINT ( 'NONE',  ( 12.80760530667942199, 1444.977579513412593, 169.4484619471895712 ) ) ;
#96484=CARTESIAN_POINT ( 'NONE',  ( -2.779180994119999859, 1465.191645338429907, 235.7831128362979882 ) ) ;
#96485=CARTESIAN_POINT ( 'NONE',  ( 21.81318580550076192, 1450.920854193619562, 143.4612878731137755 ) ) ;
#96488=AXIS2_PLACEMENT_3D ( 'NONE', #84673, #85783, #59503 ) ;
#96492=( BOUNDED_CURVE ( )  B_SPLINE_CURVE ( 3, ( #65437, #75491, #83313, #108516 ),
 .UNSPECIFIED., .F., .F. ) 
 B_SPLINE_CURVE_WITH_KNOTS ( ( 4, 4 ),
 ( 1.092045427080897246, 2.049540592268306316 ),
 .UNSPECIFIED. ) 
 CURVE ( )  GEOMETRIC_REPRESENTATION_ITEM ( )  RATIONAL_B_SPLINE_CURVE ( ( 1.000000000000000000, 0.9250483781718910059, 0.9250483781718910059, 1.000000000000000000 ) ) 
 REPRESENTATION_ITEM ( '' )  );
#96493=CARTESIAN_POINT ( 'NONE',  ( 0.3248775019619999926, 1507.888195423030083, 237.5163462374979702 ) ) ;
#96497=CARTESIAN_POINT ( 'NONE',  ( 24.88822351442950165, 1440.913060387330006, 238.7353654863360077 ) ) ;
#96500=CARTESIAN_POINT ( 'NONE',  ( 26.03221818079370209, 1448.976886533850120, 137.1487683874059940 ) ) ;
#96501=CARTESIAN_POINT ( 'NONE',  ( -13.70448594279999988, 1409.558350370729841, 190.6766190893979740 ) ) ;
#96503=CARTESIAN_POINT ( 'NONE',  ( -24.35991799298464855, 1439.691670408465825, 212.0269959679101817 ) ) ;
#96505=CARTESIAN_POINT ( 'NONE',  ( -11.03427950878080210, 1414.913526845469960, 195.9671336867000093 ) ) ;
#96506=CARTESIAN_POINT ( 'NONE',  ( 0.0002639953367722339020, 1396.486682381765377, 196.7203582614270658 ) ) ;
#96507=CARTESIAN_POINT ( 'NONE',  ( -12.92957505356057268, 1434.745003379313857, 147.0228562061483615 ) ) ;
#96508=CARTESIAN_POINT ( 'NONE',  ( -12.40397477760000022, 1434.420140970890088, 149.9806264060980254 ) ) ;
#96510=CARTESIAN_POINT ( 'NONE',  ( -0.6774325393469999845, 1465.095555782530027, 238.0673157071979915 ) ) ;
#96512=B_SPLINE_SURFACE_WITH_KNOTS ( 'NONE', 5, 5, ( 
 ( #19894, #45135, #69788, #86003, #54097, #52425, #88225, #86552, #71465 ),
 ( #17664, #51865, #96062, #69225, #36162, #103336, #53534, #60835, #2030 ),
 ( #44016, #70347, #1460, #35597, #87109, #87678, #44568, #78714, #10963 ),
 ( #89865, #82005, #4753, #5310, #31056, #89316, #13134, #72006, #47868 ),
 ( #20987, #12612, #4220, #97165, #37820, #46245, #107218, #20436, #106122 ),
 ( #64696, #72530, #30506, #56272, #98814, #80375, #97716, #65237, #29396 ) ),
 .UNSPECIFIED., .F., .F., .F.,
 ( 6, 6 ),
 ( 6, 3, 6 ),
 ( 25.26541776610000056, 42.22156255719999507 ),
 ( -1.734723475979999901E-18, 1.000000000000000000, 2.000000000000000000 ),
 .UNSPECIFIED. ) ;
#96523=ORIENTED_EDGE ( 'NONE', *, *, #34948, .T. ) ;
#96524=CARTESIAN_POINT ( 'NONE',  ( -0.5624690339869999889, 1416.828040475229955, 227.7677324846980014 ) ) ;
#96526=CARTESIAN_POINT ( 'NONE',  ( 9.325404908590000375, 1464.388850156630042, 238.2842644183980099 ) ) ;
#96527=EDGE_CURVE ( 'NONE', #74353, #45174, #5243, .T. ) ;
#96531=CARTESIAN_POINT ( 'NONE',  ( 2.192264041240000072, 1411.750906532329964, 231.9235146910980063 ) ) ;
#96532=CARTESIAN_POINT ( 'NONE',  ( -18.61729373430000223, 1457.059787195529907, 228.1786572008979874 ) ) ;
#96533=CARTESIAN_POINT ( 'NONE',  ( -23.33460350828938346, 1411.088256419169738, 205.7888481793357585 ) ) ;
#96534=CARTESIAN_POINT ( 'NONE',  ( 5.359824864149300261, 1422.430743802070083, 146.5258976672799918 ) ) ;
#96539=CARTESIAN_POINT ( 'NONE',  ( 0.7785906040469999789, 1405.721630737029955, 267.8537809838979911 ) ) ;
#96541=CARTESIAN_POINT ( 'NONE',  ( 40.68248255500660093, 1450.744721969779903, 269.6225847687520059 ) ) ;
#96542=CARTESIAN_POINT ( 'NONE',  ( 2.478110446250000098, 1439.827425895250144, 157.7784414222979876 ) ) ;
#96544=CARTESIAN_POINT ( 'NONE',  ( -27.42679497377470099, 1448.207341916110181, 136.8613450941129770 ) ) ;
#96545=CARTESIAN_POINT ( 'NONE',  ( -43.31543451723249660, 1440.913060408729962, 263.5607854574880093 ) ) ;
#96546=AXIS2_PLACEMENT_3D ( 'NONE', #67984, #92052, #22601 ) ;
#96547=CARTESIAN_POINT ( 'NONE',  ( -25.89815699820000106, 1448.079688286479950, 137.6494510301980085 ) ) ;
#96548=CARTESIAN_POINT ( 'NONE',  ( 2.366976281752488198, 1449.615526741430131, 154.4348212163478706 ) ) ;
#96549=DIRECTION ( 'NONE',  ( 0.000000000000000000, 0.9989884989440152019, -0.04496642055560280682 ) ) ;
#96555=ORIENTED_EDGE ( 'NONE', *, *, #93352, .F. ) ;
#96557=CARTESIAN_POINT ( 'NONE',  ( 0.4274149980285910089, 1409.096032488900164, 185.6227922226819942 ) ) ;
#96560=CARTESIAN_POINT ( 'NONE',  ( -0.1075335950709999933, 1475.759805456229969, 269.0456997844980265 ) ) ;
#96561=CARTESIAN_POINT ( 'NONE',  ( -27.52167012590000184, 1451.951932214330100, 134.9033768147980084 ) ) ;
#96562=CARTESIAN_POINT ( 'NONE',  ( -28.56957206459999909, 1509.608813672329916, 210.5224072855680220 ) ) ;
#96563=CARTESIAN_POINT ( 'NONE',  ( -3.507940209892664196, 1448.288539702621165, 184.8766609435331532 ) ) ;
#96565=VECTOR ( 'NONE', #24106, 1000.000000000000000 ) ;
#96566=CARTESIAN_POINT ( 'NONE',  ( -18.94857910520000033, 1416.535385209630022, 207.9974517727780210 ) ) ;
#96568=CARTESIAN_POINT ( 'NONE',  ( 26.15004714006070330, 1436.377686502539973, 136.8027247401129785 ) ) ;
#96569=CARTESIAN_POINT ( 'NONE',  ( -10.32233395612670002, 1396.273524232049795, 213.1164902434229873 ) ) ;
#96570=CARTESIAN_POINT ( 'NONE',  ( -15.03569022279999956, 1422.461937768830012, 228.7610668756979919 ) ) ;
#96571=CARTESIAN_POINT ( 'NONE',  ( -16.65433881542789862, 1409.742294580739781, 225.7750875776860369 ) ) ;
#96572=CARTESIAN_POINT ( 'NONE',  ( 22.52609212299890018, 1509.699688857919909, 227.3081665486540146 ) ) ;
#96573=ORIENTED_EDGE ( 'NONE', *, *, #91097, .T. ) ;
#96574=ADVANCED_FACE ( 'NONE', ( #80170 ), #82394, .T. ) ;
#96578=CARTESIAN_POINT ( 'NONE',  ( 11.41497667239999991, 1426.868608979929832, 121.0051946870979975 ) ) ;
#96586=CARTESIAN_POINT ( 'NONE',  ( 2.343685733500000090, 1507.684322289930151, 181.2031450514980122 ) ) ;
#96592=ORIENTED_EDGE ( 'NONE', *, *, #28400, .F. ) ;
#96594=CARTESIAN_POINT ( 'NONE',  ( -41.14953178369999875, 1443.861422506349982, 136.9341304683979956 ) ) ;
#96595=CARTESIAN_POINT ( 'NONE',  ( 1.173613536004610047, 1490.965225197780001, 236.3431785357499848 ) ) ;
#96599=CARTESIAN_POINT ( 'NONE',  ( -2.762672730830000312, 1485.977692311530063, 182.1582024225980092 ) ) ;
#96600=AXIS2_PLACEMENT_3D ( 'NONE', #69070, #27049, #15843 ) ;
#96603=FACE_OUTER_BOUND ( 'NONE', #69467, .T. ) ;
#96605=CARTESIAN_POINT ( 'NONE',  ( 8.233125739818301980, 1396.200567475059870, 216.4997438228709825 ) ) ;
#96606=CARTESIAN_POINT ( 'NONE',  ( 3.387628330345790140, 1408.970309133350156, 194.7468131480869999 ) ) ;
#96607=CARTESIAN_POINT ( 'NONE',  ( 5.344396406567219923E-05, 1406.506757891989992, 269.4987579911870057 ) ) ;
#96608=CARTESIAN_POINT ( 'NONE',  ( 40.70526341139999715, 1444.199266155760142, 137.0833901977979963 ) ) ;
#96609=VERTEX_POINT ( 'NONE', #76723 ) ;
#96610=CARTESIAN_POINT ( 'NONE',  ( -11.57581721210000048, 1432.288378091340064, 151.1967356772979940 ) ) ;
#96611=CARTESIAN_POINT ( 'NONE',  ( 13.12363690099999936, 1441.384603101129869, 188.9419487780980091 ) ) ;
#96620=ORIENTED_EDGE ( 'NONE', *, *, #85617, .F. ) ;
#96627=B_SPLINE_SURFACE_WITH_KNOTS ( 'NONE', 5, 5, ( 
 ( #24366, #859, #34986, #50158, #33317, #67513 ),
 ( #94327, #50690, #83735, #101615, #76439, #25462 ),
 ( #33878, #92137, #34440, #17605, #59110, #15412 ),
 ( #49603, #84821, #110592, #59657, #93765, #17043 ),
 ( #8668, #102717, #60208, #11456, #88717, #28246 ),
 ( #53471, #71949, #62436, #20377, #2527, #18174 ),
 ( #35537, #45632, #96562, #11997, #106061, #71399 ),
 ( #9786, #46181, #95454, #37757, #79771, #3078 ),
 ( #19834, #54039, #60776, #104956, #1970, #27150 ) ),
 .UNSPECIFIED., .F., .F., .F.,
 ( 6, 3, 6 ),
 ( 6, 6 ),
 ( 1.123321935180000120, 3.227816461920000268, 6.189575054660000575 ),
 ( 0.000000000000000000, 2.000000000000000000 ),
 .UNSPECIFIED. ) ;
#96630=CARTESIAN_POINT ( 'NONE',  ( -8.142670621130001507, 1409.364027242329939, 229.9797211375979771 ) ) ;
#96632=CARTESIAN_POINT ( 'NONE',  ( -5.691423665590000347, 1446.578623823169892, 184.8819865835980067 ) ) ;
#96635=CARTESIAN_POINT ( 'NONE',  ( 11.36600848118518137, 1425.633665734278793, 139.1352670123650341 ) ) ;
#96638=EDGE_CURVE ( 'NONE', #101763, #101515, #84566, .T. ) ;
#96639=CARTESIAN_POINT ( 'NONE',  ( 41.44433335099289195, 1427.311881607490022, 269.9656476501689326 ) ) ;
#96643=CARTESIAN_POINT ( 'NONE',  ( 0.006933964948642189902, 1508.593138409394896, 238.1018653665563534 ) ) ;
#96645=CARTESIAN_POINT ( 'NONE',  ( 20.88760228492832027, 1411.001959330801583, 199.6026542048159627 ) ) ;
#96649=CARTESIAN_POINT ( 'NONE',  ( 3.203789175851970288E-09, 1424.294192408320214, 227.6053815985079893 ) ) ;
#96650=CARTESIAN_POINT ( 'NONE',  ( -4.152492679409998999, 1417.909732061129944, 232.5032652226979906 ) ) ;
#96652=EDGE_CURVE ( 'NONE', #10270, #91917, #4794, .T. ) ;
#96656=CARTESIAN_POINT ( 'NONE',  ( 16.98147855194190470, 1478.708851325969817, 229.6812432133669972 ) ) ;
#96657=CARTESIAN_POINT ( 'NONE',  ( 20.06869819519999965, 1507.849569125829930, 189.2236336047979819 ) ) ;
#96658=CARTESIAN_POINT ( 'NONE',  ( -14.88313348660000024, 1507.493288264930015, 229.7103749383979903 ) ) ;
#96659=CARTESIAN_POINT ( 'NONE',  ( -0.5238577372009999289, 1409.870336964829903, 233.1507187614980126 ) ) ;
#96660=LINE ( 'NONE', #105055, #18246 ) ;
#96664=CARTESIAN_POINT ( 'NONE',  ( 19.11260941699999805, 1509.007777225030168, 188.0781932532979965 ) ) ;
#96668=CARTESIAN_POINT ( 'NONE',  ( -7.105427357599999217E-15, 1418.913060387330006, 172.2701767054979882 ) ) ;
#96670=CARTESIAN_POINT ( 'NONE',  ( 11.60004869885204570, 1426.698742054508330, 134.5125446557153168 ) ) ;
#96672=CARTESIAN_POINT ( 'NONE',  ( -4.155669664704369382, 1439.704322410719897, 185.4969487652249995 ) ) ;
#96673=CARTESIAN_POINT ( 'NONE',  ( 19.00254649709379606, 1416.818673806565812, 210.3102538504050472 ) ) ;
#96678=CARTESIAN_POINT ( 'NONE',  ( 18.45314936670000350, 1415.553739809529816, 210.3484166225879903 ) ) ;
#96679=CARTESIAN_POINT ( 'NONE',  ( -18.47206917109999935, 1424.236406309129961, 225.0732636529979800 ) ) ;
#96680=CARTESIAN_POINT ( 'NONE',  ( -20.86574809109999862, 1435.370602116739974, 143.5212114325979940 ) ) ;
#96687=ORIENTED_EDGE ( 'NONE', *, *, #7202, .T. ) ;
#96689=CARTESIAN_POINT ( 'NONE',  ( 22.57618181349999986, 1411.056460407229906, 206.4508663819080141 ) ) ;
#96691=CARTESIAN_POINT ( 'NONE',  ( -11.92876424382160039, 1433.442611883628388, 149.9100498133672943 ) ) ;
#96693=CARTESIAN_POINT ( 'NONE',  ( -18.61766197840000103, 1509.563203468529991, 231.0956455985979972 ) ) ;
#96695=CARTESIAN_POINT ( 'NONE',  ( 15.96958168569999970, 1519.913060387329779, 225.0914276473980067 ) ) ;
#96698=ADVANCED_FACE ( 'NONE', ( #70017 ), #43681, .T. ) ;
#96705=LINE ( 'NONE', #54170, #4971 ) ;
#96706=ORIENTED_EDGE ( 'NONE', *, *, #22928, .F. ) ;
#96709=CARTESIAN_POINT ( 'NONE',  ( -0.7603233172752421609, 1417.366985054399720, 235.2447777849411636 ) ) ;
#96710=ORIENTED_EDGE ( 'NONE', *, *, #95406, .T. ) ;
#96714=CARTESIAN_POINT ( 'NONE',  ( 13.25931364579099814, 1443.184772872878057, 169.3835527203846425 ) ) ;
#96715=CARTESIAN_POINT ( 'NONE',  ( 28.87453514628182205, 1418.771342272429820, 269.4592184128185863 ) ) ;
#96716=CARTESIAN_POINT ( 'NONE',  ( -7.132053279490000008, 1475.995192518030080, 267.2558860548979851 ) ) ;
#96719=CARTESIAN_POINT ( 'NONE',  ( -19.16475049499999983, 1485.565701775930165, 189.6829647518980266 ) ) ;
#96720=CARTESIAN_POINT ( 'NONE',  ( 12.14561940090000114, 1409.337194763229718, 191.0894207074980216 ) ) ;
#96721=CARTESIAN_POINT ( 'NONE',  ( 5.013886338179999846, 1423.124965184129906, 184.3797681692980177 ) ) ;
#96726=CARTESIAN_POINT ( 'NONE',  ( -15.30199789809999977, 1451.561028161330114, 149.9720795101980002 ) ) ;
#96727=EDGE_CURVE ( 'NONE', #64454, #24504, #81671, .T. ) ;
#96731=CARTESIAN_POINT ( 'NONE',  ( -2.409586283469999923, 1426.663880916129983, 144.1938086916980239 ) ) ;
#96734=CARTESIAN_POINT ( 'NONE',  ( -25.61285747580000205, 1467.494200632129832, 270.3573890266980015 ) ) ;
#96735=CARTESIAN_POINT ( 'NONE',  ( -23.76373184819366813, 1436.064358996370402, 211.6811140537201652 ) ) ;
#96736=CARTESIAN_POINT ( 'NONE',  ( 3.282394052629999948, 1438.199601172570055, 155.5836490844979778 ) ) ;
#96738=CARTESIAN_POINT ( 'NONE',  ( -14.45760119950000089, 1463.281480820829984, 223.3430437907979922 ) ) ;
#96739=CARTESIAN_POINT ( 'NONE',  ( 15.96958168569999970, 1519.913060387329779, 193.1522642759980215 ) ) ;
#96740=CARTESIAN_POINT ( 'NONE',  ( -13.95121136070000034, 1421.607743136130011, 228.2237463402980211 ) ) ;
#96744=CARTESIAN_POINT ( 'NONE',  ( -45.08400256209149859, 1433.680806341129937, 266.7087657724729866 ) ) ;
#96750=AXIS2_PLACEMENT_3D ( 'NONE', #57757, #7325, #59958 ) ;
#96752=CARTESIAN_POINT ( 'NONE',  ( 12.78776258895000062, 1416.851343899079893, 222.7045348340550106 ) ) ;
#96753=CARTESIAN_POINT ( 'NONE',  ( -14.95559069659999984, 1425.419646131229911, 190.0114300131980087 ) ) ;
#96763=CARTESIAN_POINT ( 'NONE',  ( -16.31723503134719877, 1412.721052651110085, 269.3692194093940202 ) ) ;
#96765=CARTESIAN_POINT ( 'NONE',  ( -27.68327768569999847, 1435.464602415119771, 135.2595507401980228 ) ) ;
#96771=CARTESIAN_POINT ( 'NONE',  ( 45.63459694424612678, 1441.288710710889291, 268.9748222008650487 ) ) ;
#96776=CARTESIAN_POINT ( 'NONE',  ( -20.59848284610770008, 1506.575640312069936, 217.1340086378183400 ) ) ;
#96777=CARTESIAN_POINT ( 'NONE',  ( -19.34575562749999733, 1435.773310684580110, 224.5584730475980280 ) ) ;
#96778=CARTESIAN_POINT ( 'NONE',  ( -14.00912997540000049, 1416.839648771730026, 221.8523350237979912 ) ) ;
#96779=CARTESIAN_POINT ( 'NONE',  ( 12.77426335350000031, 1416.547221146729953, 222.9124519587980160 ) ) ;
#96780=CARTESIAN_POINT ( 'NONE',  ( 7.205930508499999831, 1446.348252743489866, 184.8949001284980227 ) ) ;
#96782=ORIENTED_EDGE ( 'NONE', *, *, #108896, .T. ) ;
#96784=CARTESIAN_POINT ( 'NONE',  ( 1.522490431809080169, 1455.721078906920184, 183.3572470959660166 ) ) ;
#96785=ORIENTED_EDGE ( 'NONE', *, *, #42194, .T. ) ;
#96787=ADVANCED_FACE ( 'NONE', ( #54855 ), #63271, .T. ) ;
#96788=CARTESIAN_POINT ( 'NONE',  ( 25.48798889943779855, 1450.979438871130014, 137.1176068765460059 ) ) ;
#96789=CARTESIAN_POINT ( 'NONE',  ( 14.34604702270000054, 1416.547221147930031, 196.6758286521979926 ) ) ;
#96792=CARTESIAN_POINT ( 'NONE',  ( 20.28790900150000098, 1410.981725563229929, 198.0270821811979829 ) ) ;
#96793=CARTESIAN_POINT ( 'NONE',  ( 12.53380499169999851, 1445.052233488290085, 169.4755105685979970 ) ) ;
#96794=CARTESIAN_POINT ( 'NONE',  ( 17.06446797460000298, 1409.673996215429952, 225.0967169420980269 ) ) ;
#96796=CARTESIAN_POINT ( 'NONE',  ( 21.29509819372636059, 1454.121024500114800, 221.5516887311115966 ) ) ;
#96804=CARTESIAN_POINT ( 'NONE',  ( -0.5138428465688279489, 1410.035027812230055, 233.1323959473689911 ) ) ;
#96807=CARTESIAN_POINT ( 'NONE',  ( -39.69692591273509663, 1446.534400439990122, 136.7156208858029913 ) ) ;
#96810=CARTESIAN_POINT ( 'NONE',  ( -3.804422480509999982, 1458.952956304630106, 234.3916895958979865 ) ) ;
#96813=CARTESIAN_POINT ( 'NONE',  ( -0.5964932758231209498, 1474.173341595109832, 270.1376979220820544 ) ) ;
#96817=ORIENTED_EDGE ( 'NONE', *, *, #40476, .F. ) ;
#96820=DIRECTION ( 'NONE',  ( -0.000000000000000000, -0.000000000000000000, -1.000000000000000000 ) ) ;
#96822=CARTESIAN_POINT ( 'NONE',  ( -3.481446190449999811, 1485.993219827530083, 182.2119038017980017 ) ) ;
#96823=VECTOR ( 'NONE', #48505, 1000.000000000000000 ) ;
#96825=CARTESIAN_POINT ( 'NONE',  ( 2.627197941649999979, 1499.011965180429797, 235.6151326529979997 ) ) ;
#96826=EDGE_CURVE ( 'NONE', #18369, #81651, #110746, .T. ) ;
#96827=CARTESIAN_POINT ( 'NONE',  ( 24.79630737949999997, 1449.797614621719958, 213.3734452447980061 ) ) ;
#96829=CARTESIAN_POINT ( 'NONE',  ( 4.363122647530000009, 1418.913060387330006, 172.2701767054979882 ) ) ;
#96831=CARTESIAN_POINT ( 'NONE',  ( 19.74177095050000119, 1466.547268800929942, 224.7591543658979845 ) ) ;
#96832=CARTESIAN_POINT ( 'NONE',  ( -16.37730547380552082, 1414.913060387329779, 208.0632427977511725 ) ) ;
#96842=CARTESIAN_POINT ( 'NONE',  ( -18.29057181139999955, 1416.237488680629895, 208.8052359792139896 ) ) ;
#96843=VERTEX_POINT ( 'NONE', #14468 ) ;
#96848=CARTESIAN_POINT ( 'NONE',  ( -16.67302254290000008, 1414.971352895729979, 209.3683777951139859 ) ) ;
#96853=CARTESIAN_POINT ( 'NONE',  ( 14.90637800594289963, 1409.433602577639931, 208.2132206234400087 ) ) ;
#96856=CARTESIAN_POINT ( 'NONE',  ( 2.750555068763795852, 1464.695220856118340, 236.8701281407333283 ) ) ;
#96859=CARTESIAN_POINT ( 'NONE',  ( 17.22592482065197927, 1443.913060387330233, 162.9227486220069920 ) ) ;
#96861=ORIENTED_EDGE ( 'NONE', *, *, #57615, .F. ) ;
#96862=CARTESIAN_POINT ( 'NONE',  ( -11.78977346134420046, 1415.441076448340027, 195.1339339561199893 ) ) ;
#96863=CARTESIAN_POINT ( 'NONE',  ( -11.45855569280000097, 1433.892739005809972, 151.4107738152980289 ) ) ;
#96864=CARTESIAN_POINT ( 'NONE',  ( 16.18935668596350297, 1469.063782001718891, 269.3698815738000576 ) ) ;
#96866=CARTESIAN_POINT ( 'NONE',  ( -28.27265633500000064, 1508.146186371529893, 208.9956447143910054 ) ) ;
#96868=CARTESIAN_POINT ( 'NONE',  ( -0.5257632930290000450, 1462.357837080030095, 182.8478810461979833 ) ) ;
#96870=CARTESIAN_POINT ( 'NONE',  ( -25.82488450470238917, 1436.659123590438639, 137.0441985079759490 ) ) ;
#96872=CARTESIAN_POINT ( 'NONE',  ( -13.04350371379999984, 1435.138103787100135, 150.1848718228980033 ) ) ;
#96873=COLOUR_RGB ( '', 0.08235294, 0.09019608, 0.10196078) ;
#96874=CARTESIAN_POINT ( 'NONE',  ( 17.05796332999999976, 1409.508737592730085, 194.6785584388979942 ) ) ;
#96877=EDGE_LOOP ( 'NONE', ( #21733, #110235, #24954, #98110 ) ) ;
#96878=CARTESIAN_POINT ( 'NONE',  ( 41.23304493959999917, 1435.760838929649935, 261.5842297915980339 ) ) ;
#96879=CARTESIAN_POINT ( 'NONE',  ( -22.70805116070000196, 1469.235391021629994, 197.6311956375980117 ) ) ;
#96880=CARTESIAN_POINT ( 'NONE',  ( -0.5378215255980000054, 1504.643126066929881, 180.9356492381979820 ) ) ;
#96881=CARTESIAN_POINT ( 'NONE',  ( 3.203789175851970288E-09, 1424.294192408320214, 227.6053815985079893 ) ) ;
#96883=CARTESIAN_POINT ( 'NONE',  ( -24.26836096399999931, 1418.067431480530104, 255.0044362610979647 ) ) ;
#96886=CARTESIAN_POINT ( 'NONE',  ( 33.93392841120000014, 1451.575795592029863, 135.5855060888980006 ) ) ;
#96888=CARTESIAN_POINT ( 'NONE',  ( 3.741929523840420213, 1397.105479193189922, 196.2901283285229965 ) ) ;
#96891=EDGE_LOOP ( 'NONE', ( #105155, #3421, #74726, #88513 ) ) ;
#96894=CARTESIAN_POINT ( 'NONE',  ( -23.58016236440349900, 1410.013568677760077, 208.8036717605170054 ) ) ;
#96896=ORIENTED_EDGE ( 'NONE', *, *, #85035, .F. ) ;
#96897=AXIS2_PLACEMENT_3D ( 'NONE', #21484, #45650, #62457 ) ;
#96898=CARTESIAN_POINT ( 'NONE',  ( -1.358844237360000040, 1412.076917109029864, 185.5300820243980127 ) ) ;
#96900=CARTESIAN_POINT ( 'NONE',  ( 0.4407570218449999855, 1450.897668812970096, 181.9257963629979997 ) ) ;
#96901=CARTESIAN_POINT ( 'NONE',  ( -1.656928908930000111, 1479.774557543030141, 235.9029919223980016 ) ) ;
#96902=DIRECTION ( 'NONE',  ( -0.02307801285194388888, -0.7475172515513471838, 0.6638413695725249308 ) ) ;
#96903=VERTEX_POINT ( 'NONE', #92836 ) ;
#96904=CARTESIAN_POINT ( 'NONE',  ( 11.43735029920000024, 1425.481221014229959, 144.1633320283980026 ) ) ;
#96906=CARTESIAN_POINT ( 'NONE',  ( 14.52328904310000013, 1474.745154377930021, 224.9348462990979840 ) ) ;
#96909=ORIENTED_EDGE ( 'NONE', *, *, #3535, .T. ) ;
#96910=CARTESIAN_POINT ( 'NONE',  ( 11.86522610041399872, 1432.274900462119831, 149.9820474266710164 ) ) ;
#96912=EDGE_CURVE ( 'NONE', #94116, #55879, #31386, .T. ) ;
#96913=CARTESIAN_POINT ( 'NONE',  ( 13.42472599018740276, 1444.364182771770857, 187.7916057231489617 ) ) ;
#96916=CARTESIAN_POINT ( 'NONE',  ( -15.68254779151874523, 1506.474306126180863, 193.6687607889768969 ) ) ;
#96919=CARTESIAN_POINT ( 'NONE',  ( 13.19514936480000067, 1509.316610144029937, 234.6191713803979724 ) ) ;
#96921=CARTESIAN_POINT ( 'NONE',  ( -4.306224067269999622, 1423.875121241730085, 184.5583045049980058 ) ) ;
#96922=CARTESIAN_POINT ( 'NONE',  ( 0.9513729900170889708, 1410.039306745070007, 269.8654762829310130 ) ) ;
#96929=CARTESIAN_POINT ( 'NONE',  ( 15.58680661270000023, 1453.154034702829904, 195.7020206013980044 ) ) ;
#96933=ORIENTED_EDGE ( 'NONE', *, *, #12302, .T. ) ;
#96934=CARTESIAN_POINT ( 'NONE',  ( 34.97756116859999764, 1432.582706846070096, 262.6648722463980334 ) ) ;
#96935=CIRCLE ( 'NONE', #12828, 2.000007505163727828 ) ;
#96936=CARTESIAN_POINT ( 'NONE',  ( 19.74853702175585823, 1455.472137957127870, 226.4474092902466396 ) ) ;
#96943=CARTESIAN_POINT ( 'NONE',  ( -4.152733088471870282, 1435.142315282680102, 185.7019193756299842 ) ) ;
#96944=ORIENTED_EDGE ( 'NONE', *, *, #73385, .T. ) ;
#96945=FACE_OUTER_BOUND ( 'NONE', #25047, .T. ) ;
#96946=CARTESIAN_POINT ( 'NONE',  ( -24.34269059140000024, 1442.549324342949831, 212.2035682044480041 ) ) ;
#96951=CARTESIAN_POINT ( 'NONE',  ( 30.67697261150000188, 1510.112560769530091, 213.7284012127280164 ) ) ;
#96954=CARTESIAN_POINT ( 'NONE',  ( 16.34175718830000079, 1410.409901383030046, 226.6814971688980052 ) ) ;
#96956=CARTESIAN_POINT ( 'NONE',  ( -16.13005433389999865, 1459.079426146030073, 230.3616589300980024 ) ) ;
#96958=CARTESIAN_POINT ( 'NONE',  ( 45.95995674830000155, 1436.878729300550049, 268.2107401488980258 ) ) ;
#96959=CARTESIAN_POINT ( 'NONE',  ( -18.12385451149999938, 1410.042553338630114, 224.1601288465979849 ) ) ;
#96960=EDGE_CURVE ( 'NONE', #87844, #75143, #76048, .T. ) ;
#96961=CARTESIAN_POINT ( 'NONE',  ( 19.17690546040000044, 1435.982630086400150, 146.1499213334980141 ) ) ;
#96962=CARTESIAN_POINT ( 'NONE',  ( 23.21287423860000132, 1488.579583080329940, 196.1738562084979947 ) ) ;
#96963=CARTESIAN_POINT ( 'NONE',  ( -16.66096088174899847, 1410.867477246420094, 191.7374981741809847 ) ) ;
#96965=CARTESIAN_POINT ( 'NONE',  ( -16.37880298289999814, 1420.875924758830024, 227.0362411946979933 ) ) ;
#96967=CARTESIAN_POINT ( 'NONE',  ( -35.57568823278909775, 1437.203474868449803, 136.5255046917930031 ) ) ;
#96969=CARTESIAN_POINT ( 'NONE',  ( -8.706022017420000481, 1409.217081375429871, 196.8236899110980005 ) ) ;
#96970=CARTESIAN_POINT ( 'NONE',  ( -18.69410140469999959, 1415.934222461130048, 207.6343539392380251 ) ) ;
#96971=CARTESIAN_POINT ( 'NONE',  ( -17.56004599463900817, 1410.529980821251456, 193.4350317141646940 ) ) ;
#96975=CARTESIAN_POINT ( 'NONE',  ( -1.368191914778909890, 1419.344528075180278, 185.2221190139939893 ) ) ;
#96976=EDGE_LOOP ( 'NONE', ( #10385, #86505, #30711, #39340 ) ) ;
#96979=CARTESIAN_POINT ( 'NONE',  ( -0.9045544433440699805, 1408.944648124569994, 224.0901810006990047 ) ) ;
#96982=CARTESIAN_POINT ( 'NONE',  ( -17.22592475669953416, 1443.501467202839649, 162.9227486557969655 ) ) ;
#96983=CARTESIAN_POINT ( 'NONE',  ( -42.53834064419999805, 1456.148668462929891, 267.7255875186979779 ) ) ;
#96984=CARTESIAN_POINT ( 'NONE',  ( -12.97254895038339839, 1428.741066686509839, 222.4354626778209933 ) ) ;
#96985=CARTESIAN_POINT ( 'NONE',  ( 0.2181331577922970000, 1420.478474626580009, 182.9759614564109711 ) ) ;
#96991=CARTESIAN_POINT ( 'NONE',  ( -28.25996323917220110, 1508.267047293149972, 208.8520637241439886 ) ) ;
#96996=CARTESIAN_POINT ( 'NONE',  ( -5.909457418149999697, 1509.192346212930033, 179.7976553797979875 ) ) ;
#96999=CARTESIAN_POINT ( 'NONE',  ( -12.65530650809999891, 1416.254459046630018, 195.1516350870979863 ) ) ;
#97001=CARTESIAN_POINT ( 'NONE',  ( 23.54238912610000156, 1411.095556395429867, 211.7543428466179876 ) ) ;
#97002=CARTESIAN_POINT ( 'NONE',  ( 3.902542035141590038, 1426.015650130040058, 185.2953857556300079 ) ) ;
#97004=CARTESIAN_POINT ( 'NONE',  ( -5.361099102583589016, 1423.467400204739988, 149.3859628662110026 ) ) ;
#97005=CARTESIAN_POINT ( 'NONE',  ( -11.31015099709999916, 1432.869308247210029, 151.5208831367980054 ) ) ;
#97007=CARTESIAN_POINT ( 'NONE',  ( -0.5133987858209999589, 1410.300672046529826, 233.1712545434979802 ) ) ;
#97012=B_SPLINE_CURVE_WITH_KNOTS ( 'NONE', 3,
 ( #9252, #32240, #43409, #23816, #92143, #68075, #319, #101073, #93769, #17048 ),
 .UNSPECIFIED., .F., .F.,
 ( 4, 2, 2, 2, 4 ),
 ( 3.551066926146560086E-09, 0.03694625896444130031, 0.07332082148824449475, 0.1158698472050300049, 0.1380128657416029858 ),
 .UNSPECIFIED. ) ;
#97014=CARTESIAN_POINT ( 'NONE',  ( 13.37391227950199912, 1507.591760071039971, 233.0544810109369962 ) ) ;
#97015=CARTESIAN_POINT ( 'NONE',  ( -18.97045675350529947, 1486.106069708590212, 189.3881501793050290 ) ) ;
#97020=ORIENTED_EDGE ( 'NONE', *, *, #22570, .F. ) ;
#97022=CARTESIAN_POINT ( 'NONE',  ( 29.54377282369999946, 1509.965350294430209, 211.5458056821180151 ) ) ;
#97026=CARTESIAN_POINT ( 'NONE',  ( 2.368833328420000051, 1427.018531676430030, 133.6118001900980232 ) ) ;
#97027=CARTESIAN_POINT ( 'NONE',  ( 15.77036826645290191, 1409.489309249800044, 192.6567201191820118 ) ) ;
#97029=CARTESIAN_POINT ( 'NONE',  ( -24.51797533977270049, 1451.993604082630100, 136.7394497936419953 ) ) ;
#97030=FACE_OUTER_BOUND ( 'NONE', #32891, .T. ) ;
#97031=CARTESIAN_POINT ( 'NONE',  ( 11.01620263480000084, 1409.800477099530099, 229.2053215475979755 ) ) ;
#97035=CARTESIAN_POINT ( 'NONE',  ( 41.44976345430139730, 1445.539178997240015, 134.0999999985149884 ) ) ;
#97037=ORIENTED_EDGE ( 'NONE', *, *, #46642, .T. ) ;
#97038=CARTESIAN_POINT ( 'NONE',  ( 14.51818222938589997, 1436.251066462949893, 149.9197869802679861 ) ) ;
#97043=EDGE_LOOP ( 'NONE', ( #104859, #37199, #89861, #102321, #9873, #21598, #6382, #581, #97859, #43345, #103061, #96592, #62883, #98684, #70028, #92325, #99777, #102995, #105865, #7646, #54671 ) ) ;
#97046=CARTESIAN_POINT ( 'NONE',  ( 9.248771300983904098, 1451.347040920142035, 152.5423568881176948 ) ) ;
#97051=CARTESIAN_POINT ( 'NONE',  ( 4.224261702798199458, 1446.243936627659878, 166.7668577399350056 ) ) ;
#97052=CARTESIAN_POINT ( 'NONE',  ( 0.6279831788249999880, 1507.650420244430052, 237.3702373079979964 ) ) ;
#97053=ORIENTED_EDGE ( 'NONE', *, *, #28772, .F. ) ;
#97056=CARTESIAN_POINT ( 'NONE',  ( 23.52342552954910104, 1440.913060387330006, 233.8510226637129961 ) ) ;
#97057=CARTESIAN_POINT ( 'NONE',  ( -16.42216134770000124, 1507.747023505630068, 185.8766527436980027 ) ) ;
#97060=CARTESIAN_POINT ( 'NONE',  ( -14.92380019159999982, 1409.936028048729895, 190.9400102447980032 ) ) ;
#97062=CARTESIAN_POINT ( 'NONE',  ( -24.36535764299999940, 1440.954195507719987, 211.6879696047379866 ) ) ;
#97065=CARTESIAN_POINT ( 'NONE',  ( 0.0002591936723112243891, 1396.150190320668798, 197.1672001813749944 ) ) ;
#97067=CARTESIAN_POINT ( 'NONE',  ( -27.69925886641940238, 1441.434395751479997, 137.3015763626259798 ) ) ;
#97069=CARTESIAN_POINT ( 'NONE',  ( 4.725705173089999711, 1464.404288624430137, 236.3620497209980158 ) ) ;
#97075=CARTESIAN_POINT ( 'NONE',  ( 28.48686854299999993, 1509.161777454930188, 208.9464261767249980 ) ) ;
#97080=EDGE_LOOP ( 'NONE', ( #57774, #107164, #28523, #63855, #13645, #89361 ) ) ;
#97081=CARTESIAN_POINT ( 'NONE',  ( -18.47399052110256434, 1509.320896586165190, 230.4813978297956396 ) ) ;
#97082=CARTESIAN_POINT ( 'NONE',  ( 10.01186952849999834, 1466.025750516530024, 244.5548898277980072 ) ) ;
#97086=CARTESIAN_POINT ( 'NONE',  ( 1.981508872149999601, 1413.133198254829949, 232.1370634949979888 ) ) ;
#97087=CARTESIAN_POINT ( 'NONE',  ( -18.82336198069999966, 1456.812963125929855, 227.8489049708979906 ) ) ;
#97088=FACE_OUTER_BOUND ( 'NONE', #17946, .T. ) ;
#97089=CARTESIAN_POINT ( 'NONE',  ( -0.4794255386038975830, 1547.913060387330006, 208.2442633998076076 ) ) ;
#97090=CARTESIAN_POINT ( 'NONE',  ( 0.04790323992079999205, 1506.806593688130079, 187.0235095034979906 ) ) ;
#97094=CARTESIAN_POINT ( 'NONE',  ( 0.7767783220340001016, 1405.847574658930171, 267.2347138816979850 ) ) ;
#97096=CARTESIAN_POINT ( 'NONE',  ( 13.24698951656310086, 1472.683393104890229, 270.3756650808729773 ) ) ;
#97097=CARTESIAN_POINT ( 'NONE',  ( 5.459750082109999347, 1438.302868353570148, 154.7313708644979897 ) ) ;
#97098=CARTESIAN_POINT ( 'NONE',  ( 10.16645255423411065, 1422.467695525055433, 137.0999999980980135 ) ) ;
#97099=CARTESIAN_POINT ( 'NONE',  ( -37.48482910262209344, 1440.913060388469830, 255.4418995164979833 ) ) ;
#97100=CARTESIAN_POINT ( 'NONE',  ( -25.40278959089999589, 1449.930493708720178, 137.7546507675980081 ) ) ;
#97102=CARTESIAN_POINT ( 'NONE',  ( 2.494611379217050118, 1449.235110048550041, 154.7922943218019896 ) ) ;
#97105=EDGE_LOOP ( 'NONE', ( #59165, #4090, #40813, #69369, #12240 ) ) ;
#97106=CARTESIAN_POINT ( 'NONE',  ( -28.05448514099999713, 1420.250147149929944, 265.6112250856980381 ) ) ;
#97109=CARTESIAN_POINT ( 'NONE',  ( -0.1080292017569999957, 1476.076643212830049, 267.5371647991979671 ) ) ;
#97110=CARTESIAN_POINT ( 'NONE',  ( -4.279554597526510129, 1446.812741322220063, 156.5769576174630231 ) ) ;
#97114=CARTESIAN_POINT ( 'NONE',  ( -18.08041632129999954, 1415.296882296330068, 207.5662767683379855 ) ) ;
#97116=CARTESIAN_POINT ( 'NONE',  ( 26.31830653128389841, 1435.497073113130000, 135.8492962503879937 ) ) ;
#97117=CARTESIAN_POINT ( 'NONE',  ( -4.896674508190200115, 1396.084056030580086, 219.0076142901629908 ) ) ;
#97119=CARTESIAN_POINT ( 'NONE',  ( -16.14471337837490239, 1409.485024636370099, 225.3510067295860040 ) ) ;
#97120=CARTESIAN_POINT ( 'NONE',  ( 19.63348512848709504, 1455.443522392392879, 225.9404624130569914 ) ) ;
#97123=CARTESIAN_POINT ( 'NONE',  ( 1.682318894840000079, 1409.475163267829885, 232.0401757884979759 ) ) ;
#97124=CARTESIAN_POINT ( 'NONE',  ( -11.79165747303489908, 1429.416857826700152, 146.4064127303859948 ) ) ;
#97125=CARTESIAN_POINT ( 'NONE',  ( 10.79671730919999995, 1425.341881714829924, 121.0042872764980046 ) ) ;
#97127=DIRECTION ( 'NONE',  ( 3.922329127182935292E-10, 2.146905620200830005E-11, -1.000000000000000000 ) ) ;
#97128=CARTESIAN_POINT ( 'NONE',  ( 4.252688412790660344, 1423.944491522370072, 183.9806639160489965 ) ) ;
#97132=CARTESIAN_POINT ( 'NONE',  ( 5.865902423269999666, 1509.102301102529964, 180.5560850680980138 ) ) ;
#97133=CARTESIAN_POINT ( 'NONE',  ( -8.301987938657498844, 1519.913060387329779, 185.0111222839169898 ) ) ;
#97137=ORIENTED_EDGE ( 'NONE', *, *, #54271, .T. ) ;
#97139=CARTESIAN_POINT ( 'NONE',  ( -6.232532193409999977, 1398.098440471930189, 197.7132727529979945 ) ) ;
#97140=CARTESIAN_POINT ( 'NONE',  ( 1.181642411293839956, 1499.053114097589969, 236.6882745191989841 ) ) ;
#97141=CARTESIAN_POINT ( 'NONE',  ( -23.03159172119999809, 1435.301732086839138, 138.5817198000980000 ) ) ;
#97143=( BOUNDED_CURVE ( )  B_SPLINE_CURVE ( 3, ( #67639, #41319, #25038, #93358 ),
 .UNSPECIFIED., .F., .F. ) 
 B_SPLINE_CURVE_WITH_KNOTS ( ( 4, 4 ),
 ( 0.8259411502862069598, 1.074666572263723863 ),
 .UNSPECIFIED. ) 
 CURVE ( )  GEOMETRIC_REPRESENTATION_ITEM ( )  RATIONAL_B_SPLINE_CURVE ( ( 1.000000000000000000, 0.9948512797181937595, 0.9948512797181937595, 1.000000000000000000 ) ) 
 REPRESENTATION_ITEM ( '' )  );
#97145=CARTESIAN_POINT ( 'NONE',  ( -1.365744575143430062, 1417.411668549410024, 185.3040620841360067 ) ) ;
#97146=CARTESIAN_POINT ( 'NONE',  ( 2.573164677909999920, 1410.304154922730049, 185.5984138544979771 ) ) ;
#97148=CARTESIAN_POINT ( 'NONE',  ( -39.10159291891720557, 1449.758070488810063, 135.2941250337750034 ) ) ;
#97149=CARTESIAN_POINT ( 'NONE',  ( -2.500000000000000000, 1448.624837927950011, 158.8309530183670120 ) ) ;
#97151=CARTESIAN_POINT ( 'NONE',  ( -40.32569152789999833, 1443.160161259170081, 137.0611730016980232 ) ) ;
#97152=CARTESIAN_POINT ( 'NONE',  ( -5.362056993596479693, 1405.980634290770240, 267.5249872241790285 ) ) ;
#97153=CARTESIAN_POINT ( 'NONE',  ( 41.65407234159999916, 1444.067060240220144, 136.1145731235980065 ) ) ;
#97156=ORIENTED_EDGE ( 'NONE', *, *, #36424, .F. ) ;
#97162=ORIENTED_EDGE ( 'NONE', *, *, #22644, .T. ) ;
#97163=CARTESIAN_POINT ( 'NONE',  ( 0.05242611179130000215, 1509.026403085430047, 179.1712902077980232 ) ) ;
#97165=CARTESIAN_POINT ( 'NONE',  ( 2.676552135149999678, 1415.087818611729972, 225.8826422939979750 ) ) ;
#97167=CARTESIAN_POINT ( 'NONE',  ( -28.79939581020000006, 1509.589065601529910, 208.7222536069020009 ) ) ;
#97168=CARTESIAN_POINT ( 'NONE',  ( -40.12837905666719251, 1431.802959192438948, 269.6125927220242033 ) ) ;
#97169=CARTESIAN_POINT ( 'NONE',  ( -10.14900592729999929, 1410.638279238530231, 229.5672309112980258 ) ) ;
#97170=DIRECTION ( 'NONE',  ( 0.01430194049125190457, -0.9998977151614593106, 0.0001171028509539070479 ) ) ;
#97171=ORIENTED_EDGE ( 'NONE', *, *, #32902, .T. ) ;
#97172=CARTESIAN_POINT ( 'NONE',  ( 30.22858968940000324, 1451.857573268230226, 134.8239104374980002 ) ) ;
#97173=CARTESIAN_POINT ( 'NONE',  ( 28.34110756910000006, 1508.137170137529893, 208.7852603947239913 ) ) ;
#97176=CARTESIAN_POINT ( 'NONE',  ( 15.38665937780000093, 1409.887291428229901, 270.2482212356980540 ) ) ;
#97179=CARTESIAN_POINT ( 'NONE',  ( 0.02018220001661512678, 1507.197434269262885, 237.3577821747751955 ) ) ;
#97184=CARTESIAN_POINT ( 'NONE',  ( 22.60252566574085265, 1411.062741202461893, 206.6262987201641579 ) ) ;
#97185=CARTESIAN_POINT ( 'NONE',  ( -5.992618678210000382, 1415.369965543630087, 231.7268348280979922 ) ) ;
#97190=EDGE_CURVE ( 'NONE', #29004, #8321, #80013, .T. ) ;
#97191=CARTESIAN_POINT ( 'NONE',  ( 6.759474678068709608, 1416.948096802419968, 199.3542690954639909 ) ) ;
#97192=DIRECTION ( 'NONE',  ( 0.9993902469235411701, -0.03489947644508400310, -0.001077449749359510062 ) ) ;
#97200=CARTESIAN_POINT ( 'NONE',  ( -12.85972207402410028, 1415.932840154009909, 196.7491075114069758 ) ) ;
#97201=CARTESIAN_POINT ( 'NONE',  ( -6.284474420099999570, 1504.313428625830056, 181.0267274810979927 ) ) ;
#97203=CARTESIAN_POINT ( 'NONE',  ( 11.60004869885204570, 1426.721831229858708, 134.4552184562548121 ) ) ;
#97204=CARTESIAN_POINT ( 'NONE',  ( 11.05580244138281110, 1434.160380231334329, 151.7245384693764265 ) ) ;
#97206=B_SPLINE_CURVE_WITH_KNOTS ( 'NONE', 3,
 ( #28329, #62521, #12632, #10418, #96643, #63616, #36181, #46809, #89336, #70364, #104480, #19912, #61963, #106139, #72547, #45153, #19352, #10979, #71480, #72023, #3157, #79293, #11534, #46265, #106678, #61405, #2604, #36728, #97733, #80393, #54113, #21004, #45708, #28884, #97179, #20453, #12072, #83683, #89881, #40032, #47336 ),
 .UNSPECIFIED., .F., .F.,
 ( 4, 2, 2, 2, 2, 2, 2, 2, 1, 2, 2, 2, 1, 2, 2, 2, 1, 2, 2, 2, 2, 4 ),
 ( 0.000000000000000000, 0.2500000000005749845, 0.3750000000008624768, 0.4375000000010931811, 0.4687500000011134427, 0.5000000000011337598, 0.6250000000012745360, 0.6875000000013369306, 0.7187500000013611334, 0.7343750000012517765, 0.7500000000011425305, 0.8125000000011113332, 0.8437500000009711121, 0.8593750000007701617, 0.8750000000005691003, 0.9374999999997651878, 0.9531249999996305178, 0.9609374999996921352, 0.9687499999997537525, 0.9765624999998152589, 0.9843749999998768763, 1.000000000000000000 ),
 .UNSPECIFIED. ) ;
#97209=CARTESIAN_POINT ( 'NONE',  ( 16.27911523319127696, 1421.519124619010199, 227.2603791194927112 ) ) ;
#97210=B_SPLINE_CURVE_WITH_KNOTS ( 'NONE', 5,
 ( #93626, #58408, #76301, #60627, #101472, #109367, #8527, #34291, #110451, #32645, #50006, #41603, #33730, #42703, #33183, #66822, #76859, #94750, #92533, #58957, #68474, #93090, #102575, #60073 ),
 .UNSPECIFIED., .F., .F.,
 ( 6, 3, 3, 3, 3, 3, 3, 6 ),
 ( 0.000000000000000000, 0.03529544314845208669, 0.06179047381933735344, 0.08828550449022262714, 0.1412755658236120593, 0.2826075209337656768, 0.5644368487256844480, 1.000000000000000000 ),
 .UNSPECIFIED. ) ;
#97212=CARTESIAN_POINT ( 'NONE',  ( -18.48452897440000342, 1425.095849964330000, 227.3281627736979829 ) ) ;
#97213=CARTESIAN_POINT ( 'NONE',  ( -18.88473658259999866, 1435.156969464529766, 145.0455764213979819 ) ) ;
#97215=CARTESIAN_POINT ( 'NONE',  ( 17.53366402320000006, 1416.208575665629951, 192.2869590761980021 ) ) ;
#97216=CARTESIAN_POINT ( 'NONE',  ( 0.5470371568191350065, 1409.436771746549994, 232.9505920115730078 ) ) ;
#97217=CARTESIAN_POINT ( 'NONE',  ( -18.56596160438178345, 1436.937764507165639, 212.4410944778063879 ) ) ;
#97220=CARTESIAN_POINT ( 'NONE',  ( -2.109962112465985307, 1410.360755925830745, 186.3561355254459215 ) ) ;
#97227=CARTESIAN_POINT ( 'NONE',  ( -18.46505093760000094, 1509.557874173729942, 231.0973782673979713 ) ) ;
#97228=CARTESIAN_POINT ( 'NONE',  ( 0.2759407239221501884, 1408.922696449764544, 231.7129903492111396 ) ) ;
#97229=CARTESIAN_POINT ( 'NONE',  ( 12.18840501149665201, 1435.566324351502544, 151.0986007949610439 ) ) ;
#97230=CARTESIAN_POINT ( 'NONE',  ( 4.363122647530000009, 1422.407399603929889, 168.7758374889979791 ) ) ;
#97237=CARTESIAN_POINT ( 'NONE',  ( 20.61689931789999974, 1509.299814820330084, 189.0201468792980108 ) ) ;
#97238=ORIENTED_EDGE ( 'NONE', *, *, #71049, .F. ) ;
#97241=ORIENTED_EDGE ( 'NONE', *, *, #26674, .F. ) ;
#97243=CARTESIAN_POINT ( 'NONE',  ( 25.33052504582559905, 1453.000140514270015, 207.7150163121590083 ) ) ;
#97245=CARTESIAN_POINT ( 'NONE',  ( 12.77355678467065303, 1442.835118811306529, 169.4523574570036430 ) ) ;
#97246=CARTESIAN_POINT ( 'NONE',  ( 39.46380715081631507, 1430.354105498958688, 269.6007763216737203 ) ) ;
#97247=CARTESIAN_POINT ( 'NONE',  ( -29.87496815480000123, 1442.835664418360011, 238.0574314900979971 ) ) ;
#97248=CARTESIAN_POINT ( 'NONE',  ( -20.08779309810000058, 1491.274044621930216, 190.8703246068980093 ) ) ;
#97249=CARTESIAN_POINT ( 'NONE',  ( -11.38815357430000041, 1433.875739129769954, 151.4350069040980031 ) ) ;
#97250=CARTESIAN_POINT ( 'NONE',  ( 26.20829668540000057, 1507.984234506930079, 201.9879544258380122 ) ) ;
#97251=CARTESIAN_POINT ( 'NONE',  ( -19.21256531279999891, 1485.592793457429934, 189.7209763221979983 ) ) ;
#97253=CARTESIAN_POINT ( 'NONE',  ( 5.044474169190000801, 1422.662929545129828, 184.9412868827979821 ) ) ;
#97255=CARTESIAN_POINT ( 'NONE',  ( 7.733452464780000035, 1440.968359251539823, 154.0956077494979866 ) ) ;
#97256=CARTESIAN_POINT ( 'NONE',  ( 12.63038619288439968, 1428.207532477410041, 223.9332333053530135 ) ) ;
#97257=CARTESIAN_POINT ( 'NONE',  ( 0.3083741877719999858, 1507.133244740429973, 237.3561682571980214 ) ) ;
#97260=ORIENTED_EDGE ( 'NONE', *, *, #14146, .F. ) ;
#97262=EDGE_CURVE ( 'NONE', #88507, #87844, #85526, .T. ) ;
#97265=CARTESIAN_POINT ( 'NONE',  ( -20.73365673589999858, 1470.033777940730033, 270.3294707277980251 ) ) ;
#97266=CARTESIAN_POINT ( 'NONE',  ( -23.76173655485600378, 1436.066805062839194, 211.6885914087122558 ) ) ;
#97267=CARTESIAN_POINT ( 'NONE',  ( 16.60786453549999919, 1409.493019796529779, 222.4680777416979822 ) ) ;
#97269=CARTESIAN_POINT ( 'NONE',  ( -15.95383389570000077, 1506.798305147730161, 224.6865364803979901 ) ) ;
#97270=CARTESIAN_POINT ( 'NONE',  ( 0.9776412681320001408, 1475.513060387329915, 187.4983515543979991 ) ) ;
#97271=EDGE_CURVE ( 'NONE', #22747, #96120, #19432, .T. ) ;
#97272=CARTESIAN_POINT ( 'NONE',  ( -11.62261217039999828, 1420.448898375830140, 230.7381671621980104 ) ) ;
#97274=( BOUNDED_SURFACE ( )  B_SPLINE_SURFACE ( 1, 2, ( 
 ( #55977, #45386, #27823 ),
 ( #2093, #103969, #44637 ) ),
 .UNSPECIFIED., .F., .F., .T. ) 
 B_SPLINE_SURFACE_WITH_KNOTS ( ( 2, 2 ),
 ( 3, 3 ),
 ( -10000.00000000000000, 10000.00000000000000 ),
 ( 5.300753508068400066, 6.146881668114829722 ),
 .UNSPECIFIED. ) 
 GEOMETRIC_REPRESENTATION_ITEM ( )  RATIONAL_B_SPLINE_SURFACE ( (
 ( 0.8627701935022100699, 0.8231901671853920632, 0.9535799773420449155),
 ( 0.8627701935022100699, 0.8231901671853920632, 0.9535799773420449155) ) ) 
 REPRESENTATION_ITEM ( '' )  SURFACE ( )  );
#97277=CARTESIAN_POINT ( 'NONE',  ( -45.94972966655959823, 1436.699121074330151, 267.6009661011610206 ) ) ;
#97278=VERTEX_POINT ( 'NONE', #8820 ) ;
#97280=AXIS2_PLACEMENT_3D ( 'NONE', #68680, #68140, #102251 ) ;
#97281=ADVANCED_FACE ( 'NONE', ( #26738 ), #1851, .T. ) ;
#97285=CARTESIAN_POINT ( 'NONE',  ( 17.60061308773152433, 1410.712255111885952, 224.8086590843146269 ) ) ;
#97286=DIRECTION ( 'NONE',  ( -1.000000000000000000, 0.000000000000000000, 0.000000000000000000 ) ) ;
#97289=B_SPLINE_SURFACE_WITH_KNOTS ( 'NONE', 5, 5, ( 
 ( #51575, #49922, #92447, #25234, #25789, #81, #67836, #94665, #9551, #68948, #34209, #68393 ),
 ( #35313, #43177, #69499, #59988, #77874, #94105, #58873, #103622, #17376, #1182, #75678, #101382 ),
 ( #77329, #630, #103048, #26346, #60544, #93005, #24675, #86263, #109821, #15721, #84059, #67290 ),
 ( #16279, #50482, #84605, #19605, #61109, #62199, #53807, #10677, #2838, #70061, #89014, #97424 ),
 ( #29119, #80070, #95224, #79535, #78997, #63304, #20693, #96883, #54889, #18486, #104721, #12304 ),
 ( #52683, #20152, #86819, #10111, #46496, #54349, #70603, #28012, #36960, #96327, #28570, #45396 ),
 ( #80628, #44283, #87943, #71154, #3943, #78427, #53241, #11234, #38070, #71723, #105276, #1738 ),
 ( #35877, #104173, #62768, #88480, #27457, #3391, #44844, #61642, #45934, #72247, #37520, #11765 ),
 ( #95772, #19038, #26920, #87382, #2300, #105840, #36411, #4479, #108016, #74450, #6665, #21229 ),
 ( #56536, #13392, #82818, #39157, #65496, #73332, #66053, #108578, #6110, #107466, #57098, #99605 ),
 ( #106374, #30762, #73889, #64943, #47579, #31865, #57655, #40267, #99056, #22336, #90664, #13947 ),
 ( #40819, #48137, #91767, #31312, #82276, #5574, #39724, #22888, #100177, #15045, #91224, #63847 ),
 ( #29662, #14504, #49243, #89568, #38609, #23461, #48694, #90109, #83365, #97959, #81703, #106915 ),
 ( #55439, #12858, #47040, #81164, #72788, #30204, #64395, #98516, #21784, #55985, #5010, #110227 ),
 ( #58735, #50889, #7226, #26214, #34629, #83924, #77202, #17240, #32429, #16689, #16151, #504 ) ),
 .UNSPECIFIED., .F., .F., .F.,
 ( 6, 3, 3, 3, 6 ),
 ( 6, 3, 3, 6 ),
 ( 1.933773958289999984, 17.84603210599999912, 29.17820978809999843, 40.51038747020000130, 63.49323769619999780 ),
 ( 168.7272174100000086, 189.8181195859999946, 210.9090217629999984, 253.0908261149999987 ),
 .UNSPECIFIED. ) ;
#97292=EDGE_CURVE ( 'NONE', #107054, #79161, #22368, .T. ) ;
#97298=CARTESIAN_POINT ( 'NONE',  ( -13.23542543278949957, 1410.634354704430052, 270.3664647165679753 ) ) ;
#97299=CARTESIAN_POINT ( 'NONE',  ( -2.368833328420000051, 1427.018531676430030, 133.6118001900980232 ) ) ;
#97300=DIRECTION ( 'NONE',  ( -9.520249230476377039E-08, -3.411690578513119204E-09, -0.9999999999999954481 ) ) ;
#97302=ORIENTED_EDGE ( 'NONE', *, *, #22971, .T. ) ;
#97307=CARTESIAN_POINT ( 'NONE',  ( 3.750641173502857306, 1424.073545704406115, 183.6511083008927301 ) ) ;
#97308=CARTESIAN_POINT ( 'NONE',  ( -27.32596821242635343, 1412.869984779867991, 266.6662420334005219 ) ) ;
#97310=CARTESIAN_POINT ( 'NONE',  ( -17.98740375195779606, 1415.258594619250061, 207.5661176034399773 ) ) ;
#97311=CARTESIAN_POINT ( 'NONE',  ( 2.511983255966640183, 1439.367848956780108, 157.7248713869030325 ) ) ;
#97312=CARTESIAN_POINT ( 'NONE',  ( -14.40866948829999927, 1423.490938386730022, 221.9456809809980200 ) ) ;
#97313=CARTESIAN_POINT ( 'NONE',  ( 12.44325168979999852, 1415.996778985530000, 223.2102471899980003 ) ) ;
#97314=CARTESIAN_POINT ( 'NONE',  ( 4.219439073160000220, 1446.230224797059918, 182.3842143240980249 ) ) ;
#97316=ORIENTED_EDGE ( 'NONE', *, *, #26715, .T. ) ;
#97317=CARTESIAN_POINT ( 'NONE',  ( 5.164931156380000507E-11, 1452.913060387330006, 179.9625354400980086 ) ) ;
#97318=CARTESIAN_POINT ( 'NONE',  ( -22.63601521178858533, 1451.224009660701086, 219.0470436816254391 ) ) ;
#97320=CARTESIAN_POINT ( 'NONE',  ( 10.54139892624155728, 1455.171105620551089, 226.3039058597585438 ) ) ;
#97321=CARTESIAN_POINT ( 'NONE',  ( 25.25148443142990118, 1451.314349325280091, 137.1731793465510236 ) ) ;
#97326=CARTESIAN_POINT ( 'NONE',  ( -3.313293292670107082, 1446.583016671109135, 170.5342543429541422 ) ) ;
#97327=CARTESIAN_POINT ( 'NONE',  ( 16.34140767499999924, 1409.483715582329978, 225.5328183092979941 ) ) ;
#97329=CARTESIAN_POINT ( 'NONE',  ( 21.69285400322056745, 1453.394215773794485, 220.8286852162956677 ) ) ;
#97330=CARTESIAN_POINT ( 'NONE',  ( 2.500000000000000000, 1439.547542061109880, 164.8613946483260122 ) ) ;
#97336=CARTESIAN_POINT ( 'NONE',  ( -12.98226713004480004, 1414.913060387349788, 219.9156686614909972 ) ) ;
#97337=ADVANCED_FACE ( 'NONE', ( #53928 ), #64511, .F. ) ;
#97338=DIRECTION ( 'NONE',  ( 1.000000000000000000, -2.735358204715540176E-15, 3.765374186129670039E-15 ) ) ;
#97339=EDGE_CURVE ( 'NONE', #63865, #92743, #110382, .T. ) ;
#97340=CARTESIAN_POINT ( 'NONE',  ( -40.10575600315020495, 1445.309576473759989, 136.9127853735360247 ) ) ;
#97341=CARTESIAN_POINT ( 'NONE',  ( 11.60004869885571743, 1425.366405675970555, 138.1206266335812245 ) ) ;
#97344=CARTESIAN_POINT ( 'NONE',  ( 11.86848022610000086, 1433.047056341809821, 150.2049543995979946 ) ) ;
#97345=DIRECTION ( 'NONE',  ( -2.093802707073269138E-06, 0.4875922912088249683, 0.8730714504262205855 ) ) ;
#97352=CARTESIAN_POINT ( 'NONE',  ( 11.23388613411650638, 1445.063428794548372, 150.9272215568491049 ) ) ;
#97355=CARTESIAN_POINT ( 'NONE',  ( 7.146055568748121090, 1398.125191567241473, 198.2455685561245673 ) ) ;
#97356=CARTESIAN_POINT ( 'NONE',  ( 1.712115011030000078, 1498.987102142929871, 236.1549197522979853 ) ) ;
#97359=CARTESIAN_POINT ( 'NONE',  ( -17.25705191650000003, 1509.016679771029885, 230.6108905181980333 ) ) ;
#97361=CARTESIAN_POINT ( 'NONE',  ( -16.11867490360164368, 1414.913060387329779, 208.6659696099576422 ) ) ;
#97363=CARTESIAN_POINT ( 'NONE',  ( 2.562182094880000260, 1464.635166048130031, 236.5709022716980030 ) ) ;
#97367=CARTESIAN_POINT ( 'NONE',  ( -1.483649241179999967, 1450.644272461199762, 182.4983721051980012 ) ) ;
#97368=ADVANCED_FACE ( 'NONE', ( #91346 ), #21537, .F. ) ;
#97370=CARTESIAN_POINT ( 'NONE',  ( -20.58126087740000187, 1507.779106712530165, 190.0921675882979969 ) ) ;
#97371=CARTESIAN_POINT ( 'NONE',  ( 27.01381218759999925, 1450.681579806120226, 136.4483250053980044 ) ) ;
#97372=VERTEX_POINT ( 'NONE', #46618 ) ;
#97377=CARTESIAN_POINT ( 'NONE',  ( 11.89599453232379922, 1434.596263782940014, 147.6475367373340077 ) ) ;
#97382=CARTESIAN_POINT ( 'NONE',  ( 12.49050510308880035, 1409.349238429849720, 217.3209073824620248 ) ) ;
#97384=CARTESIAN_POINT ( 'NONE',  ( 18.03628730299999816, 1424.824108734929723, 224.7110847794980089 ) ) ;
#97386=CARTESIAN_POINT ( 'NONE',  ( -18.21568074059999987, 1430.634797966130009, 192.8606760977980059 ) ) ;
#97387=CARTESIAN_POINT ( 'NONE',  ( 11.57624701549999990, 1432.320296800590086, 151.1967064319979670 ) ) ;
#97388=B_SPLINE_CURVE_WITH_KNOTS ( 'NONE', 5,
 ( #85484, #33427, #65556, #9357, #14569, #84937 ),
 .UNSPECIFIED., .F., .F.,
 ( 6, 6 ),
 ( 0.000000000000000000, 11.48858425020000240 ),
 .UNSPECIFIED. ) ;
#97394=CARTESIAN_POINT ( 'NONE',  ( -2.745154014197499937, 1419.769956470485113, 137.0999999980979851 ) ) ;
#97395=AXIS2_PLACEMENT_3D ( 'NONE', #12900, #38109, #7805 ) ;
#97398=CARTESIAN_POINT ( 'NONE',  ( 21.90260416155314260, 1466.954533459972936, 269.4017626923731541 ) ) ;
#97400=CARTESIAN_POINT ( 'NONE',  ( 7.491155460734093552, 1414.913060387329779, 223.8341484298593684 ) ) ;
#97401=CARTESIAN_POINT ( 'NONE',  ( 21.91582124097350004, 1491.015010933479971, 209.7149842846540082 ) ) ;
#97402=CARTESIAN_POINT ( 'NONE',  ( -0.8687435992890001346, 1453.579571206030096, 183.3443055433980078 ) ) ;
#97409=B_SPLINE_SURFACE_WITH_KNOTS ( 'NONE', 5, 5, ( 
 ( #73076, #47866, #88772, #47316, #97163, #98260 ),
 ( #4751, #37816, #97712, #3688, #22621, #13132 ),
 ( #20984, #106657, #56824, #106117, #72003, #82001 ),
 ( #31054, #30504, #64693, #105578, #38893, #46790 ),
 ( #29393, #80919, #14247, #81440, #48436, #65235 ),
 ( #38347, #63594, #89863, #4218, #82578, #12055 ) ),
 .UNSPECIFIED., .F., .F., .F.,
 ( 6, 6 ),
 ( 6, 6 ),
 ( 113.0406221479999971, 134.6442539944619909 ),
 ( 0.3006958241500000129, 0.4689188458459999653 ),
 .UNSPECIFIED. ) ;
#97410=CARTESIAN_POINT ( 'NONE',  ( 19.54165283311759893, 1409.595469941420106, 199.8969299576039873 ) ) ;
#97411=FACE_OUTER_BOUND ( 'NONE', #53522, .T. ) ;
#97412=CARTESIAN_POINT ( 'NONE',  ( -15.72154079564279705, 1469.202802763679983, 228.9466779226059714 ) ) ;
#97413=EDGE_CURVE ( 'NONE', #91917, #76557, #6341, .T. ) ;
#97415=CARTESIAN_POINT ( 'NONE',  ( 41.65640094522370163, 1444.002002823209978, 135.7347776446760008 ) ) ;
#97417=CARTESIAN_POINT ( 'NONE',  ( 28.33103133730000067, 1431.247806717339927, 240.1819618771980061 ) ) ;
#97418=CARTESIAN_POINT ( 'NONE',  ( -20.81017607009999892, 1469.236365769730128, 194.6575948795980082 ) ) ;
#97419=CARTESIAN_POINT ( 'NONE',  ( -10.74627445883099952, 1425.683497583799863, 97.52444174273580302 ) ) ;
#97420=CARTESIAN_POINT ( 'NONE',  ( -17.57263965230000125, 1409.691669017629920, 195.6049322489980113 ) ) ;
#97421=B_SPLINE_CURVE_WITH_KNOTS ( 'NONE', 5,
 ( #23872, #13818, #73771, #48003, #5992, #107895, #65374, #91649, #31188, #74868, #108455, #31737 ),
 .UNSPECIFIED., .F., .F.,
 ( 6, 3, 3, 6 ),
 ( 0.000000000000000000, 0.4515349285676349966, 0.7455155029937545752, 1.000000000000000000 ),
 .UNSPECIFIED. ) ;
#97424=CARTESIAN_POINT ( 'NONE',  ( 1.852756268550000001E-09, 1409.477339444430072, 259.9484415776979631 ) ) ;
#97426=CARTESIAN_POINT ( 'NONE',  ( 3.373940653401940715, 1447.285893942237180, 154.8523594219587665 ) ) ;
#97427=CARTESIAN_POINT ( 'NONE',  ( 32.74960620270000078, 1451.769474672029901, 135.1835671602979971 ) ) ;
#97428=ORIENTED_EDGE ( 'NONE', *, *, #100623, .F. ) ;
#97429=CARTESIAN_POINT ( 'NONE',  ( -2.500000000000000000, 1426.216228438830058, 155.9944625376979843 ) ) ;
#97432=ORIENTED_EDGE ( 'NONE', *, *, #53466, .F. ) ;
#97435=CIRCLE ( 'NONE', #86640, 26.99999999999999645 ) ;
#97439=CARTESIAN_POINT ( 'NONE',  ( -1.361182826989999928, 1413.855685395729779, 185.4547579133979980 ) ) ;
#97443=CARTESIAN_POINT ( 'NONE',  ( 0.5253559788449999601, 1450.894714552289997, 181.2879659622979887 ) ) ;
#97444=CARTESIAN_POINT ( 'NONE',  ( -0.7153112824419999294, 1489.065501047429962, 236.4817586033979921 ) ) ;
#97447=CARTESIAN_POINT ( 'NONE',  ( 11.63668813159999971, 1425.864839735429769, 144.1681848196979843 ) ) ;
#97448=CARTESIAN_POINT ( 'NONE',  ( -12.65294384001009931, 1415.935475482089942, 221.7859427658239895 ) ) ;
#97449=CARTESIAN_POINT ( 'NONE',  ( 13.73732212659999874, 1452.821288644329798, 224.4407649501980018 ) ) ;
#97452=ORIENTED_EDGE ( 'NONE', *, *, #27805, .F. ) ;
#97453=CARTESIAN_POINT ( 'NONE',  ( 11.84627492255189907, 1430.966456813360082, 149.8093626651640022 ) ) ;
#97454=CARTESIAN_POINT ( 'NONE',  ( 12.53380665967529950, 1445.052233242549846, 186.0874955919830143 ) ) ;
#97466=CARTESIAN_POINT ( 'NONE',  ( 0.02513987172886716220, 1410.234108419300810, 233.2181343497910575 ) ) ;
#97470=CARTESIAN_POINT ( 'NONE',  ( -24.03340273735519972, 1507.991624071270053, 222.3151666817440173 ) ) ;
#97472=ORIENTED_EDGE ( 'NONE', *, *, #16548, .F. ) ;
#97473=CARTESIAN_POINT ( 'NONE',  ( 34.84383463460000030, 1427.856177373630089, 265.6112251771979800 ) ) ;
#97474=CARTESIAN_POINT ( 'NONE',  ( 18.65451742820949832, 1507.632629731499947, 188.5326158842280222 ) ) ;
#97479=CARTESIAN_POINT ( 'NONE',  ( 17.72826782676450108, 1408.955359599259964, 269.5568341151930554 ) ) ;
#97481=CARTESIAN_POINT ( 'NONE',  ( -4.149769861736410270, 1430.580313301509932, 185.9069866752190023 ) ) ;
#97483=CARTESIAN_POINT ( 'NONE',  ( 17.36801837519999836, 1414.983771848829747, 210.5058389745279896 ) ) ;
#97484=CARTESIAN_POINT ( 'NONE',  ( -24.27053168829999663, 1443.236894957179857, 212.3234000011480020 ) ) ;
#97485=CARTESIAN_POINT ( 'NONE',  ( -2.233110619234230487, 1449.897286081790298, 154.3831795966705442 ) ) ;
#97488=CARTESIAN_POINT ( 'NONE',  ( -7.303957127409999472, 1440.776932085429962, 186.0900577853979883 ) ) ;
#97490=CARTESIAN_POINT ( 'NONE',  ( 27.54845678703150114, 1509.914129475679829, 222.6825216195649944 ) ) ;
#97492=CARTESIAN_POINT ( 'NONE',  ( -0.9756374909739999879, 1431.113060387329824, 228.8047907271979966 ) ) ;
#97493=CARTESIAN_POINT ( 'NONE',  ( 7.383547498839999612, 1417.414537312230095, 231.0421684962979896 ) ) ;
#97497=CARTESIAN_POINT ( 'NONE',  ( 46.05260656040000100, 1438.905840350680137, 266.6770572228979859 ) ) ;
#97498=CARTESIAN_POINT ( 'NONE',  ( -17.45090663859999935, 1409.522459475629830, 223.7636686640979917 ) ) ;
#97499=CARTESIAN_POINT ( 'NONE',  ( 21.87661169429999575, 1435.403821294829868, 142.1301396295980055 ) ) ;
#97500=CARTESIAN_POINT ( 'NONE',  ( 20.17949039979999881, 1469.158434794429922, 192.3038326788980044 ) ) ;
#97501=CARTESIAN_POINT ( 'NONE',  ( -16.03382226631890006, 1409.472973801630133, 193.0383433025830016 ) ) ;
#97502=CARTESIAN_POINT ( 'NONE',  ( -2.765183635730000145, 1475.775321107629907, 266.9581418145979796 ) ) ;
#97504=CARTESIAN_POINT ( 'NONE',  ( -39.97226237699269547, 1438.646033188909996, 135.6295559456019930 ) ) ;
#97505=CARTESIAN_POINT ( 'NONE',  ( 0.2178157486290130118, 1452.982786607829894, 183.2541296479709843 ) ) ;
#97506=CARTESIAN_POINT ( 'NONE',  ( -13.29011429918680065, 1407.447342471949923, 210.5442722391819927 ) ) ;
#97509=EDGE_CURVE ( 'NONE', #105027, #25245, #31730, .T. ) ;
#97512=CARTESIAN_POINT ( 'NONE',  ( -35.72409870509849839, 1435.953719464810092, 134.0999999973689967 ) ) ;
#97514=ORIENTED_EDGE ( 'NONE', *, *, #23751, .F. ) ;
#97516=CARTESIAN_POINT ( 'NONE',  ( -3.210101824899569856, 1409.025159613220012, 223.7627473412850065 ) ) ;
#97518=CARTESIAN_POINT ( 'NONE',  ( -2.477970950320000032, 1440.426958604040010, 157.8055609083980073 ) ) ;
#97519=CARTESIAN_POINT ( 'NONE',  ( -16.90742456144603523, 1442.831169986190389, 162.4348202098863396 ) ) ;
#97520=CARTESIAN_POINT ( 'NONE',  ( -31.74876339820000126, 1466.573431914830053, 268.0541753359980248 ) ) ;
#97521=CARTESIAN_POINT ( 'NONE',  ( -13.30777107328369979, 1428.971706346040037, 222.3032313369639894 ) ) ;
#97527=CARTESIAN_POINT ( 'NONE',  ( 12.58432885909999932, 1415.426210663629945, 221.2617231595980059 ) ) ;
#97528=CARTESIAN_POINT ( 'NONE',  ( -6.484578373979999810, 1434.540925522399903, 154.7070604761979951 ) ) ;
#97531=ORIENTED_EDGE ( 'NONE', *, *, #57636, .T. ) ;
#97532=CARTESIAN_POINT ( 'NONE',  ( -4.026786250540000722, 1408.413060387330006, 146.1721969590979882 ) ) ;
#97534=CARTESIAN_POINT ( 'NONE',  ( -23.49263094430000010, 1409.898020881729963, 208.4774537725740231 ) ) ;
#97535=CARTESIAN_POINT ( 'NONE',  ( 26.56924837500000081, 1488.569808382929978, 207.4007344032380047 ) ) ;
#97536=CARTESIAN_POINT ( 'NONE',  ( 2.688586027246119947, 1509.006950727750109, 238.2845013960090057 ) ) ;
#97537=DIRECTION ( 'NONE',  ( -0.8771707348056354547, 0.03063147701716761526, 0.4792005995575221999 ) ) ;
#97538=EDGE_CURVE ( 'NONE', #11508, #16786, #27762, .T. ) ;
#97539=CARTESIAN_POINT ( 'NONE',  ( 23.64283040619999809, 1411.099127945830105, 211.3905525550979974 ) ) ;
#97543=CARTESIAN_POINT ( 'NONE',  ( -5.360046087876660259, 1422.261995185559954, 145.0057915772580088 ) ) ;
#97544=CARTESIAN_POINT ( 'NONE',  ( -0.1681681984989999989, 1420.473120458229914, 172.2701767054979882 ) ) ;
#97550=CARTESIAN_POINT ( 'NONE',  ( -1.101868389151629879, 1419.744089616479869, 184.9570230273619984 ) ) ;
#97554=CARTESIAN_POINT ( 'NONE',  ( -18.75257229663529657, 1485.356831147769981, 189.3986093459970164 ) ) ;
#97556=CARTESIAN_POINT ( 'NONE',  ( -4.278522756227959967, 1441.024006130319776, 156.7060794043559895 ) ) ;
#97558=EDGE_LOOP ( 'NONE', ( #88320, #72187, #20742 ) ) ;
#97559=EDGE_CURVE ( 'NONE', #77737, #2271, #1010, .T. ) ;
#97560=ORIENTED_EDGE ( 'NONE', *, *, #82010, .T. ) ;
#97561=CARTESIAN_POINT ( 'NONE',  ( 29.21606581500000033, 1509.871156554629806, 209.9693792701380062 ) ) ;
#97566=CARTESIAN_POINT ( 'NONE',  ( -15.71040652243883784, 1410.149699372532723, 226.5306214444462398 ) ) ;
#97567=CARTESIAN_POINT ( 'NONE',  ( 0.8050666512040000056, 1507.647395255030006, 180.9817899904979868 ) ) ;
#97568=CARTESIAN_POINT ( 'NONE',  ( 11.88064286090000010, 1433.444786854229960, 151.0525681022980109 ) ) ;
#97569=CARTESIAN_POINT ( 'NONE',  ( -24.56616253283889861, 1451.897895543200093, 137.1355346205309900 ) ) ;
#97571=CARTESIAN_POINT ( 'NONE',  ( 4.379432440569999585, 1409.571163557129921, 231.2061471731980191 ) ) ;
#97574=CARTESIAN_POINT ( 'NONE',  ( 40.01221335447130656, 1438.828034964499921, 134.0999999981109738 ) ) ;
#97581=VERTEX_POINT ( 'NONE', #41609 ) ;
#97585=CARTESIAN_POINT ( 'NONE',  ( 21.11358352923581094, 1450.944576484996105, 144.3255025187013985 ) ) ;
#97588=EDGE_CURVE ( 'NONE', #57276, #106344, #76417, .T. ) ;
#97589=CARTESIAN_POINT ( 'NONE',  ( -18.52965084578502086, 1445.637233098631214, 214.4783539933714849 ) ) ;
#97592=CARTESIAN_POINT ( 'NONE',  ( -0.5988589654079999880, 1507.637957935130089, 231.7691613850980161 ) ) ;
#97594=CARTESIAN_POINT ( 'NONE',  ( 7.951680115159998508, 1415.087745006229852, 194.0123767119980016 ) ) ;
#97596=ORIENTED_EDGE ( 'NONE', *, *, #49480, .T. ) ;
#97599=CARTESIAN_POINT ( 'NONE',  ( 28.01520159380029895, 1440.913060387330006, 247.6253163881469845 ) ) ;
#97604=CARTESIAN_POINT ( 'NONE',  ( -13.16630813000000089, 1409.372837998530031, 190.8918809504980061 ) ) ;
#97605=CARTESIAN_POINT ( 'NONE',  ( -23.64337456402409998, 1435.765682558080016, 212.0350035351450231 ) ) ;
#97606=CARTESIAN_POINT ( 'NONE',  ( -24.39197164660000183, 1441.205372402069997, 211.3456893288379774 ) ) ;
#97607=CARTESIAN_POINT ( 'NONE',  ( -1.547462741870939906, 1414.913060391199906, 225.9340804956229931 ) ) ;
#97610=CARTESIAN_POINT ( 'NONE',  ( 12.67137506719999962, 1407.308516313030168, 266.8981195266979967 ) ) ;
#97613=CARTESIAN_POINT ( 'NONE',  ( 2.797472701710000287, 1464.949655032329929, 234.8291015129980224 ) ) ;
#97618=AXIS2_PLACEMENT_3D ( 'NONE', #49126, #82711, #6000 ) ;
#97619=CARTESIAN_POINT ( 'NONE',  ( 14.13195592840999915, 1452.421092199690065, 222.7290593210850034 ) ) ;
#97622=CARTESIAN_POINT ( 'NONE',  ( -18.24515611230000189, 1416.817366564930126, 208.9598336527209881 ) ) ;
#97623=CARTESIAN_POINT ( 'NONE',  ( -33.91369120143989591, 1451.728768194249824, 134.0999999980979851 ) ) ;
#97624=CARTESIAN_POINT ( 'NONE',  ( -24.20882859423510070, 1435.739118765830199, 210.8967395777180229 ) ) ;
#97625=ORIENTED_EDGE ( 'NONE', *, *, #101435, .F. ) ;
#97627=CARTESIAN_POINT ( 'NONE',  ( 12.80873346849999983, 1461.536424719429988, 232.0427772018979908 ) ) ;
#97628=CARTESIAN_POINT ( 'NONE',  ( -16.17568633703940151, 1459.146939663510011, 230.7169128052520080 ) ) ;
#97630=CARTESIAN_POINT ( 'NONE',  ( -1.418980099639949977, 1507.123641610349978, 237.1495972631439884 ) ) ;
#97632=CARTESIAN_POINT ( 'NONE',  ( -19.86788408629999836, 1444.803041715769950, 224.4210983673980024 ) ) ;
#97633=CARTESIAN_POINT ( 'NONE',  ( 5.360183379389989788, 1422.857591872020066, 148.0592648305490115 ) ) ;
#97636=ORIENTED_EDGE ( 'NONE', *, *, #56955, .F. ) ;
#97638=CARTESIAN_POINT ( 'NONE',  ( 1.769677292390000156, 1406.090449095429904, 269.0444970099979969 ) ) ;
#97640=AXIS2_PLACEMENT_3D ( 'NONE', #39974, #66312, #14209 ) ;
#97641=CARTESIAN_POINT ( 'NONE',  ( 31.82247306223929328, 1465.839566737470250, 269.9247011470700386 ) ) ;
#97646=CARTESIAN_POINT ( 'NONE',  ( 7.137524478430058217, 1442.009334510292774, 183.6365729105961861 ) ) ;
#97650=ORIENTED_EDGE ( 'NONE', *, *, #32569, .F. ) ;
#97651=CARTESIAN_POINT ( 'NONE',  ( -10.04572263220000039, 1417.623152644130187, 255.3819207682979595 ) ) ;
#97654=CARTESIAN_POINT ( 'NONE',  ( -0.1075775631909999946, 1475.837061347730014, 266.9611530679979978 ) ) ;
#97655=CARTESIAN_POINT ( 'NONE',  ( 0.0001132552782701080050, 1397.914756428169994, 209.1116890797569852 ) ) ;
#97657=CARTESIAN_POINT ( 'NONE',  ( -4.074356902468740493, 1448.298665946849042, 185.0948666590034009 ) ) ;
#97661=CARTESIAN_POINT ( 'NONE',  ( 26.79414221416690012, 1436.761946617690000, 136.7822070004859825 ) ) ;
#97662=CARTESIAN_POINT ( 'NONE',  ( -9.355712483234770005, 1396.239769066399958, 215.0244685633099948 ) ) ;
#97663=CARTESIAN_POINT ( 'NONE',  ( -14.79868613460000049, 1421.900788730430122, 227.7466242548979949 ) ) ;
#97664=CARTESIAN_POINT ( 'NONE',  ( 19.58542614618488997, 1455.481092546511491, 225.8721902375976640 ) ) ;
#97666=ORIENTED_EDGE ( 'NONE', *, *, #88999, .T. ) ;
#97669=CARTESIAN_POINT ( 'NONE',  ( -3.321447364419999548, 1484.261043626330093, 183.3707343507980170 ) ) ;
#97670=CARTESIAN_POINT ( 'NONE',  ( 11.30750857299999979, 1426.033734466129999, 121.0015455956980048 ) ) ;
#97673=CARTESIAN_POINT ( 'NONE',  ( 4.363119589138680254, 1423.854801764450031, 183.5697712894070150 ) ) ;
#97677=CARTESIAN_POINT ( 'NONE',  ( 3.300397815039999738, 1508.450664834530016, 180.9822841743979893 ) ) ;
#97678=CARTESIAN_POINT ( 'NONE',  ( 0.1620860067197200105, 1416.842625005220043, 190.8755133330550109 ) ) ;
#97685=CARTESIAN_POINT ( 'NONE',  ( -10.46857477760000066, 1397.317675341630093, 201.0163134539180305 ) ) ;
#97686=CARTESIAN_POINT ( 'NONE',  ( 0.8413093506324749171, 1490.956749009019859, 236.5476227179300110 ) ) ;
#97687=CARTESIAN_POINT ( 'NONE',  ( 1.910127611640000132E-10, 1497.713060387329961, 230.7369720342980202 ) ) ;
#97690=CARTESIAN_POINT ( 'NONE',  ( 12.98226713004290112, 1414.913060387349788, 198.3280232619060257 ) ) ;
#97691=CARTESIAN_POINT ( 'NONE',  ( 12.95120320960000093, 1410.293446051630099, 190.4598861209980214 ) ) ;
#97696=CARTESIAN_POINT ( 'NONE',  ( 36.08237879343099763, 1436.861740189970078, 136.4673732261519774 ) ) ;
#97697=CARTESIAN_POINT ( 'NONE',  ( 5.571677614479849439, 1396.107627656979957, 218.6505891727530013 ) ) ;
#97698=CARTESIAN_POINT ( 'NONE',  ( -40.23588547079999245, 1442.699308055779966, 137.0099670915980141 ) ) ;
#97699=CARTESIAN_POINT ( 'NONE',  ( -2.294228461334139713, 1406.102006316850066, 269.0439725548540082 ) ) ;
#97702=CARTESIAN_POINT ( 'NONE',  ( 3.697227707439999733, 1424.334605312130179, 184.5849975447979716 ) ) ;
#97703=CARTESIAN_POINT ( 'NONE',  ( 12.95770839519999917, 1442.886199328829889, 187.4929395404980141 ) ) ;
#97710=AXIS2_PLACEMENT_3D ( 'NONE', #38400, #46836, #11008 ) ;
#97712=CARTESIAN_POINT ( 'NONE',  ( -2.957532206020210275, 1509.097982660189700, 179.2610898709129970 ) ) ;
#97714=AXIS2_PLACEMENT_3D ( 'NONE', #89529, #81122, #32386 ) ;
#97715=EDGE_CURVE ( 'NONE', #28182, #46489, #99938, .T. ) ;
#97716=CARTESIAN_POINT ( 'NONE',  ( 0.3551208790259999803, 1416.218047894730262, 227.0926726479979720 ) ) ;
#97721=CARTESIAN_POINT ( 'NONE',  ( -3.160109254029999537, 1409.527913850729874, 232.2647705438980097 ) ) ;
#97722=CARTESIAN_POINT ( 'NONE',  ( -3.820292970859999772E-10, 1475.513060387329915, 188.4759928218979894 ) ) ;
#97724=CARTESIAN_POINT ( 'NONE',  ( 2.370970874524633398, 1427.002265528473799, 137.0999999980980135 ) ) ;
#97725=CARTESIAN_POINT ( 'NONE',  ( -26.88384131406899868, 1440.913060425529920, 226.2932696055459871 ) ) ;
#97728=CARTESIAN_POINT ( 'NONE',  ( 24.70944185802769866, 1416.032703119559756, 269.4189052401779918 ) ) ;
#97732=CARTESIAN_POINT ( 'NONE',  ( 23.62663202120000250, 1410.709074283629889, 207.9332156920780221 ) ) ;
#97733=CARTESIAN_POINT ( 'NONE',  ( 0.01963003285704640472, 1507.326971762890707, 237.3724487458281658 ) ) ;
#97738=CARTESIAN_POINT ( 'NONE',  ( 4.224193449673190770, 1421.807428560099879, 184.4466668902289825 ) ) ;
#97739=CARTESIAN_POINT ( 'NONE',  ( -0.4394933405940000259, 1417.920058205030045, 233.5085631684980001 ) ) ;
#97744=CARTESIAN_POINT ( 'NONE',  ( 19.86721287640000000, 1507.838653413830116, 189.0155849983980261 ) ) ;
#97747=CARTESIAN_POINT ( 'NONE',  ( 3.043251597425320032, 1417.779699503100119, 234.3208248802520188 ) ) ;
#97750=CARTESIAN_POINT ( 'NONE',  ( 19.08918182269999875, 1507.695925188030060, 188.5883432463980114 ) ) ;
#97754=CARTESIAN_POINT ( 'NONE',  ( -13.58268883541719951, 1416.851343898680170, 221.9096085506480165 ) ) ;
#97758=CARTESIAN_POINT ( 'NONE',  ( 10.55905614399324577, 1434.900330220869137, 152.0984994257607923 ) ) ;
#97761=CARTESIAN_POINT ( 'NONE',  ( 16.57223646264887051, 1421.748021482796958, 227.0899952749205966 ) ) ;
#97762=CARTESIAN_POINT ( 'NONE',  ( 4.408870434958439333, 1425.824683284920184, 185.4670092970000042 ) ) ;
#97763=CARTESIAN_POINT ( 'NONE',  ( -18.80544325660000027, 1424.672153923130054, 224.5457550954980093 ) ) ;
#97764=CARTESIAN_POINT ( 'NONE',  ( -14.55370911430000014, 1435.825179945700029, 149.7848083361979832 ) ) ;
#97766=CARTESIAN_POINT ( 'NONE',  ( 16.94063720780000182, 1507.935533863430010, 188.0799137801979839 ) ) ;
#97768=CARTESIAN_POINT ( 'NONE',  ( -18.89139539159507919, 1438.542556416878369, 210.7143975199735735 ) ) ;
#97771=CARTESIAN_POINT ( 'NONE',  ( -16.68463225830000241, 1442.773887286369927, 162.0935120917980043 ) ) ;
#97772=CARTESIAN_POINT ( 'NONE',  ( 11.71103087170000023, 1438.058396846869982, 147.7520216503980066 ) ) ;
#97777=CARTESIAN_POINT ( 'NONE',  ( 17.83228018670000026, 1408.913060387329779, 213.2813548218979918 ) ) ;
#97778=CARTESIAN_POINT ( 'NONE',  ( -0.2658540493943280514, 1507.120020986029886, 237.3289608297170048 ) ) ;
#97785=EDGE_LOOP ( 'NONE', ( #31058, #104432, #23391, #60074 ) ) ;
#97788=ORIENTED_EDGE ( 'NONE', *, *, #86568, .F. ) ;
#97792=CARTESIAN_POINT ( 'NONE',  ( -4.363123796622770278, 1423.854800546939941, 184.2546035468919854 ) ) ;
#97793=CARTESIAN_POINT ( 'NONE',  ( 24.21285743589101358, 1415.977151558922287, 269.4183131582149713 ) ) ;
#97794=CARTESIAN_POINT ( 'NONE',  ( -26.00754374419999948, 1454.033399687029942, 240.2274372898979777 ) ) ;
#97795=CARTESIAN_POINT ( 'NONE',  ( -20.12493411150000000, 1494.494608803829806, 190.1457493620980017 ) ) ;
#97796=CARTESIAN_POINT ( 'NONE',  ( -11.91877802890000027, 1433.473306471390060, 150.2081219906980039 ) ) ;
#97797=CARTESIAN_POINT ( 'NONE',  ( 27.93020545470000471, 1509.888404654830083, 203.8551627510279900 ) ) ;
#97798=CARTESIAN_POINT ( 'NONE',  ( -19.19211169099999736, 1486.006664573430044, 189.6295759001980343 ) ) ;
#97802=CARTESIAN_POINT ( 'NONE',  ( -18.65451756193940014, 1507.632629711779828, 229.7110761618599781 ) ) ;
#97805=CARTESIAN_POINT ( 'NONE',  ( -8.333801363508515081, 1509.331394084260182, 237.9487518140551003 ) ) ;
#97806=CARTESIAN_POINT ( 'NONE',  ( 1.219850571415770094E-08, 1406.911344650290175, 265.1958365716640174 ) ) ;
#97808=ORIENTED_EDGE ( 'NONE', *, *, #83871, .T. ) ;
#97811=CARTESIAN_POINT ( 'NONE',  ( -32.97295502609999573, 1460.269649532029916, 269.5004837624980496 ) ) ;
#97812=CARTESIAN_POINT ( 'NONE',  ( -23.75022901606470782, 1436.081403467656173, 211.7336246957814296 ) ) ;
#97814=CARTESIAN_POINT ( 'NONE',  ( 35.01754215041950147, 1450.340935123170084, 136.2235620930159996 ) ) ;
#97816=CARTESIAN_POINT ( 'NONE',  ( -11.76065867670000031, 1420.498107173830022, 231.0157263700980081 ) ) ;
#97819=CARTESIAN_POINT ( 'NONE',  ( -1.136808998351487521, 1484.762897349236027, 182.1973289732482044 ) ) ;
#97821=CARTESIAN_POINT ( 'NONE',  ( -45.84226277833369778, 1436.715131148009959, 266.9824418670360160 ) ) ;
#97823=CARTESIAN_POINT ( 'NONE',  ( -3.534759143276439808, 1493.082786438550102, 181.5750439270630068 ) ) ;
#97824=EDGE_LOOP ( 'NONE', ( #33063, #102690, #85005, #61654, #23060, #104590 ) ) ;
#97828=CARTESIAN_POINT ( 'NONE',  ( -20.86053628100000168, 1508.959219212030121, 190.3806355066980132 ) ) ;
#97829=CARTESIAN_POINT ( 'NONE',  ( -15.95571536889999997, 1410.408223877029968, 191.3274944925979923 ) ) ;
#97831=CARTESIAN_POINT ( 'NONE',  ( -16.68599136316429821, 1461.161685576650143, 228.2799817407029934 ) ) ;
#97832=ORIENTED_EDGE ( 'NONE', *, *, #41943, .T. ) ;
#97834=CARTESIAN_POINT ( 'NONE',  ( 18.49117120320514829, 1508.844092022591212, 188.2543554909499335 ) ) ;
#97836=ORIENTED_EDGE ( 'NONE', *, *, #21990, .T. ) ;
#97837=CARTESIAN_POINT ( 'NONE',  ( -9.478344589416581201, 1411.163298180099900, 269.3460365866420148 ) ) ;
#97838=CARTESIAN_POINT ( 'NONE',  ( -0.7352107454670000486, 1428.413060387330006, 91.31218443469779800 ) ) ;
#97843=CARTESIAN_POINT ( 'NONE',  ( 42.08257328447562884, 1454.145434094863049, 269.0735840997347736 ) ) ;
#97844=EDGE_CURVE ( 'NONE', #99650, #95096, #77158, .T. ) ;
#97848=CARTESIAN_POINT ( 'NONE',  ( -1.456328368119999883, 1485.358061632029830, 182.2073493714979975 ) ) ;
#97849=AXIS2_PLACEMENT_3D ( 'NONE', #73105, #22104, #107245 ) ;
#97850=CARTESIAN_POINT ( 'NONE',  ( -17.27558692971449972, 1507.606285623229951, 224.2552697136770234 ) ) ;
#97851=CARTESIAN_POINT ( 'NONE',  ( -17.97429972279999788, 1430.800360081030249, 226.3842136923979922 ) ) ;
#97852=CARTESIAN_POINT ( 'NONE',  ( 15.83383049623899730, 1474.212651018609904, 267.1442246111369627 ) ) ;
#97853=CARTESIAN_POINT ( 'NONE',  ( 12.26979136719999985, 1416.828040475729949, 223.5793546564979977 ) ) ;
#97854=CARTESIAN_POINT ( 'NONE',  ( 4.129912672550000607, 1446.242909026189864, 182.6856816074980259 ) ) ;
#97856=ORIENTED_EDGE ( 'NONE', *, *, #74134, .F. ) ;
#97859=ORIENTED_EDGE ( 'NONE', *, *, #40161, .F. ) ;
#97860=CARTESIAN_POINT ( 'NONE',  ( 17.87824514789634023, 1457.869968850633313, 229.1928660838007659 ) ) ;
#97862=CARTESIAN_POINT ( 'NONE',  ( 13.56343219680000090, 1416.311719779230089, 196.3989970432979817 ) ) ;
#97864=CARTESIAN_POINT ( 'NONE',  ( 20.10486353479999977, 1410.110232032130170, 198.1151493261979795 ) ) ;
#97865=CARTESIAN_POINT ( 'NONE',  ( 16.68463233076019492, 1445.052233488289176, 162.0935120523188289 ) ) ;
#97866=CARTESIAN_POINT ( 'NONE',  ( -26.28380303640000193, 1435.415400226489737, 135.3026382325979853 ) ) ;
#97868=CARTESIAN_POINT ( 'NONE',  ( 0.7827416214407210138, 1450.881275464169903, 181.6854931341780173 ) ) ;
#97874=B_SPLINE_CURVE_WITH_KNOTS ( 'NONE', 3,
 ( #58593, #69205, #75931, #102226, #51279, #102757 ),
 .UNSPECIFIED., .F., .F.,
 ( 4, 2, 4 ),
 ( -0.02784762759737050009, -0.01392846439159300086, 0.000000000000000000 ),
 .UNSPECIFIED. ) ;
#97877=CARTESIAN_POINT ( 'NONE',  ( -3.134084166701379903, 1421.411054285269984, 144.1517906398860021 ) ) ;
#97879=CARTESIAN_POINT ( 'NONE',  ( -39.85544913743839857, 1446.150425910739841, 136.7763567636360165 ) ) ;
#97881=CARTESIAN_POINT ( 'NONE',  ( 11.60004869885203682, 1425.937227630464349, 137.5819683612840834 ) ) ;
#97882=CARTESIAN_POINT ( 'NONE',  ( 3.002008659228135201, 1417.785699668546158, 234.2809593874903555 ) ) ;
#97883=CARTESIAN_POINT ( 'NONE',  ( 17.92678331089475208, 1423.916767532210088, 225.7531818707438731 ) ) ;
#97886=CARTESIAN_POINT ( 'NONE',  ( -34.79013702040099787, 1462.198988287599832, 269.8693405702829864 ) ) ;
#97887=CARTESIAN_POINT ( 'NONE',  ( 36.66684616735739155, 1440.913060387340010, 254.0481763504310209 ) ) ;
#97893=AXIS2_PLACEMENT_3D ( 'NONE', #57007, #109058, #73807 ) ;
#97894=CARTESIAN_POINT ( 'NONE',  ( -19.11224328149206642, 1485.525743910654683, 189.6460228031468773 ) ) ;
#97896=CARTESIAN_POINT ( 'NONE',  ( 1.901185863359999839, 1498.995677176629897, 235.9662232939979845 ) ) ;
#97898=DIRECTION ( 'NONE',  ( 0.000000000000000000, -1.000000000000000000, 0.000000000000000000 ) ) ;
#97899=CARTESIAN_POINT ( 'NONE',  ( -8.313149309269999065, 1507.316766614329936, 235.1568494565980245 ) ) ;
#97902=EDGE_CURVE ( 'NONE', #15423, #99871, #58531, .T. ) ;
#97907=CARTESIAN_POINT ( 'NONE',  ( -0.7975830076839999228, 1452.841034471829971, 183.3931114573979926 ) ) ;
#97916=B_SPLINE_CURVE_WITH_KNOTS ( 'NONE', 5,
 ( #80667, #30799, #90701, #13988, #39764, #73371 ),
 .UNSPECIFIED., .F., .F.,
 ( 6, 6 ),
 ( 0.5082988451364722771, 1.000000000000000000 ),
 .UNSPECIFIED. ) ;
#97924=CIRCLE ( 'NONE', #76438, 30.60516481925333210 ) ;
#97925=CARTESIAN_POINT ( 'NONE',  ( 6.765186941703619894, 1409.149305921059749, 195.7697136597590202 ) ) ;
#97926=CARTESIAN_POINT ( 'NONE',  ( 18.52339265480000208, 1425.745301197430081, 224.9617099063980277 ) ) ;
#97930=CARTESIAN_POINT ( 'NONE',  ( -3.885481994197490074, 1448.980853271389833, 185.0328430115930018 ) ) ;
#97931=ORIENTED_EDGE ( 'NONE', *, *, #10317, .T. ) ;
#97932=VERTEX_POINT ( 'NONE', #63945 ) ;
#97934=CARTESIAN_POINT ( 'NONE',  ( -12.25713978275359928, 1416.640375558050209, 194.6766261173120256 ) ) ;
#97936=CARTESIAN_POINT ( 'NONE',  ( -5.906668414434429117E-11, 1466.311335111799963, 242.6050078029819872 ) ) ;
#97937=CARTESIAN_POINT ( 'NONE',  ( -20.33293110796009984, 1499.214264760269998, 190.6403736919519929 ) ) ;
#97938=CARTESIAN_POINT ( 'NONE',  ( 1.195323752479999779, 1396.139239339430105, 221.0537008139980060 ) ) ;
#97939=CARTESIAN_POINT ( 'NONE',  ( 19.16007812963110268, 1428.477567333490015, 209.6896849280039987 ) ) ;
#97940=CARTESIAN_POINT ( 'NONE',  ( -1.438892276100000034, 1452.191226728930133, 183.8587014809980076 ) ) ;
#97942=CARTESIAN_POINT ( 'NONE',  ( -26.53975464933690986, 1436.733422015536462, 136.8030177142773880 ) ) ;
#97943=CARTESIAN_POINT ( 'NONE',  ( -22.15347906188290139, 1496.414302325609924, 208.5267879710629870 ) ) ;
#97945=AXIS2_PLACEMENT_3D ( 'NONE', #104565, #60934, #95612 ) ;
#97946=CARTESIAN_POINT ( 'NONE',  ( 11.93966352644169859, 1433.552769406360085, 150.1888638864129746 ) ) ;
#97947=CARTESIAN_POINT ( 'NONE',  ( -13.30603026154990154, 1434.901373284009878, 148.9434964573779894 ) ) ;
#97949=CARTESIAN_POINT ( 'NONE',  ( 16.34466203799999917, 1409.483828562729968, 193.4811910679979974 ) ) ;
#97953=CARTESIAN_POINT ( 'NONE',  ( 38.77640762290000254, 1433.500815606669903, 259.1404900223979553 ) ) ;
#97954=CARTESIAN_POINT ( 'NONE',  ( -24.71942444569999964, 1469.238022050230029, 202.0311767578679962 ) ) ;
#97955=CARTESIAN_POINT ( 'NONE',  ( -10.46183320403099870, 1425.378319878120010, 99.91631404394871652 ) ) ;
#97957=B_SPLINE_CURVE_WITH_KNOTS ( 'NONE', 3,
 ( #55925, #21723, #90045, #4944, #13880, #5504, #46977, #106845, #39662, #91710 ),
 .UNSPECIFIED., .F., .F.,
 ( 4, 2, 2, 2, 4 ),
 ( 0.000000000000000000, 0.2500000000000000000, 0.5000000000000000000, 0.7500000000000000000, 1.000000000000000000 ),
 .UNSPECIFIED. ) ;
#97958=CARTESIAN_POINT ( 'NONE',  ( -19.44405420005750074, 1410.830242043655289, 270.0540949853959205 ) ) ;
#97959=CARTESIAN_POINT ( 'NONE',  ( -7.831970043950000182, 1421.243762745730010, 220.7330770330979988 ) ) ;
#97961=CARTESIAN_POINT ( 'NONE',  ( 2.503416217964581580, 1448.820465288596779, 154.6001883531548344 ) ) ;
#97962=CARTESIAN_POINT ( 'NONE',  ( 27.43975379009999926, 1451.094596967429879, 136.3642754792980156 ) ) ;
#97964=CARTESIAN_POINT ( 'NONE',  ( 3.763296693692190331, 1398.025494293209931, 196.0977038891449808 ) ) ;
#97966=CARTESIAN_POINT ( 'NONE',  ( 38.20494153861019981, 1442.993962785479880, 137.1161392804919785 ) ) ;
#97972=EDGE_CURVE ( 'NONE', #24298, #99485, #33109, .T. ) ;
#97978=CARTESIAN_POINT ( 'NONE',  ( -3.203421013219999836, 1479.771999117829864, 235.5522340181979928 ) ) ;
#97982=CARTESIAN_POINT ( 'NONE',  ( 46.15241393044949803, 1440.912967216340121, 268.2045458581380331 ) ) ;
#97983=CARTESIAN_POINT ( 'NONE',  ( -12.50318290573809854, 1415.427621830080170, 221.4521480450309809 ) ) ;
#97984=CARTESIAN_POINT ( 'NONE',  ( 0.04457229829839999546, 1420.440674599429940, 183.2993309066980032 ) ) ;
#97986=ORIENTED_EDGE ( 'NONE', *, *, #59080, .T. ) ;
#97989=CARTESIAN_POINT ( 'NONE',  ( 13.42118519619293160, 1443.449014888631837, 187.9204824381897083 ) ) ;
#97991=EDGE_LOOP ( 'NONE', ( #43201, #45445, #38577, #50533 ) ) ;
#97996=CARTESIAN_POINT ( 'NONE',  ( 20.82408115712189911, 1452.185867449390116, 142.2070257201390007 ) ) ;
#98000=CARTESIAN_POINT ( 'NONE',  ( -20.29127127059840063, 1509.661394863832811, 230.8411074860736960 ) ) ;
#98006=CARTESIAN_POINT ( 'NONE',  ( -24.42411529408670035, 1509.071565208550055, 222.5078051949110147 ) ) ;
#98008=ORIENTED_EDGE ( 'NONE', *, *, #10390, .T. ) ;
#98009=CARTESIAN_POINT ( 'NONE',  ( 27.19819524420000079, 1434.390360741930181, 248.0989693021979861 ) ) ;
#98010=CARTESIAN_POINT ( 'NONE',  ( -3.835404308833623155, 1396.046995657106436, 202.1011854665750036 ) ) ;
#98019=CARTESIAN_POINT ( 'NONE',  ( -7.341316150999999179E-16, 1441.600846913620217, 150.7224806086979640 ) ) ;
#98026=CARTESIAN_POINT ( 'NONE',  ( 16.69334696330000156, 1419.771389454430164, 226.9180811344979816 ) ) ;
#98028=AXIS2_PLACEMENT_3D ( 'NONE', #73045, #3108, #80344 ) ;
#98031=CARTESIAN_POINT ( 'NONE',  ( 46.16778666300000111, 1438.897380407539913, 266.9714988366979469 ) ) ;
#98032=CARTESIAN_POINT ( 'NONE',  ( -17.45742012540000232, 1409.522686931430144, 222.8493455500980076 ) ) ;
#98033=CARTESIAN_POINT ( 'NONE',  ( 19.95725839569999849, 1436.009163759079911, 145.3713295913979948 ) ) ;
#98034=CARTESIAN_POINT ( 'NONE',  ( 4.652384135149589817, 1440.963318168330034, 155.5568921565159997 ) ) ;
#98035=EDGE_CURVE ( 'NONE', #79540, #96354, #88892, .T. ) ;
#98036=CARTESIAN_POINT ( 'NONE',  ( -16.40119657999539982, 1409.652435746110086, 192.2255775475670134 ) ) ;
#98039=CARTESIAN_POINT ( 'NONE',  ( -38.70772116073620595, 1437.296229215239919, 135.0862262929739757 ) ) ;
#98040=CARTESIAN_POINT ( 'NONE',  ( 0.2114665854462480232, 1456.524817466450031, 183.1021823691539794 ) ) ;
#98041=CARTESIAN_POINT ( 'NONE',  ( -13.29060849360579866, 1407.754373188279942, 210.5456034691529794 ) ) ;
#98042=CARTESIAN_POINT ( 'NONE',  ( -14.33002530880000158, 1414.913060387329779, 201.6311097326980075 ) ) ;
#98045=CARTESIAN_POINT ( 'NONE',  ( 12.91331072740000074, 1434.774329726679980, 147.2731663809980205 ) ) ;
#98046=CARTESIAN_POINT ( 'NONE',  ( -38.53505232114799384, 1437.347470674169926, 134.0999999971709826 ) ) ;
#98047=DIRECTION ( 'NONE',  ( -0.8926073982886787439, 0.4508348173337058951, 0.000000000000000000 ) ) ;
#98050=CARTESIAN_POINT ( 'NONE',  ( 40.40805859990000215, 1443.620986539019896, 137.1126368707979850 ) ) ;
#98055=CARTESIAN_POINT ( 'NONE',  ( 13.36711898873540072, 1508.094956433400057, 233.0794756770270055 ) ) ;
#98056=CARTESIAN_POINT ( 'NONE',  ( 40.50869282367309410, 1425.163924263866193, 269.1154144834585509 ) ) ;
#98060=CARTESIAN_POINT ( 'NONE',  ( -26.61732439379999704, 1507.999000608030201, 214.1432811199779849 ) ) ;
#98067=CARTESIAN_POINT ( 'NONE',  ( -27.02655704099999667, 1451.108971386630174, 136.3738572239980158 ) ) ;
#98070=VERTEX_POINT ( 'NONE', #95597 ) ;
#98073=CARTESIAN_POINT ( 'NONE',  ( 4.063344664623878444, 1421.082680532014365, 137.4056175706463705 ) ) ;
#98075=CARTESIAN_POINT ( 'NONE',  ( -11.90129930089999988, 1415.245980409429876, 195.5451049489979880 ) ) ;
#98076=CARTESIAN_POINT ( 'NONE',  ( -14.03757963822240029, 1511.404482726790093, 183.4262285374240093 ) ) ;
#98077=CARTESIAN_POINT ( 'NONE',  ( 23.17009332390000154, 1410.217324300129803, 212.3038800746780055 ) ) ;
#98078=CARTESIAN_POINT ( 'NONE',  ( -1.974599305947250194, 1419.504832324920244, 185.8215509651549837 ) ) ;
#98081=CARTESIAN_POINT ( 'NONE',  ( -10.98084428610000174, 1433.016922418659988, 151.7694244828979890 ) ) ;
#98083=CARTESIAN_POINT ( 'NONE',  ( 26.02702435453459984, 1469.349391678469829, 207.6976918991759931 ) ) ;
#98090=CARTESIAN_POINT ( 'NONE',  ( -4.404857644985120224, 1485.524168335080049, 183.0886271376960224 ) ) ;
#98094=ORIENTED_EDGE ( 'NONE', *, *, #24941, .F. ) ;
#98095=CARTESIAN_POINT ( 'NONE',  ( 27.78931436370000085, 1508.066562786630129, 211.8879754161380333 ) ) ;
#98097=CARTESIAN_POINT ( 'NONE',  ( 7.316304296407109220, 1507.280216653023899, 182.6970439867345704 ) ) ;
#98098=CARTESIAN_POINT ( 'NONE',  ( 1.499372387982010224, 1414.913526845469960, 192.0176458413389753 ) ) ;
#98100=CARTESIAN_POINT ( 'NONE',  ( 15.92940539777539932, 1419.249169548590089, 191.2576731443239737 ) ) ;
#98101=CARTESIAN_POINT ( 'NONE',  ( 0.9350669245199999535, 1508.880473741730157, 179.9494619221979974 ) ) ;
#98103=CARTESIAN_POINT ( 'NONE',  ( -24.49684469894179983, 1452.057661785150003, 136.0510194727069972 ) ) ;
#98105=CARTESIAN_POINT ( 'NONE',  ( 4.165142600520000293, 1409.058510372029787, 229.9895894434979766 ) ) ;
#98108=CARTESIAN_POINT ( 'NONE',  ( 39.77086280987219880, 1438.526156309450016, 134.0999999980039945 ) ) ;
#98110=ORIENTED_EDGE ( 'NONE', *, *, #26715, .F. ) ;
#98114=ORIENTED_EDGE ( 'NONE', *, *, #17886, .F. ) ;
#98115=ORIENTED_EDGE ( 'NONE', *, *, #102497, .F. ) ;
#98116=CARTESIAN_POINT ( 'NONE',  ( 12.50587472938863876, 1410.723098928997388, 228.7755205085364878 ) ) ;
#98118=ADVANCED_FACE ( 'NONE', ( #25612 ), #27757, .F. ) ;
#98119=CARTESIAN_POINT ( 'NONE',  ( 1.817252217737630682, 1451.599092923090211, 154.0952177214090568 ) ) ;
#98121=CARTESIAN_POINT ( 'NONE',  ( -17.48093814192715101, 1448.293137033754647, 218.1689033131428346 ) ) ;
#98124=CARTESIAN_POINT ( 'NONE',  ( 9817.198718245359487, 2837.742859962510011, 1424.354596153399825 ) ) ;
#98125=CARTESIAN_POINT ( 'NONE',  ( 10.47220851269999997, 1415.931784856029935, 194.6558979389980095 ) ) ;
#98127=VERTEX_POINT ( 'NONE', #19426 ) ;
#98128=( BOUNDED_CURVE ( )  B_SPLINE_CURVE ( 3, ( #1025, #9950, #35150, #61485 ),
 .UNSPECIFIED., .F., .T. ) 
 B_SPLINE_CURVE_WITH_KNOTS ( ( 4, 4 ),
 ( 4.710628272208039924, 4.725173297074450218 ),
 .UNSPECIFIED. ) 
 CURVE ( )  GEOMETRIC_REPRESENTATION_ITEM ( )  RATIONAL_B_SPLINE_CURVE ( ( 1.000000000000000000, 0.9999823702653387603, 0.9999823702653387603, 1.000000000000000000 ) ) 
 REPRESENTATION_ITEM ( '' )  );
#98131=CARTESIAN_POINT ( 'NONE',  ( 34.82393780566600583, 1440.913060387330006, 260.5799695211790095 ) ) ;
#98133=CARTESIAN_POINT ( 'NONE',  ( -0.0002195400984297455574, 1452.178648969947972, 153.8655588343418117 ) ) ;
#98134=ORIENTED_EDGE ( 'NONE', *, *, #31550, .T. ) ;
#98135=CARTESIAN_POINT ( 'NONE',  ( -0.3153013721334770314, 1450.902049820790126, 181.2539182818010204 ) ) ;
#98136=CARTESIAN_POINT ( 'NONE',  ( -15.37044282969999998, 1410.822167989630088, 190.9607351025979938 ) ) ;
#98138=CARTESIAN_POINT ( 'NONE',  ( -24.41227777330000137, 1441.083062867809986, 212.0377087122379862 ) ) ;
#98140=EDGE_CURVE ( 'NONE', #55469, #89451, #73188, .T. ) ;
#98141=CARTESIAN_POINT ( 'NONE',  ( -21.39772323737049931, 1509.704958956720020, 229.7894127843639751 ) ) ;
#98142=CARTESIAN_POINT ( 'NONE',  ( -3.666695921210000098, 1509.114858860330060, 179.5219325993979851 ) ) ;
#98143=CARTESIAN_POINT ( 'NONE',  ( -13.50138217389999973, 1434.968982414120092, 147.1506466749980007 ) ) ;
#98145=CARTESIAN_POINT ( 'NONE',  ( 10.02061939940000102, 1462.780975112430042, 234.0615248113979874 ) ) ;
#98146=DIRECTION ( 'NONE',  ( -1.058776845917449781E-11, -0.4875922911319906516, 0.8730714504716415858 ) ) ;
#98152=CARTESIAN_POINT ( 'NONE',  ( -0.1363338795402929959, 1507.779362083510023, 180.7572018573229968 ) ) ;
#98154=CARTESIAN_POINT ( 'NONE',  ( 19.14623459136682726, 1443.795870015896298, 213.6165435391197889 ) ) ;
#98156=CARTESIAN_POINT ( 'NONE',  ( -21.25073931209999856, 1488.812149333029993, 209.2107079651389938 ) ) ;
#98159=ORIENTED_EDGE ( 'NONE', *, *, #87030, .T. ) ;
#98161=CARTESIAN_POINT ( 'NONE',  ( 24.59498549390000122, 1442.535575187109998, 213.3385281511980054 ) ) ;
#98162=EDGE_CURVE ( 'NONE', #59669, #20723, #83881, .T. ) ;
#98165=CARTESIAN_POINT ( 'NONE',  ( 2.671395959200000281, 1410.370854059430030, 231.6673943366980097 ) ) ;
#98167=CARTESIAN_POINT ( 'NONE',  ( -20.52383102562189876, 1473.184607215510141, 209.4975910873509974 ) ) ;
#98170=CARTESIAN_POINT ( 'NONE',  ( -23.57099603410000199, 1444.794699592119969, 214.9951603828779980 ) ) ;
#98171=CARTESIAN_POINT ( 'NONE',  ( 5.364000998215719740, 1424.961930034630086, 151.4178908013030309 ) ) ;
#98172=CARTESIAN_POINT ( 'NONE',  ( -1.735729300940000108, 1484.732890180429877, 182.7347388233980041 ) ) ;
#98173=AXIS2_PLACEMENT_3D ( 'NONE', #100591, #14375, #91096 ) ;
#98174=ORIENTED_EDGE ( 'NONE', *, *, #76825, .T. ) ;
#98176=CARTESIAN_POINT ( 'NONE',  ( 0.8897778044439998979, 1405.723157296330101, 267.8536995184980469 ) ) ;
#98178=EDGE_CURVE ( 'NONE', #42283, #43923, #76496, .T. ) ;
#98179=CARTESIAN_POINT ( 'NONE',  ( 20.62267221016178453, 1427.503558244864962, 220.3768387070393260 ) ) ;
#98181=CARTESIAN_POINT ( 'NONE',  ( 11.60004869893070278, 1424.990909871714166, 137.7500050950981176 ) ) ;
#98182=B_SPLINE_CURVE_WITH_KNOTS ( 'NONE', 3,
 ( #6038, #108498, #15513, #48050 ),
 .UNSPECIFIED., .F., .F.,
 ( 4, 4 ),
 ( 0.000000000000000000, 1.000000000000000000 ),
 .UNSPECIFIED. ) ;
#98186=CARTESIAN_POINT ( 'NONE',  ( 0.8745088156686119385, 1450.882521866549951, 155.0623987374809758 ) ) ;
#98188=CARTESIAN_POINT ( 'NONE',  ( 17.27558691658489920, 1507.606285602530079, 193.9884222186300065 ) ) ;
#98189=CARTESIAN_POINT ( 'NONE',  ( -26.42714720800000094, 1440.913060387330006, 243.9198229517980110 ) ) ;
#98190=EDGE_CURVE ( 'NONE', #19628, #69349, #15634, .T. ) ;
#98192=CARTESIAN_POINT ( 'NONE',  ( 3.653351625370000022, 1441.538476220570146, 168.7225134348979907 ) ) ;
#98193=CARTESIAN_POINT ( 'NONE',  ( -0.1081014814999999990, 1476.109324709130078, 267.8540375961979407 ) ) ;
#98194=CARTESIAN_POINT ( 'NONE',  ( -30.93305835920000035, 1451.832845973630128, 134.8030507067980182 ) ) ;
#98195=CARTESIAN_POINT ( 'NONE',  ( -19.87223104929999806, 1484.291808912129909, 191.2808552885979907 ) ) ;
#98197=DIRECTION ( 'NONE',  ( -0.5450600352769339185, 0.8383970168982638471, 0.000000000000000000 ) ) ;
#98201=B_SPLINE_SURFACE_WITH_KNOTS ( 'NONE', 5, 5, ( 
 ( #105519, #60781, #70295, #10907, #3082, #26584 ),
 ( #87620, #95459, #96566, #61887, #20383, #10338 ),
 ( #44511, #86495, #865, #94905, #78658, #28808 ),
 ( #2532, #62441, #79223, #54585, #45081, #1401 ),
 ( #11461, #78098, #69171, #1973, #61339, #45636 ),
 ( #97114, #19272, #103854, #96003, #19838, #88721 ),
 ( #71403, #69736, #36110, #54043, #104960, #53477 ),
 ( #36653, #46184, #104407, #12003, #27153, #9789 ),
 ( #103277, #70850, #18180, #52375, #34990, #28249 ) ),
 .UNSPECIFIED., .F., .F., .F.,
 ( 6, 3, 6 ),
 ( 6, 6 ),
 ( 0.7655572723440000615, 2.316155491860000026, 3.835724788559999876 ),
 ( 0.000000000000000000, 1.000000000000000000 ),
 .UNSPECIFIED. ) ;
#98204=CARTESIAN_POINT ( 'NONE',  ( 24.02863916850529691, 1507.902931906480035, 195.9323055859989893 ) ) ;
#98205=CARTESIAN_POINT ( 'NONE',  ( -10.21954854673889912, 1396.269934886460078, 213.3624866545780208 ) ) ;
#98206=ADVANCED_FACE ( 'NONE', ( #331 ), #81450, .T. ) ;
#98207=CARTESIAN_POINT ( 'NONE',  ( -15.20897926109999965, 1420.729871092930125, 227.0317324019979992 ) ) ;
#98209=CARTESIAN_POINT ( 'NONE',  ( -44.74160412339999482, 1437.880769410919811, 269.6947547460979990 ) ) ;
#98212=CARTESIAN_POINT ( 'NONE',  ( 2.113412023180000432, 1409.489867608229815, 231.6724619568979904 ) ) ;
#98214=CARTESIAN_POINT ( 'NONE',  ( 11.31574024959999925, 1425.558402394630093, 135.9181065939980044 ) ) ;
#98220=CARTESIAN_POINT ( 'NONE',  ( -7.276969490589999978, 1429.103926496630038, 148.8100812095979961 ) ) ;
#98221=CARTESIAN_POINT ( 'NONE',  ( 5.784760235850000321, 1509.027726486529900, 180.8299671665979815 ) ) ;
#98228=CARTESIAN_POINT ( 'NONE',  ( -6.240887352569999713, 1397.787773555530066, 197.7178371984979890 ) ) ;
#98231=CARTESIAN_POINT ( 'NONE',  ( 1.626544742530000143, 1508.996462000230167, 238.7123361027979911 ) ) ;
#98232=CARTESIAN_POINT ( 'NONE',  ( -13.48183417829717712, 1444.195713017638354, 169.3584165285456606 ) ) ;
#98233=CARTESIAN_POINT ( 'NONE',  ( 14.59882275810000074, 1475.513060387329915, 225.1032622602980098 ) ) ;
#98236=CARTESIAN_POINT ( 'NONE',  ( -1.357402501670849970, 1410.996727195599988, 185.5758023988580021 ) ) ;
#98238=CARTESIAN_POINT ( 'NONE',  ( 6.075489283959999653, 1410.296875220730044, 186.7884348254980011 ) ) ;
#98240=CARTESIAN_POINT ( 'NONE',  ( -39.72761531382059275, 1447.484040599029868, 136.5504236487229832 ) ) ;
#98242=CARTESIAN_POINT ( 'NONE',  ( 10.03865112700490059, 1396.263617810830056, 213.7795285193350026 ) ) ;
#98243=CARTESIAN_POINT ( 'NONE',  ( -27.31524396653970044, 1439.464577282379878, 137.0827076382539929 ) ) ;
#98244=CARTESIAN_POINT ( 'NONE',  ( 11.53548580120000011, 1429.271495510729892, 150.4873605658980011 ) ) ;
#98245=CARTESIAN_POINT ( 'NONE',  ( -18.90950359435113270, 1416.818673872099680, 208.2952427945739373 ) ) ;
#98247=FACE_OUTER_BOUND ( 'NONE', #73986, .T. ) ;
#98251=CARTESIAN_POINT ( 'NONE',  ( -19.07245837269699962, 1478.089605352000035, 228.2662948790070061 ) ) ;
#98253=VECTOR ( 'NONE', #63499, 1000.000000000000000 ) ;
#98254=CARTESIAN_POINT ( 'NONE',  ( -14.05029935760000015, 1452.819461534730181, 195.3943816284979960 ) ) ;
#98255=DIRECTION ( 'NONE',  ( 0.000000000000000000, 1.000000000000000000, 0.000000000000000000 ) ) ;
#98259=CARTESIAN_POINT ( 'NONE',  ( -11.56386820771918522, 1426.103378762827333, 138.8479550929265258 ) ) ;
#98260=CARTESIAN_POINT ( 'NONE',  ( 0.05328461806629999908, 1509.045414532929954, 179.1219818357980103 ) ) ;
#98262=CARTESIAN_POINT ( 'NONE',  ( 15.99522875749999962, 1414.971279908829956, 214.8034238970980141 ) ) ;
#98265=CIRCLE ( 'NONE', #80377, 1.999999954277511760 ) ;
#98267=CARTESIAN_POINT ( 'NONE',  ( -38.90097543864180807, 1429.363953125564649, 269.5912681143711325 ) ) ;
#98271=CARTESIAN_POINT ( 'NONE',  ( -0.001812510741418579775, 1450.927551375689745, 181.5184721789159994 ) ) ;
#98272=CARTESIAN_POINT ( 'NONE',  ( -32.17164623804170276, 1440.913060389470047, 244.5574100837299909 ) ) ;
#98274=CARTESIAN_POINT ( 'NONE',  ( -0.5431522787170589561, 1465.104810438569984, 238.0938638197280000 ) ) ;
#98275=CARTESIAN_POINT ( 'NONE',  ( 34.45372861117999719, 1422.622881628830100, 269.5160893324709832 ) ) ;
#98278=CARTESIAN_POINT ( 'NONE',  ( 23.21876702530000358, 1409.984068931529919, 208.2209878805410028 ) ) ;
#98284=CARTESIAN_POINT ( 'NONE',  ( -5.218238568920000375, 1417.907702606829844, 232.1391919757979849 ) ) ;
#98286=EDGE_LOOP ( 'NONE', ( #40752, #77788, #51271, #15092 ) ) ;
#98291=ADVANCED_FACE ( 'NONE', ( #58433 ), #66847, .T. ) ;
#98303=LINE ( 'NONE', #29991, #109146 ) ;
#98306=DIRECTION ( 'NONE',  ( -0.2020439960283723635, -0.9583089376822325756, -0.2020450534589698921 ) ) ;
#98307=CARTESIAN_POINT ( 'NONE',  ( 10.96098658911311752, 1434.305190191134670, 151.7979222656376521 ) ) ;
#98310=CARTESIAN_POINT ( 'NONE',  ( -26.71962680251449740, 1509.092879738190049, 201.3937371580310014 ) ) ;
#98311=CARTESIAN_POINT ( 'NONE',  ( -2.704615531770000025, 1447.046937273400090, 168.9986710401979906 ) ) ;
#98312=CARTESIAN_POINT ( 'NONE',  ( -20.58707213139999936, 1427.974737749530050, 223.4007331328979831 ) ) ;
#98315=CARTESIAN_POINT ( 'NONE',  ( 17.83984130769999865, 1445.351173051870092, 190.7420059714980027 ) ) ;
#98317=CARTESIAN_POINT ( 'NONE',  ( -18.94313757346292348, 1438.951138393643305, 210.3999238583679130 ) ) ;
#98324=CARTESIAN_POINT ( 'NONE',  ( -0.9796450454589999968, 1519.913060387329779, 232.6858900125980085 ) ) ;
#98325=VECTOR ( 'NONE', #101040, 1000.000000000000000 ) ;
#98328=CARTESIAN_POINT ( 'NONE',  ( -13.22735232723135468, 1443.148167861271531, 186.8228418827334281 ) ) ;
#98329=B_SPLINE_SURFACE_WITH_KNOTS ( 'NONE', 5, 5, ( 
 ( #24438, #58079, #52862, #84363, #44455, #86989 ),
 ( #94842, #27099, #70241, #92212, #41809, #58626 ),
 ( #10278, #83263, #52314, #32845, #18118, #15484 ),
 ( #78037, #75966, #61284, #67586, #101692, #109031 ),
 ( #14936, #9728, #6558, #49130, #74881, #92757 ),
 ( #16035, #1917, #104348, #43893, #32314, #1345 ),
 ( #7110, #50236, #35484, #69678, #103800, #95400 ),
 ( #27641, #41265, #61827, #66497, #23885, #49680 ),
 ( #83811, #75438, #67037, #101145, #70790, #55072 ),
 ( #62377, #53411, #97606, #38784, #63487, #88666 ),
 ( #98138, #19209, #4646, #88118, #20876, #89199 ),
 ( #19783, #4112, #28746, #106015, #53984, #104903 ),
 ( #29291, #12492, #80806, #45575, #46674, #3572 ),
 ( #62951, #97062, #38236, #72420, #2476, #10851 ),
 ( #29839, #45023, #28191, #11407, #71343, #79168 ) ),
 .UNSPECIFIED., .F., .F., .F.,
 ( 6, 3, 3, 3, 6 ),
 ( 6, 6 ),
 ( 7.637039622810000594, 10.13387562650000007, 11.38229362830000113, 12.23404602909999994, 12.63071163020000043 ),
 ( 0.000000000000000000, 2.000000000000000000 ),
 .UNSPECIFIED. ) ;
#98331=CARTESIAN_POINT ( 'NONE',  ( 13.39680589851269943, 1407.451641433219947, 204.6080239228549829 ) ) ;
#98334=B_SPLINE_CURVE_WITH_KNOTS ( 'NONE', 3,
 ( #37133, #52852, #60708, #20314, #54519, #11394, #1904, #18653, #69665, #88654, #10268, #103788, #3010, #28734, #18107, #71332, #52302, #43883, #78027, #53400, #27089, #79155, #70230, #3561, #62366, #2464, #45564, #87550, #79705, #86979, #53973, #46111, #95388, #97051, #36580, #88105, #44444, #78588, #1334, #104335, #61273, #10839, #70778 ),
 .UNSPECIFIED., .F., .F.,
 ( 4, 3, 3, 3, 3, 3, 3, 3, 3, 3, 3, 3, 3, 3, 4 ),
 ( 9.042384392956980932, 10.74863236500899966, 12.79857683260340018, 14.83630879456500118, 16.53028721917180022, 18.09003653870529860, 19.51885659866059797, 19.64978585823890000, 20.88045880726579995, 22.19108762358739995, 23.57188707978410136, 25.05204642891560241, 26.81066961526140346, 28.89555248377980234, 30.20342721250000295 ),
 .UNSPECIFIED. ) ;
#98339=EDGE_LOOP ( 'NONE', ( #50702, #60185, #18712, #81158 ) ) ;
#98348=CARTESIAN_POINT ( 'NONE',  ( 32.56932958284517099, 1421.650079385355411, 269.5000704786230585 ) ) ;
#98349=CARTESIAN_POINT ( 'NONE',  ( -15.47923624669999931, 1465.564491350429989, 248.5133305111980064 ) ) ;
#98350=B_SPLINE_CURVE_WITH_KNOTS ( 'NONE', 5,
 ( #66804, #25295, #25850, #94170, #58389, #93607, #24740, #51638, #75196 ),
 .UNSPECIFIED., .F., .F.,
 ( 6, 3, 6 ),
 ( -11.25975508159999983, -5.782490304330000441, 0.000000000000000000 ),
 .UNSPECIFIED. ) ;
#98351=FACE_OUTER_BOUND ( 'NONE', #97080, .T. ) ;
#98352=CARTESIAN_POINT ( 'NONE',  ( -11.94265424589999824, 1433.497477044639936, 149.9944001463979930 ) ) ;
#98354=CARTESIAN_POINT ( 'NONE',  ( -19.12120586389999843, 1485.993527487529946, 189.5707249904979790 ) ) ;
#98356=CARTESIAN_POINT ( 'NONE',  ( -25.00511632820000330, 1436.574185807339973, 137.9303955387979954 ) ) ;
#98358=CARTESIAN_POINT ( 'NONE',  ( 1.163729664429999966E-13, 1474.175172888730003, 270.1377426887980278 ) ) ;
#98361=CARTESIAN_POINT ( 'NONE',  ( -11.03244314401329795, 1509.423458058530514, 237.0196150796065808 ) ) ;
#98362=CARTESIAN_POINT ( 'NONE',  ( 7.739409189424749408E-09, 1406.348277573139967, 266.2841496100420500 ) ) ;
#98364=ORIENTED_EDGE ( 'NONE', *, *, #44079, .F. ) ;
#98365=CARTESIAN_POINT ( 'NONE',  ( -11.86167655160669909, 1432.027010461159989, 149.9735918577489997 ) ) ;
#98367=CARTESIAN_POINT ( 'NONE',  ( -20.61505026740000091, 1469.732609222430028, 270.3833838275979815 ) ) ;
#98369=DIRECTION ( 'NONE',  ( -1.000000000000000000, 0.000000000000000000, 0.000000000000000000 ) ) ;
#98370=CARTESIAN_POINT ( 'NONE',  ( 34.59578736694340506, 1451.704956805989923, 134.6972962829659934 ) ) ;
#98372=CARTESIAN_POINT ( 'NONE',  ( 0.2664901603583379464, 1451.240506610500006, 182.3742570756570274 ) ) ;
#98374=CARTESIAN_POINT ( 'NONE',  ( -15.85075050099999849, 1459.333342989330049, 230.7228811812979927 ) ) ;
#98377=CARTESIAN_POINT ( 'NONE',  ( -37.29566738313450003, 1420.414047975189987, 266.4270220111449703 ) ) ;
#98378=AXIS2_PLACEMENT_3D ( 'NONE', #91100, #109021, #14379 ) ;
#98380=CARTESIAN_POINT ( 'NONE',  ( -3.548032200200450070, 1505.730471142629767, 181.0364234874799934 ) ) ;
#98387=CARTESIAN_POINT ( 'NONE',  ( -15.05796970909999999, 1440.435147221739953, 189.3328455896980245 ) ) ;
#98389=CARTESIAN_POINT ( 'NONE',  ( -18.50064172359999759, 1416.067629290630066, 208.4803912601460070 ) ) ;
#98391=CARTESIAN_POINT ( 'NONE',  ( -26.03637496420000019, 1436.679440559009890, 136.9231354318980323 ) ) ;
#98395=CARTESIAN_POINT ( 'NONE',  ( 0.06979916920619999576, 1408.910622946630156, 194.4360052257980271 ) ) ;
#98397=CARTESIAN_POINT ( 'NONE',  ( -1.195258643130000076, 1396.139237108130146, 197.1899914320979690 ) ) ;
#98399=VERTEX_POINT ( 'NONE', #42178 ) ;
#98402=CARTESIAN_POINT ( 'NONE',  ( 45.49168718497458741, 1443.644333717846393, 268.9787543363217992 ) ) ;
#98404=CARTESIAN_POINT ( 'NONE',  ( -14.30919783444790028, 1436.257022624779893, 150.0511997702159874 ) ) ;
#98406=CARTESIAN_POINT ( 'NONE',  ( -0.5182872000439999738, 1486.281073925030114, 181.7525819957979820 ) ) ;
#98408=CARTESIAN_POINT ( 'NONE',  ( -17.52641558221370133, 1415.034069327669840, 207.5652963658199894 ) ) ;
#98409=DIRECTION ( 'NONE',  ( 0.9993908259982007269, 0.03489950309194383288, 3.993205903601619117E-05 ) ) ;
#98410=CARTESIAN_POINT ( 'NONE',  ( 22.51380231507019758, 1471.707018205450140, 268.8517371266460145 ) ) ;
#98411=CARTESIAN_POINT ( 'NONE',  ( 11.65314573679999910, 1415.128105759529944, 222.6874287277979931 ) ) ;
#98418=CARTESIAN_POINT ( 'NONE',  ( 0.9734891864660385474, 1457.809612541702109, 228.9324353732729094 ) ) ;
#98421=CARTESIAN_POINT ( 'NONE',  ( -4.103692849526556330, 1440.174184918509354, 185.4089468763897628 ) ) ;
#98423=CARTESIAN_POINT ( 'NONE',  ( 20.52148985240000201, 1409.793966177029915, 200.0941763215180060 ) ) ;
#98424=CARTESIAN_POINT ( 'NONE',  ( 28.08752589700002744, 1445.052233488288948, 160.7519773376980936 ) ) ;
#98425=CARTESIAN_POINT ( 'NONE',  ( -26.00842845082479826, 1468.897115946460190, 210.5448491430259992 ) ) ;
#98428=CARTESIAN_POINT ( 'NONE',  ( 21.70224022220987337, 1453.376422913917168, 220.8111189556726970 ) ) ;
#98429=CARTESIAN_POINT ( 'NONE',  ( 2.500000000000000000, 1439.624617072440060, 168.6282387789959785 ) ) ;
#98434=CARTESIAN_POINT ( 'NONE',  ( -18.24633262864339756, 1416.842625005220043, 208.9597599549800009 ) ) ;
#98436=CARTESIAN_POINT ( 'NONE',  ( -11.29523551895650080, 1425.738185592099853, 112.3427247082750000 ) ) ;
#98437=( BOUNDED_CURVE ( )  B_SPLINE_CURVE ( 3, ( #50570, #35972, #8542, #52233 ),
 .UNSPECIFIED., .F., .T. ) 
 B_SPLINE_CURVE_WITH_KNOTS ( ( 4, 4 ),
 ( 4.573263261563710103, 4.591728602243319912 ),
 .UNSPECIFIED. ) 
 CURVE ( )  GEOMETRIC_REPRESENTATION_ITEM ( )  RATIONAL_B_SPLINE_CURVE ( ( 1.000000000000000000, 0.9999715861346381018, 0.9999715861346381018, 1.000000000000000000 ) ) 
 REPRESENTATION_ITEM ( '' )  );
#98438=CARTESIAN_POINT ( 'NONE',  ( -36.32856917184830081, 1449.884418639690011, 136.2560105224960125 ) ) ;
#98439=CARTESIAN_POINT ( 'NONE',  ( 11.60004869885203682, 1425.927668451900445, 137.5659639343614913 ) ) ;
#98441=VECTOR ( 'NONE', #39616, 1000.000000000000114 ) ;
#98442=CARTESIAN_POINT ( 'NONE',  ( -2.500000000000000000, 1432.302173844710069, 157.4936352153980010 ) ) ;
#98444=ADVANCED_FACE ( 'NONE', ( #76889 ), #98446, .F. ) ;
#98445=CARTESIAN_POINT ( 'NONE',  ( -1.490542806272469933, 1474.158742738300134, 270.1372991191880146 ) ) ;
#98446=B_SPLINE_SURFACE_WITH_KNOTS ( 'NONE', 5, 5, ( 
 ( #34871, #68501, #34322, #95339, #25345, #84711 ),
 ( #59538, #76328, #24786, #10222, #8011, #198 ),
 ( #77439, #69059, #33756, #78542, #85827, #52800 ),
 ( #85261, #1856, #60656, #67953, #35428, #94214 ),
 ( #8558, #52252, #102599, #18600, #9124, #25900 ),
 ( #17489, #43291, #43836, #740, #103160, #94780 ) ),
 .UNSPECIFIED., .F., .F., .F.,
 ( 6, 6 ),
 ( 6, 6 ),
 ( 8.933709406209999315, 11.91636762130000093 ),
 ( 0.000000000000000000, 1.455044450599999983 ),
 .UNSPECIFIED. ) ;
#98447=CARTESIAN_POINT ( 'NONE',  ( 29.56664643221430211, 1440.913060386659936, 236.9318484411240036 ) ) ;
#98454=CARTESIAN_POINT ( 'NONE',  ( 2.127397458329999935, 1490.907483387130014, 235.4495606871979874 ) ) ;
#98456=CARTESIAN_POINT ( 'NONE',  ( 4.500000000000000000, 1439.615672362369878, 182.7715282920979973 ) ) ;
#98460=CARTESIAN_POINT ( 'NONE',  ( 5.800620439598599631, 1423.415524905749862, 91.01561172700489522 ) ) ;
#98462=CARTESIAN_POINT ( 'NONE',  ( 1.657465492969999898, 1465.141359081529799, 235.6472656048979957 ) ) ;
#98465=CARTESIAN_POINT ( 'NONE',  ( -1.213558767919999948, 1450.835243711869907, 182.4750632466980278 ) ) ;
#98468=CARTESIAN_POINT ( 'NONE',  ( -17.19251027932519804, 1415.089118586289942, 208.5383158172610081 ) ) ;
#98480=FACE_OUTER_BOUND ( 'NONE', #39298, .T. ) ;
#98483=CARTESIAN_POINT ( 'NONE',  ( -18.31584160739999945, 1437.055458693600031, 191.8806195066979967 ) ) ;
#98484=CARTESIAN_POINT ( 'NONE',  ( 11.76883256610000039, 1432.286229124249985, 150.8119424997980218 ) ) ;
#98490=CARTESIAN_POINT ( 'NONE',  ( 17.93302110244420433, 1458.863172048540036, 228.0434772327210169 ) ) ;
#98491=CARTESIAN_POINT ( 'NONE',  ( -12.78614179230000047, 1434.663150159289899, 149.2928482040979929 ) ) ;
#98494=CARTESIAN_POINT ( 'NONE',  ( -20.11105721185739981, 1492.027588246229925, 190.8484634630870005 ) ) ;
#98497=CARTESIAN_POINT ( 'NONE',  ( -0.1951232425329999798, 1486.506925057930175, 181.7766938669979879 ) ) ;
#98499=CARTESIAN_POINT ( 'NONE',  ( -26.73069746017884185, 1436.754254116213588, 136.7839827981474912 ) ) ;
#98500=CARTESIAN_POINT ( 'NONE',  ( -19.44259940939999964, 1468.969836806830017, 192.7096998052980155 ) ) ;
#98503=CARTESIAN_POINT ( 'NONE',  ( 4.130957310362520118, 1408.874543812650018, 222.6735585427379931 ) ) ;
#98504=CARTESIAN_POINT ( 'NONE',  ( -13.43623098084330003, 1434.935581815499745, 148.9651777270820219 ) ) ;
#98506=CARTESIAN_POINT ( 'NONE',  ( 11.73563908010000034, 1425.610159190430068, 144.1657657165980027 ) ) ;
#98510=CARTESIAN_POINT ( 'NONE',  ( 21.00608537029999923, 1420.811742010329908, 244.4374624613979847 ) ) ;
#98511=CARTESIAN_POINT ( 'NONE',  ( -1.188407889236729575, 1416.818673806566949, 228.1243924589994947 ) ) ;
#98512=CARTESIAN_POINT ( 'NONE',  ( -1.534027278920000015, 1494.208487614430169, 181.3504807686979916 ) ) ;
#98513=CARTESIAN_POINT ( 'NONE',  ( -16.81341251239999934, 1409.500197688229946, 195.2116452731980019 ) ) ;
#98515=CARTESIAN_POINT ( 'NONE',  ( -0.5987183604784179769, 1507.212886163649955, 231.7504617458309895 ) ) ;
#98516=CARTESIAN_POINT ( 'NONE',  ( -15.99459876049999885, 1425.540567386130078, 216.3101628860480048 ) ) ;
#98518=EDGE_CURVE ( 'NONE', #68277, #83651, #18057, .T. ) ;
#98521=CARTESIAN_POINT ( 'NONE',  ( 13.80599381087229993, 1434.979619881599774, 146.4346930152470065 ) ) ;
#98523=CARTESIAN_POINT ( 'NONE',  ( -5.386286590926849804, 1432.308352799489967, 154.6070632664950040 ) ) ;
#98527=VERTEX_POINT ( 'NONE', #97544 ) ;
#98530=ORIENTED_EDGE ( 'NONE', *, *, #7428, .T. ) ;
#98533=CARTESIAN_POINT ( 'NONE',  ( -0.4270334199479999815, 1479.777432516030103, 236.1344528893980055 ) ) ;
#98536=CARTESIAN_POINT ( 'NONE',  ( 46.16775327660280226, 1441.856324383689980, 266.9713873395010069 ) ) ;
#98537=CARTESIAN_POINT ( 'NONE',  ( -12.73643649006949907, 1414.913060387399810, 219.9105443766439976 ) ) ;
#98538=CARTESIAN_POINT ( 'NONE',  ( 0.3152240322409999851, 1418.590776207229965, 184.6848380081979997 ) ) ;
#98541=EDGE_LOOP ( 'NONE', ( #28453, #60307, #10987, #59043 ) ) ;
#98549=CARTESIAN_POINT ( 'NONE',  ( 10.99289993254109810, 1452.529179862749970, 150.1608018894459917 ) ) ;
#98553=CARTESIAN_POINT ( 'NONE',  ( -21.39772323737049931, 1509.704958956720020, 229.7894127843639751 ) ) ;
#98554=LINE ( 'NONE', #31352, #76785 ) ;
#98559=CARTESIAN_POINT ( 'NONE',  ( -24.08903237318989810, 1508.348042268949939, 222.3457766326179978 ) ) ;
#98560=CARTESIAN_POINT ( 'NONE',  ( 7.255983564230000127, 1427.866122641229822, 147.4806042202980052 ) ) ;
#98562=CARTESIAN_POINT ( 'NONE',  ( 19.46212511719999938, 1433.716220835580089, 224.8635561966979708 ) ) ;
#98563=PLANE ( 'NONE',  #103496 ) ;
#98566=DIRECTION ( 'NONE',  ( -0.08077839049150441209, -0.9967320861844480850, 0.000000000000000000 ) ) ;
#98568=VERTEX_POINT ( 'NONE', #71285 ) ;
#98571=CARTESIAN_POINT ( 'NONE',  ( -2.500000000000000000, 1443.913060387330006, 150.6726614421979775 ) ) ;
#98572=CARTESIAN_POINT ( 'NONE',  ( -14.45750876009999963, 1416.828042681729812, 221.3916373956980124 ) ) ;
#98576=CARTESIAN_POINT ( 'NONE',  ( 13.15726447890039985, 1414.913057819779851, 198.0251576192839877 ) ) ;
#98581=CARTESIAN_POINT ( 'NONE',  ( 15.89644188659999813, 1419.768287342929852, 227.4081588879980131 ) ) ;
#98585=CARTESIAN_POINT ( 'NONE',  ( -17.96854058879999982, 1409.540535651430218, 222.8263146518980022 ) ) ;
#98586=CARTESIAN_POINT ( 'NONE',  ( 1.549686116751380016, 1416.051481372750004, 190.4247184186629909 ) ) ;
#98587=AXIS2_PLACEMENT_3D ( 'NONE', #108951, #75364, #4821 ) ;
#98588=CARTESIAN_POINT ( 'NONE',  ( -1.120592404559999977, 1424.180376951730068, 228.4084508650980183 ) ) ;
#98589=CARTESIAN_POINT ( 'NONE',  ( 5.385734361233229350, 1432.177428534629826, 154.6052364180729910 ) ) ;
#98592=CARTESIAN_POINT ( 'NONE',  ( -34.80965728144240501, 1436.610390194000047, 136.4824736869349806 ) ) ;
#98594=CARTESIAN_POINT ( 'NONE',  ( 0.2136699404695540094, 1455.290770098899884, 183.1551236798499929 ) ) ;
#98595=CARTESIAN_POINT ( 'NONE',  ( -8.895217015593209098, 1407.887684287130242, 199.3644618170110050 ) ) ;
#98596=CARTESIAN_POINT ( 'NONE',  ( -13.50674874249999924, 1414.971287085330005, 199.3316683369779980 ) ) ;
#98598=CARTESIAN_POINT ( 'NONE',  ( -28.54117044909659739, 1509.686644087690183, 211.1713474645199824 ) ) ;
#98599=CARTESIAN_POINT ( 'NONE',  ( 12.91307535960000052, 1434.774358524450236, 148.5017423775979921 ) ) ;
#98600=CARTESIAN_POINT ( 'NONE',  ( -27.68327768569999847, 1435.464602415119771, 135.2595507401980228 ) ) ;
#98601=CARTESIAN_POINT ( 'NONE',  ( -7.105427357599999217E-15, 1419.973720559130015, 171.2095165336979790 ) ) ;
#98605=CARTESIAN_POINT ( 'NONE',  ( -12.32434985131369842, 1409.343436167639766, 217.5774198073310117 ) ) ;
#98608=CARTESIAN_POINT ( 'NONE',  ( 21.25167770093990072, 1489.809145040919930, 208.7427384965610031 ) ) ;
#98609=FACE_OUTER_BOUND ( 'NONE', #73356, .T. ) ;
#98610=CARTESIAN_POINT ( 'NONE',  ( 37.99169719898542041, 1421.960075112496497, 269.1794494414488099 ) ) ;
#98611=CARTESIAN_POINT ( 'NONE',  ( -19.34729233231120205, 1486.470064436709890, 189.5887045964369975 ) ) ;
#98616=CARTESIAN_POINT ( 'NONE',  ( 20.61542114510000090, 1508.364347661829925, 227.6602567121979916 ) ) ;
#98619=CARTESIAN_POINT ( 'NONE',  ( 0.5099819841823221012, 1411.336581462000140, 185.0281086908349835 ) ) ;
#98620=ORIENTED_EDGE ( 'NONE', *, *, #29192, .F. ) ;
#98624=CARTESIAN_POINT ( 'NONE',  ( -0.3948765404462910023, 1418.680225851279829, 184.7139127450849969 ) ) ;
#98625=CARTESIAN_POINT ( 'NONE',  ( 0.003118971330850000070, 1465.436580546529967, 236.3247307143980152 ) ) ;
#98626=CARTESIAN_POINT ( 'NONE',  ( 22.17859137039999951, 1410.608979800430006, 215.6094025197479880 ) ) ;
#98627=CARTESIAN_POINT ( 'NONE',  ( -2.425256225761660112, 1410.366585135190007, 186.4987601680199987 ) ) ;
#98629=CARTESIAN_POINT ( 'NONE',  ( -17.97825106899999881, 1424.673537191730020, 227.3634650722979984 ) ) ;
#98633=CARTESIAN_POINT ( 'NONE',  ( 0.3765318439190000199, 1477.269223033129947, 229.8244901576979942 ) ) ;
#98635=CARTESIAN_POINT ( 'NONE',  ( -24.20883260440000129, 1435.739129888689831, 210.8967360531979978 ) ) ;
#98642=CARTESIAN_POINT ( 'NONE',  ( 18.46483594369999892, 1415.628674276829770, 210.6745050120780149 ) ) ;
#98644=ORIENTED_EDGE ( 'NONE', *, *, #99058, .T. ) ;
#98646=CARTESIAN_POINT ( 'NONE',  ( 28.31978547999999662, 1509.874516473829999, 214.8570436738979765 ) ) ;
#98647=VERTEX_POINT ( 'NONE', #47149 ) ;
#98649=EDGE_CURVE ( 'NONE', #25815, #89812, #82504, .T. ) ;
#98651=CARTESIAN_POINT ( 'NONE',  ( 15.93782904601589934, 1419.538716697589962, 191.2487339700179803 ) ) ;
#98652=CARTESIAN_POINT ( 'NONE',  ( 15.72108344340260011, 1409.846270172940194, 191.9446229745909989 ) ) ;
#98655=ADVANCED_FACE ( 'NONE', ( #105398 ), #30512, .T. ) ;
#98657=CARTESIAN_POINT ( 'NONE',  ( -25.23720171959060110, 1451.310931879150075, 137.2167829449969929 ) ) ;
#98658=CARTESIAN_POINT ( 'NONE',  ( 33.93526097588131307, 1436.160851839354109, 136.3001501137667617 ) ) ;
#98659=CARTESIAN_POINT ( 'NONE',  ( 15.61151356360000086, 1410.390253723229989, 227.1240187857980288 ) ) ;
#98664=CARTESIAN_POINT ( 'NONE',  ( 41.60033908837840499, 1444.718971643219902, 134.0999999983919793 ) ) ;
#98665=DIRECTION ( 'NONE',  ( 0.000000000000000000, 0.000000000000000000, -1.000000000000000000 ) ) ;
#98667=CARTESIAN_POINT ( 'NONE',  ( 13.90282916737450059, 1434.989572450550213, 148.6937415729140071 ) ) ;
#98671=EDGE_CURVE ( 'NONE', #67655, #18109, #90223, .T. ) ;
#98673=CARTESIAN_POINT ( 'NONE',  ( 37.66849513895419932, 1445.052233489950140, 137.0436250799990034 ) ) ;
#98679=CARTESIAN_POINT ( 'NONE',  ( 9792.142915373007781, 50.28429875041810959, -1105.735996643114049 ) ) ;
#98680=CARTESIAN_POINT ( 'NONE',  ( -1.321968956450000121, 1497.687671660330125, 231.6439708845980192 ) ) ;
#98681=CARTESIAN_POINT ( 'NONE',  ( 6.282169504720000575, 1416.518938591829965, 191.8828167486979623 ) ) ;
#98684=ORIENTED_EDGE ( 'NONE', *, *, #64219, .F. ) ;
#98690=CARTESIAN_POINT ( 'NONE',  ( 19.12129754759999756, 1477.356669723930054, 228.1731787199980204 ) ) ;
#98691=VERTEX_POINT ( 'NONE', #7875 ) ;
#98692=CARTESIAN_POINT ( 'NONE',  ( 13.15366522099999891, 1428.703228679929907, 223.0784815109979888 ) ) ;
#98693=CARTESIAN_POINT ( 'NONE',  ( -15.82859721659999863, 1410.397881278330033, 191.2512645620979868 ) ) ;
#98697=CARTESIAN_POINT ( 'NONE',  ( 22.28103957729450002, 1410.282322871559927, 206.2410114249429967 ) ) ;
#98699=CARTESIAN_POINT ( 'NONE',  ( -2.889979094190000097, 1508.952905480530035, 179.9120178563979948 ) ) ;
#98703=CARTESIAN_POINT ( 'NONE',  ( 15.33271527600000006, 1460.168619882530038, 230.3678631353980109 ) ) ;
#98704=DIRECTION ( 'NONE',  ( 0.7071067811870476172, 0.000000000000000000, -0.7071067811860475283 ) ) ;
#98715=FACE_OUTER_BOUND ( 'NONE', #29502, .T. ) ;
#98717=CARTESIAN_POINT ( 'NONE',  ( -11.86130994329999844, 1432.001365804540001, 149.9732119217979971 ) ) ;
#98720=CARTESIAN_POINT ( 'NONE',  ( 2.420926942500000401, 1415.924425175530132, 231.9930866673979892 ) ) ;
#98722=CARTESIAN_POINT ( 'NONE',  ( 11.79002570369999958, 1447.121451514899718, 187.8029540045979786 ) ) ;
#98723=CARTESIAN_POINT ( 'NONE',  ( -20.40381310260000092, 1444.801140792109891, 223.4425445369979855 ) ) ;
#98724=CARTESIAN_POINT ( 'NONE',  ( 2.500000000000000000, 1419.383216040929938, 144.0854373786980034 ) ) ;
#98725=CARTESIAN_POINT ( 'NONE',  ( -1.590912488230000088, 1484.788632896829995, 182.5874906166980054 ) ) ;
#98728=CARTESIAN_POINT ( 'NONE',  ( 0.8891820839130000209, 1405.755862229229933, 267.5368302669979812 ) ) ;
#98731=CARTESIAN_POINT ( 'NONE',  ( 24.63111624260878685, 1440.210199689701540, 212.4614418941652900 ) ) ;
#98732=ADVANCED_FACE ( 'NONE', ( #110342 ), #73454, .F. ) ;
#98734=CARTESIAN_POINT ( 'NONE',  ( 11.60004869885203682, 1424.776121897636585, 137.5689991293697005 ) ) ;
#98737=CARTESIAN_POINT ( 'NONE',  ( -2.498115821138040538, 1449.212599764990046, 155.3362512705470238 ) ) ;
#98739=CARTESIAN_POINT ( 'NONE',  ( -19.71995158176096652, 1486.080284922995588, 190.1322500716072454 ) ) ;
#98740=CARTESIAN_POINT ( 'NONE',  ( -13.77282262973849924, 1415.219159639000054, 220.6941904408330117 ) ) ;
#98742=CARTESIAN_POINT ( 'NONE',  ( 3.108624468949999707E-15, 1424.916853932230197, 224.8635561844979804 ) ) ;
#98744=CARTESIAN_POINT ( 'NONE',  ( -26.87061429964650117, 1508.006948577689855, 211.9372255802010159 ) ) ;
#98745=FACE_OUTER_BOUND ( 'NONE', #98800, .T. ) ;
#98746=CARTESIAN_POINT ( 'NONE',  ( -1.778002813740000132, 1476.025706879929885, 268.4824706862979724 ) ) ;
#98748=CARTESIAN_POINT ( 'NONE',  ( 24.02863916850529691, 1507.902931906480035, 195.9323055859989893 ) ) ;
#98749=CARTESIAN_POINT ( 'NONE',  ( 18.10638723112739967, 1414.300371954559978, 223.0951481136329733 ) ) ;
#98757=CARTESIAN_POINT ( 'NONE',  ( -9.885612070768521775, 1396.258273567759943, 214.0867141279609882 ) ) ;
#98758=CARTESIAN_POINT ( 'NONE',  ( -14.63705847230000145, 1422.169902662129971, 229.4588690710980075 ) ) ;
#98759=EDGE_CURVE ( 'NONE', #48269, #56530, #12866, .T. ) ;
#98760=CARTESIAN_POINT ( 'NONE',  ( 19.27222582892916947, 1456.061223426223933, 225.1253623777946586 ) ) ;
#98762=CARTESIAN_POINT ( 'NONE',  ( -7.517448282616630451, 1410.548633254104288, 230.8423976230810695 ) ) ;
#98764=CARTESIAN_POINT ( 'NONE',  ( -11.86716023049999968, 1432.353341358199941, 147.6509521729980179 ) ) ;
#98767=CARTESIAN_POINT ( 'NONE',  ( -16.03585548469987998, 1409.473035015031883, 225.1837023168980352 ) ) ;
#98768=EDGE_CURVE ( 'NONE', #11318, #16982, #40801, .T. ) ;
#98780=CARTESIAN_POINT ( 'NONE',  ( -12.08279855019999971, 1398.271306150530108, 203.2690269987980116 ) ) ;
#98781=CARTESIAN_POINT ( 'NONE',  ( -21.64909456690000056, 1411.027735339629999, 216.4118746903779993 ) ) ;
#98782=CARTESIAN_POINT ( 'NONE',  ( -1.556886619979999997, 1415.063410501429871, 226.7642036972980009 ) ) ;
#98783=CARTESIAN_POINT ( 'NONE',  ( -13.22654679013079537, 1444.679112648444061, 169.3876301519718766 ) ) ;
#98789=CARTESIAN_POINT ( 'NONE',  ( 1.567402629779999890, 1410.307036984029992, 185.3288458999980151 ) ) ;
#98792=CARTESIAN_POINT ( 'NONE',  ( -40.21925577861330225, 1446.541393603889901, 136.6959051559719853 ) ) ;
#98793=CARTESIAN_POINT ( 'NONE',  ( 10.44466107780339925, 1396.277795989850119, 212.7871969495540156 ) ) ;
#98794=CARTESIAN_POINT ( 'NONE',  ( 1.343523894720000111, 1416.547221147930031, 190.1769955903980076 ) ) ;
#98795=CARTESIAN_POINT ( 'NONE',  ( 11.82328634059999928, 1429.482282172129999, 149.2137815048980087 ) ) ;
#98800=EDGE_LOOP ( 'NONE', ( #39212, #57520, #60234 ) ) ;
#98802=ADVANCED_FACE ( 'NONE', ( #75805 ), #65210, .T. ) ;
#98804=CARTESIAN_POINT ( 'NONE',  ( -14.48621421730000058, 1460.257914811229966, 230.6628917214979992 ) ) ;
#98809=ADVANCED_FACE ( 'NONE', ( #5848 ), #22445, .T. ) ;
#98810=ORIENTED_EDGE ( 'NONE', *, *, #50775, .T. ) ;
#98812=CARTESIAN_POINT ( 'NONE',  ( 2.500000000000079936, 1448.852881373850096, 156.0659984934969771 ) ) ;
#98814=CARTESIAN_POINT ( 'NONE',  ( 0.3142747836059999744, 1415.426210663629945, 226.6044997240979910 ) ) ;
#98819=CARTESIAN_POINT ( 'NONE',  ( -29.83261703232589923, 1419.454359286137787, 269.4690300932230684 ) ) ;
#98821=LINE ( 'NONE', #30515, #35118 ) ;
#98822=ORIENTED_EDGE ( 'NONE', *, *, #34627, .T. ) ;
#98824=CARTESIAN_POINT ( 'NONE',  ( -0.01304952888453610182, 1452.849458485459763, 183.2395837122380158 ) ) ;
#98825=CARTESIAN_POINT ( 'NONE',  ( -30.65930537466649852, 1440.913060387579890, 240.3862288817810224 ) ) ;
#98828=CARTESIAN_POINT ( 'NONE',  ( -0.06802918170042410173, 1467.142004300180133, 235.6414935935190158 ) ) ;
#98829=CARTESIAN_POINT ( 'NONE',  ( 39.55870798286069601, 1428.444394588759906, 270.0311279852339794 ) ) ;
#98833=CARTESIAN_POINT ( 'NONE',  ( 23.01582909600000093, 1409.742947454629984, 209.0450749743000074 ) ) ;
#98834=FACE_OUTER_BOUND ( 'NONE', #44139, .T. ) ;
#98835=CARTESIAN_POINT ( 'NONE',  ( -13.15726454016349933, 1414.996443537369942, 220.4820293315119955 ) ) ;
#98838=CARTESIAN_POINT ( 'NONE',  ( 4.203924555649190431, 1421.744692650780280, 184.5805578976949732 ) ) ;
#98841=VERTEX_POINT ( 'NONE', #102623 ) ;
#98843=CARTESIAN_POINT ( 'NONE',  ( 18.64588645199999917, 1416.828044802730119, 209.6843146608260042 ) ) ;
#98844=CARTESIAN_POINT ( 'NONE',  ( -0.02063504396140000002, 1416.982032014529977, 234.1905969501979996 ) ) ;
#98848=CARTESIAN_POINT ( 'NONE',  ( -11.89463746655019882, 1434.488622496119888, 147.6463952747150188 ) ) ;
#98850=CARTESIAN_POINT ( 'NONE',  ( -10.10004869885203682, 0.000000000000000000, 135.5999999980979851 ) ) ;
#98851=CARTESIAN_POINT ( 'NONE',  ( -25.91673698548662230, 1450.780993184907857, 136.7962322576231884 ) ) ;
#98855=CARTESIAN_POINT ( 'NONE',  ( -18.64672481365220236, 1416.851343896850040, 208.5597484336410048 ) ) ;
#98856=VERTEX_POINT ( 'NONE', #1311 ) ;
#98857=CARTESIAN_POINT ( 'NONE',  ( 11.60004869885203682, 1426.786827912535728, 134.3786173235958472 ) ) ;
#98858=CARTESIAN_POINT ( 'NONE',  ( 23.96634320729999956, 1447.652375259820019, 215.5884833387879951 ) ) ;
#98862=CARTESIAN_POINT ( 'NONE',  ( 16.32344763033163559, 1421.553467051097869, 227.2347501064996891 ) ) ;
#98864=CARTESIAN_POINT ( 'NONE',  ( -19.53791504940000223, 1426.663906195230084, 224.0751841881980226 ) ) ;
#98867=CARTESIAN_POINT ( 'NONE',  ( 18.25078530649999919, 1498.105401280229898, 188.8231487391980181 ) ) ;
#98869=CARTESIAN_POINT ( 'NONE',  ( -18.46874166461617151, 1436.582161157081146, 212.8784271109066992 ) ) ;
#98873=LINE ( 'NONE', #82066, #87547 ) ;
#98874=CARTESIAN_POINT ( 'NONE',  ( -10.79902394581574221, 1424.930925960156173, 143.1565572995466198 ) ) ;
#98876=FACE_OUTER_BOUND ( 'NONE', #79941, .T. ) ;
#98877=CARTESIAN_POINT ( 'NONE',  ( 1.457708929429750055, 1498.159145731940043, 181.5038820770699886 ) ) ;
#98878=CARTESIAN_POINT ( 'NONE',  ( -1.682318767883554278, 1409.475163258161501, 186.2035163977165269 ) ) ;
#98879=CARTESIAN_POINT ( 'NONE',  ( -13.44172084558439018, 1444.321659713776171, 186.9696591558638659 ) ) ;
#98880=CARTESIAN_POINT ( 'NONE',  ( -24.87779863397740243, 1440.202515696970067, 210.4162827866140049 ) ) ;
#98882=DIRECTION ( 'NONE',  ( 0.000000000000000000, 1.000000000000000000, 0.000000000000000000 ) ) ;
#98884=CARTESIAN_POINT ( 'NONE',  ( 24.93050923819999909, 1436.289048159549793, 137.8926102245979735 ) ) ;
#98887=ORIENTED_EDGE ( 'NONE', *, *, #23580, .F. ) ;
#98890=VERTEX_POINT ( 'NONE', #103762 ) ;
#98895=CARTESIAN_POINT ( 'NONE',  ( 25.36271876829972172, 1416.586431751986311, 269.4273607397962564 ) ) ;
#98896=CARTESIAN_POINT ( 'NONE',  ( -28.66942461689999888, 1455.243640874929952, 248.2467662535980253 ) ) ;
#98897=CARTESIAN_POINT ( 'NONE',  ( -20.28483480839999942, 1503.699721672330043, 189.5804053314980138 ) ) ;
#98898=CARTESIAN_POINT ( 'NONE',  ( -11.90306278269999929, 1433.319533555049929, 150.0454030812979909 ) ) ;
#98900=CARTESIAN_POINT ( 'NONE',  ( 11.61600128336219839, 1426.776741275609993, 135.5201114608300088 ) ) ;
#98902=CARTESIAN_POINT ( 'NONE',  ( -25.38336389990000086, 1437.595645302209959, 137.6395686390980018 ) ) ;
#98904=CARTESIAN_POINT ( 'NONE',  ( 8.510960778390000314, 1440.269029158009971, 153.6986480022980004 ) ) ;
#98907=CARTESIAN_POINT ( 'NONE',  ( -5.847473420468886296, 1509.246610639426535, 238.5602555325059484 ) ) ;
#98908=CARTESIAN_POINT ( 'NONE',  ( 1.301951668218010061E-10, 1411.335116748880182, 255.3083647514700090 ) ) ;
#98913=CARTESIAN_POINT ( 'NONE',  ( -34.31228247859999669, 1461.759392064230042, 270.3000846135980169 ) ) ;
#98914=CARTESIAN_POINT ( 'NONE',  ( -1.547930050009999947, 1416.311719782429918, 227.9539241407980228 ) ) ;
#98924=CARTESIAN_POINT ( 'NONE',  ( -37.53908224095089707, 1420.183636347619995, 266.9518714729799740 ) ) ;
#98925=ORIENTED_EDGE ( 'NONE', *, *, #41926, .F. ) ;
#98926=CARTESIAN_POINT ( 'NONE',  ( -3.539686542936679725, 1497.693967252670063, 181.3788000397719884 ) ) ;
#98927=ORIENTED_EDGE ( 'NONE', *, *, #6044, .T. ) ;
#98930=CARTESIAN_POINT ( 'NONE',  ( 33.46233750170772225, 1444.994950788469168, 154.5794059528860203 ) ) ;
#98932=CARTESIAN_POINT ( 'NONE',  ( -14.43318959600000007, 1455.449656469629872, 188.2552579046979986 ) ) ;
#98934=CARTESIAN_POINT ( 'NONE',  ( -11.60004869885203682, 1428.983126981193436, 134.0999999980979851 ) ) ;
#98935=VERTEX_POINT ( 'NONE', #67979 ) ;
#98936=CARTESIAN_POINT ( 'NONE',  ( -26.62406874550000069, 1435.731906908609972, 136.2240211947980129 ) ) ;
#98939=CARTESIAN_POINT ( 'NONE',  ( 1.317974831259093316, 1508.993303073226343, 238.7438154217258557 ) ) ;
#98940=CARTESIAN_POINT ( 'NONE',  ( -44.13013983209490476, 1435.750459799680129, 270.2165836708290385 ) ) ;
#98942=CARTESIAN_POINT ( 'NONE',  ( -1.233242815080000110, 1396.496402683329961, 196.6588694784980191 ) ) ;
#98944=ORIENTED_EDGE ( 'NONE', *, *, #39882, .F. ) ;
#98947=CARTESIAN_POINT ( 'NONE',  ( 2.897647365308007039, 1475.048391750445489, 269.6500680714580653 ) ) ;
#98949=CARTESIAN_POINT ( 'NONE',  ( -14.36669942202730077, 1436.256511924010056, 150.0155719173559987 ) ) ;
#98950=CARTESIAN_POINT ( 'NONE',  ( -1.267179638100000227, 1485.071352279529947, 182.1863245234980013 ) ) ;
#98951=EDGE_CURVE ( 'NONE', #19921, #80510, #27602, .T. ) ;
#98954=CARTESIAN_POINT ( 'NONE',  ( -18.69112752649999720, 1430.796159002630020, 225.2456904468979815 ) ) ;
#98956=CARTESIAN_POINT ( 'NONE',  ( 11.90129930089999988, 1415.245980409429876, 222.6985869743980118 ) ) ;
#98957=CARTESIAN_POINT ( 'NONE',  ( -4.221362096953909848, 1441.596168439879875, 170.5366494805969921 ) ) ;
#98959=EDGE_CURVE ( 'NONE', #9890, #85608, #70205, .T. ) ;
#98960=ORIENTED_EDGE ( 'NONE', *, *, #49480, .F. ) ;
#98961=CARTESIAN_POINT ( 'NONE',  ( -42.60628464300700102, 1443.705283383359983, 135.3761640576199738 ) ) ;
#98962=CARTESIAN_POINT ( 'NONE',  ( -22.71570642892181624, 1451.001388305250430, 218.7895664819020283 ) ) ;
#98964=CARTESIAN_POINT ( 'NONE',  ( 18.07930019939639621, 1457.670260863833164, 229.7183053949007956 ) ) ;
#98965=CARTESIAN_POINT ( 'NONE',  ( 25.15410452086170068, 1451.315323596600138, 137.3483238205280088 ) ) ;
#98966=CARTESIAN_POINT ( 'NONE',  ( 13.91384509699999938, 1415.996778984329922, 196.5752437455980157 ) ) ;
#98968=CARTESIAN_POINT ( 'NONE',  ( 19.29764154210000271, 1410.948454093429746, 195.8526098399979958 ) ) ;
#98971=CARTESIAN_POINT ( 'NONE',  ( -13.80541478530910027, 1434.979604282769969, 148.5370187744020143 ) ) ;
#98972=CARTESIAN_POINT ( 'NONE',  ( 24.59103204445768043, 1443.271088975028761, 213.0685705457873382 ) ) ;
#98977=CARTESIAN_POINT ( 'NONE',  ( -39.29615804430000026, 1457.459686057429963, 269.7910478776980199 ) ) ;
#98978=CARTESIAN_POINT ( 'NONE',  ( 16.68463225900990210, 1445.052233488270076, 162.0935120915889911 ) ) ;
#98979=CARTESIAN_POINT ( 'NONE',  ( -5.850883015700239831, 1422.777641411109926, 112.2634153026260009 ) ) ;
#98981=CARTESIAN_POINT ( 'NONE',  ( 11.60004869885203682, 1426.432599161485996, 138.7994597023310916 ) ) ;
#98982=CARTESIAN_POINT ( 'NONE',  ( 2.077066168525637302, 1417.353822717204594, 233.2012438648220893 ) ) ;
#98983=CARTESIAN_POINT ( 'NONE',  ( 17.89881597930054014, 1423.835250522596425, 225.8299768472458311 ) ) ;
#98986=CARTESIAN_POINT ( 'NONE',  ( 35.19864010958440304, 1440.913060386249981, 251.3230737458970054 ) ) ;
#98989=ORIENTED_EDGE ( 'NONE', *, *, #17252, .T. ) ;
#98992=CARTESIAN_POINT ( 'NONE',  ( -19.09472837541543555, 1485.512501651969160, 189.6337084803414541 ) ) ;
#98995=CARTESIAN_POINT ( 'NONE',  ( 0.02089822245711980137, 1507.111760766699945, 237.3522839811660106 ) ) ;
#99000=CARTESIAN_POINT ( 'NONE',  ( -12.61640430610000152, 1416.837080253930026, 194.9197996555979842 ) ) ;
#99002=CARTESIAN_POINT ( 'NONE',  ( 1.348363903870000158, 1466.040058020430024, 235.1849732789979726 ) ) ;
#99006=CARTESIAN_POINT ( 'NONE',  ( -0.8000066638249999640, 1450.880929917359936, 181.7283017618979954 ) ) ;
#99015=DIRECTION ( 'NONE',  ( -0.3282391760791589785, 0.000000000000000000, -0.9445946449598763284 ) ) ;
#99016=CIRCLE ( 'NONE', #50761, 2.000000000000059064 ) ;
#99021=CARTESIAN_POINT ( 'NONE',  ( 19.59040869416958941, 1509.614908582205999, 186.9437411615208475 ) ) ;
#99022=CARTESIAN_POINT ( 'NONE',  ( 12.66229353878289920, 1409.355237421249967, 201.1910009548570031 ) ) ;
#99023=CARTESIAN_POINT ( 'NONE',  ( 0.6328050152959999730, 1408.935158425530062, 186.1228243921979981 ) ) ;
#99024=CARTESIAN_POINT ( 'NONE',  ( 1.959361663749999982, 1419.250139722030099, 185.0399661677979850 ) ) ;
#99025=CARTESIAN_POINT ( 'NONE',  ( -18.87607639370000001, 1452.025551963729868, 192.2339656219979815 ) ) ;
#99032=CARTESIAN_POINT ( 'NONE',  ( 18.12943984651419882, 1457.942338673419954, 228.1937571059060019 ) ) ;
#99033=CARTESIAN_POINT ( 'NONE',  ( -12.89823998259999982, 1434.736470928759900, 149.6930873346979922 ) ) ;
#99035=CARTESIAN_POINT ( 'NONE',  ( -20.40237847379039948, 1501.463721599679957, 190.5751277017120060 ) ) ;
#99036=FACE_BOUND ( 'NONE', #16171, .T. ) ;
#99041=CARTESIAN_POINT ( 'NONE',  ( -21.03123196750000190, 1507.789098030329797, 192.1781278414979965 ) ) ;
#99044=CARTESIAN_POINT ( 'NONE',  ( 1.369523653644170169, 1408.899450504319930, 223.4949184458459968 ) ) ;
#99045=CARTESIAN_POINT ( 'NONE',  ( -13.27386107244829994, 1434.917007507699964, 149.3091083363100040 ) ) ;
#99047=CARTESIAN_POINT ( 'NONE',  ( 0.3641805758275279969, 1424.317995888269934, 227.5054904079770211 ) ) ;
#99051=CARTESIAN_POINT ( 'NONE',  ( 31.44036153859999771, 1425.375771343829911, 254.7811647136979900 ) ) ;
#99052=CARTESIAN_POINT ( 'NONE',  ( -1.546949757679999760, 1416.828040475729949, 228.0209010782980101 ) ) ;
#99056=CARTESIAN_POINT ( 'NONE',  ( -12.77010823640000048, 1420.349902697730158, 231.7712046106979926 ) ) ;
#99057=CARTESIAN_POINT ( 'NONE',  ( -29.70214828285509867, 1509.984309146039777, 208.0179991509364470 ) ) ;
#99058=EDGE_CURVE ( 'NONE', #21837, #24662, #46163, .T. ) ;
#99059=CARTESIAN_POINT ( 'NONE',  ( -17.05409589288600003, 1452.317518235730176, 146.2609911881839651 ) ) ;
#99060=CARTESIAN_POINT ( 'NONE',  ( -18.96298731639999602, 1416.825532216530064, 208.0004950568580000 ) ) ;
#99064=CARTESIAN_POINT ( 'NONE',  ( 14.30536690592939841, 1421.516539548159926, 228.9956906566140162 ) ) ;
#99065=ORIENTED_EDGE ( 'NONE', *, *, #32198, .T. ) ;
#99066=VERTEX_POINT ( 'NONE', #102086 ) ;
#99072=DIRECTION ( 'NONE',  ( 0.02546698206423540778, -0.0008893270957687149847, -0.9996752682355689590 ) ) ;
#99073=CARTESIAN_POINT ( 'NONE',  ( 5.519893427111519202, 1440.499866072189889, 154.7645221071819890 ) ) ;
#99074=ORIENTED_EDGE ( 'NONE', *, *, #32367, .F. ) ;
#99075=CARTESIAN_POINT ( 'NONE',  ( 45.82909222224540002, 1446.182179057269877, 267.6052008258039905 ) ) ;
#99076=CARTESIAN_POINT ( 'NONE',  ( -13.15726442270000085, 1416.851343897030119, 221.9096085505980227 ) ) ;
#99080=EDGE_CURVE ( 'NONE', #43475, #22743, #94369, .T. ) ;
#99082=LINE ( 'NONE', #3969, #40127 ) ;
#99083=CARTESIAN_POINT ( 'NONE',  ( 13.51514909825042565, 1443.972136820036440, 188.0277010184605899 ) ) ;
#99088=CARTESIAN_POINT ( 'NONE',  ( -4.324698967714178721, 1424.665291916374827, 185.8068982220774217 ) ) ;
#99089=CARTESIAN_POINT ( 'NONE',  ( 10.06559049306389930, 1452.561562221930217, 150.5716378858789994 ) ) ;
#99090=CARTESIAN_POINT ( 'NONE',  ( -1.726328313212220289E-05, 1407.650947845630071, 270.1377426662980383 ) ) ;
#99091=CARTESIAN_POINT ( 'NONE',  ( 33.91369968912619726, 1451.728767897860052, 134.7155302171979940 ) ) ;
#99093=CARTESIAN_POINT ( 'NONE',  ( -10.97860844464990038, 1432.885878357189995, 151.7696306460070161 ) ) ;
#99095=DIRECTION ( 'NONE',  ( 0.000000000000000000, 0.000000000000000000, -1.000000000000000000 ) ) ;
#99096=CARTESIAN_POINT ( 'NONE',  ( -16.66101146819999812, 1410.867390116229899, 191.7375337716979971 ) ) ;
#99099=CARTESIAN_POINT ( 'NONE',  ( -24.23681317631879750, 1508.759042070240184, 222.4186787974370247 ) ) ;
#99100=CARTESIAN_POINT ( 'NONE',  ( 9.634835741540001663, 1430.981823154709900, 148.7079730222979776 ) ) ;
#99102=CARTESIAN_POINT ( 'NONE',  ( 20.41675352909999930, 1438.655740921959932, 219.6133833292979887 ) ) ;
#99103=AXIS2_PLACEMENT_3D ( 'NONE', #80594, #71122, #105243 ) ;
#99104=CARTESIAN_POINT ( 'NONE',  ( -0.2232534084008130082, 1424.263167169779990, 227.7533338486369985 ) ) ;
#99106=B_SPLINE_SURFACE_WITH_KNOTS ( 'NONE', 5, 4, ( 
 ( #68105, #3663, #10936, #28281, #37792 ),
 ( #106632, #73049, #20960, #45666, #12583 ),
 ( #70878, #104989, #19867, #62476, #54616 ),
 ( #30479, #21502, #64112, #28840, #98233 ),
 ( #97687, #2561, #71980, #107190, #89287 ),
 ( #46764, #46212, #4191, #80894, #79252 ) ),
 .UNSPECIFIED., .F., .F., .F.,
 ( 6, 6 ),
 ( 5, 5 ),
 ( 0.000000000000000000, 111.1101480259999903 ),
 ( 25.81581217359999769, 39.03307591160000101 ),
 .UNSPECIFIED. ) ;
#99113=CARTESIAN_POINT ( 'NONE',  ( -14.20190154360000179, 1416.831305866930279, 221.7380342762980092 ) ) ;
#99114=CARTESIAN_POINT ( 'NONE',  ( 11.28251112829999947, 1433.921144945409878, 151.5399218156979941 ) ) ;
#99115=CARTESIAN_POINT ( 'NONE',  ( -11.60004869885203682, 1425.894669202444675, 137.5118601406020673 ) ) ;
#99116=CARTESIAN_POINT ( 'NONE',  ( 12.48769551257159982, 1414.971717244360207, 197.6617324145900056 ) ) ;
#99119=CARTESIAN_POINT ( 'NONE',  ( 13.65755722549999973, 1419.762562827630063, 228.6500612441979854 ) ) ;
#99123=CARTESIAN_POINT ( 'NONE',  ( -0.5639001407619999018, 1420.522959561429843, 227.9306795899979932 ) ) ;
#99124=CARTESIAN_POINT ( 'NONE',  ( -26.97127426239999792, 1450.931412349030097, 136.4066425356980119 ) ) ;
#99126=CARTESIAN_POINT ( 'NONE',  ( 12.61566547299999996, 1416.819759814730105, 223.3235036042979971 ) ) ;
#99129=CARTESIAN_POINT ( 'NONE',  ( -7.803087493140000497, 1414.971262582530017, 223.9800507790980362 ) ) ;
#99131=CARTESIAN_POINT ( 'NONE',  ( 0.2091846300955290117, 1457.806774526239906, 183.0471825358959848 ) ) ;
#99133=CARTESIAN_POINT ( 'NONE',  ( -8.860300303135609568, 1407.578384618130031, 199.4146916745189912 ) ) ;
#99134=CARTESIAN_POINT ( 'NONE',  ( -12.85971948620000127, 1415.932840167130053, 196.7491045163979777 ) ) ;
#99135=CARTESIAN_POINT ( 'NONE',  ( -28.30972139877570015, 1509.473640034179880, 210.9653718159219977 ) ) ;
#99136=CARTESIAN_POINT ( 'NONE',  ( 12.40421625309999953, 1434.420021183800145, 148.5016035624979907 ) ) ;
#99137=CARTESIAN_POINT ( 'NONE',  ( -28.14146986589999955, 1435.479030298939961, 135.6828298310979903 ) ) ;
#99138=CARTESIAN_POINT ( 'NONE',  ( 8.709291548640001324, 1441.011683078770147, 186.3963333776979709 ) ) ;
#99139=ORIENTED_EDGE ( 'NONE', *, *, #31923, .F. ) ;
#99146=CARTESIAN_POINT ( 'NONE',  ( 31.88106177436622701, 1416.458733636820853, 269.3181919498966295 ) ) ;
#99148=CARTESIAN_POINT ( 'NONE',  ( 20.15452300067990166, 1507.845791525220193, 189.3412703910400126 ) ) ;
#99149=CARTESIAN_POINT ( 'NONE',  ( -4.219439073160000220, 1441.595895977600094, 177.0328731553979935 ) ) ;
#99152=CARTESIAN_POINT ( 'NONE',  ( -27.79585007420000053, 1451.789558028530109, 135.7670632556980195 ) ) ;
#99153=CARTESIAN_POINT ( 'NONE',  ( 41.66134420550000073, 1443.796851579070108, 135.6885409488979803 ) ) ;
#99154=CARTESIAN_POINT ( 'NONE',  ( -15.86684091882549907, 1409.475427479080281, 225.4728633087160006 ) ) ;
#99155=CARTESIAN_POINT ( 'NONE',  ( 0.4983054691675419257, 1414.932839379760026, 184.8741889412040393 ) ) ;
#99159=CARTESIAN_POINT ( 'NONE',  ( -22.11218108847071306, 1411.043597553445352, 214.4701686222656178 ) ) ;
#99161=CARTESIAN_POINT ( 'NONE',  ( -0.09623828610459078670, 1420.380023493850103, 183.2616177384549871 ) ) ;
#99162=CARTESIAN_POINT ( 'NONE',  ( 1.108178853160000088, 1466.523263909929938, 235.2969450623980094 ) ) ;
#99163=CARTESIAN_POINT ( 'NONE',  ( 22.66638050679999949, 1410.625956981130230, 214.3745493218679883 ) ) ;
#99164=DIRECTION ( 'NONE',  ( -0.07035059757514136591, -0.9966174162490445410, -0.04247963100003462888 ) ) ;
#99166=CARTESIAN_POINT ( 'NONE',  ( -17.67465541829999864, 1423.538376080030048, 226.2965632852980207 ) ) ;
#99169=CARTESIAN_POINT ( 'NONE',  ( 27.41515664521250173, 1488.740012672480134, 209.4249987372610065 ) ) ;
#99172=CARTESIAN_POINT ( 'NONE',  ( -0.9621744844780000250, 1415.477225457230134, 233.2860938207980155 ) ) ;
#99176=CARTESIAN_POINT ( 'NONE',  ( -11.36618588219640102, 1485.531419837760041, 185.0615275845599967 ) ) ;
#99177=ORIENTED_EDGE ( 'NONE', *, *, #26089, .T. ) ;
#99180=CARTESIAN_POINT ( 'NONE',  ( -4.242759794694189956, 1441.416754616080198, 162.3033463234470162 ) ) ;
#99186=ORIENTED_EDGE ( 'NONE', *, *, #9671, .F. ) ;
#99189=CARTESIAN_POINT ( 'NONE',  ( -10.82182428428866672, 1424.917064109405146, 144.5864024659527729 ) ) ;
#99190=CARTESIAN_POINT ( 'NONE',  ( 1.446896864630000001, 1507.663901920830085, 181.0890709196980026 ) ) ;
#99192=CARTESIAN_POINT ( 'NONE',  ( -24.86261486476140092, 1452.044834405480060, 135.5980773263869992 ) ) ;
#99193=CARTESIAN_POINT ( 'NONE',  ( -11.73709356449999852, 1426.695943566229971, 144.1748013792980032 ) ) ;
#99199=CARTESIAN_POINT ( 'NONE',  ( -39.65801192383619167, 1440.831642379499954, 136.8099676560480020 ) ) ;
#99204=CARTESIAN_POINT ( 'NONE',  ( 10.66111875780481633, 1410.659669277416242, 229.5690789417564019 ) ) ;
#99206=CARTESIAN_POINT ( 'NONE',  ( 0.04542731285949999642, 1451.694725257930031, 183.0340308383979959 ) ) ;
#99207=CARTESIAN_POINT ( 'NONE',  ( -3.311547598719999819, 1485.996598843729998, 182.1826784800979908 ) ) ;
#99208=CARTESIAN_POINT ( 'NONE',  ( -2.500000000000199840, 1439.253552895449957, 159.5302512421249901 ) ) ;
#99213=CARTESIAN_POINT ( 'NONE',  ( 28.28208337139999884, 1508.151294399930066, 209.1094497554269935 ) ) ;
#99214=CARTESIAN_POINT ( 'NONE',  ( 12.51099981729999833, 1416.825784011830137, 196.0986189375979905 ) ) ;
#99220=CARTESIAN_POINT ( 'NONE',  ( 11.03427950888080211, 1414.913526845469960, 222.2765582366960189 ) ) ;
#99221=CARTESIAN_POINT ( 'NONE',  ( -0.0002585518234266428279, 1452.563254695420028, 153.5184766442947080 ) ) ;
#99224=CARTESIAN_POINT ( 'NONE',  ( -15.04452981080000029, 1409.438426944829871, 191.9174468092980135 ) ) ;
#99229=CARTESIAN_POINT ( 'NONE',  ( -2.197413446379999691, 1507.220826626529970, 180.8381795196980022 ) ) ;
#99232=EDGE_CURVE ( 'NONE', #36566, #36154, #24949, .T. ) ;
#99233=CARTESIAN_POINT ( 'NONE',  ( 11.86013743380000030, 1462.256145969930003, 232.2216276054980142 ) ) ;
#99234=CARTESIAN_POINT ( 'NONE',  ( -11.60004869884504686, 1423.657758649147581, 137.0691908906612753 ) ) ;
#99235=B_SPLINE_CURVE_WITH_KNOTS ( 'NONE', 2,
 ( #87418, #27498, #10714, #95263, #1779 ),
 .UNSPECIFIED., .F., .F.,
 ( 3, 2, 3 ),
 ( 0.000000000000000000, 0.5000000000000000000, 1.000000000000000000 ),
 .UNSPECIFIED. ) ;
#99236=CARTESIAN_POINT ( 'NONE',  ( -0.1562295872588534418, 1410.302064320732597, 233.2305516458151828 ) ) ;
#99237=B_SPLINE_SURFACE_WITH_KNOTS ( 'NONE', 5, 5, ( 
 ( #68178, #100628, #102285, #109061, #25566, #51338, #32344, #66524, #41294 ),
 ( #75468, #109602, #101170, #53019, #87154, #18273, #2626, #52466, #37310 ),
 ( #105062, #61984, #88262, #19375, #53578, #87725, #1507, #95005, #79316 ),
 ( #86596, #77651, #11003, #63103, #45175, #2072, #36203, #11555, #43507 ),
 ( #35638, #36752, #78757, #70944, #70387, #62546, #9888, #45732, #44056 ),
 ( #78196, #104504, #965, #69832, #28351, #97200, #28908, #20473, #103949 ) ),
 .UNSPECIFIED., .F., .F., .F.,
 ( 6, 6 ),
 ( 6, 3, 6 ),
 ( 0.4666582265029999843, 2.797885342349890170 ),
 ( -1.082959988738329909E-05, 1.000000000000000000, 2.000000000000000000 ),
 .UNSPECIFIED. ) ;
#99240=CARTESIAN_POINT ( 'NONE',  ( -0.1052129130517930056, 1508.249961362639851, 180.4882525773680015 ) ) ;
#99249=CARTESIAN_POINT ( 'NONE',  ( -11.30047077689999924, 1432.243567658440043, 151.5215873816980263 ) ) ;
#99253=CARTESIAN_POINT ( 'NONE',  ( 6.413908346207559674, 1429.087432367279916, 154.6253934533610277 ) ) ;
#99256=CARTESIAN_POINT ( 'NONE',  ( -18.79847754549999905, 1457.450606964430108, 227.1476812467979869 ) ) ;
#99258=CARTESIAN_POINT ( 'NONE',  ( -1.783662796859999844, 1484.717543678729953, 182.7833423215980133 ) ) ;
#99259=ORIENTED_EDGE ( 'NONE', *, *, #83400, .T. ) ;
#99261=CARTESIAN_POINT ( 'NONE',  ( 9.884505093230000483, 1406.768685218130031, 266.9235441556980390 ) ) ;
#99263=CARTESIAN_POINT ( 'NONE',  ( 20.10957645199999888, 1410.870268510630012, 197.6120402619980041 ) ) ;
#99264=ADVANCED_FACE ( 'NONE', ( #20838 ), #45695, .F. ) ;
#99265=CARTESIAN_POINT ( 'NONE',  ( 24.58038383556951700, 1439.418613111171453, 212.5155431820280683 ) ) ;
#99266=EDGE_CURVE ( 'NONE', #54755, #110792, #12099, .T. ) ;
#99267=CARTESIAN_POINT ( 'NONE',  ( 10.37019963556298841, 1423.186367574259748, 137.2231398063942436 ) ) ;
#99268=EDGE_CURVE ( 'NONE', #80633, #104047, #22165, .T. ) ;
#99269=CARTESIAN_POINT ( 'NONE',  ( 4.363122647530000009, 1421.075575420230052, 170.1076616725979989 ) ) ;
#99270=CARTESIAN_POINT ( 'NONE',  ( -1.981093173629999926, 1450.324655959600022, 155.6080925165979920 ) ) ;
#99272=ADVANCED_FACE ( 'NONE', ( #56669 ), #58893, .T. ) ;
#99273=CARTESIAN_POINT ( 'NONE',  ( -19.84490639471488649, 1485.616324373336283, 190.5157334858500633 ) ) ;
#99274=ADVANCED_FACE ( 'NONE', ( #63301 ), #108328, .T. ) ;
#99277=CARTESIAN_POINT ( 'NONE',  ( 8.881784197000000993E-16, 1412.362567936729874, 265.6112251771979800 ) ) ;
#99279=CARTESIAN_POINT ( 'NONE',  ( 4.222563055010000177, 1441.596179668460081, 170.5493975461980085 ) ) ;
#99280=CARTESIAN_POINT ( 'NONE',  ( -2.112521956910000220, 1476.073962097629874, 267.8521519262979496 ) ) ;
#99281=CARTESIAN_POINT ( 'NONE',  ( -10.73514658959810752, 1424.973046406437561, 139.1354236156141724 ) ) ;
#99282=CARTESIAN_POINT ( 'NONE',  ( -5.360152366205530150, 1422.242722016050038, 144.1549655170190078 ) ) ;
#99283=CARTESIAN_POINT ( 'NONE',  ( -11.67151907566795366, 1486.510180171227375, 184.2271218764052776 ) ) ;
#99291=CARTESIAN_POINT ( 'NONE',  ( -22.68024642580000005, 1410.626440472329932, 203.9056876081779990 ) ) ;
#99293=CARTESIAN_POINT ( 'NONE',  ( -15.03439673157799916, 1422.460132116142177, 229.1221540998959938 ) ) ;
#99300=CARTESIAN_POINT ( 'NONE',  ( 11.37055338930000126, 1425.522980547530096, 139.6335801328979755 ) ) ;
#99304=CARTESIAN_POINT ( 'NONE',  ( 40.08574870070000173, 1445.562093085849938, 136.8698620028980031 ) ) ;
#99307=CARTESIAN_POINT ( 'NONE',  ( -13.28956057169999916, 1415.163755984229965, 220.9230430223980193 ) ) ;
#99313=B_SPLINE_CURVE_WITH_KNOTS ( 'NONE', 5,
 ( #4716, #48953, #66858, #47281, #32679, #24264 ),
 .UNSPECIFIED., .F., .F.,
 ( 6, 6 ),
 ( 0.000000000000000000, 1.000000000000000000 ),
 .UNSPECIFIED. ) ;
#99317=CARTESIAN_POINT ( 'NONE',  ( -13.96458935331429174, 1446.023135734114703, 188.4738057646961806 ) ) ;
#99318=CARTESIAN_POINT ( 'NONE',  ( -22.02326011579999943, 1411.040515729830076, 214.9716949974079796 ) ) ;
#99319=CARTESIAN_POINT ( 'NONE',  ( 2.087781203659999640, 1508.813655593830163, 237.6275677719980024 ) ) ;
#99320=CARTESIAN_POINT ( 'NONE',  ( -12.99573497267853739, 1444.878364782870221, 169.4220454143612073 ) ) ;
#99321=CARTESIAN_POINT ( 'NONE',  ( -24.90417444750000087, 1509.109214294029925, 197.4104332050980304 ) ) ;
#99324=CARTESIAN_POINT ( 'NONE',  ( 17.46592908230000063, 1416.259332967430055, 226.1411364642979720 ) ) ;
#99325=CARTESIAN_POINT ( 'NONE',  ( 2.498440639099999583, 1429.771114423330118, 184.7212983517980263 ) ) ;
#99327=CARTESIAN_POINT ( 'NONE',  ( -41.45642610774959991, 1445.626696643309970, 135.8732978911219789 ) ) ;
#99328=CARTESIAN_POINT ( 'NONE',  ( 9.141780084607901813, 1396.232298419879726, 202.9009529963200009 ) ) ;
#99329=CARTESIAN_POINT ( 'NONE',  ( 33.91375399455670703, 1437.010669090869897, 136.5612025278969952 ) ) ;
#99330=CARTESIAN_POINT ( 'NONE',  ( 11.73709356400000026, 1426.695943121429991, 144.1748013713979901 ) ) ;
#99331=CARTESIAN_POINT ( 'NONE',  ( 8.979367357839899810, 1509.226626805293563, 181.2302862350315991 ) ) ;
#99333=CARTESIAN_POINT ( 'NONE',  ( 3.791089716489999706, 1424.059099777229903, 184.0089410633980265 ) ) ;
#99334=CARTESIAN_POINT ( 'NONE',  ( 1.737175160616053260, 1450.466040294496452, 181.7986353519378326 ) ) ;
#99340=CARTESIAN_POINT ( 'NONE',  ( 13.06509470220000146, 1434.822844257089855, 195.5376774312979933 ) ) ;
#99343=ORIENTED_EDGE ( 'NONE', *, *, #15204, .T. ) ;
#99345=CARTESIAN_POINT ( 'NONE',  ( 2.500000000000000000, 1448.894380902750072, 155.6080914261119972 ) ) ;
#99348=CARTESIAN_POINT ( 'NONE',  ( 16.32914645889999861, 1414.913060387329779, 212.3586363723179886 ) ) ;
#99352=CARTESIAN_POINT ( 'NONE',  ( -19.89462864549999921, 1508.347918161529833, 229.2892912506979997 ) ) ;
#99353=B_SPLINE_SURFACE_WITH_KNOTS ( 'NONE', 2, 5, ( 
 ( #21607, #72597, #29471, #64206, #30016, #3208 ),
 ( #46859, #37890, #72073, #56347, #38422, #37336 ),
 ( #28939, #89389, #12679, #47395, #80445, #4294 ) ),
 .UNSPECIFIED., .F., .F., .F.,
 ( 3, 3 ),
 ( 6, 6 ),
 ( 1.399803019399999959, 2.016961153140000018 ),
 ( 0.000000000000000000, 1.000000000000000000 ),
 .UNSPECIFIED. ) ;
#99354=CARTESIAN_POINT ( 'NONE',  ( -16.18025473180839668, 1412.759566377935926, 269.3698341425424587 ) ) ;
#99356=CARTESIAN_POINT ( 'NONE',  ( 1.600048698852036821, 1411.254281879943164, 135.5999999980979851 ) ) ;
#99357=ORIENTED_EDGE ( 'NONE', *, *, #366, .F. ) ;
#99358=CARTESIAN_POINT ( 'NONE',  ( 2.500000000000000000, 1419.623475504530006, 147.1347451145979903 ) ) ;
#99359=CARTESIAN_POINT ( 'NONE',  ( -33.37279912171400298, 1440.913060389960037, 247.4612066733249947 ) ) ;
#99361=CARTESIAN_POINT ( 'NONE',  ( -0.2518430497564930204, 1466.381564116799836, 235.6808877654009962 ) ) ;
#99364=CARTESIAN_POINT ( 'NONE',  ( 6.238299656213650124, 1410.363799256209859, 269.8684970340120231 ) ) ;
#99367=CARTESIAN_POINT ( 'NONE',  ( 23.92887862800000320, 1410.398442247130106, 209.4513301797530005 ) ) ;
#99368=CARTESIAN_POINT ( 'NONE',  ( -20.54038862950000066, 1509.293030658830048, 188.7525476221979943 ) ) ;
#99373=CARTESIAN_POINT ( 'NONE',  ( 0.3641805758275279969, 1424.317995888269934, 227.5054904079770211 ) ) ;
#99374=CARTESIAN_POINT ( 'NONE',  ( 0.07204396340539999388, 1420.438790373129905, 183.3235068346980086 ) ) ;
#99375=CARTESIAN_POINT ( 'NONE',  ( 10.71453348701945885, 1425.002631316717952, 137.0999999980979283 ) ) ;
#99377=EDGE_LOOP ( 'NONE', ( #95764, #110094, #80651, #78794 ) ) ;
#99379=EDGE_CURVE ( 'NONE', #71213, #96354, #90908, .T. ) ;
#99380=CARTESIAN_POINT ( 'NONE',  ( 18.95816156469999925, 1416.822692809329965, 210.4639564331680219 ) ) ;
#99384=CARTESIAN_POINT ( 'NONE',  ( -5.506656393879999278, 1440.093542876940091, 154.7592574253979762 ) ) ;
#99393=VERTEX_POINT ( 'NONE', #35733 ) ;
#99394=CARTESIAN_POINT ( 'NONE',  ( 28.32265144099999787, 1509.673549454430031, 207.2611521168180104 ) ) ;
#99396=CARTESIAN_POINT ( 'NONE',  ( 21.00628566139999975, 1454.076385129430037, 222.0485915842979807 ) ) ;
#99397=( BOUNDED_CURVE ( )  B_SPLINE_CURVE ( 3, ( #106605, #56214, #82521, #64084 ),
 .UNSPECIFIED., .F., .F. ) 
 B_SPLINE_CURVE_WITH_KNOTS ( ( 4, 4 ),
 ( 1.227519483377339959, 1.249431231073490078 ),
 .UNSPECIFIED. ) 
 CURVE ( )  GEOMETRIC_REPRESENTATION_ITEM ( )  RATIONAL_B_SPLINE_CURVE ( ( 1.000000000000000000, 0.9999599900096145522, 0.9999599900096145522, 1.000000000000000000 ) ) 
 REPRESENTATION_ITEM ( '' )  );
#99398=CARTESIAN_POINT ( 'NONE',  ( 7.878720380360996423, 1438.230628562198945, 153.7443670316927182 ) ) ;
#99401=CARTESIAN_POINT ( 'NONE',  ( -26.80674662115270124, 1509.211243910479880, 201.3592588738389964 ) ) ;
#99402=B_SPLINE_CURVE_WITH_KNOTS ( 'NONE', 3,
 ( #98857, #89363, #54137, #12656, #97203, #96670, #47914, #46835, #106166, #89905, #88813, #80963, #37313, #64744, #64184, #73119 ),
 .UNSPECIFIED., .F., .F.,
 ( 4, 2, 2, 2, 2, 2, 2, 4 ),
 ( 3.254750701746227874E-09, 6.242996095738161545E-05, 0.0001248566671640615031, 0.0002497100795776726776, 0.0004994169044049760709, 0.0009988305540596259004, 0.001997657853369099248, 0.003995312451988130079 ),
 .UNSPECIFIED. ) ;
#99403=CARTESIAN_POINT ( 'NONE',  ( -3.667959980290000033, 1446.440575669779946, 162.7182840746979764 ) ) ;
#99404=CARTESIAN_POINT ( 'NONE',  ( -18.76055448960000049, 1425.655531962830082, 225.4079628041980072 ) ) ;
#99407=CARTESIAN_POINT ( 'NONE',  ( 18.54207614579999941, 1507.885690588130046, 188.5212023680979883 ) ) ;
#99408=CARTESIAN_POINT ( 'NONE',  ( -34.76957446138440844, 1458.023740881216781, 269.5283794133094943 ) ) ;
#99415=CARTESIAN_POINT ( 'NONE',  ( -1.137831637353148961, 1408.952794343696041, 186.7671043909383570 ) ) ;
#99416=B_SPLINE_CURVE_WITH_KNOTS ( 'NONE', 3,
 ( #35879, #1740, #70063, #26922, #95774, #53243, #68395, #19040, #95226, #34762, #18489, #103050, #68950, #86821, #78999, #44846, #104724, #28014, #94107, #10113, #44285, #87384, #27459, #62201, #10679, #2302, #53809, #36413, #70605, #96329, #26348, #77876, #79537, #102501, #60546, #43722, #19607 ),
 .UNSPECIFIED., .F., .F.,
 ( 4, 3, 3, 3, 3, 3, 3, 3, 3, 3, 3, 3, 4 ),
 ( -1.999999848934280067, -1.897891338336010092, -1.728761199251590108, -1.557452154569009872, -1.384905005406759981, -1.210695233754919942, -1.035838574448660010, -0.8607549794867428439, -0.6858798840580180300, -0.5121999522673421623, -0.3398111951967790478, -0.1690102479686510506, -5.799765116165644940E-06 ),
 .UNSPECIFIED. ) ;
#99417=CARTESIAN_POINT ( 'NONE',  ( -13.40117755332782856, 1443.408819078402530, 187.0327686018816280 ) ) ;
#99418=CARTESIAN_POINT ( 'NONE',  ( -3.827327205999999649, 1409.546157813730133, 121.6099336315979969 ) ) ;
#99419=FACE_OUTER_BOUND ( 'NONE', #88641, .T. ) ;
#99420=EDGE_CURVE ( 'NONE', #31602, #8790, #101484, .T. ) ;
#99421=CARTESIAN_POINT ( 'NONE',  ( -2.052509464423307950, 1415.610420790406124, 233.0191148808001458 ) ) ;
#99424=CARTESIAN_POINT ( 'NONE',  ( 24.40297774660000485, 1435.533511806519982, 137.4233649837979954 ) ) ;
#99425=CARTESIAN_POINT ( 'NONE',  ( -13.25973371150704416, 1443.185291380165609, 169.3834991182581007 ) ) ;
#99426=CARTESIAN_POINT ( 'NONE',  ( -14.30199729709999978, 1410.347835160429895, 226.8241708172980111 ) ) ;
#99430=ORIENTED_EDGE ( 'NONE', *, *, #102147, .T. ) ;
#99435=CARTESIAN_POINT ( 'NONE',  ( -27.24390625670000077, 1454.605078679430108, 244.3119003928979964 ) ) ;
#99437=EDGE_CURVE ( 'NONE', #57683, #89981, #105109, .T. ) ;
#99438=CARTESIAN_POINT ( 'NONE',  ( -11.51652132750000135, 1433.525180497049860, 151.2587270096979921 ) ) ;
#99439=CARTESIAN_POINT ( 'NONE',  ( 14.38276615817169635, 1509.537722092532931, 235.4493228184925897 ) ) ;
#99446=CARTESIAN_POINT ( 'NONE',  ( 451.6689809271080094, 1435.140433208369814, 155.5900787298459704 ) ) ;
#99448=CARTESIAN_POINT ( 'NONE',  ( -16.65108875018284706, 1509.615391758380611, 234.1414537928058337 ) ) ;
#99450=CARTESIAN_POINT ( 'NONE',  ( -7.915285451137539677E-10, 1412.889808523510055, 251.0689582627720426 ) ) ;
#99453=CARTESIAN_POINT ( 'NONE',  ( -11.85932238006850170, 1431.862983400520079, 149.9619179884730045 ) ) ;
#99455=CARTESIAN_POINT ( 'NONE',  ( -5.184304023010000151, 1471.561735541330108, 269.8675879627980407 ) ) ;
#99456=CARTESIAN_POINT ( 'NONE',  ( 12.89273669479999995, 1508.859229393329997, 233.8778408584979900 ) ) ;
#99458=CARTESIAN_POINT ( 'NONE',  ( -13.97684781309999913, 1452.404795722730114, 223.0329335630979983 ) ) ;
#99459=CARTESIAN_POINT ( 'NONE',  ( 0.3742949575629109793, 1450.903878863470027, 181.4136564121010053 ) ) ;
#99464=CARTESIAN_POINT ( 'NONE',  ( -27.39518923616549984, 1412.781094389850068, 268.7457036271840138 ) ) ;
#99466=CARTESIAN_POINT ( 'NONE',  ( -3.535949085321830498, 1494.186315171800061, 181.5280936908750107 ) ) ;
#99470=FACE_OUTER_BOUND ( 'NONE', #76659, .T. ) ;
#99471=CARTESIAN_POINT ( 'NONE',  ( 41.65675406397859604, 1443.992462633329978, 135.6790809494980010 ) ) ;
#99474=CARTESIAN_POINT ( 'NONE',  ( -15.19110828580000039, 1440.435427132970062, 189.4075412060980170 ) ) ;
#99475=CARTESIAN_POINT ( 'NONE',  ( -2.447859506707243060, 1449.353156360412186, 183.0517911818036794 ) ) ;
#99476=VERTEX_POINT ( 'NONE', #34438 ) ;
#99480=CARTESIAN_POINT ( 'NONE',  ( -42.54898869008160034, 1440.913047336420050, 270.0692026506110324 ) ) ;
#99482=CARTESIAN_POINT ( 'NONE',  ( -4.606808002230000199, 1396.134576369729984, 198.3574891071980062 ) ) ;
#99485=VERTEX_POINT ( 'NONE', #59109 ) ;
#99486=CARTESIAN_POINT ( 'NONE',  ( -1.793335950739999962, 1419.496365638530051, 185.6406336190979971 ) ) ;
#99487=CARTESIAN_POINT ( 'NONE',  ( 3.746090737668994031, 1425.475261178803976, 185.1844613459034576 ) ) ;
#99488=CARTESIAN_POINT ( 'NONE',  ( -14.25613302710000063, 1464.413060387330006, 194.1747703853979772 ) ) ;
#99490=CARTESIAN_POINT ( 'NONE',  ( 18.65451742820949832, 1507.632629731499947, 188.5326158842280222 ) ) ;
#99494=CARTESIAN_POINT ( 'NONE',  ( 5.492221782479999703, 1439.600215925499924, 154.7521915351979942 ) ) ;
#99497=CARTESIAN_POINT ( 'NONE',  ( 18.80463393750000023, 1425.801073282529842, 225.6039001781980176 ) ) ;
#99501=CARTESIAN_POINT ( 'NONE',  ( -40.71747596589660390, 1438.773003664010048, 134.7398499747960159 ) ) ;
#99502=CARTESIAN_POINT ( 'NONE',  ( -11.74015320060000001, 1428.979986575930070, 144.1938086916980239 ) ) ;
#99507=CARTESIAN_POINT ( 'NONE',  ( 23.84493162013280099, 1452.080376998370184, 136.9869860125139951 ) ) ;
#99508=CARTESIAN_POINT ( 'NONE',  ( 13.88473851270000026, 1415.296882296330068, 197.4370144994979910 ) ) ;
#99510=CARTESIAN_POINT ( 'NONE',  ( 26.69873419689999849, 1451.980699541129979, 134.9231770738980174 ) ) ;
#99511=CARTESIAN_POINT ( 'NONE',  ( -26.79413315976150045, 1435.433175095809929, 135.2874648155150226 ) ) ;
#99514=DIRECTION ( 'NONE',  ( 0.000000000000000000, -1.000000000000000000, 0.000000000000000000 ) ) ;
#99515=CARTESIAN_POINT ( 'NONE',  ( 2.500000000000000000, 1439.509563800350179, 163.9071484463910053 ) ) ;
#99516=CARTESIAN_POINT ( 'NONE',  ( -16.19086242769280304, 1409.478452467050147, 225.0103265570539861 ) ) ;
#99520=CARTESIAN_POINT ( 'NONE',  ( -2.339369569539999638, 1474.134115800729887, 270.1366117264980176 ) ) ;
#99521=CARTESIAN_POINT ( 'NONE',  ( -3.090243552160000018, 1448.623823917879918, 184.7128630361980015 ) ) ;
#99524=CARTESIAN_POINT ( 'NONE',  ( 0.2178157486290130118, 1452.982786607829894, 183.2541296479709843 ) ) ;
#99526=CARTESIAN_POINT ( 'NONE',  ( 30.83123567651259833, 1510.067171565570106, 207.3056169179679671 ) ) ;
#99527=CARTESIAN_POINT ( 'NONE',  ( 11.60004869885203682, 1426.461398603654288, 139.0972022331852145 ) ) ;
#99528=DIRECTION ( 'NONE',  ( 0.000000000000000000, 0.000000000000000000, -1.000000000000000000 ) ) ;
#99529=CARTESIAN_POINT ( 'NONE',  ( -2.500000000000000000, 1421.745358796729988, 151.9633565684980283 ) ) ;
#99532=CARTESIAN_POINT ( 'NONE',  ( -4.790712462651379169E-07, 1408.860257374809862, 223.5938187205209999 ) ) ;
#99533=CARTESIAN_POINT ( 'NONE',  ( 29.92073223143840011, 1440.913060386099914, 238.0971241985569975 ) ) ;
#99542=CARTESIAN_POINT ( 'NONE',  ( 17.38482601099109814, 1410.884446382940041, 192.4603632472940262 ) ) ;
#99545=CARTESIAN_POINT ( 'NONE',  ( 2.279486850145009846, 1508.935250638985735, 237.8394454178328488 ) ) ;
#99546=CARTESIAN_POINT ( 'NONE',  ( 18.18137293399999876, 1507.546748832030062, 186.5307135875980009 ) ) ;
#99547=EDGE_CURVE ( 'NONE', #91877, #93336, #89021, .T. ) ;
#99548=CARTESIAN_POINT ( 'NONE',  ( 15.09682228229999978, 1409.610690924630035, 192.0685155598980032 ) ) ;
#99549=CARTESIAN_POINT ( 'NONE',  ( -5.430576729993609852, 1440.816380553300178, 154.8042786586000261 ) ) ;
#99552=CARTESIAN_POINT ( 'NONE',  ( -12.78755494719999852, 1416.844618642330033, 195.3259368849979865 ) ) ;
#99555=CARTESIAN_POINT ( 'NONE',  ( 2.502826361999999971, 1464.606218255329850, 236.1230330374980042 ) ) ;
#99557=ORIENTED_EDGE ( 'NONE', *, *, #53463, .T. ) ;
#99558=CARTESIAN_POINT ( 'NONE',  ( -0.8228443623879999613, 1450.943455458130074, 182.1014883083980180 ) ) ;
#99561=CARTESIAN_POINT ( 'NONE',  ( -18.05542472024740164, 1416.825783990419950, 209.4840485447890046 ) ) ;
#99563=ORIENTED_EDGE ( 'NONE', *, *, #44571, .F. ) ;
#99565=CARTESIAN_POINT ( 'NONE',  ( 35.75324696180250328, 1437.345929592409902, 136.5360666854240037 ) ) ;
#99567=CARTESIAN_POINT ( 'NONE',  ( -37.65047686723229958, 1442.773887284729881, 137.1096749952629921 ) ) ;
#99570=DIRECTION ( 'NONE',  ( -0.9417419115949053898, -0.3363363969979660806, 9.559255346349054600E-15 ) ) ;
#99571=CARTESIAN_POINT ( 'NONE',  ( 7.948017842360480145, 1409.190611286300282, 196.4401314888699801 ) ) ;
#99572=CARTESIAN_POINT ( 'NONE',  ( 18.12086373898799962, 1425.009007305328169, 225.3873405099579941 ) ) ;
#99578=CARTESIAN_POINT ( 'NONE',  ( -3.884405768773259826, 1449.583267633219975, 185.0056059189860207 ) ) ;
#99579=ORIENTED_EDGE ( 'NONE', *, *, #14706, .T. ) ;
#99580=EDGE_CURVE ( 'NONE', #109851, #56546, #72913, .T. ) ;
#99583=CARTESIAN_POINT ( 'NONE',  ( -12.82272891259999881, 1434.845015028379976, 150.1638710903980041 ) ) ;
#99585=CARTESIAN_POINT ( 'NONE',  ( -20.27149120612340027, 1497.224176212940165, 190.6980538895379880 ) ) ;
#99590=CARTESIAN_POINT ( 'NONE',  ( -46.14542121321060364, 1440.248490524040108, 268.2047085544609786 ) ) ;
#99591=CARTESIAN_POINT ( 'NONE',  ( 13.42361184146170139, 1508.223676004419985, 233.2139651083469971 ) ) ;
#99592=CARTESIAN_POINT ( 'NONE',  ( -19.99752153760000084, 1488.350075126529873, 191.5586291822979774 ) ) ;
#99594=CARTESIAN_POINT ( 'NONE',  ( 4.214930602837739571, 1408.999354465240231, 222.9586692084779997 ) ) ;
#99599=VERTEX_POINT ( 'NONE', #20925 ) ;
#99600=CARTESIAN_POINT ( 'NONE',  ( 14.70061896029999993, 1417.388462482229897, 244.5173668933980196 ) ) ;
#99602=CARTESIAN_POINT ( 'NONE',  ( -3.518337011159999861, 1478.170661589230122, 182.2087550695979985 ) ) ;
#99604=CARTESIAN_POINT ( 'NONE',  ( 1.514918641329773497, 1508.378724870832229, 180.6682338045059169 ) ) ;
#99605=CARTESIAN_POINT ( 'NONE',  ( 1.436583437199999868E-09, 1416.682256489629935, 238.2947547783980156 ) ) ;
#99606=CARTESIAN_POINT ( 'NONE',  ( -29.63440978849957474, 1509.974483337211041, 207.3636310854570866 ) ) ;
#99607=CARTESIAN_POINT ( 'NONE',  ( -18.16938274068190040, 1452.278571560799946, 145.2377407453319904 ) ) ;
#99608=CARTESIAN_POINT ( 'NONE',  ( 27.85266659460000227, 1451.078832383830104, 136.3466686027980188 ) ) ;
#99610=CARTESIAN_POINT ( 'NONE',  ( -2.500000000000000000, 1420.232870451130111, 149.2693594355980053 ) ) ;
#99612=CARTESIAN_POINT ( 'NONE',  ( 16.65265346172540006, 1423.208279008830004, 227.6530141284199829 ) ) ;
#99614=ORIENTED_EDGE ( 'NONE', *, *, #28932, .T. ) ;
#99615=ORIENTED_EDGE ( 'NONE', *, *, #83871, .F. ) ;
#99617=CARTESIAN_POINT ( 'NONE',  ( -24.12531086176590378, 1410.986997877699878, 208.8764144295159895 ) ) ;
#99619=DIRECTION ( 'NONE',  ( -0.09060005235378243427, 0.000000000000000000, 0.9958873583460591261 ) ) ;
#99622=CARTESIAN_POINT ( 'NONE',  ( -9.872048858160001217, 1498.343720009429944, 234.1146122690979894 ) ) ;
#99623=CARTESIAN_POINT ( 'NONE',  ( -1.775935834183570261, 1421.047323150906550, 184.1901391204128799 ) ) ;
#99624=CARTESIAN_POINT ( 'NONE',  ( 43.21760421406469987, 1452.663687658380013, 268.8371515474040052 ) ) ;
#99625=CARTESIAN_POINT ( 'NONE',  ( -12.81744069099319994, 1415.938742849230039, 221.7277189786869940 ) ) ;
#99631=CARTESIAN_POINT ( 'NONE',  ( 12.89353391096544676, 1442.888115666797830, 187.0162393882783078 ) ) ;
#99632=ORIENTED_EDGE ( 'NONE', *, *, #52901, .T. ) ;
#99633=VERTEX_POINT ( 'NONE', #89251 ) ;
#99638=CARTESIAN_POINT ( 'NONE',  ( -1.718340007434250173E-05, 1407.928426573429988, 270.2927087787980440 ) ) ;
#99640=CARTESIAN_POINT ( 'NONE',  ( 10.98083629090000102, 1433.016921068679949, 151.7694307944979926 ) ) ;
#99642=PLANE ( 'NONE',  #66102 ) ;
#99643=CARTESIAN_POINT ( 'NONE',  ( -16.75267927776890176, 1413.684132339210009, 191.6587516336579995 ) ) ;
#99648=CARTESIAN_POINT ( 'NONE',  ( -24.66395196768430154, 1509.340428037599850, 222.6198678659309849 ) ) ;
#99650=VERTEX_POINT ( 'NONE', #104955 ) ;
#99651=CARTESIAN_POINT ( 'NONE',  ( 19.00000000000000000, 1438.871025162500018, 209.1218459616979999 ) ) ;
#99652=CARTESIAN_POINT ( 'NONE',  ( -0.2626388801599250367, 1424.255108689230156, 227.7923674788299877 ) ) ;
#99658=VERTEX_POINT ( 'NONE', #46179 ) ;
#99661=CARTESIAN_POINT ( 'NONE',  ( -14.35469252290000064, 1416.832348304330026, 221.5787001177979789 ) ) ;
#99662=FACE_OUTER_BOUND ( 'NONE', #55574, .T. ) ;
#99663=EDGE_CURVE ( 'NONE', #100437, #5014, #41038, .T. ) ;
#99664=CARTESIAN_POINT ( 'NONE',  ( 36.06124927020000115, 1445.049634744800187, 262.6648722463980334 ) ) ;
#99669=CARTESIAN_POINT ( 'NONE',  ( 7.421564111899999538, 1419.755070490029993, 231.1403862899979913 ) ) ;
#99670=CARTESIAN_POINT ( 'NONE',  ( 0.000000000000000000, 1512.413060387330006, 209.1218459616979999 ) ) ;
#99672=DIRECTION ( 'NONE',  ( 0.000000000000000000, 1.000000000000000000, 0.000000000000000000 ) ) ;
#99676=EDGE_CURVE ( 'NONE', #20182, #62097, #52960, .T. ) ;
#99680=CARTESIAN_POINT ( 'NONE',  ( -5.681577072609999668, 1414.971279908829956, 225.1170751815979827 ) ) ;
#99681=CARTESIAN_POINT ( 'NONE',  ( 0.2155153167960190130, 1454.260632470949986, 183.1993150321829944 ) ) ;
#99682=CARTESIAN_POINT ( 'NONE',  ( -13.31542525870250060, 1407.755358688280012, 207.9544151864530193 ) ) ;
#99685=EDGE_CURVE ( 'NONE', #104141, #85887, #103331, .T. ) ;
#99686=CARTESIAN_POINT ( 'NONE',  ( -28.22512692420650282, 1509.373780534800062, 210.8894252387570134 ) ) ;
#99687=CARTESIAN_POINT ( 'NONE',  ( 12.91294366230000179, 1434.774374641290024, 149.1897813115979829 ) ) ;
#99688=CARTESIAN_POINT ( 'NONE',  ( -34.51820589334170108, 1435.725758536279955, 134.0999999979759707 ) ) ;
#99689=CARTESIAN_POINT ( 'NONE',  ( 12.24119640919999874, 1442.732430062529829, 186.9125350121979920 ) ) ;
#99690=VERTEX_POINT ( 'NONE', #92541 ) ;
#99693=CARTESIAN_POINT ( 'NONE',  ( 39.08053441540000250, 1436.812233320949872, 136.3561087622979926 ) ) ;
#99696=CARTESIAN_POINT ( 'NONE',  ( 16.69548807383920064, 1509.501171630579847, 233.4225513957580063 ) ) ;
#99697=AXIS2_PLACEMENT_3D ( 'NONE', #103418, #77690, #44097 ) ;
#99698=CARTESIAN_POINT ( 'NONE',  ( 42.02056136452171842, 1427.554426610052360, 269.0752184054053373 ) ) ;
#99704=CARTESIAN_POINT ( 'NONE',  ( 21.33070998320000200, 1509.431296620630064, 227.6602567435979836 ) ) ;
#99706=CARTESIAN_POINT ( 'NONE',  ( -28.32839677941640133, 1508.625224776620144, 208.8290590941180085 ) ) ;
#99707=CARTESIAN_POINT ( 'NONE',  ( -16.03670630470179859, 1410.715819712529992, 226.6960494820459928 ) ) ;
#99712=ADVANCED_FACE ( 'NONE', ( #31540 ), #64627, .F. ) ;
#99715=CARTESIAN_POINT ( 'NONE',  ( -0.1030177700933130047, 1419.835433905890113, 184.1455088873570105 ) ) ;
#99716=CARTESIAN_POINT ( 'NONE',  ( 1.089618986890000141, 1466.173027012529928, 235.3909690008979965 ) ) ;
#99717=CARTESIAN_POINT ( 'NONE',  ( 23.18583117279999684, 1410.644154559629897, 212.8685298154279906 ) ) ;
#99718=CARTESIAN_POINT ( 'NONE',  ( -2.191379157991490079, 1412.648780287710224, 186.2800507015870153 ) ) ;
#99720=CARTESIAN_POINT ( 'NONE',  ( -17.45904667960000012, 1423.446827278330147, 226.6221925633979879 ) ) ;
#99722=CARTESIAN_POINT ( 'NONE',  ( -3.087788399999999989, 1439.686999668429962, 185.1123624746980170 ) ) ;
#99726=CARTESIAN_POINT ( 'NONE',  ( -23.53568538760000095, 1430.818610655530165, 211.5316886895479911 ) ) ;
#99727=AXIS2_PLACEMENT_3D ( 'NONE', #19695, #2933, #63397 ) ;
#99730=CARTESIAN_POINT ( 'NONE',  ( -3.427607156821979917, 1485.816111524730104, 182.6024182081450249 ) ) ;
#99731=ORIENTED_EDGE ( 'NONE', *, *, #84985, .F. ) ;
#99733=PLANE ( 'NONE',  #35801 ) ;
#99739=ORIENTED_EDGE ( 'NONE', *, *, #106127, .F. ) ;
#99740=VECTOR ( 'NONE', #1332, 999.9999999999998863 ) ;
#99743=CARTESIAN_POINT ( 'NONE',  ( 0.7352107454670000486, 1428.413060387330006, 91.31218443469779800 ) ) ;
#99744=CARTESIAN_POINT ( 'NONE',  ( 15.93516857634840278, 1410.115694288839904, 191.7361898460559928 ) ) ;
#99747=CARTESIAN_POINT ( 'NONE',  ( 40.22912568530000499, 1442.658719917350027, 137.0054168744979961 ) ) ;
#99750=CARTESIAN_POINT ( 'NONE',  ( 14.61595079141635622, 1462.229544524060429, 230.2230838894210478 ) ) ;
#99752=LINE ( 'NONE', #65635, #55202 ) ;
#99753=DIRECTION ( 'NONE',  ( 0.9993902469235412811, 0.03489947644508400310, -0.001077449749359510062 ) ) ;
#99755=DIRECTION ( 'NONE',  ( -1.000000000000000000, 0.000000000000000000, 0.000000000000000000 ) ) ;
#99757=ORIENTED_EDGE ( 'NONE', *, *, #33639, .T. ) ;
#99760=CARTESIAN_POINT ( 'NONE',  ( 0.002706352938670000211, 1450.912965879100057, 181.8859610906980038 ) ) ;
#99761=VECTOR ( 'NONE', #19688, 1000.000000000000114 ) ;
#99763=CARTESIAN_POINT ( 'NONE',  ( -2.500000000000000000, 1439.114301494319989, 157.7261950941980331 ) ) ;
#99765=CARTESIAN_POINT ( 'NONE',  ( 36.37832868398670172, 1451.642701156830071, 135.3769930297369797 ) ) ;
#99767=CARTESIAN_POINT ( 'NONE',  ( 26.68042020029999861, 1438.488799039590049, 136.9899190847980037 ) ) ;
#99768=CARTESIAN_POINT ( 'NONE',  ( 7.490736227920000267, 1414.913060387329779, 194.7918206520979822 ) ) ;
#99769=B_SPLINE_CURVE_WITH_KNOTS ( 'NONE', 3,
 ( #75771, #43279, #85249, #77425 ),
 .UNSPECIFIED., .F., .F.,
 ( 4, 4 ),
 ( 0.000000000000000000, 1.000000000000000000 ),
 .UNSPECIFIED. ) ;
#99775=CARTESIAN_POINT ( 'NONE',  ( 34.26305872384260454, 1440.913060387330006, 259.7236778358719675 ) ) ;
#99776=CARTESIAN_POINT ( 'NONE',  ( -0.0001975589939290832919, 1452.328857962840857, 153.7571063932752224 ) ) ;
#99777=ORIENTED_EDGE ( 'NONE', *, *, #90389, .F. ) ;
#99779=CARTESIAN_POINT ( 'NONE',  ( -15.51104348340000172, 1410.386807788529950, 191.0641050774980272 ) ) ;
#99782=CARTESIAN_POINT ( 'NONE',  ( -4.316841735459999718, 1421.954789602430083, 184.7991042349980262 ) ) ;
#99788=CARTESIAN_POINT ( 'NONE',  ( 17.22921662220000272, 1459.838650815730034, 228.5711330225980191 ) ) ;
#99789=CARTESIAN_POINT ( 'NONE',  ( -10.10004869885101009, 1422.222932908415260, 137.0999999980978714 ) ) ;
#99790=CARTESIAN_POINT ( 'NONE',  ( -4.618315814097702976, 1422.106628702972557, 184.6512326330956171 ) ) ;
#99796=CARTESIAN_POINT ( 'NONE',  ( 16.73897281474028631, 1449.350004377781488, 218.9967825959608092 ) ) ;
#99798=CARTESIAN_POINT ( 'NONE',  ( 18.52446843400000276, 1509.559949079429998, 186.5302684548980210 ) ) ;
#99802=CARTESIAN_POINT ( 'NONE',  ( -18.65451756193940014, 1507.632629711779828, 229.7110761618599781 ) ) ;
#99803=CARTESIAN_POINT ( 'NONE',  ( 24.59498549419999947, 1440.913060393719888, 213.3385281389280124 ) ) ;
#99804=CARTESIAN_POINT ( 'NONE',  ( -11.86483741480000198, 1432.251307157519932, 150.3967669623980044 ) ) ;
#99807=CARTESIAN_POINT ( 'NONE',  ( 6.330596736919809508, 1422.104800651550022, 147.4057713054710064 ) ) ;
#99811=CARTESIAN_POINT ( 'NONE',  ( -20.25856915909999856, 1457.444690063829967, 224.8321900254979937 ) ) ;
#99817=CARTESIAN_POINT ( 'NONE',  ( 3.401339724939999698, 1406.599585306829795, 269.4945997090979972 ) ) ;
#99818=CARTESIAN_POINT ( 'NONE',  ( -0.1600491160670000079, 1410.295025987830059, 185.0245251824980244 ) ) ;
#99819=VECTOR ( 'NONE', #16886, 1000.000000000000000 ) ;
#99820=CARTESIAN_POINT ( 'NONE',  ( 18.23351301940000369, 1410.878721802529981, 193.8722903718979751 ) ) ;
#99822=CARTESIAN_POINT ( 'NONE',  ( 24.18941653212194254, 1436.492649024060938, 213.3767979003249025 ) ) ;
#99824=CARTESIAN_POINT ( 'NONE',  ( -0.5697989934069560558, 1450.893162568020216, 155.6080925154190027 ) ) ;
#99827=CARTESIAN_POINT ( 'NONE',  ( -1.177008307996480152, 1450.813907466269711, 155.0627524578040095 ) ) ;
#99828=CARTESIAN_POINT ( 'NONE',  ( -12.41051836359999960, 1445.069699529200079, 185.9600399849980192 ) ) ;
#99830=CARTESIAN_POINT ( 'NONE',  ( -19.88955515405384133, 1484.852955906364514, 190.9985515883152516 ) ) ;
#99831=CARTESIAN_POINT ( 'NONE',  ( -14.13596061218840028, 1415.658863692520072, 221.0621937284620060 ) ) ;
#99833=CARTESIAN_POINT ( 'NONE',  ( -9.100166781252440273, 1409.230845213859993, 197.2463952335830015 ) ) ;
#99834=CARTESIAN_POINT ( 'NONE',  ( -26.96340810044629777, 1508.002441355999736, 211.5727766284590246 ) ) ;
#99835=CARTESIAN_POINT ( 'NONE',  ( 2.500000000000000000, 1438.975727077510101, 156.0986697955979992 ) ) ;
#99836=CARTESIAN_POINT ( 'NONE',  ( -2.776721148250000049, 1475.989443049229976, 268.4805436461979866 ) ) ;
#99837=CARTESIAN_POINT ( 'NONE',  ( -4.226172892403809556, 1446.259735967549886, 166.0433939504960108 ) ) ;
#99847=CARTESIAN_POINT ( 'NONE',  ( -19.70672637799999904, 1410.962757928930159, 197.6880275815980212 ) ) ;
#99854=CARTESIAN_POINT ( 'NONE',  ( 11.08531958919999916, 1425.204049180429820, 139.6337526468980172 ) ) ;
#99857=DIRECTION ( 'NONE',  ( -1.000000000000000000, 0.000000000000000000, 0.000000000000000000 ) ) ;
#99858=CARTESIAN_POINT ( 'NONE',  ( 39.86302261571789529, 1446.848482913750104, 136.6554637131669949 ) ) ;
#99861=CARTESIAN_POINT ( 'NONE',  ( -12.73682884018698758, 1398.290620877891797, 211.7349528390541593 ) ) ;
#99865=CARTESIAN_POINT ( 'NONE',  ( 20.81497463947879822, 1509.689032670049983, 230.4046146822830110 ) ) ;
#99869=CARTESIAN_POINT ( 'NONE',  ( -2.328768353080000075, 1395.994382770230231, 220.1364017053979865 ) ) ;
#99870=CARTESIAN_POINT ( 'NONE',  ( -21.63131569299999768, 1410.588498113729884, 216.4024978495980065 ) ) ;
#99871=VERTEX_POINT ( 'NONE', #92001 ) ;
#99872=CARTESIAN_POINT ( 'NONE',  ( -13.33598659858382618, 1444.533481128697531, 169.3750784523817003 ) ) ;
#99873=CARTESIAN_POINT ( 'NONE',  ( 21.89171915302359039, 1509.706674751428181, 229.1511294852978438 ) ) ;
#99874=DIRECTION ( 'NONE',  ( 0.000000000000000000, 0.000000000000000000, -1.000000000000000000 ) ) ;
#99876=CARTESIAN_POINT ( 'NONE',  ( -13.74978541103059904, 1508.254514242250025, 184.1447064633670152 ) ) ;
#99877=CARTESIAN_POINT ( 'NONE',  ( 1.415376035039999758, 1449.240524800240109, 183.6130213356980221 ) ) ;
#99881=B_SPLINE_SURFACE_WITH_KNOTS ( 'NONE', 5, 5, ( 
 ( #82808, #41375, #66041, #30188, #100165, #14492, #40256, #15577, #64382 ),
 ( #6655, #91211, #100702, #109137, #21771, #55972, #75540, #65485, #92307 ),
 ( #40809, #74987, #99594, #98503, #90096, #39713, #90652, #32419, #13379 ),
 ( #6101, #74438, #48123, #23449, #81691, #83911, #39142, #107455, #30750 ),
 ( #64931, #57644, #99044, #22322, #13936, #82262, #73877, #108005, #93124 ),
 ( #84718, #60104, #41071, #85267, #24792, #83617, #42184, #50043, #51141 ) ),
 .UNSPECIFIED., .F., .F., .F.,
 ( 6, 6 ),
 ( 6, 3, 6 ),
 ( 0.000000000000000000, 9.931187219381479636 ),
 ( 0.000000000000000000, 1.000000000000000000, 2.000000002426730372 ),
 .UNSPECIFIED. ) ;
#99882=CARTESIAN_POINT ( 'NONE',  ( 5.771317186272449717, 1396.114599253079859, 199.7147697363969883 ) ) ;
#99883=CARTESIAN_POINT ( 'NONE',  ( 1.237038659510000027, 1415.048591087029763, 191.5546371455980079 ) ) ;
#99884=CARTESIAN_POINT ( 'NONE',  ( 11.78240326789999948, 1427.379900601830059, 147.2810486092980113 ) ) ;
#99885=CARTESIAN_POINT ( 'NONE',  ( 2.409586283469999923, 1426.663880916129983, 144.1938086916980239 ) ) ;
#99886=ORIENTED_EDGE ( 'NONE', *, *, #64539, .F. ) ;
#99887=CARTESIAN_POINT ( 'NONE',  ( 13.12526434545569920, 1435.132197141100050, 150.0848052037160016 ) ) ;
#99891=CARTESIAN_POINT ( 'NONE',  ( -18.49177796861540202, 1468.166699000810013, 228.2165253284340167 ) ) ;
#99892=CARTESIAN_POINT ( 'NONE',  ( -2.799250156989999905, 1466.496106898330027, 235.0820921407980109 ) ) ;
#99898=ORIENTED_EDGE ( 'NONE', *, *, #39908, .T. ) ;
#99900=CARTESIAN_POINT ( 'NONE',  ( 2.500000000000000000, 1448.271836152329797, 165.0530739316030235 ) ) ;
#99906=ORIENTED_EDGE ( 'NONE', *, *, #83792, .T. ) ;
#99908=CARTESIAN_POINT ( 'NONE',  ( -20.84366584300000014, 1509.634592552130016, 230.0407975123980009 ) ) ;
#99909=ADVANCED_FACE ( 'NONE', ( #39398 ), #15018, .F. ) ;
#99910=CARTESIAN_POINT ( 'NONE',  ( -29.91807324427193748, 1419.517122880768056, 269.4699333455887995 ) ) ;
#99911=ADVANCED_FACE ( 'NONE', ( #100403 ), #34823, .F. ) ;
#99913=CARTESIAN_POINT ( 'NONE',  ( 0.007886336566007640797, 1415.935475482089942, 227.0236970807289936 ) ) ;
#99915=CARTESIAN_POINT ( 'NONE',  ( 24.57126086520000285, 1440.930726575820017, 213.1726801958579927 ) ) ;
#99916=CARTESIAN_POINT ( 'NONE',  ( -32.83528556352659677, 1440.913060389920020, 246.2013707445869954 ) ) ;
#99918=CARTESIAN_POINT ( 'NONE',  ( -0.2727009628635130301, 1465.116480817439879, 238.1272600893040021 ) ) ;
#99920=CARTESIAN_POINT ( 'NONE',  ( 15.21920960200000117, 1410.493944514729947, 270.4035064526980250 ) ) ;
#99922=CARTESIAN_POINT ( 'NONE',  ( 23.73706522670000041, 1410.130559204529845, 209.1801705544619949 ) ) ;
#99927=B_SPLINE_CURVE_WITH_KNOTS ( 'NONE', 5,
 ( #56667, #90803, #98097, #47166, #55578, #14084, #38742, #57782, #40395 ),
 .UNSPECIFIED., .F., .F.,
 ( 6, 3, 6 ),
 ( 0.000000000000000000, 0.3780778814934559473, 1.000000000000000000 ),
 .UNSPECIFIED. ) ;
#99928=CARTESIAN_POINT ( 'NONE',  ( -3.381815025240311634, 1447.294493428453052, 154.8487956087455473 ) ) ;
#99930=CARTESIAN_POINT ( 'NONE',  ( -10.11438356259093041, 1486.011445013448338, 183.8897573256294322 ) ) ;
#99932=EDGE_LOOP ( 'NONE', ( #104023, #24955, #72438 ) ) ;
#99934=CARTESIAN_POINT ( 'NONE',  ( 18.90749324119999741, 1416.833018152629847, 210.0260543018609951 ) ) ;
#99936=EDGE_CURVE ( 'NONE', #104782, #109848, #59699, .T. ) ;
#99937=CARTESIAN_POINT ( 'NONE',  ( -8.878956589741459737, 1509.223142555890036, 236.7286733813189983 ) ) ;
#99938=B_SPLINE_CURVE_WITH_KNOTS ( 'NONE', 5,
 ( #95318, #28667, #36513, #61741, #38160, #62872, #96424, #62297, #12404 ),
 .UNSPECIFIED., .F., .F.,
 ( 6, 3, 6 ),
 ( -157.9539410499999974, -142.4618993580000108, -78.28065404276159711 ),
 .UNSPECIFIED. ) ;
#99950=VECTOR ( 'NONE', #15673, 1000.000000000000000 ) ;
#99951=CARTESIAN_POINT ( 'NONE',  ( 19.81774543710000103, 1455.367724597530014, 224.1005748771979995 ) ) ;
#99955=CARTESIAN_POINT ( 'NONE',  ( 15.42145445766184686, 1420.877149889689235, 227.7429447766757846 ) ) ;
#99957=CARTESIAN_POINT ( 'NONE',  ( 39.97998863047710216, 1445.784950460129949, 136.8350985949439860 ) ) ;
#99958=CARTESIAN_POINT ( 'NONE',  ( -20.09064370129999944, 1427.417574131329957, 223.6716081326979975 ) ) ;
#99963=CARTESIAN_POINT ( 'NONE',  ( 19.58740883549999978, 1488.302744340930076, 189.9643116126979976 ) ) ;
#99964=CARTESIAN_POINT ( 'NONE',  ( -0.01757669524774119890, 1409.855414155669905, 233.2048809017120163 ) ) ;
#99965=CARTESIAN_POINT ( 'NONE',  ( -35.03848265734369960, 1457.732937364906093, 269.5320884425483428 ) ) ;
#99968=CARTESIAN_POINT ( 'NONE',  ( -19.60062230800302885, 1409.993166476541774, 269.5268391383848439 ) ) ;
#99970=CARTESIAN_POINT ( 'NONE',  ( -10.60236678890000128, 1431.113060387329824, 224.6557647168980338 ) ) ;
#99971=B_SPLINE_CURVE_WITH_KNOTS ( 'NONE', 3,
 ( #48669, #40241, #25074, #84454, #84987, #100149 ),
 .UNSPECIFIED., .F., .F.,
 ( 4, 2, 4 ),
 ( 1.000000006357030081E-06, 0.7542730840691190819, 1.502771284927904238 ),
 .UNSPECIFIED. ) ;
#99972=CARTESIAN_POINT ( 'NONE',  ( 11.60004869885203327, 1428.043774929915571, 134.2198016428816914 ) ) ;
#99973=CARTESIAN_POINT ( 'NONE',  ( -12.92817269062425467, 1442.906901620904819, 186.4515505936974762 ) ) ;
#99974=DIRECTION ( 'NONE',  ( -0.8564730265368828421, -0.5161917810414574648, 0.000000000000000000 ) ) ;
#99977=CARTESIAN_POINT ( 'NONE',  ( -2.773560967585325887, 1415.718487882860018, 232.8280475519434560 ) ) ;
#99980=CARTESIAN_POINT ( 'NONE',  ( 23.85742997590000414, 1435.349283830410059, 137.3962418501980380 ) ) ;
#99982=B_SPLINE_CURVE_WITH_KNOTS ( 'NONE', 5,
 ( #55609, #47193, #99213, #81319, #4633, #38771, #72945, #107083, #64562 ),
 .UNSPECIFIED., .F., .F.,
 ( 6, 3, 6 ),
 ( 0.000000000000000000, 0.4153918097741242099, 1.000000000000000000 ),
 .UNSPECIFIED. ) ;
#99983=CARTESIAN_POINT ( 'NONE',  ( -13.55937074789999919, 1409.552479676130133, 226.6517356775979977 ) ) ;
#99984=EDGE_LOOP ( 'NONE', ( #74889, #46524, #68762, #3915, #85024 ) ) ;
#99985=CARTESIAN_POINT ( 'NONE',  ( 0.1496009369300290159, 1415.938742849230039, 191.1448484385929873 ) ) ;
#99986=CARTESIAN_POINT ( 'NONE',  ( -0.5979851740210000433, 1408.933942489730043, 231.6757385099979842 ) ) ;
#99989=CARTESIAN_POINT ( 'NONE',  ( 18.09157779502649888, 1416.524489948229984, 209.0416182593249914 ) ) ;
#99992=CARTESIAN_POINT ( 'NONE',  ( -26.35776619319999980, 1444.383684710270018, 225.2710189609979921 ) ) ;
#99995=CARTESIAN_POINT ( 'NONE',  ( -11.87691384789999915, 1433.083180736939994, 150.0777257821980015 ) ) ;
#99999=CARTESIAN_POINT ( 'NONE',  ( 25.37391927814179837, 1441.218297505840155, 209.5413194381530104 ) ) ;
#100000=ADVANCED_FACE ( 'NONE', ( #69010 ), #42601, .F. ) ;
#100001=CARTESIAN_POINT ( 'NONE',  ( -27.50325879720000444, 1440.422393616930094, 137.1890872278979998 ) ) ;
#100002=CARTESIAN_POINT ( 'NONE',  ( -24.17043414239999777, 1438.260851936789777, 211.4235143265279930 ) ) ;
#100006=CARTESIAN_POINT ( 'NONE',  ( -11.47024688358358091, 1509.438411113718075, 236.8433996648743687 ) ) ;
#100007=CARTESIAN_POINT ( 'NONE',  ( -2.240280033315860162E-09, 1413.999988936019918, 247.7072834788440048 ) ) ;
#100010=CARTESIAN_POINT ( 'NONE',  ( -11.76110721155049887, 1426.914523167039988, 145.8371853733709997 ) ) ;
#100012=CARTESIAN_POINT ( 'NONE',  ( -3.565775599929999817, 1474.072336424830155, 270.1349117941979898 ) ) ;
#100016=CARTESIAN_POINT ( 'NONE',  ( 0.2085018806018199833, 1452.672090412190073, 183.2418198939489855 ) ) ;
#100017=CARTESIAN_POINT ( 'NONE',  ( 19.58650745723603137, 1456.033696075030775, 227.9567582387556683 ) ) ;
#100022=CARTESIAN_POINT ( 'NONE',  ( -39.78916335803459958, 1422.796236866350000, 266.8817143848179967 ) ) ;
#100025=B_SPLINE_SURFACE_WITH_KNOTS ( 'NONE', 5, 5, ( 
 ( #64195, #46304, #4806, #80432, #55243, #72061 ),
 ( #72586, #30004, #13191, #55801, #89917, #47379 ),
 ( #22134, #81504, #64758, #62393, #45588, #94855 ),
 ( #34938, #18677, #69691, #97075, #79181, #45036 ),
 ( #53427, #18130, #71359, #105472, #1928, #813 ),
 ( #103811, #28759, #52328, #88678, #11956, #86451 ),
 ( #20340, #19795, #1357, #95413, #104358, #9741 ),
 ( #78049, #35499, #61295, #52873, #60734, #36066 ),
 ( #79729, #2488, #10864, #36605, #54545, #28204 ) ),
 .UNSPECIFIED., .F., .F., .F.,
 ( 6, 3, 6 ),
 ( 6, 6 ),
 ( 1.123296626329999937, 3.227739016200000144, 6.189459079109999706 ),
 ( 0.000000000000000000, 2.000000000000000000 ),
 .UNSPECIFIED. ) ;
#100029=CARTESIAN_POINT ( 'NONE',  ( 38.71370889343818078, 1443.913060387330916, 136.9324510732293732 ) ) ;
#100030=CARTESIAN_POINT ( 'NONE',  ( -2.500000000000000000, 1439.615672362210034, 183.5288080682979910 ) ) ;
#100033=CARTESIAN_POINT ( 'NONE',  ( -2.801317293797483288, 1440.706042130769220, 170.5311005417991623 ) ) ;
#100034=CARTESIAN_POINT ( 'NONE',  ( -14.65731754589999802, 1440.434325343710043, 189.1109637770979930 ) ) ;
#100036=CARTESIAN_POINT ( 'NONE',  ( -11.60004869885203682, 1428.983126981193436, 137.0999999980979851 ) ) ;
#100037=B_SPLINE_SURFACE_WITH_KNOTS ( 'NONE', 5, 5, ( 
 ( #47795, #99828, #107698, #31530, #66278, #29877, #39388, #57324, #6337 ),
 ( #5800, #30982, #82498, #39941, #73565, #74111, #108241, #81371, #100394 ),
 ( #64066, #15266, #91990, #33727, #49458, #67920, #41034, #101469, #102028 ),
 ( #66819, #75211, #25866, #33179, #41600, #67370, #166, #84136, #15798 ),
 ( #43257, #92530, #76856, #708, #50556, #42700, #34288, #109364, #6878 ),
 ( #51654, #25312, #58954, #59511, #24219, #103130, #75754, #26430, #24756 ),
 ( #102572, #9091, #83580, #7435, #60069, #32642, #100920, #109900, #58405 ),
 ( #50001, #93085, #16358, #76297, #68469, #94186, #85231, #84683, #7981 ),
 ( #16901, #17455, #42147, #110448, #93622, #85794, #51106, #8523, #77404 ),
 ( #34838, #69027, #2383, #18025, #36501, #9629, #70144, #70697, #19120 ),
 ( #43799, #105364, #1823, #10192, #35958, #79626, #52763, #95308, #103702 ),
 ( #37603, #2930, #87469, #53323, #86899, #77950, #62284, #44366, #27001 ),
 ( #104808, #27549, #28096, #61191, #71805, #78512, #105924, #104258, #18568 ),
 ( #88569, #94746, #61731, #28655, #60625, #52218, #95854, #69584, #96414 ),
 ( #10761, #1256, #44931, #45483, #62859, #53895, #79078, #19691, #88030 ) ),
 .UNSPECIFIED., .F., .F., .F.,
 ( 6, 3, 3, 3, 6 ),
 ( 6, 3, 6 ),
 ( 3.076410786119999852, 5.721725431660000361, 7.579817615749999682, 10.83727443650000133, 12.56788425660000108 ),
 ( 0.000000000000000000, 1.000000000000000000, 2.000000000000000000 ),
 .UNSPECIFIED. ) ;
#100038=ORIENTED_EDGE ( 'NONE', *, *, #77429, .F. ) ;
#100039=CARTESIAN_POINT ( 'NONE',  ( -26.02813552489999793, 1435.406381042510020, 135.3446223067979872 ) ) ;
#100040=EDGE_CURVE ( 'NONE', #78889, #59125, #98350, .T. ) ;
#100041=EDGE_CURVE ( 'NONE', #69919, #104433, #92514, .T. ) ;
#100044=B_SPLINE_SURFACE_WITH_KNOTS ( 'NONE', 4, 5, ( 
 ( #60855, #44032, #16040, #75970, #43485, #94980 ),
 ( #51885, #84903, #50241, #42362, #68693, #26094 ),
 ( #84368, #59733, #8195, #69809, #76516, #101697 ),
 ( #110667, #93852, #17123, #86021, #8747, #77088 ),
 ( #18248, #52444, #94403, #60284, #34515, #102797 ) ),
 .UNSPECIFIED., .F., .F., .F.,
 ( 5, 5 ),
 ( 6, 6 ),
 ( 6.591324572230000456, 20.28790020619999979 ),
 ( 0.000000000000000000, 2.000000000000000000 ),
 .UNSPECIFIED. ) ;
#100047=CARTESIAN_POINT ( 'NONE',  ( -38.22512636920640006, 1426.932643485439939, 269.5724048218409621 ) ) ;
#100049=CARTESIAN_POINT ( 'NONE',  ( -3.502932684640000183, 1396.096286483429822, 197.9227087040979995 ) ) ;
#100051=CARTESIAN_POINT ( 'NONE',  ( 15.95383384960000228, 1506.798305107329952, 193.5571554442980187 ) ) ;
#100052=ORIENTED_EDGE ( 'NONE', *, *, #11972, .F. ) ;
#100053=ORIENTED_EDGE ( 'NONE', *, *, #31533, .F. ) ;
#100054=CARTESIAN_POINT ( 'NONE',  ( 0.3740406684259999781, 1452.976565745030030, 183.2744760548980025 ) ) ;
#100056=ADVANCED_FACE ( 'NONE', ( #51091 ), #91340, .F. ) ;
#100058=CARTESIAN_POINT ( 'NONE',  ( -14.48051094013809958, 1436.252343529019981, 149.9435809378360318 ) ) ;
#100059=CARTESIAN_POINT ( 'NONE',  ( -0.03672266410218510274, 1409.548389820189868, 185.2684399885600044 ) ) ;
#100064=CARTESIAN_POINT ( 'NONE',  ( 5.426920751279999955, 1436.492768174659886, 154.6973185947979914 ) ) ;
#100066=CARTESIAN_POINT ( 'NONE',  ( 4.164920226616133370, 1440.953747641006203, 156.0413096252420644 ) ) ;
#100067=CARTESIAN_POINT ( 'NONE',  ( 11.79002767249999906, 1447.121451531979801, 187.8029512936980154 ) ) ;
#100075=ORIENTED_EDGE ( 'NONE', *, *, #41271, .T. ) ;
#100078=CARTESIAN_POINT ( 'NONE',  ( 13.15726448919999925, 1414.996444518330009, 197.7616626325980178 ) ) ;
#100080=CARTESIAN_POINT ( 'NONE',  ( -3.549608351769999892, 1507.276797637930031, 180.9704965309979912 ) ) ;
#100081=DIRECTION ( 'NONE',  ( 0.7382608262429739554, 0.6622882068469760908, -0.1278486742459950254 ) ) ;
#100082=CARTESIAN_POINT ( 'NONE',  ( 2.838432861149654318, 1451.798331723987985, 183.8400387955967403 ) ) ;
#100084=EDGE_CURVE ( 'NONE', #67251, #103179, #35688, .T. ) ;
#100086=CARTESIAN_POINT ( 'NONE',  ( 4.282037523864819839, 1440.980613445030031, 156.2001673258700123 ) ) ;
#100087=AXIS2_PLACEMENT_3D ( 'NONE', #15283, #50574, #8548 ) ;
#100088=CARTESIAN_POINT ( 'NONE',  ( -11.96661585360000046, 1440.449248668989867, 150.8629738177980073 ) ) ;
#100091=VERTEX_POINT ( 'NONE', #68324 ) ;
#100097=CARTESIAN_POINT ( 'NONE',  ( -8.902413453548941646, 1424.022967874639789, 122.9079028789289936 ) ) ;
#100100=CARTESIAN_POINT ( 'NONE',  ( 11.44617005173907209, 1425.796920914145858, 139.1405512805114597 ) ) ;
#100102=CARTESIAN_POINT ( 'NONE',  ( -1.743193279576590093, 1464.853942634930036, 183.6101355626199734 ) ) ;
#100104=CARTESIAN_POINT ( 'NONE',  ( -2.379883222516000230E-07, 1408.913060379049739, 223.8563942630169947 ) ) ;
#100105=CARTESIAN_POINT ( 'NONE',  ( 33.18315033877439646, 1440.913060383530137, 247.0235257256299803 ) ) ;
#100107=CARTESIAN_POINT ( 'NONE',  ( -15.75336812958823884, 1414.913060387329779, 213.0330643493421121 ) ) ;
#100108=CARTESIAN_POINT ( 'NONE',  ( 12.97616279770000070, 1422.953780371429957, 222.3281805362979924 ) ) ;
#100112=CARTESIAN_POINT ( 'NONE',  ( -19.67371442948930849, 1485.252007959948060, 190.3247210294366596 ) ) ;
#100113=CARTESIAN_POINT ( 'NONE',  ( -27.68516856759999811, 1508.595246549830108, 210.6013668364779789 ) ) ;
#100117=CARTESIAN_POINT ( 'NONE',  ( -3.500000000000000000, 1421.663060387330006, 172.2701767054979882 ) ) ;
#100120=CARTESIAN_POINT ( 'NONE',  ( -15.44132444299999918, 1507.624369720630057, 192.1037569956980064 ) ) ;
#100121=EDGE_CURVE ( 'NONE', #36366, #24304, #47586, .T. ) ;
#100131=ORIENTED_EDGE ( 'NONE', *, *, #70945, .T. ) ;
#100138=EDGE_CURVE ( 'NONE', #78944, #110307, #54356, .T. ) ;
#100141=CARTESIAN_POINT ( 'NONE',  ( 5.217757123237790395, 1409.095268481059975, 195.0806377026630116 ) ) ;
#100142=CARTESIAN_POINT ( 'NONE',  ( 18.12190093680000302, 1425.048267533830085, 225.2390196191980181 ) ) ;
#100143=CARTESIAN_POINT ( 'NONE',  ( 4.071927273580000062, 1420.049653579930009, 185.6171871639980111 ) ) ;
#100145=CARTESIAN_POINT ( 'NONE',  ( -4.228686410976469467, 1441.557731059559956, 165.0907915641419947 ) ) ;
#100147=DIRECTION ( 'NONE',  ( -0.03489949627507600571, 0.9993908270340192690, 7.149496293836860302E-08 ) ) ;
#100149=CARTESIAN_POINT ( 'NONE',  ( 14.38276615817169635, 1509.537722092532931, 235.4493228184925897 ) ) ;
#100150=CARTESIAN_POINT ( 'NONE',  ( 17.94043310207709752, 1458.161672853299933, 228.3106580608940135 ) ) ;
#100151=CARTESIAN_POINT ( 'NONE',  ( -12.16672036689999814, 1434.609987438209828, 150.8335117639980183 ) ) ;
#100152=EDGE_CURVE ( 'NONE', #68424, #104636, #8896, .T. ) ;
#100153=CARTESIAN_POINT ( 'NONE',  ( -7.271832385515029613E-10, 1467.401133680060184, 246.3384324245209882 ) ) ;
#100154=CARTESIAN_POINT ( 'NONE',  ( -20.49879694356830129, 1504.586794500839915, 190.4844630885789911 ) ) ;
#100162=CARTESIAN_POINT ( 'NONE',  ( -20.26037020649999576, 1488.374911902629947, 192.5828114397980073 ) ) ;
#100165=CARTESIAN_POINT ( 'NONE',  ( 6.448255092998069316, 1408.606950371990024, 221.0175999112360046 ) ) ;
#100170=EDGE_LOOP ( 'NONE', ( #34004, #40530, #28293 ) ) ;
#100171=CARTESIAN_POINT ( 'NONE',  ( 25.63688228349999676, 1437.526525769599857, 221.5010247020979932 ) ) ;
#100172=CARTESIAN_POINT ( 'NONE',  ( -27.00673398009999815, 1508.127684928829922, 203.3798472705879874 ) ) ;
#100173=CARTESIAN_POINT ( 'NONE',  ( 1.478882416969999891, 1478.166263375429935, 182.3756109040980107 ) ) ;
#100174=CARTESIAN_POINT ( 'NONE',  ( 22.52609212299890018, 1509.699688857919909, 227.3081665486540146 ) ) ;
#100177=CARTESIAN_POINT ( 'NONE',  ( -12.00843801870000149, 1421.605076870430139, 225.2224014919979993 ) ) ;
#100180=CARTESIAN_POINT ( 'NONE',  ( -9.354210145178099012, 1452.586404171080176, 150.8537525510609782 ) ) ;
#100181=CARTESIAN_POINT ( 'NONE',  ( 29.26107752939999784, 1451.736821630529903, 135.7240151124980230 ) ) ;
#100182=ORIENTED_EDGE ( 'NONE', *, *, #19926, .T. ) ;
#100183=CARTESIAN_POINT ( 'NONE',  ( -5.361476397494260304, 1423.659291631490078, 149.6373755565670081 ) ) ;
#100185=CARTESIAN_POINT ( 'NONE',  ( 16.53448445007540357, 1423.354062263319975, 228.9298141595320146 ) ) ;
#100186=CARTESIAN_POINT ( 'NONE',  ( 17.17007368304201975, 1414.941152333512946, 210.4884745552690504 ) ) ;
#100190=CARTESIAN_POINT ( 'NONE',  ( -23.24847510427670016, 1409.840678955939893, 209.5428208297719834 ) ) ;
#100191=ADVANCED_FACE ( 'NONE', ( #5502 ), #109560, .T. ) ;
#100196=CARTESIAN_POINT ( 'NONE',  ( -23.81755502456005047, 1436.557569478829009, 140.3494998115120325 ) ) ;
#100197=CARTESIAN_POINT ( 'NONE',  ( -19.24674285640000093, 1410.873837133030065, 222.4867807485979938 ) ) ;
#100198=CARTESIAN_POINT ( 'NONE',  ( 44.66341284919820254, 1448.409646889560008, 266.2171260073000099 ) ) ;
#100200=CARTESIAN_POINT ( 'NONE',  ( 0.02539148181239999844, 1420.205191554729936, 183.8956754969979954 ) ) ;
#100206=CARTESIAN_POINT ( 'NONE',  ( 12.76981295728383081, 1442.833559347544679, 186.8056601929062595 ) ) ;
#100207=ORIENTED_EDGE ( 'NONE', *, *, #15978, .T. ) ;
#100213=CARTESIAN_POINT ( 'NONE',  ( 5.716743777814420113, 1452.713427295639804, 151.9346595207390180 ) ) ;
#100217=CARTESIAN_POINT ( 'NONE',  ( 16.19086104229999989, 1409.478457713630178, 193.2334207647979838 ) ) ;
#100220=CARTESIAN_POINT ( 'NONE',  ( 2.127093723893670241, 1408.987340136950024, 186.9630477151469847 ) ) ;
#100221=CARTESIAN_POINT ( 'NONE',  ( -12.95358049610739926, 1434.757105051030067, 149.1854028063150110 ) ) ;
#100222=CARTESIAN_POINT ( 'NONE',  ( -18.27190865341688308, 1423.986030104572819, 225.3810334195744076 ) ) ;
#100226=LINE ( 'NONE', #23506, #32053 ) ;
#100228=CARTESIAN_POINT ( 'NONE',  ( 8.800012970690000103, 1429.116251061429921, 209.1218459616979999 ) ) ;
#100235=CARTESIAN_POINT ( 'NONE',  ( 13.23453334633730094, 1423.606062042400026, 221.8416081335510057 ) ) ;
#100237=CARTESIAN_POINT ( 'NONE',  ( -13.79555465660000024, 1416.822694272029821, 221.9085256446979884 ) ) ;
#100239=CARTESIAN_POINT ( 'NONE',  ( 6.438546668759999925, 1470.874276671130019, 268.3665355201979992 ) ) ;
#100240=B_SPLINE_CURVE_WITH_KNOTS ( 'NONE', 5,
 ( #80137, #54419, #2367, #45466, #21298, #88014 ),
 .UNSPECIFIED., .F., .F.,
 ( 6, 6 ),
 ( -21.89489252110000095, -4.528383794635178816 ),
 .UNSPECIFIED. ) ;
#100242=VECTOR ( 'NONE', #101194, 1000.000000000000114 ) ;
#100246=CARTESIAN_POINT ( 'NONE',  ( -17.66088505599999792, 1486.101186812730020, 188.1926570484980346 ) ) ;
#100249=CARTESIAN_POINT ( 'NONE',  ( -16.93199317389999692, 1409.669516225829966, 225.4753726314980042 ) ) ;
#100250=CARTESIAN_POINT ( 'NONE',  ( -1.121059198139999991, 1418.672904462529914, 228.1661418348980135 ) ) ;
#100256=CARTESIAN_POINT ( 'NONE',  ( -12.51099981729999833, 1416.825784011830137, 222.1450729858979969 ) ) ;
#100257=CARTESIAN_POINT ( 'NONE',  ( 0.1746847925749699937, 1477.583909127160041, 182.1981708306240080 ) ) ;
#100258=CARTESIAN_POINT ( 'NONE',  ( 0.05087725381669139929, 1408.368774909579997, 222.6640242875809861 ) ) ;
#100260=CARTESIAN_POINT ( 'NONE',  ( -28.06188869160000010, 1444.994950788469851, 168.7697867250980153 ) ) ;
#100263=CARTESIAN_POINT ( 'NONE',  ( -28.39832174097189821, 1509.566674240429847, 211.0445668619889830 ) ) ;
#100264=CARTESIAN_POINT ( 'NONE',  ( 11.87515583119999896, 1433.007142645810063, 149.4775923092979895 ) ) ;
#100265=CARTESIAN_POINT ( 'NONE',  ( -41.66188030070000536, 1443.705283505669740, 134.0999999982089719 ) ) ;
#100266=DIRECTION ( 'NONE',  ( -0.3363363969981477131, -0.6659120918162938496, 0.6659120918162938496 ) ) ;
#100272=CARTESIAN_POINT ( 'NONE',  ( 19.21579935105259906, 1443.315311240889969, 208.7528447609300031 ) ) ;
#100273=CARTESIAN_POINT ( 'NONE',  ( 29.17712929358009077, 1414.632439072223178, 269.3720782604887631 ) ) ;
#100281=CARTESIAN_POINT ( 'NONE',  ( -29.54414221549020070, 1509.931130578880129, 208.5939597344579965 ) ) ;
#100282=CARTESIAN_POINT ( 'NONE',  ( -16.03779784396279950, 1410.573261502639753, 226.6730129231060289 ) ) ;
#100286=CARTESIAN_POINT ( 'NONE',  ( 40.27306231122417302, 1443.623772255950371, 137.1176861334613477 ) ) ;
#100289=CARTESIAN_POINT ( 'NONE',  ( -0.07605448290418309609, 1420.080655933570142, 183.8600900220690164 ) ) ;
#100290=CARTESIAN_POINT ( 'NONE',  ( 22.10980528540000023, 1409.685151801829761, 213.0533367086480041 ) ) ;
#100292=CARTESIAN_POINT ( 'NONE',  ( -17.50943625649999902, 1423.244172935829965, 226.4867715792979936 ) ) ;
#100296=CARTESIAN_POINT ( 'NONE',  ( 15.28420222189999933, 1497.713060387329961, 225.7900586086979899 ) ) ;
#100299=CARTESIAN_POINT ( 'NONE',  ( -12.78907454407420019, 1485.543771368729949, 185.6852311013239785 ) ) ;
#100305=ORIENTED_EDGE ( 'NONE', *, *, #33706, .F. ) ;
#100307=ORIENTED_EDGE ( 'NONE', *, *, #78685, .F. ) ;
#100309=CARTESIAN_POINT ( 'NONE',  ( -22.95381948389999849, 1410.909818712429797, 204.6459351782779947 ) ) ;
#100310=CARTESIAN_POINT ( 'NONE',  ( -9.064548087047670677, 1441.200071124479791, 153.7187301749719950 ) ) ;
#100311=CARTESIAN_POINT ( 'NONE',  ( 15.92282521243189919, 1409.477284117250065, 192.7841990163499872 ) ) ;
#100313=CARTESIAN_POINT ( 'NONE',  ( 40.71426153566390127, 1443.112331678010150, 137.0418675333559975 ) ) ;
#100316=CARTESIAN_POINT ( 'NONE',  ( 5.852294824033087650, 1466.142654960249729, 233.6444853126671148 ) ) ;
#100318=CARTESIAN_POINT ( 'NONE',  ( 37.10988369666650044, 1450.944967383590210, 134.0999999986949831 ) ) ;
#100320=CARTESIAN_POINT ( 'NONE',  ( -24.02854066789229748, 1507.902906607559999, 222.3115874531950169 ) ) ;
#100325=ORIENTED_EDGE ( 'NONE', *, *, #64461, .F. ) ;
#100329=CARTESIAN_POINT ( 'NONE',  ( 0.1468926284139999983, 1452.343333621129887, 183.2733069738979736 ) ) ;
#100330=CARTESIAN_POINT ( 'NONE',  ( -3.071983047080000251, 1484.702655605429982, 183.3182174088979934 ) ) ;
#100339=VERTEX_POINT ( 'NONE', #102704 ) ;
#100342=ORIENTED_EDGE ( 'NONE', *, *, #34408, .T. ) ;
#100343=CARTESIAN_POINT ( 'NONE',  ( 37.01368886828679905, 1440.913060387330006, 263.6769638602469854 ) ) ;
#100345=CARTESIAN_POINT ( 'NONE',  ( -0.0007967155919044118005, 1451.919253836483904, 154.0005622324263470 ) ) ;
#100347=CARTESIAN_POINT ( 'NONE',  ( -13.57591587749999995, 1415.063410501429871, 220.4959916660980070 ) ) ;
#100348=CARTESIAN_POINT ( 'NONE',  ( -11.85318840119790096, 1432.336023631749867, 150.2214164863760004 ) ) ;
#100350=CARTESIAN_POINT ( 'NONE',  ( 17.38482601099109814, 1410.884446382940041, 192.4603632472940262 ) ) ;
#100351=CARTESIAN_POINT ( 'NONE',  ( 21.58361403490490105, 1409.738374864039997, 206.3476434096999981 ) ) ;
#100354=CARTESIAN_POINT ( 'NONE',  ( -11.87936887709999922, 1433.311451768779989, 148.5636887028979913 ) ) ;
#100355=CARTESIAN_POINT ( 'NONE',  ( 26.30822731440100171, 1495.554174878970116, 206.2282085093290220 ) ) ;
#100356=CARTESIAN_POINT ( 'NONE',  ( 17.41280886879999912, 1458.364526861729928, 230.6041451782980118 ) ) ;
#100357=CARTESIAN_POINT ( 'NONE',  ( -1.674817372199999932, 1416.913060387330006, 226.0542104739980118 ) ) ;
#100358=CARTESIAN_POINT ( 'NONE',  ( 4.613723315850000479E-06, 1474.175172091230024, 270.1377426632980132 ) ) ;
#100364=CARTESIAN_POINT ( 'NONE',  ( -0.1584504759644470018, 1507.222331208859941, 180.8948199759900035 ) ) ;
#100367=CARTESIAN_POINT ( 'NONE',  ( 18.56679396470000043, 1509.561427119029759, 187.1464481793979928 ) ) ;
#100369=CARTESIAN_POINT ( 'NONE',  ( -10.85852386199281661, 1424.794007418467800, 138.1924915073045099 ) ) ;
#100372=CARTESIAN_POINT ( 'NONE',  ( -10.10004869885203682, -0.000000000000000000, 137.0999999980979851 ) ) ;
#100374=CARTESIAN_POINT ( 'NONE',  ( -11.57324738139999987, 1432.089115936239978, 151.1932558213979974 ) ) ;
#100377=CARTESIAN_POINT ( 'NONE',  ( 27.02695150585199357, 1451.203551446300708, 136.2753212570038102 ) ) ;
#100380=CARTESIAN_POINT ( 'NONE',  ( -24.01773571409999875, 1482.721384371930071, 219.5181103496979915 ) ) ;
#100382=DIRECTION ( 'NONE',  ( 0.7074300732877097930, -0.02470400237317429276, 0.7063514731880239372 ) ) ;
#100385=CARTESIAN_POINT ( 'NONE',  ( 6.194088323349999925, 1406.153407140329819, 267.2191889491979850 ) ) ;
#100386=CARTESIAN_POINT ( 'NONE',  ( 38.60856580501570079, 1443.613625263020140, 137.1750438873210101 ) ) ;
#100388=CARTESIAN_POINT ( 'NONE',  ( 23.82579336797228819, 1434.875857586895791, 214.2505971287225748 ) ) ;
#100390=DIRECTION ( 'NONE',  ( 0.000000000000000000, 1.000000000000000000, 0.000000000000000000 ) ) ;
#100394=CARTESIAN_POINT ( 'NONE',  ( -12.51069050239999925, 1447.046592316670058, 187.7237828829979946 ) ) ;
#100395=CARTESIAN_POINT ( 'NONE',  ( -19.75952018396922227, 1485.979955017908424, 190.2281124034579136 ) ) ;
#100398=CARTESIAN_POINT ( 'NONE',  ( -17.24149055319999846, 1434.891998881070094, 209.1218459616979999 ) ) ;
#100400=CARTESIAN_POINT ( 'NONE',  ( 2.500000001330000110, 1439.558446910639987, 156.0470066727980054 ) ) ;
#100402=CARTESIAN_POINT ( 'NONE',  ( -6.205390840879999814, 1475.766608774730003, 267.5209476633980330 ) ) ;
#100403=FACE_OUTER_BOUND ( 'NONE', #19662, .T. ) ;
#100405=CARTESIAN_POINT ( 'NONE',  ( -11.92971211075766291, 1486.509503358195616, 184.3501215366537167 ) ) ;
#100408=DIRECTION ( 'NONE',  ( 0.000000000000000000, 0.000000000000000000, -1.000000000000000000 ) ) ;
#100409=CARTESIAN_POINT ( 'NONE',  ( -24.42951531446290048, 1444.777949477279890, 211.0705837658230166 ) ) ;
#100412=CARTESIAN_POINT ( 'NONE',  ( -22.01686062879999994, 1410.177021064929932, 202.7226449493980169 ) ) ;
#100413=( BOUNDED_CURVE ( )  B_SPLINE_CURVE ( 3, ( #97607, #20877, #46675, #74478 ),
 .UNSPECIFIED., .F., .F. ) 
 B_SPLINE_CURVE_WITH_KNOTS ( ( 4, 4 ),
 ( 4.409610696067515434, 5.070003797870570317 ),
 .UNSPECIFIED. ) 
 CURVE ( )  GEOMETRIC_REPRESENTATION_ITEM ( )  RATIONAL_B_SPLINE_CURVE ( ( 1.000000000000000000, 0.9639857562037046357, 0.9639857562037046357, 1.000000000000000000 ) ) 
 REPRESENTATION_ITEM ( '' )  );
#100419=CARTESIAN_POINT ( 'NONE',  ( -10.30418465418137153, 1410.643618912880129, 229.4321436142978996 ) ) ;
#100422=CARTESIAN_POINT ( 'NONE',  ( 11.14405623819999924, 1425.166915822629790, 143.4624449666980297 ) ) ;
#100423=CARTESIAN_POINT ( 'NONE',  ( 13.89659397336691171, 1452.767297056081361, 223.5433327310063873 ) ) ;
#100428=CARTESIAN_POINT ( 'NONE',  ( 11.86606288651399588, 1432.348820292879054, 150.6996693143473465 ) ) ;
#100429=CARTESIAN_POINT ( 'NONE',  ( -4.823778297959999684, 1426.859560269130043, 144.1938086916980239 ) ) ;
#100432=CARTESIAN_POINT ( 'NONE',  ( 7.628773448410000491, 1416.913060387330006, 216.7506196533479965 ) ) ;
#100434=CARTESIAN_POINT ( 'NONE',  ( 22.51756696979500205, 1509.699391153020088, 227.9212068633959802 ) ) ;
#100436=ORIENTED_EDGE ( 'NONE', *, *, #90427, .F. ) ;
#100437=VERTEX_POINT ( 'NONE', #109080 ) ;
#100438=CARTESIAN_POINT ( 'NONE',  ( 11.41627450834240065, 1434.253991202039970, 151.4464532660140037 ) ) ;
#100439=CARTESIAN_POINT ( 'NONE',  ( -5.420556941769999248, 1397.452469479530009, 221.3623452826979872 ) ) ;
#100440=CARTESIAN_POINT ( 'NONE',  ( -19.73686209359999921, 1410.963192513930153, 221.4818400716980307 ) ) ;
#100442=CARTESIAN_POINT ( 'NONE',  ( -13.14780857342640807, 1444.759452443107193, 169.3987409578616052 ) ) ;
#100443=CARTESIAN_POINT ( 'NONE',  ( 22.00282045326062175, 1509.704813241454076, 228.9760804587602649 ) ) ;
#100446=CARTESIAN_POINT ( 'NONE',  ( -13.71395690008879953, 1507.898280399110035, 184.2319266679010070 ) ) ;
#100447=CARTESIAN_POINT ( 'NONE',  ( 2.108249574319999819, 1468.706075860329975, 182.9191506125980027 ) ) ;
#100448=CARTESIAN_POINT ( 'NONE',  ( -9.839465017559998472, 1415.426091369230107, 193.9823038429979931 ) ) ;
#100450=CARTESIAN_POINT ( 'NONE',  ( 10.91120509363300073, 1396.294088065360029, 210.9837282830089862 ) ) ;
#100451=CARTESIAN_POINT ( 'NONE',  ( 1.393184507720000020, 1415.579607678529783, 190.6507824856979880 ) ) ;
#100452=CARTESIAN_POINT ( 'NONE',  ( 11.83689489290000019, 1430.337612590129993, 149.6288192558980086 ) ) ;
#100453=CARTESIAN_POINT ( 'NONE',  ( 5.639308305133535093, 1426.925666188799596, 144.1938086916980524 ) ) ;
#100454=ORIENTED_EDGE ( 'NONE', *, *, #48064, .F. ) ;
#100455=CARTESIAN_POINT ( 'NONE',  ( 13.24048663314659890, 1434.881627497140016, 149.0998486302219987 ) ) ;
#100458=CARTESIAN_POINT ( 'NONE',  ( 13.45896606823204600, 1444.273004732949403, 169.3617971741905421 ) ) ;
#100459=CARTESIAN_POINT ( 'NONE',  ( -8.404281262359999616, 1463.438804155129901, 234.4303259422979977 ) ) ;
#100460=CARTESIAN_POINT ( 'NONE',  ( -13.36764582699999870, 1434.818091166239810, 195.6891582639979958 ) ) ;
#100463=( GEOMETRIC_REPRESENTATION_CONTEXT ( 3 ) GLOBAL_UNCERTAINTY_ASSIGNED_CONTEXT ( ( #43514 ) ) GLOBAL_UNIT_ASSIGNED_CONTEXT ( ( #45546, #4082, #38207 ) ) REPRESENTATION_CONTEXT ( 'NONE', 'WORKASPACE' ) );
#100473=CARTESIAN_POINT ( 'NONE',  ( -20.99960920810000076, 1509.542875960729816, 229.5003925517980008 ) ) ;
#100475=CARTESIAN_POINT ( 'NONE',  ( -17.16049493890136546, 1413.067501001438586, 269.3744597087676311 ) ) ;
#100477=CARTESIAN_POINT ( 'NONE',  ( -0.2241001114496510016, 1414.913060387399810, 225.2212286822969816 ) ) ;
#100479=CARTESIAN_POINT ( 'NONE',  ( 2.500000000000000000, 1422.854123512330034, 153.3880924786980131 ) ) ;
#100480=CARTESIAN_POINT ( 'NONE',  ( -27.68018901532030185, 1440.913060394170088, 229.8355793643949880 ) ) ;
#100482=CARTESIAN_POINT ( 'NONE',  ( -0.1457467676193440198, 1465.435012609549858, 236.3215832813700104 ) ) ;
#100484=CARTESIAN_POINT ( 'NONE',  ( 10.92641736269999875, 1408.882512851029787, 270.2707055153979923 ) ) ;
#100486=CARTESIAN_POINT ( 'NONE',  ( 22.71325450959999870, 1409.706218420429877, 209.2588089802279967 ) ) ;
#100493=CARTESIAN_POINT ( 'NONE',  ( -11.66377130828579389, 1486.022747640305397, 184.5416405436658351 ) ) ;
#100495=VERTEX_POINT ( 'NONE', #11446 ) ;
#100498=DIRECTION ( 'NONE',  ( 0.000000000000000000, -1.036208156316811829E-12, 1.000000000000000000 ) ) ;
#100500=B_SPLINE_CURVE_WITH_KNOTS ( 'NONE', 3,
 ( #687, #34817, #69004, #103108, #26409, #32623, #100898, #24195, #58382, #15775, #27521, #52741 ),
 .UNSPECIFIED., .F., .F.,
 ( 4, 2, 2, 2, 2, 4 ),
 ( -0.1123552058535770004, -0.09789079797561310581, -0.08345975750668109538, -0.05408602645508549939, -0.02844277172862970382, 0.000000000000000000 ),
 .UNSPECIFIED. ) ;
#100503=CARTESIAN_POINT ( 'NONE',  ( -23.51884061340000187, 1448.078341978100070, 217.4024159431679664 ) ) ;
#100513=CARTESIAN_POINT ( 'NONE',  ( 15.14035858829999981, 1484.828642735030144, 223.7275130474980074 ) ) ;
#100514=CARTESIAN_POINT ( 'NONE',  ( 22.91083410329999737, 1450.813759947410063, 218.3463015468979904 ) ) ;
#100518=CARTESIAN_POINT ( 'NONE',  ( 15.20205009985922828, 1420.720005487666640, 227.8617693338353547 ) ) ;
#100520=CARTESIAN_POINT ( 'NONE',  ( -21.29751270369999716, 1429.161938467929986, 221.7940764617979994 ) ) ;
#100523=CARTESIAN_POINT ( 'NONE',  ( -15.75701339500000131, 1413.316754371529896, 226.8028676289979728 ) ) ;
#100525=CARTESIAN_POINT ( 'NONE',  ( -14.55555340835505618, 1469.534367028784800, 269.3628596919716642 ) ) ;
#100527=FACE_OUTER_BOUND ( 'NONE', #84910, .T. ) ;
#100528=CARTESIAN_POINT ( 'NONE',  ( -42.22973048505161131, 1427.945894564693617, 269.0695617814723164 ) ) ;
#100531=CARTESIAN_POINT ( 'NONE',  ( -14.77861346903486073, 1452.029250706874791, 222.9956542297432804 ) ) ;
#100532=CARTESIAN_POINT ( 'NONE',  ( -13.45936570671707422, 1444.272002885449183, 187.0016728524507528 ) ) ;
#100535=CARTESIAN_POINT ( 'NONE',  ( -2.293473560577727444, 1415.644794225288933, 232.9564924084930908 ) ) ;
#100538=CARTESIAN_POINT ( 'NONE',  ( -13.14373765855973453, 1443.062906526838788, 169.3993406322344981 ) ) ;
#100539=CARTESIAN_POINT ( 'NONE',  ( -13.04207716350000013, 1409.368499757629934, 225.9431851714979871 ) ) ;
#100540=ORIENTED_EDGE ( 'NONE', *, *, #18889, .T. ) ;
#100542=CARTESIAN_POINT ( 'NONE',  ( 0.2679975439089999911, 1416.543503932829935, 190.7826617148979835 ) ) ;
#100545=EDGE_LOOP ( 'NONE', ( #69254, #1873, #36050 ) ) ;
#100546=CARTESIAN_POINT ( 'NONE',  ( 17.50151672410429882, 1415.426561690370136, 209.0279233183210010 ) ) ;
#100549=CARTESIAN_POINT ( 'NONE',  ( -4.105765241160000301, 1462.105318180830182, 225.2361590896979919 ) ) ;
#100551=CARTESIAN_POINT ( 'NONE',  ( -11.26041480129999961, 1433.222928179650125, 151.5319910271979893 ) ) ;
#100552=CARTESIAN_POINT ( 'NONE',  ( -12.53380652166779896, 1445.052232296300190, 185.6742736269380032 ) ) ;
#100553=DIRECTION ( 'NONE',  ( -0.5220042966316842392, -0.8520752641501264657, -0.03846113000878779997 ) ) ;
#100555=CARTESIAN_POINT ( 'NONE',  ( -24.89152731869999968, 1440.652444856679949, 210.4229212863880036 ) ) ;
#100557=CARTESIAN_POINT ( 'NONE',  ( 2.409539184149999791, 1449.743190781309977, 182.7459288299980074 ) ) ;
#100562=ORIENTED_EDGE ( 'NONE', *, *, #13050, .T. ) ;
#100563=CARTESIAN_POINT ( 'NONE',  ( -11.80736846912400040, 1428.600782186070091, 148.5414466374529923 ) ) ;
#100565=CARTESIAN_POINT ( 'NONE',  ( -8.021038987360000760, 1471.498700897329854, 270.0743385271980515 ) ) ;
#100568=CARTESIAN_POINT ( 'NONE',  ( 41.36928039706089777, 1446.256855822869966, 135.7759721705720040 ) ) ;
#100570=CARTESIAN_POINT ( 'NONE',  ( 19.68696007051993035, 1455.842560867163456, 227.5801044884133262 ) ) ;
#100571=CARTESIAN_POINT ( 'NONE',  ( -25.62242681216090290, 1435.677401875209853, 212.3103032994399939 ) ) ;
#100574=CARTESIAN_POINT ( 'NONE',  ( -28.90439777006010047, 1413.811818966640203, 266.6319722207740028 ) ) ;
#100575=VERTEX_POINT ( 'NONE', #29878 ) ;
#100577=ORIENTED_EDGE ( 'NONE', *, *, #93521, .F. ) ;
#100578=ORIENTED_EDGE ( 'NONE', *, *, #97339, .F. ) ;
#100580=CARTESIAN_POINT ( 'NONE',  ( 4.828144534977668378, 1423.511443209914432, 184.1101743659536965 ) ) ;
#100584=CARTESIAN_POINT ( 'NONE',  ( -16.74965842090000123, 1425.425121304829872, 191.0834941450980011 ) ) ;
#100588=CARTESIAN_POINT ( 'NONE',  ( -26.79413269730000025, 1436.761936273179799, 136.7822071774980088 ) ) ;
#100590=EDGE_CURVE ( 'NONE', #86024, #78014, #46225, .T. ) ;
#100591=CARTESIAN_POINT ( 'NONE',  ( 0.000000000000000000, 1518.913060387330006, 209.1218459616979999 ) ) ;
#100593=CARTESIAN_POINT ( 'NONE',  ( -43.27233402150790198, 1430.332577981739860, 269.9334234287720165 ) ) ;
#100595=CARTESIAN_POINT ( 'NONE',  ( -6.232532172530000025, 1398.098440467730143, 197.7132727550980178 ) ) ;
#100598=ORIENTED_EDGE ( 'NONE', *, *, #56235, .T. ) ;
#100599=CARTESIAN_POINT ( 'NONE',  ( 0.1984549593710000226, 1451.686688173929952, 183.0460368089979966 ) ) ;
#100602=CARTESIAN_POINT ( 'NONE',  ( -25.08556694820000033, 1436.445275169010074, 137.7014522548979869 ) ) ;
#100603=CARTESIAN_POINT ( 'NONE',  ( 22.59589169820000265, 1507.700907224229923, 227.3081670307980175 ) ) ;
#100606=CARTESIAN_POINT ( 'NONE',  ( -1.811215688146619929, 1484.240532944710139, 182.8268356034129738 ) ) ;
#100610=CARTESIAN_POINT ( 'NONE',  ( -2.691724795918589486, 1451.958513340359787, 184.7155965712029797 ) ) ;
#100612=CARTESIAN_POINT ( 'NONE',  ( -19.90154680646875818, 1456.621465229937257, 225.3649839440089409 ) ) ;
#100613=EDGE_LOOP ( 'NONE', ( #92598, #34256, #86296, #39755, #23067, #8467 ) ) ;
#100615=CARTESIAN_POINT ( 'NONE',  ( -22.17127944006911378, 1509.715749581838509, 228.8537622112010581 ) ) ;
#100616=CARTESIAN_POINT ( 'NONE',  ( -4.071992749581919036, 1441.017388854438877, 184.8896994088449901 ) ) ;
#100617=CARTESIAN_POINT ( 'NONE',  ( 16.93532580710000346, 1468.845588117029820, 189.7264854529979914 ) ) ;
#100618=CARTESIAN_POINT ( 'NONE',  ( -11.27553706004265166, 1425.429034480955124, 138.6747463096305353 ) ) ;
#100619=CARTESIAN_POINT ( 'NONE',  ( -31.54050611717723740, 1436.927665025879378, 136.6348558985098975 ) ) ;
#100623=EDGE_CURVE ( 'NONE', #42334, #44736, #56912, .T. ) ;
#100624=CARTESIAN_POINT ( 'NONE',  ( -11.89544747750000120, 1434.541746328260160, 147.6465872843980094 ) ) ;
#100625=CARTESIAN_POINT ( 'NONE',  ( 16.66257064975578928, 1410.427173609350120, 226.4839826715480342 ) ) ;
#100627=ORIENTED_EDGE ( 'NONE', *, *, #11363, .T. ) ;
#100628=CARTESIAN_POINT ( 'NONE',  ( -11.09668834241330160, 1414.913057819779851, 195.9645814827970014 ) ) ;
#100635=CARTESIAN_POINT ( 'NONE',  ( 18.76071169450000298, 1415.996778985530000, 210.2851423563980120 ) ) ;
#100638=CARTESIAN_POINT ( 'NONE',  ( 41.85283392122409651, 1440.913060353459969, 261.7677866120769750 ) ) ;
#100641=DIRECTION ( 'NONE',  ( -0.000000000000000000, 1.000000000000000000, 0.000000000000000000 ) ) ;
#100646=CARTESIAN_POINT ( 'NONE',  ( -15.27152961130000008, 1506.433683729329914, 224.9338604266980326 ) ) ;
#100650=CARTESIAN_POINT ( 'NONE',  ( -26.02647937380000087, 1444.708500955269983, 212.3004752285879988 ) ) ;
#100655=CARTESIAN_POINT ( 'NONE',  ( -16.42420382550000113, 1507.212883782629888, 224.6993357452979865 ) ) ;
#100656=ADVANCED_FACE ( 'NONE', ( #37196 ), #17691, .T. ) ;
#100657=CARTESIAN_POINT ( 'NONE',  ( 25.16854692840000141, 1451.224506325429957, 137.5711277893979911 ) ) ;
#100658=CARTESIAN_POINT ( 'NONE',  ( -27.42787280202326983, 1509.319616074060832, 212.0823359202047982 ) ) ;
#100660=EDGE_CURVE ( 'NONE', #13629, #49383, #66260, .T. ) ;
#100666=CARTESIAN_POINT ( 'NONE',  ( -20.64057905079999955, 1409.633845290530189, 214.6320756031479959 ) ) ;
#100669=EDGE_CURVE ( 'NONE', #88595, #94000, #91452, .T. ) ;
#100675=ADVANCED_FACE ( 'NONE', ( #14730 ), #78570, .T. ) ;
#100679=CARTESIAN_POINT ( 'NONE',  ( -0.3530891408735000181, 1467.116854267079816, 235.6078141451939985 ) ) ;
#100680=CARTESIAN_POINT ( 'NONE',  ( 0.5309744090729999755, 1408.931602422230071, 186.5522665233980035 ) ) ;
#100683=CARTESIAN_POINT ( 'NONE',  ( -3.686335301026030020, 1441.157504315399819, 159.2179879833419989 ) ) ;
#100684=CARTESIAN_POINT ( 'NONE',  ( -1.865418649941090079, 1450.587766904189948, 183.6624891833139941 ) ) ;
#100685=ORIENTED_EDGE ( 'NONE', *, *, #110442, .T. ) ;
#100687=EDGE_CURVE ( 'NONE', #110307, #12048, #95165, .T. ) ;
#100688=CARTESIAN_POINT ( 'NONE',  ( 18.09254145655199864, 1458.632396074990083, 227.9585907476449904 ) ) ;
#100689=CARTESIAN_POINT ( 'NONE',  ( -13.06415183560000060, 1435.235088203829946, 150.3757994387979977 ) ) ;
#100690=CARTESIAN_POINT ( 'NONE',  ( -1.160048314478139921E-08, 1473.720592319110210, 262.7804507126890030 ) ) ;
#100691=CARTESIAN_POINT ( 'NONE',  ( 19.74917098016377892, 1436.419552527919677, 145.7041280508210548 ) ) ;
#100692=CARTESIAN_POINT ( 'NONE',  ( -23.61227025210000008, 1435.322036687620084, 137.2858276859979867 ) ) ;
#100695=CARTESIAN_POINT ( 'NONE',  ( -1.464098976280000075, 1482.221117674429934, 182.5727748270979873 ) ) ;
#100698=CARTESIAN_POINT ( 'NONE',  ( 13.77652653775929892, 1509.191610193870019, 234.0674600905030047 ) ) ;
#100702=CARTESIAN_POINT ( 'NONE',  ( 5.563397900820960196, 1409.046698828469971, 222.4283399726890025 ) ) ;
#100707=CARTESIAN_POINT ( 'NONE',  ( 3.806770864790000264, 1421.349368237130193, 217.1428155965579947 ) ) ;
#100708=CARTESIAN_POINT ( 'NONE',  ( 0.4692969167009999887, 1499.385980790829990, 181.2668337229979727 ) ) ;
#100710=( BOUNDED_CURVE ( )  B_SPLINE_CURVE ( 3, ( #24120, #31994, #74566, #33089 ),
 .UNSPECIFIED., .F., .F. ) 
 B_SPLINE_CURVE_WITH_KNOTS ( ( 4, 4 ),
 ( 1.914873758155674954, 2.475997143201050132 ),
 .UNSPECIFIED. ) 
 CURVE ( )  GEOMETRIC_REPRESENTATION_ITEM ( )  RATIONAL_B_SPLINE_CURVE ( ( 1.000000000000000000, 0.9739333732078443440, 0.9739333732078443440, 1.000000000000000000 ) ) 
 REPRESENTATION_ITEM ( '' )  );
#100712=CARTESIAN_POINT ( 'NONE',  ( 12.53380499174499896, 1445.052233488290085, 169.4755105688890069 ) ) ;
#100714=CARTESIAN_POINT ( 'NONE',  ( -5.957780160061970420, 1452.705010119680082, 151.8756781206909920 ) ) ;
#100717=CARTESIAN_POINT ( 'NONE',  ( 17.04881831986960350, 1423.676757034399998, 228.9400447418400120 ) ) ;
#100719=ORIENTED_EDGE ( 'NONE', *, *, #7569, .F. ) ;
#100722=CARTESIAN_POINT ( 'NONE',  ( -24.07468318869999990, 1410.986369303230049, 209.5863555680950014 ) ) ;
#100723=CARTESIAN_POINT ( 'NONE',  ( -4.066872906969999590, 1425.385209600230155, 186.1255799332980132 ) ) ;
#100725=CARTESIAN_POINT ( 'NONE',  ( -45.48552204837235990, 1437.736068879899449, 266.1938101863335078 ) ) ;
#100726=CARTESIAN_POINT ( 'NONE',  ( -13.72848320130000133, 1498.343405282130107, 232.0117512395979986 ) ) ;
#100727=CARTESIAN_POINT ( 'NONE',  ( -18.13779422170000188, 1410.879222528129958, 224.5374549592980031 ) ) ;
#100728=CARTESIAN_POINT ( 'NONE',  ( 44.59751383069639985, 1448.382420665780046, 269.0041120828120143 ) ) ;
#100734=CARTESIAN_POINT ( 'NONE',  ( 18.35990977646854105, 1459.057757268718206, 227.7645059598757484 ) ) ;
#100739=CARTESIAN_POINT ( 'NONE',  ( 26.92975820915080121, 1451.047125116810093, 136.3586291375359849 ) ) ;
#100745=CARTESIAN_POINT ( 'NONE',  ( 10.74022137903229890, 1409.288117182390124, 190.7342599600210065 ) ) ;
#100746=DIRECTION ( 'NONE',  ( 0.9999999999999875655, -4.362347470284412856E-08, -1.513066404587939241E-07 ) ) ;
#100751=CARTESIAN_POINT ( 'NONE',  ( 7.276969490589999978, 1429.103926496630038, 148.8100812095979961 ) ) ;
#100753=CARTESIAN_POINT ( 'NONE',  ( 10.78869841494559978, 1414.913060387399810, 221.8582824516670087 ) ) ;
#100755=CARTESIAN_POINT ( 'NONE',  ( 20.59684415639999955, 1507.762623716630060, 227.3081670307980175 ) ) ;
#100760=CARTESIAN_POINT ( 'NONE',  ( -16.86383896579999941, 1465.456048507830019, 262.6648722463980334 ) ) ;
#100764=CARTESIAN_POINT ( 'NONE',  ( 11.14671186430000027, 1434.019362591839808, 151.6529851529979851 ) ) ;
#100765=CARTESIAN_POINT ( 'NONE',  ( 43.50000000000000000, 1445.861068816730040, 271.1218459616979999 ) ) ;
#100766=CARTESIAN_POINT ( 'NONE',  ( 12.73643648997659916, 1414.913060387399810, 198.3331475467240068 ) ) ;
#100768=CARTESIAN_POINT ( 'NONE',  ( 0.04809667444139999887, 1420.202366602630036, 183.9005171462980002 ) ) ;
#100769=AXIS2_PLACEMENT_3D ( 'NONE', #95114, #43063, #25124 ) ;
#100770=CARTESIAN_POINT ( 'NONE',  ( -15.06279714670009362, 1422.388303180917092, 229.4662111538715976 ) ) ;
#100771=DIRECTION ( 'NONE',  ( 0.000000000000000000, 0.000000000000000000, -1.000000000000000000 ) ) ;
#100772=CARTESIAN_POINT ( 'NONE',  ( 45.63712948719999218, 1440.913080918340029, 268.9747524690979503 ) ) ;
#100773=CARTESIAN_POINT ( 'NONE',  ( 17.92792478850000037, 1415.296882282229944, 210.0737307021219920 ) ) ;
#100774=CARTESIAN_POINT ( 'NONE',  ( 21.30585457869999999, 1410.903636177029966, 217.6543277114180057 ) ) ;
#100778=CARTESIAN_POINT ( 'NONE',  ( 4.945361357476200142E-08, 1407.050502962379824, 196.1173069476189994 ) ) ;
#100782=CARTESIAN_POINT ( 'NONE',  ( -10.47220825560000002, 1415.931784855930118, 223.5877942017980047 ) ) ;
#100783=CARTESIAN_POINT ( 'NONE',  ( 0.2068092021342020081, 1459.144971641600023, 182.9897654969599898 ) ) ;
#100784=CARTESIAN_POINT ( 'NONE',  ( 0.06333885262469998723, 1408.725629458430149, 223.1955288097980201 ) ) ;
#100786=CARTESIAN_POINT ( 'NONE',  ( -13.35741048202589809, 1444.324653571830822, 164.9741927960640453 ) ) ;
#100787=B_SPLINE_CURVE_WITH_KNOTS ( 'NONE', 3,
 ( #2872, #36992, #62232, #95256, #17970, #77904, #70638, #34792 ),
 .UNSPECIFIED., .F., .F.,
 ( 4, 2, 2, 4 ),
 ( 0.000000000000000000, 0.001508139020063445400, 0.003016278040126890801, 0.006032556080253484096 ),
 .UNSPECIFIED. ) ;
#100791=CARTESIAN_POINT ( 'NONE',  ( -41.06928241268209234, 1446.732447648640118, 134.0999999985529882 ) ) ;
#100793=ORIENTED_EDGE ( 'NONE', *, *, #7428, .F. ) ;
#100794=B_SPLINE_SURFACE_WITH_KNOTS ( 'NONE', 5, 1, ( 
 ( #22378, #30806 ),
 ( #24038, #90152 ),
 ( #57144, #109727 ),
 ( #64443, #13434 ),
 ( #15091, #49837 ),
 ( #91271, #21828 ) ),
 .UNSPECIFIED., .F., .F., .F.,
 ( 6, 6 ),
 ( 2, 2 ),
 ( 0.000000000000000000, 52.98902693510000006 ),
 ( -1.500000000000000000, 1.500000000000000000 ),
 .UNSPECIFIED. ) ;
#100798=LINE ( 'NONE', #92400, #99950 ) ;
#100801=DIRECTION ( 'NONE',  ( -0.1285470394059259891, 0.7041304581555918318, -0.6983379959285959115 ) ) ;
#100802=CARTESIAN_POINT ( 'NONE',  ( 21.36149126229999951, 1471.309244719029948, 210.4493499929980089 ) ) ;
#100803=DIRECTION ( 'NONE',  ( -0.9417419115949662300, -0.2378257470769920556, 0.2378257470769920556 ) ) ;
#100805=B_SPLINE_SURFACE_WITH_KNOTS ( 'NONE', 5, 4, ( 
 ( #98506, #55975, #53795, #90100, #44830 ),
 ( #78984, #2287, #36399, #2827, #105263 ),
 ( #109139, #6657, #30753, #39716, #15579 ),
 ( #23451, #108568, #73880, #83913, #57089 ),
 ( #15035, #82810, #40811, #31857, #74988 ),
 ( #109676, #90656, #66043, #82266, #13939 ) ),
 .UNSPECIFIED., .F., .F., .F.,
 ( 6, 6 ),
 ( 5, 5 ),
 ( 0.000000000000000000, 52.98902693510000006 ),
 ( 25.78146411700000229, 39.23969207129999859 ),
 .UNSPECIFIED. ) ;
#100810=EDGE_CURVE ( 'NONE', #100850, #2071, #54151, .T. ) ;
#100811=CARTESIAN_POINT ( 'NONE',  ( -15.86483609532009886, 1409.570356571889988, 225.8689455459189901 ) ) ;
#100816=CARTESIAN_POINT ( 'NONE',  ( -19.24471802889106442, 1410.946680197057731, 222.4942342983714809 ) ) ;
#100818=CARTESIAN_POINT ( 'NONE',  ( -0.1109497542296510042, 1419.781979276719994, 184.1980523464999919 ) ) ;
#100821=CARTESIAN_POINT ( 'NONE',  ( -17.69798016750000258, 1424.268916621029803, 226.8670750680979893 ) ) ;
#100825=CARTESIAN_POINT ( 'NONE',  ( 15.96958168569999970, 1519.913060387329779, 226.4768549569980109 ) ) ;
#100828=CARTESIAN_POINT ( 'NONE',  ( 3.115733349899999727, 1446.573609258350189, 168.9983159132980006 ) ) ;
#100829=ORIENTED_EDGE ( 'NONE', *, *, #27571, .T. ) ;
#100832=DIRECTION ( 'NONE',  ( -0.9417419115949053898, 0.3363363969979660806, 0.000000000000000000 ) ) ;
#100839=CARTESIAN_POINT ( 'NONE',  ( -10.81843803384433400, 1424.919119117232640, 144.3742235356994001 ) ) ;
#100840=CARTESIAN_POINT ( 'NONE',  ( 16.01103362314420053, 1409.480392854180081, 192.8179007169949841 ) ) ;
#100842=CARTESIAN_POINT ( 'NONE',  ( 41.15021254218909519, 1443.107472741189895, 136.8558449723329886 ) ) ;
#100844=SPHERICAL_SURFACE ( 'NONE', #16096, 1.999999999990000221 ) ;
#100845=CARTESIAN_POINT ( 'NONE',  ( 16.60410810222508715, 1460.741495510953882, 229.0095566175009196 ) ) ;
#100850=VERTEX_POINT ( 'NONE', #14589 ) ;
#100856=CARTESIAN_POINT ( 'NONE',  ( -29.78202337382098719, 1510.000480301286643, 209.1081380337732014 ) ) ;
#100860=VECTOR ( 'NONE', #105218, 1000.000000000000000 ) ;
#100861=CARTESIAN_POINT ( 'NONE',  ( -26.55602695130000157, 1507.993014311030038, 202.0788793302480144 ) ) ;
#100862=CARTESIAN_POINT ( 'NONE',  ( 36.37832872589339672, 1451.642701155429904, 134.7402676982789842 ) ) ;
#100863=CARTESIAN_POINT ( 'NONE',  ( 2.412365803710859957, 1421.274619602949997, 183.2637791671220100 ) ) ;
#100864=CARTESIAN_POINT ( 'NONE',  ( 25.98834105490000113, 1441.634093238639934, 138.4860864432980065 ) ) ;
#100870=ORIENTED_EDGE ( 'NONE', *, *, #31011, .F. ) ;
#100871=CARTESIAN_POINT ( 'NONE',  ( 11.82157071559280048, 1429.389078854110039, 149.1371689452649889 ) ) ;
#100874=CARTESIAN_POINT ( 'NONE',  ( -14.41084201949999866, 1416.311719782429918, 221.3435843107980077 ) ) ;
#100878=CARTESIAN_POINT ( 'NONE',  ( -12.93109072819999916, 1422.976826963529902, 222.1731802233979920 ) ) ;
#100882=CARTESIAN_POINT ( 'NONE',  ( -17.01808899029999722, 1507.624369750830056, 224.5631704104980031 ) ) ;
#100883=CARTESIAN_POINT ( 'NONE',  ( 12.85312037260000118, 1463.342809956830024, 231.1568051887979891 ) ) ;
#100884=PLANE ( 'NONE',  #54751 ) ;
#100885=CARTESIAN_POINT ( 'NONE',  ( -24.18363701780000241, 1464.258769156330118, 212.1671259816380086 ) ) ;
#100888=ORIENTED_EDGE ( 'NONE', *, *, #32585, .F. ) ;
#100889=CARTESIAN_POINT ( 'NONE',  ( -22.70357455280006320, 1409.705856010732305, 209.2041244077560691 ) ) ;
#100890=CARTESIAN_POINT ( 'NONE',  ( -0.2682795917991919743, 1457.891717849350016, 229.2666142623699841 ) ) ;
#100896=ORIENTED_EDGE ( 'NONE', *, *, #57038, .F. ) ;
#100898=CARTESIAN_POINT ( 'NONE',  ( -15.45814007687169855, 1507.562497965019929, 192.1857156550819923 ) ) ;
#100900=CARTESIAN_POINT ( 'NONE',  ( -11.86556339589999887, 1432.298474684649818, 149.9824464742980012 ) ) ;
#100903=CARTESIAN_POINT ( 'NONE',  ( 27.03107205873159913, 1451.493498638970550, 136.0706325128519438 ) ) ;
#100906=CARTESIAN_POINT ( 'NONE',  ( -25.21444118569999659, 1482.720987867629901, 215.4305335357680065 ) ) ;
#100908=CARTESIAN_POINT ( 'NONE',  ( -16.97075622830800157, 1460.580119305637936, 228.2620270748900282 ) ) ;
#100909=ORIENTED_EDGE ( 'NONE', *, *, #104233, .T. ) ;
#100911=CARTESIAN_POINT ( 'NONE',  ( 3.773527540909999978, 1405.891018842429730, 268.4776619642979654 ) ) ;
#100912=CARTESIAN_POINT ( 'NONE',  ( 0.02533456534659999856, 1409.857531607930014, 185.0280042643979925 ) ) ;
#100914=B_SPLINE_CURVE_WITH_KNOTS ( 'NONE', 3,
 ( #26424, #41721, #34832, #60618, #66947, #52757, #75881, #41173, #61724, #19113, #110029, #23799, #69018, #45476, #89641 ),
 .UNSPECIFIED., .F., .F.,
 ( 4, 2, 2, 1, 1, 1, 2, 2, 4 ),
 ( 0.000000000000000000, 0.2500000000000387468, 0.3750000000000583422, 0.4375000000000648370, 0.4687500000000691114, 0.4843750000000749956, 0.4921875000000756617, 0.5000000000000762723, 1.000000000000000000 ),
 .UNSPECIFIED. ) ;
#100915=CARTESIAN_POINT ( 'NONE',  ( -0.3501503302830000219, 1508.580655915329999, 237.8908601207980098 ) ) ;
#100917=CARTESIAN_POINT ( 'NONE',  ( 11.89463746674639921, 1434.488622511689982, 147.6463952746719883 ) ) ;
#100918=CARTESIAN_POINT ( 'NONE',  ( 18.22873622136830107, 1457.634151734390116, 229.9687917111629929 ) ) ;
#100920=CARTESIAN_POINT ( 'NONE',  ( -14.09544100519999965, 1444.804768886640204, 188.5648275900980195 ) ) ;
#100922=CARTESIAN_POINT ( 'NONE',  ( -19.88319835444530881, 1485.218947032791220, 190.7798981299888226 ) ) ;
#100925=EDGE_CURVE ( 'NONE', #104047, #18275, #55527, .T. ) ;
#100927=CARTESIAN_POINT ( 'NONE',  ( 4.440892098500000496E-16, 1426.979439823029907, 214.3676144195279676 ) ) ;
#100928=CIRCLE ( 'NONE', #63432, 1.999999999984720223 ) ;
#100933=CARTESIAN_POINT ( 'NONE',  ( -3.730291349180000271, 1475.207392057629932, 269.4937594316980380 ) ) ;
#100934=CARTESIAN_POINT ( 'NONE',  ( -4.231249791687170081, 1446.302986648280239, 164.6653561940370025 ) ) ;
#100935=CARTESIAN_POINT ( 'NONE',  ( -21.47619586280000092, 1509.724487542230008, 188.4280987144979633 ) ) ;
#100937=CARTESIAN_POINT ( 'NONE',  ( -11.91486543419761546, 1486.509543025264520, 184.3429713432209383 ) ) ;
#100941=CARTESIAN_POINT ( 'NONE',  ( -9.522333297019999421, 1438.200918636809774, 153.1793569429979982 ) ) ;
#100942=ADVANCED_FACE ( 'NONE', ( #42013 ), #84555, .T. ) ;
#100949=CARTESIAN_POINT ( 'NONE',  ( -15.23519492719600166, 1422.125166135662084, 227.7537822221859756 ) ) ;
#100951=ORIENTED_EDGE ( 'NONE', *, *, #55761, .T. ) ;
#100952=B_SPLINE_SURFACE_WITH_KNOTS ( 'NONE', 5, 5, ( 
 ( #23105, #4673, #98170, #5786, #55102, #57311, #81359, #72988, #37723, #98723, #29864, #107683, #97632, #89774, #11973, #38811, #71927, #29316, #82484, #55651, #47232, #107125, #30967, #39927 ),
 ( #14159, #81915, #89226, #56735, #46154, #30417, #5220, #4139, #21984, #63516, #56175, #90871, #99811, #12522, #46700, #22534, #108225, #72448, #65693, #48345, #65143, #80284, #99256, #80830 ),
 ( #90314, #13592, #106039, #20900, #47780, #106578, #64051, #21441, #74096, #39374, #13043, #73549, #67904, #85217, #102559, #40470, #7966, #102013, #68455, #50542, #15251, #25852, #41018, #67355 ),
 ( #152, #66805, #100906, #48903, #100380, #109348, #24741, #91976, #51092, #16344, #8508, #32629, #58390, #75741, #101452, #91437, #24204, #14713, #57848, #49442, #110432, #84121, #83030, #15783 ),
 ( #33711, #92515, #23665, #25296, #59497, #49984, #109885, #33165, #6321, #93070, #93608, #42133, #7420, #41586, #58939, #84667, #42681, #76283, #32072, #16887, #74644, #34274, #108780, #76839 ),
 ( #66263, #83565, #6858, #75197, #71652, #96255, #17441, #28499, #88404, #69011, #45870, #79462, #72716, #60053, #27947, #53736, #105211, #62694, #12794, #9077, #71086, #63772, #695, #46972 ) ),
 .UNSPECIFIED., .F., .F., .F.,
 ( 6, 6 ),
 ( 6, 3, 3, 3, 3, 3, 3, 6 ),
 ( 36.14021738890000535, 99.41336324060000607 ),
 ( 27.66640413320000036, 34.04499835230000571, 36.53903713200000425, 37.78605652179999908, 38.40956621670000004, 39.03307591160000101, 39.72833424150000070, 40.42359257149999507 ),
 .UNSPECIFIED. ) ;
#100953=CARTESIAN_POINT ( 'NONE',  ( -2.566563053771131475, 1410.380655407001086, 232.6501522581528434 ) ) ;
#100957=CARTESIAN_POINT ( 'NONE',  ( -0.4885701619419999808, 1464.413060387330006, 229.7716327975979880 ) ) ;
#100962=CARTESIAN_POINT ( 'NONE',  ( -1.011208509896629915, 1420.774206283469766, 183.0065381184390105 ) ) ;
#100965=CARTESIAN_POINT ( 'NONE',  ( -13.58235846979999906, 1416.828040475229955, 221.9087530951979659 ) ) ;
#100970=CARTESIAN_POINT ( 'NONE',  ( 19.89292065997459957, 1508.347995227200045, 229.2234713626579889 ) ) ;
#100972=ORIENTED_EDGE ( 'NONE', *, *, #27175, .F. ) ;
#100974=CARTESIAN_POINT ( 'NONE',  ( 11.63825043920830105, 1433.980580709160222, 151.1735222970980033 ) ) ;
#100975=CARTESIAN_POINT ( 'NONE',  ( -12.50012693489999904, 1397.670467479229956, 212.9149460363679793 ) ) ;
#100979=DIRECTION ( 'NONE',  ( -0.6638413695745983834, -0.7475172490850811036, -0.02307809267670082876 ) ) ;
#100982=CARTESIAN_POINT ( 'NONE',  ( -13.83792090743880010, 1508.660897340560041, 183.9592593128280100 ) ) ;
#100984=CARTESIAN_POINT ( 'NONE',  ( 6.918006061659999872, 1449.231408575739806, 185.2825139585980025 ) ) ;
#100988=CARTESIAN_POINT ( 'NONE',  ( 5.047496844141320160, 1396.089322873039919, 199.3124458601029971 ) ) ;
#100989=CARTESIAN_POINT ( 'NONE',  ( 1.061258286910000015, 1415.553739807329976, 190.7107924731980120 ) ) ;
#100990=CARTESIAN_POINT ( 'NONE',  ( 11.56455571449999908, 1431.422381474849999, 151.1349765661979916 ) ) ;
#100993=CARTESIAN_POINT ( 'NONE',  ( 12.89178610096769972, 1435.806136340959938, 150.7524150612520089 ) ) ;
#100996=CARTESIAN_POINT ( 'NONE',  ( 13.35361680572849075, 1444.505398037199257, 169.3732864882159106 ) ) ;
#100997=CARTESIAN_POINT ( 'NONE',  ( -8.485858099410000577, 1465.307528046030257, 233.0823719839980015 ) ) ;
#101001=ORIENTED_EDGE ( 'NONE', *, *, #54775, .F. ) ;
#101005=VERTEX_POINT ( 'NONE', #60484 ) ;
#101010=CARTESIAN_POINT ( 'NONE',  ( -2.935740633370000019, 1409.954265578529885, 186.6342734662979979 ) ) ;
#101012=CARTESIAN_POINT ( 'NONE',  ( 0.2223009155142280091, 1416.826860677879949, 227.1890218400880030 ) ) ;
#101013=VERTEX_POINT ( 'NONE', #23 ) ;
#101014=CARTESIAN_POINT ( 'NONE',  ( 22.45965404249999864, 1431.566040525590097, 217.4494758438079884 ) ) ;
#101019=CARTESIAN_POINT ( 'NONE',  ( 10.46129002499089999, 1411.316052440500243, 269.3482828489609915 ) ) ;
#101022=CARTESIAN_POINT ( 'NONE',  ( 24.07543316050000115, 1410.713981489629987, 209.3273838987269926 ) ) ;
#101023=CARTESIAN_POINT ( 'NONE',  ( -22.01123596709999930, 1509.713525028729919, 189.1765381185980175 ) ) ;
#101028=CARTESIAN_POINT ( 'NONE',  ( 0.1681681976620000019, 1420.473120457930008, 182.7464973445979979 ) ) ;
#101029=CARTESIAN_POINT ( 'NONE',  ( 10.97658109374170010, 1432.766920830290019, 151.7697937633350023 ) ) ;
#101034=CARTESIAN_POINT ( 'NONE',  ( 41.56056514950000036, 1440.913060317639975, 261.5690365818979330 ) ) ;
#101037=CARTESIAN_POINT ( 'NONE',  ( -5.402311893739999427, 1434.355786020779988, 154.6519262295979900 ) ) ;
#101040=DIRECTION ( 'NONE',  ( 0.000000000000000000, 0.000000000000000000, 1.000000000000000000 ) ) ;
#101046=CARTESIAN_POINT ( 'NONE',  ( -0.2682674118730000723, 1457.813445294729945, 229.2631846297979905 ) ) ;
#101048=CARTESIAN_POINT ( 'NONE',  ( 23.03439503529999755, 1449.683642696550123, 219.5641606253980171 ) ) ;
#101049=CARTESIAN_POINT ( 'NONE',  ( 7.957394096424367902, 1438.145637585891109, 153.7040555654163256 ) ) ;
#101050=CARTESIAN_POINT ( 'NONE',  ( -6.086798803919999834, 1421.074767261429997, 186.7378509026979998 ) ) ;
#101051=( BOUNDED_SURFACE ( )  B_SPLINE_SURFACE ( 3, 2, ( 
 ( #28788, #54570, #13604 ),
 ( #20911, #29874, #97098 ),
 ( #37736, #65154, #63527 ),
 ( #64615, #107694, #88153 ),
 ( #21995, #54024, #99267 ),
 ( #62987, #106588, #11441 ),
 ( #37191, #38275, #30428 ),
 ( #47241, #71937, #106049 ),
 ( #13055, #90325, #55116 ),
 ( #30979, #98734, #105497 ),
 ( #45615, #98181, #79756 ),
 ( #3062, #81369, #21451 ) ),
 .UNSPECIFIED., .F., .F., .T. ) 
 B_SPLINE_SURFACE_WITH_KNOTS ( ( 4, 2, 2, 2, 2, 4 ),
 ( 3, 3 ),
 ( 0.000000000000000000, 0.001069428368779032790, 0.001604142553168549186, 0.002138856737558065581, 0.003208285106337098371, 0.004277713475116131162 ),
 ( 0.000000000000000000, 1.000000000000000000 ),
 .UNSPECIFIED. ) 
 GEOMETRIC_REPRESENTATION_ITEM ( )  RATIONAL_B_SPLINE_SURFACE ( (
 ( 1.000000000000000000, 0.7071067811866051933, 1.000000000000000000),
 ( 1.000000000000000000, 0.7227579664598644538, 1.000000000000000000),
 ( 1.000000000000000000, 0.7381056972207281630, 1.000000000000000000),
 ( 1.000000000000000000, 0.7607155509935809024, 1.000000000000000000),
 ( 1.000000000000000000, 0.7681829160207560570, 1.000000000000000000),
 ( 1.000000000000000000, 0.7829721389379027396, 1.000000000000000000),
 ( 1.000000000000000000, 0.7902925692255797774, 1.000000000000000000),
 ( 1.000000000000000000, 0.8113688493901506371, 1.000000000000000000),
 ( 1.000000000000000000, 0.8244846461023084272, 1.000000000000000000),
 ( 1.000000000000000000, 0.8485067901407726820, 1.000000000000000000),
 ( 1.000000000000000000, 0.8591713199357238206, 1.000000000000000000),
 ( 1.000000000000000000, 0.8676405061997034540, 1.000000000000000000) ) ) 
 REPRESENTATION_ITEM ( '' )  SURFACE ( )  );
#101053=CARTESIAN_POINT ( 'NONE',  ( 4.053537042790000378, 1441.572390738320109, 183.3424090224980034 ) ) ;
#101054=CARTESIAN_POINT ( 'NONE',  ( 27.32002834875690311, 1436.780620296950019, 136.7657361291360019 ) ) ;
#101055=CARTESIAN_POINT ( 'NONE',  ( 39.06740725280500470, 1447.641448397309887, 136.5466146009009947 ) ) ;
#101056=CARTESIAN_POINT ( 'NONE',  ( -23.42261135620000090, 1434.595605500659985, 214.6024269201780044 ) ) ;
#101057=CARTESIAN_POINT ( 'NONE',  ( -36.06148001838602113, 1461.985359838420209, 269.2267996494942395 ) ) ;
#101060=CARTESIAN_POINT ( 'NONE',  ( -17.59370741740000099, 1418.348682474430007, 226.0262961122979846 ) ) ;
#101063=CARTESIAN_POINT ( 'NONE',  ( -5.510509099684978374, 1471.237799169209666, 269.3375995838932226 ) ) ;
#101066=CARTESIAN_POINT ( 'NONE',  ( -32.06316538499910251, 1416.592306352786409, 269.3144317999657460 ) ) ;
#101067=CARTESIAN_POINT ( 'NONE',  ( 14.80452861058799918, 1440.352436769449923, 190.1999221398900204 ) ) ;
#101068=CARTESIAN_POINT ( 'NONE',  ( -14.86238962927253837, 1451.964376860417815, 222.9824286697244418 ) ) ;
#101072=CARTESIAN_POINT ( 'NONE',  ( 0.000000000000000000, 1412.913060387329779, 209.1218459616979999 ) ) ;
#101073=CARTESIAN_POINT ( 'NONE',  ( -38.58235177178170261, 1444.329162691080228, 137.1361782391459769 ) ) ;
#101074=ADVANCED_FACE ( 'NONE', ( #24618 ), #24080, .T. ) ;
#101075=CARTESIAN_POINT ( 'NONE',  ( 25.34079329589999929, 1436.168901596849992, 137.1732139229980021 ) ) ;
#101076=CARTESIAN_POINT ( 'NONE',  ( -13.11972090476676733, 1443.041373250473725, 169.4030072996578724 ) ) ;
#101077=CARTESIAN_POINT ( 'NONE',  ( -13.61519277519999882, 1409.388513392130108, 226.0716413619979903 ) ) ;
#101078=VERTEX_POINT ( 'NONE', #16226 ) ;
#101079=CARTESIAN_POINT ( 'NONE',  ( 0.08760820899984020360, 1414.971390223319986, 192.4206628386800162 ) ) ;
#101081=ADVANCED_FACE ( 'NONE', ( #17321 ), #67391, .T. ) ;
#101086=CARTESIAN_POINT ( 'NONE',  ( 41.25815740437244017, 1435.010063311743352, 269.6334395952857221 ) ) ;
#101087=CARTESIAN_POINT ( 'NONE',  ( -11.53898582669999939, 1459.427238891729985, 220.7971265779980286 ) ) ;
#101089=CARTESIAN_POINT ( 'NONE',  ( -11.17066468859999873, 1433.159422583310061, 151.6197124790980126 ) ) ;
#101093=CARTESIAN_POINT ( 'NONE',  ( -12.37159932449999822, 1415.628674266529742, 195.6623782650979990 ) ) ;
#101095=CARTESIAN_POINT ( 'NONE',  ( -2.883410015801580073, 1409.181736952820074, 187.1726418057029946 ) ) ;
#101097=CARTESIAN_POINT ( 'NONE',  ( -27.60455267767378729, 1509.989042806181033, 197.3747958975489212 ) ) ;
#101098=CARTESIAN_POINT ( 'NONE',  ( -1.558958650196000183E-09, 1416.365570055059834, 239.4563497976100166 ) ) ;
#101101=CARTESIAN_POINT ( 'NONE',  ( -11.76590084519579982, 1427.017745790240042, 146.1561352580970095 ) ) ;
#101103=CARTESIAN_POINT ( 'NONE',  ( -5.151088789370000143, 1471.205953851929962, 269.3380511851980259 ) ) ;
#101107=CARTESIAN_POINT ( 'NONE',  ( 38.00281594157139864, 1449.406348292719940, 136.2793115458389934 ) ) ;
#101108=CARTESIAN_POINT ( 'NONE',  ( 16.75801468479999912, 1408.913060387329779, 202.5679462747779667 ) ) ;
#101110=B_SPLINE_SURFACE_WITH_KNOTS ( 'NONE', 5, 5, ( 
 ( #20958, #90369, #46762, #90931, #12580, #3661, #47837, #98228, #97139 ),
 ( #31023, #105551, #37790, #107185, #63569, #22591, #106628, #54614, #28838 ),
 ( #64663, #81970, #30475, #29917, #55162, #97685, #13104, #5278, #80891 ),
 ( #21498, #71978, #55711, #65204, #81410, #14218, #47287, #4722, #98780 ),
 ( #22043, #56240, #39433, #73609, #56794, #32136, #33230, #59556, #24805 ),
 ( #93137, #67419, #74708, #23722, #91495, #76348, #109410, #83631, #7483 ),
 ( #48960, #32686, #58452, #108289, #14774, #39982, #100975, #93670, #6927 ),
 ( #108839, #102081, #41084, #75261, #57907, #31575, #83091, #65752, #15313 ),
 ( #59010, #16405, #92041, #33777, #84184, #57368, #6384, #40532, #41644 ),
 ( #66321, #66867, #109951, #110497, #82548, #75800, #100439, #67973, #74158 ),
 ( #99869, #50599, #49506, #23168, #24271, #84731, #92579, #15851, #50056 ),
 ( #101518, #48404, #8028, #5842, #42197, #25364, #95358, #87519, #69077 ) ),
 .UNSPECIFIED., .F., .F., .F.,
 ( 6, 3, 3, 6 ),
 ( 6, 3, 6 ),
 ( 12.74698783810000080, 30.29491413010000045, 39.81482060289999936, 57.85069212530000016 ),
 ( 0.000000000000000000, 1.000000000000000000, 2.000000000000000000 ),
 .UNSPECIFIED. ) ;
#101112=DIRECTION ( 'NONE',  ( -0.3522034561021770704, -0.9359206307609502229, -0.002301830946695800680 ) ) ;
#101115=CARTESIAN_POINT ( 'NONE',  ( -10.60590658980659917, 1406.964585531180091, 269.0015838391640273 ) ) ;
#101116=CARTESIAN_POINT ( 'NONE',  ( -13.40001318606720027, 1436.143823819350018, 150.5590804106440146 ) ) ;
#101119=EDGE_LOOP ( 'NONE', ( #79350, #54227, #96351, #96573 ) ) ;
#101120=ORIENTED_EDGE ( 'NONE', *, *, #87057, .T. ) ;
#101121=CARTESIAN_POINT ( 'NONE',  ( 5.009343724018470390, 1422.720564319518871, 184.4316651301672891 ) ) ;
#101127=CARTESIAN_POINT ( 'NONE',  ( 2.502366908949907653, 1409.000444965305178, 224.1100396174575167 ) ) ;
#101128=ORIENTED_EDGE ( 'NONE', *, *, #35804, .T. ) ;
#101132=CARTESIAN_POINT ( 'NONE',  ( -4.319145873661043744, 1421.270721947785205, 186.1375689364567165 ) ) ;
#101134=AXIS2_PLACEMENT_3D ( 'NONE', #34088, #68281, #51447 ) ;
#101135=CARTESIAN_POINT ( 'NONE',  ( -5.091556393439999439, 1407.116996366430158, 197.0899548111979698 ) ) ;
#101137=CARTESIAN_POINT ( 'NONE',  ( -38.10537780832459731, 1442.926987427690165, 137.1117395883960057 ) ) ;
#101139=CARTESIAN_POINT ( 'NONE',  ( -24.05132347639830215, 1411.090389413789808, 209.8326646502659969 ) ) ;
#101140=CARTESIAN_POINT ( 'NONE',  ( 28.13115138590000086, 1508.134099165530188, 210.1250122821180071 ) ) ;
#101141=CARTESIAN_POINT ( 'NONE',  ( 3.761652188060691682, 1425.538669997582474, 185.2058339228567263 ) ) ;
#101143=CARTESIAN_POINT ( 'NONE',  ( -24.52144259279999972, 1435.632488953809798, 137.5271284461979917 ) ) ;
#101144=B_SPLINE_CURVE_WITH_KNOTS ( 'NONE', 3,
 ( #101447, #67900, #42676, #18550 ),
 .UNSPECIFIED., .F., .F.,
 ( 4, 4 ),
 ( 0.000000000000000000, 1.000000000000000000 ),
 .UNSPECIFIED. ) ;
#101145=CARTESIAN_POINT ( 'NONE',  ( -24.49688161579999957, 1441.286190042660110, 211.0056646591280014 ) ) ;
#101150=DIRECTION ( 'NONE',  ( 7.205227288424627209E-20, 0.9876883405951701889, 0.1564344650400262826 ) ) ;
#101155=CARTESIAN_POINT ( 'NONE',  ( -20.89050673521863999, 1455.005279222091303, 223.4623653643373302 ) ) ;
#101156=VERTEX_POINT ( 'NONE', #52078 ) ;
#101158=CARTESIAN_POINT ( 'NONE',  ( 12.93087728801789993, 1434.999496278460128, 150.1242520500200044 ) ) ;
#101159=CARTESIAN_POINT ( 'NONE',  ( 17.51310050168130061, 1459.308345724359924, 228.3567006344079857 ) ) ;
#101161=CARTESIAN_POINT ( 'NONE',  ( 27.01382310970000233, 1451.969724731730139, 134.9184576876980088 ) ) ;
#101164=CARTESIAN_POINT ( 'NONE',  ( -15.10324083849999965, 1409.440477179229902, 225.7327363557979822 ) ) ;
#101166=CARTESIAN_POINT ( 'NONE',  ( -0.1681681984989999989, 1413.717199569329750, 164.8680577770979880 ) ) ;
#101169=VERTEX_POINT ( 'NONE', #86210 ) ;
#101170=CARTESIAN_POINT ( 'NONE',  ( -11.40293847520729997, 1414.971993471380074, 196.2990445993690116 ) ) ;
#101172=CARTESIAN_POINT ( 'NONE',  ( 2.235819005889999822, 1419.966584392630011, 185.0820763846980128 ) ) ;
#101180=CARTESIAN_POINT ( 'NONE',  ( 17.20238589132565821, 1422.398122266642531, 226.7110313106093145 ) ) ;
#101181=CARTESIAN_POINT ( 'NONE',  ( 18.59509526533679136, 1425.782355783442199, 224.9721248484763692 ) ) ;
#101182=CARTESIAN_POINT ( 'NONE',  ( -9.603657968282620217E-07, 1408.141559225309948, 222.5225557192960082 ) ) ;
#101183=LINE ( 'NONE', #93895, #52700 ) ;
#101186=CARTESIAN_POINT ( 'NONE',  ( 13.00108844889999915, 1422.957393747230071, 222.1873873175979952 ) ) ;
#101190=CARTESIAN_POINT ( 'NONE',  ( -19.42715338204342501, 1485.587694890019065, 189.9367742298745156 ) ) ;
#101191=CARTESIAN_POINT ( 'NONE',  ( -29.11003132769999624, 1509.929605081229965, 211.9058968252579973 ) ) ;
#101194=DIRECTION ( 'NONE',  ( -0.7071067811860475283, 0.000000000000000000, -0.7071067811870476172 ) ) ;
#101196=CIRCLE ( 'NONE', #56554, 2.008813507203440096 ) ;
#101199=CARTESIAN_POINT ( 'NONE',  ( 15.96653243319999937, 1452.355496787929951, 148.2552934822979864 ) ) ;
#101206=CARTESIAN_POINT ( 'NONE',  ( -19.18108385108779856, 1409.582878595139846, 219.3495538156010127 ) ) ;
#101210=CARTESIAN_POINT ( 'NONE',  ( 34.15097007435170440, 1437.022904788399956, 136.5542998879990080 ) ) ;
#101211=CARTESIAN_POINT ( 'NONE',  ( -11.90008666459999986, 1434.920851464509951, 147.6452002888979962 ) ) ;
#101212=DIRECTION ( 'NONE',  ( 1.987342477590000096E-13, -6.939952856119990566E-15, -1.000000000000000000 ) ) ;
#101215=CARTESIAN_POINT ( 'NONE',  ( -11.42988456683059617, 1434.706941777702468, 151.4745012951066201 ) ) ;
#101217=CARTESIAN_POINT ( 'NONE',  ( 1.201030227405109896, 1507.126550697769972, 181.0678294923270073 ) ) ;
#101218=CARTESIAN_POINT ( 'NONE',  ( 18.03271313680000176, 1424.708338662830101, 225.1466562137979963 ) ) ;
#101220=CARTESIAN_POINT ( 'NONE',  ( -11.86606300521394353, 1432.348818993920986, 150.6996689860163485 ) ) ;
#101221=CARTESIAN_POINT ( 'NONE',  ( -2.710844305144630262, 1440.404038868829957, 159.2733880920049785 ) ) ;
#101222=DIRECTION ( 'NONE',  ( 0.000000000000000000, 1.000000000000000000, 0.000000000000000000 ) ) ;
#101223=ORIENTED_EDGE ( 'NONE', *, *, #36617, .F. ) ;
#101224=CARTESIAN_POINT ( 'NONE',  ( 4.074350933259999502E-15, 1428.579607037230062, 149.5143047311979672 ) ) ;
#101225=CARTESIAN_POINT ( 'NONE',  ( 19.68865308375039902, 1455.839336106299925, 227.5737452897460003 ) ) ;
#101226=CARTESIAN_POINT ( 'NONE',  ( 15.78884811940000077, 1449.507807645780076, 190.2809706474979805 ) ) ;
#101227=CARTESIAN_POINT ( 'NONE',  ( -8.859375228535989748E-12, 1470.046988918149964, 254.1474031498040063 ) ) ;
#101232=CARTESIAN_POINT ( 'NONE',  ( -0.04889493835150059836, 1486.217974350728127, 181.8156037349973246 ) ) ;
#101234=CARTESIAN_POINT ( 'NONE',  ( -45.62076656701439958, 1439.252528880889940, 266.1899235483149937 ) ) ;
#101235=FACE_OUTER_BOUND ( 'NONE', #103468, .T. ) ;
#101238=CARTESIAN_POINT ( 'NONE',  ( -2.478946879530000036, 1432.276406454319840, 157.5139443807979944 ) ) ;
#101242=CARTESIAN_POINT ( 'NONE',  ( -26.85028794030449717, 1451.809831805880094, 135.6476290392230055 ) ) ;
#101244=CARTESIAN_POINT ( 'NONE',  ( 26.67762292569999971, 1440.913060399449932, 225.6805344092979908 ) ) ;
#101246=CARTESIAN_POINT ( 'NONE',  ( -4.363122647530000009, 1419.257904667329967, 165.6263425522979844 ) ) ;
#101248=CARTESIAN_POINT ( 'NONE',  ( -24.09814616333339998, 1444.255785637029931, 212.5772553280679915 ) ) ;
#101249=CARTESIAN_POINT ( 'NONE',  ( -29.11537602464361640, 1509.936047831340375, 204.3288344588696930 ) ) ;
#101250=CARTESIAN_POINT ( 'NONE',  ( 22.57319362359999815, 1409.701316935530031, 208.7927549349429910 ) ) ;
#101254=CARTESIAN_POINT ( 'NONE',  ( 16.50119538672600328, 1422.031755069739802, 227.1504397986250012 ) ) ;
#101259=CARTESIAN_POINT ( 'NONE',  ( -23.58958983610000359, 1410.013969636130014, 209.3130814696430093 ) ) ;
#101262=DIRECTION ( 'NONE',  ( 0.000000000000000000, 0.000000000000000000, -1.000000000000000000 ) ) ;
#101263=CARTESIAN_POINT ( 'NONE',  ( -1.024257868869999921, 1498.353689748030092, 236.8278422010980080 ) ) ;
#101264=CARTESIAN_POINT ( 'NONE',  ( -21.04576247069999795, 1410.867134376630247, 218.2990911740579918 ) ) ;
#101265=AXIS2_PLACEMENT_3D ( 'NONE', #59859, #109297, #30917 ) ;
#101267=CARTESIAN_POINT ( 'NONE',  ( 44.56610056812340304, 1449.954323543940063, 266.7258405368609715 ) ) ;
#101270=CARTESIAN_POINT ( 'NONE',  ( -17.07650506179803784, 1422.150741894849034, 226.7700359724246937 ) ) ;
#101272=ORIENTED_EDGE ( 'NONE', *, *, #100687, .F. ) ;
#101273=CARTESIAN_POINT ( 'NONE',  ( 18.48198528575022692, 1458.805764898813550, 227.6411767142042493 ) ) ;
#101276=ORIENTED_EDGE ( 'NONE', *, *, #71407, .F. ) ;
#101284=CARTESIAN_POINT ( 'NONE',  ( 19.74914731032970039, 1409.602715808129915, 217.6725271438159837 ) ) ;
#101286=CARTESIAN_POINT ( 'NONE',  ( 12.62627334406020019, 1409.353979568340037, 191.9928717526780133 ) ) ;
#101287=CARTESIAN_POINT ( 'NONE',  ( 1.053929134969999959, 1415.609761246630114, 233.1238235151980120 ) ) ;
#101288=CARTESIAN_POINT ( 'NONE',  ( 3.827327205999999649, 1425.634807632230149, 171.7326279529979729 ) ) ;
#101289=CARTESIAN_POINT ( 'NONE',  ( 14.91703010720000044, 1409.433974557229931, 225.8933006754979829 ) ) ;
#101291=CARTESIAN_POINT ( 'NONE',  ( 12.88172607065413544, 1420.897005229514207, 231.3054420824058184 ) ) ;
#101293=CARTESIAN_POINT ( 'NONE',  ( 13.02322915956219873, 1416.825783990419950, 221.6328433159220026 ) ) ;
#101294=CARTESIAN_POINT ( 'NONE',  ( 11.62445986000279952, 1432.338721181900155, 150.9949992740019979 ) ) ;
#101297=B_SPLINE_CURVE_WITH_KNOTS ( 'NONE', 3,
 ( #22956, #83983, #15645, #24058, #8368, #76690, #40328, #32492, #49851, #1, #66664, #24601 ),
 .UNSPECIFIED., .F., .F.,
 ( 4, 2, 2, 2, 2, 4 ),
 ( 0.000000000000000000, 0.2500000000000786038, 0.3750000000001127987, 0.4375000000000939249, 0.5000000000000750511, 1.000000000000000000 ),
 .UNSPECIFIED. ) ;
#101302=CARTESIAN_POINT ( 'NONE',  ( -17.87874080430000134, 1466.750581352830068, 265.6112252686980355 ) ) ;
#101303=CARTESIAN_POINT ( 'NONE',  ( -22.28175276906668856, 1509.670458419194802, 191.1299263873633265 ) ) ;
#101304=CARTESIAN_POINT ( 'NONE',  ( 11.23027220810000060, 1433.733175409749947, 151.5806659527979718 ) ) ;
#101305=CARTESIAN_POINT ( 'NONE',  ( 32.79207798030000021, 1453.265480487729974, 262.6648722511980054 ) ) ;
#101307=ADVANCED_FACE ( 'NONE', ( #4303 ), #6939, .F. ) ;
#101312=CARTESIAN_POINT ( 'NONE',  ( 22.74352444629999681, 1409.874439160429802, 207.7226808069280253 ) ) ;
#101313=CARTESIAN_POINT ( 'NONE',  ( 10.21356127135914349, 1398.215732791116807, 217.1961878391145149 ) ) ;
#101314=CARTESIAN_POINT ( 'NONE',  ( -16.56429154530000147, 1409.491498197430019, 225.2428481817979957 ) ) ;
#101315=CARTESIAN_POINT ( 'NONE',  ( 18.68355583210000148, 1410.903490284329791, 222.0895934915980092 ) ) ;
#101316=AXIS2_PLACEMENT_3D ( 'NONE', #71936, #4147, #30978 ) ;
#101317=B_SPLINE_CURVE_WITH_KNOTS ( 'NONE', 3,
 ( #47810, #5248, #6894, #13073 ),
 .UNSPECIFIED., .F., .F.,
 ( 4, 4 ),
 ( 0.000000000000000000, 1.000000000000000000 ),
 .UNSPECIFIED. ) ;
#101319=CARTESIAN_POINT ( 'NONE',  ( -16.16107894238729870, 1409.477417702470120, 193.2192893929600075 ) ) ;
#101324=CARTESIAN_POINT ( 'NONE',  ( 0.1696119624267240222, 1480.557672209769862, 182.0704353423009820 ) ) ;
#101325=CARTESIAN_POINT ( 'NONE',  ( -3.109694234880000074, 1409.021653302929735, 223.8091977979979958 ) ) ;
#101326=ORIENTED_EDGE ( 'NONE', *, *, #5669, .F. ) ;
#101327=CARTESIAN_POINT ( 'NONE',  ( -13.51610093809999924, 1444.324653571829913, 169.3501091259980171 ) ) ;
#101329=CARTESIAN_POINT ( 'NONE',  ( 11.87907512690000011, 1433.311753932999864, 149.8850494226980175 ) ) ;
#101330=CARTESIAN_POINT ( 'NONE',  ( -40.49955491220639914, 1447.865363690129925, 134.0999999983799853 ) ) ;
#101340=VECTOR ( 'NONE', #70375, 1000.000000000000114 ) ;
#101346=ORIENTED_EDGE ( 'NONE', *, *, #77392, .T. ) ;
#101347=CARTESIAN_POINT ( 'NONE',  ( -33.92643339480000719, 1450.868067258620158, 136.1711496515980286 ) ) ;
#101348=CARTESIAN_POINT ( 'NONE',  ( -15.73572830516989995, 1409.462552141119886, 225.2909338128490049 ) ) ;
#101350=VERTEX_POINT ( 'NONE', #93776 ) ;
#101353=CARTESIAN_POINT ( 'NONE',  ( -21.47452075964614338, 1411.021838315141167, 216.8631755304516560 ) ) ;
#101356=B_SPLINE_CURVE_WITH_KNOTS ( 'NONE', 5,
 ( #82738, #100625, #74364, #6029, #23908, #41291 ),
 .UNSPECIFIED., .F., .F.,
 ( 6, 6 ),
 ( 0.000000000000000000, 1.000000000000000000 ),
 .UNSPECIFIED. ) ;
#101357=CARTESIAN_POINT ( 'NONE',  ( 41.29477646232137289, 1446.681373312819233, 269.6341301600875227 ) ) ;
#101358=CARTESIAN_POINT ( 'NONE',  ( 15.40733310992444061, 1431.102793365615526, 219.5436081709931102 ) ) ;
#101359=CARTESIAN_POINT ( 'NONE',  ( 1.537569739530000090, 1415.820179752829972, 232.6983187733980003 ) ) ;
#101362=CARTESIAN_POINT ( 'NONE',  ( 8.486299124169999430, 1519.913060387329779, 230.6230627099979813 ) ) ;
#101367=CARTESIAN_POINT ( 'NONE',  ( 2.712106673540000124, 1447.524052171519770, 157.8378389823980115 ) ) ;
#101369=VERTEX_POINT ( 'NONE', #70300 ) ;
#101370=CARTESIAN_POINT ( 'NONE',  ( 13.58268853699999923, 1416.851343894929869, 196.3340833729979806 ) ) ;
#101373=CARTESIAN_POINT ( 'NONE',  ( -16.17440652799999867, 1423.017051802529977, 229.3744292183979780 ) ) ;
#101376=CARTESIAN_POINT ( 'NONE',  ( -25.25968088059999772, 1449.800564160949989, 206.5373934562080080 ) ) ;
#101377=CARTESIAN_POINT ( 'NONE',  ( -10.80134480061109947, 1441.261220175989820, 153.0805715986579969 ) ) ;
#101378=CARTESIAN_POINT ( 'NONE',  ( 16.04662172663540076, 1409.498810407800192, 192.7255589890200156 ) ) ;
#101380=CARTESIAN_POINT ( 'NONE',  ( 40.14205882339999221, 1442.180247714630013, 136.9520358780980018 ) ) ;
#101381=ADVANCED_FACE ( 'NONE', ( #60218 ), #101708, .T. ) ;
#101382=CARTESIAN_POINT ( 'NONE',  ( 2.939888137859999853E-10, 1407.100405669929842, 264.8986903017979557 ) ) ;
#101383=CARTESIAN_POINT ( 'NONE',  ( 2.883409711490000138, 1409.181735907030088, 231.0710487667979862 ) ) ;
#101387=CARTESIAN_POINT ( 'NONE',  ( -34.35202081865160295, 1437.040941089060198, 136.5493581184059906 ) ) ;
#101390=CARTESIAN_POINT ( 'NONE',  ( -18.60076228999999870, 1457.261067633329958, 228.0100651602980122 ) ) ;
#101395=CARTESIAN_POINT ( 'NONE',  ( 29.38941569566759782, 1446.173485254500065, 137.1432708255389912 ) ) ;
#101403=CARTESIAN_POINT ( 'NONE',  ( 40.71747596959940552, 1448.637563236709866, 134.4205493173820116 ) ) ;
#101405=EDGE_CURVE ( 'NONE', #80510, #42283, #39069, .T. ) ;
#101406=CARTESIAN_POINT ( 'NONE',  ( 25.77823332670000056, 1439.625665060110123, 137.8633119874980082 ) ) ;
#101412=ORIENTED_EDGE ( 'NONE', *, *, #13778, .F. ) ;
#101413=CARTESIAN_POINT ( 'NONE',  ( 11.79395621469850042, 1427.957957693540038, 147.8640485709500183 ) ) ;
#101414=ADVANCED_FACE ( 'NONE', ( #34724 ), #6543, .T. ) ;
#101416=CARTESIAN_POINT ( 'NONE',  ( 19.78107824579999985, 1507.861720175329992, 229.2768328414980203 ) ) ;
#101418=CARTESIAN_POINT ( 'NONE',  ( -13.65307821740000094, 1415.140114704729967, 220.7168886283980100 ) ) ;
#101419=CARTESIAN_POINT ( 'NONE',  ( -11.86610048948770135, 1432.336024750160050, 149.9824232984959735 ) ) ;
#101422=CARTESIAN_POINT ( 'NONE',  ( -4.280412110000000325, 1421.771089477929763, 185.3634408331980126 ) ) ;
#101423=CARTESIAN_POINT ( 'NONE',  ( 14.51815713490480064, 1436.250993400889911, 149.9197837022770159 ) ) ;
#101425=CARTESIAN_POINT ( 'NONE',  ( -9.958615577691062981, 1410.635533730419411, 188.4118002158843126 ) ) ;
#101427=CARTESIAN_POINT ( 'NONE',  ( -16.66912029359999892, 1496.363909377430218, 224.2133594559979883 ) ) ;
#101435=EDGE_CURVE ( 'NONE', #16284, #39656, #69486, .T. ) ;
#101440=CARTESIAN_POINT ( 'NONE',  ( -11.43219139277870688, 1425.761513233309643, 138.9711987641360338 ) ) ;
#101445=CARTESIAN_POINT ( 'NONE',  ( -11.64843198310000005, 1425.854362680330041, 145.0892392246979909 ) ) ;
#101447=CARTESIAN_POINT ( 'NONE',  ( 33.91369266730000476, 1450.440660192670066, 136.2454535554979884 ) ) ;
#101448=CARTESIAN_POINT ( 'NONE',  ( 27.03067664649999813, 1451.714498883330180, 135.7945611549980072 ) ) ;
#101449=CARTESIAN_POINT ( 'NONE',  ( -2.500000000000000000, 1417.575542696430148, 161.0097146498980010 ) ) ;
#101450=EDGE_CURVE ( 'NONE', #78256, #34085, #13916, .T. ) ;
#101451=DIRECTION ( 'NONE',  ( 0.000000000000000000, -0.7071067811865467956, 0.7071067811865481278 ) ) ;
#101452=CARTESIAN_POINT ( 'NONE',  ( -20.67946632569999821, 1482.729195731830032, 226.2368318870979920 ) ) ;
#101453=CARTESIAN_POINT ( 'NONE',  ( -10.49833687454975717, 1422.381355195064998, 137.0999999980979567 ) ) ;
#101455=VERTEX_POINT ( 'NONE', #82792 ) ;
#101457=CARTESIAN_POINT ( 'NONE',  ( 7.072283668360000775, 1406.251336213230161, 267.2142513328980158 ) ) ;
#101459=CARTESIAN_POINT ( 'NONE',  ( 0.3485282687889999509, 1410.306756019930162, 185.0335118036979907 ) ) ;
#101462=B_SPLINE_CURVE_WITH_KNOTS ( 'NONE', 3,
 ( #77446, #33217, #67960, #50587 ),
 .UNSPECIFIED., .F., .F.,
 ( 4, 4 ),
 ( 0.000000000000000000, 0.003000049121573526711 ),
 .UNSPECIFIED. ) ;
#101463=CARTESIAN_POINT ( 'NONE',  ( 20.43741061629999933, 1430.298857861630040, 196.2683185269980015 ) ) ;
#101464=CARTESIAN_POINT ( 'NONE',  ( 8.010394309675456626, 1506.575487365668323, 229.7209142108047786 ) ) ;
#101467=CARTESIAN_POINT ( 'NONE',  ( -18.55872592996471582, 1457.839997766627903, 227.5285588845430595 ) ) ;
#101469=CARTESIAN_POINT ( 'NONE',  ( -12.85666456360000076, 1446.605478062839893, 187.9028615879979895 ) ) ;
#101470=CARTESIAN_POINT ( 'NONE',  ( -20.55257633559999775, 1497.713060387329961, 217.2216651986680063 ) ) ;
#101472=CARTESIAN_POINT ( 'NONE',  ( 2.339369641392206489, 1407.692004974928750, 270.1366117262977014 ) ) ;
#101473=CARTESIAN_POINT ( 'NONE',  ( 1.460551075230569928, 1495.400065749579881, 181.6242104856870299 ) ) ;
#101478=CARTESIAN_POINT ( 'NONE',  ( -18.29970625680000040, 1473.000870360929866, 266.8291869051980143 ) ) ;
#101481=CARTESIAN_POINT ( 'NONE',  ( 17.96224420295349944, 1421.095635167079763, 223.9963144870330041 ) ) ;
#101484=CIRCLE ( 'NONE', #6712, 1.000000000000000000 ) ;
#101485=FACE_OUTER_BOUND ( 'NONE', #86088, .T. ) ;
#101486=CARTESIAN_POINT ( 'NONE',  ( 2.021659750777782261, 1408.983658301473724, 230.3023721903324486 ) ) ;
#101488=CARTESIAN_POINT ( 'NONE',  ( -45.85459844547133912, 1440.913031240881764, 268.7562811153424605 ) ) ;
#101490=CARTESIAN_POINT ( 'NONE',  ( -17.71984068230000275, 1409.531850859229962, 197.2724686579979902 ) ) ;
#101494=CARTESIAN_POINT ( 'NONE',  ( 1.661536740469999884, 1441.600846913620217, 150.6803463261979914 ) ) ;
#101498=( BOUNDED_CURVE ( )  B_SPLINE_CURVE ( 3, ( #84941, #58121, #25030, #8234 ),
 .UNSPECIFIED., .F., .F. ) 
 B_SPLINE_CURVE_WITH_KNOTS ( ( 4, 4 ),
 ( 0.1704839434639374984, 0.4574025252004559894 ),
 .UNSPECIFIED. ) 
 CURVE ( )  GEOMETRIC_REPRESENTATION_ITEM ( )  RATIONAL_B_SPLINE_CURVE ( ( 1.000000000000000000, 0.9931515681023461717, 0.9931515681023461717, 1.000000000000000000 ) ) 
 REPRESENTATION_ITEM ( '' )  );
#101504=CARTESIAN_POINT ( 'NONE',  ( -0.3973293944376590225, 1418.672797618759887, 184.7148006323309914 ) ) ;
#101509=CARTESIAN_POINT ( 'NONE',  ( -11.76598840989999850, 1428.979790717830156, 145.3128034382980047 ) ) ;
#101513=CARTESIAN_POINT ( 'NONE',  ( 20.69641686248409940, 1508.889931363489723, 228.4591762237180035 ) ) ;
#101515=VERTEX_POINT ( 'NONE', #48667 ) ;
#101516=VERTEX_POINT ( 'NONE', #109118 ) ;
#101517=CARTESIAN_POINT ( 'NONE',  ( 12.04255032705700046, 1433.784197904049961, 149.9177363570349826 ) ) ;
#101518=CARTESIAN_POINT ( 'NONE',  ( 9.147507710520001797E-12, 1395.913060387330006, 220.1216245146979986 ) ) ;
#101519=ORIENTED_EDGE ( 'NONE', *, *, #52162, .F. ) ;
#101521=CARTESIAN_POINT ( 'NONE',  ( -25.58986275070000005, 1507.958108862429981, 199.5218862797180179 ) ) ;
#101525=CARTESIAN_POINT ( 'NONE',  ( 6.598247897499999404, 1507.806513241529956, 235.4227652625980056 ) ) ;
#101526=EDGE_CURVE ( 'NONE', #46649, #6784, #15429, .T. ) ;
#101527=CARTESIAN_POINT ( 'NONE',  ( 6.332098049610000778, 1449.232071652019840, 185.0551591760979875 ) ) ;
#101528=CARTESIAN_POINT ( 'NONE',  ( -2.845602367250000153, 1416.216739748630062, 191.3599216423980067 ) ) ;
#101529=CARTESIAN_POINT ( 'NONE',  ( 43.48865799104739693, 1440.913053441320244, 270.3367078669490411 ) ) ;
#101530=CARTESIAN_POINT ( 'NONE',  ( 3.824658609203980042, 1396.046620409630123, 198.7789396447920183 ) ) ;
#101531=CARTESIAN_POINT ( 'NONE',  ( 2.500000000000000000, 1419.466030184288229, 140.1627189556986650 ) ) ;
#101532=CARTESIAN_POINT ( 'NONE',  ( 11.86482925309999992, 1432.250691705679856, 150.3967422869979771 ) ) ;
#101535=CARTESIAN_POINT ( 'NONE',  ( 13.30447859826429990, 1435.414542389009966, 150.2505690479650013 ) ) ;
#101536=EDGE_CURVE ( 'NONE', #34381, #48449, #69575, .T. ) ;
#101537=ORIENTED_EDGE ( 'NONE', *, *, #31306, .F. ) ;
#101538=ORIENTED_EDGE ( 'NONE', *, *, #12621, .F. ) ;
#101540=CARTESIAN_POINT ( 'NONE',  ( -9.295549619430000021, 1464.969213748930088, 232.6937024852979903 ) ) ;
#101546=CARTESIAN_POINT ( 'NONE',  ( 13.75903321446010175, 1409.893113914890137, 191.3057351114860296 ) ) ;
#101550=EDGE_LOOP ( 'NONE', ( #103284, #74544, #98960, #37309 ) ) ;
#101551=CARTESIAN_POINT ( 'NONE',  ( 20.46181040842379772, 1440.913060387330006, 219.2827885314970331 ) ) ;
#101553=EDGE_CURVE ( 'NONE', #79447, #3400, #107023, .T. ) ;
#101554=CARTESIAN_POINT ( 'NONE',  ( -12.77781222480000167, 1409.526058053829956, 190.2114732551980296 ) ) ;
#101557=CARTESIAN_POINT ( 'NONE',  ( 0.08492873675443529669, 1416.830086716310007, 227.2254341622459890 ) ) ;
#101559=CARTESIAN_POINT ( 'NONE',  ( 24.19987966749999941, 1436.809810026820060, 213.5205588716879959 ) ) ;
#101564=ADVANCED_FACE ( 'NONE', ( #15016 ), #67782, .F. ) ;
#101565=B_SPLINE_CURVE_WITH_KNOTS ( 'NONE', 5,
 ( #15262, #40483, #48355, #56747, #108238, #66273, #6874, #31526, #82495, #48914, #65704, #23116 ),
 .UNSPECIFIED., .F., .F.,
 ( 6, 3, 3, 6 ),
 ( 0.000000000000000000, 0.5248584659502879557, 0.7624265191794091789, 1.000000000000000000 ),
 .UNSPECIFIED. ) ;
#101570=CARTESIAN_POINT ( 'NONE',  ( -21.73076286450000083, 1509.627908364130008, 189.8044754037979942 ) ) ;
#101574=CARTESIAN_POINT ( 'NONE',  ( -2.684328089744040469, 1448.124395745682250, 154.7387311340914948 ) ) ;
#101575=CARTESIAN_POINT ( 'NONE',  ( 13.39865760989999899, 1409.380951821229928, 192.5599167449979916 ) ) ;
#101576=DIRECTION ( 'NONE',  ( -0.4530882417517332339, -0.7475172582769017415, -0.4857252245503692611 ) ) ;
#101580=B_SPLINE_CURVE_WITH_KNOTS ( 'NONE', 5,
 ( #99511, #72696, #97866, #81074, #56441, #29568, #4390, #80541, #46408, #3856, #63752, #21141 ),
 .UNSPECIFIED., .F., .F.,
 ( 6, 3, 3, 6 ),
 ( 0.000000000000000000, 0.3427427782409787627, 0.7510084151527882668, 1.000000000000000000 ),
 .UNSPECIFIED. ) ;
#101581=CARTESIAN_POINT ( 'NONE',  ( 34.21460434910000004, 1445.299194187479998, 250.0133502167980453 ) ) ;
#101584=EDGE_CURVE ( 'NONE', #102960, #12156, #51647, .T. ) ;
#101595=CARTESIAN_POINT ( 'NONE',  ( 0.3804419299169999880, 1497.014155752930037, 230.6889103195979942 ) ) ;
#101596=CARTESIAN_POINT ( 'NONE',  ( 12.87903121499999948, 1419.807609159930053, 223.0107373717980010 ) ) ;
#101598=ADVANCED_FACE ( 'NONE', ( #110197 ), #58819, .F. ) ;
#101601=CARTESIAN_POINT ( 'NONE',  ( 5.615853708540889500, 1416.377937261669103, 231.4220595556466264 ) ) ;
#101602=CARTESIAN_POINT ( 'NONE',  ( 32.02225460880060126, 1435.615636428170092, 135.5615768203190044 ) ) ;
#101603=CARTESIAN_POINT ( 'NONE',  ( 37.96685885719930553, 1448.851682310969863, 136.3764525557429863 ) ) ;
#101606=CARTESIAN_POINT ( 'NONE',  ( 8.309202182009999049, 1507.619014552029967, 183.0708173328979740 ) ) ;
#101608=CARTESIAN_POINT ( 'NONE',  ( -40.03500165408544120, 1450.467487820260430, 269.6105336665062282 ) ) ;
#101611=CARTESIAN_POINT ( 'NONE',  ( -42.04495720335383169, 1427.613817688321205, 269.0745714257215013 ) ) ;
#101612=CARTESIAN_POINT ( 'NONE',  ( 14.22586472836579929, 1422.194230000339758, 190.7685836825260139 ) ) ;
#101613=CARTESIAN_POINT ( 'NONE',  ( -0.3842696321549999849, 1415.775732286429957, 233.4299280523979974 ) ) ;
#101615=CARTESIAN_POINT ( 'NONE',  ( -28.47876014660000266, 1509.161042325230028, 208.9577188500109912 ) ) ;
#101619=CARTESIAN_POINT ( 'NONE',  ( -7.854791674351897512, 1451.394299795975940, 152.9879781448754841 ) ) ;
#101620=CARTESIAN_POINT ( 'NONE',  ( -16.20819593131889746, 1414.913060387399810, 208.4856282769769962 ) ) ;
#101621=CARTESIAN_POINT ( 'NONE',  ( 25.38824507410000209, 1436.314429228820245, 137.2293497432980018 ) ) ;
#101624=CARTESIAN_POINT ( 'NONE',  ( 1.003994675819599891, 1414.971993471370070, 191.9916610432980235 ) ) ;
#101625=CARTESIAN_POINT ( 'NONE',  ( -5.984203303400000173, 1409.122033371430007, 229.9503900095979816 ) ) ;
#101626=ORIENTED_EDGE ( 'NONE', *, *, #15225, .F. ) ;
#101631=CARTESIAN_POINT ( 'NONE',  ( -7.245608758899999557, 1458.975067297229998, 211.8132954410479840 ) ) ;
#101633=CARTESIAN_POINT ( 'NONE',  ( 4.144234488730229593, 1424.436899653439923, 184.8007390397289953 ) ) ;
#101635=CARTESIAN_POINT ( 'NONE',  ( -2.813926873014771068, 1419.840084512981548, 186.1457758105879634 ) ) ;
#101638=CARTESIAN_POINT ( 'NONE',  ( -24.09223960049999747, 1438.023760012700222, 211.8323666990379763 ) ) ;
#101640=CARTESIAN_POINT ( 'NONE',  ( 2.489956268369999837, 1451.499402758130145, 183.7031856439980118 ) ) ;
#101643=CARTESIAN_POINT ( 'NONE',  ( -20.59181392461939808, 1509.749895152629961, 230.9387993182432126 ) ) ;
#101645=ORIENTED_EDGE ( 'NONE', *, *, #39138, .F. ) ;
#101646=ORIENTED_EDGE ( 'NONE', *, *, #48750, .T. ) ;
#101647=CARTESIAN_POINT ( 'NONE',  ( -11.76350460807940124, 1426.962723605229939, 145.9979234665020158 ) ) ;
#101648=AXIS2_PLACEMENT_3D ( 'NONE', #40450, #49424, #66789 ) ;
#101650=CARTESIAN_POINT ( 'NONE',  ( -3.530738011219999528, 1473.488020316229949, 270.3906828180979574 ) ) ;
#101653=CARTESIAN_POINT ( 'NONE',  ( 22.58439900540000167, 1519.913060387329779, 209.1218459616979999 ) ) ;
#101656=CARTESIAN_POINT ( 'NONE',  ( -18.71266994490000002, 1408.913060387329779, 208.1472103593870031 ) ) ;
#101657=B_SPLINE_CURVE_WITH_KNOTS ( 'NONE', 3,
 ( #19344, #20445, #78726, #53544, #96635, #28322 ),
 .UNSPECIFIED., .F., .F.,
 ( 4, 2, 4 ),
 ( -6.000000023196556560E-08, 0.0005507591112004208908, 0.001101578222401073878 ),
 .UNSPECIFIED. ) ;
#101660=CARTESIAN_POINT ( 'NONE',  ( -10.53083746087449946, 1407.392537625429895, 269.4602285795690477 ) ) ;
#101661=CARTESIAN_POINT ( 'NONE',  ( -13.23941283839999983, 1435.104810100029908, 149.9220718869979976 ) ) ;
#101662=ORIENTED_EDGE ( 'NONE', *, *, #108912, .T. ) ;
#101664=CARTESIAN_POINT ( 'NONE',  ( 13.99038557849999975, 1444.015975867750058, 189.3175554311980022 ) ) ;
#101665=ORIENTED_EDGE ( 'NONE', *, *, #30216, .F. ) ;
#101667=CARTESIAN_POINT ( 'NONE',  ( 4.902054967530699692, 1422.428228210868156, 184.3467753365531507 ) ) ;
#101674=ORIENTED_EDGE ( 'NONE', *, *, #103611, .T. ) ;
#101676=( BOUNDED_CURVE ( )  B_SPLINE_CURVE ( 3, ( #47983, #67000, #13797, #56943 ),
 .UNSPECIFIED., .F., .F. ) 
 B_SPLINE_CURVE_WITH_KNOTS ( ( 4, 4 ),
 ( 1.036132151715712713, 2.105460582192766772 ),
 .UNSPECIFIED. ) 
 CURVE ( )  GEOMETRIC_REPRESENTATION_ITEM ( )  RATIONAL_B_SPLINE_CURVE ( ( 1.000000000000000000, 0.9069598517500692125, 0.9069598517500692125, 1.000000000000000000 ) ) 
 REPRESENTATION_ITEM ( '' )  );
#101678=ADVANCED_FACE ( 'NONE', ( #68782 ), #108851, .F. ) ;
#101679=CARTESIAN_POINT ( 'NONE',  ( -27.50534346099999894, 1509.159577300329829, 204.1676302040880273 ) ) ;
#101681=CARTESIAN_POINT ( 'NONE',  ( -1.328495774590000122, 1467.878694257229881, 230.3318996346980043 ) ) ;
#101683=CARTESIAN_POINT ( 'NONE',  ( -2.751920914360000303, 1408.825585090129834, 195.2201059653979769 ) ) ;
#101685=CARTESIAN_POINT ( 'NONE',  ( 15.45308517192525599, 1506.474306125858902, 193.4392981697745029 ) ) ;
#101688=CARTESIAN_POINT ( 'NONE',  ( 26.99303384979999976, 1488.687911583929917, 211.6160553286979962 ) ) ;
#101692=CARTESIAN_POINT ( 'NONE',  ( -24.66052414600000020, 1442.238365636329945, 210.7405400769080188 ) ) ;
#101697=CARTESIAN_POINT ( 'NONE',  ( -15.20812112729999832, 1415.576510420729846, 226.8726329618980060 ) ) ;
#101698=CARTESIAN_POINT ( 'NONE',  ( 18.80339027203730140, 1425.953307585449693, 225.0197318394450008 ) ) ;
#101701=CARTESIAN_POINT ( 'NONE',  ( 33.91376666158910069, 1435.681799711289841, 142.5056097149810057 ) ) ;
#101707=CARTESIAN_POINT ( 'NONE',  ( -22.72723102240144044, 1509.727045134374066, 228.1120738395736964 ) ) ;
#101708=B_SPLINE_SURFACE_WITH_KNOTS ( 'NONE', 5, 5, ( 
 ( #104412, #85957, #69741, #34450, #45088, #103282, #103860, #28255, #104966, #94336, #27705, #87625 ),
 ( #44517, #78104, #26589, #54049, #88175, #62448, #68626, #102728, #1405, #27161, #9257, #53481 ),
 ( #43416, #77566, #872, #69176, #9796, #35546, #94912, #51817, #36116, #60786, #18186, #78663 ),
 ( #52924, #61345, #87058, #86502, #10913, #95465, #79228, #19279, #34996, #10345, #1981, #77019 ),
 ( #61892, #96008, #2537, #36661, #70855, #96571, #19844, #325, #73442, #31969, #58288, #90208 ),
 ( #14051, #20388, #97119, #81811, #71411, #105526, #22432, #63013, #56083, #40919, #79782, #13492 ),
 ( #74546, #65594, #28815, #92413, #15148, #47683, #48240, #23562, #3087, #24099, #14613, #37215 ),
 ( #5113, #48800, #82923, #40365, #108118, #73988, #30862, #6214, #49337, #39269, #31412, #109247 ),
 ( #107576, #65037, #99154, #6759, #66161, #56635, #90770, #82383, #108678, #100282, #99707, #57756 ),
 ( #5682, #39826, #91875, #23000, #100811, #83464, #57204, #45642, #91328, #75099, #32531, #66702 ),
 ( #17902, #52099, #34175, #1149, #42033, #8969, #67254, #59957, #103016, #25201, #26312, #7324 ),
 ( #101348, #50449, #43141, #41488, #103583, #75648, #86229, #35280, #50991, #9520, #85120, #26885 ) ),
 .UNSPECIFIED., .F., .F., .F.,
 ( 6, 3, 3, 6 ),
 ( 6, 3, 3, 6 ),
 ( 6.265790646049559598, 6.759971547659999302, 7.748257017729999419, 8.343532910357360777 ),
 ( -4.426502619661019944E-05, 0.3262962046579999664, 0.9788886139739999548, 1.447530370220490026 ),
 .UNSPECIFIED. ) ;
#101709=CARTESIAN_POINT ( 'NONE',  ( 10.11876717485079880, 1468.998983517520173, 232.5874711531799903 ) ) ;
#101712=B_SPLINE_CURVE_WITH_KNOTS ( 'NONE', 3,
 ( #7241, #22351, #100196, #57671, #82292, #56552, #48157, #5592, #68283, #77218, #104054, #76647, #8327, #95109, #18374, #1620, #1069, #35197, #76103, #9445, #17258 ),
 .UNSPECIFIED., .F., .F.,
 ( 4, 2, 2, 2, 1, 1, 1, 1, 1, 2, 2, 2, 4 ),
 ( 0.000000000000000000, 0.2499999999997003508, 0.3749999999995501931, 0.4374999999994747535, 0.4687499999994392819, 0.4843749999994212962, 0.4921874999994121369, 0.4960937499994074740, 0.4980468749994027000, 0.4990234374994019229, 0.4999999999994011457, 0.7499999999997005729, 1.000000000000000000 ),
 .UNSPECIFIED. ) ;
#101715=CARTESIAN_POINT ( 'NONE',  ( 4.225886903421089968, 1441.568770927039850, 166.1380412392189783 ) ) ;
#101718=AXIS2_PLACEMENT_3D ( 'NONE', #49233, #37328, #12114 ) ;
#101721=ORIENTED_EDGE ( 'NONE', *, *, #9062, .T. ) ;
#101722=CARTESIAN_POINT ( 'NONE',  ( -12.27010798569999928, 1416.835808384130132, 194.6641343254979972 ) ) ;
#101723=B_SPLINE_SURFACE_WITH_KNOTS ( 'NONE', 5, 5, ( 
 ( #21505, #56247, #55719, #90376, #55167, #90938 ),
 ( #38873, #38327, #72506, #73052, #107193, #81977 ),
 ( #64670, #5849, #99324, #13654, #47844, #105556 ),
 ( #5285, #39441, #16411, #8034, #108846, #40539 ),
 ( #24277, #108296, #75806, #110503, #91502, #7489 ),
 ( #92048, #50605, #6934, #49514, #85284, #41091 ) ),
 .UNSPECIFIED., .F., .F., .F.,
 ( 6, 6 ),
 ( 6, 6 ),
 ( 7.053188784610000539, 25.42450307460000047 ),
 ( 0.000000000000000000, 2.000000000000000000 ),
 .UNSPECIFIED. ) ;
#101729=AXIS2_PLACEMENT_3D ( 'NONE', #59353, #17286, #59900 ) ;
#101731=EDGE_CURVE ( 'NONE', #102747, #66886, #4827, .T. ) ;
#101733=CARTESIAN_POINT ( 'NONE',  ( -1.804213505890000180, 1410.351307731129964, 186.0507930254979954 ) ) ;
#101735=CARTESIAN_POINT ( 'NONE',  ( -23.61227025210000008, 1435.322036687620084, 137.2858276859979867 ) ) ;
#101736=CARTESIAN_POINT ( 'NONE',  ( 18.90690566160000330, 1416.819756528429934, 210.0263056463570024 ) ) ;
#101739=CARTESIAN_POINT ( 'NONE',  ( -4.967309476820000569, 1440.444625599219989, 150.3089546883979892 ) ) ;
#101740=CARTESIAN_POINT ( 'NONE',  ( 41.26114072546569389, 1440.913060355679818, 261.0027848306349938 ) ) ;
#101742=FACE_OUTER_BOUND ( 'NONE', #87255, .T. ) ;
#101743=CARTESIAN_POINT ( 'NONE',  ( 13.24083268210000064, 1429.096486322929877, 222.2418765336980186 ) ) ;
#101745=VERTEX_POINT ( 'NONE', #44676 ) ;
#101746=CARTESIAN_POINT ( 'NONE',  ( 1.547740551532809983, 1416.449138223310001, 190.2779371676239748 ) ) ;
#101747=CARTESIAN_POINT ( 'NONE',  ( -19.66414603918734727, 1485.273356660164609, 190.3047461115721433 ) ) ;
#101748=CARTESIAN_POINT ( 'NONE',  ( -27.89933041909999645, 1509.196990922029954, 210.7395031776179906 ) ) ;
#101751=CARTESIAN_POINT ( 'NONE',  ( 26.27087616454108598, 1509.943490157906808, 223.6899730734042748 ) ) ;
#101755=CARTESIAN_POINT ( 'NONE',  ( 20.63450640349999787, 1452.049652659229878, 144.1338810006979827 ) ) ;
#101756=CARTESIAN_POINT ( 'NONE',  ( -28.45107852102471924, 1509.906593941153687, 212.2021872825625621 ) ) ;
#101762=CARTESIAN_POINT ( 'NONE',  ( 19.77969251879999746, 1507.818093401829856, 229.2755605921979907 ) ) ;
#101763=VERTEX_POINT ( 'NONE', #47966 ) ;
#101765=CARTESIAN_POINT ( 'NONE',  ( 16.84231947438349764, 1508.205205765930032, 231.2670381483619906 ) ) ;
#101767=CARTESIAN_POINT ( 'NONE',  ( -15.95383389570000077, 1506.798305147730161, 224.6865364803979901 ) ) ;
#101774=CARTESIAN_POINT ( 'NONE',  ( 3.738841759920000118, 1409.547781092230025, 186.1588687207980115 ) ) ;
#101775=CARTESIAN_POINT ( 'NONE',  ( 12.91074692609340069, 1420.834906917639955, 222.4031488991760170 ) ) ;
#101777=CARTESIAN_POINT ( 'NONE',  ( -2.704923982728260068, 1440.770577247940082, 166.9241038796999987 ) ) ;
#101778=AXIS2_PLACEMENT_3D ( 'NONE', #71216, #45999, #105340 ) ;
#101779=CARTESIAN_POINT ( 'NONE',  ( -2.706741865136000236, 1451.733424401669936, 184.7389962060059929 ) ) ;
#101780=CARTESIAN_POINT ( 'NONE',  ( 0.4595755069420000005, 1467.109512415230029, 235.5974104456980172 ) ) ;
#101781=VERTEX_POINT ( 'NONE', #31703 ) ;
#101784=CARTESIAN_POINT ( 'NONE',  ( 11.60004869885206880, 1428.983126981192754, 137.0999999980979851 ) ) ;
#101786=CARTESIAN_POINT ( 'NONE',  ( 18.89905511659999959, 1416.828040475729949, 210.6687957193779823 ) ) ;
#101788=CIRCLE ( 'NONE', #62532, 1.999998248449969873 ) ;
#101789=CARTESIAN_POINT ( 'NONE',  ( -4.384471102255430024E-11, 1469.871482233950019, 253.6786592827409663 ) ) ;
#101792=CARTESIAN_POINT ( 'NONE',  ( -1.263571840090000009, 1417.414027388429986, 235.3744744869979968 ) ) ;
#101795=CARTESIAN_POINT ( 'NONE',  ( -0.1926505725269009039, 1486.021514730641229, 181.8289695123539786 ) ) ;
#101797=CARTESIAN_POINT ( 'NONE',  ( -45.95009646603779885, 1438.847167528959972, 268.4985374090409778 ) ) ;
#101798=CARTESIAN_POINT ( 'NONE',  ( 13.46016752625740054, 1508.422424633640048, 233.3101797675730040 ) ) ;
#101805=CARTESIAN_POINT ( 'NONE',  ( -26.56969918195860103, 1451.519818403060071, 136.0976908218790129 ) ) ;
#101807=CARTESIAN_POINT ( 'NONE',  ( 7.968534124619999904E-12, 1418.241830526630110, 231.9989422678980304 ) ) ;
#101810=CARTESIAN_POINT ( 'NONE',  ( -2.243003920383240146, 1419.511934557899849, 185.9793846685319920 ) ) ;
#101813=CARTESIAN_POINT ( 'NONE',  ( 2.500000000000000000, 1448.894380913990062, 182.3534011237979939 ) ) ;
#101816=CARTESIAN_POINT ( 'NONE',  ( -0.6031919701292450808, 1409.206624385790064, 270.3713721421309515 ) ) ;
#101817=CARTESIAN_POINT ( 'NONE',  ( 6.346443515254469148, 1418.380699742210254, 232.6272524216070110 ) ) ;
#101819=VERTEX_POINT ( 'NONE', #91056 ) ;
#101822=ORIENTED_EDGE ( 'NONE', *, *, #78971, .T. ) ;
#101823=PLANE ( 'NONE',  #95646 ) ;
#101825=CARTESIAN_POINT ( 'NONE',  ( -2.409586283469999923, 1426.663880916129983, 144.1938086916980239 ) ) ;
#101826=CARTESIAN_POINT ( 'NONE',  ( -18.58858086442659996, 1429.707054241190008, 194.6563974369069854 ) ) ;
#101829=CARTESIAN_POINT ( 'NONE',  ( 36.94315808685519187, 1461.917959960340113, 268.5012768873260143 ) ) ;
#101831=CARTESIAN_POINT ( 'NONE',  ( -17.21301869208722124, 1422.369372973762665, 226.6884971801745792 ) ) ;
#101834=CARTESIAN_POINT ( 'NONE',  ( 18.23897009793844859, 1459.291141722666453, 227.8679119275740561 ) ) ;
#101841=EDGE_CURVE ( 'NONE', #39681, #47741, #26245, .T. ) ;
#101847=CARTESIAN_POINT ( 'NONE',  ( 2.098606530373039902, 1408.986345342219920, 186.9550871089749933 ) ) ;
#101848=CARTESIAN_POINT ( 'NONE',  ( 1.200765764030000238, 1417.120114711829956, 233.8531050740980106 ) ) ;
#101850=DIRECTION ( 'NONE',  ( -7.283063041540821170E-15, 0.9876883405951697448, 0.1564344650400280867 ) ) ;
#101854=CARTESIAN_POINT ( 'NONE',  ( 11.73069774356920014, 1414.913057862230062, 220.5398999955840225 ) ) ;
#101857=B_SPLINE_SURFACE_WITH_KNOTS ( 'NONE', 5, 4, ( 
 ( #92512, #5781, #108775, #5216, #56731 ),
 ( #15247, #65139, #99253, #6318, #39923 ),
 ( #66802, #90868, #14156, #48342, #82481 ),
 ( #31509, #24738, #15779, #49981, #23102 ),
 ( #41015, #91972, #99807, #32069, #67351 ),
 ( #49439, #83561, #40465, #109345, #75194 ) ),
 .UNSPECIFIED., .F., .F., .F.,
 ( 6, 6 ),
 ( 5, 5 ),
 ( -1.139299598668300043E-05, 11.48858425020000062 ),
 ( 25.78146411700000229, 39.23969207129999859 ),
 .UNSPECIFIED. ) ;
#101861=CARTESIAN_POINT ( 'NONE',  ( 13.02322703161950024, 1416.825784015089994, 221.6328457863429833 ) ) ;
#101862=CARTESIAN_POINT ( 'NONE',  ( -6.092217291859999939, 1469.463552789130063, 265.6112252686980355 ) ) ;
#101864=CARTESIAN_POINT ( 'NONE',  ( -21.47555121375469867, 1509.121809597113042, 191.7875346140812951 ) ) ;
#101865=CARTESIAN_POINT ( 'NONE',  ( 11.87331171179999956, 1433.127290053990009, 150.2013614949980251 ) ) ;
#101866=CARTESIAN_POINT ( 'NONE',  ( 8.800012970690000103, 1452.709869713229864, 209.1218459616979999 ) ) ;
#101867=B_SPLINE_SURFACE_WITH_KNOTS ( 'NONE', 5, 5, ( 
 ( #28290, #34484, #95493, #102759, #68659, #902, #27736, #78699, #357 ),
 ( #61926, #79261, #96606, #26055, #2012, #96043, #62486, #44550, #9285 ),
 ( #35028, #61374, #18761, #53515, #8714, #94945, #77596, #19875, #85987 ),
 ( #87092, #85415, #77051, #60250, #36148, #94367, #17649, #69207, #10947 ),
 ( #10377, #52958, #18214, #43447, #70332, #103316, #52410, #42893, #26624 ),
 ( #86535, #60820, #19314, #87658, #9829, #103892, #104444, #45119, #43998 ),
 ( #2571, #36693, #78133, #1436, #35582, #69774, #70887, #27191, #105001 ),
 ( #45883, #105787, #44783, #78933, #55381, #11178, #63787, #87887, #106318 ),
 ( #12804, #64337, #54835, #46984, #29070, #80020, #80572, #72729, #96269 ) ),
 .UNSPECIFIED., .F., .F., .F.,
 ( 6, 3, 6 ),
 ( 6, 3, 6 ),
 ( 22.40717020724860120, 46.28443321930000565, 74.85727727459999414 ),
 ( 0.000000000000000000, 1.000000000000000000, 2.000000000000000000 ),
 .UNSPECIFIED. ) ;
#101870=CIRCLE ( 'NONE', #10712, 1.999999954393705037 ) ;
#101874=CARTESIAN_POINT ( 'NONE',  ( -29.72561318641060168, 1509.951099604490082, 208.7905312278460030 ) ) ;
#101879=CARTESIAN_POINT ( 'NONE',  ( -39.99258969340072412, 1438.670160836478544, 135.1922399653822708 ) ) ;
#101885=CARTESIAN_POINT ( 'NONE',  ( 0.1979593984663390038, 1464.158265199940161, 182.7746200214319856 ) ) ;
#101886=CARTESIAN_POINT ( 'NONE',  ( -3.911218387651921979, 1414.913060387329779, 193.3684778321149622 ) ) ;
#101888=CARTESIAN_POINT ( 'NONE',  ( -13.76936860679999874, 1443.913060387329097, 176.3340081878980641 ) ) ;
#101890=CARTESIAN_POINT ( 'NONE',  ( 12.06084908070000061, 1433.903750942899933, 149.8851033673979884 ) ) ;
#101891=CARTESIAN_POINT ( 'NONE',  ( -40.38917806203690475, 1448.047423120109897, 134.0999999983369833 ) ) ;
#101892=CARTESIAN_POINT ( 'NONE',  ( -36.02435062347289829, 1445.276583446800032, 137.0631246289250100 ) ) ;
#101893=EDGE_LOOP ( 'NONE', ( #52020, #28856, #53059, #44557, #35682 ) ) ;
#101895=CARTESIAN_POINT ( 'NONE',  ( -2.793439186891359949, 1486.025328193850100, 182.0741020391329812 ) ) ;
#101896=CARTESIAN_POINT ( 'NONE',  ( -17.37509865559999866, 1416.823418193129783, 214.4574835448779879 ) ) ;
#101900=AXIS2_PLACEMENT_3D ( 'NONE', #61214, #79649, #52240 ) ;
#101903=CARTESIAN_POINT ( 'NONE',  ( 3.902542241760000419, 1426.015650185330060, 185.2953857086980065 ) ) ;
#101908=CARTESIAN_POINT ( 'NONE',  ( -28.55764294989999996, 1451.460584126430149, 136.1042256204979708 ) ) ;
#101909=CARTESIAN_POINT ( 'NONE',  ( 13.51702042466233600, 1443.501467202829645, 169.3754641244197217 ) ) ;
#101921=CARTESIAN_POINT ( 'NONE',  ( 42.06232107555830169, 1440.913060387330006, 269.6487541170399709 ) ) ;
#101924=CARTESIAN_POINT ( 'NONE',  ( 16.25240189476375008, 1432.151868409839153, 218.3259014903973991 ) ) ;
#101925=CARTESIAN_POINT ( 'NONE',  ( 1.450664468150000053, 1415.792771685530170, 232.7840273826980138 ) ) ;
#101928=CARTESIAN_POINT ( 'NONE',  ( 21.75648121771956411, 1509.708962386752546, 188.8810923022467705 ) ) ;
#101931=CARTESIAN_POINT ( 'NONE',  ( 2.499999989320000005, 1447.977245594400074, 159.5593905798980074 ) ) ;
#101932=CARTESIAN_POINT ( 'NONE',  ( -2.500000000000000000, 1436.180951016360041, 157.6151257071979899 ) ) ;
#101936=CARTESIAN_POINT ( 'NONE',  ( 40.71279077584669892, 1444.187195803030136, 137.0114455636829973 ) ) ;
#101939=CARTESIAN_POINT ( 'NONE',  ( -23.99427320719999912, 1410.919622273529967, 208.2638409563230084 ) ) ;
#101940=CARTESIAN_POINT ( 'NONE',  ( -11.19545718725239958, 1426.041279750870217, 113.0052507005540008 ) ) ;
#101941=CARTESIAN_POINT ( 'NONE',  ( 15.86112125244039817, 1410.431337872899803, 191.5898895329879963 ) ) ;
#101943=CARTESIAN_POINT ( 'NONE',  ( 18.34728769450661900, 1509.673048444232336, 185.3862757340986320 ) ) ;
#101945=CARTESIAN_POINT ( 'NONE',  ( 2.292469552788555465, 1449.805609130731227, 182.1508050511279180 ) ) ;
#101946=B_SPLINE_SURFACE_WITH_KNOTS ( 'NONE', 3, 5, ( 
 ( #103558, #77819, #53758, #61587, #52076, #28517 ),
 ( #576, #10054, #9502, #36911, #44228, #2791 ),
 ( #85646, #62148, #102996, #1128, #95720, #71106 ),
 ( #105230, #62718, #18985, #94601, #95172, #20106 ) ),
 .UNSPECIFIED., .F., .F., .F.,
 ( 4, 4 ),
 ( 6, 6 ),
 ( 5.479555871570000569, 5.505626611620000332 ),
 ( 0.000000000000000000, 1.000000000000000000 ),
 .UNSPECIFIED. ) ;
#101952=CARTESIAN_POINT ( 'NONE',  ( -34.59119253931500282, 1437.071637960610133, 136.5445694851690064 ) ) ;
#101953=EDGE_LOOP ( 'NONE', ( #98008, #49823, #5276, #2015 ) ) ;
#101954=CARTESIAN_POINT ( 'NONE',  ( 13.41275991522839917, 1396.898936538649878, 207.0368130037109893 ) ) ;
#101957=CARTESIAN_POINT ( 'NONE',  ( -19.00906408819999882, 1456.707065538329971, 228.7066581731980079 ) ) ;
#101958=ORIENTED_EDGE ( 'NONE', *, *, #94010, .T. ) ;
#101960=CARTESIAN_POINT ( 'NONE',  ( -11.99447448239999936, 1410.787978745530154, 219.9627945351979861 ) ) ;
#101967=CARTESIAN_POINT ( 'NONE',  ( -13.04207679966010147, 1409.368499744919745, 225.9431846064669855 ) ) ;
#101969=CARTESIAN_POINT ( 'NONE',  ( 27.07184576870000114, 1440.506430296650024, 137.2141704726979867 ) ) ;
#101975=ORIENTED_EDGE ( 'NONE', *, *, #63596, .T. ) ;
#101979=EDGE_LOOP ( 'NONE', ( #25281, #23199, #78121, #89034 ) ) ;
#101980=CARTESIAN_POINT ( 'NONE',  ( -14.23393746390000025, 1416.021639799829927, 221.4291795454980161 ) ) ;
#101985=CARTESIAN_POINT ( 'NONE',  ( -4.540052047909999722, 1423.807313613229780, 184.6930058418980138 ) ) ;
#101986=CARTESIAN_POINT ( 'NONE',  ( -9.775296951400726186, 1446.595182981042853, 153.4780497659124023 ) ) ;
#101990=CARTESIAN_POINT ( 'NONE',  ( -16.81933045710000130, 1496.363585094529981, 224.0712623398979986 ) ) ;
#101991=CARTESIAN_POINT ( 'NONE',  ( 17.60692135329999886, 1458.113405358530144, 229.3981720485979849 ) ) ;
#101993=CARTESIAN_POINT ( 'NONE',  ( -4.859690594346670167, 1423.466502886267790, 184.6308178099481552 ) ) ;
#101995=CARTESIAN_POINT ( 'NONE',  ( -5.360127758099149986, 1422.242654706269832, 144.1589408359039908 ) ) ;
#101997=CARTESIAN_POINT ( 'NONE',  ( 18.24652371554340036, 1424.504995576649890, 223.7081814311490007 ) ) ;
#101999=CARTESIAN_POINT ( 'NONE',  ( -2.896892187767880156, 1484.263391075600111, 183.3160938869699805 ) ) ;
#102000=CARTESIAN_POINT ( 'NONE',  ( -17.19449298599652920, 1410.877585917538909, 192.1747057623898911 ) ) ;
#102003=CARTESIAN_POINT ( 'NONE',  ( 0.5790313230850000492, 1453.165958254130146, 188.8726570487980041 ) ) ;
#102006=CARTESIAN_POINT ( 'NONE',  ( -11.82677958210000035, 1429.701853304430188, 149.3212236813980098 ) ) ;
#102009=LINE ( 'NONE', #17437, #27152 ) ;
#102012=ADVANCED_FACE ( 'NONE', ( #81358 ), #18633, .F. ) ;
#102013=CARTESIAN_POINT ( 'NONE',  ( -19.82812931440000170, 1470.089036833630189, 226.5638250403980010 ) ) ;
#102018=CARTESIAN_POINT ( 'NONE',  ( 21.98324444889999896, 1409.895860934730081, 267.6462823665979727 ) ) ;
#102020=CARTESIAN_POINT ( 'NONE',  ( 21.11335034690000256, 1449.726224339279952, 195.7155535830980000 ) ) ;
#102021=CARTESIAN_POINT ( 'NONE',  ( 0.06596416509929559080, 1508.967883553199954, 238.8759510148510117 ) ) ;
#102024=CARTESIAN_POINT ( 'NONE',  ( -40.67152590493699904, 1442.641813676910033, 136.9878664284970000 ) ) ;
#102025=DIRECTION ( 'NONE',  ( 0.000000000000000000, 0.000000000000000000, 1.000000000000000000 ) ) ;
#102028=CARTESIAN_POINT ( 'NONE',  ( -12.97256195459999795, 1446.865982279580066, 187.9439210766980182 ) ) ;
#102032=ORIENTED_EDGE ( 'NONE', *, *, #52198, .F. ) ;
#102034=CARTESIAN_POINT ( 'NONE',  ( -11.30426874151759975, 1409.307814150319928, 199.3369101544629700 ) ) ;
#102037=CARTESIAN_POINT ( 'NONE',  ( -14.57658230699999891, 1474.036347059630089, 268.9619602272979932 ) ) ;
#102040=CARTESIAN_POINT ( 'NONE',  ( -24.11238158259271813, 1444.454182330793856, 211.7733111310209608 ) ) ;
#102044=CARTESIAN_POINT ( 'NONE',  ( 11.23669755143010107, 1415.007830321379970, 222.5597074813329925 ) ) ;
#102045=CARTESIAN_POINT ( 'NONE',  ( 0.8265244082521410185, 1408.941923255679967, 231.1644249228330068 ) ) ;
#102049=EDGE_CURVE ( 'NONE', #12260, #73043, #28844, .T. ) ;
#102050=CARTESIAN_POINT ( 'NONE',  ( -22.42121221859999736, 1409.696026370929985, 207.7819003571480039 ) ) ;
#102051=EDGE_CURVE ( 'NONE', #89942, #8151, #84935, .T. ) ;
#102057=CARTESIAN_POINT ( 'NONE',  ( -1.247677516857949989E-10, 1452.913060387320002, 152.5211338456990120 ) ) ;
#102061=CARTESIAN_POINT ( 'NONE',  ( -11.73709356449999852, 1426.695943566229971, 144.1748013794979784 ) ) ;
#102063=VECTOR ( 'NONE', #6609, 1000.000000000000000 ) ;
#102065=CARTESIAN_POINT ( 'NONE',  ( 11.73275740876320050, 1426.698660301100062, 143.8638901049260141 ) ) ;
#102069=LINE ( 'NONE', #76334, #34120 ) ;
#102072=CARTESIAN_POINT ( 'NONE',  ( -3.187512671122507690, 1398.008355567684930, 221.7452893070936568 ) ) ;
#102073=FACE_OUTER_BOUND ( 'NONE', #5583, .T. ) ;
#102075=DIRECTION ( 'NONE',  ( 0.000000000000000000, -1.000000000000000000, 0.000000000000000000 ) ) ;
#102076=CARTESIAN_POINT ( 'NONE',  ( 20.82852640818889967, 1508.920542461920149, 228.0213171461830086 ) ) ;
#102078=ORIENTED_EDGE ( 'NONE', *, *, #90530, .F. ) ;
#102080=CARTESIAN_POINT ( 'NONE',  ( 11.94112542547770062, 1433.728687859460024, 150.4558864976919779 ) ) ;
#102081=CARTESIAN_POINT ( 'NONE',  ( -9.622035674789998438, 1396.249069277030003, 215.8735477280980035 ) ) ;
#102082=ORIENTED_EDGE ( 'NONE', *, *, #71721, .F. ) ;
#102086=CARTESIAN_POINT ( 'NONE',  ( -13.90334061950993139, 1519.913060387329779, 183.6719516668990480 ) ) ;
#102089=ADVANCED_FACE ( 'NONE', ( #58872 ), #7849, .T. ) ;
#102090=CIRCLE ( 'NONE', #19842, 39.03564169359999170 ) ;
#102091=CARTESIAN_POINT ( 'NONE',  ( 3.174524293809999786, 1468.704260245830028, 183.1758726002980211 ) ) ;
#102093=CARTESIAN_POINT ( 'NONE',  ( 16.31544538450000204, 1410.855193277729995, 226.7200764645979802 ) ) ;
#102095=CARTESIAN_POINT ( 'NONE',  ( 4.319575047684679703, 1396.063903275030043, 198.9757873032580164 ) ) ;
#102096=ADVANCED_FACE ( 'NONE', ( #11233 ), #87942, .F. ) ;
#102097=CARTESIAN_POINT ( 'NONE',  ( 13.59781065039149972, 1415.089996094040089, 197.7253638271529894 ) ) ;
#102098=CARTESIAN_POINT ( 'NONE',  ( 11.85528857480000120, 1431.583028049670020, 149.9311469192980155 ) ) ;
#102101=VERTEX_POINT ( 'NONE', #61641 ) ;
#102102=CARTESIAN_POINT ( 'NONE',  ( 13.02703478251429914, 1435.306670126899917, 150.3834776061850107 ) ) ;
#102106=CARTESIAN_POINT ( 'NONE',  ( 13.31747089092944769, 1444.561669151125898, 169.3769345727364737 ) ) ;
#102107=CARTESIAN_POINT ( 'NONE',  ( -6.617277180400000347, 1464.914593472730076, 234.0919820975980201 ) ) ;
#102112=CARTESIAN_POINT ( 'NONE',  ( -4.115857443736018695, 1425.929640604822680, 186.1083528362279651 ) ) ;
#102117=ORIENTED_EDGE ( 'NONE', *, *, #109055, .T. ) ;
#102118=CARTESIAN_POINT ( 'NONE',  ( 20.20849196857150432, 1440.913060387330006, 217.7572800574920109 ) ) ;
#102119=CARTESIAN_POINT ( 'NONE',  ( -19.26469919840000244, 1508.010672792329842, 229.6096138898979859 ) ) ;
#102120=CARTESIAN_POINT ( 'NONE',  ( -9.192816412500000922, 1410.609185766430073, 188.0952304701980040 ) ) ;
#102122=CARTESIAN_POINT ( 'NONE',  ( 0.1744917581285969910, 1415.933499560010205, 226.9784926752139995 ) ) ;
#102123=ORIENTED_EDGE ( 'NONE', *, *, #95986, .F. ) ;
#102124=CARTESIAN_POINT ( 'NONE',  ( 24.43147358619999565, 1438.163733812159990, 212.9042240985579895 ) ) ;
#102127=CARTESIAN_POINT ( 'NONE',  ( 10.96946812545280103, 1432.347663862999980, 151.7701354189910035 ) ) ;
#102132=CARTESIAN_POINT ( 'NONE',  ( -21.52112661409999816, 1509.604705971930116, 189.3622936410980060 ) ) ;
#102136=EDGE_CURVE ( 'NONE', #4089, #9923, #26605, .T. ) ;
#102137=CARTESIAN_POINT ( 'NONE',  ( 13.30361809040000054, 1409.377632970929881, 191.9462305274980167 ) ) ;
#102138=CARTESIAN_POINT ( 'NONE',  ( -13.08655243744227370, 1486.036966649576243, 185.2250414900032922 ) ) ;
#102142=CARTESIAN_POINT ( 'NONE',  ( 43.50124905439999878, 1443.586705889949826, 263.8967010718980077 ) ) ;
#102143=CARTESIAN_POINT ( 'NONE',  ( -26.94471178607729911, 1509.853990456620068, 220.7433800216579982 ) ) ;
#102144=CARTESIAN_POINT ( 'NONE',  ( -3.755850673020599828, 1508.470365865729946, 237.1708643925190074 ) ) ;
#102145=CARTESIAN_POINT ( 'NONE',  ( -24.04659120089999647, 1444.796772349789762, 212.0316830079879935 ) ) ;
#102146=CARTESIAN_POINT ( 'NONE',  ( 27.69925877688100258, 1441.434395746940027, 137.3015763641899980 ) ) ;
#102147=EDGE_CURVE ( 'NONE', #22181, #19615, #53806, .T. ) ;
#102150=FACE_OUTER_BOUND ( 'NONE', #107206, .T. ) ;
#102153=ORIENTED_EDGE ( 'NONE', *, *, #57084, .T. ) ;
#102157=CARTESIAN_POINT ( 'NONE',  ( 24.55110742759999809, 1443.479132512090018, 214.0305984285579939 ) ) ;
#102159=CARTESIAN_POINT ( 'NONE',  ( -6.719886226586697653, 1423.239092103852499, 186.8024023424373752 ) ) ;
#102163=CARTESIAN_POINT ( 'NONE',  ( 27.58302672510169629, 1436.789581487599889, 136.7578142616270043 ) ) ;
#102165=CARTESIAN_POINT ( 'NONE',  ( -38.61927355701700293, 1444.188087899089851, 137.1592452686400065 ) ) ;
#102166=CARTESIAN_POINT ( 'NONE',  ( -3.045280019940000305, 1464.258769156330118, 184.9382089438980188 ) ) ;
#102168=CARTESIAN_POINT ( 'NONE',  ( 11.97338606960000007, 1507.452600680129763, 184.7136217416980060 ) ) ;
#102170=VECTOR ( 'NONE', #9355, 1000.000000000000000 ) ;
#102176=CARTESIAN_POINT ( 'NONE',  ( -32.22920765839177903, 1416.715264199195417, 269.3109577515642172 ) ) ;
#102179=CARTESIAN_POINT ( 'NONE',  ( 10.86223758978695919, 1424.799205147552584, 138.1967566982364417 ) ) ;
#102182=CARTESIAN_POINT ( 'NONE',  ( -13.04677262373687086, 1444.843571945705435, 186.3517559318727024 ) ) ;
#102186=CARTESIAN_POINT ( 'NONE',  ( -12.98683036598197660, 1419.640195994466694, 228.2241801252318680 ) ) ;
#102187=CARTESIAN_POINT ( 'NONE',  ( -7.499939553001469861, 1451.406347848051610, 153.0894475933693286 ) ) ;
#102188=CARTESIAN_POINT ( 'NONE',  ( -17.90185111903100079, 1415.935475482089942, 209.1297322982429989 ) ) ;
#102189=CARTESIAN_POINT ( 'NONE',  ( 24.52609508589999976, 1435.360108756510044, 136.2737900993979849 ) ) ;
#102191=CARTESIAN_POINT ( 'NONE',  ( -13.51731348217402306, 1443.821176527551415, 169.3508350027707934 ) ) ;
#102192=VERTEX_POINT ( 'NONE', #98515 ) ;
#102193=CARTESIAN_POINT ( 'NONE',  ( -0.2465388108111499776, 1414.971349104640012, 192.4488333816270256 ) ) ;
#102195=CARTESIAN_POINT ( 'NONE',  ( -10.71339921265560058, 1409.287180531749982, 227.5724379022690016 ) ) ;
#102196=ORIENTED_EDGE ( 'NONE', *, *, #40376, .T. ) ;
#102197=ORIENTED_EDGE ( 'NONE', *, *, #38793, .T. ) ;
#102200=CARTESIAN_POINT ( 'NONE',  ( 10.97483803849999973, 1426.062443049630019, 97.29894937469791216 ) ) ;
#102201=CARTESIAN_POINT ( 'NONE',  ( -26.58541136060000198, 1442.644663293830035, 225.2688052828980005 ) ) ;
#102203=CARTESIAN_POINT ( 'NONE',  ( 4.275225064648620510, 1425.369712006890040, 185.3838194923779952 ) ) ;
#102204=EDGE_CURVE ( 'NONE', #92390, #22181, #10191, .T. ) ;
#102206=CARTESIAN_POINT ( 'NONE',  ( -2.704797619127560004, 1420.195902051749727, 186.0070988970391568 ) ) ;
#102208=CARTESIAN_POINT ( 'NONE',  ( -12.62835224979999893, 1416.067629290630066, 195.5863397732979934 ) ) ;
#102210=CARTESIAN_POINT ( 'NONE',  ( 2.623518071850000410, 1448.928635941619859, 183.1137651247979932 ) ) ;
#102212=EDGE_CURVE ( 'NONE', #29403, #6013, #77044, .T. ) ;
#102213=CARTESIAN_POINT ( 'NONE',  ( -26.94609914958298091, 1509.966636646189500, 222.4048654676792296 ) ) ;
#102215=CARTESIAN_POINT ( 'NONE',  ( -7.706458268878440518E-10, 1416.874386753929912, 237.4765920278839815 ) ) ;
#102216=ORIENTED_EDGE ( 'NONE', *, *, #35114, .F. ) ;
#102218=CARTESIAN_POINT ( 'NONE',  ( -11.83030941994529961, 1429.922132322770040, 149.4306578747379888 ) ) ;
#102220=CARTESIAN_POINT ( 'NONE',  ( -3.068143279839999682, 1471.712358786229970, 269.8661856461979482 ) ) ;
#102226=CARTESIAN_POINT ( 'NONE',  ( 38.64468768876599825, 1444.005792394500077, 137.1818110905059882 ) ) ;
#102229=CARTESIAN_POINT ( 'NONE',  ( -8.384869426575338736, 1406.402803996059902, 267.2065357290120460 ) ) ;
#102230=CARTESIAN_POINT ( 'NONE',  ( -14.33169648120709994, 1436.128833957109919, 150.0042863882840152 ) ) ;
#102233=EDGE_CURVE ( 'NONE', #5500, #51188, #31610, .T. ) ;
#102234=CARTESIAN_POINT ( 'NONE',  ( 13.63158477449999850, 1446.168541001489984, 189.0290012264979964 ) ) ;
#102239=LINE ( 'NONE', #369, #106346 ) ;
#102243=CARTESIAN_POINT ( 'NONE',  ( -16.35102150754449823, 1489.056232056260114, 229.5676014274860108 ) ) ;
#102245=DIRECTION ( 'NONE',  ( 0.000000000000000000, -0.7071067811865474617, -0.7071067811865474617 ) ) ;
#102248=CARTESIAN_POINT ( 'NONE',  ( -27.92008070680000031, 1508.619330697029909, 206.8298810821879954 ) ) ;
#102249=CARTESIAN_POINT ( 'NONE',  ( -4.463702467710766619, 1420.728434188236406, 186.4092242688610668 ) ) ;
#102251=DIRECTION ( 'NONE',  ( 0.2922845185089309461, -0.1043872945603406127, -0.9506171958124757237 ) ) ;
#102255=CARTESIAN_POINT ( 'NONE',  ( -24.37209804522549916, 1430.523523475739921, 210.5057520659609906 ) ) ;
#102256=CARTESIAN_POINT ( 'NONE',  ( 23.50062167809999991, 1488.679648897129937, 220.9815905391980095 ) ) ;
#102259=CARTESIAN_POINT ( 'NONE',  ( -12.99826179536609949, 1436.002654027139897, 150.7444092751300388 ) ) ;
#102263=CARTESIAN_POINT ( 'NONE',  ( -25.98102620619109970, 1446.564900598659960, 138.2990622187889755 ) ) ;
#102266=CARTESIAN_POINT ( 'NONE',  ( -2.535709347209119890, 1451.956901329029961, 184.6703102415019941 ) ) ;
#102267=CARTESIAN_POINT ( 'NONE',  ( -2.377121702169999740, 1410.304607662629905, 232.7018834577980044 ) ) ;
#102269=CARTESIAN_POINT ( 'NONE',  ( -20.07303063531396603, 1456.359329617847379, 225.0559024278571769 ) ) ;
#102271=CARTESIAN_POINT ( 'NONE',  ( -41.65674268029999894, 1443.992461967939789, 135.6790812281979868 ) ) ;
#102273=CARTESIAN_POINT ( 'NONE',  ( 12.35981619036649981, 1435.019032516630205, 150.7822008033989789 ) ) ;
#102274=CARTESIAN_POINT ( 'NONE',  ( -4.074752427351803874, 1441.099746912515457, 184.8041399762123547 ) ) ;
#102285=CARTESIAN_POINT ( 'NONE',  ( -11.40468314538169992, 1414.972329067380088, 195.9645814929980077 ) ) ;
#102286=CARTESIAN_POINT ( 'NONE',  ( 15.80579254656381138, 1409.464994508550490, 192.9618219584179997 ) ) ;
#102287=VERTEX_POINT ( 'NONE', #85018 ) ;
#102292=CARTESIAN_POINT ( 'NONE',  ( 1.807973860705883729, 1416.690826690935182, 232.7107328888371001 ) ) ;
#102293=CARTESIAN_POINT ( 'NONE',  ( 18.63578313170000200, 1416.568813547830132, 209.6898099495820134 ) ) ;
#102295=CARTESIAN_POINT ( 'NONE',  ( -4.915203104360000630, 1434.541746329560056, 150.1320020560979742 ) ) ;
#102296=CARTESIAN_POINT ( 'NONE',  ( 45.64477911114779829, 1440.913060379309854, 266.1600766877090223 ) ) ;
#102298=DIRECTION ( 'NONE',  ( 1.000000000000000000, 0.000000000000000000, 0.000000000000000000 ) ) ;
#102302=CARTESIAN_POINT ( 'NONE',  ( -11.86610048948770135, 1432.336024750160050, 149.9824232984959735 ) ) ;
#102304=CARTESIAN_POINT ( 'NONE',  ( -24.40358107970000034, 1441.574771168059897, 212.0768376997980056 ) ) ;
#102305=CARTESIAN_POINT ( 'NONE',  ( 7.985525884112817607, 1410.564564186529651, 187.6169077096484159 ) ) ;
#102306=CARTESIAN_POINT ( 'NONE',  ( -3.200428057587697328, 1425.998269221526471, 185.6653851470253755 ) ) ;
#102312=CARTESIAN_POINT ( 'NONE',  ( 16.22045774760000114, 1452.203078162129941, 148.6092594038979939 ) ) ;
#102316=CARTESIAN_POINT ( 'NONE',  ( -18.26113587671628835, 1459.251075348199493, 227.8504342410868446 ) ) ;
#102320=CARTESIAN_POINT ( 'NONE',  ( 19.77970646006350108, 1507.962483444719965, 229.2896370130209789 ) ) ;
#102321=ORIENTED_EDGE ( 'NONE', *, *, #68742, .F. ) ;
#102323=CARTESIAN_POINT ( 'NONE',  ( 17.40063846696789795, 1509.472889227200085, 232.3001343056659778 ) ) ;
#102324=DIRECTION ( 'NONE',  ( 0.000000000000000000, 1.000000000000000000, 0.000000000000000000 ) ) ;
#102325=CARTESIAN_POINT ( 'NONE',  ( 38.40016583756019486, 1439.005933973110132, 136.6388233531990011 ) ) ;
#102326=CARTESIAN_POINT ( 'NONE',  ( 22.28696231330000188, 1506.798305107930219, 209.3970118511340104 ) ) ;
#102328=EDGE_CURVE ( 'NONE', #16982, #63865, #91696, .T. ) ;
#102333=CARTESIAN_POINT ( 'NONE',  ( 41.65675406397859604, 1443.992462633329978, 135.6790809494980010 ) ) ;
#102335=CARTESIAN_POINT ( 'NONE',  ( 3.024002413519999877, 1409.955320795729904, 185.7438941976979834 ) ) ;
#102337=CARTESIAN_POINT ( 'NONE',  ( 2.382436964801011303, 1426.901689560120076, 137.0999999980980135 ) ) ;
#102338=CARTESIAN_POINT ( 'NONE',  ( -2.500000009292929981, 1439.653988136930138, 157.1385067185380251 ) ) ;
#102341=CARTESIAN_POINT ( 'NONE',  ( -2.653122947949710042, 1450.219879838080033, 184.3098072337210169 ) ) ;
#102342=CARTESIAN_POINT ( 'NONE',  ( 0.5800689402049999943, 1465.108714862629995, 238.1056003411979987 ) ) ;
#102344=( BOUNDED_CURVE ( )  B_SPLINE_CURVE ( 3, ( #74449, #76088, #16688, #110226 ),
 .UNSPECIFIED., .F., .T. ) 
 B_SPLINE_CURVE_WITH_KNOTS ( ( 4, 4 ),
 ( 3.097738652567880280, 3.109953943715398683 ),
 .UNSPECIFIED. ) 
 CURVE ( )  GEOMETRIC_REPRESENTATION_ITEM ( )  RATIONAL_B_SPLINE_CURVE ( ( 1.000000000000000000, 0.9999875655938355035, 0.9999875655938355035, 1.000000000000000000 ) ) 
 REPRESENTATION_ITEM ( '' )  );
#102347=CARTESIAN_POINT ( 'NONE',  ( -42.06231081589999832, 1442.393258506680013, 269.6487546124980099 ) ) ;
#102349=CARTESIAN_POINT ( 'NONE',  ( 21.98270307507978671, 1506.436298853234575, 208.8042839102180039 ) ) ;
#102351=CARTESIAN_POINT ( 'NONE',  ( -2.986490615134639819E-10, 1470.706479902790079, 255.8596430159340116 ) ) ;
#102352=CARTESIAN_POINT ( 'NONE',  ( 19.54265149998314754, 1436.412494327520335, 145.9155188746681802 ) ) ;
#102353=CARTESIAN_POINT ( 'NONE',  ( -1.555569193359999991, 1415.296882296330068, 227.2022622829979639 ) ) ;
#102354=CARTESIAN_POINT ( 'NONE',  ( -7.535715290459999771, 1417.922762214429895, 231.4272348479980224 ) ) ;
#102357=CARTESIAN_POINT ( 'NONE',  ( -0.2591898832630973870, 1485.931169546443243, 181.8387173835997146 ) ) ;
#102359=CARTESIAN_POINT ( 'NONE',  ( -45.52430914911710147, 1438.500102775369896, 268.9779564349610155 ) ) ;
#102360=CARTESIAN_POINT ( 'NONE',  ( 13.44640270494290135, 1508.358158129190087, 233.2747887588230071 ) ) ;
#102364=CARTESIAN_POINT ( 'NONE',  ( -2.478862593460000152, 1433.766044927639996, 157.5584562999979994 ) ) ;
#102366=EDGE_CURVE ( 'NONE', #79565, #65905, #102344, .T. ) ;
#102367=CARTESIAN_POINT ( 'NONE',  ( 19.40941048885533249, 1456.875960972931580, 224.4905711428775419 ) ) ;
#102369=CARTESIAN_POINT ( 'NONE',  ( -25.83594673127759833, 1451.994654212179967, 135.3393805079549850 ) ) ;
#102371=CARTESIAN_POINT ( 'NONE',  ( -5.472761979749999715E-09, 1419.629243942729772, 225.6556823431979808 ) ) ;
#102376=CARTESIAN_POINT ( 'NONE',  ( -22.76393692011477654, 1450.407194713662193, 220.5314342327505130 ) ) ;
#102378=LINE ( 'NONE', #101813, #1644 ) ;
#102380=ORIENTED_EDGE ( 'NONE', *, *, #39933, .T. ) ;
#102381=CARTESIAN_POINT ( 'NONE',  ( -3.081586005759989977, 1408.632027716779930, 270.4281154310780266 ) ) ;
#102382=CARTESIAN_POINT ( 'NONE',  ( 4.804957937011430147, 1418.134047065659843, 233.3128310201539932 ) ) ;
#102383=CARTESIAN_POINT ( 'NONE',  ( -0.3285615615811641188, 1508.336832367442184, 237.7487474441950042 ) ) ;
#102388=CARTESIAN_POINT ( 'NONE',  ( -1.039113094294850104, 1409.452461688270205, 185.5619659655799865 ) ) ;
#102390=CARTESIAN_POINT ( 'NONE',  ( -43.73460936356224238, 1430.821771421699395, 266.2442057452738595 ) ) ;
#102391=CARTESIAN_POINT ( 'NONE',  ( -20.00429177317949936, 1474.940804442650006, 193.2183630961679910 ) ) ;
#102392=CARTESIAN_POINT ( 'NONE',  ( -22.68195972959999906, 1425.804545574829945, 215.0649984192980071 ) ) ;
#102393=CARTESIAN_POINT ( 'NONE',  ( 35.44508287519440159, 1462.853361191130034, 269.0528564058240022 ) ) ;
#102398=CARTESIAN_POINT ( 'NONE',  ( 18.25718033079806091, 1459.257182848304637, 227.8536879214166504 ) ) ;
#102401=ORIENTED_EDGE ( 'NONE', *, *, #59297, .F. ) ;
#102402=CARTESIAN_POINT ( 'NONE',  ( 3.440555586329999915, 1448.974144786239776, 184.1239056742980154 ) ) ;
#102404=CARTESIAN_POINT ( 'NONE',  ( 27.01916100210560145, 1450.861483528779900, 136.4170495654999797 ) ) ;
#102410=CARTESIAN_POINT ( 'NONE',  ( 1.608553044152920108, 1408.969232297379904, 186.8221281591610250 ) ) ;
#102416=ORIENTED_EDGE ( 'NONE', *, *, #33520, .T. ) ;
#102417=CARTESIAN_POINT ( 'NONE',  ( 11.99589392260669918, 1415.088136167450102, 221.1498175758559910 ) ) ;
#102418=B_SPLINE_SURFACE_WITH_KNOTS ( 'NONE', 5, 1, ( 
 ( #73024, #4168 ),
 ( #63549, #55689 ),
 ( #72479, #63014 ),
 ( #28816, #20937 ),
 ( #107163, #3088 ),
 ( #89811, #106609 ),
 ( #30455, #64639 ),
 ( #22021, #29893 ),
 ( #3639, #71412 ),
 ( #98209, #13628 ),
 ( #21477, #47816 ),
 ( #81951, #73588 ),
 ( #14194, #14751 ),
 ( #24245, #74135 ),
 ( #5821, #66840 ),
 ( #108266, #75236 ),
 ( #91471, #33751 ),
 ( #15289, #31552 ),
 ( #65729, #92018 ),
 ( #67947, #58980 ),
 ( #58427, #48938 ),
 ( #57347, #6360 ),
 ( #40508, #83068 ),
 ( #75775, #42171 ) ),
 .UNSPECIFIED., .F., .F., .F.,
 ( 6, 3, 3, 3, 3, 3, 3, 6 ),
 ( 2, 2 ),
 ( 0.000000000000000000, 1.521747480829999999, 3.044513117910000233, 6.090044392050000255, 24.62876410220000167, 44.04928580589999854, 64.58019525850001230, 84.36259054880000008 ),
 ( 2.018291271429999867, 3.029411390890000000 ),
 .UNSPECIFIED. ) ;
#102419=CARTESIAN_POINT ( 'NONE',  ( 11.45641041208300059, 1432.340941410350069, 151.2730070997519931 ) ) ;
#102423=CARTESIAN_POINT ( 'NONE',  ( -35.12261413890779949, 1450.282964114529932, 136.2298589479320015 ) ) ;
#102425=CARTESIAN_POINT ( 'NONE',  ( -14.73695825029999895, 1462.639194746130215, 255.3819207742980097 ) ) ;
#102427=CARTESIAN_POINT ( 'NONE',  ( 11.86805344210000079, 1433.542299609339807, 150.5539803834979864 ) ) ;
#102428=CARTESIAN_POINT ( 'NONE',  ( 1.554312234479999851E-15, 1455.844446582929777, 219.6133832206979832 ) ) ;
#102433=CARTESIAN_POINT ( 'NONE',  ( 22.43804736130000066, 1409.696614266430061, 208.0348436616479830 ) ) ;
#102434=CARTESIAN_POINT ( 'NONE',  ( 12.60060242696761179, 1398.286606401453810, 205.9241517394453638 ) ) ;
#102435=CARTESIAN_POINT ( 'NONE',  ( -28.33771605659999793, 1510.031322598729957, 222.5657443468980148 ) ) ;
#102444=CARTESIAN_POINT ( 'NONE',  ( 0.1709732279705020175, 1479.758167021719828, 182.1047789143250100 ) ) ;
#102445=CARTESIAN_POINT ( 'NONE',  ( -23.84533141485470153, 1452.080363065020038, 136.9869391916130041 ) ) ;
#102446=ORIENTED_EDGE ( 'NONE', *, *, #80382, .T. ) ;
#102447=CARTESIAN_POINT ( 'NONE',  ( -27.95977047539996718, 1444.740067931808653, 175.9996750486979238 ) ) ;
#102448=DIRECTION ( 'NONE',  ( 0.7067700363771036720, 0.03085824620770448445, 0.7067700363771035610 ) ) ;
#102449=CARTESIAN_POINT ( 'NONE',  ( 11.87909651009999834, 1433.311731933790043, 149.7888166638980181 ) ) ;
#102450=CARTESIAN_POINT ( 'NONE',  ( -40.11569180352149999, 1438.966375984959768, 134.0999999981379744 ) ) ;
#102458=CARTESIAN_POINT ( 'NONE',  ( -15.56469051740000076, 1506.798305107229908, 193.1680121121979994 ) ) ;
#102465=ORIENTED_EDGE ( 'NONE', *, *, #81705, .T. ) ;
#102466=CARTESIAN_POINT ( 'NONE',  ( -29.29916111349999852, 1451.889927077430229, 134.8511816846980196 ) ) ;
#102467=CARTESIAN_POINT ( 'NONE',  ( 12.53380499169999851, 1442.773887286369927, 169.4755105685979970 ) ) ;
#102470=EDGE_LOOP ( 'NONE', ( #32423, #85043, #66971, #92437 ) ) ;
#102476=CARTESIAN_POINT ( 'NONE',  ( 38.90393960482792579, 1452.456950825172953, 269.5913181406285730 ) ) ;
#102477=CARTESIAN_POINT ( 'NONE',  ( -11.60004869885203682, 1426.786830457828273, 134.3786150874268799 ) ) ;
#102478=CARTESIAN_POINT ( 'NONE',  ( 16.17654417561950098, 1432.051473137853691, 218.4400530825793396 ) ) ;
#102485=CARTESIAN_POINT ( 'NONE',  ( 3.117854674740000220, 1446.609948951180058, 165.9235411017980084 ) ) ;
#102487=CARTESIAN_POINT ( 'NONE',  ( 14.35456882750000140, 1416.827520077930103, 196.6651910167979906 ) ) ;
#102491=VERTEX_POINT ( 'NONE', #69364 ) ;
#102493=CARTESIAN_POINT ( 'NONE',  ( -23.34982412229999937, 1410.912491278129892, 205.8672349166580204 ) ) ;
#102494=CARTESIAN_POINT ( 'NONE',  ( -11.12799046640000178, 1426.892988489029904, 99.91667177869788929 ) ) ;
#102495=CARTESIAN_POINT ( 'NONE',  ( 17.19010109773460115, 1410.596273358489725, 192.2276381356939794 ) ) ;
#102497=EDGE_CURVE ( 'NONE', #98691, #22920, #14151, .T. ) ;
#102498=CARTESIAN_POINT ( 'NONE',  ( 9.369692350036283202, 1509.366787681659162, 180.5745519987570162 ) ) ;
#102499=CARTESIAN_POINT ( 'NONE',  ( 2.123651873717662841, 1450.063259378257044, 182.0352679771010003 ) ) ;
#102501=CARTESIAN_POINT ( 'NONE',  ( 29.54414221403980179, 1509.931130577039994, 209.6497321865869878 ) ) ;
#102503=CARTESIAN_POINT ( 'NONE',  ( -37.40887072121479662, 1438.171435685040024, 136.5752352137649837 ) ) ;
#102505=CARTESIAN_POINT ( 'NONE',  ( 10.77209975170500122, 1396.289230399710050, 213.2400182897270042 ) ) ;
#102507=CARTESIAN_POINT ( 'NONE',  ( -17.26192056690000243, 1459.742557600430018, 228.3453419790980092 ) ) ;
#102510=CARTESIAN_POINT ( 'NONE',  ( -29.55500859232640209, 1509.961759442807761, 210.8697166764131339 ) ) ;
#102516=CARTESIAN_POINT ( 'NONE',  ( -1.228114782090000023, 1461.197819184229957, 235.1858097754980008 ) ) ;
#102517=DIRECTION ( 'NONE',  ( -1.987897879952545076E-13, 0.000000000000000000, 1.000000000000000000 ) ) ;
#102525=CARTESIAN_POINT ( 'NONE',  ( 19.97245611310000157, 1487.538185644830037, 227.4393568152979981 ) ) ;
#102527=CARTESIAN_POINT ( 'NONE',  ( -13.36059434050000050, 1414.988017874730076, 220.3623401557979946 ) ) ;
#102528=CARTESIAN_POINT ( 'NONE',  ( -11.54407319952080080, 1432.339775637740104, 151.1365582528090101 ) ) ;
#102531=CARTESIAN_POINT ( 'NONE',  ( -5.042932594320000739, 1422.466626064029924, 185.3903934186979825 ) ) ;
#102537=CARTESIAN_POINT ( 'NONE',  ( 24.80387804530560203, 1461.773651900399955, 206.2179137791540029 ) ) ;
#102539=DIRECTION ( 'NONE',  ( 0.000000000000000000, -0.9990482215818579093, 0.04361938736533144123 ) ) ;
#102540=CARTESIAN_POINT ( 'NONE',  ( -4.529993016832083441, 1423.777408052882720, 184.3664072715177724 ) ) ;
#102541=CARTESIAN_POINT ( 'NONE',  ( -3.472209666708114817, 1506.379719591498088, 187.4566518126731864 ) ) ;
#102543=CARTESIAN_POINT ( 'NONE',  ( -2.414372322354871425, 1486.072943997549146, 181.9601385338485500 ) ) ;
#102545=CARTESIAN_POINT ( 'NONE',  ( -2.917573657582420044, 1484.880000574953101, 183.1918739895752140 ) ) ;
#102546=DIRECTION ( 'NONE',  ( -0.000000000000000000, -1.000000000000000000, -0.000000000000000000 ) ) ;
#102548=ORIENTED_EDGE ( 'NONE', *, *, #52715, .T. ) ;
#102549=CARTESIAN_POINT ( 'NONE',  ( 0.7253211429939999677, 1453.159462793229750, 188.7266509659980045 ) ) ;
#102551=CARTESIAN_POINT ( 'NONE',  ( -11.53630120159999883, 1429.335606864229931, 150.4996243470979778 ) ) ;
#102552=CARTESIAN_POINT ( 'NONE',  ( -10.85273938805417160, 1425.445994626150878, 147.0837058438643226 ) ) ;
#102556=CARTESIAN_POINT ( 'NONE',  ( 11.95011813770030429, 1433.524584343693277, 149.8874522332942547 ) ) ;
#102557=B_SPLINE_CURVE_WITH_KNOTS ( 'NONE', 3,
 ( #18475, #35868, #34750, #44833, #70052, #27449, #78988, #33630, #67824, #101936, #25223, #2830, #57515, #48558, #91082, #46488, #36949, #39591, #31726, #28003, #29111, #28561, #79527, #63297, #65364, #65912, #36402, #73762, #11226, #23322, #104709, #89007, #62190, #62759, #91639, #37511, #53798, #96317, #97415, #99471 ),
 .UNSPECIFIED., .F., .F.,
 ( 4, 3, 3, 3, 3, 3, 3, 3, 3, 3, 3, 3, 3, 4 ),
 ( -1.512517454966539887, -1.431847012466620050, -1.315728653153140026, -1.197778018496070018, -1.078754818121699932, -0.9581669488396040713, -0.8368756102960169807, -0.7152076346036029264, -0.5935212885821531392, -0.4725472813379960613, -0.3524846561758310237, -0.2335963589277290087, -0.1160647746509679834, -2.220446049250313081E-16 ),
 .UNSPECIFIED. ) ;
#102558=CARTESIAN_POINT ( 'NONE',  ( -11.60004869885203682, 0.000000000000000000, 137.0999999980979851 ) ) ;
#102559=CARTESIAN_POINT ( 'NONE',  ( -20.30114903109999958, 1470.087487068429937, 225.8186208082980215 ) ) ;
#102562=VERTEX_POINT ( 'NONE', #36838 ) ;
#102564=CARTESIAN_POINT ( 'NONE',  ( 14.47246893939999879, 1408.205947428329864, 269.4256199600980040 ) ) ;
#102565=CARTESIAN_POINT ( 'NONE',  ( 24.39393896809999873, 1435.492404634590002, 137.6392883061979830 ) ) ;
#102566=CARTESIAN_POINT ( 'NONE',  ( 18.47093090970000162, 1430.306966399830117, 192.6788482552979929 ) ) ;
#102569=CARTESIAN_POINT ( 'NONE',  ( 22.51756156282889876, 1509.699390964210124, 227.9212218486820234 ) ) ;
#102570=CARTESIAN_POINT ( 'NONE',  ( 4.725705173089999711, 1464.404288624430137, 236.3620497209980158 ) ) ;
#102572=CARTESIAN_POINT ( 'NONE',  ( -13.47130175449999889, 1444.268114455909881, 187.0193666120979685 ) ) ;
#102575=CARTESIAN_POINT ( 'NONE',  ( 44.93133208270179324, 1436.268902546335994, 269.6838198007974370 ) ) ;
#102577=CARTESIAN_POINT ( 'NONE',  ( 1.458127919845290110, 1497.749922849950053, 181.5217294836100166 ) ) ;
#102578=CARTESIAN_POINT ( 'NONE',  ( -13.17864806199019867, 1409.373268918529902, 216.1559522034339977 ) ) ;
#102581=CARTESIAN_POINT ( 'NONE',  ( -9.928260447259999566, 1475.299515453429876, 267.4967718279980318 ) ) ;
#102584=CARTESIAN_POINT ( 'NONE',  ( 18.02593473381579514, 1424.491817304190135, 224.3631323497979793 ) ) ;
#102586=CARTESIAN_POINT ( 'NONE',  ( -24.55973745244772388, 1437.066950768452216, 210.6038051167893173 ) ) ;
#102587=CARTESIAN_POINT ( 'NONE',  ( -3.312638106410000116, 1440.449723275869928, 155.6633363266980155 ) ) ;
#102590=DIRECTION ( 'NONE',  ( 0.7074300732568278294, 0.02470400251969398497, 0.7063514732138287400 ) ) ;
#102591=CARTESIAN_POINT ( 'NONE',  ( -23.77655729059999956, 1410.665078721029886, 207.4249854038280034 ) ) ;
#102592=CARTESIAN_POINT ( 'NONE',  ( 17.27701498020000059, 1415.425644477329797, 206.3581100805980100 ) ) ;
#102599=CARTESIAN_POINT ( 'NONE',  ( -22.50660609259999845, 1409.865199589130043, 210.7488977859379986 ) ) ;
#102600=DIRECTION ( 'NONE',  ( -0.7054602837451257047, 1.421085471461279404E-14, -0.7087494536564008518 ) ) ;
#102601=CARTESIAN_POINT ( 'NONE',  ( 11.69802026906100068, 1426.721460024069984, 141.3784292230029678 ) ) ;
#102606=FACE_OUTER_BOUND ( 'NONE', #10540, .T. ) ;
#102608=CARTESIAN_POINT ( 'NONE',  ( -10.12929865658589890, 1398.213355889394961, 217.3039673584101479 ) ) ;
#102609=CARTESIAN_POINT ( 'NONE',  ( -0.1955981723043500320, 1414.913060387329779, 193.0575580317509718 ) ) ;
#102611=CARTESIAN_POINT ( 'NONE',  ( -18.45185438929999933, 1430.290683276829895, 194.4308410190979828 ) ) ;
#102615=ORIENTED_EDGE ( 'NONE', *, *, #52796, .T. ) ;
#102616=ORIENTED_EDGE ( 'NONE', *, *, #34092, .F. ) ;
#102617=CARTESIAN_POINT ( 'NONE',  ( 11.61080405201120058, 1434.661580301569984, 151.3319073679200244 ) ) ;
#102623=CARTESIAN_POINT ( 'NONE',  ( -17.38483621660000011, 1410.884422118429939, 225.7833436061980024 ) ) ;
#102624=CARTESIAN_POINT ( 'NONE',  ( 13.64449414243759939, 1453.162678562290012, 224.5410799634850036 ) ) ;
#102625=CARTESIAN_POINT ( 'NONE',  ( 19.34051166222370099, 1498.116123037349780, 229.0881779061390091 ) ) ;
#102626=CARTESIAN_POINT ( 'NONE',  ( 16.93884295710000387, 1507.634939731529812, 188.0954314088980084 ) ) ;
#102627=CARTESIAN_POINT ( 'NONE',  ( -0.3610880125209999791, 1416.520646107730045, 191.0797029597979986 ) ) ;
#102629=B_SPLINE_SURFACE_WITH_KNOTS ( 'NONE', 5, 5, ( 
 ( #36019, #104314, #27607, #19174, #70756, #62345, #96470, #19749, #30898, #3537, #90250, #80770 ),
 ( #4078, #88632, #88084, #39308, #46637, #97569, #81299, #80219, #38203, #28713, #56116, #55586 ),
 ( #106515, #107064, #30349, #13532, #12988, #47171, #11911, #4614, #55037, #21377, #37660, #64540 ),
 ( #89164, #73480, #71866, #38748, #97029, #72386, #105983, #72925, #98657, #21921, #37108, #29804 ),
 ( #62919, #98103, #89710, #47718, #81849, #11372, #12455, #20292, #5152, #107616, #65077, #29259 ),
 ( #99192, #63992, #22472, #45543, #79683, #2989, #71309, #105422, #54496, #46087, #63450, #20841 ),
 ( #24541, #51990, #50880, #9424, #43038, #77195, #25096, #43587, #84473, #51428, #109679, #33495 ),
 ( #69357, #76625, #49783, #102369, #7760, #8306, #34069, #41927, #41379, #85012, #35174, #58729 ),
 ( #77736, #497, #93967, #76083, #68261, #83916, #32955, #101805, #59302, #92310, #67144, #85558 ),
 ( #103467, #7221, #93416, #110221, #1049, #50348, #25652, #67696, #8855, #59843, #16683, #42467 ),
 ( #110778, #17234, #34622, #68806, #102908, #101242, #26207, #60396, #94515, #17790, #86131, #56672 ),
 ( #15581, #75543, #92865, #16144, #37949, #105147, #26774, #28437, #11097, #36835, #12178, #60961 ) ),
 .UNSPECIFIED., .F., .F., .F.,
 ( 6, 3, 3, 6 ),
 ( 6, 3, 3, 6 ),
 ( 13.14947839535670049, 14.22551365930000067, 16.37671448909999938, 17.67727092117560161 ),
 ( -0.0005573452897113489839, 0.3064376381380000125, 0.9193129144130000041, 1.583189345828600159 ),
 .UNSPECIFIED. ) ;
#102632=CARTESIAN_POINT ( 'NONE',  ( 13.49369409791039942, 1415.034069335220238, 197.8294454127749873 ) ) ;
#102633=CARTESIAN_POINT ( 'NONE',  ( 11.86544875260000076, 1432.297029634840101, 150.3972660524979972 ) ) ;
#102636=CARTESIAN_POINT ( 'NONE',  ( 13.72147666485579975, 1434.975561705699874, 148.6099413304839914 ) ) ;
#102637=ORIENTED_EDGE ( 'NONE', *, *, #61635, .T. ) ;
#102640=CARTESIAN_POINT ( 'NONE',  ( 13.33628935843344543, 1444.532992900501313, 169.3750409159077037 ) ) ;
#102641=CARTESIAN_POINT ( 'NONE',  ( -0.3266743759550000403, 1466.747038422030073, 235.5969264059980333 ) ) ;
#102646=CARTESIAN_POINT ( 'NONE',  ( -18.63123577993770752, 1445.268454213514360, 213.9833683865410308 ) ) ;
#102655=CARTESIAN_POINT ( 'NONE',  ( -12.07537077539999970, 1409.501584340330055, 189.8778375757980257 ) ) ;
#102657=CARTESIAN_POINT ( 'NONE',  ( -4.738498500012391368, 1427.169020172040746, 134.0999999980979851 ) ) ;
#102659=CARTESIAN_POINT ( 'NONE',  ( 24.27347683669999867, 1436.628682044180096, 213.1746251037879745 ) ) ;
#102662=CARTESIAN_POINT ( 'NONE',  ( 4.500000000000000000, 1425.929641636930000, 183.3886486283980162 ) ) ;
#102667=CARTESIAN_POINT ( 'NONE',  ( -22.27620224390000203, 1509.702625319529943, 189.6894443050980215 ) ) ;
#102672=CARTESIAN_POINT ( 'NONE',  ( 13.75903549669999926, 1409.893112527829999, 191.3057326489980028 ) ) ;
#102674=CARTESIAN_POINT ( 'NONE',  ( -18.04045458515061995, 1486.173875672780696, 188.5074830145843521 ) ) ;
#102675=EDGE_CURVE ( 'NONE', #31992, #944, #40929, .T. ) ;
#102679=CARTESIAN_POINT ( 'NONE',  ( 36.52134894070000115, 1445.557347021360101, 254.5790014346980286 ) ) ;
#102683=CARTESIAN_POINT ( 'NONE',  ( -1.547605067268360113, 1508.721288987890148, 238.0070242337440050 ) ) ;
#102684=CARTESIAN_POINT ( 'NONE',  ( -23.70328061310000223, 1446.840119191189842, 215.0759071426080311 ) ) ;
#102687=CARTESIAN_POINT ( 'NONE',  ( 19.24600158930000049, 1456.014086358630038, 226.4361891347980134 ) ) ;
#102690=ORIENTED_EDGE ( 'NONE', *, *, #98671, .T. ) ;
#102692=CARTESIAN_POINT ( 'NONE',  ( 0.2144067139459999993, 1406.265208649629812, 269.2947081879980260 ) ) ;
#102694=AXIS2_PLACEMENT_3D ( 'NONE', #6188, #83439, #7297 ) ;
#102695=CARTESIAN_POINT ( 'NONE',  ( 12.82945534090000095, 1428.689089259029743, 223.8443168781979864 ) ) ;
#102700=CARTESIAN_POINT ( 'NONE',  ( 27.07063991995919849, 1435.441545612230129, 135.7158103180489945 ) ) ;
#102701=CARTESIAN_POINT ( 'NONE',  ( 37.56297661588190095, 1449.170392729680088, 136.3356801895480146 ) ) ;
#102702=CARTESIAN_POINT ( 'NONE',  ( -31.98368035039945312, 1465.292284392873171, 269.3160916878242688 ) ) ;
#102704=CARTESIAN_POINT ( 'NONE',  ( -4.148647832312248873, 1448.210448412289907, 185.1107006651311906 ) ) ;
#102706=EDGE_CURVE ( 'NONE', #12743, #22102, #60996, .T. ) ;
#102709=CARTESIAN_POINT ( 'NONE',  ( 0.5238716634341910039, 1409.870337634420139, 185.0929748826949890 ) ) ;
#102710=CARTESIAN_POINT ( 'NONE',  ( 12.91347167809999874, 1434.774310044250115, 146.4344529612980068 ) ) ;
#102711=ADVANCED_FACE ( 'NONE', ( #49421 ), #23900, .F. ) ;
#102713=CARTESIAN_POINT ( 'NONE',  ( 15.47406948735730126, 1461.410564919109902, 189.5408260342219933 ) ) ;
#102714=CARTESIAN_POINT ( 'NONE',  ( 10.88562390665740054, 1424.831925956591249, 138.2234943703446390 ) ) ;
#102717=CARTESIAN_POINT ( 'NONE',  ( -29.24528536989999949, 1509.871747141630067, 209.9183570146090005 ) ) ;
#102718=CIRCLE ( 'NONE', #49224, 27.48039273450891073 ) ;
#102721=CARTESIAN_POINT ( 'NONE',  ( 42.28240996344969460, 1440.913018452919914, 269.8809620301270229 ) ) ;
#102722=CARTESIAN_POINT ( 'NONE',  ( -15.03694588066141868, 1451.150679764012921, 149.6984823041283335 ) ) ;
#102724=CARTESIAN_POINT ( 'NONE',  ( 25.15255372800000089, 1436.299077768329880, 137.5035669820980218 ) ) ;
#102725=CARTESIAN_POINT ( 'NONE',  ( -11.00145890658190062, 1396.297239797879911, 207.8695728886200129 ) ) ;
#102728=CARTESIAN_POINT ( 'NONE',  ( -17.17297594112050163, 1410.145097443089981, 225.7364921415430103 ) ) ;
#102729=CARTESIAN_POINT ( 'NONE',  ( 2.471608048749999842, 1438.194204504490017, 150.4833623973980252 ) ) ;
#102730=VERTEX_POINT ( 'NONE', #78474 ) ;
#102731=ORIENTED_EDGE ( 'NONE', *, *, #33237, .F. ) ;
#102736=CARTESIAN_POINT ( 'NONE',  ( 24.01654869009999871, 1411.112688614930221, 209.9218154780569989 ) ) ;
#102737=CARTESIAN_POINT ( 'NONE',  ( 4.164654618643389483, 1424.779710594659946, 185.0949776876690009 ) ) ;
#102738=CARTESIAN_POINT ( 'NONE',  ( -2.604853897581669742, 1420.561510432767136, 185.7674481731004050 ) ) ;
#102741=CARTESIAN_POINT ( 'NONE',  ( 8.460916142840000376, 1509.208523567629982, 181.0428522260980060 ) ) ;
#102742=CARTESIAN_POINT ( 'NONE',  ( 3.649946445679999485, 1449.553923602460145, 184.1602381183980128 ) ) ;
#102747=VERTEX_POINT ( 'NONE', #34808 ) ;
#102748=ORIENTED_EDGE ( 'NONE', *, *, #94458, .T. ) ;
#102750=CARTESIAN_POINT ( 'NONE',  ( -1.089377596668410053, 1508.669637244069918, 201.3050124727430159 ) ) ;
#102751=CARTESIAN_POINT ( 'NONE',  ( -2.462320445819999909E-09, 1473.897694201330069, 270.2927087787980440 ) ) ;
#102752=CARTESIAN_POINT ( 'NONE',  ( 13.23538125255438125, 1434.875856760270153, 146.8238586004999320 ) ) ;
#102753=CARTESIAN_POINT ( 'NONE',  ( -2.794270253690000150, 1486.375510484630013, 181.7653640124980257 ) ) ;
#102754=CARTESIAN_POINT ( 'NONE',  ( -5.519906363166400709, 1440.499855196290127, 154.7645174855159951 ) ) ;
#102757=CARTESIAN_POINT ( 'NONE',  ( 38.64637139974560398, 1443.913060387190171, 137.1864063390110005 ) ) ;
#102759=CARTESIAN_POINT ( 'NONE',  ( -0.06333902539661169506, 1408.725629450729912, 195.0481631183849913 ) ) ;
#102760=CARTESIAN_POINT ( 'NONE',  ( -20.55457359352670110, 1409.641135491380055, 268.8772925003830210 ) ) ;
#102761=CARTESIAN_POINT ( 'NONE',  ( -14.53519835277139904, 1435.864472234740106, 149.7571133851789966 ) ) ;
#102764=CARTESIAN_POINT ( 'NONE',  ( 13.62998674540000010, 1443.967433543380139, 188.6491937973979987 ) ) ;
#102767=EDGE_LOOP ( 'NONE', ( #9975, #14793, #97856, #97625 ) ) ;
#102768=ORIENTED_EDGE ( 'NONE', *, *, #94108, .T. ) ;
#102772=EDGE_CURVE ( 'NONE', #37255, #64180, #35573, .T. ) ;
#102773=CIRCLE ( 'NONE', #54565, 1.999999954375424105 ) ;
#102778=ORIENTED_EDGE ( 'NONE', *, *, #102904, .T. ) ;
#102783=CARTESIAN_POINT ( 'NONE',  ( -26.74681214179999955, 1508.000506563529825, 202.6166866765980217 ) ) ;
#102785=CARTESIAN_POINT ( 'NONE',  ( -4.250070793035421346, 1421.703404060810726, 185.6649461142346524 ) ) ;
#102787=CARTESIAN_POINT ( 'NONE',  ( -5.135476803700000481, 1408.035052921730085, 196.9098792946979870 ) ) ;
#102789=CARTESIAN_POINT ( 'NONE',  ( -7.341715959830000138, 1447.503732850919960, 185.7896193941979845 ) ) ;
#102790=EDGE_LOOP ( 'NONE', ( #76577, #61671, #104812, #3221, #56809 ) ) ;
#102792=CARTESIAN_POINT ( 'NONE',  ( 26.22657672280000085, 1469.244931003429883, 211.2286983240879863 ) ) ;
#102793=CARTESIAN_POINT ( 'NONE',  ( 19.78687179431750209, 1477.275181142720157, 225.5437915623070069 ) ) ;
#102794=CARTESIAN_POINT ( 'NONE',  ( -25.77733573009999901, 1435.590736967609928, 136.2196633588979751 ) ) ;
#102797=CARTESIAN_POINT ( 'NONE',  ( -15.36549427709999982, 1420.414141551129887, 227.0219849000980048 ) ) ;
#102800=ADVANCED_FACE ( 'NONE', ( #81751 ), #100794, .F. ) ;
#102803=CARTESIAN_POINT ( 'NONE',  ( -1.987196561129769945, 1451.943606313749797, 184.3861899504009898 ) ) ;
#102804=CARTESIAN_POINT ( 'NONE',  ( -4.411357854800000311, 1412.836356211030079, 232.1857068625979821 ) ) ;
#102806=ADVANCED_FACE ( 'NONE', ( #57698 ), #68707, .F. ) ;
#102807=VERTEX_POINT ( 'NONE', #40311 ) ;
#102810=ORIENTED_EDGE ( 'NONE', *, *, #11089, .F. ) ;
#102811=CARTESIAN_POINT ( 'NONE',  ( 12.30222356331140077, 1434.228817860290064, 149.7285221497980103 ) ) ;
#102812=CARTESIAN_POINT ( 'NONE',  ( -4.112992287346649789, 1441.414772796051693, 184.3124314157482502 ) ) ;
#102814=CARTESIAN_POINT ( 'NONE',  ( -22.26576771697250123, 1509.633339851660139, 227.8536643167900309 ) ) ;
#102815=CARTESIAN_POINT ( 'NONE',  ( -1.137831540960000165, 1408.952794340330001, 186.7671042942980080 ) ) ;
#102817=CARTESIAN_POINT ( 'NONE',  ( 4.235259697215119523, 1441.487973001730097, 163.7720251071719986 ) ) ;
#102818=EDGE_CURVE ( 'NONE', #51888, #15423, #100226, .T. ) ;
#102820=CARTESIAN_POINT ( 'NONE',  ( -2.828449817540000133, 1421.423221026929923, 184.8604656580980077 ) ) ;
#102821=FACE_OUTER_BOUND ( 'NONE', #68363, .T. ) ;
#102824=CARTESIAN_POINT ( 'NONE',  ( -12.78701144699999936, 1416.830000968330069, 195.3261870004980096 ) ) ;
#102825=DIRECTION ( 'NONE',  ( 0.000000000000000000, -1.000000000000000000, 0.000000000000000000 ) ) ;
#102827=CARTESIAN_POINT ( 'NONE',  ( 2.848182016099999547, 1421.430268250230029, 183.3773441410979785 ) ) ;
#102835=CARTESIAN_POINT ( 'NONE',  ( 17.76981827703365013, 1423.499564355630127, 226.0984388876629225 ) ) ;
#102838=CARTESIAN_POINT ( 'NONE',  ( 15.58656453949999943, 1453.146242307530201, 195.7022669009980120 ) ) ;
#102839=CARTESIAN_POINT ( 'NONE',  ( 37.94792208049119608, 1440.913060383530137, 256.1973595134240327 ) ) ;
#102841=CARTESIAN_POINT ( 'NONE',  ( -2.880242083973940215, 1486.014389300230050, 182.1002674444409877 ) ) ;
#102842=CARTESIAN_POINT ( 'NONE',  ( 11.93818824289999903, 1433.480083226980014, 149.8972169559980046 ) ) ;
#102845=CARTESIAN_POINT ( 'NONE',  ( 26.38087806250000256, 1488.565686197229979, 207.2125440848780045 ) ) ;
#102847=CARTESIAN_POINT ( 'NONE',  ( -29.22958589439999955, 1509.933780018729749, 211.7723606779179875 ) ) ;
#102848=CARTESIAN_POINT ( 'NONE',  ( 6.928228050084153544, 1410.528584160930222, 187.1351645713825462 ) ) ;
#102850=EDGE_CURVE ( 'NONE', #23029, #84300, #34669, .T. ) ;
#102851=CARTESIAN_POINT ( 'NONE',  ( 9.515252399970000496, 1407.295241224529946, 218.7370609393180132 ) ) ;
#102860=CARTESIAN_POINT ( 'NONE',  ( 25.23673856130000104, 1509.794357971529962, 195.3594004736979741 ) ) ;
#102862=CARTESIAN_POINT ( 'NONE',  ( -17.69970948712861158, 1460.181651798936628, 228.1664494889768093 ) ) ;
#102865=ORIENTED_EDGE ( 'NONE', *, *, #102497, .T. ) ;
#102867=CARTESIAN_POINT ( 'NONE',  ( 19.17417272014210283, 1508.304322950820278, 229.7399540503319884 ) ) ;
#102869=CARTESIAN_POINT ( 'NONE',  ( 38.79039661010919815, 1439.444248131590030, 136.6768088287299747 ) ) ;
#102870=CARTESIAN_POINT ( 'NONE',  ( 18.89028803260000089, 1434.820761660039807, 209.0360204046969841 ) ) ;
#102871=CARTESIAN_POINT ( 'NONE',  ( -35.93744657210000071, 1447.859701337770048, 254.6052923994979835 ) ) ;
#102875=CARTESIAN_POINT ( 'NONE',  ( -19.91083394019999986, 1484.850239523630080, 191.2132470572979912 ) ) ;
#102876=CARTESIAN_POINT ( 'NONE',  ( 2.135518920310000013, 1409.155356716130200, 186.0513290997979823 ) ) ;
#102878=CARTESIAN_POINT ( 'NONE',  ( -5.445836181560000711, 1441.097906891670164, 154.8052917044979893 ) ) ;
#102881=CARTESIAN_POINT ( 'NONE',  ( -3.534844613916279688, 1450.759385590300099, 184.8958323056850190 ) ) ;
#102882=CARTESIAN_POINT ( 'NONE',  ( 1.999662964720000158, 1464.770985739130083, 236.6485670609980048 ) ) ;
#102886=CARTESIAN_POINT ( 'NONE',  ( -44.70562379640000472, 1442.567860055949950, 269.9105898675979915 ) ) ;
#102887=CARTESIAN_POINT ( 'NONE',  ( -27.50547247590620259, 1446.424453594049965, 137.1666655446350092 ) ) ;
#102888=CARTESIAN_POINT ( 'NONE',  ( -3.604910588070000088, 1439.699991058859950, 185.4007874081979992 ) ) ;
#102889=CARTESIAN_POINT ( 'NONE',  ( 16.32506211009999930, 1488.226337218230128, 188.7019445247979945 ) ) ;
#102890=CARTESIAN_POINT ( 'NONE',  ( -9.987187384052590294E-09, 1473.076079583149976, 261.4091305460700028 ) ) ;
#102892=CARTESIAN_POINT ( 'NONE',  ( -1.393184507720000020, 1415.579607678529783, 227.5929094376980117 ) ) ;
#102893=CARTESIAN_POINT ( 'NONE',  ( -10.08879832530000087, 1419.700932331030117, 231.6349072129980016 ) ) ;
#102897=CARTESIAN_POINT ( 'NONE',  ( -0.2497437932752624434, 1485.943969500690173, 181.8371981571018239 ) ) ;
#102899=CARTESIAN_POINT ( 'NONE',  ( -45.83609828259869801, 1437.696264054630092, 268.5022178222189950 ) ) ;
#102900=CARTESIAN_POINT ( 'NONE',  ( -2.694370070079999735, 1428.717074573929949, 185.1363698905980186 ) ) ;
#102904=EDGE_CURVE ( 'NONE', #38555, #27144, #64942, .T. ) ;
#102908=CARTESIAN_POINT ( 'NONE',  ( -26.83284804043870153, 1451.909710471250037, 135.4138440258689968 ) ) ;
#102909=ORIENTED_EDGE ( 'NONE', *, *, #16997, .T. ) ;
#102910=CARTESIAN_POINT ( 'NONE',  ( -14.60873270509999955, 1470.816572150829870, 194.8395487178979977 ) ) ;
#102912=CARTESIAN_POINT ( 'NONE',  ( 15.39218709410000052, 1506.810797420630024, 193.3968663410979900 ) ) ;
#102914=CARTESIAN_POINT ( 'NONE',  ( -19.55701159338780215, 1456.127805513401881, 228.1967745818641049 ) ) ;
#102915=EDGE_CURVE ( 'NONE', #16730, #104691, #79404, .T. ) ;
#102919=CARTESIAN_POINT ( 'NONE',  ( -4.308968488989159518, 1408.710846737909833, 270.4270427888720292 ) ) ;
#102921=CARTESIAN_POINT ( 'NONE',  ( 8.893954816108170291, 1419.211828825139946, 232.2343367069420310 ) ) ;
#102925=ORIENTED_EDGE ( 'NONE', *, *, #15031, .F. ) ;
#102926=CARTESIAN_POINT ( 'NONE',  ( -22.64963451372929981, 1409.703995751010098, 209.5275992923249930 ) ) ;
#102927=CARTESIAN_POINT ( 'NONE',  ( -0.4457311135394249613, 1409.096194338759915, 185.6363386297540217 ) ) ;
#102930=CARTESIAN_POINT ( 'NONE',  ( -18.14005346051209955, 1415.388767200230177, 195.1132133976919931 ) ) ;
#102931=CARTESIAN_POINT ( 'NONE',  ( -19.86345851500000137, 1425.811316569130213, 222.6950000957980080 ) ) ;
#102932=CARTESIAN_POINT ( 'NONE',  ( 37.07563244675080227, 1462.054830057500112, 267.9004510718949632 ) ) ;
#102934=CARTESIAN_POINT ( 'NONE',  ( -2.390460581662895656, 1466.906621117755549, 235.1802628545677010 ) ) ;
#102938=CARTESIAN_POINT ( 'NONE',  ( -11.94265413316043656, 1433.497479536225455, 149.9944130464578222 ) ) ;
#102939=CARTESIAN_POINT ( 'NONE',  ( 1.527006335184809993, 1453.898422402579854, 183.4371394172420082 ) ) ;
#102941=ORIENTED_EDGE ( 'NONE', *, *, #42194, .F. ) ;
#102942=CARTESIAN_POINT ( 'NONE',  ( -1.451575880177540023, 1457.988782316290099, 229.8657700608300161 ) ) ;
#102944=CARTESIAN_POINT ( 'NONE',  ( 26.07109846599830050, 1452.002629622410041, 135.0133573619999936 ) ) ;
#102949=CARTESIAN_POINT ( 'NONE',  ( 17.90246463440000113, 1410.035002130830208, 193.6991388332980080 ) ) ;
#102951=CARTESIAN_POINT ( 'NONE',  ( 2.637369437447386389, 1439.648528781137884, 183.5003223541247905 ) ) ;
#102952=CARTESIAN_POINT ( 'NONE',  ( 1.331911112270000030, 1417.152951162330055, 233.7702109215979931 ) ) ;
#102953=CARTESIAN_POINT ( 'NONE',  ( -19.40632858663824933, 1425.506857333870357, 223.5429138958425597 ) ) ;
#102954=CARTESIAN_POINT ( 'NONE',  ( 1.067515872454499970, 1451.920614097839916, 183.2424258504900081 ) ) ;
#102959=CARTESIAN_POINT ( 'NONE',  ( 6.750002614367778264, 1418.487218233497970, 233.5578456803374934 ) ) ;
#102960=VERTEX_POINT ( 'NONE', #78903 ) ;
#102962=CARTESIAN_POINT ( 'NONE',  ( 10.96946812545280103, 1432.347663862999980, 151.7701354189910035 ) ) ;
#102970=CARTESIAN_POINT ( 'NONE',  ( -21.37693747720000204, 1443.303628178600093, 224.8635561966979708 ) ) ;
#102971=CARTESIAN_POINT ( 'NONE',  ( -21.44621506493709973, 1509.083182011242798, 191.8119323521389106 ) ) ;
#102972=CARTESIAN_POINT ( 'NONE',  ( 11.63847943070000035, 1433.482589826759977, 151.0612159216979933 ) ) ;
#102973=CARTESIAN_POINT ( 'NONE',  ( 11.06589455810000011, 1457.157324861229881, 234.3916895697979612 ) ) ;
#102974=CARTESIAN_POINT ( 'NONE',  ( 11.80289467588129959, 1415.088012641449950, 196.9360298139739882 ) ) ;
#102975=AXIS2_PLACEMENT_3D ( 'NONE', #52458, #70937, #105053 ) ;
#102979=CARTESIAN_POINT ( 'NONE',  ( -15.78890742300000127, 1486.496171638329997, 186.5216181066980141 ) ) ;
#102980=CARTESIAN_POINT ( 'NONE',  ( 7.615013220904412350, 1398.139290501694404, 219.7751663341437620 ) ) ;
#102981=CARTESIAN_POINT ( 'NONE',  ( -26.08589733633370145, 1509.953121808929836, 192.9123034651479998 ) ) ;
#102984=CARTESIAN_POINT ( 'NONE',  ( 3.313292261855492082, 1446.583017422768989, 170.5342543665201163 ) ) ;
#102985=CARTESIAN_POINT ( 'NONE',  ( -41.18635921427883062, 1440.753220515532576, 135.3771779697534328 ) ) ;
#102987=CARTESIAN_POINT ( 'NONE',  ( 11.36538105552331501, 1434.589103438910797, 151.5115492014778908 ) ) ;
#102988=( BOUNDED_CURVE ( )  B_SPLINE_CURVE ( 3, ( #91757, #15033, #108564, #31301 ),
 .UNSPECIFIED., .F., .F. ) 
 B_SPLINE_CURVE_WITH_KNOTS ( ( 4, 4 ),
 ( 2.603837571717090071, 2.914415234293290080 ),
 .UNSPECIFIED. ) 
 CURVE ( )  GEOMETRIC_REPRESENTATION_ITEM ( )  RATIONAL_B_SPLINE_CURVE ( ( 1.000000000000000000, 0.9919779331734855932, 0.9919779331734855932, 1.000000000000000000 ) ) 
 REPRESENTATION_ITEM ( '' )  );
#102993=CARTESIAN_POINT ( 'NONE',  ( 0.1684383342722930166, 1481.247972760530047, 182.0407818193630192 ) ) ;
#102995=ORIENTED_EDGE ( 'NONE', *, *, #69977, .F. ) ;
#102996=CARTESIAN_POINT ( 'NONE',  ( -1.121351043030000216, 1416.825532269230052, 228.0848332775979941 ) ) ;
#102997=CARTESIAN_POINT ( 'NONE',  ( -33.08110269718211072, 1445.052233488288266, 154.3415468483447910 ) ) ;
#103010=B_SPLINE_CURVE_WITH_KNOTS ( 'NONE', 5,
 ( #69297, #60903, #25594, #86620, #17730, #10470 ),
 .UNSPECIFIED., .F., .F.,
 ( 6, 6 ),
 ( 0.000000000000000000, 1.000000000000000000 ),
 .UNSPECIFIED. ) ;
#103013=CARTESIAN_POINT ( 'NONE',  ( 2.994688454485729956, 1464.609795419120246, 236.6065850994260131 ) ) ;
#103016=CARTESIAN_POINT ( 'NONE',  ( -15.81248221509479812, 1410.431092464730000, 226.6593714454470216 ) ) ;
#103017=CARTESIAN_POINT ( 'NONE',  ( 2.253566441613126910E-10, 1426.918876941764893, 134.0999999980979851 ) ) ;
#103020=ORIENTED_EDGE ( 'NONE', *, *, #10600, .T. ) ;
#103021=CARTESIAN_POINT ( 'NONE',  ( 23.82032192280000160, 1509.070381045429940, 222.7384874576979996 ) ) ;
#103024=CARTESIAN_POINT ( 'NONE',  ( -5.021037887259439003, 1440.968375784700129, 155.1907004240329968 ) ) ;
#103025=CARTESIAN_POINT ( 'NONE',  ( 15.10371975099999986, 1409.440493903229935, 192.9533947891980006 ) ) ;
#103026=CARTESIAN_POINT ( 'NONE',  ( 19.42500282749999840, 1440.913060387330006, 212.4633492400480179 ) ) ;
#103028=CARTESIAN_POINT ( 'NONE',  ( 20.11865583365249677, 1457.295773309100014, 209.3900325861709746 ) ) ;
#103029=CARTESIAN_POINT ( 'NONE',  ( -21.84222938500011679, 1507.845663673426770, 226.4317239180982710 ) ) ;
#103031=CARTESIAN_POINT ( 'NONE',  ( 20.59684415428669979, 1507.762623717989982, 227.6602567528719874 ) ) ;
#103033=CARTESIAN_POINT ( 'NONE',  ( 4.293785987919999769, 1447.009251274299913, 154.3906956833980075 ) ) ;
#103035=CARTESIAN_POINT ( 'NONE',  ( 14.45750875900000132, 1416.828042640230024, 196.8520545293980319 ) ) ;
#103042=CARTESIAN_POINT ( 'NONE',  ( -24.09077679880000034, 1449.794656643329972, 202.7835535694879923 ) ) ;
#103043=CARTESIAN_POINT ( 'NONE',  ( -11.50815781787750147, 1426.421521582019977, 127.8416712200489940 ) ) ;
#103044=CARTESIAN_POINT ( 'NONE',  ( 16.29419587174599826, 1409.489892375330101, 193.0344759318469983 ) ) ;
#103046=CARTESIAN_POINT ( 'NONE',  ( 17.38707324475434746, 1509.640293562321631, 184.6720443489594459 ) ) ;
#103047=CARTESIAN_POINT ( 'NONE',  ( -21.04915883790000208, 1471.323284330029992, 208.5356106908370180 ) ) ;
#103048=CARTESIAN_POINT ( 'NONE',  ( -41.23304013239999932, 1435.760839457339898, 261.5842231913979958 ) ) ;
#103050=CARTESIAN_POINT ( 'NONE',  ( 28.40191814900270018, 1508.834101303340049, 209.4333091118389802 ) ) ;
#103053=B_SPLINE_CURVE_WITH_KNOTS ( 'NONE', 3,
 ( #83432, #56050, #98034, #65563, #6729, #81778 ),
 .UNSPECIFIED., .F., .F.,
 ( 4, 2, 4 ),
 ( -0.1558952665523989922, -0.07794716665277695578, -2.594126852384359694E-06 ),
 .UNSPECIFIED. ) ;
#103054=CARTESIAN_POINT ( 'NONE',  ( -38.00991624508050393, 1438.636109681070138, 136.6089179658529815 ) ) ;
#103055=ORIENTED_EDGE ( 'NONE', *, *, #25710, .F. ) ;
#103056=CARTESIAN_POINT ( 'NONE',  ( 13.78199155278950094, 1397.422248721489950, 206.9763111428489992 ) ) ;
#103058=AXIS2_PLACEMENT_3D ( 'NONE', #84613, #58332, #84067 ) ;
#103059=CARTESIAN_POINT ( 'NONE',  ( -17.12053142319999921, 1459.474259415330152, 228.5189956839979857 ) ) ;
#103061=ORIENTED_EDGE ( 'NONE', *, *, #18144, .F. ) ;
#103062=CARTESIAN_POINT ( 'NONE',  ( -18.97219799319119815, 1486.246528605739741, 189.3000344508529906 ) ) ;
#103063=CARTESIAN_POINT ( 'NONE',  ( 7.105419199340579675E-15, 1425.409945881219983, 153.8891009232719966 ) ) ;
#103067=DIRECTION ( 'NONE',  ( 0.000000000000000000, 1.000000000000000000, 0.000000000000000000 ) ) ;
#103068=CARTESIAN_POINT ( 'NONE',  ( 27.56721560699687146, 1509.458871272823671, 206.1447979657547478 ) ) ;
#103076=ORIENTED_EDGE ( 'NONE', *, *, #10386, .F. ) ;
#103077=CARTESIAN_POINT ( 'NONE',  ( 11.81166646117249996, 1428.828521759150135, 148.7357659156419913 ) ) ;
#103080=CARTESIAN_POINT ( 'NONE',  ( -1.452061816759999902, 1467.474562141730075, 183.2045861867980250 ) ) ;
#103081=ADVANCED_FACE ( 'NONE', ( #36323 ), #25739, .T. ) ;
#103085=CARTESIAN_POINT ( 'NONE',  ( -4.915892415680000127, 1423.440305011429928, 184.6741102763979825 ) ) ;
#103086=CARTESIAN_POINT ( 'NONE',  ( 13.09236780528799926, 1411.228464131030023, 270.0792911668929719 ) ) ;
#103089=CARTESIAN_POINT ( 'NONE',  ( -10.05941745090078143, 1410.638996758815210, 188.4493189201661210 ) ) ;
#103091=CARTESIAN_POINT ( 'NONE',  ( -15.93334107429999946, 1485.110845200029871, 224.0169806397979926 ) ) ;
#103092=CARTESIAN_POINT ( 'NONE',  ( 17.79624440539999952, 1458.182673695930134, 228.6901989446980110 ) ) ;
#103094=CARTESIAN_POINT ( 'NONE',  ( -4.752998812148558017, 1423.601010648300417, 184.5372248178350958 ) ) ;
#103095=CARTESIAN_POINT ( 'NONE',  ( -10.73514660131351839, 1424.973046421745494, 139.1354236205272343 ) ) ;
#103099=AXIS2_PLACEMENT_3D ( 'NONE', #15261, #91446, #14722 ) ;
#103102=CARTESIAN_POINT ( 'NONE',  ( -2.927028964964125457, 1485.034416825944163, 183.1263100967265416 ) ) ;
#103107=CARTESIAN_POINT ( 'NONE',  ( 0.7305497199880000014, 1471.316885392330050, 187.9286521196980004 ) ) ;
#103108=CARTESIAN_POINT ( 'NONE',  ( -15.28377182955919977, 1507.620489270460212, 191.9630984214329885 ) ) ;
#103109=CARTESIAN_POINT ( 'NONE',  ( -11.83460451569999883, 1430.051560513030154, 149.9498806582980137 ) ) ;
#103110=CARTESIAN_POINT ( 'NONE',  ( 19.40526558876458907, 1456.941577366487991, 224.5007284994117072 ) ) ;
#103116=CARTESIAN_POINT ( 'NONE',  ( 33.91369278643569629, 1437.010534640189690, 136.5611839302279691 ) ) ;
#103118=CARTESIAN_POINT ( 'NONE',  ( -16.55764869240000081, 1460.395321624930148, 228.3393650202980041 ) ) ;
#103120=CARTESIAN_POINT ( 'NONE',  ( 14.40766152700000013, 1408.465220730830197, 269.5837135859979981 ) ) ;
#103121=CARTESIAN_POINT ( 'NONE',  ( 2.689344463419570452, 1464.716346866380036, 236.9361821190090041 ) ) ;
#103122=CARTESIAN_POINT ( 'NONE',  ( 18.90842699680000294, 1430.304836455529994, 193.3988046526980042 ) ) ;
#103123=CARTESIAN_POINT ( 'NONE',  ( -23.69221647310000023, 1436.197216314300022, 212.4790823011979910 ) ) ;
#103124=CARTESIAN_POINT ( 'NONE',  ( 6.555713241385960011, 1506.475290693023453, 230.1454641328169259 ) ) ;
#103126=CARTESIAN_POINT ( 'NONE',  ( -40.71429805386350154, 1443.131898661159994, 137.0441744550780072 ) ) ;
#103127=EDGE_CURVE ( 'NONE', #20179, #5014, #104784, .T. ) ;
#103130=CARTESIAN_POINT ( 'NONE',  ( -13.83903651480000008, 1444.969018072280051, 188.3469987607979874 ) ) ;
#103132=CARTESIAN_POINT ( 'NONE',  ( -30.78499955540000244, 1436.901323119660219, 136.6581730245979713 ) ) ;
#103136=CARTESIAN_POINT ( 'NONE',  ( -12.68420265674900094, 1409.356002504509888, 217.0171520026799783 ) ) ;
#103137=CARTESIAN_POINT ( 'NONE',  ( 11.26969769241764219, 1425.486564486241832, 139.1357072137798809 ) ) ;
#103138=CARTESIAN_POINT ( 'NONE',  ( -2.500000000000000000, 1411.429641636930000, 127.2892455880980123 ) ) ;
#103140=CARTESIAN_POINT ( 'NONE',  ( -12.52817736919999980, 1473.792528260629979, 269.6003666339980214 ) ) ;
#103142=DIRECTION ( 'NONE',  ( 0.9750097311986455351, 0.1381407795329493426, -0.1739918075599369285 ) ) ;
#103143=FACE_OUTER_BOUND ( 'NONE', #73444, .T. ) ;
#103146=CARTESIAN_POINT ( 'NONE',  ( -13.75903449370000153, 1409.893112547430064, 226.9379585588980035 ) ) ;
#103147=CARTESIAN_POINT ( 'NONE',  ( 11.97935895607569989, 1415.724942524390144, 223.2960686490259832 ) ) ;
#103151=CARTESIAN_POINT ( 'NONE',  ( -22.51439127229999926, 1409.699280255230178, 208.1503399454410328 ) ) ;
#103152=CARTESIAN_POINT ( 'NONE',  ( 15.66638256379999916, 1416.825421875629900, 199.0472708910980089 ) ) ;
#103154=DIRECTION ( 'NONE',  ( 0.000000000000000000, 0.000000000000000000, -1.000000000000000000 ) ) ;
#103155=CARTESIAN_POINT ( 'NONE',  ( 7.341316150999999179E-16, 1441.600846913620217, 150.7224806086979640 ) ) ;
#103156=CIRCLE ( 'NONE', #6623, 0.5000000000000000000 ) ;
#103160=CARTESIAN_POINT ( 'NONE',  ( -23.10251492229999926, 1410.654477831930080, 210.9078341742080056 ) ) ;
#103161=CARTESIAN_POINT ( 'NONE',  ( 11.20854089337319870, 1414.996442620860080, 222.5314268542019818 ) ) ;
#103169=DIRECTION ( 'NONE',  ( 0.000000000000000000, 1.000000000000000000, 0.000000000000000000 ) ) ;
#103171=CARTESIAN_POINT ( 'NONE',  ( 2.771712507760000221, 1509.009850720929990, 238.2056319702980147 ) ) ;
#103172=CARTESIAN_POINT ( 'NONE',  ( 40.01057657059909900, 1448.816588776699973, 135.4138680875709895 ) ) ;
#103175=ORIENTED_EDGE ( 'NONE', *, *, #64415, .T. ) ;
#103177=CARTESIAN_POINT ( 'NONE',  ( 11.95523955411000117, 1433.542691738470012, 149.9852572030879969 ) ) ;
#103178=CARTESIAN_POINT ( 'NONE',  ( 26.65386906330000016, 1508.586510756630105, 215.9800495173180082 ) ) ;
#103179=VERTEX_POINT ( 'NONE', #5751 ) ;
#103182=DIRECTION ( 'NONE',  ( 0.000000000000000000, 1.000000000000000000, 0.000000000000000000 ) ) ;
#103183=CARTESIAN_POINT ( 'NONE',  ( 16.00482466429749806, 1421.840373356649934, 191.1776750418199811 ) ) ;
#103184=CARTESIAN_POINT ( 'NONE',  ( 4.418986906789999836, 1428.481734779130193, 91.31218443469779800 ) ) ;
#103185=CARTESIAN_POINT ( 'NONE',  ( 19.18761048174300043, 1498.115689341469988, 229.1975969832560054 ) ) ;
#103186=CARTESIAN_POINT ( 'NONE',  ( 1.697557679380000017, 1507.641431191929996, 181.1359668789980049 ) ) ;
#103190=CARTESIAN_POINT ( 'NONE',  ( 36.70996913324480460, 1436.286710641320269, 134.0999999969339740 ) ) ;
#103194=CARTESIAN_POINT ( 'NONE',  ( 13.72600532257040129, 1434.976387550540039, 148.7247796194869807 ) ) ;
#103199=CARTESIAN_POINT ( 'NONE',  ( -0.7165940425340000530, 1466.721451273230059, 235.5244447404979837 ) ) ;
#103200=CARTESIAN_POINT ( 'NONE',  ( -11.92254695265209996, 1407.392238798829794, 215.8238487423210188 ) ) ;
#103207=CARTESIAN_POINT ( 'NONE',  ( 1.515709095849999910, 1508.947667959530008, 238.4644442293979978 ) ) ;
#103211=CARTESIAN_POINT ( 'NONE',  ( 21.04234019475320139, 1440.913060387330006, 222.5617771367410000 ) ) ;
#103212=CARTESIAN_POINT ( 'NONE',  ( -19.05944678440000217, 1508.258419023829902, 229.7388470496979949 ) ) ;
#103213=VERTEX_POINT ( 'NONE', #98692 ) ;
#103214=CARTESIAN_POINT ( 'NONE',  ( -13.22514030490000003, 1410.307657465529928, 189.8332610226980250 ) ) ;
#103216=CARTESIAN_POINT ( 'NONE',  ( -10.79382126600000014, 1414.913060387329779, 196.1395803457980094 ) ) ;
#103218=CARTESIAN_POINT ( 'NONE',  ( 22.94699394379999902, 1432.795231260740138, 217.1269739022579870 ) ) ;
#103223=CARTESIAN_POINT ( 'NONE',  ( 5.398680167209999325, 1433.945743868580166, 154.6429197126979886 ) ) ;
#103235=CARTESIAN_POINT ( 'NONE',  ( 27.41412850780000099, 1466.213804920729899, 262.1296345509980483 ) ) ;
#103237=CARTESIAN_POINT ( 'NONE',  ( 2.787859546404547917, 1451.851357346741679, 183.8246711244312053 ) ) ;
#103239=CARTESIAN_POINT ( 'NONE',  ( -3.692180645651279569, 1507.990633139789907, 236.8685678891660018 ) ) ;
#103241=AXIS2_PLACEMENT_3D ( 'NONE', #99670, #22960, #100771 ) ;
#103242=CARTESIAN_POINT ( 'NONE',  ( 11.87300248480000064, 1432.863459016110028, 150.3956791023980202 ) ) ;
#103243=CARTESIAN_POINT ( 'NONE',  ( 19.03008511520000212, 1457.014020104829797, 226.0360847140979956 ) ) ;
#103248=CARTESIAN_POINT ( 'NONE',  ( 0.1080140957969999982, 1405.749477561829963, 267.5371647991979671 ) ) ;
#103249=CARTESIAN_POINT ( 'NONE',  ( 27.72455317350000215, 1507.994297268330001, 207.7087345480979934 ) ) ;
#103250=AXIS2_PLACEMENT_3D ( 'NONE', #6391, #32692, #14780 ) ;
#103255=CARTESIAN_POINT ( 'NONE',  ( -43.73019116030650366, 1440.913060406610157, 264.0439818999259955 ) ) ;
#103257=CARTESIAN_POINT ( 'NONE',  ( 3.774758283729999557E-15, 1461.407663422529822, 243.9198229339980060 ) ) ;
#103261=CYLINDRICAL_SURFACE ( 'NONE', #24154, 0.9999999999999465983 ) ;
#103263=CARTESIAN_POINT ( 'NONE',  ( 0.3331981960608920157, 1408.924696555890023, 186.0526659833350038 ) ) ;
#103266=CARTESIAN_POINT ( 'NONE',  ( -33.91369110859999836, 1435.681798638700002, 135.0664268289980043 ) ) ;
#103267=CARTESIAN_POINT ( 'NONE',  ( 5.417888360169999669E-14, 1475.048391926230124, 269.6500679732980075 ) ) ;
#103271=CARTESIAN_POINT ( 'NONE',  ( 19.74164504280149757, 1455.376031929259852, 226.0788368184279875 ) ) ;
#103277=CARTESIAN_POINT ( 'NONE',  ( -17.40764059099999628, 1414.996444526030018, 207.5654758040780052 ) ) ;
#103279=CARTESIAN_POINT ( 'NONE',  ( 24.61958478200000044, 1435.541888381590070, 137.0853135175979958 ) ) ;
#103280=CARTESIAN_POINT ( 'NONE',  ( -8.998480011645090926, 1396.227294235010049, 202.6956182965139988 ) ) ;
#103282=CARTESIAN_POINT ( 'NONE',  ( -16.90341314920719995, 1409.749895306139933, 225.4593008893319848 ) ) ;
#103283=CARTESIAN_POINT ( 'NONE',  ( 11.96519809220000141, 1440.444625599219989, 147.6189886498980002 ) ) ;
#103284=ORIENTED_EDGE ( 'NONE', *, *, #13099, .F. ) ;
#103285=ORIENTED_EDGE ( 'NONE', *, *, #42666, .F. ) ;
#103288=DIRECTION ( 'NONE',  ( -0.01486624123577086690, -0.9944765560314704489, -0.1039007910234840543 ) ) ;
#103291=CARTESIAN_POINT ( 'NONE',  ( -11.25103233189999941, 1433.013630249540029, 151.5370651328979932 ) ) ;
#103293=CARTESIAN_POINT ( 'NONE',  ( -2.557132965088358745, 1420.768154751241354, 185.5685875094732751 ) ) ;
#103296=CARTESIAN_POINT ( 'NONE',  ( 8.313290118299999421, 1507.316777386929971, 183.0869028357980142 ) ) ;
#103299=DIRECTION ( 'NONE',  ( 1.000000000000000000, 0.000000000000000000, 1.942890293094025713E-13 ) ) ;
#103302=CARTESIAN_POINT ( 'NONE',  ( -41.15075926320000121, 1443.752932596629989, 136.9300405401980072 ) ) ;
#103303=ADVANCED_FACE ( 'NONE', ( #55069 ), #33790, .F. ) ;
#103304=FACE_OUTER_BOUND ( 'NONE', #48029, .T. ) ;
#103305=CARTESIAN_POINT ( 'NONE',  ( -2.255308465020000153, 1472.005448226929957, 270.0715991240979861 ) ) ;
#103306=CARTESIAN_POINT ( 'NONE',  ( 12.32497982002866266, 1434.251326250639295, 147.3969771501246839 ) ) ;
#103307=CARTESIAN_POINT ( 'NONE',  ( -0.5851024498960000209, 1486.106971620530203, 181.8803045006980028 ) ) ;
#103312=CARTESIAN_POINT ( 'NONE',  ( -36.33136068457189793, 1451.260137002700048, 135.5554792738989818 ) ) ;
#103313=ADVANCED_FACE ( 'NONE', ( #29288 ), #82907, .F. ) ;
#103314=CARTESIAN_POINT ( 'NONE',  ( -2.500000000000000000, 1448.203469879150134, 169.7706540686479855 ) ) ;
#103316=CARTESIAN_POINT ( 'NONE',  ( 13.58011004080560014, 1408.357478272720073, 204.5339713451270143 ) ) ;
#103317=CARTESIAN_POINT ( 'NONE',  ( -10.48381364300569984, 1407.657513889099846, 269.6151450982960114 ) ) ;
#103318=CARTESIAN_POINT ( 'NONE',  ( -13.75801960019769865, 1434.977933834450141, 148.5785497869700009 ) ) ;
#103319=VERTEX_POINT ( 'NONE', #25819 ) ;
#103320=CARTESIAN_POINT ( 'NONE',  ( 3.658687503250000361, 1424.106386281430105, 183.9658221167980230 ) ) ;
#103321=CARTESIAN_POINT ( 'NONE',  ( 13.57984947760000161, 1443.954740135339762, 188.4659268699979862 ) ) ;
#103324=VERTEX_POINT ( 'NONE', #50512 ) ;
#103325=CARTESIAN_POINT ( 'NONE',  ( 4.796254352853694058, 1422.272280406457867, 184.2473515962519173 ) ) ;
#103329=CARTESIAN_POINT ( 'NONE',  ( -17.77992640079999731, 1470.471868837129932, 189.4977790897980015 ) ) ;
#103331=CIRCLE ( 'NONE', #37264, 29.84605316648919526 ) ;
#103334=VECTOR ( 'NONE', #56388, 1000.000000000000114 ) ;
#103336=CARTESIAN_POINT ( 'NONE',  ( 9.986924024219998586, 1415.932617990029939, 224.5919156272979933 ) ) ;
#103338=CARTESIAN_POINT ( 'NONE',  ( -28.15433623620000247, 1508.637654267429980, 208.1158776034079949 ) ) ;
#103343=CARTESIAN_POINT ( 'NONE',  ( -4.131009387019999757, 1408.874545657929957, 195.5701569932979851 ) ) ;
#103344=CARTESIAN_POINT ( 'NONE',  ( -12.57480364899999969, 1409.852123968930073, 227.8141353385980210 ) ) ;
#103345=CARTESIAN_POINT ( 'NONE',  ( -12.41052241149999880, 1445.069700341559837, 185.9600454165980068 ) ) ;
#103347=CARTESIAN_POINT ( 'NONE',  ( -24.08291145960179946, 1411.090674597109910, 208.6097594128350181 ) ) ;
#103348=CARTESIAN_POINT ( 'NONE',  ( 27.02980867440000168, 1488.688182087729956, 211.4493640585079959 ) ) ;
#103350=CARTESIAN_POINT ( 'NONE',  ( -25.04275794140000144, 1435.378124283050056, 135.9084131103979871 ) ) ;
#103357=EDGE_LOOP ( 'NONE', ( #63444, #55575, #37492, #52634 ) ) ;
#103358=CARTESIAN_POINT ( 'NONE',  ( -26.39367551872020101, 1440.913056983640217, 211.7580267479229974 ) ) ;
#103359=CARTESIAN_POINT ( 'NONE',  ( -2.832144297430000179, 1410.303523779030002, 232.5720248812980060 ) ) ;
#103363=CARTESIAN_POINT ( 'NONE',  ( 11.60004869885203682, 1411.254281879943164, 135.5999999980979851 ) ) ;
#103364=CARTESIAN_POINT ( 'NONE',  ( 12.48155824441049866, 1435.524277019780129, 150.9067716058439714 ) ) ;
#103366=CARTESIAN_POINT ( 'NONE',  ( 15.64058445933870090, 1488.407880391730032, 230.9639646109729938 ) ) ;
#103367=CARTESIAN_POINT ( 'NONE',  ( -24.40973383587160228, 1509.744644423489945, 224.4882036239870047 ) ) ;
#103368=CARTESIAN_POINT ( 'NONE',  ( -1.674594060629999825, 1409.138563759730005, 186.6870598632980034 ) ) ;
#103373=CARTESIAN_POINT ( 'NONE',  ( 19.58834138799999991, 1508.062712335030028, 188.7849770318979949 ) ) ;
#103375=B_SPLINE_CURVE_WITH_KNOTS ( 'NONE', 3,
 ( #31492, #108758, #6300, #32609, #65672, #32050, #99790, #66239, #15228, #83544, #6838, #73528, #109867, #92494, #40997, #107662, #75176, #109326, #65123, #675, #70105, #51070, #34805, #84648, #67884, #94150, #77373, #59480, #110410, #131, #16867, #25279, #68437, #68993, #93591, #101993, #27506, #85200, #103094, #60589, #8487, #42661, #26394, #95815, #76816, #34254, #94709, #69546, #52728, #77917, #7945, #102540, #9596, #52181, #86863 ),
 .UNSPECIFIED., .F., .F.,
 ( 4, 2, 2, 1, 2, 2, 2, 2, 2, 2, 2, 2, 2, 2, 2, 2, 1, 1, 2, 2, 2, 2, 1, 1, 2, 2, 2, 2, 2, 4 ),
 ( 0.000000000000000000, 0.06250000000056427085, 0.09375000000084640628, 0.1093750000009878487, 0.1171875000010581952, 0.1250000000011285139, 0.1875000000010392243, 0.2187500000009074685, 0.2500000000007757128, 0.3750000000002559064, 0.4374999999998605560, 0.4999999999994652056, 0.5624999999990698551, 0.5937499999988681276, 0.6249999999986662891, 0.6874999999985312860, 0.7187499999984703347, 0.7343749999985430543, 0.7421874999986711741, 0.7499999999987991828, 0.8124999999987877475, 0.8437499999987821964, 0.8593749999987091437, 0.8671874999986661781, 0.8710937499986443067, 0.8749999999986225463, 0.9062499999989295230, 0.9218749999990830668, 0.9374999999992364996, 1.000000000000000000 ),
 .UNSPECIFIED. ) ;
#103380=CARTESIAN_POINT ( 'NONE',  ( 2.523331955360000212, 1419.463757169429982, 185.1820755668979643 ) ) ;
#103386=CARTESIAN_POINT ( 'NONE',  ( -3.709912251880000067, 1447.069507299949919, 154.3963887763979983 ) ) ;
#103389=CARTESIAN_POINT ( 'NONE',  ( -5.001772368710000194, 1443.913060387330006, 150.4106346902979965 ) ) ;
#103390=CARTESIAN_POINT ( 'NONE',  ( 15.84151803160000327, 1416.228840385830154, 191.3509196118980071 ) ) ;
#103392=CARTESIAN_POINT ( 'NONE',  ( 0.5834642750313309145, 1464.825178575939844, 188.3591715439980021 ) ) ;
#103396=CARTESIAN_POINT ( 'NONE',  ( 27.08643475359999897, 1507.996733211630044, 207.0060423009980184 ) ) ;
#103398=EDGE_CURVE ( 'NONE', #96461, #91877, #100787, .T. ) ;
#103402=EDGE_CURVE ( 'NONE', #86024, #43369, #13922, .T. ) ;
#103404=PLANE ( 'NONE',  #5527 ) ;
#103408=CARTESIAN_POINT ( 'NONE',  ( 12.98226561589999939, 1414.913060387329779, 198.3280246956980193 ) ) ;
#103410=AXIS2_PLACEMENT_3D ( 'NONE', #81188, #73360, #4505 ) ;
#103411=CARTESIAN_POINT ( 'NONE',  ( 16.56219860610000083, 1451.518047273530101, 149.1091192963980063 ) ) ;
#103414=CARTESIAN_POINT ( 'NONE',  ( 25.00063024130000144, 1509.786765447930065, 193.6023525624979982 ) ) ;
#103416=CARTESIAN_POINT ( 'NONE',  ( -1.471222536434999784, 1414.913526854310021, 226.2200213458429801 ) ) ;
#103418=CARTESIAN_POINT ( 'NONE',  ( 18.18137504628520063, 1507.546748557000001, 186.5307075251750177 ) ) ;
#103420=ORIENTED_EDGE ( 'NONE', *, *, #109763, .F. ) ;
#103421=CARTESIAN_POINT ( 'NONE',  ( 14.09542765070000137, 1445.387346742360023, 189.3996806953979899 ) ) ;
#103422=B_SPLINE_CURVE_WITH_KNOTS ( 'NONE', 3,
 ( #82795, #48670, #67125, #6090, #39697, #83344, #74974, #24524, #50329 ),
 .UNSPECIFIED., .F., .F.,
 ( 4, 1, 2, 2, 4 ),
 ( 0.000000000000000000, 0.2500000000000182632, 0.3750000000000175970, 0.5000000000000169864, 1.000000000000000000 ),
 .UNSPECIFIED. ) ;
#103424=CARTESIAN_POINT ( 'NONE',  ( 37.27029739945400166, 1438.078572600510142, 136.5691528236939973 ) ) ;
#103425=CARTESIAN_POINT ( 'NONE',  ( 13.57505907252250310, 1412.033808172750469, 269.3590162744131931 ) ) ;
#103426=CARTESIAN_POINT ( 'NONE',  ( -42.47347404569999441, 1448.912595586219823, 263.9447133204980105 ) ) ;
#103429=CARTESIAN_POINT ( 'NONE',  ( -12.06466153778595540, 1435.468980856949202, 151.1548757136271774 ) ) ;
#103430=CARTESIAN_POINT ( 'NONE',  ( -18.72407526530000155, 1458.246115540929850, 227.3156487912980026 ) ) ;
#103433=CARTESIAN_POINT ( 'NONE',  ( 2.216568699310000223, 1409.495539288629971, 185.7088051529979964 ) ) ;
#103434=CARTESIAN_POINT ( 'NONE',  ( 4.098401964949999865, 1424.674504371229887, 185.1777059284979998 ) ) ;
#103435=CARTESIAN_POINT ( 'NONE',  ( -11.26681287859999969, 1433.831804755629946, 151.5577293853980052 ) ) ;
#103436=CARTESIAN_POINT ( 'NONE',  ( 9.894254036040001310, 1435.855537113729724, 152.5794184490980001 ) ) ;
#103437=CARTESIAN_POINT ( 'NONE',  ( -4.500000000000000000, 1448.210448412289907, 170.2811368938980081 ) ) ;
#103438=CARTESIAN_POINT ( 'NONE',  ( -6.301803161020000488, 1452.256379489029996, 153.3432975151980031 ) ) ;
#103442=EDGE_CURVE ( 'NONE', #58469, #38935, #49889, .T. ) ;
#103444=CARTESIAN_POINT ( 'NONE',  ( -42.57409307820000066, 1450.173233224009891, 270.2305074514979992 ) ) ;
#103446=CARTESIAN_POINT ( 'NONE',  ( 16.81340943980000091, 1409.500197579730184, 223.0320505808980158 ) ) ;
#103449=CARTESIAN_POINT ( 'NONE',  ( 11.16733641199999916, 1453.313060387329870, 192.7512321736979857 ) ) ;
#103452=CARTESIAN_POINT ( 'NONE',  ( -8.076961596850001257, 1418.814380367629838, 233.3636024205979993 ) ) ;
#103454=CARTESIAN_POINT ( 'NONE',  ( 0.1595995995380000143, 1486.508831850330125, 181.8147405652979671 ) ) ;
#103456=CARTESIAN_POINT ( 'NONE',  ( -46.07249033020909934, 1438.837360396860049, 268.2071385507119885 ) ) ;
#103464=CARTESIAN_POINT ( 'NONE',  ( 19.34249370211351504, 1456.699829906176774, 224.6011546362110778 ) ) ;
#103466=EDGE_CURVE ( 'NONE', #19775, #23739, #70120, .T. ) ;
#103467=CARTESIAN_POINT ( 'NONE',  ( -26.56033579598179983, 1451.985519570539964, 134.9300129401310073 ) ) ;
#103468=EDGE_LOOP ( 'NONE', ( #29270, #96933, #58049, #90153 ) ) ;
#103469=CARTESIAN_POINT ( 'NONE',  ( 4.500000000000000000, 1411.429641636930000, 126.8043280305979863 ) ) ;
#103472=EDGE_CURVE ( 'NONE', #50075, #46649, #1618, .T. ) ;
#103473=CARTESIAN_POINT ( 'NONE',  ( 11.60004869885204037, 1422.941107825514564, 135.6422303046223306 ) ) ;
#103479=CARTESIAN_POINT ( 'NONE',  ( -4.868932048487660147, 1409.401550909529988, 270.3706725577400221 ) ) ;
#103481=CARTESIAN_POINT ( 'NONE',  ( 6.407815220088149744, 1418.463448909649969, 232.9647645899679844 ) ) ;
#103486=EDGE_CURVE ( 'NONE', #80080, #52184, #91029, .T. ) ;
#103487=CARTESIAN_POINT ( 'NONE',  ( -23.81627866638899960, 1411.112638069600280, 210.1641640956580090 ) ) ;
#103489=CARTESIAN_POINT ( 'NONE',  ( 3.650560473782963555, 1424.964407230763072, 184.9206000695610896 ) ) ;
#103490=CARTESIAN_POINT ( 'NONE',  ( -5.339448499717754260, 1406.221036493157044, 266.9498660043132077 ) ) ;
#103494=CARTESIAN_POINT ( 'NONE',  ( -18.06981095964670203, 1413.146983966680182, 195.1848155250099808 ) ) ;
#103495=CARTESIAN_POINT ( 'NONE',  ( -17.79320747690000104, 1415.861465824730203, 225.5139460155979805 ) ) ;
#103496=AXIS2_PLACEMENT_3D ( 'NONE', #108625, #90156, #6711 ) ;
#103497=CARTESIAN_POINT ( 'NONE',  ( 36.97629126828699953, 1461.966573722429985, 266.9662940315810147 ) ) ;
#103498=CARTESIAN_POINT ( 'NONE',  ( -1.832174820364002032, 1466.979387277607429, 235.3086100617430532 ) ) ;
#103501=ORIENTED_EDGE ( 'NONE', *, *, #31031, .T. ) ;
#103502=CARTESIAN_POINT ( 'NONE',  ( 21.74861278406057252, 1411.032916471346880, 216.6292070377826633 ) ) ;
#103504=CARTESIAN_POINT ( 'NONE',  ( 22.83404369579999837, 1409.737016915530148, 208.6318390177190167 ) ) ;
#103507=CARTESIAN_POINT ( 'NONE',  ( 24.32398584962239951, 1452.063651768310137, 136.1369888671689807 ) ) ;
#103511=CARTESIAN_POINT ( 'NONE',  ( 17.37907441389999974, 1410.017153215830149, 192.8320702375980318 ) ) ;
#103512=CARTESIAN_POINT ( 'NONE',  ( 17.22592482065188335, 1443.913060387329779, 162.9227486220069352 ) ) ;
#103513=DIRECTION ( 'NONE',  ( 1.000000000000000000, 0.000000000000000000, 0.000000000000000000 ) ) ;
#103515=CARTESIAN_POINT ( 'NONE',  ( -21.37277430946751267, 1428.837918873476156, 219.6028782859573880 ) ) ;
#103522=CARTESIAN_POINT ( 'NONE',  ( 17.11714618750000128, 1444.740067931809790, 162.7561046190980107 ) ) ;
#103526=CARTESIAN_POINT ( 'NONE',  ( -16.68599179819999989, 1461.099982565929849, 230.2790296985980092 ) ) ;
#103528=CARTESIAN_POINT ( 'NONE',  ( -9857.840209715130186, 50.13405481578730161, -1086.115145476999942 ) ) ;
#103529=ADVANCED_FACE ( 'NONE', ( #50379 ), #772, .F. ) ;
#103533=B_SPLINE_CURVE_WITH_KNOTS ( 'NONE', 3,
 ( #99763, #49389, #8869, #91387, #99208, #74595, #108732, #65096, #22487, #75149, #94530, #56687, #83516, #82978, #17804, #66757, #40969, #25666, #23052, #93983, #107633, #48295, #90824, #82438, #57260, #14105, #14665, #17249, #81867, #23616, #51442, #5735, #73500, #74045, #39878, #48854, #108174 ),
 .UNSPECIFIED., .F., .F.,
 ( 4, 3, 3, 3, 3, 3, 3, 3, 3, 3, 3, 3, 4 ),
 ( -69.20990094339998677, -67.35627552521479799, -65.67677515525750209, -64.13305301190000307, -63.72413547986320026, -62.52805632474360209, -61.28625140089109635, -60.00527021219100021, -58.62934261228799926, -57.23376785416390078, -55.62731357942359978, -53.66775153965929945, -51.68681987860000504 ),
 .UNSPECIFIED. ) ;
#103534=CARTESIAN_POINT ( 'NONE',  ( -14.97660074559999899, 1451.660971642529830, 219.6133832206979832 ) ) ;
#103535=CARTESIAN_POINT ( 'NONE',  ( -2.156670372940499902, 1451.947498740930087, 184.5271336820339911 ) ) ;
#103536=CARTESIAN_POINT ( 'NONE',  ( 11.20455999689999871, 1433.617589470330131, 151.5998260058979952 ) ) ;
#103537=CARTESIAN_POINT ( 'NONE',  ( 3.108624468949999707E-15, 1461.407663422529822, 243.9198229339980060 ) ) ;
#103544=CARTESIAN_POINT ( 'NONE',  ( -4.696284960629999894, 1486.251895520230164, 182.0546551604979868 ) ) ;
#103545=CARTESIAN_POINT ( 'NONE',  ( -13.98457847890000139, 1414.635582449330059, 227.2382995055980075 ) ) ;
#103546=CARTESIAN_POINT ( 'NONE',  ( -30.15184734697509938, 1510.043527037290005, 208.7857410632290112 ) ) ;
#103547=AXIS2_PLACEMENT_3D ( 'NONE', #12067, #46257, #37830 ) ;
#103548=CARTESIAN_POINT ( 'NONE',  ( 25.61862525230000287, 1449.804154363369889, 210.1382241221579932 ) ) ;
#103549=DIRECTION ( 'NONE',  ( -0.9995237709234254808, 0.03085824620771311644, -1.986951185180850780E-13 ) ) ;
#103550=CARTESIAN_POINT ( 'NONE',  ( 25.71670629617132064, 1436.648920519811327, 137.1099281659991220 ) ) ;
#103555=CARTESIAN_POINT ( 'NONE',  ( 0.1620797138729939690, 1485.018021426579935, 181.8788060555280026 ) ) ;
#103556=CARTESIAN_POINT ( 'NONE',  ( -18.18137268718939836, 1507.546750198529935, 231.7129778879169635 ) ) ;
#103558=CARTESIAN_POINT ( 'NONE',  ( -1.546867746950000067, 1416.839692131129823, 228.0214409762979813 ) ) ;
#103562=CARTESIAN_POINT ( 'NONE',  ( -3.008615722576569951, 1440.893621901990173, 157.1951554466570258 ) ) ;
#103566=ORIENTED_EDGE ( 'NONE', *, *, #64461, .T. ) ;
#103568=FACE_OUTER_BOUND ( 'NONE', #16967, .T. ) ;
#103570=CARTESIAN_POINT ( 'NONE',  ( -14.11509852220000028, 1414.913060387329779, 218.5043773088879959 ) ) ;
#103571=CARTESIAN_POINT ( 'NONE',  ( -2.739840682029376584, 1509.032634909519629, 238.5893384668526096 ) ) ;
#103576=CARTESIAN_POINT ( 'NONE',  ( 13.80599399769999991, 1434.979619872729927, 146.4346935412979747 ) ) ;
#103579=CARTESIAN_POINT ( 'NONE',  ( -17.03916695150000038, 1411.910831074529824, 191.9225384856980270 ) ) ;
#103581=ORIENTED_EDGE ( 'NONE', *, *, #17484, .T. ) ;
#103583=CARTESIAN_POINT ( 'NONE',  ( -15.73147536331710050, 1409.565876699960199, 225.8795040344060112 ) ) ;
#103585=VERTEX_POINT ( 'NONE', #51461 ) ;
#103590=CARTESIAN_POINT ( 'NONE',  ( 25.58984387490000145, 1507.958107147929923, 218.7218739854080241 ) ) ;
#103593=EDGE_CURVE ( 'NONE', #62909, #42879, #90084, .T. ) ;
#103594=CARTESIAN_POINT ( 'NONE',  ( 18.44501327497894749, 1468.322017823991700, 269.3810620050319926 ) ) ;
#103596=CARTESIAN_POINT ( 'NONE',  ( 15.23211778679590545, 1430.904153654725633, 219.7804539585919770 ) ) ;
#103597=CARTESIAN_POINT ( 'NONE',  ( 2.124286289930000127, 1417.654161064629989, 233.3475255464980194 ) ) ;
#103599=CARTESIAN_POINT ( 'NONE',  ( -9.496501384368448484, 1440.505055584230377, 186.7254819606929175 ) ) ;
#103601=DIRECTION ( 'NONE',  ( 1.000000000000000000, 0.000000000000000000, 0.000000000000000000 ) ) ;
#103605=CARTESIAN_POINT ( 'NONE',  ( -13.04141444983799936, 1435.645536544770039, 150.5902749682459785 ) ) ;
#103606=B_SPLINE_SURFACE_WITH_KNOTS ( 'NONE', 5, 5, ( 
 ( #106766, #65350, #30057, #5417, #64248, #56386 ),
 ( #98370, #21643, #14351, #90518, #91068, #108430 ),
 ( #14902, #55848, #13244, #47434, #22736, #97814 ),
 ( #13793, #82117, #39577, #56939, #48543, #82681 ),
 ( #23306, #49093, #5971, #83228, #6518, #40671 ),
 ( #29512, #63704, #18072, #66457, #69072, #61239 ),
 ( #7071, #66996, #49640, #69629, #101107, #26475 ),
 ( #103751, #103172, #41228, #27053, #95353, #18613 ),
 ( #43304, #27592, #23849, #85842, #78553, #15449 ),
 ( #104302, #100568, #58041, #9141, #92178, #10235 ),
 ( #60111, #109537, #83777, #86391, #86944, #52267 ),
 ( #60670, #52813, #87514, #61777, #25913, #95901 ) ),
 .UNSPECIFIED., .F., .F., .F.,
 ( 6, 3, 3, 6 ),
 ( 6, 6 ),
 ( 18.22821421442209910, 21.75967651710000084, 24.82024664080000065, 32.41288959079599863 ),
 ( -8.204439600732860269E-05, 1.512517455850000081 ),
 .UNSPECIFIED. ) ;
#103607=CARTESIAN_POINT ( 'NONE',  ( -2.500000000000000000, 1437.833057476529802, 157.6748628238979961 ) ) ;
#103608=CARTESIAN_POINT ( 'NONE',  ( -7.127716695479999294E-11, 1475.057956560229968, 269.6447263235979790 ) ) ;
#103610=ORIENTED_EDGE ( 'NONE', *, *, #108576, .F. ) ;
#103611=EDGE_CURVE ( 'NONE', #65361, #6784, #61542, .T. ) ;
#103614=CARTESIAN_POINT ( 'NONE',  ( 41.56052307180000582, 1438.341700298520209, 261.5689801973979911 ) ) ;
#103615=CARTESIAN_POINT ( 'NONE',  ( -23.79684662080000024, 1410.916736090329778, 207.4665339750179953 ) ) ;
#103616=CARTESIAN_POINT ( 'NONE',  ( -11.34549315327149976, 1426.458520874449960, 115.9708627263430003 ) ) ;
#103617=CARTESIAN_POINT ( 'NONE',  ( 16.81493322035340299, 1409.874137557720132, 192.4133040450060150 ) ) ;
#103619=CARTESIAN_POINT ( 'NONE',  ( 7.683404440216066611, 1509.309260261254394, 180.0625472504430888 ) ) ;
#103620=DIRECTION ( 'NONE',  ( -0.000000000000000000, -0.000000000000000000, 1.000000000000000000 ) ) ;
#103622=CARTESIAN_POINT ( 'NONE',  ( -28.68961640089999676, 1414.662827630530046, 264.4914002609979775 ) ) ;
#103624=CARTESIAN_POINT ( 'NONE',  ( 17.48489369962524620, 1459.987562467892076, 228.4085929379347135 ) ) ;
#103626=CARTESIAN_POINT ( 'NONE',  ( -38.33296738232420608, 1438.937668912289837, 136.6331331180969926 ) ) ;
#103628=CARTESIAN_POINT ( 'NONE',  ( 7.629428199119460352, 1397.829558206759884, 197.4986098258069944 ) ) ;
#103631=CARTESIAN_POINT ( 'NONE',  ( -16.87366308760000067, 1458.693985979230092, 229.6006262403980145 ) ) ;
#103633=ORIENTED_EDGE ( 'NONE', *, *, #58768, .T. ) ;
#103637=CARTESIAN_POINT ( 'NONE',  ( 0.3635313643190000166, 1421.820591800929833, 227.3960884296979827 ) ) ;
#103641=CARTESIAN_POINT ( 'NONE',  ( 26.92366755636065889, 1508.479994616119484, 206.2224058939788733 ) ) ;
#103642=CARTESIAN_POINT ( 'NONE',  ( 17.79018706778330028, 1578.884106212270126, 161.8975890202569872 ) ) ;
#103644=PLANE ( 'NONE',  #75398 ) ;
#103649=ORIENTED_EDGE ( 'NONE', *, *, #11781, .T. ) ;
#103650=CARTESIAN_POINT ( 'NONE',  ( 11.86538456922300000, 1432.285977292769985, 149.9821679606649809 ) ) ;
#103655=CARTESIAN_POINT ( 'NONE',  ( -17.22654844235838567, 1443.913060387328869, 162.9224179604370590 ) ) ;
#103657=CARTESIAN_POINT ( 'NONE',  ( -4.853079720760000271, 1422.238069890129964, 185.0630658123980083 ) ) ;
#103659=CARTESIAN_POINT ( 'NONE',  ( 2.255304544822630319, 1409.820689363890097, 270.0715902656349954 ) ) ;
#103667=CARTESIAN_POINT ( 'NONE',  ( 15.57416844496259856, 1507.336002650009959, 225.6913864299219767 ) ) ;
#103668=CARTESIAN_POINT ( 'NONE',  ( 17.69747404500670029, 1413.849660306819715, 224.8943591048869735 ) ) ;
#103671=AXIS2_PLACEMENT_3D ( 'NONE', #44488, #78633, #36086 ) ;
#103672=CARTESIAN_POINT ( 'NONE',  ( 18.02574679518840028, 1424.482682570480165, 224.6196048480980210 ) ) ;
#103673=CARTESIAN_POINT ( 'NONE',  ( 41.39118081080529521, 1446.191675961305009, 135.3420714969400649 ) ) ;
#103674=CARTESIAN_POINT ( 'NONE',  ( -3.054816033052110136, 1485.996906143959905, 182.1538611115439892 ) ) ;
#103681=CARTESIAN_POINT ( 'NONE',  ( -2.339614227286648696, 1449.682732101595775, 154.4221585652428246 ) ) ;
#103682=CARTESIAN_POINT ( 'NONE',  ( -10.92547548560405168, 1429.189822794765632, 151.1096517011108062 ) ) ;
#103687=CARTESIAN_POINT ( 'NONE',  ( 11.68080434900000064, 1412.737827518229778, 229.2464092685980290 ) ) ;
#103689=CARTESIAN_POINT ( 'NONE',  ( -15.99364927919999779, 1459.641266709229967, 228.9570266767980229 ) ) ;
#103692=CARTESIAN_POINT ( 'NONE',  ( 18.10151846899999839, 1409.478927776330011, 269.5454010446980533 ) ) ;
#103693=CARTESIAN_POINT ( 'NONE',  ( 23.06010171139999798, 1435.302639552910023, 139.4254245235980250 ) ) ;
#103694=CARTESIAN_POINT ( 'NONE',  ( 23.77245939000000163, 1449.721689247069889, 203.1279807519480016 ) ) ;
#103695=CARTESIAN_POINT ( 'NONE',  ( -22.72361341210000063, 1432.255922540859956, 217.6431687005280082 ) ) ;
#103696=LINE ( 'NONE', #70139, #89262 ) ;
#103698=CARTESIAN_POINT ( 'NONE',  ( -1.632217591109999866, 1452.043058095030119, 184.0584959782980263 ) ) ;
#103699=CARTESIAN_POINT ( 'NONE',  ( -6.224176945601150202, 1407.473636839899882, 197.7087082607250181 ) ) ;
#103702=CARTESIAN_POINT ( 'NONE',  ( -13.73335268700000000, 1441.669543367469942, 188.5645195036979942 ) ) ;
#103703=CARTESIAN_POINT ( 'NONE',  ( 18.89942246145942306, 1416.835807492850108, 210.6687153380977122 ) ) ;
#103704=CARTESIAN_POINT ( 'NONE',  ( -30.19569990680000160, 1436.880670734120258, 136.6769221344979712 ) ) ;
#103708=CARTESIAN_POINT ( 'NONE',  ( -14.61215934965860086, 1409.423328235749977, 212.1943553262919977 ) ) ;
#103709=B_SPLINE_SURFACE_WITH_KNOTS ( 'NONE', 2, 5, ( 
 ( #79170, #9189, #18119, #27642, #86438, #51751 ),
 ( #25957, #78600, #96505, #34384, #36595, #95401 ),
 ( #61828, #53413, #103801, #27100, #103216, #52863 ) ),
 .UNSPECIFIED., .F., .F., .F.,
 ( 3, 3 ),
 ( 6, 6 ),
 ( 1.399803019409999960, 2.016961153150000019 ),
 ( 0.000000000000000000, 1.000000000000000000 ),
 .UNSPECIFIED. ) ;
#103710=CYLINDRICAL_SURFACE ( 'NONE', #64526, 2.000000000000001776 ) ;
#103712=CARTESIAN_POINT ( 'NONE',  ( -21.73253653299999755, 1471.283060775529975, 269.3316831886979799 ) ) ;
#103714=CARTESIAN_POINT ( 'NONE',  ( 0.2302574898499950007, 1419.640707946279917, 184.3378087949079998 ) ) ;
#103715=CARTESIAN_POINT ( 'NONE',  ( -24.16750533216984564, 1444.510136686808892, 211.5893432462075339 ) ) ;
#103717=CARTESIAN_POINT ( 'NONE',  ( -24.68077630836099701, 1437.736159206269804, 210.5119845322900005 ) ) ;
#103718=CARTESIAN_POINT ( 'NONE',  ( 18.71502584834279759, 1425.461731811239815, 226.6158928661320147 ) ) ;
#103719=CARTESIAN_POINT ( 'NONE',  ( 21.92460402160000044, 1509.678684430729845, 227.7046112463980023 ) ) ;
#103720=CARTESIAN_POINT ( 'NONE',  ( 1.665334536940000025E-15, 1434.541756592460160, 155.4759165859979930 ) ) ;
#103721=B_SPLINE_CURVE_WITH_KNOTS ( 'NONE', 3,
 ( #16856, #109316, #25268, #24168 ),
 .UNSPECIFIED., .F., .F.,
 ( 4, 4 ),
 ( 7.189030196343478827E-14, 0.002384643111680485698 ),
 .UNSPECIFIED. ) ;
#103725=CARTESIAN_POINT ( 'NONE',  ( -22.30007645030000063, 1409.691796216729927, 207.3274002725380285 ) ) ;
#103726=CARTESIAN_POINT ( 'NONE',  ( 14.38361772900000091, 1416.219761279530076, 196.8926598285980276 ) ) ;
#103727=EDGE_CURVE ( 'NONE', #64952, #77609, #29562, .T. ) ;
#103732=B_SPLINE_SURFACE_WITH_KNOTS ( 'NONE', 5, 5, ( 
 ( #29138, #30225, #63866, #63327, #19625, #97982, #21248, #36981, #89588 ),
 ( #39177, #28032, #64414, #98536, #13411, #47599, #81725, #87966, #5033 ),
 ( #62222, #11256, #108599, #83388, #16167, #67168, #31887, #7786, #41952 ),
 ( #64962, #50370, #90684, #6130, #40843, #22354, #23482, #92336, #107487 ),
 ( #22911, #92893, #7244, #15608, #99075, #49814, #31330, #32979, #40286 ),
 ( #100198, #84496, #56556, #6686, #13972, #48160, #57118, #83944, #100728 ),
 ( #91244, #41405, #101267, #30782, #82296, #24013, #75572, #5595, #66628 ),
 ( #39744, #14524, #75016, #109166, #109705, #73908, #74471, #99624, #108036 ),
 ( #65517, #32452, #48715, #82838, #66073, #58208, #57674, #91788, #15064 ),
 ( #24564, #58755, #49262, #85584, #8329, #86156, #110801, #8879, #87264 ),
 ( #95111, #43061, #42493, #86706, #52572, #77221, #94542, #43612, #9999 ),
 ( #85038, #18376, #103497, #110246, #102932, #101829, #93437, #35758, #522 ),
 ( #34647, #68285, #26235, #93995, #10558, #76105, #76650, #102393, #68831 ),
 ( #27348, #25122, #60424, #78306, #16706, #61533, #104056, #59326, #50908 ),
 ( #34093, #44169, #95663, #59868, #25676, #17260, #9448, #1622, #17815 ),
 ( #60986, #51452, #69942, #33519, #52014, #18930, #77762, #1072, #35199 ),
 ( #69386, #53127, #26799, #67721, #37417, #98410, #104614, #54781, #62092 ),
 ( #71050, #97852, #37968, #70496, #105172, #21127, #38503, #55888, #27910 ),
 ( #55334, #21682, #3841, #79425, #90007, #28463, #20581, #88913, #12760 ),
 ( #54243, #36857, #44732, #11125, #2187, #46394, #78882, #36301, #96217 ),
 ( #53696, #19494, #62656, #81059, #89466, #80525, #12199, #88369, #87837 ) ),
 .UNSPECIFIED., .F., .F., .F.,
 ( 6, 3, 3, 3, 3, 3, 6 ),
 ( 6, 3, 6 ),
 ( 23.99353787332109889, 34.04292652270000019, 49.85499997250000348, 65.66707342230000677, 82.30866304890000151, 98.98173700649999773, 143.2994570502170006 ),
 ( -0.0001774529578859669783, 1.000000000000000000, 2.000198712178860028 ),
 .UNSPECIFIED. ) ;
#103743=CARTESIAN_POINT ( 'NONE',  ( -0.8933028310894340907, 1419.625179221010058, 184.8271038220919991 ) ) ;
#103748=CARTESIAN_POINT ( 'NONE',  ( 2.277483798560000050, 1508.992591874329946, 237.8394411828980139 ) ) ;
#103751=CARTESIAN_POINT ( 'NONE',  ( 40.04388406862929628, 1448.778234248659828, 134.9800677253420247 ) ) ;
#103754=EDGE_CURVE ( 'NONE', #19757, #105869, #46118, .T. ) ;
#103756=CARTESIAN_POINT ( 'NONE',  ( 11.60507608815730052, 1433.884017739829915, 151.1942475904019716 ) ) ;
#103760=CARTESIAN_POINT ( 'NONE',  ( -23.59414818020000126, 1507.884704231529895, 195.6683835580979860 ) ) ;
#103762=CARTESIAN_POINT ( 'NONE',  ( -14.69331829855070026, 1452.091493848030041, 222.9975758587799817 ) ) ;
#103763=CARTESIAN_POINT ( 'NONE',  ( 7.214502255410000231, 1427.316505021429975, 144.1938086916980239 ) ) ;
#103766=CARTESIAN_POINT ( 'NONE',  ( 6.609130007410000118, 1488.167526812230108, 183.3322403809980301 ) ) ;
#103768=CARTESIAN_POINT ( 'NONE',  ( 15.70989997510000080, 1409.628288509730055, 226.4425047134980105 ) ) ;
#103770=CARTESIAN_POINT ( 'NONE',  ( 14.20217058005079913, 1415.778512723909898, 197.1139478086609813 ) ) ;
#103773=ORIENTED_EDGE ( 'NONE', *, *, #15514, .F. ) ;
#103774=CARTESIAN_POINT ( 'NONE',  ( 13.81140031233439913, 1434.980667563419956, 148.6522636971369877 ) ) ;
#103776=B_SPLINE_CURVE_WITH_KNOTS ( 'NONE', 3,
 ( #3484, #44939, #52226, #27012, #79636, #71254, #70705, #28665, #20245, #37613, #88039, #11323, #86354, #96422 ),
 .UNSPECIFIED., .F., .F.,
 ( 4, 2, 2, 2, 2, 2, 4 ),
 ( 0.000000000000000000, 0.0005712213022518396709, 0.001142442604503679342, 0.001713663906755519013, 0.002284885209007358683, 0.003427327813511035857, 0.004569770418014713030 ),
 .UNSPECIFIED. ) ;
#103778=ORIENTED_EDGE ( 'NONE', *, *, #13293, .F. ) ;
#103781=CIRCLE ( 'NONE', #71610, 2.000000000000000000 ) ;
#103786=CARTESIAN_POINT ( 'NONE',  ( -19.08997683846052951, 1441.125342513460055, 209.8663685049180003 ) ) ;
#103788=CARTESIAN_POINT ( 'NONE',  ( 4.256778553939329690, 1446.547191167049959, 160.0313428239830102 ) ) ;
#103789=EDGE_CURVE ( 'NONE', #22625, #68839, #95464, .T. ) ;
#103790=CARTESIAN_POINT ( 'NONE',  ( 0.9272409414739999356, 1508.839993243730078, 238.3381952508979964 ) ) ;
#103791=ORIENTED_EDGE ( 'NONE', *, *, #10991, .F. ) ;
#103793=ORIENTED_EDGE ( 'NONE', *, *, #86265, .F. ) ;
#103796=CARTESIAN_POINT ( 'NONE',  ( -18.63535451609999782, 1508.532394786730038, 229.9190513451980280 ) ) ;
#103797=ORIENTED_EDGE ( 'NONE', *, *, #18482, .F. ) ;
#103799=CARTESIAN_POINT ( 'NONE',  ( -13.84714808919999918, 1409.396613453830014, 191.2465958026980104 ) ) ;
#103800=CARTESIAN_POINT ( 'NONE',  ( -24.67281693759999683, 1441.610155857880045, 210.7086710232079838 ) ) ;
#103801=CARTESIAN_POINT ( 'NONE',  ( -10.79382126600000014, 1414.913060387329779, 196.1395803457980094 ) ) ;
#103803=CARTESIAN_POINT ( 'NONE',  ( 26.31342956949939804, 1441.279830909470093, 137.8584465659640159 ) ) ;
#103805=CARTESIAN_POINT ( 'NONE',  ( 17.05308613158098652, 1435.093823724508866, 146.1608033541734244 ) ) ;
#103811=CARTESIAN_POINT ( 'NONE',  ( 29.61947514750000110, 1509.969965907130018, 207.5603945732279954 ) ) ;
#103813=CARTESIAN_POINT ( 'NONE',  ( 42.06232107555830169, 1440.913060387330006, 269.6487541170399709 ) ) ;
#103814=CARTESIAN_POINT ( 'NONE',  ( -17.27690404115233846, 1486.136442936737922, 187.9034219468923368 ) ) ;
#103816=VERTEX_POINT ( 'NONE', #3849 ) ;
#103818=CARTESIAN_POINT ( 'NONE',  ( 27.70845952490000030, 1450.383243101060089, 238.1060716476980019 ) ) ;
#103820=CARTESIAN_POINT ( 'NONE',  ( -28.27428436538610157, 1509.900420154179983, 216.9929459379879972 ) ) ;
#103821=CARTESIAN_POINT ( 'NONE',  ( -3.662605128175850489, 1507.447374573099978, 236.6990675022970265 ) ) ;
#103822=CARTESIAN_POINT ( 'NONE',  ( -21.04541642230000065, 1454.767645325029889, 223.1813744721980015 ) ) ;
#103823=CARTESIAN_POINT ( 'NONE',  ( 10.97839330989999951, 1432.873337069130002, 151.7696626780980012 ) ) ;
#103824=CARTESIAN_POINT ( 'NONE',  ( 19.24454973920000000, 1455.981838887030108, 226.3136641516979921 ) ) ;
#103829=CARTESIAN_POINT ( 'NONE',  ( 1.297592866489999927E-09, 1405.775964805530066, 268.4837719564979466 ) ) ;
#103832=CARTESIAN_POINT ( 'NONE',  ( 12.98581290379999942, 1428.689068522430034, 223.6918876029980083 ) ) ;
#103833=CARTESIAN_POINT ( 'NONE',  ( 5.436747755899999923, 1437.112761795790220, 154.7095357218980212 ) ) ;
#103834=CARTESIAN_POINT ( 'NONE',  ( -26.99540727154380093, 1450.681735027889999, 136.4489462876310313 ) ) ;
#103836=CARTESIAN_POINT ( 'NONE',  ( -42.29870041503930622, 1440.913060411070092, 262.3297496996750056 ) ) ;
#103837=CARTESIAN_POINT ( 'NONE',  ( -26.84535680910000011, 1449.047047365870185, 136.7368231881980023 ) ) ;
#103838=CARTESIAN_POINT ( 'NONE',  ( 4.363122647530000009, 1414.776585547029981, 163.8086717993979846 ) ) ;
#103843=CARTESIAN_POINT ( 'NONE',  ( -42.06231979437640689, 1440.913089571769888, 269.6487552725350270 ) ) ;
#103844=EDGE_LOOP ( 'NONE', ( #57649, #41331, #87099, #15254, #13787, #71637, #14947, #98810 ) ) ;
#103845=CARTESIAN_POINT ( 'NONE',  ( 0.5133626083067620582, 1410.311097044259895, 185.0719925509139898 ) ) ;
#103849=CARTESIAN_POINT ( 'NONE',  ( -0.8130327484720001330, 1417.377572236629931, 235.4819850726979951 ) ) ;
#103854=CARTESIAN_POINT ( 'NONE',  ( -18.04709463619999710, 1415.245980412329800, 207.8128127142179835 ) ) ;
#103857=CARTESIAN_POINT ( 'NONE',  ( 5.389719913101400195, 1440.971386073809981, 154.8246291173960003 ) ) ;
#103859=AXIS2_PLACEMENT_3D ( 'NONE', #42965, #93893, #67623 ) ;
#103860=CARTESIAN_POINT ( 'NONE',  ( -17.03291860866149676, 1409.881251985120116, 225.5426873045980187 ) ) ;
#103861=CARTESIAN_POINT ( 'NONE',  ( 2.446787376320000096, 1432.353341358199941, 150.2884730787980061 ) ) ;
#103863=ORIENTED_EDGE ( 'NONE', *, *, #34397, .F. ) ;
#103866=CARTESIAN_POINT ( 'NONE',  ( 11.09190030210000089, 1426.903748879130035, 97.30362720369791418 ) ) ;
#103869=CARTESIAN_POINT ( 'NONE',  ( 4.311753873931529313, 1425.506783100830035, 185.4196544955500201 ) ) ;
#103870=CARTESIAN_POINT ( 'NONE',  ( -2.497703869279095379, 1421.154004695713866, 184.9625613379778315 ) ) ;
#103873=CARTESIAN_POINT ( 'NONE',  ( 7.829163140769999529, 1507.896460528530042, 182.8030300680979963 ) ) ;
#103880=CARTESIAN_POINT ( 'NONE',  ( -41.66090858750000336, 1443.836096447190130, 135.6920785174980040 ) ) ;
#103881=LINE ( 'NONE', #68104, #63699 ) ;
#103882=CARTESIAN_POINT ( 'NONE',  ( -2.245209799710000009, 1471.752125626330098, 269.8658162814979846 ) ) ;
#103885=CARTESIAN_POINT ( 'NONE',  ( 23.34540950859999953, 1507.878524956530100, 194.4697486434980078 ) ) ;
#103888=CARTESIAN_POINT ( 'NONE',  ( -35.12460981859439357, 1451.531087103250002, 135.5516170584860163 ) ) ;
#103890=CARTESIAN_POINT ( 'NONE',  ( 18.02093535799999913, 1424.326836137830014, 225.1991050518980160 ) ) ;
#103892=CARTESIAN_POINT ( 'NONE',  ( 13.75707076230000148, 1408.364212814029997, 211.9527283592179856 ) ) ;
#103893=CARTESIAN_POINT ( 'NONE',  ( -0.7631012575699189782, 1406.777862902510151, 269.6501330761860231 ) ) ;
#103894=CARTESIAN_POINT ( 'NONE',  ( -14.38420833757800033, 1435.582840502069757, 149.6588806134069785 ) ) ;
#103895=ORIENTED_EDGE ( 'NONE', *, *, #69666, .F. ) ;
#103896=CARTESIAN_POINT ( 'NONE',  ( -2.500000000000000000, 1440.913060387330006, 209.1218459616979999 ) ) ;
#103897=CARTESIAN_POINT ( 'NONE',  ( 13.27118260120000137, 1442.692795410319832, 188.6610245367980099 ) ) ;
#103910=CARTESIAN_POINT ( 'NONE',  ( -28.31645363330000009, 1509.601692267130147, 205.7529699828779997 ) ) ;
#103912=CARTESIAN_POINT ( 'NONE',  ( 11.87502392341400004, 1433.007271648830056, 149.9804723818110119 ) ) ;
#103917=CARTESIAN_POINT ( 'NONE',  ( -4.043557851940000170, 1446.816496427589982, 184.5928732699980230 ) ) ;
#103918=ORIENTED_EDGE ( 'NONE', *, *, #38793, .F. ) ;
#103919=CARTESIAN_POINT ( 'NONE',  ( 28.25319066630000009, 1451.926638454029899, 134.8820817050979883 ) ) ;
#103920=CARTESIAN_POINT ( 'NONE',  ( -24.88581067337899810, 1440.913060480750119, 215.3118859389570048 ) ) ;
#103922=CARTESIAN_POINT ( 'NONE',  ( -24.78163162830000132, 1435.369157292130012, 136.0792171752979982 ) ) ;
#103931=CARTESIAN_POINT ( 'NONE',  ( 2.500000000000000000, 1439.077099669189920, 157.7246394012979920 ) ) ;
#103932=CARTESIAN_POINT ( 'NONE',  ( -12.75379259890000050, 1412.829786118129960, 228.0544790036979919 ) ) ;
#103934=ORIENTED_EDGE ( 'NONE', *, *, #69455, .F. ) ;
#103936=VECTOR ( 'NONE', #4697, 1000.000000000000227 ) ;
#103938=CARTESIAN_POINT ( 'NONE',  ( 12.05097526569999822, 1434.216276041280025, 150.6184982174980007 ) ) ;
#103939=CARTESIAN_POINT ( 'NONE',  ( 17.73694109413560227, 1478.710361465350161, 229.1951871287480174 ) ) ;
#103942=CARTESIAN_POINT ( 'NONE',  ( -0.06620051369889999593, 1409.084365175830044, 232.6715855378979825 ) ) ;
#103943=CARTESIAN_POINT ( 'NONE',  ( 2.879377773099999871, 1417.724437854929874, 234.4927649805979968 ) ) ;
#103945=FACE_OUTER_BOUND ( 'NONE', #85588, .T. ) ;
#103946=CARTESIAN_POINT ( 'NONE',  ( 18.65749896639999861, 1509.387464492230038, 187.4422726698979886 ) ) ;
#103949=CARTESIAN_POINT ( 'NONE',  ( -13.02322915955869931, 1416.825783990419950, 196.6108486074699897 ) ) ;
#103950=CARTESIAN_POINT ( 'NONE',  ( -20.63236152680000046, 1508.913060324029857, 189.5446908899980087 ) ) ;
#103951=ORIENTED_EDGE ( 'NONE', *, *, #24856, .F. ) ;
#103956=DIRECTION ( 'NONE',  ( -8.453952912920146445E-06, -0.03084653019238408483, 0.9995241325268845456 ) ) ;
#103959=CARTESIAN_POINT ( 'NONE',  ( 18.06884258770000073, 1415.263254653229978, 210.5556769813279914 ) ) ;
#103960=CARTESIAN_POINT ( 'NONE',  ( -18.67603340750000029, 1425.535634798130104, 226.2166979841979924 ) ) ;
#103965=CARTESIAN_POINT ( 'NONE',  ( -19.06177424568263845, 1440.331832736574825, 209.7871912064330786 ) ) ;
#103968=CARTESIAN_POINT ( 'NONE',  ( 1.551173678986830007, 1415.834070661230044, 190.5513134611869930 ) ) ;
#103969=CARTESIAN_POINT ( 'NONE',  ( -9221.844916327461760, 50.28429875023816464, -5636.577220017842592 ) ) ;
#103970=CARTESIAN_POINT ( 'NONE',  ( -24.32341588750000128, 1436.131012997689822, 210.7992627561380061 ) ) ;
#103971=CARTESIAN_POINT ( 'NONE',  ( 4.098232394932746381, 1410.432529984579560, 186.0633403236960248 ) ) ;
#103972=CARTESIAN_POINT ( 'NONE',  ( -4.107671006832890548, 1426.017999997803372, 186.1051448316069354 ) ) ;
#103975=FACE_OUTER_BOUND ( 'NONE', #48698, .T. ) ;
#103980=CARTESIAN_POINT ( 'NONE',  ( -15.56983240930392043, 1506.527232285067157, 224.7512174644303684 ) ) ;
#103981=CARTESIAN_POINT ( 'NONE',  ( 11.49747574013809981, 1416.913060341719984, 220.3427041143820020 ) ) ;
#103982=CARTESIAN_POINT ( 'NONE',  ( 22.97053994450000047, 1507.867546928429874, 193.7497404625980266 ) ) ;
#103984=CARTESIAN_POINT ( 'NONE',  ( -1.441539424119999913, 1414.983771850430003, 226.5042059068979938 ) ) ;
#103987=ORIENTED_EDGE ( 'NONE', *, *, #77840, .T. ) ;
#103989=CARTESIAN_POINT ( 'NONE',  ( 17.88477383430709722, 1509.485346479319787, 231.9786773698629929 ) ) ;
#103991=CARTESIAN_POINT ( 'NONE',  ( 13.13626245617426669, 1443.056086229705443, 169.4004656986877819 ) ) ;
#103992=CARTESIAN_POINT ( 'NONE',  ( 19.92213876099999936, 1452.807100928230057, 209.3894951820489894 ) ) ;
#103993=CARTESIAN_POINT ( 'NONE',  ( -26.19682434950000172, 1465.282665911629920, 259.6167014773980100 ) ) ;
#103997=CARTESIAN_POINT ( 'NONE',  ( 26.88792401699999957, 1508.603612559529893, 206.2262326685279845 ) ) ;
#103998=CARTESIAN_POINT ( 'NONE',  ( -19.83538623540000145, 1485.649277471630057, 190.4852910309980132 ) ) ;
#103999=CARTESIAN_POINT ( 'NONE',  ( 2.641394305209999960, 1409.510112843430079, 185.8263422457980028 ) ) ;
#104000=CARTESIAN_POINT ( 'NONE',  ( 5.950109296629999989, 1421.372702594429938, 186.2244564570979719 ) ) ;
#104001=CARTESIAN_POINT ( 'NONE',  ( -6.017144072120000686, 1442.258634816289941, 154.7968030204980039 ) ) ;
#104003=CYLINDRICAL_SURFACE ( 'NONE', #64508, 2.000000000000000000 ) ;
#104009=CARTESIAN_POINT ( 'NONE',  ( -39.10257508149999950, 1457.313645690129988, 270.0008335182980090 ) ) ;
#104011=( BOUNDED_SURFACE ( )  B_SPLINE_SURFACE ( 2, 1, ( 
 ( #79237, #28825 ),
 ( #61902, #29357 ),
 ( #88734, #89271 ),
 ( #88184, #104976 ),
 ( #4176, #12568 ),
 ( #79791, #54057 ),
 ( #46748, #37225 ),
 ( #46197, #80880 ),
 ( #11476, #63022 ),
 ( #38308, #80332 ),
 ( #28264, #45098 ) ),
 .UNSPECIFIED., .T., .F., .F. ) 
 B_SPLINE_SURFACE_WITH_KNOTS ( ( 3, 2, 2, 2, 2, 3 ),
 ( 2, 2 ),
 ( 1.721761971665859647, 3.141592653589790007, 4.712388980384689674, 6.283185307179590673, 7.853981633974480125, 8.004947278845451208 ),
 ( -17.86299485559450062, 35.72598970969769994 ),
 .UNSPECIFIED. ) 
 GEOMETRIC_REPRESENTATION_ITEM ( )  RATIONAL_B_SPLINE_SURFACE ( (
 ( 0.9491121336701279221, 0.9491121336701279221),
 ( 0.7352560790313750205, 0.7352560790313750205),
 ( 1.000000000000000000, 1.000000000000000000),
 ( 0.7071067811865510144, 0.7071067811865510144),
 ( 1.000000000000000000, 1.000000000000000000),
 ( 0.7071067811865510144, 0.7071067811865510144),
 ( 1.000000000000000000, 1.000000000000000000),
 ( 0.7071067811865510144, 0.7071067811865510144),
 ( 1.000000000000000000, 1.000000000000000000),
 ( 0.9718507021551759939, 0.9718507021551759939),
 ( 0.9491121336701279221, 0.9491121336701279221) ) ) 
 REPRESENTATION_ITEM ( '' )  SURFACE ( )  );
#104012=CARTESIAN_POINT ( 'NONE',  ( 17.63079482879999915, 1410.452322071830167, 223.6591261867980052 ) ) ;
#104018=CARTESIAN_POINT ( 'NONE',  ( -6.279660886640000328, 1416.867457637430107, 231.6963788028980105 ) ) ;
#104019=CARTESIAN_POINT ( 'NONE',  ( -1.108701933971497633, 1484.799112515838033, 182.1781186121703513 ) ) ;
#104021=CARTESIAN_POINT ( 'NONE',  ( -44.70539842100279770, 1432.153755970550264, 268.2536652372499475 ) ) ;
#104022=CARTESIAN_POINT ( 'NONE',  ( -2.499999999990000443, 1434.166392531650217, 184.3332466033980097 ) ) ;
#104023=ORIENTED_EDGE ( 'NONE', *, *, #102328, .T. ) ;
#104033=CARTESIAN_POINT ( 'NONE',  ( -16.19086242769280304, 1409.478452467050147, 225.0103265570539861 ) ) ;
#104037=CARTESIAN_POINT ( 'NONE',  ( 1.800204229380000243, 1413.682656150029970, 232.3423579875980067 ) ) ;
#104038=CARTESIAN_POINT ( 'NONE',  ( -11.44665353847253186, 1425.798163151176823, 139.1345268192609126 ) ) ;
#104042=CARTESIAN_POINT ( 'NONE',  ( -1.800556938495289971, 1410.057666395089882, 269.8656564991380264 ) ) ;
#104044=CARTESIAN_POINT ( 'NONE',  ( 7.833511190420000325, 1418.000725493129949, 231.1317660673979901 ) ) ;
#104047=VERTEX_POINT ( 'NONE', #32329 ) ;
#104048=EDGE_LOOP ( 'NONE', ( #59383, #36083, #49104, #90240, #19498 ) ) ;
#104049=CARTESIAN_POINT ( 'NONE',  ( -22.57316855434390135, 1409.701313687740139, 209.4509182103790010 ) ) ;
#104051=CARTESIAN_POINT ( 'NONE',  ( -0.2723609444870630503, 1409.428891713289886, 185.2334270307050019 ) ) ;
#104052=CARTESIAN_POINT ( 'NONE',  ( 3.651998852415098362, 1424.315861867868080, 184.2127881604313586 ) ) ;
#104053=CARTESIAN_POINT ( 'NONE',  ( -28.90443088959890261, 1413.811766471930923, 266.6320645011991814 ) ) ;
#104054=CARTESIAN_POINT ( 'NONE',  ( -20.62644837504292283, 1436.449369547013475, 144.7505193540382322 ) ) ;
#104055=CARTESIAN_POINT ( 'NONE',  ( -20.78701115710000025, 1430.788020833330165, 221.2610285622980086 ) ) ;
#104056=CARTESIAN_POINT ( 'NONE',  ( 32.91329245024750350, 1465.287215665440044, 268.8838783738780194 ) ) ;
#104058=CARTESIAN_POINT ( 'NONE',  ( 8.739359048380000772, 1447.264120250649967, 186.1039452748980239 ) ) ;
#104060=ORIENTED_EDGE ( 'NONE', *, *, #27771, .T. ) ;
#104062=CARTESIAN_POINT ( 'NONE',  ( 1.530052826864370052, 1452.704406626560058, 183.4894965714629791 ) ) ;
#104063=CARTESIAN_POINT ( 'NONE',  ( 22.96024162530000368, 1409.741098516330112, 208.8471077697990097 ) ) ;
#104066=CARTESIAN_POINT ( 'NONE',  ( 26.39039547659079687, 1451.532858036890048, 136.1253493193630106 ) ) ;
#104067=CARTESIAN_POINT ( 'NONE',  ( 16.09743769923632328, 1409.475195298647122, 225.1611831289835379 ) ) ;
#104070=CARTESIAN_POINT ( 'NONE',  ( 18.81211946219999831, 1410.932182625230098, 194.9082043907980051 ) ) ;
#104071=CARTESIAN_POINT ( 'NONE',  ( 27.73716673060003757, 1444.324653571829003, 175.8274728504979976 ) ) ;
#104072=CARTESIAN_POINT ( 'NONE',  ( 2.606044709233462875, 1439.644608576006249, 183.4134873266624766 ) ) ;
#104073=CARTESIAN_POINT ( 'NONE',  ( 1.103328532679999974, 1417.357629882630135, 234.6276851089980084 ) ) ;
#104074=CARTESIAN_POINT ( 'NONE',  ( -19.49500888343222371, 1425.635160192849980, 223.3892665050759945 ) ) ;
#104075=CARTESIAN_POINT ( 'NONE',  ( 0.7396591144891080383, 1450.952091773529901, 181.9981990658489792 ) ) ;
#104076=AXIS2_PLACEMENT_3D ( 'NONE', #32815, #101112, #24408 ) ;
#104081=ORIENTED_EDGE ( 'NONE', *, *, #57074, .T. ) ;
#104084=CARTESIAN_POINT ( 'NONE',  ( -0.5133638609672289688, 1410.311096993930050, 233.1717005261690190 ) ) ;
#104086=CARTESIAN_POINT ( 'NONE',  ( -9829.078716724869082, 2833.596074015789782, -1083.720023828399917 ) ) ;
#104090=CARTESIAN_POINT ( 'NONE',  ( 0.3175620880625033005, 1506.436298843700342, 231.1045490282727144 ) ) ;
#104091=VECTOR ( 'NONE', #40762, 1000.000000000000114 ) ;
#104092=CARTESIAN_POINT ( 'NONE',  ( -20.41675352909999930, 1440.913060387330006, 219.6133834379979817 ) ) ;
#104093=CARTESIAN_POINT ( 'NONE',  ( 5.319460837823512200, 1475.837047823878947, 266.9611527779425728 ) ) ;
#104095=CARTESIAN_POINT ( 'NONE',  ( 11.79714158089999998, 1433.102084680620010, 150.6246159734980097 ) ) ;
#104096=CARTESIAN_POINT ( 'NONE',  ( 19.02913997099999932, 1445.216574189620133, 214.3676144204279694 ) ) ;
#104100=CARTESIAN_POINT ( 'NONE',  ( 22.81156273903739873, 1507.439214557190098, 209.9480014011130038 ) ) ;
#104102=CARTESIAN_POINT ( 'NONE',  ( -12.21452983799999892, 1486.126195478929958, 184.5549420154979998 ) ) ;
#104103=CARTESIAN_POINT ( 'NONE',  ( 8.704405229141865874, 1398.171440019795000, 199.4642630465137358 ) ) ;
#104104=CARTESIAN_POINT ( 'NONE',  ( -29.60289517418189931, 1509.946814196759988, 211.8389432164699713 ) ) ;
#104106=CARTESIAN_POINT ( 'NONE',  ( 20.10054293860000030, 1449.792076505040086, 223.0884697793979967 ) ) ;
#104108=CARTESIAN_POINT ( 'NONE',  ( -41.66135440509999910, 1443.796918820770088, 135.6885369501979994 ) ) ;
#104114=CARTESIAN_POINT ( 'NONE',  ( 0.1680335629641069861, 1481.486285909129947, 182.0305442892730241 ) ) ;
#104116=VERTEX_POINT ( 'NONE', #91124 ) ;
#104120=CARTESIAN_POINT ( 'NONE',  ( -38.71265708134060191, 1449.925712785010091, 134.0999999982089719 ) ) ;
#104121=ORIENTED_EDGE ( 'NONE', *, *, #109055, .F. ) ;
#104126=CARTESIAN_POINT ( 'NONE',  ( -16.56387270879999818, 1416.216596894629902, 216.8457408595079983 ) ) ;
#104127=CARTESIAN_POINT ( 'NONE',  ( -3.289824944146642505, 1509.047015717335171, 238.5027799606278620 ) ) ;
#104132=CARTESIAN_POINT ( 'NONE',  ( 14.59686494579730009, 1409.422794143049941, 212.2812494645380355 ) ) ;
#104135=CARTESIAN_POINT ( 'NONE',  ( -17.81798938879999739, 1417.753250616630112, 193.2359899303979773 ) ) ;
#104138=EDGE_CURVE ( 'NONE', #75798, #94093, #57091, .T. ) ;
#104140=CARTESIAN_POINT ( 'NONE',  ( -18.46871759262399948, 1509.558002187349757, 227.6992299154879902 ) ) ;
#104141=VERTEX_POINT ( 'NONE', #51321 ) ;
#104146=CARTESIAN_POINT ( 'NONE',  ( -11.95607891459999905, 1433.549464727329905, 149.8823818600980076 ) ) ;
#104147=CARTESIAN_POINT ( 'NONE',  ( 28.81246749003422636, 1509.921441786180822, 215.1936146894269370 ) ) ;
#104149=CARTESIAN_POINT ( 'NONE',  ( 2.560697147539999996, 1397.364458149729899, 221.9069322208979997 ) ) ;
#104150=CARTESIAN_POINT ( 'NONE',  ( 2.158915719780000408, 1417.717804633830156, 234.2951490207980214 ) ) ;
#104152=CARTESIAN_POINT ( 'NONE',  ( -0.5113759145960000696, 1452.167377557530017, 183.2820360629980030 ) ) ;
#104154=DIRECTION ( 'NONE',  ( 0.000000000000000000, 0.000000000000000000, 1.000000000000000000 ) ) ;
#104155=CARTESIAN_POINT ( 'NONE',  ( -16.17567887616449696, 1459.146938910900644, 230.7169172525407532 ) ) ;
#104159=DIRECTION ( 'NONE',  ( -0.000000000000000000, -1.000000000000000000, -0.000000000000000000 ) ) ;
#104160=CARTESIAN_POINT ( 'NONE',  ( 40.97060334260000047, 1457.521043316630085, 269.1083649037979626 ) ) ;
#104163=LINE ( 'NONE', #85698, #13363 ) ;
#104164=VERTEX_POINT ( 'NONE', #87709 ) ;
#104166=CARTESIAN_POINT ( 'NONE',  ( -27.39000294650000100, 1488.691910936830027, 208.6711224243079812 ) ) ;
#104167=CARTESIAN_POINT ( 'NONE',  ( -10.01040736821559918, 1425.213511949329813, 95.14036416481241076 ) ) ;
#104168=CARTESIAN_POINT ( 'NONE',  ( 16.78176103308070211, 1409.746178557840040, 192.6058444741499898 ) ) ;
#104170=B_SPLINE_CURVE_WITH_KNOTS ( 'NONE', 3,
 ( #73334, #39159, #5576, #109149, #49245, #81706, #39726, #32432, #49793, #55988, #5012, #6668, #100714, #90111, #15047, #90666, #13394, #73892, #31867, #100180, #23994, #31315, #65498, #47581, #64945, #108018, #23463, #56538, #15589, #58190, #83926, #74999, #13950, #107468, #92318, #30766, #57657, #99059, #22338, #48139, #99607, #22891, #7228, #57101, #91226, #14506, #48696, #75553, #109687, #91769, #6112, #40269, #74453, #66056, #108580, #34078, #35738, #76091, #43595, #68271, #67704 ),
 .UNSPECIFIED., .F., .F.,
 ( 4, 3, 3, 3, 3, 3, 3, 3, 3, 3, 3, 3, 3, 3, 3, 3, 3, 3, 3, 3, 4 ),
 ( -62.49762447071550042, -60.33300340686220409, -58.10206884789899817, -55.86175009356129806, -53.61759029967220158, -51.36985323930030489, -49.12223441177160055, -46.87661061982559829, -44.63480547542509669, -42.40295230826649941, -40.17980702489999345, -38.04092854621969622, -35.81788295326150262, -33.58648471440059780, -31.35170678149719947, -29.11424439197629965, -26.87748251352680029, -24.64329050055170001, -22.41346991023220170, -20.19442837096610077, -17.98520087693835023 ),
 .UNSPECIFIED. ) ;
#104171=CARTESIAN_POINT ( 'NONE',  ( -21.31406882940000358, 1471.311257370629846, 207.5959200529579789 ) ) ;
#104172=B_SPLINE_CURVE_WITH_KNOTS ( 'NONE', 3,
 ( #54149, #94442, #981, #18839, #19956, #70962 ),
 .UNSPECIFIED., .F., .F.,
 ( 4, 2, 4 ),
 ( -1.508484740986450134, -0.7560090653526220228, -0.005718497747917217211 ),
 .UNSPECIFIED. ) ;
#104173=CARTESIAN_POINT ( 'NONE',  ( -31.95512683309999957, 1438.870446863360030, 244.1805851191980139 ) ) ;
#104174=CARTESIAN_POINT ( 'NONE',  ( 16.01892750471949611, 1509.475672623540049, 233.8163314141949911 ) ) ;
#104177=CARTESIAN_POINT ( 'NONE',  ( 30.81588940880000038, 1451.836835031929922, 135.2403377932980106 ) ) ;
#104178=VERTEX_POINT ( 'NONE', #102271 ) ;
#104179=CARTESIAN_POINT ( 'NONE',  ( 6.240881287431440327, 1397.787785794319916, 220.5258607916529741 ) ) ;
#104181=CARTESIAN_POINT ( 'NONE',  ( -16.96763829480000041, 1458.557240647530080, 230.2736757858980354 ) ) ;
#104185=CARTESIAN_POINT ( 'NONE',  ( -29.24402035022065505, 1509.934316807730966, 211.7409440427389882 ) ) ;
#104186=CARTESIAN_POINT ( 'NONE',  ( -3.199225686647339639, 1428.849802092149957, 155.3746640963260006 ) ) ;
#104187=EDGE_CURVE ( 'NONE', #2114, #33795, #87457, .T. ) ;
#104188=EDGE_LOOP ( 'NONE', ( #54281, #47428, #81576, #74634 ) ) ;
#104189=CARTESIAN_POINT ( 'NONE',  ( -1.365868668549999887, 1417.499497643730137, 185.3003514764980082 ) ) ;
#104191=DIRECTION ( 'NONE',  ( 0.9417419115949053898, -0.3363363969979660806, -9.559255346349042767E-16 ) ) ;
#104193=CARTESIAN_POINT ( 'NONE',  ( 1.422913744236389944, 1420.921243867379872, 183.0214009822149990 ) ) ;
#104197=ORIENTED_EDGE ( 'NONE', *, *, #9459, .T. ) ;
#104200=ORIENTED_EDGE ( 'NONE', *, *, #109177, .T. ) ;
#104201=CARTESIAN_POINT ( 'NONE',  ( 11.86589750230659845, 1432.321833896879980, 149.9823969317070009 ) ) ;
#104203=CARTESIAN_POINT ( 'NONE',  ( 13.21142979970633391, 1444.695576628558683, 187.3344715631244242 ) ) ;
#104204=EDGE_LOOP ( 'NONE', ( #105236, #69464, #28707, #72570 ) ) ;
#104207=CARTESIAN_POINT ( 'NONE',  ( 2.879160622090000121, 1507.714518183930068, 236.0305531890979864 ) ) ;
#104209=CARTESIAN_POINT ( 'NONE',  ( -4.746199047880000244, 1421.572606312730159, 185.9709308222979871 ) ) ;
#104210=CARTESIAN_POINT ( 'NONE',  ( 4.101683555128318837, 1410.534017730810092, 269.3367430748480160 ) ) ;
#104219=CARTESIAN_POINT ( 'NONE',  ( 17.86527779738699806, 1419.284960752339884, 225.0523055677910236 ) ) ;
#104223=CARTESIAN_POINT ( 'NONE',  ( 6.850948851990000144, 1425.447270609629868, 224.8635561661979807 ) ) ;
#104224=CARTESIAN_POINT ( 'NONE',  ( 22.62861454470000311, 1507.212883763329955, 209.7205631874760172 ) ) ;
#104232=CARTESIAN_POINT ( 'NONE',  ( -24.68922764939999936, 1444.388416874039876, 210.7939770334679963 ) ) ;
#104233=EDGE_CURVE ( 'NONE', #2577, #32822, #14139, .T. ) ;
#104234=CARTESIAN_POINT ( 'NONE',  ( -1.251355130419650408, 1450.749714363028261, 154.2555256373233590 ) ) ;
#104237=CARTESIAN_POINT ( 'NONE',  ( 5.369951645833737963, 1422.353275737341164, 139.3006397450932070 ) ) ;
#104238=CARTESIAN_POINT ( 'NONE',  ( 14.24650394540639908, 1509.423839838560298, 235.0732898097659813 ) ) ;
#104240=CARTESIAN_POINT ( 'NONE',  ( -12.54268436849999979, 1408.913060387329779, 221.6645303301980050 ) ) ;
#104241=CARTESIAN_POINT ( 'NONE',  ( 14.50036989130000009, 1415.083979989329919, 227.9808212963979770 ) ) ;
#104244=CARTESIAN_POINT ( 'NONE',  ( -16.50128791789999738, 1460.031619852429912, 228.4944370095979878 ) ) ;
#104246=CARTESIAN_POINT ( 'NONE',  ( 46.15245612160000377, 1438.899492667230106, 268.2044261578979558 ) ) ;
#104249=CARTESIAN_POINT ( 'NONE',  ( 18.93814215579999782, 1469.163538426630112, 190.4333472056979986 ) ) ;
#104250=EDGE_CURVE ( 'NONE', #43874, #94269, #85928, .T. ) ;
#104251=CARTESIAN_POINT ( 'NONE',  ( -22.98928886499999891, 1433.123621001740048, 215.0581590339280069 ) ) ;
#104253=CARTESIAN_POINT ( 'NONE',  ( -15.68560381450000207, 1410.853898355630008, 226.7268320013979803 ) ) ;
#104255=CARTESIAN_POINT ( 'NONE',  ( -1.403723453710000069, 1451.693831228530144, 183.8452497173979907 ) ) ;
#104256=CARTESIAN_POINT ( 'NONE',  ( -22.91663120903140083, 1507.606285602550088, 207.6071078552859888 ) ) ;
#104258=CARTESIAN_POINT ( 'NONE',  ( -12.57157822410000136, 1441.286360236680139, 188.0308888572979811 ) ) ;
#104260=CARTESIAN_POINT ( 'NONE',  ( -29.17524271230000110, 1436.412047157749839, 136.6555645778979908 ) ) ;
#104264=CARTESIAN_POINT ( 'NONE',  ( -14.35947579292080079, 1409.414504331519765, 213.2202510431029907 ) ) ;
#104268=CARTESIAN_POINT ( 'NONE',  ( -46.27885839279999658, 1446.077177910260161, 267.5894350431979660 ) ) ;
#104270=CARTESIAN_POINT ( 'NONE',  ( 0.1825647296195060110, 1419.920266353400166, 184.0904206890710100 ) ) ;
#104271=EDGE_CURVE ( 'NONE', #93687, #76760, #43320, .T. ) ;
#104272=CARTESIAN_POINT ( 'NONE',  ( -26.71144765010000199, 1509.845844693529898, 221.0617760641979999 ) ) ;
#104274=B_SPLINE_SURFACE_WITH_KNOTS ( 'NONE', 5, 5, ( 
 ( #12393, #28657, #72330, #102710, #71244, #60770, #17037, #54439, #62862 ),
 ( #88572, #69160, #11855, #60202, #51234, #46028, #94894, #8662, #80156 ),
 ( #3477, #71807, #18169, #105927, #94321, #42840, #29206, #43398, #63395 ),
 ( #852, #34979, #86484, #43946, #78089, #1392, #20780, #54980, #89105 ),
 ( #5660, #55523, #72868, #98045, #48222, #64484, #89650, #56616, #49319 ),
 ( #15129, #82362, #107556, #12936, #38692, #47117, #73420, #107003, #83445 ),
 ( #82903, #39808, #30291, #31395, #23543, #21319, #22413, #91853, #108099 ),
 ( #65575, #65018, #22979, #98599, #99136, #73968, #81244, #21863, #90751 ),
 ( #56062, #4559, #90189, #40347, #47663, #13473, #81790, #14590, #5093 ),
 ( #14030, #57735, #30842, #99687, #39246, #57184, #91308, #48778, #6195 ),
 ( #40898, #74528, #6740, #106460, #108659, #29744, #31947, #66141, #100264 ),
 ( #63932, #94605, #34157, #17881, #52079, #24081, #75079, #84004, #68343 ),
 ( #25183, #93497, #59937, #67778, #59386, #94054, #43122, #102449, #33585 ),
 ( #92954, #85101, #77281, #84556, #92393, #101890, #58270, #101329, #60485 ),
 ( #86211, #15666, #75630, #16768, #8390, #49870, #41470, #66684, #50971 ) ),
 .UNSPECIFIED., .F., .F., .F.,
 ( 6, 3, 3, 3, 6 ),
 ( 6, 3, 6 ),
 ( 25.13132725520000221, 26.41639650289999963, 27.94257249489999850, 28.70566049089999794, 29.46874848689999737 ),
 ( 0.000000000000000000, 1.000000000000000000, 2.000000000000000000 ),
 .UNSPECIFIED. ) ;
#104276=CARTESIAN_POINT ( 'NONE',  ( 17.59745923480189944, 1424.099926364739986, 226.7452899292189841 ) ) ;
#104277=CARTESIAN_POINT ( 'NONE',  ( 12.18581598819999989, 1415.088016306429836, 220.9247494550979809 ) ) ;
#104278=CARTESIAN_POINT ( 'NONE',  ( 14.55732100150000008, 1474.168784421129885, 223.9170786068980021 ) ) ;
#104279=CARTESIAN_POINT ( 'NONE',  ( -25.96374710035300026, 1482.712064823979972, 211.2547906125309964 ) ) ;
#104282=CARTESIAN_POINT ( 'NONE',  ( -22.74730998069999544, 1409.707413955830134, 207.2976303262279885 ) ) ;
#104283=CARTESIAN_POINT ( 'NONE',  ( 17.97082668629999702, 1416.218047894730262, 208.7667250827289820 ) ) ;
#104284=FACE_OUTER_BOUND ( 'NONE', #17264, .T. ) ;
#104289=B_SPLINE_SURFACE_WITH_KNOTS ( 'NONE', 5, 5, ( 
 ( #48755, #100765, #22954, #31924, #48198, #5636, #82336, #108636, #108076 ),
 ( #41444, #109739, #82878, #33020, #66662, #83425, #22392, #100239, #58792 ),
 ( #40877, #75056, #23519, #24054, #58248, #64997, #39786, #67207, #31371 ),
 ( #65554, #99664, #91828, #101305, #24599, #92931, #50408, #91284, #57712 ),
 ( #6172, #7821, #92371, #73395, #30821, #15643, #15106, #49298, #6721 ),
 ( #109205, #17296, #8366, #1659, #86190, #8922, #17855, #85074, #53162 ),
 ( #87304, #51492, #42534, #52608, #94032, #34132, #77799, #69980, #103537 ),
 ( #86744, #76687, #68871, #76141, #93472, #102973, #9482, #25159, #59363 ),
 ( #22586, #94579, #77258, #95150, #26271, #61027, #95700, #67755, #43097 ),
 ( #10036, #85623, #35236, #60461, #43646, #52055, #68320, #1109, #102428 ),
 ( #69424, #26840, #104096, #110285, #41991, #18410, #33561, #44207, #78350 ),
 ( #25711, #35796, #27387, #61566, #18967, #101866, #16742, #557, #50949 ) ),
 .UNSPECIFIED., .F., .F., .F.,
 ( 6, 3, 3, 6 ),
 ( 6, 3, 6 ),
 ( 0.000000000000000000, 17.84603210599999912, 40.51038747020000130, 67.03953034199999195 ),
 ( -7.105427357600000794E-15, 42.18180435250000215, 84.36360870500000431 ),
 .UNSPECIFIED. ) ;
#104290=CARTESIAN_POINT ( 'NONE',  ( -5.385728839570650628, 1432.176526655569887, 154.6052246632760045 ) ) ;
#104296=CARTESIAN_POINT ( 'NONE',  ( -23.76631617309999811, 1425.856202520030138, 210.9077545568479763 ) ) ;
#104297=CARTESIAN_POINT ( 'NONE',  ( -2.109090801651389846, 1421.166307101949997, 183.8085686438699895 ) ) ;
#104299=CARTESIAN_POINT ( 'NONE',  ( -3.565162963136402574, 1440.799174861838537, 156.6581779582986087 ) ) ;
#104300=CARTESIAN_POINT ( 'NONE',  ( -18.68342712143339668, 1486.059792560550022, 189.1570398102469994 ) ) ;
#104301=CARTESIAN_POINT ( 'NONE',  ( 1.415932851160000006, 1507.678098756430018, 236.8296152846979794 ) ) ;
#104302=CARTESIAN_POINT ( 'NONE',  ( 41.39120048966680088, 1446.191622651899934, 135.3419589341729932 ) ) ;
#104304=EDGE_LOOP ( 'NONE', ( #59877, #61262, #80890, #11248 ) ) ;
#104306=CARTESIAN_POINT ( 'NONE',  ( 11.96031942147230076, 1433.620261006660030, 150.1736231411599647 ) ) ;
#104307=CARTESIAN_POINT ( 'NONE',  ( -21.03123196678649975, 1507.789098018889945, 192.1781278620359785 ) ) ;
#104308=VERTEX_POINT ( 'NONE', #41434 ) ;
#104311=CARTESIAN_POINT ( 'NONE',  ( 9.042313521169999646, 1416.851343894929869, 218.1641597260979779 ) ) ;
#104312=CARTESIAN_POINT ( 'NONE',  ( -0.1372456665499999784, 1508.561285218730063, 180.3391500124980098 ) ) ;
#104314=CARTESIAN_POINT ( 'NONE',  ( -23.92105762916159861, 1452.077756819290016, 137.0200261151539962 ) ) ;
#104316=CARTESIAN_POINT ( 'NONE',  ( 16.66255704860000009, 1410.427173532229972, 226.4839786049979864 ) ) ;
#104318=CARTESIAN_POINT ( 'NONE',  ( 38.36650730338939752, 1437.217469518439884, 134.0999999970779868 ) ) ;
#104320=CARTESIAN_POINT ( 'NONE',  ( 18.53437515553029868, 1509.560294966549918, 227.6602647230590151 ) ) ;
#104321=ORIENTED_EDGE ( 'NONE', *, *, #12130, .F. ) ;
#104322=CARTESIAN_POINT ( 'NONE',  ( 13.76875196565650050, 1434.979433280920148, 148.6886221399630017 ) ) ;
#104326=ORIENTED_EDGE ( 'NONE', *, *, #99663, .T. ) ;
#104328=CARTESIAN_POINT ( 'NONE',  ( -0.7017359387820000238, 1466.348790855930019, 235.5986157078980057 ) ) ;
#104330=CARTESIAN_POINT ( 'NONE',  ( 21.07099741623147438, 1450.946020818080342, 144.3761871749956640 ) ) ;
#104331=DIRECTION ( 'NONE',  ( 0.000000000000000000, 1.000000000000000000, 0.000000000000000000 ) ) ;
#104333=CARTESIAN_POINT ( 'NONE',  ( -19.01838096944922540, 1443.067311164506009, 211.2996751566819569 ) ) ;
#104335=CARTESIAN_POINT ( 'NONE',  ( 4.221567158387570018, 1446.221985844579876, 169.5782296013129837 ) ) ;
#104337=CARTESIAN_POINT ( 'NONE',  ( 0.4361291165900000322, 1508.823583087030102, 238.3913694569979782 ) ) ;
#104338=ORIENTED_EDGE ( 'NONE', *, *, #24961, .F. ) ;
#104341=CARTESIAN_POINT ( 'NONE',  ( 33.01805644497149927, 1440.913060387330006, 257.7170065347000332 ) ) ;
#104343=CARTESIAN_POINT ( 'NONE',  ( -15.09146821900000113, 1507.698585867829934, 185.0194906632980008 ) ) ;
#104344=ORIENTED_EDGE ( 'NONE', *, *, #28225, .F. ) ;
#104346=CARTESIAN_POINT ( 'NONE',  ( -14.94350077410000033, 1410.807377667530091, 190.7174140115980094 ) ) ;
#104348=CARTESIAN_POINT ( 'NONE',  ( -24.38264615309999783, 1441.634144454579882, 211.3700308316280143 ) ) ;
#104350=CARTESIAN_POINT ( 'NONE',  ( 0.0002665247232048016256, 1396.263874589266152, 196.9886544196637885 ) ) ;
#104351=CARTESIAN_POINT ( 'NONE',  ( -11.87563350447849864, 1433.006677213540115, 147.6591432354780125 ) ) ;
#104352=CARTESIAN_POINT ( 'NONE',  ( -27.68841619517039732, 1441.378412040929788, 137.2953534901809860 ) ) ;
#104358=CARTESIAN_POINT ( 'NONE',  ( 28.04637368570000078, 1508.608406896529914, 208.0794640871779677 ) ) ;
#104361=CARTESIAN_POINT ( 'NONE',  ( -18.14031316878698163, 1486.179785434160522, 188.5896102339170284 ) ) ;
#104363=ORIENTED_EDGE ( 'NONE', *, *, #55112, .T. ) ;
#104365=CARTESIAN_POINT ( 'NONE',  ( 27.17992431449999913, 1457.024587824730133, 248.2870168946980129 ) ) ;
#104368=CARTESIAN_POINT ( 'NONE',  ( -11.84242369139999873, 1431.324257919750153, 147.6543138610979895 ) ) ;
#104369=CARTESIAN_POINT ( 'NONE',  ( -7.338679992370000349, 1507.281025754529992, 235.5381382512980224 ) ) ;
#104371=CARTESIAN_POINT ( 'NONE',  ( -19.02557409639999975, 1456.564017630530088, 227.5201806683979839 ) ) ;
#104373=CARTESIAN_POINT ( 'NONE',  ( -17.99954540876850118, 1410.904693920620048, 195.2564682659330231 ) ) ;
#104374=CARTESIAN_POINT ( 'NONE',  ( 19.74623141760000067, 1455.440022657330019, 226.3245780267980081 ) ) ;
#104381=ADVANCED_FACE ( 'NONE', ( #549 ), #43639, .F. ) ;
#104382=CARTESIAN_POINT ( 'NONE',  ( 40.06163307034069732, 1457.034817765570097, 269.9895890114499934 ) ) ;
#104383=CARTESIAN_POINT ( 'NONE',  ( 5.414082080120000917, 1435.477060051989838, 154.6761060569980089 ) ) ;
#104384=CARTESIAN_POINT ( 'NONE',  ( -39.67220881037469837, 1448.134517022349883, 136.4399726006329843 ) ) ;
#104387=CARTESIAN_POINT ( 'NONE',  ( -40.34049200596960105, 1440.913060404669977, 259.7628775194000355 ) ) ;
#104388=CARTESIAN_POINT ( 'NONE',  ( 37.01672902516649799, 1449.531401005109956, 136.2926409833710295 ) ) ;
#104389=CARTESIAN_POINT ( 'NONE',  ( 2.351380987493629338, 1449.654710599547343, 154.4274086630604188 ) ) ;
#104392=CARTESIAN_POINT ( 'NONE',  ( 14.43289921540000087, 1509.539432541030010, 235.4218729623979982 ) ) ;
#104393=CARTESIAN_POINT ( 'NONE',  ( 26.86204993032690069, 1508.007394616730153, 206.2315948942269870 ) ) ;
#104400=CARTESIAN_POINT ( 'NONE',  ( -0.2153814148640000037, 1475.836819236129941, 266.9611412552980028 ) ) ;
#104403=EDGE_CURVE ( 'NONE', #52385, #61381, #63368, .T. ) ;
#104406=B_SPLINE_SURFACE_WITH_KNOTS ( 'NONE', 5, 5, ( 
 ( #92901, #76113, #110253, #83951, #33527, #8336, #29416, #63615, #55206, #4769, #77769, #3706 ),
 ( #95670, #1629, #26806, #1080, #35206, #98278, #89335, #89880, #69393, #64160, #53134, #78314 ),
 ( #12631, #46808, #13150, #103504, #38913, #60993, #46264, #73095, #97732, #27356, #80938, #21554 ),
 ( #4236, #95119, #86714, #17822, #47335, #37836, #81463, #10006, #72022, #107234, #55765, #72546 ),
 ( #94549, #30525, #106677, #52023, #38371, #86163, #9455, #43621, #106138, #29968, #18383, #52580 ),
 ( #35765, #44177, #69949, #104063, #61540, #87272, #21003, #18939, #10565, #80392, #31624, #41689 ),
 ( #91542, #13699, #48457, #47886, #82023, #14819, #23216, #65256, #6979, #82595, #31074, #83681 ),
 ( #41130, #108340, #49006, #98833, #39487, #92632, #22092, #90978, #32733, #65801, #73658, #66367 ),
 ( #75848, #90420, #83142, #6436, #5885, #75311, #99922, #23767, #57416, #24319, #66913, #109454 ),
 ( #15363, #57954, #56292, #64717, #40581, #32183, #74753, #40031, #101022, #15905, #58503, #108890 ),
 ( #100486, #92087, #49555, #50106, #84231, #7533, #5327, #99367, #109998, #107790, #22640, #56846 ),
 ( #14266, #74213, #78610, #59602, #27108, #9739, #52871, #68022, #69689, #94853, #25965, #86999 ) ),
 .UNSPECIFIED., .F., .F., .F.,
 ( 6, 3, 3, 6 ),
 ( 6, 3, 3, 6 ),
 ( 6.292816022300000256, 6.725418754890000628, 7.590624220079999596, 8.366051734470000056 ),
 ( 0.000000000000000000, 0.3341520964660000259, 1.002456289399999978, 1.447932314210000015 ),
 .UNSPECIFIED. ) ;
#104407=CARTESIAN_POINT ( 'NONE',  ( -17.60960321790000194, 1415.041103191630100, 207.7251207467879794 ) ) ;
#104409=CARTESIAN_POINT ( 'NONE',  ( 26.68215560010769849, 1436.749144562530091, 136.7846546353530073 ) ) ;
#104410=CARTESIAN_POINT ( 'NONE',  ( -8.242998637256569339, 1396.200912243170023, 201.7549567842249871 ) ) ;
#104411=EDGE_CURVE ( 'NONE', #96120, #79540, #68702, .T. ) ;
#104412=CARTESIAN_POINT ( 'NONE',  ( -16.19081144212590218, 1409.478450687899795, 225.0102812049649970 ) ) ;
#104413=CARTESIAN_POINT ( 'NONE',  ( 4.926829097150000614, 1435.943783413959864, 150.1744789664979862 ) ) ;
#104415=CARTESIAN_POINT ( 'NONE',  ( -22.52564151159999639, 1509.699673122230024, 190.3321270482979912 ) ) ;
#104432=ORIENTED_EDGE ( 'NONE', *, *, #26767, .F. ) ;
#104433=VERTEX_POINT ( 'NONE', #5483 ) ;
#104435=CARTESIAN_POINT ( 'NONE',  ( 1.435309881534390097, 1482.888641461259795, 235.7288509090289779 ) ) ;
#104436=DIRECTION ( 'NONE',  ( -0.7067700376992160916, 0.03085825578589865628, -0.7067700346367981057 ) ) ;
#104441=CARTESIAN_POINT ( 'NONE',  ( 21.56891739610000158, 1409.666263584230137, 206.3502057800680234 ) ) ;
#104442=CARTESIAN_POINT ( 'NONE',  ( -2.500000000000000000, 1448.335391685370041, 163.4888273390829738 ) ) ;
#104443=CARTESIAN_POINT ( 'NONE',  ( 9.823147811128091433, 1396.256092269869896, 214.2094273585269946 ) ) ;
#104444=CARTESIAN_POINT ( 'NONE',  ( 13.63315086529999931, 1408.072387522930057, 211.9251830309279967 ) ) ;
#104445=CARTESIAN_POINT ( 'NONE',  ( -3.836741580020079923, 1405.826033084110122, 267.8481700188149830 ) ) ;
#104446=CARTESIAN_POINT ( 'NONE',  ( -14.13194304323140038, 1435.227729348820048, 149.3555327301409932 ) ) ;
#104450=ORIENTED_EDGE ( 'NONE', *, *, #81750, .T. ) ;
#104456=ORIENTED_EDGE ( 'NONE', *, *, #3739, .F. ) ;
#104466=CARTESIAN_POINT ( 'NONE',  ( -4.193343561389999863, 1409.059495171729850, 231.0986301954980036 ) ) ;
#104471=CONICAL_SURFACE ( 'NONE', #95522, 4.000000000000003553, 0.3430239404209998177 ) ;
#104474=CARTESIAN_POINT ( 'NONE',  ( -25.44254861969999837, 1435.672616488330050, 136.5529500328979964 ) ) ;
#104476=B_SPLINE_CURVE_WITH_KNOTS ( 'NONE', 3,
 ( #16169, #34649, #41954, #26801, #85041, #68833, #60426, #50372, #110248, #84498, #50910, #8331, #52574, #60988, #33522, #18378, #17817, #7246, #1075, #94544, #7788, #86158, #75574, #77764, #109707, #67171, #101270, #25678, #24567, #76108, #67723, #101831, #42495, #59870, #34095, #93998, #96219, #18933, #88915, #45286, #3843, #105737, #71617, #28465, #54783 ),
 .UNSPECIFIED., .F., .F.,
 ( 4, 2, 2, 1, 1, 2, 2, 2, 2, 1, 1, 1, 1, 2, 2, 2, 2, 2, 2, 2, 2, 1, 1, 1, 2, 2, 4 ),
 ( 0.000000000000000000, 0.1249999999994212130, 0.1874999999990521748, 0.2187499999989441779, 0.2343749999988924970, 0.2421874999988680721, 0.2499999999988436472, 0.3749999999997821742, 0.4375000000003342326, 0.4687500000005341838, 0.4843750000007066570, 0.4921875000007929768, 0.4960937500009067747, 0.4980468750009636736, 0.5000000000010205170, 0.5625000000007670531, 0.5937500000007199796, 0.6093750000006320500, 0.6250000000005442313, 0.6875000000005638823, 0.7187500000005786482, 0.7343750000005859757, 0.7421875000004842793, 0.7460937500005387912, 0.7480468750005661027, 0.7500000000005933032, 1.000000000000000000 ),
 .UNSPECIFIED. ) ;
#104480=CARTESIAN_POINT ( 'NONE',  ( 0.009664285302395179966, 1508.316642170103023, 237.8215122148098999 ) ) ;
#104482=CARTESIAN_POINT ( 'NONE',  ( 18.08349198060839313, 1410.907708222537167, 193.6100829980179583 ) ) ;
#104485=DIRECTION ( 'NONE',  ( 0.7257729707430152777, -3.515610711370605188E-08, 0.6879342955100125057 ) ) ;
#104486=CARTESIAN_POINT ( 'NONE',  ( 5.487972679035699741, 1440.608688546609983, 154.7779097438309748 ) ) ;
#104488=ORIENTED_EDGE ( 'NONE', *, *, #92401, .T. ) ;
#104491=CARTESIAN_POINT ( 'NONE',  ( 12.72506363647149996, 1434.731722876650110, 149.9707054014059793 ) ) ;
#104493=PRODUCT ( 'Grinder Body', 'Grinder Body', '', ( #49376 ) ) ;
#104494=CARTESIAN_POINT ( 'NONE',  ( 15.34910765019810164, 1478.706085042730138, 230.6431425157049944 ) ) ;
#104495=CARTESIAN_POINT ( 'NONE',  ( -22.38397194849720151, 1509.390755197840008, 226.7792598521729985 ) ) ;
#104496=CARTESIAN_POINT ( 'NONE',  ( -2.193532793379999735, 1410.364270746530110, 186.3820960473979937 ) ) ;
#104498=CARTESIAN_POINT ( 'NONE',  ( -0.1069634773768380065, 1420.455459563880140, 182.7125832242149954 ) ) ;
#104500=CARTESIAN_POINT ( 'NONE',  ( -2.919622620539999769, 1419.522956624030030, 186.2043862055979844 ) ) ;
#104504=CARTESIAN_POINT ( 'NONE',  ( -11.73069774347650096, 1414.913057862230062, 197.7037919276860123 ) ) ;
#104505=CARTESIAN_POINT ( 'NONE',  ( -16.20888296009999863, 1485.913060386929828, 186.2979123506979988 ) ) ;
#104507=CARTESIAN_POINT ( 'NONE',  ( 3.410503593230000074, 1419.799443580629941, 185.4204322456980094 ) ) ;
#104508=EDGE_CURVE ( 'NONE', #33349, #27375, #105761, .T. ) ;
#104509=B_SPLINE_CURVE_WITH_KNOTS ( 'NONE', 5,
 ( #8401, #37, #109779, #25747, #67792, #34717 ),
 .UNSPECIFIED., .F., .F.,
 ( 6, 6 ),
 ( 0.000000000000000000, 0.09439357723473694450 ),
 .UNSPECIFIED. ) ;
#104513=CARTESIAN_POINT ( 'NONE',  ( -26.35583388131840010, 1508.014892778499870, 201.5454125265999892 ) ) ;
#104515=CARTESIAN_POINT ( 'NONE',  ( 18.34708879960000161, 1415.579607672129896, 210.0281939247909975 ) ) ;
#104516=CARTESIAN_POINT ( 'NONE',  ( -17.72811920550000053, 1424.454094666429910, 227.0280627830979938 ) ) ;
#104517=CARTESIAN_POINT ( 'NONE',  ( -22.01249284969999920, 1435.265941330599844, 141.1946398826979703 ) ) ;
#104520=CARTESIAN_POINT ( 'NONE',  ( 17.88646199680000137, 1428.770680955329908, 191.8789351869980067 ) ) ;
#104522=CARTESIAN_POINT ( 'NONE',  ( -18.98465183149178159, 1439.320828499731761, 210.1502228767389227 ) ) ;
#104526=CARTESIAN_POINT ( 'NONE',  ( 25.24387641800000281, 1469.171074702029955, 206.7381186227779892 ) ) ;
#104527=CARTESIAN_POINT ( 'NONE',  ( -11.90126295645609922, 1433.308378356310186, 149.9471753442728641 ) ) ;
#104531=B_SPLINE_SURFACE_WITH_KNOTS ( 'NONE', 5, 5, ( 
 ( #22675, #30557, #57982, #32214, #5356, #64745 ),
 ( #23246, #23792, #99951, #32757, #66394, #90452 ),
 ( #47367, #57444, #109480, #38940, #107816, #58532 ),
 ( #74782, #99396, #4795, #49582, #39515, #92117 ),
 ( #48484, #83712, #107261, #6462, #66940, #73690 ),
 ( #100514, #5915, #7007, #41165, #31105, #101048 ),
 ( #75339, #24348, #81493, #91570, #73120, #49036 ),
 ( #98858, #83171, #56875, #56321, #40061, #13730 ),
 ( #47915, #65284, #91005, #14295, #82623, #74241 ),
 ( #1378, #84802, #17586, #94307, #60188, #102157 ),
 ( #26561, #50669, #25439, #51220, #69146, #93744 ),
 ( #68591, #42268, #51785, #292, #76985, #92658 ) ),
 .UNSPECIFIED., .F., .F., .F.,
 ( 6, 3, 3, 6 ),
 ( 6, 6 ),
 ( 75.80574312749999422, 89.42327280100001019, 103.1886234069999944, 121.4516539489999900 ),
 ( 0.000000000000000000, 2.000000000000000000 ),
 .UNSPECIFIED. ) ;
#104533=CARTESIAN_POINT ( 'NONE',  ( -18.77070031028269881, 1509.608129496780066, 185.4799149847799811 ) ) ;
#104539=CARTESIAN_POINT ( 'NONE',  ( 15.94345596297699963, 1409.469818137940138, 225.2684692625209948 ) ) ;
#104541=CARTESIAN_POINT ( 'NONE',  ( 24.87051451770000199, 1509.771876611130210, 194.6077560229979895 ) ) ;
#104543=CARTESIAN_POINT ( 'NONE',  ( -17.63310548600473027, 1460.277549070645819, 228.1886722138392543 ) ) ;
#104545=CARTESIAN_POINT ( 'NONE',  ( 20.47964310962990098, 1509.616076180499931, 230.4126872671060084 ) ) ;
#104546=VERTEX_POINT ( 'NONE', #37993 ) ;
#104548=CARTESIAN_POINT ( 'NONE',  ( 18.29057181139999955, 1416.237488680629895, 209.4384559441829765 ) ) ;
#104550=CARTESIAN_POINT ( 'NONE',  ( 13.51726861618126385, 1443.820864582427475, 169.3508485337632976 ) ) ;
#104551=CARTESIAN_POINT ( 'NONE',  ( 20.52471789389999657, 1470.812340170629795, 209.1688890340030014 ) ) ;
#104552=CARTESIAN_POINT ( 'NONE',  ( -32.18001708380000281, 1459.550822088330051, 259.4130758622980011 ) ) ;
#104556=CARTESIAN_POINT ( 'NONE',  ( 26.91030929520000115, 1509.852789098830044, 199.4984680808380233 ) ) ;
#104558=CARTESIAN_POINT ( 'NONE',  ( 13.75903288890000198, 1409.893112510430001, 191.3057356182980016 ) ) ;
#104559=CARTESIAN_POINT ( 'NONE',  ( 4.209031965520000362, 1421.916286089330242, 184.3722572684980037 ) ) ;
#104561=CARTESIAN_POINT ( 'NONE',  ( -7.259422120870000050, 1440.164841281420195, 154.1325279538980055 ) ) ;
#104562=CARTESIAN_POINT ( 'NONE',  ( 10.72974958539999868, 1437.118219821549928, 152.1700466173979862 ) ) ;
#104564=CARTESIAN_POINT ( 'NONE',  ( -3.017631988560000256, 1452.807682356229861, 152.5478258260980340 ) ) ;
#104565=CARTESIAN_POINT ( 'NONE',  ( -4.363122647530000009, 1418.913060387330006, 172.2701767054979882 ) ) ;
#104566=VERTEX_POINT ( 'NONE', #20607 ) ;
#104569=CARTESIAN_POINT ( 'NONE',  ( -42.71995277159999915, 1443.972229192440182, 270.1998966713979939 ) ) ;
#104571=CARTESIAN_POINT ( 'NONE',  ( 11.97827956719999776, 1441.604408666619975, 150.7817505876979851 ) ) ;
#104573=B_SPLINE_CURVE_WITH_KNOTS ( 'NONE', 3,
 ( #77132, #110164, #17165, #42973, #42406, #25034, #101746, #59236, #73405, #30830, #93354, #34005, #34557, #98586, #21852, #56049, #79888, #94445, #103968, #9908, #54153, #95023, #70965, #61448, #26138, #95572, #69290, #68740, #19959, #27265, #78215, #62002, #60898, #18842, #9364, #36773, #36221, #45193, #87174, #87744, #11022, #1527, #35660 ),
 .UNSPECIFIED., .F., .F.,
 ( 4, 3, 3, 3, 3, 3, 3, 3, 3, 3, 3, 3, 3, 3, 4 ),
 ( 0.7655572723410000169, 0.9910019270782730594, 1.224379706194399953, 1.462078625956309885, 1.704827365190310084, 1.793853281190000093, 2.038466590501220033, 2.281256473202240009, 2.316155491850000026, 2.583989317130000352, 2.855920918771889916, 3.139267317773660082, 3.387490792969999553, 3.680707211540199530, 3.835724788479999425 ),
 .UNSPECIFIED. ) ;
#104574=CARTESIAN_POINT ( 'NONE',  ( 13.91344329490000042, 1453.313060387329870, 195.2084026661979976 ) ) ;
#104575=CARTESIAN_POINT ( 'NONE',  ( 2.926631436004109688, 1410.008353746950206, 231.5604053785249903 ) ) ;
#104576=CARTESIAN_POINT ( 'NONE',  ( 1.717348298979999965, 1508.746280155129853, 237.8324610923980060 ) ) ;
#104577=CARTESIAN_POINT ( 'NONE',  ( -4.849515614649999584, 1416.821738697630053, 232.3035063180979876 ) ) ;
#104580=CARTESIAN_POINT ( 'NONE',  ( -44.17901015457650260, 1430.646547340430061, 267.0395108202489496 ) ) ;
#104581=CARTESIAN_POINT ( 'NONE',  ( -4.153907728910000152, 1436.967118409070054, 185.6199311185980036 ) ) ;
#104583=CARTESIAN_POINT ( 'NONE',  ( 25.19713807460000154, 1435.377389496489741, 135.6160520644979783 ) ) ;
#104588=CARTESIAN_POINT ( 'NONE',  ( -16.18847876140000253, 1410.409213345830040, 191.4685065236979824 ) ) ;
#104590=ORIENTED_EDGE ( 'NONE', *, *, #41892, .F. ) ;
#104591=CARTESIAN_POINT ( 'NONE',  ( -15.82374664200000147, 1506.811133727029983, 193.8386827112979631 ) ) ;
#104594=AXIS2_PLACEMENT_3D ( 'NONE', #74316, #31176, #22751 ) ;
#104597=CARTESIAN_POINT ( 'NONE',  ( 18.51267884070961145, 1508.236097879769432, 188.5103842653526272 ) ) ;
#104600=ORIENTED_EDGE ( 'NONE', *, *, #9035, .F. ) ;
#104601=CARTESIAN_POINT ( 'NONE',  ( -18.62763287599860007, 1413.086711950159952, 269.8943054501950201 ) ) ;
#104608=CARTESIAN_POINT ( 'NONE',  ( 45.62788796885585185, 1441.601644691920001, 268.9750038475548877 ) ) ;
#104611=CARTESIAN_POINT ( 'NONE',  ( -0.01421524400490130000, 1408.952300071870013, 186.1308435959000178 ) ) ;
#104612=CARTESIAN_POINT ( 'NONE',  ( -18.64275274472940325, 1415.948038441080143, 207.5714938949250268 ) ) ;
#104613=CARTESIAN_POINT ( 'NONE',  ( -23.20509094550000029, 1425.806681453030023, 211.9918775447279984 ) ) ;
#104614=CARTESIAN_POINT ( 'NONE',  ( 22.44355668859300224, 1471.536005699779935, 269.1117652856750055 ) ) ;
#104615=CARTESIAN_POINT ( 'NONE',  ( -9.019884638846754399, 1465.064825884716129, 232.8089404004333574 ) ) ;
#104616=CARTESIAN_POINT ( 'NONE',  ( 12.53380176329999784, 1445.052233945699982, 186.0874982363980052 ) ) ;
#104619=CARTESIAN_POINT ( 'NONE',  ( -13.81919561380460060, 1452.718877875840008, 223.1176038296620163 ) ) ;
#104620=CARTESIAN_POINT ( 'NONE',  ( 1.474324447131689864, 1482.591219605810011, 182.1827347203019940 ) ) ;
#104623=CARTESIAN_POINT ( 'NONE',  ( 26.04939065782729912, 1450.947403696690117, 136.6506608130579821 ) ) ;
#104624=CARTESIAN_POINT ( 'NONE',  ( 11.27215015582655688, 1425.068134849736907, 138.0224606737560578 ) ) ;
#104627=CARTESIAN_POINT ( 'NONE',  ( 16.71902292089999875, 1409.496901533429991, 193.2501433177980346 ) ) ;
#104628=CARTESIAN_POINT ( 'NONE',  ( 27.73716673060003757, 1443.913060387329097, 175.8274728504979976 ) ) ;
#104629=CARTESIAN_POINT ( 'NONE',  ( 2.579410839141357936, 1439.640988620472626, 183.3331822185549811 ) ) ;
#104630=CARTESIAN_POINT ( 'NONE',  ( 0.2990840903870000123, 1416.120339285229875, 233.5289124774980110 ) ) ;
#104631=CARTESIAN_POINT ( 'NONE',  ( -18.88027416897331179, 1424.772622057686704, 224.4247119630791758 ) ) ;
#104635=CARTESIAN_POINT ( 'NONE',  ( 26.88225067539190150, 1446.276343828759991, 137.3355637594920040 ) ) ;
#104636=VERTEX_POINT ( 'NONE', #65415 ) ;
#104639=CARTESIAN_POINT ( 'NONE',  ( -0.4291274509555380035, 1409.251717294920127, 232.6516010116560267 ) ) ;
#104640=EDGE_CURVE ( 'NONE', #99633, #30773, #106606, .T. ) ;
#104645=CARTESIAN_POINT ( 'NONE',  ( 7.993605777300000598E-15, 1455.844446582929777, 219.6133832206979832 ) ) ;
#104647=CARTESIAN_POINT ( 'NONE',  ( 11.68271886119999969, 1433.062043557109973, 150.9218026163979687 ) ) ;
#104648=CARTESIAN_POINT ( 'NONE',  ( -15.40709604279999922, 1473.361390454229877, 269.5773951781980031 ) ) ;
#104649=B_SPLINE_SURFACE_WITH_KNOTS ( 'NONE', 5, 5, ( 
 ( #97940, #44824, #96307, #104152, #95753, #89551 ),
 ( #45916, #106355, #97402, #2821, #88461, #63288 ),
 ( #105824, #21208, #87927, #36940, #105257, #55417 ),
 ( #70040, #19586, #104701, #11747, #80609, #62750 ),
 ( #45378, #79517, #4460, #96868, #80052, #12840 ),
 ( #27438, #37500, #71706, #19017, #29102, #11214 ),
 ( #20672, #87359, #54872, #78977, #36395, #70584 ),
 ( #12283, #27996, #62181, #40250, #91204, #49225 ),
 ( #100695, #14486, #15571, #49773, #23978, #30182 ),
 ( #5555, #65479, #47561, #15026, #39704, #4989 ),
 ( #91751, #74981, #74432, #108558, #38588, #82801 ),
 ( #90089, #58173, #66591, #64374, #98497, #48115 ) ),
 .UNSPECIFIED., .F., .F., .F.,
 ( 6, 3, 3, 6 ),
 ( 6, 6 ),
 ( 22.90453168350000013, 35.06371889219999360, 67.00219837880000284, 82.96876465699999414 ),
 ( 0.000000000000000000, 2.000000000000000000 ),
 .UNSPECIFIED. ) ;
#104650=CARTESIAN_POINT ( 'NONE',  ( 26.44889291085189953, 1440.913060394389959, 224.1891630988550048 ) ) ;
#104654=CARTESIAN_POINT ( 'NONE',  ( 23.85742997590000414, 1435.349283830410059, 137.3962418501980380 ) ) ;
#104655=CARTESIAN_POINT ( 'NONE',  ( -7.000066174799999708, 1486.134313416229816, 182.6266077387979863 ) ) ;
#104657=LINE ( 'NONE', #71661, #100860 ) ;
#104658=CARTESIAN_POINT ( 'NONE',  ( 25.92853884430000377, 1469.242862523229860, 212.4557546463379936 ) ) ;
#104660=CARTESIAN_POINT ( 'NONE',  ( -8.309064975820000143, 1507.619008861029897, 235.1729359256979990 ) ) ;
#104664=CARTESIAN_POINT ( 'NONE',  ( 5.516975442445060551, 1422.876349978269900, 115.6516328984649959 ) ) ;
#104665=CARTESIAN_POINT ( 'NONE',  ( -22.52564151159999639, 1509.699673122230024, 190.3321270482979912 ) ) ;
#104666=( BOUNDED_CURVE ( )  B_SPLINE_CURVE ( 3, ( #13195, #97220, #46850, #89920 ),
 .UNSPECIFIED., .F., .T. ) 
 B_SPLINE_CURVE_WITH_KNOTS ( ( 4, 4 ),
 ( 0.02238567329313790114, 0.6605756095507959724 ),
 .UNSPECIFIED. ) 
 CURVE ( )  GEOMETRIC_REPRESENTATION_ITEM ( )  RATIONAL_B_SPLINE_CURVE ( ( 1.000000000000000000, 0.9663464813702775658, 0.9663464813702775658, 1.000000000000000000 ) ) 
 REPRESENTATION_ITEM ( '' )  );
#104667=CARTESIAN_POINT ( 'NONE',  ( 0.1661509758321400021, 1482.596978913680005, 181.9828288344639873 ) ) ;
#104668=CARTESIAN_POINT ( 'NONE',  ( 16.68463225830000241, 1445.052233488290085, 162.0935120917980043 ) ) ;
#104669=ORIENTED_EDGE ( 'NONE', *, *, #8545, .F. ) ;
#104670=CARTESIAN_POINT ( 'NONE',  ( -0.3594932245259999659, 1451.468209969430063, 182.7573421931980135 ) ) ;
#104678=CARTESIAN_POINT ( 'NONE',  ( 12.26996133436636249, 1416.831922870707331, 223.5794496286292485 ) ) ;
#104683=CARTESIAN_POINT ( 'NONE',  ( 13.59476445004379919, 1409.387800022989950, 202.9347135095200088 ) ) ;
#104684=CARTESIAN_POINT ( 'NONE',  ( 7.789933822538570141, 1421.055612659608187, 137.0999999980982409 ) ) ;
#104689=CARTESIAN_POINT ( 'NONE',  ( 13.51702042466233600, 1443.913060387330006, 169.3754641244197217 ) ) ;
#104690=CARTESIAN_POINT ( 'NONE',  ( -1.552364036650669687, 1414.913060595378738, 226.1349304001991527 ) ) ;
#104691=VERTEX_POINT ( 'NONE', #98978 ) ;
#104693=CARTESIAN_POINT ( 'NONE',  ( 20.59684415639999955, 1507.762623716630060, 227.3081670307980175 ) ) ;
#104696=CARTESIAN_POINT ( 'NONE',  ( 29.92046006148340709, 1462.307239681074179, 269.4699585593555753 ) ) ;
#104697=CARTESIAN_POINT ( 'NONE',  ( 15.20184466319999927, 1507.442701412029919, 225.8641442827980086 ) ) ;
#104698=CARTESIAN_POINT ( 'NONE',  ( 3.817422068910000021, 1397.107870743330068, 221.4612898547980251 ) ) ;
#104700=CARTESIAN_POINT ( 'NONE',  ( 18.93704081231690139, 1430.332813895809977, 209.3856457964110120 ) ) ;
#104701=CARTESIAN_POINT ( 'NONE',  ( -0.8731571743890000903, 1457.276952884830052, 183.1868505578979978 ) ) ;
#104703=CARTESIAN_POINT ( 'NONE',  ( -26.36655729521032754, 1436.714562387939850, 136.8351542746285645 ) ) ;
#104706=CARTESIAN_POINT ( 'NONE',  ( 16.85557976710000005, 1409.501670203030017, 194.3276026113979924 ) ) ;
#104709=CARTESIAN_POINT ( 'NONE',  ( 41.56283943469610165, 1444.074288271499881, 136.1757548026400002 ) ) ;
#104710=EDGE_LOOP ( 'NONE', ( #105567, #85382, #107954, #55289 ) ) ;
#104711=CARTESIAN_POINT ( 'NONE',  ( 33.67852062189999884, 1421.560015059330226, 261.9077681813980121 ) ) ;
#104712=ADVANCED_FACE ( 'NONE', ( #88936 ), #48972, .T. ) ;
#104713=CARTESIAN_POINT ( 'NONE',  ( -22.56155901339999659, 1488.679832658830264, 195.6780914239980120 ) ) ;
#104714=CARTESIAN_POINT ( 'NONE',  ( 0.4607471438239999495, 1507.266167991529983, 180.9276013137979930 ) ) ;
#104720=CARTESIAN_POINT ( 'NONE',  ( -22.89347097630000150, 1507.627022993330229, 208.2062336298450020 ) ) ;
#104721=CARTESIAN_POINT ( 'NONE',  ( -5.805165550179999912, 1411.425361495129891, 255.2684082155979866 ) ) ;
#104722=CARTESIAN_POINT ( 'NONE',  ( 19.47564118608110206, 1509.620631326759849, 231.4858733237100239 ) ) ;
#104724=CARTESIAN_POINT ( 'NONE',  ( 28.57599588785479838, 1509.162863316300218, 209.4718383517779898 ) ) ;
#104727=CARTESIAN_POINT ( 'NONE',  ( 33.93392607710000419, 1451.271780568129998, 135.9464999937979997 ) ) ;
#104729=CARTESIAN_POINT ( 'NONE',  ( 3.767303529005479934, 1397.401587145810026, 196.1650422737100143 ) ) ;
#104731=CARTESIAN_POINT ( 'NONE',  ( -16.61244639070000062, 1459.967033444430172, 228.4924314892979851 ) ) ;
#104732=B_SPLINE_CURVE_WITH_KNOTS ( 'NONE', 3,
 ( #20499, #74259, #84285, #47937 ),
 .UNSPECIFIED., .F., .F.,
 ( 4, 4 ),
 ( 0.000000000000000000, 1.000000000000000000 ),
 .UNSPECIFIED. ) ;
#104738=FACE_OUTER_BOUND ( 'NONE', #14681, .T. ) ;
#104741=CARTESIAN_POINT ( 'NONE',  ( -3.378818643640000285, 1461.193638821730019, 234.6789676215979910 ) ) ;
#104743=VECTOR ( 'NONE', #91034, 1000.000000000000114 ) ;
#104746=ADVANCED_FACE ( 'NONE', ( #75471 ), #31951, .T. ) ;
#104747=CARTESIAN_POINT ( 'NONE',  ( 0.1437158803840000165, 1420.464389115830045, 182.7235331698980190 ) ) ;
#104753=CARTESIAN_POINT ( 'NONE',  ( 1.582067810090000045E-15, 1406.443991414029824, 121.6099336315979969 ) ) ;
#104759=CIRCLE ( 'NONE', #97395, 8.500000000000000000 ) ;
#104761=CARTESIAN_POINT ( 'NONE',  ( 16.66808812225220038, 1452.330997924170106, 146.5817830544619937 ) ) ;
#104762=CARTESIAN_POINT ( 'NONE',  ( 1.412130994944630125, 1410.254392240469997, 269.6150871368109847 ) ) ;
#104768=CARTESIAN_POINT ( 'NONE',  ( 0.03226293719758020068, 1410.297897419189894, 233.2219341505459909 ) ) ;
#104775=CARTESIAN_POINT ( 'NONE',  ( 8.215650382230000152E-15, 1424.916853932230197, 224.8635561844979804 ) ) ;
#104782=VERTEX_POINT ( 'NONE', #69835 ) ;
#104784=B_SPLINE_CURVE_WITH_KNOTS ( 'NONE', 5,
 ( #71340, #54529, #61282, #46671, #74061, #73516 ),
 .UNSPECIFIED., .F., .F.,
 ( 6, 6 ),
 ( 0.000000000000000000, 1.000000000000000000 ),
 .UNSPECIFIED. ) ;
#104789=CARTESIAN_POINT ( 'NONE',  ( -12.53380394689999910, 1442.773887138329883, 185.9733701915980078 ) ) ;
#104790=CARTESIAN_POINT ( 'NONE',  ( 21.40227409560650074, 1509.660444267860157, 229.5162084721659994 ) ) ;
#104792=CARTESIAN_POINT ( 'NONE',  ( -0.9766393796380001824, 1453.313060387329870, 229.7750655478980093 ) ) ;
#104793=CARTESIAN_POINT ( 'NONE',  ( 16.64350137070000102, 1410.411353414630184, 226.4950628044979908 ) ) ;
#104795=CARTESIAN_POINT ( 'NONE',  ( -16.01735770899999878, 1459.144465034730047, 229.9898643770979731 ) ) ;
#104797=CARTESIAN_POINT ( 'NONE',  ( 39.55285272340000091, 1422.351058411129998, 267.1954752406980447 ) ) ;
#104799=CARTESIAN_POINT ( 'NONE',  ( 19.23474158209999985, 1436.402232428999923, 146.2239547538979991 ) ) ;
#104800=CARTESIAN_POINT ( 'NONE',  ( 21.81674547060000080, 1488.582783796430022, 193.4203703249980038 ) ) ;
#104801=CARTESIAN_POINT ( 'NONE',  ( 29.60476317767313148, 1509.968981583988352, 207.5719681184634169 ) ) ;
#104803=CARTESIAN_POINT ( 'NONE',  ( 12.78752278269999998, 1416.843576368729828, 222.7044122178979819 ) ) ;
#104805=CARTESIAN_POINT ( 'NONE',  ( 25.00977876991279913, 1436.598012848749931, 137.9330263815630246 ) ) ;
#104807=CARTESIAN_POINT ( 'NONE',  ( -16.97980319039999841, 1414.913060387329779, 208.1309929760350315 ) ) ;
#104808=CARTESIAN_POINT ( 'NONE',  ( -12.77622632179999940, 1442.825377011449973, 186.2636718277979924 ) ) ;
#104810=CARTESIAN_POINT ( 'NONE',  ( -33.14720771140000011, 1435.654777855230122, 135.5270110727979898 ) ) ;
#104812=ORIENTED_EDGE ( 'NONE', *, *, #24961, .T. ) ;
#104813=CARTESIAN_POINT ( 'NONE',  ( -4.026786250540000722, 1422.913060387330006, 179.5815723472979926 ) ) ;
#104814=CARTESIAN_POINT ( 'NONE',  ( -2.224601527347340291, 1408.990745184500156, 223.9491347404019734 ) ) ;
#104817=B_SPLINE_CURVE_WITH_KNOTS ( 'NONE', 3,
 ( #62260, #54412, #37579, #12365, #38123, #29179, #104234, #88009, #61707, #27522, #19665, #87441, #63370, #28629, #97485, #86876, #96389, #2904, #2360, #103681, #88544, #28072, #19097 ),
 .UNSPECIFIED., .F., .F.,
 ( 4, 2, 2, 2, 2, 2, 2, 2, 1, 2, 2, 4 ),
 ( 0.000000000000000000, 0.1250000000000727474, 0.1875000000000847378, 0.2500000000000967559, 0.3750000000001207368, 0.5000000000001447731, 0.6250000000001687539, 0.6875000000001788569, 0.7187500000000898170, 0.7343750000001433298, 0.7500000000001967315, 1.000000000000000000 ),
 .UNSPECIFIED. ) ;
#104819=CARTESIAN_POINT ( 'NONE',  ( -37.49400285100000474, 1461.515165505230016, 269.0078955473979931 ) ) ;
#104821=CARTESIAN_POINT ( 'NONE',  ( 0.2406210619857520050, 1420.498996480750066, 182.8345142462969761 ) ) ;
#104822=EDGE_CURVE ( 'NONE', #38088, #22249, #57987, .T. ) ;
#104823=CARTESIAN_POINT ( 'NONE',  ( -26.23322848259999773, 1508.580494355830069, 216.2666545556479889 ) ) ;
#104826=CARTESIAN_POINT ( 'NONE',  ( 17.24529142091330058, 1423.692487554319996, 227.0492506374200161 ) ) ;
#104827=CARTESIAN_POINT ( 'NONE',  ( 21.91792426430000162, 1509.678451168530273, 227.8819284608979956 ) ) ;
#104828=CARTESIAN_POINT ( 'NONE',  ( -3.255911231930000316, 1435.946191916090129, 155.5160642224979881 ) ) ;
#104830=CARTESIAN_POINT ( 'NONE',  ( -26.89242289587770074, 1508.005886644420116, 211.7458576771490186 ) ) ;
#104832=CARTESIAN_POINT ( 'NONE',  ( -3.666700706489999906, 1509.114858798330033, 179.5219359138980053 ) ) ;
#104833=DIRECTION ( 'NONE',  ( 0.7636119845598413614, -0.004098122786949555049, 0.6456624059260408499 ) ) ;
#104834=CARTESIAN_POINT ( 'NONE',  ( 13.24264731299999909, 1414.971439108430104, 197.5210417955980233 ) ) ;
#104835=CARTESIAN_POINT ( 'NONE',  ( -12.71459596929999947, 1416.274718422629803, 195.3550244208979905 ) ) ;
#104838=CARTESIAN_POINT ( 'NONE',  ( 22.70506338740000274, 1409.705938672130060, 209.2982490380130116 ) ) ;
#104841=CARTESIAN_POINT ( 'NONE',  ( -16.28172202780000077, 1421.049848839029892, 227.0416102452980169 ) ) ;
#104842=B_SPLINE_CURVE_WITH_KNOTS ( 'NONE', 5,
 ( #79652, #97535, #71833, #56088, #46605, #107581 ),
 .UNSPECIFIED., .F., .F.,
 ( 6, 6 ),
 ( -168.1723206030000028, -30.75981893479999485 ),
 .UNSPECIFIED. ) ;
#104843=CARTESIAN_POINT ( 'NONE',  ( 11.90003109757362409, 1434.915657497907659, 147.6452320157113149 ) ) ;
#104846=DIRECTION ( 'NONE',  ( 9.624611914481800761E-06, -0.9328681587603299130, 0.3602179871667691713 ) ) ;
#104848=CARTESIAN_POINT ( 'NONE',  ( -23.36374832350000119, 1420.923074028029987, 211.0949373619980065 ) ) ;
#104852=FACE_OUTER_BOUND ( 'NONE', #106777, .T. ) ;
#104856=ORIENTED_EDGE ( 'NONE', *, *, #109314, .F. ) ;
#104857=ORIENTED_EDGE ( 'NONE', *, *, #103727, .T. ) ;
#104858=CARTESIAN_POINT ( 'NONE',  ( 26.37675685490000177, 1508.582722881630161, 216.7139244022480113 ) ) ;
#104859=ORIENTED_EDGE ( 'NONE', *, *, #61432, .F. ) ;
#104862=CARTESIAN_POINT ( 'NONE',  ( 3.156166260290000025, 1466.544008048530031, 236.1241471695980181 ) ) ;
#104863=CARTESIAN_POINT ( 'NONE',  ( -15.71589887163418098, 1409.995731639605310, 226.4233246076490786 ) ) ;
#104864=CARTESIAN_POINT ( 'NONE',  ( 0.2427466632179999806, 1508.856333042329879, 179.8940944152980137 ) ) ;
#104865=DIRECTION ( 'NONE',  ( 1.593356620438984032E-14, -0.7071067811865475727, -0.7071067811865475727 ) ) ;
#104866=EDGE_CURVE ( 'NONE', #107054, #83948, #99402, .T. ) ;
#104867=CARTESIAN_POINT ( 'NONE',  ( 4.651532691979999967, 1488.169727963030255, 182.7049705295980004 ) ) ;
#104869=CARTESIAN_POINT ( 'NONE',  ( 6.936014448009999889, 1409.155271349029817, 229.3511990319979930 ) ) ;
#104872=CARTESIAN_POINT ( 'NONE',  ( 39.90438676500410509, 1438.693166630719816, 134.0999999980629980 ) ) ;
#104874=CARTESIAN_POINT ( 'NONE',  ( 10613.67162216127690, 54.28084071072816386, 5061.882847296718865 ) ) ;
#104876=CARTESIAN_POINT ( 'NONE',  ( 14.24929417786319874, 1435.536138497730008, 149.6993440739240100 ) ) ;
#104879=EDGE_LOOP ( 'NONE', ( #81752, #12782, #40276, #61277, #40509 ) ) ;
#104880=VERTEX_POINT ( 'NONE', #107260 ) ;
#104884=CARTESIAN_POINT ( 'NONE',  ( 24.73993050763418822, 1450.821579931246333, 138.7998613157621719 ) ) ;
#104888=CARTESIAN_POINT ( 'NONE',  ( -18.53161554139801126, 1445.630398175708706, 214.4691203362832539 ) ) ;
#104891=B_SPLINE_CURVE_WITH_KNOTS ( 'NONE', 3,
 ( #73220, #64844, #56426, #90556, #88912, #5457, #62655, #97311, #88368, #11658 ),
 .UNSPECIFIED., .F., .F.,
 ( 4, 2, 2, 2, 4 ),
 ( -0.1573215296859830081, -0.1159487415761059903, -0.07685134973319139584, -0.03820936005390598855, -7.424679884793228268E-08 ),
 .UNSPECIFIED. ) ;
#104895=ORIENTED_EDGE ( 'NONE', *, *, #87025, .T. ) ;
#104896=CARTESIAN_POINT ( 'NONE',  ( 29.16429843505859765, 1440.913060387330006, 250.3001267888409984 ) ) ;
#104897=CARTESIAN_POINT ( 'NONE',  ( -0.0001095867327352822572, 1452.800716251688982, 153.1161686451791013 ) ) ;
#104899=CARTESIAN_POINT ( 'NONE',  ( 26.25908477761629811, 1449.904608170299980, 136.7328078875380015 ) ) ;
#104900=CARTESIAN_POINT ( 'NONE',  ( -13.92984420660000033, 1410.332022920429836, 190.1904693403979820 ) ) ;
#104902=EDGE_CURVE ( 'NONE', #90951, #41783, #49967, .T. ) ;
#104903=CARTESIAN_POINT ( 'NONE',  ( -24.90171366719999924, 1441.078953671579939, 210.4323502101080123 ) ) ;
#104905=CARTESIAN_POINT ( 'NONE',  ( -11.60004869885203682, 1428.983126981193436, 134.0999999980979851 ) ) ;
#104906=CARTESIAN_POINT ( 'NONE',  ( 0.0002411117317979708972, 1396.089785486056144, 197.2899115322371131 ) ) ;
#104908=CARTESIAN_POINT ( 'NONE',  ( -11.87520966259999966, 1433.007090144579934, 149.2720797894980080 ) ) ;
#104910=CARTESIAN_POINT ( 'NONE',  ( 7.657194240169999944, 1464.005168892129859, 233.8507629060979980 ) ) ;
#104913=EDGE_CURVE ( 'NONE', #7633, #56404, #52353, .T. ) ;
#104914=B_SPLINE_CURVE_WITH_KNOTS ( 'NONE', 3,
 ( #9492, #86757, #1120, #61040, #25724, #77269, #11, #18420, #103550, #69435, #26284, #25170, #61579, #35250, #51503, #26852, #567, #34146, #86201, #34693, #1670, #95711, #76150, #95163, #52068, #94043, #52620, #68884, #67766 ),
 .UNSPECIFIED., .F., .F.,
 ( 4, 2, 2, 1, 1, 2, 2, 2, 2, 2, 2, 2, 1, 2, 2, 4 ),
 ( 0.000000000000000000, 0.2500000000000895950, 0.3750000000001428302, 0.4375000000001597056, 0.4687500000001595946, 0.4843750000001595946, 0.5000000000001595390, 0.6250000000001475486, 0.6875000000001415534, 0.7187500000001406653, 0.7500000000001397771, 0.8125000000001320055, 0.8437500000001281197, 0.8593750000001226796, 0.8750000000001172396, 1.000000000000000000 ),
 .UNSPECIFIED. ) ;
#104917=B_SPLINE_CURVE_WITH_KNOTS ( 'NONE', 3,
 ( #40706, #31197, #30653, #91658, #14933, #74336, #7107, #101141, #56419, #48577, #23882, #65384, #99487 ),
 .UNSPECIFIED., .F., .F.,
 ( 4, 2, 2, 2, 1, 2, 4 ),
 ( 0.000000000000000000, 0.09521579484686493178, 0.1428236922702973977, 0.1666276409821136339, 0.1785296153381099038, 0.1844806025161973007, 0.1904315896942847253 ),
 .UNSPECIFIED. ) ;
#104919=CARTESIAN_POINT ( 'NONE',  ( -16.68463225901000158, 1442.773887286389936, 162.0935120915889911 ) ) ;
#104921=CARTESIAN_POINT ( 'NONE',  ( -20.42020019299999944, 1470.816980701829834, 209.4971671475969970 ) ) ;
#104924=ORIENTED_EDGE ( 'NONE', *, *, #42327, .F. ) ;
#104926=CARTESIAN_POINT ( 'NONE',  ( 3.897123952299999576E-10, 1465.695272585530120, 240.4142140030979817 ) ) ;
#104930=CARTESIAN_POINT ( 'NONE',  ( -19.17279900190000319, 1457.063330234229852, 226.5609651273980205 ) ) ;
#104931=CARTESIAN_POINT ( 'NONE',  ( -21.74576665880016080, 1411.032818084173414, 201.6082284287891468 ) ) ;
#104932=CARTESIAN_POINT ( 'NONE',  ( 2.500000000000000000, 1419.623475504530006, 147.1347451145979903 ) ) ;
#104933=CARTESIAN_POINT ( 'NONE',  ( -0.2254851406240000189, 1434.822352678220113, 190.2673095969979897 ) ) ;
#104935=ORIENTED_EDGE ( 'NONE', *, *, #29505, .T. ) ;
#104937=CARTESIAN_POINT ( 'NONE',  ( 2.771812352850000494, 1405.904361742329911, 267.2318186464980272 ) ) ;
#104939=CARTESIAN_POINT ( 'NONE',  ( 13.37887548737149856, 1473.256433280859937, 270.1124100584160033 ) ) ;
#104940=CARTESIAN_POINT ( 'NONE',  ( 5.465008655120000114, 1438.535486872679940, 154.7353332079979964 ) ) ;
#104942=CARTESIAN_POINT ( 'NONE',  ( -37.81805297112759945, 1440.913060389500060, 255.9894328691030410 ) ) ;
#104943=CARTESIAN_POINT ( 'NONE',  ( -26.50175984629999704, 1446.255663087950097, 137.5973547775980137 ) ) ;
#104950=CARTESIAN_POINT ( 'NONE',  ( -43.50000000000000000, 1435.965051957929973, 271.1218459616979999 ) ) ;
#104953=CARTESIAN_POINT ( 'NONE',  ( -14.38276615812611681, 1514.413060387330006, 182.7943691049868278 ) ) ;
#104954=CARTESIAN_POINT ( 'NONE',  ( -0.2151320649219999881, 1475.759570378829949, 269.0456880799980013 ) ) ;
#104955=CARTESIAN_POINT ( 'NONE',  ( -13.53916864874639892, 1429.119333790580185, 222.2883575635510169 ) ) ;
#104956=CARTESIAN_POINT ( 'NONE',  ( -27.96976557860000057, 1509.201555289429962, 210.6640596492780162 ) ) ;
#104957=CARTESIAN_POINT ( 'NONE',  ( -3.579852315081284431, 1448.290319961710338, 184.9158413581277500 ) ) ;
#104960=CARTESIAN_POINT ( 'NONE',  ( -17.77615777719999812, 1415.140114695929924, 207.9728109415779898 ) ) ;
#104962=CARTESIAN_POINT ( 'NONE',  ( 26.42721169618110011, 1435.958680060049801, 136.4983543512450126 ) ) ;
#104963=CARTESIAN_POINT ( 'NONE',  ( -9.715427105718768885, 1396.252330577819976, 214.4129421473980130 ) ) ;
#104964=CARTESIAN_POINT ( 'NONE',  ( -15.80894304229999925, 1421.035217125530153, 227.0411593344980190 ) ) ;
#104965=ADVANCED_FACE ( 'NONE', ( #21582 ), #32860, .F. ) ;
#104966=CARTESIAN_POINT ( 'NONE',  ( -17.33018476747690073, 1410.462527268070062, 225.7401589819789933 ) ) ;
#104967=CARTESIAN_POINT ( 'NONE',  ( 11.88140585900000090, 1433.447543843229823, 147.6490162021979984 ) ) ;
#104971=CARTESIAN_POINT ( 'NONE',  ( -8.348318400919996662, 1484.298477954530199, 184.3911661821975372 ) ) ;
#104972=CARTESIAN_POINT ( 'NONE',  ( 10.81150411640000009, 1425.669232956329779, 101.9066733906980033 ) ) ;
#104974=CARTESIAN_POINT ( 'NONE',  ( -0.3155435254770000419, 1483.118057600029942, 236.2956536266979981 ) ) ;
#104976=CARTESIAN_POINT ( 'NONE',  ( -13.51610093808350577, 1445.063428794548372, 205.0760988357350527 ) ) ;
#104981=CARTESIAN_POINT ( 'NONE',  ( 2.360320924850000335, 1507.942448366130066, 181.1000475259980078 ) ) ;
#104986=ORIENTED_EDGE ( 'NONE', *, *, #41792, .F. ) ;
#104987=VERTEX_POINT ( 'NONE', #14294 ) ;
#104988=CARTESIAN_POINT ( 'NONE',  ( 0.07608147880745361191, 1490.951086335209993, 236.6948437218040056 ) ) ;
#104989=CARTESIAN_POINT ( 'NONE',  ( 3.679272716979999913, 1453.313060387329870, 228.5941172881979924 ) ) ;
#104991=( BOUNDED_CURVE ( )  B_SPLINE_CURVE ( 3, ( #15189, #109285, #84062, #32570 ),
 .UNSPECIFIED., .F., .F. ) 
 B_SPLINE_CURVE_WITH_KNOTS ( ( 4, 4 ),
 ( 4.177675961634177426, 5.247004545667287800 ),
 .UNSPECIFIED. ) 
 CURVE ( )  GEOMETRIC_REPRESENTATION_ITEM ( )  RATIONAL_B_SPLINE_CURVE ( ( 1.000000000000000000, 0.9069598256684616722, 0.9069598256684616722, 1.000000000000000000 ) ) 
 REPRESENTATION_ITEM ( '' )  );
#104993=CARTESIAN_POINT ( 'NONE',  ( 0.1287657911039999936, 1486.015939899330078, 182.0783122775980303 ) ) ;
#104994=CARTESIAN_POINT ( 'NONE',  ( 21.40470761700000324, 1507.840874668130027, 191.1187993005979990 ) ) ;
#104999=CARTESIAN_POINT ( 'NONE',  ( 3.876049381683142059, 1447.746239516663763, 184.2268197018375133 ) ) ;
#105001=CARTESIAN_POINT ( 'NONE',  ( 12.15678282470000049, 1407.401676941830146, 215.7644370117779999 ) ) ;
#105002=CARTESIAN_POINT ( 'NONE',  ( -1.533256472543610194, 1405.729012779230061, 267.8533381434389753 ) ) ;
#105004=CARTESIAN_POINT ( 'NONE',  ( 41.66090683250000382, 1443.836063800979900, 135.6920700532980106 ) ) ;
#105008=ORIENTED_EDGE ( 'NONE', *, *, #104913, .F. ) ;
#105010=EDGE_CURVE ( 'NONE', #93315, #100437, #21839, .T. ) ;
#105013=AXIS2_PLACEMENT_3D ( 'NONE', #74358, #108486, #110134 ) ;
#105016=EDGE_CURVE ( 'NONE', #45663, #46504, #107348, .T. ) ;
#105025=CARTESIAN_POINT ( 'NONE',  ( -5.993306093509999322, 1410.496812455530062, 231.4967973790980125 ) ) ;
#105026=CARTESIAN_POINT ( 'NONE',  ( -8.927951907720000690, 1446.111221346229968, 185.7534680273980143 ) ) ;
#105027=VERTEX_POINT ( 'NONE', #66938 ) ;
#105028=ADVANCED_FACE ( 'NONE', ( #75871 ), #24818, .F. ) ;
#105030=CARTESIAN_POINT ( 'NONE',  ( -24.78096948487849716, 1440.913060472049892, 214.6184464147330004 ) ) ;
#105033=CARTESIAN_POINT ( 'NONE',  ( 15.57930626881383063, 1506.606278689549981, 224.8356771238971703 ) ) ;
#105034=CARTESIAN_POINT ( 'NONE',  ( -25.67043386000000282, 1436.190963422269988, 136.9403443359979917 ) ) ;
#105035=CARTESIAN_POINT ( 'NONE',  ( 41.09353168516779675, 1432.680545450300087, 269.6304333787269911 ) ) ;
#105036=EDGE_CURVE ( 'NONE', #69912, #53899, #35519, .T. ) ;
#105044=EDGE_LOOP ( 'NONE', ( #28428, #22119, #11778 ) ) ;
#105045=CARTESIAN_POINT ( 'NONE',  ( -1.757532416683340148, 1451.933574871519795, 184.1885909450070073 ) ) ;
#105046=CARTESIAN_POINT ( 'NONE',  ( -6.511472450310000326, 1415.369202044029862, 231.5173866912979861 ) ) ;
#105051=CARTESIAN_POINT ( 'NONE',  ( 12.57300769832470166, 1478.702740668469914, 232.0245263613259965 ) ) ;
#105053=DIRECTION ( 'NONE',  ( 0.4794255386042030054, 0.000000000000000000, 0.8775825618903727587 ) ) ;
#105054=CARTESIAN_POINT ( 'NONE',  ( -0.1940356176690000156, 1409.861619114730047, 233.2114736749980182 ) ) ;
#105055=CARTESIAN_POINT ( 'NONE',  ( -16.19492410460000187, 1409.478599598930032, 217.9908631324380224 ) ) ;
#105057=CARTESIAN_POINT ( 'NONE',  ( -0.02062249914556560024, 1508.912340185780067, 235.3515326150290150 ) ) ;
#105061=ORIENTED_EDGE ( 'NONE', *, *, #80850, .T. ) ;
#105062=CARTESIAN_POINT ( 'NONE',  ( -10.86245182433490086, 1414.913060387399810, 196.8063316368690039 ) ) ;
#105063=CARTESIAN_POINT ( 'NONE',  ( -20.20633738500000121, 1495.113783644630075, 189.9444582722979931 ) ) ;
#105066=CARTESIAN_POINT ( 'NONE',  ( 9.788842362726176916, 1435.966427250319612, 152.6339651303872245 ) ) ;
#105071=CARTESIAN_POINT ( 'NONE',  ( -2.500000000000000000, 1448.989771683439812, 154.5778230850980037 ) ) ;
#105072=CARTESIAN_POINT ( 'NONE',  ( -17.72524821669999895, 1424.247088718729856, 226.5195189683980175 ) ) ;
#105073=CARTESIAN_POINT ( 'NONE',  ( -19.66037016059999942, 1436.416578655439935, 145.8483816223979943 ) ) ;
#105074=CARTESIAN_POINT ( 'NONE',  ( -2.451271202390000070, 1433.447543843880112, 150.3250444719979839 ) ) ;
#105075=CARTESIAN_POINT ( 'NONE',  ( 17.37020517850000090, 1428.766723024330076, 191.2625755937980045 ) ) ;
#105076=CARTESIAN_POINT ( 'NONE',  ( 0.8389417669273790956, 1409.109435131980035, 232.3914498246509766 ) ) ;
#105080=CARTESIAN_POINT ( 'NONE',  ( 14.75914027823870001, 1489.809285284449970, 193.8265667301440089 ) ) ;
#105081=CARTESIAN_POINT ( 'NONE',  ( 23.79022469739999934, 1430.448705190130113, 207.1593330058379934 ) ) ;
#105083=CARTESIAN_POINT ( 'NONE',  ( -23.94935474710000278, 1437.296773319940030, 211.9556018033580074 ) ) ;
#105085=CARTESIAN_POINT ( 'NONE',  ( -18.51562429780000230, 1509.322649224630140, 230.4822182655979645 ) ) ;
#105087=CARTESIAN_POINT ( 'NONE',  ( -11.14671771210699980, 1434.019356486030119, 151.6529807626459956 ) ) ;
#105088=CARTESIAN_POINT ( 'NONE',  ( 26.79413740735880367, 1436.761939593030093, 136.7822073642480234 ) ) ;
#105093=B_SPLINE_CURVE_WITH_KNOTS ( 'NONE', 5,
 ( #64283, #46935, #90552, #6004, #39612, #22223, #65386, #12753, #81592 ),
 .UNSPECIFIED., .F., .F.,
 ( 6, 3, 6 ),
 ( 91.71614156710000998, 91.73016858649999961, 101.6051519397803986 ),
 .UNSPECIFIED. ) ;
#105095=DIRECTION ( 'NONE',  ( -0.3363363969979660806, 0.9417419115949053898, 0.000000000000000000 ) ) ;
#105102=ORIENTED_EDGE ( 'NONE', *, *, #83005, .F. ) ;
#105106=CARTESIAN_POINT ( 'NONE',  ( 12.66098461250295593, 1442.798989634974077, 169.4635270419445305 ) ) ;
#105107=CARTESIAN_POINT ( 'NONE',  ( 29.82646034656356093, 1419.449848292917295, 269.4689676523768753 ) ) ;
#105108=CARTESIAN_POINT ( 'NONE',  ( -45.67178389499999724, 1440.913060392759917, 266.1886045325979921 ) ) ;
#105109=B_SPLINE_CURVE_WITH_KNOTS ( 'NONE', 5,
 ( #27887, #62070, #70473, #78856, #11637, #2165 ),
 .UNSPECIFIED., .F., .F.,
 ( 6, 6 ),
 ( 0.000000000000000000, 1.000000000000000000 ),
 .UNSPECIFIED. ) ;
#105112=CARTESIAN_POINT ( 'NONE',  ( -11.59421085610000013, 1433.816539371060117, 151.1950375012979748 ) ) ;
#105114=CARTESIAN_POINT ( 'NONE',  ( -19.19076381549999866, 1485.870189056229719, 189.6692896468980223 ) ) ;
#105116=CARTESIAN_POINT ( 'NONE',  ( 4.363122647530000009, 1421.971318475729959, 183.8271339139979830 ) ) ;
#105117=CARTESIAN_POINT ( 'NONE',  ( -9.273216395669999557, 1438.130896815179995, 153.0611341270980006 ) ) ;
#105128=CARTESIAN_POINT ( 'NONE',  ( -14.76285983090000187, 1469.689762253530034, 269.6387426946980099 ) ) ;
#105130=CARTESIAN_POINT ( 'NONE',  ( 6.558760908210000906, 1438.201672707379885, 154.7769642619979891 ) ) ;
#105131=CARTESIAN_POINT ( 'NONE',  ( -15.51935360190000068, 1506.809279358730009, 224.7680893556980095 ) ) ;
#105137=CARTESIAN_POINT ( 'NONE',  ( -44.85754428203180311, 1434.551014250809885, 268.9966666965190143 ) ) ;
#105145=CARTESIAN_POINT ( 'NONE',  ( -14.18063018520000007, 1425.417875233729774, 189.5894151879979859 ) ) ;
#105146=ADVANCED_FACE ( 'NONE', ( #95435 ), #51808, .F. ) ;
#105147=CARTESIAN_POINT ( 'NONE',  ( -27.02986278700840117, 1451.800463763470134, 135.6518028302020014 ) ) ;
#105152=B_SPLINE_CURVE_WITH_KNOTS ( 'NONE', 5,
 ( #92938, #40882, #8371, #76693, #25164, #40332 ),
 .UNSPECIFIED., .F., .F.,
 ( 6, 6 ),
 ( 0.000000000000000000, 1.000000000000000000 ),
 .UNSPECIFIED. ) ;
#105155=ORIENTED_EDGE ( 'NONE', *, *, #79640, .F. ) ;
#105156=CARTESIAN_POINT ( 'NONE',  ( -25.77614403568950152, 1416.582427450090108, 269.6950798014430006 ) ) ;
#105164=CARTESIAN_POINT ( 'NONE',  ( 45.44342259735076084, 1444.063149475110094, 268.9800971098556488 ) ) ;
#105166=CARTESIAN_POINT ( 'NONE',  ( -10.86110766952070605, 1438.504893499145965, 152.3919029481315874 ) ) ;
#105170=CARTESIAN_POINT ( 'NONE',  ( -21.27157138767482891, 1506.426094410640417, 214.6803200238785791 ) ) ;
#105171=CARTESIAN_POINT ( 'NONE',  ( -17.87298439029999741, 1430.801053286930028, 226.5401518608979927 ) ) ;
#105172=CARTESIAN_POINT ( 'NONE',  ( 15.86377822757070000, 1474.307034152129972, 268.3909166498499985 ) ) ;
#105173=CARTESIAN_POINT ( 'NONE',  ( 11.37414570439999828, 1415.063410501429871, 222.6977618391979945 ) ) ;
#105174=CARTESIAN_POINT ( 'NONE',  ( 3.860674342979999896, 1447.670908790060139, 184.2423422240979960 ) ) ;
#105178=CARTESIAN_POINT ( 'NONE',  ( 21.10423771450547292, 1411.010697888440063, 217.9724924710270102 ) ) ;
#105179=CARTESIAN_POINT ( 'NONE',  ( 1.517721997056749927, 1457.716913820190030, 183.2697976461230098 ) ) ;
#105182=CARTESIAN_POINT ( 'NONE',  ( 25.33603192065969978, 1451.791194868420007, 136.3363360771870134 ) ) ;
#105186=CARTESIAN_POINT ( 'NONE',  ( 17.80440947700000365, 1409.534804066629931, 196.0485523064980100 ) ) ;
#105187=FACE_OUTER_BOUND ( 'NONE', #51768, .T. ) ;
#105188=CARTESIAN_POINT ( 'NONE',  ( 2.991516284728592989, 1439.674840613275364, 184.0837186423407275 ) ) ;
#105189=CARTESIAN_POINT ( 'NONE',  ( -22.82498224624805516, 1432.425316134065952, 215.5066816192843362 ) ) ;
#105191=CARTESIAN_POINT ( 'NONE',  ( -4.518180742295140181E-06, 1509.047264790930058, 179.1218459713510072 ) ) ;
#105195=CARTESIAN_POINT ( 'NONE',  ( 26.05330421372899963, 1447.171924260989954, 137.7989882634119851 ) ) ;
#105197=CARTESIAN_POINT ( 'NONE',  ( -7.427207796130010031, 1509.244793066193324, 179.9842687496544613 ) ) ;
#105201=CIRCLE ( 'NONE', #103410, 2.000000000000068390 ) ;
#105202=CARTESIAN_POINT ( 'NONE',  ( -4.026786250540000722, 1432.413060387330006, 146.1721969590979882 ) ) ;
#105203=CARTESIAN_POINT ( 'NONE',  ( -39.36129609902809534, 1447.182057882140043, 136.6155912094569942 ) ) ;
#105206=CARTESIAN_POINT ( 'NONE',  ( -20.63825566599999917, 1456.438754565230056, 248.0989693021979861 ) ) ;
#105208=CARTESIAN_POINT ( 'NONE',  ( 11.79531744139999994, 1433.054727169869921, 150.6259952627979999 ) ) ;
#105209=CARTESIAN_POINT ( 'NONE',  ( -2.486951778696359749, 1446.758387635790086, 222.8330888875190112 ) ) ;
#105211=CARTESIAN_POINT ( 'NONE',  ( -21.12410134230000125, 1508.013533195929995, 227.5424588953979992 ) ) ;
#105214=FACE_OUTER_BOUND ( 'NONE', #74856, .T. ) ;
#105216=CARTESIAN_POINT ( 'NONE',  ( -13.69870936760000113, 1486.370890417729925, 185.2067811559980157 ) ) ;
#105218=DIRECTION ( 'NONE',  ( 0.000000000000000000, 0.000000000000000000, -1.000000000000000000 ) ) ;
#105220=CARTESIAN_POINT ( 'NONE',  ( 21.91488070589999992, 1449.791133979859978, 220.2443267750980169 ) ) ;
#105222=CARTESIAN_POINT ( 'NONE',  ( -12.86131642979999867, 1509.362187453730030, 235.2891919111980030 ) ) ;
#105225=CARTESIAN_POINT ( 'NONE',  ( 2.499943159395269898, 1419.755139738720118, 123.2722782263270034 ) ) ;
#105227=CARTESIAN_POINT ( 'NONE',  ( 0.1672222338998649860, 1481.964487760609927, 182.0100010911949937 ) ) ;
#105230=CARTESIAN_POINT ( 'NONE',  ( -1.546949756590000113, 1416.828042686930075, 228.0209011719979912 ) ) ;
#105232=CARTESIAN_POINT ( 'NONE',  ( -3.034145623640000178, 1440.440283128710007, 157.2495509660979849 ) ) ;
#105236=ORIENTED_EDGE ( 'NONE', *, *, #5748, .F. ) ;
#105238=CARTESIAN_POINT ( 'NONE',  ( -16.36865316639999790, 1414.913060387329779, 209.3429107935929778 ) ) ;
#105239=CARTESIAN_POINT ( 'NONE',  ( 28.77729953137099983, 1509.917985831029910, 206.0039978706130057 ) ) ;
#105242=CARTESIAN_POINT ( 'NONE',  ( 12.46263537197410010, 1409.348265197239925, 217.3636187787240033 ) ) ;
#105243=DIRECTION ( 'NONE',  ( 0.000000000000000000, 1.000000000000000000, -2.081668171172166620E-14 ) ) ;
#105245=CARTESIAN_POINT ( 'NONE',  ( -16.76281960579999719, 1413.995603259130121, 191.6500452088980069 ) ) ;
#105251=CARTESIAN_POINT ( 'NONE',  ( -12.15368974921969958, 1416.134159100540046, 194.7772796687779930 ) ) ;
#105253=CARTESIAN_POINT ( 'NONE',  ( 13.60370406562014622, 1469.851559027462599, 269.3580926999919143 ) ) ;
#105255=CARTESIAN_POINT ( 'NONE',  ( -0.006135579268280000158, 1395.974572298630164, 220.7500239771979693 ) ) ;
#105257=CARTESIAN_POINT ( 'NONE',  ( -0.1457309951619999711, 1455.055482580329908, 183.1213254899980143 ) ) ;
#105259=CARTESIAN_POINT ( 'NONE',  ( -26.63837744890847858, 1436.744137532187551, 136.7910871693582919 ) ) ;
#105262=CARTESIAN_POINT ( 'NONE',  ( -13.17555111980130000, 1435.420252581789782, 150.3576300310929810 ) ) ;
#105263=CARTESIAN_POINT ( 'NONE',  ( -1.931788062849999808E-14, 1421.852999791829916, 133.5962737641980027 ) ) ;
#105266=CARTESIAN_POINT ( 'NONE',  ( -16.93884325354670040, 1507.634939694479954, 230.1482608329069990 ) ) ;
#105270=VECTOR ( 'NONE', #47363, 1000.000000000000114 ) ;
#105271=CARTESIAN_POINT ( 'NONE',  ( 37.17588053200000076, 1423.049456354930044, 264.1764833033980153 ) ) ;
#105272=CARTESIAN_POINT ( 'NONE',  ( -26.57328462060000263, 1469.248969696529912, 208.7426067427740008 ) ) ;
#105273=CARTESIAN_POINT ( 'NONE',  ( -11.00536801767579931, 1426.523244036580081, 91.15358938771061048 ) ) ;
#105274=CARTESIAN_POINT ( 'NONE',  ( 3.263569602579999775E-14, 1416.961989284729952, 254.9666375902979780 ) ) ;
#105275=CARTESIAN_POINT ( 'NONE',  ( -20.39519499389999879, 1453.159462793029888, 208.3965248203290059 ) ) ;
#105276=CARTESIAN_POINT ( 'NONE',  ( -5.301749024289999390, 1413.741945239130018, 248.5896189572980006 ) ) ;
#105277=CARTESIAN_POINT ( 'NONE',  ( 19.73644163875970037, 1509.633137979659978, 231.2831758493399832 ) ) ;
#105279=CARTESIAN_POINT ( 'NONE',  ( 3.813631208918726312, 1447.061710304021517, 154.8462439947786038 ) ) ;
#105280=CARTESIAN_POINT ( 'NONE',  ( 31.78276358479999786, 1451.803508859929934, 135.2120624569979839 ) ) ;
#105281=EDGE_LOOP ( 'NONE', ( #88964, #98134, #65104, #92951 ) ) ;
#105282=CARTESIAN_POINT ( 'NONE',  ( -2.500000000000000000, 1430.723343392929792, 157.4401612927979954 ) ) ;
#105284=CARTESIAN_POINT ( 'NONE',  ( 14.10737876370000166, 1509.405700909230063, 234.8174633738979935 ) ) ;
#105285=ORIENTED_EDGE ( 'NONE', *, *, #51945, .F. ) ;
#105287=CARTESIAN_POINT ( 'NONE',  ( -29.22965625836564385, 1509.933782476033912, 211.7723397217503987 ) ) ;
#105288=CARTESIAN_POINT ( 'NONE',  ( -23.30841755010380112, 1409.842253946060055, 208.8031150648170353 ) ) ;
#105289=VERTEX_POINT ( 'NONE', #55658 ) ;
#105290=CARTESIAN_POINT ( 'NONE',  ( 0.5017934223950000217, 1413.835511642630081, 184.9211686299979931 ) ) ;
#105294=CARTESIAN_POINT ( 'NONE',  ( -5.701487894879999629, 1479.768604539729949, 234.8346338655979935 ) ) ;
#105296=VERTEX_POINT ( 'NONE', #89781 ) ;
#105297=CARTESIAN_POINT ( 'NONE',  ( 11.43732278620000109, 1425.481241381329937, 144.1613654183979918 ) ) ;
#105300=CARTESIAN_POINT ( 'NONE',  ( 13.84474581289999939, 1452.823898879430089, 224.2523962804980044 ) ) ;
#105304=CARTESIAN_POINT ( 'NONE',  ( 11.86490175767010058, 1432.252230835709952, 149.9817356757799871 ) ) ;
#105305=CARTESIAN_POINT ( 'NONE',  ( 13.41855466063566560, 1444.378506783447392, 187.7774200406155387 ) ) ;
#105306=VERTEX_POINT ( 'NONE', #13049 ) ;
#105308=CARTESIAN_POINT ( 'NONE',  ( -1.464145755870850163, 1482.281356462570102, 182.5701915244350175 ) ) ;
#105309=CARTESIAN_POINT ( 'NONE',  ( -17.22592482065197927, 1443.913060387330233, 162.9227486220069920 ) ) ;
#105312=CARTESIAN_POINT ( 'NONE',  ( -4.384282716360000443, 1424.957687000730175, 186.0191632644979904 ) ) ;
#105313=CARTESIAN_POINT ( 'NONE',  ( 0.9653168468964550275, 1409.211512109100113, 270.3713481135980032 ) ) ;
#105318=CARTESIAN_POINT ( 'NONE',  ( 0.02577720648996629366, 1410.273974002400792, 233.2210067926105239 ) ) ;
#105322=CARTESIAN_POINT ( 'NONE',  ( 17.60627508980000044, 1410.895669370830092, 224.8086596393980017 ) ) ;
#105325=CARTESIAN_POINT ( 'NONE',  ( 28.52406123459999776, 1430.067484666330074, 255.3819207742980097 ) ) ;
#105327=CARTESIAN_POINT ( 'NONE',  ( 18.64442764522555862, 1507.939506224435718, 188.5219863285041129 ) ) ;
#105335=ORIENTED_EDGE ( 'NONE', *, *, #28345, .T. ) ;
#105337=CARTESIAN_POINT ( 'NONE',  ( -24.59914094579999855, 1443.155180290510089, 210.8302193746780233 ) ) ;
#105340=DIRECTION ( 'NONE',  ( -1.000000000000000000, 0.000000000000000000, 0.000000000000000000 ) ) ;
#105343=DIRECTION ( 'NONE',  ( 0.9965178241646045487, -2.165862640214384426E-12, -0.08338001032766965970 ) ) ;
#105344=CARTESIAN_POINT ( 'NONE',  ( 21.91388558050159929, 1509.808238952129841, 230.0100389666999945 ) ) ;
#105346=CARTESIAN_POINT ( 'NONE',  ( -0.9776412681320001408, 1475.513060387329915, 230.7453403689980007 ) ) ;
#105347=CARTESIAN_POINT ( 'NONE',  ( 14.82212541029999819, 1417.425064580829940, 227.9176054998980021 ) ) ;
#105349=CARTESIAN_POINT ( 'NONE',  ( -16.05553604150000169, 1459.222164567730033, 229.6221585443979905 ) ) ;
#105351=CARTESIAN_POINT ( 'NONE',  ( 39.21111056970000419, 1422.625647128129913, 266.3742241808980111 ) ) ;
#105352=CARTESIAN_POINT ( 'NONE',  ( -17.56180752129999689, 1409.526332219330016, 223.5690793764979958 ) ) ;
#105353=CARTESIAN_POINT ( 'NONE',  ( 18.78564773260000109, 1435.583069123479845, 146.2005943789979767 ) ) ;
#105354=VECTOR ( 'NONE', #63747, 1000.000000000000114 ) ;
#105355=CARTESIAN_POINT ( 'NONE',  ( 21.29824326579999649, 1488.584156283829998, 192.5314371079979878 ) ) ;
#105356=CARTESIAN_POINT ( 'NONE',  ( -16.57644247905169976, 1409.993773362210050, 191.9232830829909915 ) ) ;
#105358=CARTESIAN_POINT ( 'NONE',  ( -16.45001201050000006, 1423.352090360930106, 227.1126878444979980 ) ) ;
#105361=CARTESIAN_POINT ( 'NONE',  ( -33.91368157693270291, 1437.010587976510124, 136.5611906174850105 ) ) ;
#105364=CARTESIAN_POINT ( 'NONE',  ( -13.13758325809999938, 1443.000245701009817, 187.0090600251980106 ) ) ;
#105367=ADVANCED_FACE ( 'NONE', ( #31518 ), #110679, .F. ) ;
#105368=CARTESIAN_POINT ( 'NONE',  ( -30.21730347749999979, 1435.712217778030208, 136.0584395910979651 ) ) ;
#105369=CARTESIAN_POINT ( 'NONE',  ( -6.862505600778585624, 1456.752482962994009, 227.8870320116735684 ) ) ;
#105370=VERTEX_POINT ( 'NONE', #15790 ) ;
#105372=CARTESIAN_POINT ( 'NONE',  ( 27.31525032189999891, 1439.464609863130136, 137.0827112581980032 ) ) ;
#105376=CARTESIAN_POINT ( 'NONE',  ( -33.98065672744881027, 1443.501467202838512, 154.9321739644268234 ) ) ;
#105377=CARTESIAN_POINT ( 'NONE',  ( -46.16776967539999532, 1440.913036915769908, 266.9714970989979861 ) ) ;
#105380=CARTESIAN_POINT ( 'NONE',  ( 0.2567085482048540035, 1419.518028698059879, 184.4201755903200137 ) ) ;
#105385=CARTESIAN_POINT ( 'NONE',  ( 12.95840179510000034, 1416.218047894730262, 221.5780309934980039 ) ) ;
#105386=CARTESIAN_POINT ( 'NONE',  ( 14.22134611999999976, 1463.286284084930003, 223.7238266604979628 ) ) ;
#105389=CARTESIAN_POINT ( 'NONE',  ( -3.540698356210000064, 1508.270058940830040, 180.7688477407980088 ) ) ;
#105391=CARTESIAN_POINT ( 'NONE',  ( -12.26815783919999880, 1415.553739807329976, 195.3528422598979830 ) ) ;
#105393=CARTESIAN_POINT ( 'NONE',  ( 24.08425203100000189, 1411.115211432230126, 209.6325621231380012 ) ) ;
#105397=CARTESIAN_POINT ( 'NONE',  ( -5.386185223340929973, 1432.347042777500064, 154.6076275972019971 ) ) ;
#105398=FACE_OUTER_BOUND ( 'NONE', #27076, .T. ) ;
#105400=CARTESIAN_POINT ( 'NONE',  ( 0.7091528421289999828, 1410.300367797830177, 233.1399324052979978 ) ) ;
#105403=CARTESIAN_POINT ( 'NONE',  ( -26.80147237664635185, 1509.848988426266942, 197.2601629728074499 ) ) ;
#105406=CARTESIAN_POINT ( 'NONE',  ( -18.37606861500000122, 1424.967732719430160, 227.5064700491979863 ) ) ;
#105407=CARTESIAN_POINT ( 'NONE',  ( -18.97278584537820123, 1486.247047112609835, 189.3002463451680057 ) ) ;
#105413=VERTEX_POINT ( 'NONE', #57316 ) ;
#105414=CARTESIAN_POINT ( 'NONE',  ( 27.13583296430000047, 1509.164684264529797, 215.3181691316380011 ) ) ;
#105417=CARTESIAN_POINT ( 'NONE',  ( 1.547463840030000037, 1414.913060387329779, 192.3096136973980208 ) ) ;
#105418=CARTESIAN_POINT ( 'NONE',  ( 15.91223255370150014, 1418.658837366640000, 191.2758984395539983 ) ) ;
#105419=CARTESIAN_POINT ( 'NONE',  ( 23.35526608410000193, 1448.827836771670036, 218.6598503475479731 ) ) ;
#105420=CARTESIAN_POINT ( 'NONE',  ( 4.026786250540000722, 1421.741487512030062, 169.4417495807979890 ) ) ;
#105421=VECTOR ( 'NONE', #25344, 1000.000000000000114 ) ;
#105422=CARTESIAN_POINT ( 'NONE',  ( -25.57416082987599992, 1451.572412185829990, 136.5135885075040107 ) ) ;
#105423=CARTESIAN_POINT ( 'NONE',  ( 8.622487674225027376, 1440.776277238063585, 153.7651958641682768 ) ) ;
#105424=CARTESIAN_POINT ( 'NONE',  ( 13.71870890039999935, 1409.558843311929877, 227.5656532589979975 ) ) ;
#105425=EDGE_CURVE ( 'NONE', #54104, #86029, #80578, .T. ) ;
#105428=CARTESIAN_POINT ( 'NONE',  ( 41.63323805095519958, 1443.027121608840162, 134.0999999981200119 ) ) ;
#105431=ORIENTED_EDGE ( 'NONE', *, *, #16760, .F. ) ;
#105435=ORIENTED_EDGE ( 'NONE', *, *, #80868, .T. ) ;
#105436=ORIENTED_EDGE ( 'NONE', *, *, #10291, .T. ) ;
#105440=CARTESIAN_POINT ( 'NONE',  ( 15.81648005058062090, 1451.124245892486215, 149.1749219823134638 ) ) ;
#105441=CARTESIAN_POINT ( 'NONE',  ( -3.089264994810000164, 1485.815196309429894, 182.5613893784980064 ) ) ;
#105444=CARTESIAN_POINT ( 'NONE',  ( -17.39703151571873008, 1448.459128900735550, 218.4035087908428352 ) ) ;
#105448=EDGE_LOOP ( 'NONE', ( #52270, #42017, #12883, #83822 ) ) ;
#105450=VERTEX_POINT ( 'NONE', #23671 ) ;
#105451=CARTESIAN_POINT ( 'NONE',  ( 32.16729354855799983, 1440.913060387330006, 256.2481582175259973 ) ) ;
#105452=CARTESIAN_POINT ( 'NONE',  ( -15.33686075110000147, 1509.107788877129906, 184.5497581577979815 ) ) ;
#105454=CARTESIAN_POINT ( 'NONE',  ( 26.69188107298460011, 1449.953547536330007, 136.5849450126470117 ) ) ;
#105455=CARTESIAN_POINT ( 'NONE',  ( -14.33393486070000122, 1409.413612422530150, 192.0174323315980018 ) ) ;
#105460=CARTESIAN_POINT ( 'NONE',  ( 13.90496272978541725, 1414.913060387330006, 217.4955100473378025 ) ) ;
#105462=CARTESIAN_POINT ( 'NONE',  ( -12.06107998010000060, 1433.903545125019946, 148.5637427420979861 ) ) ;
#105465=CARTESIAN_POINT ( 'NONE',  ( 10.27415084429999936, 1462.789161984029761, 234.7156815036980220 ) ) ;
#105468=B_SPLINE_SURFACE_WITH_KNOTS ( 'NONE', 5, 5, ( 
 ( #86826, #26926, #35883, #44289, #86271, #70067, #1188, #104179, #53247 ),
 ( #9557, #76774, #27463, #43727, #25795, #94112, #43184, #110370, #85163 ),
 ( #61115, #33649, #42622, #90, #95230, #34767, #18494, #10117, #52690 ),
 ( #102505, #87388, #34215, #69506, #67843, #77880, #78433, #76226, #68401 ),
 ( #59994, #17383, #61651, #638, #101954, #103056, #10683, #52139, #95778 ),
 ( #19045, #59444, #17943, #25241, #26354, #93555, #35319, #8449, #51582 ),
 ( #16827, #94672, #51028, #85714, #77336, #9010, #60550, #103628, #63852 ),
 ( #81169, #80634, #3948, #44851, #89019, #96888, #104729, #20698, #97964 ),
 ( #54894, #64400, #4484, #45939, #55991, #90114, #21234, #3396, #29667 ) ),
 .UNSPECIFIED., .F., .F., .F.,
 ( 6, 3, 6 ),
 ( 6, 3, 6 ),
 ( -1.001153178291219951E-05, 19.90003809979999971, 45.10384108370000433 ),
 ( 0.000000000000000000, 1.000000000000000000, 2.000010011531780041 ),
 .UNSPECIFIED. ) ;
#105472=CARTESIAN_POINT ( 'NONE',  ( 28.44347333380000364, 1509.158830953930192, 208.5401038306789872 ) ) ;
#105474=CARTESIAN_POINT ( 'NONE',  ( -18.85453636469999950, 1434.822352678670086, 209.3473311023250005 ) ) ;
#105477=ORIENTED_EDGE ( 'NONE', *, *, #28178, .T. ) ;
#105478=CARTESIAN_POINT ( 'NONE',  ( 0.000000000000000000, 1452.913060387330006, 179.9625354391980068 ) ) ;
#105480=CARTESIAN_POINT ( 'NONE',  ( 31.69751081770000312, 1445.012237274630024, 244.1892870184980211 ) ) ;
#105484=CARTESIAN_POINT ( 'NONE',  ( -19.44003422200000131, 1456.042540789730083, 227.5400276923980130 ) ) ;
#105485=CARTESIAN_POINT ( 'NONE',  ( -18.74957845327451622, 1410.930162482557989, 196.2665709180884051 ) ) ;
#105486=CARTESIAN_POINT ( 'NONE',  ( 5.359829535970479952, 1422.291879003420036, 145.7409380638519849 ) ) ;
#105491=CARTESIAN_POINT ( 'NONE',  ( 0.7780366837319999673, 1405.780753921430005, 268.4835186043979434 ) ) ;
#105494=CARTESIAN_POINT ( 'NONE',  ( 42.06232253459919690, 1445.825096420900081, 269.6487541258160263 ) ) ;
#105496=CARTESIAN_POINT ( 'NONE',  ( 2.478947879950000210, 1432.276406471479959, 157.5139433850980026 ) ) ;
#105497=CARTESIAN_POINT ( 'NONE',  ( 10.75950721900864693, 1424.480083424939039, 137.8581109189600227 ) ) ;
#105499=CARTESIAN_POINT ( 'NONE',  ( -43.93650039737229918, 1440.913060405460101, 264.2825071479210237 ) ) ;
#105501=CARTESIAN_POINT ( 'NONE',  ( 1.746243614909547714, 1450.465158970312586, 154.2919968866931981 ) ) ;
#105508=ORIENTED_EDGE ( 'NONE', *, *, #62202, .F. ) ;
#105510=CARTESIAN_POINT ( 'NONE',  ( 5.995204332980000249E-15, 1419.211677883429957, 248.0989693021979861 ) ) ;
#105513=CARTESIAN_POINT ( 'NONE',  ( -0.1062961612130000066, 1475.048391926030035, 269.6500679733979950 ) ) ;
#105514=CARTESIAN_POINT ( 'NONE',  ( -27.77560365120000085, 1451.943158935029942, 134.8960326030979786 ) ) ;
#105518=AXIS2_PLACEMENT_3D ( 'NONE', #91626, #49094, #83229 ) ;
#105519=CARTESIAN_POINT ( 'NONE',  ( -18.89905511659999959, 1416.828040475729949, 207.5748962040180174 ) ) ;
#105520=DIRECTION ( 'NONE',  ( 1.000000000000000000, 0.000000000000000000, 0.000000000000000000 ) ) ;
#105521=CARTESIAN_POINT ( 'NONE',  ( 26.23576681230780139, 1435.413602865789926, 135.4068554872490040 ) ) ;
#105522=CARTESIAN_POINT ( 'NONE',  ( -9.802578310169730358, 1396.255373964939963, 214.2508701772540007 ) ) ;
#105523=EDGE_CURVE ( 'NONE', #24414, #4089, #43249, .T. ) ;
#105525=CARTESIAN_POINT ( 'NONE',  ( -15.49426842564200157, 1421.633204956707914, 227.2929607267749930 ) ) ;
#105526=CARTESIAN_POINT ( 'NONE',  ( -16.49508940950000024, 1409.737691204929888, 225.9011186669980304 ) ) ;
#105527=CARTESIAN_POINT ( 'NONE',  ( 19.41800382249774515, 1455.667198361140663, 225.5846027043448032 ) ) ;
#105528=ORIENTED_EDGE ( 'NONE', *, *, #41168, .T. ) ;
#105531=EDGE_CURVE ( 'NONE', #104116, #19921, #46465, .T. ) ;
#105532=CARTESIAN_POINT ( 'NONE',  ( -18.43641199600227765, 1485.257797375915743, 189.1831268613264854 ) ) ;
#105533=CARTESIAN_POINT ( 'NONE',  ( 10.91367058839999871, 1425.302818804329945, 128.4898600348980153 ) ) ;
#105535=CARTESIAN_POINT ( 'NONE',  ( 5.157704406284129827E-09, 1406.911841301380036, 222.1218459627310153 ) ) ;
#105536=EDGE_CURVE ( 'NONE', #65282, #64454, #17666, .T. ) ;
#105541=CARTESIAN_POINT ( 'NONE',  ( -9.634835741540001663, 1430.981823154709900, 148.7079730222979776 ) ) ;
#105542=CARTESIAN_POINT ( 'NONE',  ( 5.469793405669999942, 1507.795163446829747, 181.9824978760979945 ) ) ;
#105545=ADVANCED_FACE ( 'NONE', ( #35950 ), #35627, .F. ) ;
#105549=B_SPLINE_CURVE_WITH_KNOTS ( 'NONE', 3,
 ( #31374, #39223, #46005, #80693 ),
 .UNSPECIFIED., .F., .F.,
 ( 4, 4 ),
 ( -14.36013183198100052, -6.524295923422950061 ),
 .UNSPECIFIED. ) ;
#105551=CARTESIAN_POINT ( 'NONE',  ( -7.536504302460000027, 1396.176240917429823, 200.3138106880579983 ) ) ;
#105552=CARTESIAN_POINT ( 'NONE',  ( 1.189285361496680071, 1507.141006053059982, 237.0337565598269975 ) ) ;
#105556=CARTESIAN_POINT ( 'NONE',  ( 17.77263048209999852, 1416.284038623030028, 224.9649977725980250 ) ) ;
#105558=CARTESIAN_POINT ( 'NONE',  ( 1.838213786079999856, 1410.306157565029935, 185.3985639462979975 ) ) ;
#105562=CARTESIAN_POINT ( 'NONE',  ( -2.500000000000000000, 1448.365115610690054, 162.8856519709460144 ) ) ;
#105563=DIRECTION ( 'NONE',  ( 0.000000000000000000, -0.7071067811865474617, -0.7071067811865474617 ) ) ;
#105564=CARTESIAN_POINT ( 'NONE',  ( -27.13955216900179934, 1438.563659682299885, 136.9826056857960168 ) ) ;
#105565=CARTESIAN_POINT ( 'NONE',  ( -1.532227443785459942, 1405.761751320050053, 267.5364479672910534 ) ) ;
#105566=CARTESIAN_POINT ( 'NONE',  ( -27.69925886641940238, 1441.434395751479997, 137.3015763626259798 ) ) ;
#105567=ORIENTED_EDGE ( 'NONE', *, *, #57744, .T. ) ;
#105569=CARTESIAN_POINT ( 'NONE',  ( 12.84752083859999949, 1442.662704864849957, 187.9133791926979882 ) ) ;
#105571=ORIENTED_EDGE ( 'NONE', *, *, #14854, .T. ) ;
#105577=ORIENTED_EDGE ( 'NONE', *, *, #65200, .F. ) ;
#105578=CARTESIAN_POINT ( 'NONE',  ( -8.928474135859682193, 1509.321320493349958, 180.3286574278590138 ) ) ;
#105584=AXIS2_PLACEMENT_3D ( 'NONE', #99446, #12151, #47963 ) ;
#105585=CARTESIAN_POINT ( 'NONE',  ( -35.61911272319999711, 1440.913060387330006, 261.9797944256979463 ) ) ;
#105586=B_SPLINE_SURFACE_WITH_KNOTS ( 'NONE', 3, 1, ( 
 ( #109788, #33605 ),
 ( #15686, #32532 ),
 ( #85672, #49892 ),
 ( #46, #85122 ),
 ( #42582, #24100 ),
 ( #66703, #94073 ) ),
 .UNSPECIFIED., .F., .F., .F.,
 ( 4, 2, 4 ),
 ( 2, 2 ),
 ( 0.000000000000000000, 0.4999999999999998890, 1.000000000000000000 ),
 ( 0.000000000000000000, 1.000000000000000000 ),
 .UNSPECIFIED. ) ;
#105587=CARTESIAN_POINT ( 'NONE',  ( -40.71298012283864409, 1433.226053685588113, 269.6231774168464881 ) ) ;
#105588=CARTESIAN_POINT ( 'NONE',  ( -4.434803163540000703, 1409.571684121930048, 231.8514698793979960 ) ) ;
#105591=ORIENTED_EDGE ( 'NONE', *, *, #90567, .T. ) ;
#105593=CARTESIAN_POINT ( 'NONE',  ( 33.52142403570000084, 1451.742483455429920, 134.7272099485979879 ) ) ;
#105595=CARTESIAN_POINT ( 'NONE',  ( -1.465793917108519917, 1484.360957496709943, 182.4810413606819850 ) ) ;
#105596=CARTESIAN_POINT ( 'NONE',  ( 15.56469051819999905, 1506.798305132829910, 225.0756798403980099 ) ) ;
#105598=CARTESIAN_POINT ( 'NONE',  ( 29.18127911709999722, 1415.346630214729885, 269.9487154676979799 ) ) ;
#105601=CARTESIAN_POINT ( 'NONE',  ( -11.26183798051521734, 1427.523654888847886, 223.7584288158600714 ) ) ;
#105606=CARTESIAN_POINT ( 'NONE',  ( 4.282777390491250280, 1420.607940666440072, 185.6069246241769974 ) ) ;
#105607=CARTESIAN_POINT ( 'NONE',  ( -1.870446701440000137, 1420.451316163830143, 233.2770772963979766 ) ) ;
#105612=CARTESIAN_POINT ( 'NONE',  ( 18.96350866050000050, 1416.837080243330092, 210.2430642888180046 ) ) ;
#105614=EDGE_CURVE ( 'NONE', #75668, #36772, #68493, .T. ) ;
#105616=FACE_OUTER_BOUND ( 'NONE', #107460, .T. ) ;
#105617=CARTESIAN_POINT ( 'NONE',  ( -0.08623196090545810766, 1420.451368587459910, 182.6995769445769895 ) ) ;
#105621=CARTESIAN_POINT ( 'NONE',  ( 18.97264949710000081, 1509.488247120830010, 187.2484463636980081 ) ) ;
#105622=FACE_OUTER_BOUND ( 'NONE', #92185, .T. ) ;
#105623=VERTEX_POINT ( 'NONE', #102302 ) ;
#105632=CARTESIAN_POINT ( 'NONE',  ( -26.67785352284090195, 1509.032684147069858, 201.4103146283430021 ) ) ;
#105634=CARTESIAN_POINT ( 'NONE',  ( -2.704720143830000367, 1447.053020115450181, 167.4681766834979726 ) ) ;
#105635=CARTESIAN_POINT ( 'NONE',  ( -17.60866373010000174, 1424.118365038330012, 226.6925037000980012 ) ) ;
#105640=CARTESIAN_POINT ( 'NONE',  ( 0.3105706251539200324, 1408.923906415619967, 232.1808711561190250 ) ) ;
#105641=CARTESIAN_POINT ( 'NONE',  ( -18.96055153501447421, 1439.098414281957730, 210.2943801834743454 ) ) ;
#105648=CARTESIAN_POINT ( 'NONE',  ( -24.15153577330000090, 1438.063256318689810, 212.1983434544380032 ) ) ;
#105650=CARTESIAN_POINT ( 'NONE',  ( -18.59438479510000164, 1507.626747889230046, 229.7138951080980007 ) ) ;
#105653=CARTESIAN_POINT ( 'NONE',  ( -24.89839821108130025, 1440.936833924440180, 210.4291215488500200 ) ) ;
#105655=EDGE_CURVE ( 'NONE', #36202, #41783, #104573, .T. ) ;
#105656=EDGE_CURVE ( 'NONE', #59250, #87156, #33749, .T. ) ;
#105664=ORIENTED_EDGE ( 'NONE', *, *, #50251, .T. ) ;
#105667=CARTESIAN_POINT ( 'NONE',  ( 20.03226456047849879, 1509.090742603719946, 229.7466210559209969 ) ) ;
#105669=ORIENTED_EDGE ( 'NONE', *, *, #76878, .T. ) ;
#105670=CARTESIAN_POINT ( 'NONE',  ( 17.13018491840009716, 1414.971993471370070, 210.1258406375170011 ) ) ;
#105671=CARTESIAN_POINT ( 'NONE',  ( 13.03597514149999981, 1508.085462669229855, 233.2284867411979974 ) ) ;
#105672=CARTESIAN_POINT ( 'NONE',  ( 13.33697072603180622, 1443.292755780022844, 169.3747417453497235 ) ) ;
#105673=CARTESIAN_POINT ( 'NONE',  ( 29.81586140656836292, 1419.442089572837176, 269.4688564823842398 ) ) ;
#105674=CARTESIAN_POINT ( 'NONE',  ( -5.038677013370000068, 1466.838857908529917, 244.5742075694979860 ) ) ;
#105675=CARTESIAN_POINT ( 'NONE',  ( -20.37201606160000367, 1506.520234984129957, 189.4987160947980271 ) ) ;
#105676=CARTESIAN_POINT ( 'NONE',  ( -11.86277575849999977, 1433.458230554240117, 150.5156657703979874 ) ) ;
#105678=CARTESIAN_POINT ( 'NONE',  ( -19.62677431030000008, 1486.135797666930102, 190.0069177851979987 ) ) ;
#105679=CARTESIAN_POINT ( 'NONE',  ( 6.022115808500000611, 1410.057305242329903, 186.7793557827980067 ) ) ;
#105680=CARTESIAN_POINT ( 'NONE',  ( 4.921337687010000295, 1421.568449892030003, 185.6518752963980035 ) ) ;
#105682=EDGE_CURVE ( 'NONE', #89942, #72154, #3063, .T. ) ;
#105683=CARTESIAN_POINT ( 'NONE',  ( 7.259422694309999535, 1440.164840772029947, 154.1325276865980243 ) ) ;
#105686=B_SPLINE_CURVE_WITH_KNOTS ( 'NONE', 3,
 ( #78755, #59757, #60305, #94425 ),
 .UNSPECIFIED., .F., .F.,
 ( 4, 4 ),
 ( 0.000000000000000000, 1.000000000000000000 ),
 .UNSPECIFIED. ) ;
#105687=CARTESIAN_POINT ( 'NONE',  ( -9.384832308269999146, 1452.150223719329915, 152.4418518133980172 ) ) ;
#105690=ORIENTED_EDGE ( 'NONE', *, *, #15109, .T. ) ;
#105693=CARTESIAN_POINT ( 'NONE',  ( -33.10222556109999914, 1460.414048409229963, 269.7553217547979898 ) ) ;
#105695=CARTESIAN_POINT ( 'NONE',  ( 6.484578373979999810, 1434.540925522399903, 154.7070604761979951 ) ) ;
#105700=CIRCLE ( 'NONE', #59180, 2.000000000730000949 ) ;
#105703=CARTESIAN_POINT ( 'NONE',  ( -45.82251511589010562, 1436.720346514069888, 268.2155769059959880 ) ) ;
#105705=CARTESIAN_POINT ( 'NONE',  ( -3.532607207562010299, 1491.098995286199852, 181.6594233187500151 ) ) ;
#105706=EDGE_LOOP ( 'NONE', ( #100562, #102416, #81247, #69872 ) ) ;
#105708=CIRCLE ( 'NONE', #86018, 1.500000000000001332 ) ;
#105710=CARTESIAN_POINT ( 'NONE',  ( -20.61551574950000187, 1508.364577319530099, 190.3819664504979983 ) ) ;
#105711=CARTESIAN_POINT ( 'NONE',  ( -15.55320418710000041, 1425.421141778929950, 190.3538950101980163 ) ) ;
#105713=ORIENTED_EDGE ( 'NONE', *, *, #9714, .F. ) ;
#105721=CARTESIAN_POINT ( 'NONE',  ( -19.35248331488120144, 1411.084690813580210, 270.2222661304289772 ) ) ;
#105723=CARTESIAN_POINT ( 'NONE',  ( 3.620601295783090201, 1417.932068788450124, 233.8910581729880391 ) ) ;
#105728=CARTESIAN_POINT ( 'NONE',  ( 45.62376250662960331, 1441.740454976975570, 268.9751154461204692 ) ) ;
#105730=CARTESIAN_POINT ( 'NONE',  ( -8.178500771994089646, 1441.152429774469965, 153.9860759686779943 ) ) ;
#105731=CARTESIAN_POINT ( 'NONE',  ( -0.006923030120857438796, 1408.920737911269953, 186.3147001159109948 ) ) ;
#105732=CIRCLE ( 'NONE', #57466, 29.84605316870980829 ) ;
#105734=CARTESIAN_POINT ( 'NONE',  ( -18.07596433670000025, 1430.799689938030269, 226.2266804869980206 ) ) ;
#105735=CARTESIAN_POINT ( 'NONE',  ( -14.20204669740000014, 1416.837080256030276, 221.7382503415979897 ) ) ;
#105736=CARTESIAN_POINT ( 'NONE',  ( 11.95871496589999872, 1415.628674276829770, 223.2763524143979907 ) ) ;
#105737=CARTESIAN_POINT ( 'NONE',  ( -17.37024900971054109, 1422.638029353652428, 226.5732080476987562 ) ) ;
#105743=CARTESIAN_POINT ( 'NONE',  ( 4.562141516099857519, 1457.338505932022372, 228.3743572140680556 ) ) ;
#105745=CARTESIAN_POINT ( 'NONE',  ( 23.96827632182870005, 1452.076072134780134, 136.6874999515719935 ) ) ;
#105746=FACE_OUTER_BOUND ( 'NONE', #47784, .T. ) ;
#105748=DIRECTION ( 'NONE',  ( 0.9965074780645594155, -0.004098122787112013637, -0.08340294689657867799 ) ) ;
#105749=CARTESIAN_POINT ( 'NONE',  ( 20.11149129760000065, 1409.615369146429884, 200.2383580101779899 ) ) ;
#105750=CARTESIAN_POINT ( 'NONE',  ( -4.054154399340952786, 1446.253642567111228, 170.5365981393944992 ) ) ;
#105751=CARTESIAN_POINT ( 'NONE',  ( 17.31558285710000078, 1410.013623662029886, 225.5276143365979920 ) ) ;
#105753=CARTESIAN_POINT ( 'NONE',  ( 19.44117294853580091, 1456.941945407359981, 224.4539793896520052 ) ) ;
#105754=CARTESIAN_POINT ( 'NONE',  ( 2.500000000000270450, 1439.222450974139974, 159.1124396249019810 ) ) ;
#105757=ORIENTED_EDGE ( 'NONE', *, *, #70167, .F. ) ;
#105761=LINE ( 'NONE', #80549, #41078 ) ;
#105762=CARTESIAN_POINT ( 'NONE',  ( 11.90008666459999986, 1434.920851464509951, 147.6452002888979962 ) ) ;
#105763=CARTESIAN_POINT ( 'NONE',  ( -38.67142060801120351, 1448.149028305610045, 136.4729251882360188 ) ) ;
#105764=CARTESIAN_POINT ( 'NONE',  ( 10.85931684761558458, 1424.796817104864203, 138.1961031260640311 ) ) ;
#105765=CARTESIAN_POINT ( 'NONE',  ( 1.930776842151626926, 1417.106403351838935, 232.9720933022255167 ) ) ;
#105766=CARTESIAN_POINT ( 'NONE',  ( -3.721063415729999695E-09, 1475.837061091930082, 266.9611530633980010 ) ) ;
#105767=CARTESIAN_POINT ( 'NONE',  ( 11.13931297870000137, 1433.088362659679888, 151.6441982395979835 ) ) ;
#105775=CARTESIAN_POINT ( 'NONE',  ( 22.68012700155740191, 1507.275789587059990, 209.7693291172490149 ) ) ;
#105777=EDGE_CURVE ( 'NONE', #77212, #85181, #98873, .T. ) ;
#105781=CARTESIAN_POINT ( 'NONE',  ( 1.894852802010000170, 1507.091060773529989, 236.3260084363980127 ) ) ;
#105782=EDGE_CURVE ( 'NONE', #80633, #68673, #54703, .T. ) ;
#105784=CARTESIAN_POINT ( 'NONE',  ( -11.99699175549999985, 1508.052959061330057, 233.6129359570980171 ) ) ;
#105787=CARTESIAN_POINT ( 'NONE',  ( 10.68290885440000082, 1409.286115784929962, 219.9879125262980040 ) ) ;
#105790=CARTESIAN_POINT ( 'NONE',  ( -10.29630665101337073, 1435.300287559097114, 152.3007955122366184 ) ) ;
#105791=VERTEX_POINT ( 'NONE', #89380 ) ;
#105792=CARTESIAN_POINT ( 'NONE',  ( -1.216112039750000040, 1452.488429528330016, 183.6485174699979837 ) ) ;
#105795=CARTESIAN_POINT ( 'NONE',  ( -3.023153272364219823, 1440.625623213970130, 157.2242917382399980 ) ) ;
#105796=CARTESIAN_POINT ( 'NONE',  ( -17.15013451049770055, 1414.913057819779851, 207.6647986024049999 ) ) ;
#105807=CARTESIAN_POINT ( 'NONE',  ( 13.48456462084389962, 1409.383951757389923, 215.5448620521310090 ) ) ;
#105811=CARTESIAN_POINT ( 'NONE',  ( -19.12773309319999981, 1463.218120443330008, 191.1290552211980014 ) ) ;
#105818=CARTESIAN_POINT ( 'NONE',  ( -12.00789815305109975, 1415.778512723939912, 194.9196753816330272 ) ) ;
#105820=CARTESIAN_POINT ( 'NONE',  ( 30.03297113387935013, 1462.224093527517880, 269.4711606006897568 ) ) ;
#105822=CARTESIAN_POINT ( 'NONE',  ( 5.071972357519999974, 1397.441751889229863, 221.0975735167979792 ) ) ;
#105824=CARTESIAN_POINT ( 'NONE',  ( -1.441435333030000043, 1455.080611006229901, 183.7350912959979894 ) ) ;
#105826=CARTESIAN_POINT ( 'NONE',  ( -26.28247728721726162, 1436.705573956322723, 136.8563548585942726 ) ) ;
#105828=CARTESIAN_POINT ( 'NONE',  ( -13.10870366159999989, 1435.054409783779874, 149.9910397837979872 ) ) ;
#105830=CARTESIAN_POINT ( 'NONE',  ( 1.342027776509999937, 1416.827520077930103, 190.1634478202980176 ) ) ;
#105832=CARTESIAN_POINT ( 'NONE',  ( -15.97576971693890080, 1477.217383298640016, 229.1973553141059767 ) ) ;
#105836=CARTESIAN_POINT ( 'NONE',  ( -26.99303384999999977, 1488.687911585429902, 206.6276365953079903 ) ) ;
#105837=CARTESIAN_POINT ( 'NONE',  ( -9.971616305214038078, 1425.233230934379890, 92.74877973774999873 ) ) ;
#105838=FACE_OUTER_BOUND ( 'NONE', #19800, .T. ) ;
#105839=CARTESIAN_POINT ( 'NONE',  ( 1.716045945209999868, 1509.007693206030126, 179.5167849949980052 ) ) ;
#105840=CARTESIAN_POINT ( 'NONE',  ( -26.00754374319999940, 1427.792721086330175, 240.2274373024979752 ) ) ;
#105841=CARTESIAN_POINT ( 'NONE',  ( 20.59987592950000135, 1509.677367935830262, 230.5839143914980127 ) ) ;
#105842=CARTESIAN_POINT ( 'NONE',  ( 0.9825367709745502776, 1415.585804587858775, 233.1616798236157990 ) ) ;
#105843=CARTESIAN_POINT ( 'NONE',  ( 33.14937533060000163, 1451.602147045430002, 135.6094880980980122 ) ) ;
#105845=CARTESIAN_POINT ( 'NONE',  ( -5.386516158502840490, 1432.363696384169998, 154.6077582407299928 ) ) ;
#105848=ORIENTED_EDGE ( 'NONE', *, *, #5732, .F. ) ;
#105854=CARTESIAN_POINT ( 'NONE',  ( -0.7163550209979999694, 1413.835382546030132, 184.9556001181979923 ) ) ;
#105856=CARTESIAN_POINT ( 'NONE',  ( 0.3483522942510000053, 1452.334144580529937, 183.2984807459980061 ) ) ;
#105857=CARTESIAN_POINT ( 'NONE',  ( -1.072720051239999917, 1489.064677756729907, 236.4182509688979792 ) ) ;
#105858=CARTESIAN_POINT ( 'NONE',  ( -1.288405174186285418, 1419.848498354222329, 185.1203288673806924 ) ) ;
#105860=CARTESIAN_POINT ( 'NONE',  ( 11.63661014589999887, 1425.864895317229866, 144.1626081066980021 ) ) ;
#105861=CARTESIAN_POINT ( 'NONE',  ( -12.31551432481460040, 1414.913060387399810, 219.9842977860079998 ) ) ;
#105862=CARTESIAN_POINT ( 'NONE',  ( 14.86247180250000000, 1485.705779184129824, 225.2758283624980038 ) ) ;
#105865=ORIENTED_EDGE ( 'NONE', *, *, #22789, .F. ) ;
#105866=CARTESIAN_POINT ( 'NONE',  ( 11.86444742414140130, 1432.220480012309963, 149.9811424069689849 ) ) ;
#105867=CARTESIAN_POINT ( 'NONE',  ( 12.72342974552460682, 1445.008495287113647, 186.4128679283859356 ) ) ;
#105868=ORIENTED_EDGE ( 'NONE', *, *, #26363, .T. ) ;
#105869=VERTEX_POINT ( 'NONE', #48789 ) ;
#105870=CARTESIAN_POINT ( 'NONE',  ( -18.18137283769999968, 1507.546748828630143, 231.7129783355979669 ) ) ;
#105874=DIRECTION ( 'NONE',  ( 0.6987313624946034363, 0.07895079864675673409, -0.7110142434997167582 ) ) ;
#105875=CARTESIAN_POINT ( 'NONE',  ( 0.9866695707572261664, 1407.933421795380127, 270.2925939168970331 ) ) ;
#105876=CARTESIAN_POINT ( 'NONE',  ( -4.146782895030730387, 1426.018316030089863, 186.1121555109529879 ) ) ;
#105878=CARTESIAN_POINT ( 'NONE',  ( -19.94575122458989469, 1509.638991226211601, 231.0845654444641468 ) ) ;
#105879=CARTESIAN_POINT ( 'NONE',  ( 0.03112280646364588149, 1410.164110630448931, 233.2100737522354734 ) ) ;
#105883=CARTESIAN_POINT ( 'NONE',  ( -24.95049239925220164, 1509.561083361290002, 222.7521736304589979 ) ) ;
#105886=CARTESIAN_POINT ( 'NONE',  ( 10.04572263670000076, 1417.623152644130187, 255.3819207803980191 ) ) ;
#105888=B_SPLINE_CURVE_WITH_KNOTS ( 'NONE', 4,
 ( #32149, #5856, #108305, #109968, #50072 ),
 .UNSPECIFIED., .F., .F.,
 ( 5, 5 ),
 ( 1.967616199060000071, 3.613988937050000239 ),
 .UNSPECIFIED. ) ;
#105889=CARTESIAN_POINT ( 'NONE',  ( 18.67054467737644075, 1509.506033878418975, 187.1506692568550534 ) ) ;
#105898=CARTESIAN_POINT ( 'NONE',  ( 12.71038982811789886, 1507.471771741610155, 233.3404631503599944 ) ) ;
#105901=EDGE_CURVE ( 'NONE', #65085, #29403, #8492, .T. ) ;
#105903=CARTESIAN_POINT ( 'NONE',  ( -12.30608628080000067, 1442.741623762909967, 186.5150421474980078 ) ) ;
#105904=CARTESIAN_POINT ( 'NONE',  ( 19.38267550565620212, 1509.603095404120040, 231.8230532176900169 ) ) ;
#105906=CARTESIAN_POINT ( 'NONE',  ( 12.63095811414796898, 1434.552017584898522, 149.3952382085417696 ) ) ;
#105907=CARTESIAN_POINT ( 'NONE',  ( 15.96415235769999974, 1412.748275509629821, 227.0251384850979832 ) ) ;
#105911=CARTESIAN_POINT ( 'NONE',  ( 45.97783906840000157, 1436.874426342759989, 266.9777547047980306 ) ) ;
#105912=CARTESIAN_POINT ( 'NONE',  ( -17.93887750940000103, 1409.704405018330135, 223.7856054849979728 ) ) ;
#105913=CARTESIAN_POINT ( 'NONE',  ( 16.37332010780000147, 1435.060612807570124, 147.2880571655980191 ) ) ;
#105914=CARTESIAN_POINT ( 'NONE',  ( 26.86204967519999798, 1508.007394501330054, 206.2315949059079969 ) ) ;
#105915=CARTESIAN_POINT ( 'NONE',  ( 29.77439797945870126, 1509.998809754348486, 209.4099699424615153 ) ) ;
#105918=CARTESIAN_POINT ( 'NONE',  ( -23.58453086489999961, 1470.876928620230046, 266.7402721287979830 ) ) ;
#105922=CARTESIAN_POINT ( 'NONE',  ( -14.37237490289999897, 1409.238075345830111, 207.8572050715280000 ) ) ;
#105924=CARTESIAN_POINT ( 'NONE',  ( -12.51292156319999904, 1441.547097317919906, 187.9392280838980014 ) ) ;
#105925=EDGE_CURVE ( 'NONE', #86024, #27781, #88511, .T. ) ;
#105927=CARTESIAN_POINT ( 'NONE',  ( 12.91340936269999951, 1434.774317664089949, 146.7590612318980163 ) ) ;
#105928=CARTESIAN_POINT ( 'NONE',  ( -34.11564357272870041, 1435.688851149340280, 134.0999999980979851 ) ) ;
#105930=ORIENTED_EDGE ( 'NONE', *, *, #61681, .F. ) ;
#105932=CARTESIAN_POINT ( 'NONE',  ( 40.13864028269999551, 1442.238426966730003, 136.9590191442979972 ) ) ;
#105933=CARTESIAN_POINT ( 'NONE',  ( 18.46438756856120023, 1509.557851009430124, 186.5303332237980101 ) ) ;
#105934=B_SPLINE_CURVE_WITH_KNOTS ( 'NONE', 5,
 ( #97669, #88730, #70860, #89267, #104971, #55146, #106613, #88180, #71417, #20941, #28260, #11472, #45093, #46743, #37220, #105532, #80875, #28821 ),
 .UNSPECIFIED., .F., .F.,
 ( 6, 3, 3, 3, 3, 6 ),
 ( 0.000000000000000000, 0.3094080260441300911, 0.6147993323560541068, 0.7644424561903261361, 0.8931847307547668979, 1.000000000000000000 ),
 .UNSPECIFIED. ) ;
#105937=CARTESIAN_POINT ( 'NONE',  ( -26.99778882349999876, 1469.302995409530013, 268.7552990114980389 ) ) ;
#105940=CARTESIAN_POINT ( 'NONE',  ( -28.51853658599999974, 1509.908949629729932, 214.4930692104080094 ) ) ;
#105941=CARTESIAN_POINT ( 'NONE',  ( -0.8945946638535250406, 1417.298095655010002, 235.8147265033050246 ) ) ;
#105943=CARTESIAN_POINT ( 'NONE',  ( 17.89572889415259738, 1423.787865911519930, 225.8712852353089886 ) ) ;
#105944=CARTESIAN_POINT ( 'NONE',  ( 21.33071589520000089, 1509.431526492729972, 227.7332358683979976 ) ) ;
#105945=CARTESIAN_POINT ( 'NONE',  ( 15.38768853080000198, 1495.932765146430029, 224.1785865777980291 ) ) ;
#105946=DIRECTION ( 'NONE',  ( -0.3282391760791590340, 0.000000000000000000, -0.9445946449598763284 ) ) ;
#105950=CARTESIAN_POINT ( 'NONE',  ( 1.427985284410939970, 1474.785119020410093, 235.3823680754540248 ) ) ;
#105953=CARTESIAN_POINT ( 'NONE',  ( -12.44601730950000018, 1416.547221147930031, 194.7757989389979798 ) ) ;
#105954=CARTESIAN_POINT ( 'NONE',  ( 0.000000000000000000, 1401.254281879943164, 134.0999999980979851 ) ) ;
#105955=CARTESIAN_POINT ( 'NONE',  ( 23.94687154950000263, 1411.110112760130050, 210.2130935636480160 ) ) ;
#105956=CARTESIAN_POINT ( 'NONE',  ( -12.40096745299999981, 1434.347023119479900, 149.5501479441980166 ) ) ;
#105959=CARTESIAN_POINT ( 'NONE',  ( -11.86923217650000062, 1432.580379542929904, 150.3965903535979862 ) ) ;
#105961=DIRECTION ( 'NONE',  ( -0.1541492146682660325, 0.06142059477871750911, -0.9861366691053453648 ) ) ;
#105964=CARTESIAN_POINT ( 'NONE',  ( -22.53878282410000011, 1411.058442784730232, 212.0450770655079964 ) ) ;
#105967=CARTESIAN_POINT ( 'NONE',  ( 13.37406854550570046, 1507.496451373729997, 233.0472692220099873 ) ) ;
#105968=CARTESIAN_POINT ( 'NONE',  ( -15.45533207179999913, 1484.705735421829786, 187.3543539206980029 ) ) ;
#105971=CARTESIAN_POINT ( 'NONE',  ( -4.282792884661109412, 1440.970302453239810, 156.0836163958929887 ) ) ;
#105975=CARTESIAN_POINT ( 'NONE',  ( 28.39970178019999736, 1509.598990362429959, 212.0559822206679996 ) ) ;
#105980=CARTESIAN_POINT ( 'NONE',  ( 0.7484295816749999553, 1428.043997280830126, 101.8807690336980016 ) ) ;
#105981=CARTESIAN_POINT ( 'NONE',  ( 15.73136618761820316, 1409.565780267800164, 192.3644800552150116 ) ) ;
#105982=CARTESIAN_POINT ( 'NONE',  ( 11.89522282729999958, 1434.541161981840105, 151.0452005854980086 ) ) ;
#105983=CARTESIAN_POINT ( 'NONE',  ( -24.83308109816510267, 1451.807016045359887, 136.9460679876989957 ) ) ;
#105984=CARTESIAN_POINT ( 'NONE',  ( 9.998927153253520217, 1439.449791891414179, 152.9676570072420247 ) ) ;
#105985=CARTESIAN_POINT ( 'NONE',  ( 4.324697132450000758, 1409.231835851730011, 230.8572462717979761 ) ) ;
#105988=CARTESIAN_POINT ( 'NONE',  ( 40.66293689370180431, 1439.821779689370032, 134.0999999980979851 ) ) ;
#105992=CARTESIAN_POINT ( 'NONE',  ( -4.363122647529283249, 1407.471318475732005, 137.0999999980979851 ) ) ;
#105995=ORIENTED_EDGE ( 'NONE', *, *, #1741, .T. ) ;
#106001=CARTESIAN_POINT ( 'NONE',  ( -18.42693662763718265, 1445.993580523349237, 214.9599593228655294 ) ) ;
#106004=CARTESIAN_POINT ( 'NONE',  ( 6.250809056239999606, 1416.216596894529857, 191.9478012161979734 ) ) ;
#106005=ORIENTED_EDGE ( 'NONE', *, *, #48382, .T. ) ;
#106008=ORIENTED_EDGE ( 'NONE', *, *, #91905, .F. ) ;
#106009=CARTESIAN_POINT ( 'NONE',  ( 32.33557200478939819, 1440.913060387330006, 256.5466809373250499 ) ) ;
#106010=CARTESIAN_POINT ( 'NONE',  ( -13.92523054340000144, 1509.057792502929715, 183.7758903212979931 ) ) ;
#106011=ORIENTED_EDGE ( 'NONE', *, *, #49453, .F. ) ;
#106012=CARTESIAN_POINT ( 'NONE',  ( -0.2694122152484670352, 1452.981480044009913, 183.2530805241289897 ) ) ;
#106013=CARTESIAN_POINT ( 'NONE',  ( -15.12468517189999950, 1409.607859681430000, 191.4574115868979902 ) ) ;
#106015=CARTESIAN_POINT ( 'NONE',  ( -24.49695175729999974, 1441.051797180180074, 210.9974392583980034 ) ) ;
#106018=CARTESIAN_POINT ( 'NONE',  ( 0.0002641894870882123352, 1396.493308979614994, 196.7136476201564506 ) ) ;
#106019=CARTESIAN_POINT ( 'NONE',  ( 0.1075625203479999986, 1405.989059426929998, 266.9611530679979978 ) ) ;
#106020=CARTESIAN_POINT ( 'NONE',  ( -12.40420594909999963, 1434.420026268609945, 148.5638390392980170 ) ) ;
#106022=CARTESIAN_POINT ( 'NONE',  ( 15.68557540059999766, 1410.853897593529837, 191.5168599455980143 ) ) ;
#106029=CARTESIAN_POINT ( 'NONE',  ( -22.00315959520000320, 1506.810797421130019, 209.3571658142759873 ) ) ;
#106030=CARTESIAN_POINT ( 'NONE',  ( -2.745154014197499937, 1419.769956470485113, 137.0999999980979851 ) ) ;
#106034=CARTESIAN_POINT ( 'NONE',  ( 30.28727320069999962, 1444.847842080569990, 240.1330978332979669 ) ) ;
#106035=CARTESIAN_POINT ( 'NONE',  ( -16.78608357809999774, 1458.775951820630098, 230.6691475833980007 ) ) ;
#106037=CARTESIAN_POINT ( 'NONE',  ( 1.802538876310000093, 1411.735565077730143, 232.2550115084980007 ) ) ;
#106039=CARTESIAN_POINT ( 'NONE',  ( -24.66664643669999890, 1470.078893469029936, 215.2854056718580296 ) ) ;
#106045=CARTESIAN_POINT ( 'NONE',  ( 2.110729450650000061, 1405.810983166630194, 268.4819085761979522 ) ) ;
#106047=CARTESIAN_POINT ( 'NONE',  ( 30.17003485434790022, 1463.451681519390149, 269.4565801611439610 ) ) ;
#106049=CARTESIAN_POINT ( 'NONE',  ( 10.57441464843243750, 1423.877695273033623, 137.4726654012514189 ) ) ;
#106057=CARTESIAN_POINT ( 'NONE',  ( -34.84383443810000358, 1427.856177413630121, 265.6112249940979950 ) ) ;
#106059=CARTESIAN_POINT ( 'NONE',  ( -0.7786989082230000303, 1476.104488692030145, 267.8537809120979887 ) ) ;
#106060=CARTESIAN_POINT ( 'NONE',  ( 10.73171637939167233, 1424.977692942605472, 138.8095723872937413 ) ) ;
#106061=CARTESIAN_POINT ( 'NONE',  ( -28.04637438780000025, 1508.608407033030062, 210.1642266462579869 ) ) ;
#106062=CARTESIAN_POINT ( 'NONE',  ( -3.065717400587616215, 1448.273177092793958, 184.5346825199581815 ) ) ;
#106066=CARTESIAN_POINT ( 'NONE',  ( 26.81253513141949796, 1435.745391332569852, 136.2312305098039928 ) ) ;
#106067=CARTESIAN_POINT ( 'NONE',  ( -8.906481764856058803, 1396.224081584079840, 215.6780524493100017 ) ) ;
#106068=CARTESIAN_POINT ( 'NONE',  ( -15.05245933179999973, 1421.043214595429845, 227.1190893059979885 ) ) ;
#106069=CARTESIAN_POINT ( 'NONE',  ( 19.28951026099334598, 1455.968020544745059, 225.2216972307680010 ) ) ;
#106072=CARTESIAN_POINT ( 'NONE',  ( 2.193535739449999689, 1410.364270874430076, 231.8615948999980105 ) ) ;
#106074=CARTESIAN_POINT ( 'NONE',  ( 10.45694972170000092, 1425.379544169830069, 99.60600324669779582 ) ) ;
#106076=B_SPLINE_CURVE_WITH_KNOTS ( 'NONE', 3,
 ( #37649, #107052, #81287, #105971, #63438, #97556, #79121, #53938, #96458, #30337, #2429, #20830, #55025, #64528, #56105, #90236, #36544, #70742, #28142, #62333, #108147, #14638, #23026, #49358, #75121, #99180, #91358, #48823, #57777, #83487, #30885, #39296, #7344, #58311, #73468, #22460, #5705, #107602, #91895, #66728, #65065, #65620, #32553, #6238, #57228, #56661, #6781, #90795, #15172, #81835, #82947, #40389, #14078, #31437, #48267, #40944, #82412, #39851 ),
 .UNSPECIFIED., .F., .F.,
 ( 4, 3, 3, 3, 3, 3, 3, 3, 3, 3, 3, 3, 3, 3, 3, 3, 3, 3, 3, 4 ),
 ( -71.37784974196719645, -71.16605863430530121, -69.93410874380388975, -68.73248683439000217, -67.54973204371560769, -66.39512066597440310, -65.25685987814000555, -64.13305301190000307, -63.25887383612570147, -62.19532168835289809, -61.12456690189929986, -60.04779693945010166, -58.95843042468590056, -57.85897264479999791, -57.12128301158499966, -55.97157416834189547, -54.78165593109999776, -54.16598274440690375, -52.96632159195399936, -51.70433921739999761 ),
 .UNSPECIFIED. ) ;
#106078=CARTESIAN_POINT ( 'NONE',  ( 4.322220531106200525, 1423.873566462119925, 183.7070391214139988 ) ) ;
#106083=CARTESIAN_POINT ( 'NONE',  ( 1.625726771530000114, 1508.862184707429833, 180.0252976342979991 ) ) ;
#106087=B_SPLINE_CURVE_WITH_KNOTS ( 'NONE', 3,
 ( #86626, #9920, #69305, #53615, #88294, #95585, #103980, #45766, #44091, #87757, #11039 ),
 .UNSPECIFIED., .F., .F.,
 ( 4, 2, 1, 2, 2, 4 ),
 ( 0.000000000000000000, 0.2499999999997748468, 0.3749999999997812861, 0.4374999999997651878, 0.4999999999997490896, 1.000000000000000000 ),
 .UNSPECIFIED. ) ;
#106091=CARTESIAN_POINT ( 'NONE',  ( -14.34064213879999983, 1445.290870928000004, 188.7064315755980033 ) ) ;
#106092=CARTESIAN_POINT ( 'NONE',  ( -14.27906159650000006, 1409.411696205929957, 191.9865084241980071 ) ) ;
#106093=CARTESIAN_POINT ( 'NONE',  ( 19.44117294853580091, 1456.941945407359981, 224.4539793896520052 ) ) ;
#106097=CARTESIAN_POINT ( 'NONE',  ( 4.473648201620000542, 1410.299799965830061, 186.1951180057979798 ) ) ;
#106099=CARTESIAN_POINT ( 'NONE',  ( -39.34713282899999598, 1447.269474492200061, 136.6009879164979850 ) ) ;
#106101=CARTESIAN_POINT ( 'NONE',  ( 41.20351939146799936, 1440.849798643580016, 135.3869769205820148 ) ) ;
#106104=CARTESIAN_POINT ( 'NONE',  ( -2.277971195341919941, 1406.541924822740157, 269.4972091294530401 ) ) ;
#106105=CARTESIAN_POINT ( 'NONE',  ( 40.70885980849999441, 1444.084951190109905, 137.1037942526980089 ) ) ;
#106108=CARTESIAN_POINT ( 'NONE',  ( 12.19742149640000051, 1441.220184892860061, 188.3545874510979843 ) ) ;
#106110=ORIENTED_EDGE ( 'NONE', *, *, #100138, .F. ) ;
#106112=CARTESIAN_POINT ( 'NONE',  ( -14.63759143169999888, 1461.861471536829868, 229.3720751777979956 ) ) ;
#106116=ORIENTED_EDGE ( 'NONE', *, *, #82253, .F. ) ;
#106117=CARTESIAN_POINT ( 'NONE',  ( -5.976455546807909691, 1509.218656960890030, 179.5797749763599995 ) ) ;
#106122=CARTESIAN_POINT ( 'NONE',  ( 2.859824348760000134, 1416.824060884729988, 226.9682156876980059 ) ) ;
#106127=EDGE_CURVE ( 'NONE', #80584, #83258, #69898, .T. ) ;
#106128=CARTESIAN_POINT ( 'NONE',  ( -2.947857299329999847, 1409.016001832629854, 231.5025266905979890 ) ) ;
#106131=CARTESIAN_POINT ( 'NONE',  ( -14.53515913103558610, 1435.864451241055349, 149.7571230983877228 ) ) ;
#106132=CARTESIAN_POINT ( 'NONE',  ( -26.65848496185190086, 1440.913060438550019, 225.2196237981240188 ) ) ;
#106135=CARTESIAN_POINT ( 'NONE',  ( 39.15206306312100537, 1428.692637880929851, 269.5910580954339935 ) ) ;
#106138=CARTESIAN_POINT ( 'NONE',  ( 23.81949531699999767, 1410.711204269130121, 208.1966712349829720 ) ) ;
#106139=CARTESIAN_POINT ( 'NONE',  ( 0.01313586619463304531, 1507.980182440329145, 237.5914718841819990 ) ) ;
#106144=CARTESIAN_POINT ( 'NONE',  ( 4.179007317879920080, 1421.587745001310168, 184.8346002776440002 ) ) ;
#106145=CARTESIAN_POINT ( 'NONE',  ( -0.4639000096230000425, 1415.383732484729990, 233.3963766452980053 ) ) ;
#106146=EDGE_CURVE ( 'NONE', #85181, #27055, #40870, .T. ) ;
#106151=EDGE_CURVE ( 'NONE', #52007, #66425, #53768, .T. ) ;
#106152=CARTESIAN_POINT ( 'NONE',  ( -20.60174636844089946, 1508.366643450050105, 228.3235642671120047 ) ) ;
#106156=CARTESIAN_POINT ( 'NONE',  ( 0.1236923762493960105, 1420.459419726229953, 182.7104392795739898 ) ) ;
#106160=CARTESIAN_POINT ( 'NONE',  ( 19.28053483500000098, 1508.539880148729935, 188.4639099547979981 ) ) ;
#106162=ORIENTED_EDGE ( 'NONE', *, *, #9658, .T. ) ;
#106166=CARTESIAN_POINT ( 'NONE',  ( 11.60004869885205459, 1426.637431749262760, 134.7518136753569706 ) ) ;
#106167=CARTESIAN_POINT ( 'NONE',  ( 10.36367428452916428, 1435.180720288839666, 152.2397717789484375 ) ) ;
#106170=CARTESIAN_POINT ( 'NONE',  ( -27.48965073337759790, 1509.741665821160041, 201.0942380509760028 ) ) ;
#106171=CARTESIAN_POINT ( 'NONE',  ( -3.133278228710000501, 1446.922685362290167, 159.4827083638979843 ) ) ;
#106172=CARTESIAN_POINT ( 'NONE',  ( -18.48615752410000113, 1425.307041905530014, 226.5289461057980134 ) ) ;
#106173=CARTESIAN_POINT ( 'NONE',  ( -15.20520707470000232, 1435.028465714059848, 147.6080287230979877 ) ) ;
#106175=CARTESIAN_POINT ( 'NONE',  ( 17.92485922270000032, 1509.539010264429862, 186.7667139844979829 ) ) ;
#106177=CARTESIAN_POINT ( 'NONE',  ( -17.28825620729984536, 1433.649598815182799, 216.8113180210153246 ) ) ;
#106182=CARTESIAN_POINT ( 'NONE',  ( 3.827327165375219664, 1424.046157828239984, 183.3886487722830054 ) ) ;
#106186=CARTESIAN_POINT ( 'NONE',  ( -2.966648571466143025, 1425.987482934672926, 185.4283574743214444 ) ) ;
#106187=CARTESIAN_POINT ( 'NONE',  ( 15.53391875520000021, 1431.113060387329824, 219.7242127505980136 ) ) ;
#106188=CARTESIAN_POINT ( 'NONE',  ( 26.81573205290009554, 1435.593033338389205, 136.1631037710002943 ) ) ;
#106196=VERTEX_POINT ( 'NONE', #27974 ) ;
#106198=CARTESIAN_POINT ( 'NONE',  ( -0.4770279523499595942, 1415.729984941675639, 233.4079075601304964 ) ) ;
#106199=ORIENTED_EDGE ( 'NONE', *, *, #83387, .T. ) ;
#106200=ORIENTED_EDGE ( 'NONE', *, *, #56503, .T. ) ;
#106201=CARTESIAN_POINT ( 'NONE',  ( 17.36791971707869919, 1414.972329067380088, 210.3611080999600063 ) ) ;
#106203=CARTESIAN_POINT ( 'NONE',  ( 13.51610093808349333, 1443.885067043062236, 169.3501091255430140 ) ) ;
#106204=CARTESIAN_POINT ( 'NONE',  ( 41.03828203346069614, 1434.252829246168858, 269.6293022805288615 ) ) ;
#106205=CARTESIAN_POINT ( 'NONE',  ( -10.82132306919999998, 1467.865346123229983, 250.5360043744979635 ) ) ;
#106207=CARTESIAN_POINT ( 'NONE',  ( -11.88086828319999988, 1433.529714312930082, 150.4967080263980108 ) ) ;
#106208=EDGE_CURVE ( 'NONE', #103319, #59275, #64363, .T. ) ;
#106210=CARTESIAN_POINT ( 'NONE',  ( -19.36887732249999772, 1485.900336442130083, 189.8252615598980242 ) ) ;
#106212=CARTESIAN_POINT ( 'NONE',  ( 13.04207579039999843, 1409.368499709730031, 192.3005086496980027 ) ) ;
#106213=EDGE_CURVE ( 'NONE', #29227, #108746, #28539, .T. ) ;
#106214=CARTESIAN_POINT ( 'NONE',  ( 5.609660757850000401, 1424.149675858230012, 185.9623400711979855 ) ) ;
#106216=CARTESIAN_POINT ( 'NONE',  ( 7.981991770210000503, 1441.362204039569860, 154.1152756057979900 ) ) ;
#106219=CARTESIAN_POINT ( 'NONE',  ( -1.213043055954409927E-09, 1413.218559050369777, 250.1013962713409740 ) ) ;
#106221=ORIENTED_EDGE ( 'NONE', *, *, #20821, .T. ) ;
#106222=CARTESIAN_POINT ( 'NONE',  ( -11.86472222573770097, 1432.239683487029879, 149.9815285707079795 ) ) ;
#106224=CARTESIAN_POINT ( 'NONE',  ( -15.21920960299999948, 1471.332176259930065, 270.4035064524979930 ) ) ;
#106225=DIRECTION ( 'NONE',  ( 0.9846671174924281900, -0.1149361401860498344, -0.1312263365650570279 ) ) ;
#106229=CARTESIAN_POINT ( 'NONE',  ( 0.2546547860042029932, 1451.330736227379930, 182.4946635726779789 ) ) ;
#106230=CARTESIAN_POINT ( 'NONE',  ( -13.12457881600000142, 1420.616264208729945, 228.4003993496980058 ) ) ;
#106232=CARTESIAN_POINT ( 'NONE',  ( -1.243940167669593144, 1484.627497658113271, 182.2780586529670757 ) ) ;
#106234=CARTESIAN_POINT ( 'NONE',  ( -45.58440001455219459, 1437.147777294319894, 268.7645413928499920 ) ) ;
#106236=CARTESIAN_POINT ( 'NONE',  ( -3.540559338901060116, 1498.522212189139964, 181.3435358006369995 ) ) ;
#106238=ORIENTED_EDGE ( 'NONE', *, *, #59039, .F. ) ;
#106239=VERTEX_POINT ( 'NONE', #99567 ) ;
#106242=CARTESIAN_POINT ( 'NONE',  ( -22.52609270580000000, 1509.699688878229836, 190.3721637121980166 ) ) ;
#106243=CARTESIAN_POINT ( 'NONE',  ( -9.065232144620001264, 1410.393916203129947, 188.0587484761979908 ) ) ;
#106245=CARTESIAN_POINT ( 'NONE',  ( 2.500020115319840031, 1419.382923540379807, 144.1035841389490031 ) ) ;
#106251=CARTESIAN_POINT ( 'NONE',  ( 18.47399034927997974, 1509.320896583164085, 187.7622940969008027 ) ) ;
#106253=ORIENTED_EDGE ( 'NONE', *, *, #38968, .T. ) ;
#106254=CARTESIAN_POINT ( 'NONE',  ( -28.62992350010170028, 1415.197349097820052, 269.9536374735400273 ) ) ;
#106255=CARTESIAN_POINT ( 'NONE',  ( 2.882077220935269857, 1416.276656370609999, 231.8998151304730015 ) ) ;
#106256=CARTESIAN_POINT ( 'NONE',  ( -33.91369114349999592, 1451.728768196330066, 134.7155300131979914 ) ) ;
#106259=EDGE_LOOP ( 'NONE', ( #15469, #52292, #103420, #92878 ) ) ;
#106260=CARTESIAN_POINT ( 'NONE',  ( 45.53497092200698404, 1443.217213248229655, 268.9775536060090531 ) ) ;
#106263=CARTESIAN_POINT ( 'NONE',  ( -13.80240444773970054, 1436.220381468010146, 150.3462313445339760 ) ) ;
#106264=CARTESIAN_POINT ( 'NONE',  ( -1.808737601750000090, 1485.212291732630092, 182.6011977753979920 ) ) ;
#106267=CARTESIAN_POINT ( 'NONE',  ( -20.59277739099999849, 1435.768631358810126, 222.2025041439979987 ) ) ;
#106268=CARTESIAN_POINT ( 'NONE',  ( -14.21664609989999839, 1423.493515736829977, 222.0584263151980053 ) ) ;
#106269=CARTESIAN_POINT ( 'NONE',  ( -0.7357022321859555403, 1467.091276340035392, 235.5366063015856923 ) ) ;
#106270=CARTESIAN_POINT ( 'NONE',  ( 5.965627396590000409, 1445.982822326609949, 182.9131883685979858 ) ) ;
#106273=CARTESIAN_POINT ( 'NONE',  ( -33.91369104892859809, 1435.681798505350116, 135.6928025923940027 ) ) ;
#106274=CARTESIAN_POINT ( 'NONE',  ( -20.98707344033122979, 1454.832818946160842, 223.2596928627122281 ) ) ;
#106277=CARTESIAN_POINT ( 'NONE',  ( 24.88920569565430085, 1451.596982390830135, 137.4451123274170072 ) ) ;
#106280=CARTESIAN_POINT ( 'NONE',  ( 19.26695685190000162, 1409.750441825429789, 197.0538186098980020 ) ) ;
#106281=CARTESIAN_POINT ( 'NONE',  ( 21.54410709489999931, 1409.665397185129905, 207.6797030671280027 ) ) ;
#106285=CARTESIAN_POINT ( 'NONE',  ( 0.5266315203254070543, 1450.894659745209992, 181.6127199232379894 ) ) ;
#106286=CARTESIAN_POINT ( 'NONE',  ( 2.500000000000000000, 1439.621710183279902, 168.1588810856449925 ) ) ;
#106292=CARTESIAN_POINT ( 'NONE',  ( -2.696156926760000072, 1448.260832249920213, 184.2611194951979883 ) ) ;
#106293=B_SPLINE_CURVE_WITH_KNOTS ( 'NONE', 5,
 ( #25577, #77663, #9356, #50806, #69282, #92800, #86060, #76550, #975, #43520, #17716, #42964 ),
 .UNSPECIFIED., .F., .F.,
 ( 6, 3, 3, 6 ),
 ( 0.000000000000000000, 0.3787668335507043960, 0.7575336671025384438, 1.000000000000000000 ),
 .UNSPECIFIED. ) ;
#106296=( BOUNDED_CURVE ( )  B_SPLINE_CURVE ( 3, ( #6351, #15279, #68485, #60084 ),
 .UNSPECIFIED., .F., .T. ) 
 B_SPLINE_CURVE_WITH_KNOTS ( ( 4, 4 ),
 ( 2.498705433189824632, 2.510790977241040167 ),
 .UNSPECIFIED. ) 
 CURVE ( )  GEOMETRIC_REPRESENTATION_ITEM ( )  RATIONAL_B_SPLINE_CURVE ( ( 1.000000000000000000, 0.9999878283391195888, 0.9999878283391195888, 1.000000000000000000 ) ) 
 REPRESENTATION_ITEM ( '' )  );
#106297=CARTESIAN_POINT ( 'NONE',  ( -39.20581607928339452, 1447.436852605690092, 136.5770680602419986 ) ) ;
#106300=CARTESIAN_POINT ( 'NONE',  ( 17.83740504339754551, 1423.668137810906956, 225.9714325268276696 ) ) ;
#106301=CARTESIAN_POINT ( 'NONE',  ( 11.21649392120000144, 1433.156491609380282, 151.5728939339980172 ) ) ;
#106302=CARTESIAN_POINT ( 'NONE',  ( -43.35454757139999771, 1452.005318730930185, 269.0376331129979803 ) ) ;
#106303=CARTESIAN_POINT ( 'NONE',  ( 31.53547013313849590, 1440.913060383619950, 242.8798340245609779 ) ) ;
#106308=CARTESIAN_POINT ( 'NONE',  ( 12.37499353609999986, 1445.063428794549964, 206.9242620747189960 ) ) ;
#106309=CARTESIAN_POINT ( 'NONE',  ( -19.40696031517546771, 1485.597849508721538, 189.9130132395831367 ) ) ;
#106315=CARTESIAN_POINT ( 'NONE',  ( -16.10723672499999992, 1509.418792458129928, 232.5337701105979988 ) ) ;
#106318=CARTESIAN_POINT ( 'NONE',  ( 9.515252399970000496, 1407.295241224529946, 218.7370609393180132 ) ) ;
#106321=CARTESIAN_POINT ( 'NONE',  ( 1.484869686569999958, 1466.691734608930119, 234.9721188785979962 ) ) ;
#106324=CARTESIAN_POINT ( 'NONE',  ( -1.453301145269999983, 1450.656428793419991, 182.0378587995979842 ) ) ;
#106331=ORIENTED_EDGE ( 'NONE', *, *, #36043, .T. ) ;
#106337=CARTESIAN_POINT ( 'NONE',  ( 20.29125555118498525, 1509.661241771571213, 187.4025316824865968 ) ) ;
#106338=CARTESIAN_POINT ( 'NONE',  ( 14.88243897759089940, 1409.432766608349993, 207.8795444941929986 ) ) ;
#106339=DIRECTION ( 'NONE',  ( -2.275957200481568541E-15, -0.7071067811865475727, -0.7071067811865475727 ) ) ;
#106341=CARTESIAN_POINT ( 'NONE',  ( -19.68344085950000277, 1478.176749358629877, 191.0788175296980000 ) ) ;
#106344=VERTEX_POINT ( 'NONE', #77159 ) ;
#106346=VECTOR ( 'NONE', #76493, 1000.000000000000114 ) ;
#106347=CARTESIAN_POINT ( 'NONE',  ( -12.23023785423269949, 1416.449138231070037, 194.7027724284880037 ) ) ;
#106351=CARTESIAN_POINT ( 'NONE',  ( -5.185116111308140457E-10, 1466.995839566859786, 244.9882531609609941 ) ) ;
#106352=CARTESIAN_POINT ( 'NONE',  ( -20.12529541769230335, 1492.488775349680054, 190.8351265624610278 ) ) ;
#106353=CARTESIAN_POINT ( 'NONE',  ( 4.606757942329999800, 1396.134574633329976, 219.8862302532979811 ) ) ;
#106354=CARTESIAN_POINT ( 'NONE',  ( 21.33942550552290029, 1477.920013592180112, 209.7103284805230032 ) ) ;
#106355=CARTESIAN_POINT ( 'NONE',  ( -1.183503983870000109, 1453.587766892330137, 183.5423389305979924 ) ) ;
#106357=CARTESIAN_POINT ( 'NONE',  ( -26.30168575793273433, 1436.707617520661415, 136.8511971899106925 ) ) ;
#106361=CARTESIAN_POINT ( 'NONE',  ( 11.58602478873720010, 1433.820729704430050, 151.2070532014469961 ) ) ;
#106362=CARTESIAN_POINT ( 'NONE',  ( -13.84400707361050209, 1436.103923087979865, 150.2928912686649880 ) ) ;
#106369=CARTESIAN_POINT ( 'NONE',  ( 34.21460435970000447, 1436.526926586619993, 250.0133502344980059 ) ) ;
#106370=CARTESIAN_POINT ( 'NONE',  ( -27.02980867449999991, 1488.688182089229940, 206.7943278652880110 ) ) ;
#106371=CARTESIAN_POINT ( 'NONE',  ( 1.453785988909999771, 1502.021732069830023, 181.3354227047979919 ) ) ;
#106372=CARTESIAN_POINT ( 'NONE',  ( -1.135155600555850075, 1507.593744725489842, 232.0500749651639865 ) ) ;
#106373=CARTESIAN_POINT ( 'NONE',  ( 21.03310440807343440, 1506.473666149375049, 202.6084271311502505 ) ) ;
#106374=CARTESIAN_POINT ( 'NONE',  ( -28.01490336850000062, 1440.913060392510033, 231.6874816156980046 ) ) ;
#106378=CARTESIAN_POINT ( 'NONE',  ( 33.54166316889999422, 1451.286620755330205, 135.9569810539979926 ) ) ;
#106380=DIRECTION ( 'NONE',  ( -0.6450708608674635691, -0.04363816414198488230, 0.7628756747269024308 ) ) ;
#106383=CARTESIAN_POINT ( 'NONE',  ( 11.74018743070000070, 1509.402761548730041, 236.7672879654979852 ) ) ;
#106384=ORIENTED_EDGE ( 'NONE', *, *, #42673, .F. ) ;
#106388=CARTESIAN_POINT ( 'NONE',  ( -23.72940098905899831, 1410.154294345949893, 208.7747630995070267 ) ) ;
#106392=FACE_OUTER_BOUND ( 'NONE', #21103, .T. ) ;
#106393=CIRCLE ( 'NONE', #27676, 4.004156303888216861 ) ;
#106395=CARTESIAN_POINT ( 'NONE',  ( -2.386325087049999905, 1470.484332729530024, 235.3385911319980153 ) ) ;
#106398=CARTESIAN_POINT ( 'NONE',  ( 11.73700276120000119, 1426.696009609329849, 144.1682878317980112 ) ) ;
#106399=CARTESIAN_POINT ( 'NONE',  ( -12.86384817108250189, 1415.089948427370018, 220.8168020335180017 ) ) ;
#106400=CARTESIAN_POINT ( 'NONE',  ( 0.3823997583379999954, 1418.629108576230010, 184.6943103907979946 ) ) ;
#106403=ORIENTED_EDGE ( 'NONE', *, *, #70186, .T. ) ;
#106406=ORIENTED_EDGE ( 'NONE', *, *, #65112, .T. ) ;
#106410=CARTESIAN_POINT ( 'NONE',  ( -22.70509189929999749, 1409.705932116229860, 208.9454376012710100 ) ) ;
#106414=ADVANCED_FACE ( 'NONE', ( #98351 ), #15864, .F. ) ;
#106416=CARTESIAN_POINT ( 'NONE',  ( 11.14671379024469999, 1434.019377051509991, 151.6529839732360188 ) ) ;
#106419=CARTESIAN_POINT ( 'NONE',  ( 16.45537802140000139, 1489.466917449630046, 194.2445904713979985 ) ) ;
#106421=CARTESIAN_POINT ( 'NONE',  ( -24.15206955952350043, 1508.556946117430016, 222.3774010852600043 ) ) ;
#106425=CARTESIAN_POINT ( 'NONE',  ( 21.34957048960000137, 1432.854863361970047, 234.3916895697979612 ) ) ;
#106428=AXIS2_PLACEMENT_3D ( 'NONE', #74592, #7369, #82975 ) ;
#106430=ADVANCED_FACE ( 'NONE', ( #54465 ), #77640, .F. ) ;
#106433=ORIENTED_EDGE ( 'NONE', *, *, #24836, .T. ) ;
#106434=CARTESIAN_POINT ( 'NONE',  ( 16.81223226430000039, 1414.913060387329779, 210.6693098017280192 ) ) ;
#106441=CARTESIAN_POINT ( 'NONE',  ( 6.468780810475760035, 1509.138952694780073, 179.6697712966799827 ) ) ;
#106442=CARTESIAN_POINT ( 'NONE',  ( -41.66193840216117650, 1443.744945820009661, 136.1277624208983639 ) ) ;
#106444=CARTESIAN_POINT ( 'NONE',  ( 15.81240911520000125, 1417.427885388930008, 227.3441162537980347 ) ) ;
#106447=CARTESIAN_POINT ( 'NONE',  ( 41.16455037149999896, 1425.337515733230020, 266.3184770345980041 ) ) ;
#106448=CARTESIAN_POINT ( 'NONE',  ( -18.55304899770000304, 1410.484400192730163, 223.7713282511979855 ) ) ;
#106449=CARTESIAN_POINT ( 'NONE',  ( 22.35103205260000081, 1436.090882114679971, 142.4834648293980024 ) ) ;
#106450=CARTESIAN_POINT ( 'NONE',  ( -0.9044168070210000243, 1418.675475465229965, 228.1103104084980373 ) ) ;
#106451=CARTESIAN_POINT ( 'NONE',  ( 5.379930311655070518, 1430.658779919180006, 154.4493466840170015 ) ) ;
#106452=CARTESIAN_POINT ( 'NONE',  ( -37.54398636633066388, 1461.570449753633966, 266.4251595816978124 ) ) ;
#106454=CARTESIAN_POINT ( 'NONE',  ( -38.86240415199999632, 1439.430083176099970, 136.6726061590980237 ) ) ;
#106455=CARTESIAN_POINT ( 'NONE',  ( 0.2086211941929050073, 1458.123855251709983, 183.0335782383330070 ) ) ;
#106456=CARTESIAN_POINT ( 'NONE',  ( -9.967857204701429552, 1407.622385665449883, 200.5556886166019979 ) ) ;
#106457=CARTESIAN_POINT ( 'NONE',  ( -11.73070209449999979, 1414.913060387329779, 197.7037767505979957 ) ) ;
#106459=CARTESIAN_POINT ( 'NONE',  ( -28.04361090164860215, 1509.087630844720024, 210.7243009158079872 ) ) ;
#106460=CARTESIAN_POINT ( 'NONE',  ( 12.91288853569999873, 1434.774381388219808, 149.4778850478979848 ) ) ;
#106461=CARTESIAN_POINT ( 'NONE',  ( -38.01446494613939819, 1436.977963748669936, 134.0999999969440069 ) ) ;
#106462=CARTESIAN_POINT ( 'NONE',  ( 3.851527341300000185, 1440.290862272119966, 184.6363558007980146 ) ) ;
#106465=CARTESIAN_POINT ( 'NONE',  ( 40.31826125219999568, 1443.160130861930156, 137.0614306859980047 ) ) ;
#106469=CARTESIAN_POINT ( 'NONE',  ( -31.53040958840000485, 1466.256159665430005, 268.9167898976980382 ) ) ;
#106472=CARTESIAN_POINT ( 'NONE',  ( -26.15182807060000059, 1509.826302347529918, 220.8502595356980009 ) ) ;
#106476=CARTESIAN_POINT ( 'NONE',  ( 20.86040077210000021, 1508.959081887729781, 227.6602567232980050 ) ) ;
#106477=CARTESIAN_POINT ( 'NONE',  ( -29.40921901757340251, 1509.877385649660027, 208.6169211888969812 ) ) ;
#106479=CARTESIAN_POINT ( 'NONE',  ( 0.5065993652445669460, 1412.370428418450047, 184.9838650198409766 ) ) ;
#106481=CARTESIAN_POINT ( 'NONE',  ( -13.77715290559999950, 1508.637939534930183, 184.0711877140979880 ) ) ;
#106483=CIRCLE ( 'NONE', #74294, 23.99999935407219454 ) ;
#106486=CARTESIAN_POINT ( 'NONE',  ( -12.62835224979999893, 1416.067629290630066, 195.5863397732979934 ) ) ;
#106488=CARTESIAN_POINT ( 'NONE',  ( 23.24624089760000345, 1410.220001169729812, 212.0510662298279954 ) ) ;
#106493=CARTESIAN_POINT ( 'NONE',  ( -11.57799723109999945, 1432.441865831549876, 151.1964732625980048 ) ) ;
#106498=CARTESIAN_POINT ( 'NONE',  ( -23.87304943890000075, 1435.754597106050142, 211.2923954554679824 ) ) ;
#106501=CARTESIAN_POINT ( 'NONE',  ( -17.37601589566219928, 1485.496354615790096, 188.4150023406379830 ) ) ;
#106505=ORIENTED_EDGE ( 'NONE', *, *, #46749, .T. ) ;
#106507=CARTESIAN_POINT ( 'NONE',  ( 28.21332323700000089, 1508.643929370829937, 209.7679031484589984 ) ) ;
#106512=CARTESIAN_POINT ( 'NONE',  ( 15.84085386514549931, 1416.203647188709738, 191.3516974002209849 ) ) ;
#106513=CARTESIAN_POINT ( 'NONE',  ( 24.39988810369999683, 1444.709222782450070, 214.8827041012880272 ) ) ;
#106515=CARTESIAN_POINT ( 'NONE',  ( -24.00451132643230068, 1452.074800784660056, 136.6367033768989927 ) ) ;
#106516=DIRECTION ( 'NONE',  ( 0.000000000000000000, 0.5877852522921415135, -0.8090169943751884807 ) ) ;
#106517=CARTESIAN_POINT ( 'NONE',  ( 14.70688542969999979, 1409.928487481030061, 227.4346275906979997 ) ) ;
#106521=CARTESIAN_POINT ( 'NONE',  ( 40.14707100556169905, 1448.397814785060064, 134.0999999982449822 ) ) ;
#106525=CARTESIAN_POINT ( 'NONE',  ( 14.52275784015550109, 1435.809058665319981, 149.7340231952910017 ) ) ;
#106530=CARTESIAN_POINT ( 'NONE',  ( 12.08338312575843787, 1410.708559485759224, 228.9665408485644491 ) ) ;
#106532=CARTESIAN_POINT ( 'NONE',  ( 16.51877150081237389, 1451.100436498563113, 148.6701188902696344 ) ) ;
#106533=CARTESIAN_POINT ( 'NONE',  ( -22.86388141493510062, 1452.114636054849825, 134.0999999999999943 ) ) ;
#106534=CARTESIAN_POINT ( 'NONE',  ( -18.58116375392060249, 1445.454363348780362, 214.2320557096282130 ) ) ;
#106537=EDGE_CURVE ( 'NONE', #76557, #92712, #60513, .T. ) ;
#106539=CARTESIAN_POINT ( 'NONE',  ( 3.560382106670000102, 1415.087974639930053, 191.9480497089980133 ) ) ;
#106543=ORIENTED_EDGE ( 'NONE', *, *, #32311, .F. ) ;
#106544=CARTESIAN_POINT ( 'NONE',  ( 30.67453579933340180, 1440.913060387330006, 253.4609548031900204 ) ) ;
#106547=ORIENTED_EDGE ( 'NONE', *, *, #26077, .T. ) ;
#106548=CARTESIAN_POINT ( 'NONE',  ( -0.5697989934050000649, 1450.893162568020216, 181.2886233453980083 ) ) ;
#106549=CARTESIAN_POINT ( 'NONE',  ( -15.82667276960000180, 1410.838063423429958, 191.2287379893979846 ) ) ;
#106551=CARTESIAN_POINT ( 'NONE',  ( -24.41186848580399982, 1440.913060429360030, 212.0284777848129920 ) ) ;
#106553=CARTESIAN_POINT ( 'NONE',  ( 13.90221994160000030, 1436.238121858259774, 150.2928703997980051 ) ) ;
#106554=CARTESIAN_POINT ( 'NONE',  ( 43.71400182546053514, 1430.030204529002958, 266.2448334775871785 ) ) ;
#106558=CARTESIAN_POINT ( 'NONE',  ( 8.038768963489999919, 1463.606875709430142, 235.5281748529980064 ) ) ;
#106559=CARTESIAN_POINT ( 'NONE',  ( -10.23378643512955577, 1422.709436974594610, 137.1241386678474043 ) ) ;
#106563=CARTESIAN_POINT ( 'NONE',  ( -0.1550544472294869969, 1507.335707632679942, 180.8803381700240038 ) ) ;
#106572=CARTESIAN_POINT ( 'NONE',  ( 25.18985267090000235, 1442.566560664089820, 217.4969598497380048 ) ) ;
#106573=CARTESIAN_POINT ( 'NONE',  ( -11.86665551350000136, 1432.374829077889899, 149.9823017929979869 ) ) ;
#106575=CARTESIAN_POINT ( 'NONE',  ( 2.670551802009999864, 1411.760187836130171, 231.7294704944980026 ) ) ;
#106578=CARTESIAN_POINT ( 'NONE',  ( -22.57989227939999921, 1470.081218446630146, 221.4829011586980130 ) ) ;
#106579=CARTESIAN_POINT ( 'NONE',  ( 2.500000000000000000, 1425.201036443130079, 155.3321294796979828 ) ) ;
#106580=CARTESIAN_POINT ( 'NONE',  ( -2.546419266200000475, 1485.854131597229980, 182.3738517892980155 ) ) ;
#106583=CARTESIAN_POINT ( 'NONE',  ( 2.763724491000000061, 1406.126245782430033, 269.0427161091980111 ) ) ;
#106586=CARTESIAN_POINT ( 'NONE',  ( 41.41036356811409291, 1451.093780838620205, 270.1893080176820376 ) ) ;
#106587=CARTESIAN_POINT ( 'NONE',  ( -25.18563703530000097, 1452.033577648029905, 135.3787234722980202 ) ) ;
#106588=CARTESIAN_POINT ( 'NONE',  ( 11.60004869884103407, 1423.521825948030937, 137.0424065539601770 ) ) ;
#106591=CARTESIAN_POINT ( 'NONE',  ( -1.672144570133835995, 1451.729478148845374, 184.0944664686900296 ) ) ;
#106592=CARTESIAN_POINT ( 'NONE',  ( -1.676215897828090107, 1450.511945644329899, 182.4451613505460159 ) ) ;
#106593=CARTESIAN_POINT ( 'NONE',  ( -13.64809019991630024, 1415.124054205850143, 220.5687789520499962 ) ) ;
#106595=ORIENTED_EDGE ( 'NONE', *, *, #77840, .F. ) ;
#106596=CARTESIAN_POINT ( 'NONE',  ( 2.886579864029999753E-15, 1413.763055110029882, 262.6648722463980334 ) ) ;
#106597=CARTESIAN_POINT ( 'NONE',  ( 2.500000000000000000, 1439.625347662450167, 166.9460400662979964 ) ) ;
#106598=CARTESIAN_POINT ( 'NONE',  ( -0.5593523789189999151, 1476.106998426729888, 267.8539144646980503 ) ) ;
#106599=CARTESIAN_POINT ( 'NONE',  ( -32.67729582440000513, 1451.771913520829912, 134.7516611205979871 ) ) ;
#106605=CARTESIAN_POINT ( 'NONE',  ( 0.2538829723067779764, 1420.503732877419907, 182.7635795570130028 ) ) ;
#106606=( BOUNDED_CURVE ( )  B_SPLINE_CURVE ( 3, ( #97336, #3314, #39644, #3865 ),
 .UNSPECIFIED., .F., .F. ) 
 B_SPLINE_CURVE_WITH_KNOTS ( ( 4, 4 ),
 ( 4.409610437282244888, 5.070003789806990291 ),
 .UNSPECIFIED. ) 
 CURVE ( )  GEOMETRIC_REPRESENTATION_ITEM ( )  RATIONAL_B_SPLINE_CURVE ( ( 1.000000000000000000, 0.9639857291066213918, 0.9639857291066213918, 1.000000000000000000 ) ) 
 REPRESENTATION_ITEM ( '' )  );
#106607=CARTESIAN_POINT ( 'NONE',  ( -5.750244769764350394, 1396.113863361650147, 218.5416372912760039 ) ) ;
#106609=CARTESIAN_POINT ( 'NONE',  ( -45.60176523299999474, 1439.545916309389895, 268.9757053294979983 ) ) ;
#106610=VERTEX_POINT ( 'NONE', #17349 ) ;
#106613=CARTESIAN_POINT ( 'NONE',  ( -11.28228388660000014, 1484.392611670030192, 185.3973464570979957 ) ) ;
#106614=CARTESIAN_POINT ( 'NONE',  ( 11.62090964459999931, 1426.357348742330032, 135.9230500439979892 ) ) ;
#106621=CARTESIAN_POINT ( 'NONE',  ( 1.448678579899999930, 1507.129710292329946, 181.1126013549980200 ) ) ;
#106626=ORIENTED_EDGE ( 'NONE', *, *, #98035, .T. ) ;
#106628=CARTESIAN_POINT ( 'NONE',  ( -8.555999076900000944, 1397.549004006330051, 199.0552853815979972 ) ) ;
#106629=CARTESIAN_POINT ( 'NONE',  ( 2.887715917392400300, 1409.376950096379915, 231.1465570425760063 ) ) ;
#106631=CARTESIAN_POINT ( 'NONE',  ( -6.931887347990000059, 1409.155127227530102, 188.8914258914980167 ) ) ;
#106632=CARTESIAN_POINT ( 'NONE',  ( 1.910126501409999789E-10, 1431.113060387329824, 227.8291532366980050 ) ) ;
#106636=CARTESIAN_POINT ( 'NONE',  ( 0.6856161522000000508, 1410.310357111729900, 185.1124255419979932 ) ) ;
#106637=CARTESIAN_POINT ( 'NONE',  ( -37.26789664401470503, 1450.479926032020103, 135.9651663335700107 ) ) ;
#106638=CARTESIAN_POINT ( 'NONE',  ( 41.66194080536450173, 1443.744915603149821, 136.1277488527510116 ) ) ;
#106639=CARTESIAN_POINT ( 'NONE',  ( 33.27870177008182395, 1435.659577329578951, 135.0862789282056724 ) ) ;
#106640=CARTESIAN_POINT ( 'NONE',  ( -27.93599228559999759, 1442.648988978950001, 137.4365311676980355 ) ) ;
#106641=CARTESIAN_POINT ( 'NONE',  ( 10.94295718250000071, 1430.426329750230252, 151.5194551083980059 ) ) ;
#106644=CARTESIAN_POINT ( 'NONE',  ( 4.229500449809999729, 1423.902524512430091, 183.5234483264979986 ) ) ;
#106650=CARTESIAN_POINT ( 'NONE',  ( 15.60314760730000039, 1425.942174865029983, 212.9755122303479880 ) ) ;
#106657=CARTESIAN_POINT ( 'NONE',  ( -5.957503935620779956, 1509.188430844039885, 179.6796226404359800 ) ) ;
#106659=EDGE_CURVE ( 'NONE', #65282, #101005, #87619, .T. ) ;
#106660=CARTESIAN_POINT ( 'NONE',  ( 18.12194535329999923, 1416.217772597929979, 213.0453993036479972 ) ) ;
#106663=CARTESIAN_POINT ( 'NONE',  ( -19.70969297780000318, 1440.913060387330006, 214.9271664100980104 ) ) ;
#106664=EDGE_CURVE ( 'NONE', #18275, #70222, #19066, .T. ) ;
#106665=CARTESIAN_POINT ( 'NONE',  ( -29.83114707306344826, 1419.453282592096002, 269.4690146648258064 ) ) ;
#106666=CIRCLE ( 'NONE', #38239, 93.02998377600577840 ) ;
#106667=CARTESIAN_POINT ( 'NONE',  ( -4.781335570289999559, 1409.080028304630105, 230.4240303851980229 ) ) ;
#106668=CARTESIAN_POINT ( 'NONE',  ( -3.487133837120000024, 1431.113060387329824, 190.6407012183980214 ) ) ;
#106670=CARTESIAN_POINT ( 'NONE',  ( 2.500000000000000000, 1419.382872273060002, 144.1054344980790063 ) ) ;
#106671=CARTESIAN_POINT ( 'NONE',  ( -26.99520746976219954, 1440.913060419549993, 226.8119193977670136 ) ) ;
#106674=CARTESIAN_POINT ( 'NONE',  ( 42.06226826553579912, 1436.795776192510175, 269.6487248881980463 ) ) ;
#106677=CARTESIAN_POINT ( 'NONE',  ( 22.82834858460000049, 1409.718736107430232, 208.8015344678899794 ) ) ;
#106678=CARTESIAN_POINT ( 'NONE',  ( 0.01851582568700120210, 1507.478319835492812, 237.4021211056988818 ) ) ;
#106683=CARTESIAN_POINT ( 'NONE',  ( -2.801976539950000067, 1420.449080726529928, 233.0291344731980132 ) ) ;
#106688=CARTESIAN_POINT ( 'NONE',  ( -0.004541069570850000091, 1417.346727570329904, 235.5710176400980060 ) ) ;
#106703=B_SPLINE_CURVE_WITH_KNOTS ( 'NONE', 3,
 ( #29203, #89102, #80710, #4556 ),
 .UNSPECIFIED., .F., .F.,
 ( 4, 4 ),
 ( 7.189088551655727393E-14, 0.002384643111680536873 ),
 .UNSPECIFIED. ) ;
#106707=CARTESIAN_POINT ( 'NONE',  ( -27.68503987499639862, 1509.816463871160067, 201.0194270758620121 ) ) ;
#106708=CARTESIAN_POINT ( 'NONE',  ( -2.499999999959999997, 1447.637843966430182, 170.5315787469979796 ) ) ;
#106709=CARTESIAN_POINT ( 'NONE',  ( -20.34455516050000057, 1426.954645372529967, 221.8177795676979827 ) ) ;
#106712=CARTESIAN_POINT ( 'NONE',  ( 15.94624203079999702, 1509.299608116730042, 185.9453027169979862 ) ) ;
#106713=CARTESIAN_POINT ( 'NONE',  ( -0.03277866176829110495, 1410.296501491089884, 233.2237263845800044 ) ) ;
#106714=CARTESIAN_POINT ( 'NONE',  ( -17.30083075200003151, 1433.673648912240196, 216.7777474620279463 ) ) ;
#106716=ORIENTED_EDGE ( 'NONE', *, *, #28880, .T. ) ;
#106722=CARTESIAN_POINT ( 'NONE',  ( -18.64460733019999950, 1509.564144422130084, 231.7099517930980142 ) ) ;
#106725=CARTESIAN_POINT ( 'NONE',  ( -12.92150563921792461, 1442.903198327644077, 186.4433106084745759 ) ) ;
#106726=CARTESIAN_POINT ( 'NONE',  ( -24.68077630836099701, 1437.736159206269804, 210.5119845322900005 ) ) ;
#106730=EDGE_CURVE ( 'NONE', #89451, #7508, #79205, .T. ) ;
#106731=CARTESIAN_POINT ( 'NONE',  ( 24.86520790779999857, 1436.144674809589787, 137.8610291600980133 ) ) ;
#106736=EDGE_CURVE ( 'NONE', #31004, #54528, #8361, .T. ) ;
#106738=ORIENTED_EDGE ( 'NONE', *, *, #62580, .F. ) ;
#106742=CARTESIAN_POINT ( 'NONE',  ( 13.28728145560000051, 1508.680272370929970, 233.3924286979980138 ) ) ;
#106744=CARTESIAN_POINT ( 'NONE',  ( 29.95045141167489433, 1419.540663059560529, 269.4702688073739409 ) ) ;
#106745=CARTESIAN_POINT ( 'NONE',  ( -27.90885395439999783, 1457.406260642230109, 250.2249407924980176 ) ) ;
#106746=CARTESIAN_POINT ( 'NONE',  ( -20.32989725279999860, 1499.115995715829968, 190.6432919934979964 ) ) ;
#106747=CARTESIAN_POINT ( 'NONE',  ( -11.14671480820000049, 1434.019355918939937, 151.6529837240979930 ) ) ;
#106749=CARTESIAN_POINT ( 'NONE',  ( -19.06723480449999997, 1485.490520234629912, 189.6150008477979725 ) ) ;
#106754=DIRECTION ( 'NONE',  ( 1.000000000000000000, 0.000000000000000000, 0.000000000000000000 ) ) ;
#106758=CARTESIAN_POINT ( 'NONE',  ( 1.452038864671010018E-08, 1407.324376059620135, 264.3779639133369983 ) ) ;
#106759=ORIENTED_EDGE ( 'NONE', *, *, #24815, .T. ) ;
#106760=EDGE_LOOP ( 'NONE', ( #62648, #89189, #30340 ) ) ;
#106761=CARTESIAN_POINT ( 'NONE',  ( -11.86387080393020099, 1432.180192430769921, 149.9801236230049710 ) ) ;
#106763=CARTESIAN_POINT ( 'NONE',  ( -34.52598909179999964, 1461.996329814830005, 270.2126011320979728 ) ) ;
#106764=CARTESIAN_POINT ( 'NONE',  ( -23.92569337129095786, 1435.916919288760027, 211.2787512685800095 ) ) ;
#106765=CARTESIAN_POINT ( 'NONE',  ( 6.446325585610000353, 1432.345375419369930, 154.6647257196979979 ) ) ;
#106766=CARTESIAN_POINT ( 'NONE',  ( 33.91361689144800096, 1451.728768045109973, 134.7154145114139965 ) ) ;
#106767=CARTESIAN_POINT ( 'NONE',  ( 0.2064069609369219849, 1452.175221133040168, 183.1192452647970015 ) ) ;
#106768=CARTESIAN_POINT ( 'NONE',  ( -12.41153351569999863, 1420.834873760830078, 229.8963213914979917 ) ) ;
#106769=CARTESIAN_POINT ( 'NONE',  ( -16.17568633703940151, 1459.146939663510011, 230.7169128052520080 ) ) ;
#106772=CARTESIAN_POINT ( 'NONE',  ( -27.31148204492600229, 1412.934667530339993, 269.0113653186659803 ) ) ;
#106774=CARTESIAN_POINT ( 'NONE',  ( -3.537598770401839676, 1495.725909260799881, 181.4625765259970080 ) ) ;
#106775=EDGE_LOOP ( 'NONE', ( #20705, #95355, #54174, #93574 ) ) ;
#106776=AXIS2_PLACEMENT_3D ( 'NONE', #55783, #56312, #13170 ) ;
#106777=EDGE_LOOP ( 'NONE', ( #109634, #59628, #56725, #53975 ) ) ;
#106779=FACE_OUTER_BOUND ( 'NONE', #59482, .T. ) ;
#106781=CARTESIAN_POINT ( 'NONE',  ( -20.61553203140000434, 1508.364800381330042, 190.3717489592980030 ) ) ;
#106782=CARTESIAN_POINT ( 'NONE',  ( -11.77258770480000116, 1440.429812290090013, 187.7126807368979939 ) ) ;
#106783=AXIS2_PLACEMENT_3D ( 'NONE', #17893, #28532, #77832 ) ;
#106784=CARTESIAN_POINT ( 'NONE',  ( -15.97031451047940109, 1470.475814234120207, 228.8250343533829891 ) ) ;
#106785=ORIENTED_EDGE ( 'NONE', *, *, #57733, .T. ) ;
#106786=CARTESIAN_POINT ( 'NONE',  ( -26.80688184059999912, 1436.287257724250139, 136.6586291973980281 ) ) ;
#106791=CARTESIAN_POINT ( 'NONE',  ( -19.13958158392089715, 1411.674646606650185, 270.3886806677189725 ) ) ;
#106792=CARTESIAN_POINT ( 'NONE',  ( -1.470421131539999982, 1428.420680932830237, 91.31218443469779800 ) ) ;
#106796=ORIENTED_EDGE ( 'NONE', *, *, #38349, .T. ) ;
#106797=CARTESIAN_POINT ( 'NONE',  ( 36.90008876993807263, 1461.061631172933403, 269.2062195636714250 ) ) ;
#106801=CIRCLE ( 'NONE', #37127, 1.530931026689996699 ) ;
#106803=CARTESIAN_POINT ( 'NONE',  ( -18.67445339878970145, 1416.007771869960152, 207.5718808771989927 ) ) ;
#106804=CARTESIAN_POINT ( 'NONE',  ( -18.94569428040000147, 1430.795004337129967, 224.8243481170979976 ) ) ;
#106805=CARTESIAN_POINT ( 'NONE',  ( -14.76826616709999840, 1426.820312322130121, 221.7083327112979987 ) ) ;
#106806=CARTESIAN_POINT ( 'NONE',  ( 12.39598156289999942, 1416.274718424630009, 223.4274628688980044 ) ) ;
#106809=ORIENTED_EDGE ( 'NONE', *, *, #11168, .T. ) ;
#106814=CARTESIAN_POINT ( 'NONE',  ( -18.89959486414000267, 1416.839692127460012, 207.5749783441650038 ) ) ;
#106815=CARTESIAN_POINT ( 'NONE',  ( 13.79060599709999835, 1416.547221146729953, 196.3475826081979960 ) ) ;
#106817=CARTESIAN_POINT ( 'NONE',  ( 19.28368759869999849, 1410.509001784329939, 195.8671163398980184 ) ) ;
#106818=CARTESIAN_POINT ( 'NONE',  ( 16.68463233076019492, 1445.052233488289176, 162.0935120523188289 ) ) ;
#106819=CARTESIAN_POINT ( 'NONE',  ( 10.10004869885234058, 1422.222932908421171, 137.0999999980978430 ) ) ;
#106822=CARTESIAN_POINT ( 'NONE',  ( 4.241818682233510884, 1441.427818084279806, 162.5168752623719968 ) ) ;
#106825=CARTESIAN_POINT ( 'NONE',  ( 2.500000000000300204, 1439.152015563370014, 158.1892132547360177 ) ) ;
#106830=CARTESIAN_POINT ( 'NONE',  ( -2.696187843830000208, 1448.602801166340214, 184.2458148013979837 ) ) ;
#106831=CARTESIAN_POINT ( 'NONE',  ( -11.43480974721719967, 1425.837050099640010, 122.9429429844429933 ) ) ;
#106832=CARTESIAN_POINT ( 'NONE',  ( -38.37365570824950112, 1448.472291891780060, 136.4276078884599883 ) ) ;
#106833=CARTESIAN_POINT ( 'NONE',  ( 11.60004869885203682, 1426.233066092331683, 138.1607928833331584 ) ) ;
#106834=CARTESIAN_POINT ( 'NONE',  ( 2.514509550398654536, 1417.714408133527741, 233.7630435220257823 ) ) ;
#106835=CARTESIAN_POINT ( 'NONE',  ( -2.500000000000000000, 1419.649642134729902, 147.2763244958979953 ) ) ;
#106837=CARTESIAN_POINT ( 'NONE',  ( -39.27028727949999620, 1458.780602943529857, 269.1469756859979725 ) ) ;
#106838=CARTESIAN_POINT ( 'NONE',  ( 30.82334546788949936, 1440.913060384559913, 240.8675706011379987 ) ) ;
#106842=CARTESIAN_POINT ( 'NONE',  ( 12.53380498098208840, 1442.773887284840384, 150.7612718761199062 ) ) ;
#106843=CIRCLE ( 'NONE', #106776, 1.999999999999912514 ) ;
#106845=CARTESIAN_POINT ( 'NONE',  ( -0.6369869090064108619, 1408.970540970598222, 186.3721633967661830 ) ) ;
#106850=CARTESIAN_POINT ( 'NONE',  ( -16.97760529929999862, 1508.233635166930071, 230.2235885397980155 ) ) ;
#106852=EDGE_CURVE ( 'NONE', #65282, #35589, #95161, .T. ) ;
#106854=CARTESIAN_POINT ( 'NONE',  ( -16.06428792994629973, 1414.913060387329779, 209.3174441339999987 ) ) ;
#106856=FACE_OUTER_BOUND ( 'NONE', #59196, .T. ) ;
#106859=ORIENTED_EDGE ( 'NONE', *, *, #80949, .T. ) ;
#106860=CARTESIAN_POINT ( 'NONE',  ( -1.216452466170000024, 1450.942157347929879, 182.7783913332980035 ) ) ;
#106864=CARTESIAN_POINT ( 'NONE',  ( -18.18162401578809906, 1416.230844595159851, 208.9105673229449849 ) ) ;
#106865=EDGE_LOOP ( 'NONE', ( #54214, #57313, #4676, #85902, #105591, #78707 ) ) ;
#106870=CARTESIAN_POINT ( 'NONE',  ( -18.11157384430000050, 1509.545530482630056, 231.7129783355979669 ) ) ;
#106876=AXIS2_PLACEMENT_3D ( 'NONE', #73252, #65421, #81088 ) ;
#106880=CARTESIAN_POINT ( 'NONE',  ( -18.31748438839999693, 1452.000482346729996, 190.7950199775980025 ) ) ;
#106883=ORIENTED_EDGE ( 'NONE', *, *, #33158, .T. ) ;
#106887=CARTESIAN_POINT ( 'NONE',  ( -2.581689387682173376, 1419.606464184852484, 137.0999999981000883 ) ) ;
#106888=CARTESIAN_POINT ( 'NONE',  ( -12.48312717700000007, 1434.436312747890042, 149.9522253733979937 ) ) ;
#106890=CARTESIAN_POINT ( 'NONE',  ( -5.215130879758570953E-10, 1468.939591304350188, 251.0785144346289712 ) ) ;
#106891=CARTESIAN_POINT ( 'NONE',  ( -20.38352471697730195, 1500.853033034210057, 190.5928454434599928 ) ) ;
#106892=FACE_OUTER_BOUND ( 'NONE', #30652, .T. ) ;
#106894=ADVANCED_FACE ( 'NONE', ( #36264 ), #92774, .T. ) ;
#106902=CARTESIAN_POINT ( 'NONE',  ( 11.94888771486709977, 1433.583934366519998, 150.1820132112760007 ) ) ;
#106903=CARTESIAN_POINT ( 'NONE',  ( -13.42182309979999921, 1435.162926645730067, 149.8212854273980099 ) ) ;
#106906=CARTESIAN_POINT ( 'NONE',  ( 19.32254953540159903, 1466.487181286699979, 226.4358010736329732 ) ) ;
#106907=LINE ( 'NONE', #45926, #56891 ) ;
#106909=ORIENTED_EDGE ( 'NONE', *, *, #28761, .T. ) ;
#106910=CARTESIAN_POINT ( 'NONE',  ( 28.66942460980000007, 1426.582479900129783, 248.2467662509980073 ) ) ;
#106911=CARTESIAN_POINT ( 'NONE',  ( -28.24200347660000077, 1508.135538546330281, 208.7967122801030087 ) ) ;
#106912=CARTESIAN_POINT ( 'NONE',  ( 1.515335126600000137, 1458.417426270730175, 183.2389660611979991 ) ) ;
#106913=CARTESIAN_POINT ( 'NONE',  ( 13.15726447020000123, 1414.996442546130083, 197.7616625855980033 ) ) ;
#106914=CARTESIAN_POINT ( 'NONE',  ( 21.27157138040592343, 1506.426094406462198, 203.5633718702692079 ) ) ;
#106915=CARTESIAN_POINT ( 'NONE',  ( -1.271605103970000069E-07, 1420.650940017329958, 220.7242732315979765 ) ) ;
#106918=CARTESIAN_POINT ( 'NONE',  ( -18.90749324119999741, 1416.833018152629847, 208.2176376215240055 ) ) ;
#106919=EDGE_LOOP ( 'NONE', ( #84224, #62525, #1153, #100829 ) ) ;
#106920=CARTESIAN_POINT ( 'NONE',  ( -2.500000000000000000, 1432.344429588900084, 157.4943015532979871 ) ) ;
#106922=CARTESIAN_POINT ( 'NONE',  ( 2.919540490770000218, 1509.015012987830232, 238.5603143811979976 ) ) ;
#106924=ORIENTED_EDGE ( 'NONE', *, *, #24375, .T. ) ;
#106927=CARTESIAN_POINT ( 'NONE',  ( -23.03290791463370013, 1409.747221716589820, 208.9467762737129988 ) ) ;
#106933=CARTESIAN_POINT ( 'NONE',  ( -9.739009285419999884, 1489.054442968930061, 233.7183489316979887 ) ) ;
#106936=VERTEX_POINT ( 'NONE', #31713 ) ;
#106938=CARTESIAN_POINT ( 'NONE',  ( 11.63663615270000129, 1425.864876078829866, 144.1644678884979953 ) ) ;
#106939=CARTESIAN_POINT ( 'NONE',  ( -12.51099735422430115, 1416.825783990419950, 222.1450751212599926 ) ) ;
#106940=EDGE_CURVE ( 'NONE', #80100, #19422, #69808, .T. ) ;
#106941=CARTESIAN_POINT ( 'NONE',  ( -0.1681676274470000065, 1420.473121337229941, 182.7663689088979879 ) ) ;
#106942=( BOUNDED_CURVE ( )  B_SPLINE_CURVE ( 3, ( #64946, #48697, #31316, #98521 ),
 .UNSPECIFIED., .F., .F. ) 
 B_SPLINE_CURVE_WITH_KNOTS ( ( 4, 4 ),
 ( 0.3089224742796055079, 0.9578869033099139951 ),
 .UNSPECIFIED. ) 
 CURVE ( )  GEOMETRIC_REPRESENTATION_ITEM ( )  RATIONAL_B_SPLINE_CURVE ( ( 1.000000000000000000, 0.9652106218856630893, 0.9652106218856630893, 1.000000000000000000 ) ) 
 REPRESENTATION_ITEM ( '' )  );
#106946=CARTESIAN_POINT ( 'NONE',  ( 13.33831059585898160, 1443.295405362211341, 187.7819447126144325 ) ) ;
#106950=B_SPLINE_CURVE_WITH_KNOTS ( 'NONE', 3,
 ( #104768, #35919, #61690, #62242, #105318, #61152, #95812, #63348, #52177, #53850, #97466, #52725, #87987, #11275, #10152, #9593, #1782, #105879, #45438, #29160, #13990, #20735, #29702, #90703, #47076, #12344, #63886, #3983, #46535, #72826, #89058, #74489, #22933, #90147, #106959, #38651, #30801, #57138, #30244, #38107, #13429, #64979, #47619, #72285, #82859, #21271, #81201, #22373, #89606, #54930, #5051, #81744, #56022, #39196, #107511, #73373, #80669, #5613 ),
 .UNSPECIFIED., .F., .F.,
 ( 4, 2, 2, 2, 2, 2, 2, 1, 2, 2, 1, 1, 1, 2, 2, 2, 2, 1, 1, 2, 2, 2, 2, 1, 2, 2, 2, 2, 2, 1, 2, 2, 4 ),
 ( 0.000000000000000000, 0.007812500000247135645, 0.01171875000047535587, 0.01562500000070357609, 0.02343750000116001653, 0.03125000000161645697, 0.04687500000205005457, 0.05468750000226685337, 0.05859375000237715403, 0.06250000000248745469, 0.09375000000158209557, 0.1093750000009845319, 0.1171875000006857570, 0.1210937500006842721, 0.1250000000006827872, 0.1875000000010061396, 0.2187500000011678158, 0.2343750000010602907, 0.2421875000010208778, 0.2460937500010011714, 0.2500000000009814372, 0.3750000000016789348, 0.4375000000019070301, 0.4687500000019094726, 0.4843750000018978152, 0.5000000000018861579, 0.6250000000012420065, 0.6875000000008204548, 0.7031250000008050227, 0.7187500000007895906, 0.7500000000007327472, 0.8750000000003663736, 1.000000000000000000 ),
 .UNSPECIFIED. ) ;
#106954=CARTESIAN_POINT ( 'NONE',  ( 11.90642948233699983, 1452.497278707910027, 149.7233324945059678 ) ) ;
#106958=CARTESIAN_POINT ( 'NONE',  ( -11.87502386937130083, 1433.007271227619867, 149.9804723889419904 ) ) ;
#106959=CARTESIAN_POINT ( 'NONE',  ( 0.03684989003742775160, 1409.759860126017429, 233.0927588586005186 ) ) ;
#106963=EDGE_CURVE ( 'NONE', #27637, #64407, #40421, .T. ) ;
#106965=CARTESIAN_POINT ( 'NONE',  ( -24.03118224474849995, 1507.962100464060086, 222.3137046748230148 ) ) ;
#106968=CARTESIAN_POINT ( 'NONE',  ( 11.09581607402950176, 1414.913057834409983, 221.9014645491780016 ) ) ;
#106974=ORIENTED_EDGE ( 'NONE', *, *, #103466, .T. ) ;
#106975=CARTESIAN_POINT ( 'NONE',  ( 16.81223226430000039, 1414.913060387329779, 210.6693098017280192 ) ) ;
#106976=CARTESIAN_POINT ( 'NONE',  ( -0.8251472201360000591, 1438.194204504490017, 150.6035180695979818 ) ) ;
#106982=ADVANCED_FACE ( 'NONE', ( #15997 ), #75812, .T. ) ;
#106983=CARTESIAN_POINT ( 'NONE',  ( -40.71506490407468704, 1443.618868061724470, 137.1015916554986802 ) ) ;
#106985=CARTESIAN_POINT ( 'NONE',  ( 16.62404756210000301, 1422.111108379129973, 227.0758637081979998 ) ) ;
#106989=CARTESIAN_POINT ( 'NONE',  ( -17.82265795360000027, 1409.535441317430241, 222.1575796720979952 ) ) ;
#106990=CARTESIAN_POINT ( 'NONE',  ( 19.53759129830000063, 1435.323542146659975, 144.9538018687979957 ) ) ;
#106991=CARTESIAN_POINT ( 'NONE',  ( -0.5630044002530000258, 1418.687151651130080, 227.8496307451979703 ) ) ;
#106992=CARTESIAN_POINT ( 'NONE',  ( 5.381136289437809417, 1430.993983722579969, 154.5045433217829896 ) ) ;
#106993=CARTESIAN_POINT ( 'NONE',  ( 12.78730314359999909, 1416.837309316629899, 222.9176234487979968 ) ) ;
#106994=DIRECTION ( 'NONE',  ( 7.447054910797601740E-07, -0.9583089392864349021, -0.2857341017154824137 ) ) ;
#106996=CARTESIAN_POINT ( 'NONE',  ( -36.54919900496939533, 1437.103027518239969, 136.4794237381429696 ) ) ;
#106997=CARTESIAN_POINT ( 'NONE',  ( 0.2153128718845489786, 1454.373455522330005, 183.1944751942430116 ) ) ;
#106998=CARTESIAN_POINT ( 'NONE',  ( -15.26494846990000021, 1409.446124134130059, 210.7631067400780012 ) ) ;
#106999=CARTESIAN_POINT ( 'NONE',  ( -13.02322702410000055, 1416.825784011830137, 196.6108461443980104 ) ) ;
#107001=ADVANCED_FACE ( 'NONE', ( #33915 ), #68109, .T. ) ;
#107003=CARTESIAN_POINT ( 'NONE',  ( 11.87957822189999924, 1433.311236608589979, 147.6243455281980061 ) ) ;
#107004=CARTESIAN_POINT ( 'NONE',  ( -27.23873044170000313, 1435.448403991980058, 135.2737774014979948 ) ) ;
#107005=CARTESIAN_POINT ( 'NONE',  ( 5.567438724339999645, 1439.949778329529863, 185.1713536890979981 ) ) ;
#107006=VERTEX_POINT ( 'NONE', #6519 ) ;
#107007=CARTESIAN_POINT ( 'NONE',  ( -1.322993174137927719, 1450.717402541238243, 181.8644873159974225 ) ) ;
#107009=CARTESIAN_POINT ( 'NONE',  ( 27.84617737630000178, 1442.188138044969946, 137.3853255074979813 ) ) ;
#107013=CARTESIAN_POINT ( 'NONE',  ( 14.87800470701120048, 1508.139627058890028, 232.3565943604129984 ) ) ;
#107014=CARTESIAN_POINT ( 'NONE',  ( 31.99634982962822605, 1416.543175412537494, 269.3157931535475313 ) ) ;
#107023=CIRCLE ( 'NONE', #80267, 1.999996097696930430 ) ;
#107025=EDGE_CURVE ( 'NONE', #96030, #86293, #35064, .T. ) ;
#107027=CARTESIAN_POINT ( 'NONE',  ( 0.4995595210673769437, 1414.543198520750138, 184.8908676557550166 ) ) ;
#107028=ORIENTED_EDGE ( 'NONE', *, *, #107504, .T. ) ;
#107031=CARTESIAN_POINT ( 'NONE',  ( 40.27131413995757470, 1443.849994623672728, 137.1307286851228184 ) ) ;
#107033=CARTESIAN_POINT ( 'NONE',  ( -0.1041750762200730068, 1420.399864921520020, 183.1908796769659773 ) ) ;
#107035=CARTESIAN_POINT ( 'NONE',  ( 21.61088119619999759, 1409.667728988130193, 213.1529199375679866 ) ) ;
#107036=CARTESIAN_POINT ( 'NONE',  ( 14.94707557629999961, 1464.258769156330118, 189.8680940798979861 ) ) ;
#107038=CARTESIAN_POINT ( 'NONE',  ( -17.66402273019999924, 1423.191735939130240, 226.2866990750980278 ) ) ;
#107045=CARTESIAN_POINT ( 'NONE',  ( -2.001405295990000166, 1417.433771689029982, 234.4571982132979997 ) ) ;
#107048=CARTESIAN_POINT ( 'NONE',  ( -5.350563530668329904, 1484.262296847969992, 183.6824371965580269 ) ) ;
#107052=CARTESIAN_POINT ( 'NONE',  ( -4.283506096700399723, 1440.960946171619980, 155.9766071721359992 ) ) ;
#107054=VERTEX_POINT ( 'NONE', #79255 ) ;
#107056=EDGE_LOOP ( 'NONE', ( #103501, #23560, #68, #95903 ) ) ;
#107057=CARTESIAN_POINT ( 'NONE',  ( 28.25086440160000123, 1508.135696994329919, 209.3857010626460067 ) ) ;
#107061=CARTESIAN_POINT ( 'NONE',  ( 15.85916472032949898, 1416.833704394080087, 191.3322456763750097 ) ) ;
#107062=CARTESIAN_POINT ( 'NONE',  ( 1.623739401199999932, 1508.906036784929938, 180.0335669106979992 ) ) ;
#107064=CARTESIAN_POINT ( 'NONE',  ( -24.07745899746860019, 1452.072289599009991, 136.6778791173090042 ) ) ;
#107065=CARTESIAN_POINT ( 'NONE',  ( -11.73650491189999912, 1426.280347616930158, 144.1690576440980180 ) ) ;
#107066=CARTESIAN_POINT ( 'NONE',  ( 14.54631876779999899, 1409.587692354329874, 227.1236616575980065 ) ) ;
#107069=CARTESIAN_POINT ( 'NONE',  ( 41.66155871505439734, 1443.633333538899933, 134.0999999981970063 ) ) ;
#107070=FACE_OUTER_BOUND ( 'NONE', #64312, .T. ) ;
#107076=CARTESIAN_POINT ( 'NONE',  ( 4.231647580394414021, 1410.439481984662734, 231.4381811129047435 ) ) ;
#107078=CARTESIAN_POINT ( 'NONE',  ( -0.05678672266099999560, 1451.699960474029922, 183.0333059144979870 ) ) ;
#107079=CARTESIAN_POINT ( 'NONE',  ( -3.397007901869999902, 1485.996548673229881, 182.1933214028979933 ) ) ;
#107083=CARTESIAN_POINT ( 'NONE',  ( 27.93158904759999928, 1508.017348895330088, 207.9454904019079891 ) ) ;
#107084=CARTESIAN_POINT ( 'NONE',  ( 9.435157646520000441, 1414.913060387329779, 196.1144213233980054 ) ) ;
#107087=DIRECTION ( 'NONE',  ( 0.000000000000000000, 0.000000000000000000, -1.000000000000000000 ) ) ;
#107089=B_SPLINE_CURVE_WITH_KNOTS ( 'NONE', 5,
 ( #4592, #3513, #62322, #20816, #37637, #72900, #30327, #64516, #71842, #13509, #55014, #21899 ),
 .UNSPECIFIED., .F., .F.,
 ( 6, 3, 3, 6 ),
 ( 14.91778236361800047, 20.16173081580000215, 25.40568016630000159, 28.75057693464048469 ),
 .UNSPECIFIED. ) ;
#107091=CARTESIAN_POINT ( 'NONE',  ( 39.34366195029559776, 1440.913060387330006, 266.6071495697630098 ) ) ;
#107092=CARTESIAN_POINT ( 'NONE',  ( -0.0003458708581578771369, 1452.035320502890499, 153.9482814617377073 ) ) ;
#107093=ORIENTED_EDGE ( 'NONE', *, *, #70417, .F. ) ;
#107094=CARTESIAN_POINT ( 'NONE',  ( -0.1083607850349780077, 1451.692459334710065, 183.0338343828840095 ) ) ;
#107095=CARTESIAN_POINT ( 'NONE',  ( -16.05577010409999872, 1409.975501755830010, 191.6037359313979778 ) ) ;
#107096=FACE_OUTER_BOUND ( 'NONE', #96891, .T. ) ;
#107098=CARTESIAN_POINT ( 'NONE',  ( 22.44517203296219776, 1410.596246135090041, 206.2149503098679872 ) ) ;
#107099=B_SPLINE_CURVE_WITH_KNOTS ( 'NONE', 3,
 ( #99345, #98812, #22074, #28866, #107216, #72527, #29947, #64140, #55743, #5869, #56269, #40011, #90960, #5307, #39466, #107768, #63058, #20433, #54640, #46241, #83662, #93699, #59041, #40562, #93163, #108320, #58482, #59584, #99900, #57937, #8603, #16433, #24838, #49537, #65782, #76375, #32162, #84759, #48988, #66349, #92610, #110524, #68002, #50086, #23197, #91523 ),
 .UNSPECIFIED., .F., .F.,
 ( 4, 3, 3, 3, 3, 3, 3, 3, 3, 3, 3, 3, 3, 3, 3, 4 ),
 ( 9.875699484660000138, 11.70136201872880122, 11.94830905290000089, 14.13772687250919979, 15.85048082565690031, 17.40076151789799752, 18.81555256143910171, 19.64990296329999708, 20.88619740925589952, 22.17317058353600245, 23.52607082560420082, 25.04768890600420050, 26.74277199947320227, 29.05331164702660018, 29.41780153859999913, 30.22064862599999913 ),
 .UNSPECIFIED. ) ;
#107101=CARTESIAN_POINT ( 'NONE',  ( -3.535390471679999980, 1507.776749383930110, 180.9473287213979802 ) ) ;
#107102=CARTESIAN_POINT ( 'NONE',  ( -12.91319902290000066, 1434.774343387339968, 147.8554079201980187 ) ) ;
#107104=CARTESIAN_POINT ( 'NONE',  ( 16.47764957789999940, 1459.038222156129905, 230.9212189925980283 ) ) ;
#107105=DIRECTION ( 'NONE',  ( 0.000000000000000000, 0.000000000000000000, -1.000000000000000000 ) ) ;
#107111=CARTESIAN_POINT ( 'NONE',  ( 19.33837180206075956, 1442.618379756513150, 212.9432736166801874 ) ) ;
#107118=CARTESIAN_POINT ( 'NONE',  ( 23.91643402620000103, 1445.742613539229978, 213.3354513389379861 ) ) ;
#107119=CARTESIAN_POINT ( 'NONE',  ( -11.27974580559999929, 1430.696192609630089, 151.3350657528979752 ) ) ;
#107123=CARTESIAN_POINT ( 'NONE',  ( -18.05542497264810109, 1416.825784014559986, 209.4840452940109969 ) ) ;
#107124=CARTESIAN_POINT ( 'NONE',  ( 11.87714051300000051, 1445.674110462049839, 187.3195967386980101 ) ) ;
#107125=CARTESIAN_POINT ( 'NONE',  ( -18.56493692389999950, 1444.808688822819931, 226.5443963784980212 ) ) ;
#107126=CARTESIAN_POINT ( 'NONE',  ( 5.361309434614839553, 1423.568641984250007, 149.4828989101069965 ) ) ;
#107127=CARTESIAN_POINT ( 'NONE',  ( -0.3621993314549999954, 1416.825784017130218, 191.0664210094979865 ) ) ;
#107128=AXIS2_PLACEMENT_3D ( 'NONE', #61130, #47058, #96348 ) ;
#107129=VERTEX_POINT ( 'NONE', #102754 ) ;
#107131=CARTESIAN_POINT ( 'NONE',  ( 1.331407961979999888, 1405.856278196329868, 267.2342693101979876 ) ) ;
#107134=CARTESIAN_POINT ( 'NONE',  ( 22.10779026040307826, 1430.188740980609509, 217.8605039218372212 ) ) ;
#107135=CARTESIAN_POINT ( 'NONE',  ( -26.78836348560000147, 1451.977613598030075, 134.9156010057980097 ) ) ;
#107138=CARTESIAN_POINT ( 'NONE',  ( -2.494611402081910345, 1449.235109927490157, 154.7923003029100073 ) ) ;
#107139=CARTESIAN_POINT ( 'NONE',  ( -1.557563050309025421, 1451.010411511857455, 183.5840749928846094 ) ) ;
#107141=CARTESIAN_POINT ( 'NONE',  ( -19.59053950279439960, 1486.265866315750145, 189.8955481462990065 ) ) ;
#107144=CARTESIAN_POINT ( 'NONE',  ( -19.80583354730000067, 1436.359101690570242, 219.6133835737980178 ) ) ;
#107145=CARTESIAN_POINT ( 'NONE',  ( 19.89552980014500250, 1507.835517169810373, 229.1917673227054024 ) ) ;
#107146=CARTESIAN_POINT ( 'NONE',  ( 2.713894501950000038, 1440.141166743770100, 155.9953435499980117 ) ) ;
#107147=CARTESIAN_POINT ( 'NONE',  ( -1.769923271310000157, 1475.735664967129878, 269.0444966765980439 ) ) ;
#107148=CARTESIAN_POINT ( 'NONE',  ( -11.47040950403622617, 1425.342285957420017, 138.1876487757173493 ) ) ;
#107154=CARTESIAN_POINT ( 'NONE',  ( 12.26979804483799974, 1416.828039243390094, 223.5793509210460002 ) ) ;
#107160=CARTESIAN_POINT ( 'NONE',  ( -10.89711927764389898, 1396.293596177750032, 211.0634950529329785 ) ) ;
#107161=FACE_OUTER_BOUND ( 'NONE', #73724, .T. ) ;
#107163=CARTESIAN_POINT ( 'NONE',  ( -44.90740486440000012, 1439.964170239070199, 269.6916829979979866 ) ) ;
#107164=ORIENTED_EDGE ( 'NONE', *, *, #20564, .F. ) ;
#107165=CARTESIAN_POINT ( 'NONE',  ( 2.500000000000000000, 1411.429641636930000, 146.1721969590979882 ) ) ;
#107167=CARTESIAN_POINT ( 'NONE',  ( -11.81421902116150058, 1428.091850136479934, 150.2203612155920212 ) ) ;
#107168=CARTESIAN_POINT ( 'NONE',  ( 11.12608870130000049, 1426.040907521229883, 108.0448315156979930 ) ) ;
#107172=B_SPLINE_CURVE_WITH_KNOTS ( 'NONE', 5,
 ( #82459, #14128, #39898, #5757, #4115, #98141 ),
 .UNSPECIFIED., .F., .F.,
 ( 6, 6 ),
 ( 0.000000000000000000, 1.000000000000000000 ),
 .UNSPECIFIED. ) ;
#107176=CARTESIAN_POINT ( 'NONE',  ( 2.411010536460000075, 1508.412767799730091, 180.8118562158980183 ) ) ;
#107179=ADVANCED_FACE ( 'NONE', ( #55720 ), #59745, .F. ) ;
#107185=CARTESIAN_POINT ( 'NONE',  ( -7.928786415319999392, 1396.369758677929894, 199.8437903500179686 ) ) ;
#107187=CARTESIAN_POINT ( 'NONE',  ( -21.82696587910000119, 1410.169385423830136, 214.9179092355680041 ) ) ;
#107189=CARTESIAN_POINT ( 'NONE',  ( -12.68794671246196515, 1445.019395964141040, 169.4610012160564736 ) ) ;
#107190=CARTESIAN_POINT ( 'NONE',  ( 11.89850863680000082, 1497.713060387329961, 228.0402318450979919 ) ) ;
#107193=CARTESIAN_POINT ( 'NONE',  ( 17.68800140140000110, 1413.542839617829941, 225.2903305969980181 ) ) ;
#107197=CARTESIAN_POINT ( 'NONE',  ( -37.53081473069939733, 1450.871859837360034, 135.1685289577449964 ) ) ;
#107199=CARTESIAN_POINT ( 'NONE',  ( 10.87134764885750116, 1396.292696212680084, 207.0252786116620030 ) ) ;
#107201=CARTESIAN_POINT ( 'NONE',  ( 11.45344409740000202, 1425.467136357829986, 145.4513200822979968 ) ) ;
#107202=CARTESIAN_POINT ( 'NONE',  ( 41.14441233990000057, 1444.077580987459896, 136.9184759350980016 ) ) ;
#107204=CARTESIAN_POINT ( 'NONE',  ( 16.93884299705920071, 1507.634939766059915, 188.0954313100240256 ) ) ;
#107206=EDGE_LOOP ( 'NONE', ( #57069, #62147, #18309, #97636, #85960 ) ) ;
#107207=EDGE_LOOP ( 'NONE', ( #37940, #25265, #2227, #22061, #37826, #34497, #46190, #94465, #29681, #65226, #102731, #82330, #4905, #54194, #6961, #9794, #39161, #31479, #104450, #45791 ) ) ;
#107209=FACE_OUTER_BOUND ( 'NONE', #26208, .T. ) ;
#107211=CARTESIAN_POINT ( 'NONE',  ( 13.01583361309999809, 1416.817366564930126, 196.3351323531979915 ) ) ;
#107216=CARTESIAN_POINT ( 'NONE',  ( 2.500000000000000000, 1448.768630321689898, 157.0420996650450149 ) ) ;
#107218=CARTESIAN_POINT ( 'NONE',  ( 2.845602704200000055, 1416.216739748429973, 226.8837702527980298 ) ) ;
#107220=ORIENTED_EDGE ( 'NONE', *, *, #19041, .T. ) ;
#107223=CARTESIAN_POINT ( 'NONE',  ( -35.04866985580577676, 1424.104380813952048, 269.5321808552227481 ) ) ;
#107225=CARTESIAN_POINT ( 'NONE',  ( -8.486299124169999430, 1519.913060387329779, 187.6206292133980185 ) ) ;
#107227=CARTESIAN_POINT ( 'NONE',  ( -0.0009079351378022920520, 1450.913092093069963, 181.3802231108539900 ) ) ;
#107228=CARTESIAN_POINT ( 'NONE',  ( -27.56560605785089990, 1440.913060397009986, 229.3484830648729940 ) ) ;
#107230=CARTESIAN_POINT ( 'NONE',  ( -0.2143714289189239952, 1465.016896992510055, 237.3853670223340089 ) ) ;
#107231=CARTESIAN_POINT ( 'NONE',  ( 34.76658121969929738, 1422.301991258000271, 269.9820564234090057 ) ) ;
#107234=CARTESIAN_POINT ( 'NONE',  ( 23.70457460020000084, 1410.841732588929972, 207.9725391979379765 ) ) ;
#107239=CARTESIAN_POINT ( 'NONE',  ( 4.333461763824229429, 1420.406249667820020, 185.6739041016720080 ) ) ;
#107240=CARTESIAN_POINT ( 'NONE',  ( -4.419614911900000109, 1417.909206216429993, 232.4142678098980070 ) ) ;
#107241=CARTESIAN_POINT ( 'NONE',  ( 9.046206015765411834, 1421.595877805006012, 137.0999999980981841 ) ) ;
#107244=AXIS2_PLACEMENT_3D ( 'NONE', #84565, #75639, #8399 ) ;
#107245=DIRECTION ( 'NONE',  ( 9.267597007367818816E-06, 0.03085854715862546352, -0.9995237615891732208 ) ) ;
#107246=CARTESIAN_POINT ( 'NONE',  ( 0.4962749089960000193, 1415.445620500730001, 233.3779880030980109 ) ) ;
#107247=CARTESIAN_POINT ( 'NONE',  ( -20.99189748682200118, 1509.583339404279968, 229.4943028042000321 ) ) ;
#107253=CARTESIAN_POINT ( 'NONE',  ( 18.05542497264820057, 1416.825784014559986, 208.7596466293869923 ) ) ;
#107255=EDGE_LOOP ( 'NONE', ( #84318, #50631, #102123, #86833 ) ) ;
#107260=CARTESIAN_POINT ( 'NONE',  ( 16.68463225901000158, 1442.773887286389936, 162.0935120915889911 ) ) ;
#107261=CARTESIAN_POINT ( 'NONE',  ( 21.94066466509999813, 1452.058359354930190, 220.5450223258980031 ) ) ;
#107263=CARTESIAN_POINT ( 'NONE',  ( 8.113228662610344699, 1437.975597658936522, 153.6229958193256380 ) ) ;
#107264=CARTESIAN_POINT ( 'NONE',  ( 0.03226293719758020068, 1410.297897419189894, 233.2219341505459909 ) ) ;
#107266=CARTESIAN_POINT ( 'NONE',  ( 16.47590419726208921, 1421.672314134083535, 227.1462306721412290 ) ) ;
#107268=CARTESIAN_POINT ( 'NONE',  ( -19.34922152300000064, 1425.422359720030045, 223.6439256038979693 ) ) ;
#107271=CARTESIAN_POINT ( 'NONE',  ( 19.36651210059999784, 1488.299738432130198, 189.6546506392980120 ) ) ;
#107273=CARTESIAN_POINT ( 'NONE',  ( -17.40400757659919506, 1433.874116228432058, 216.4982986272186167 ) ) ;
#107281=VECTOR ( 'NONE', #34954, 1000.000000000000000 ) ;
#107282=CARTESIAN_POINT ( 'NONE',  ( 1.469666176117540246, 1486.774276370960024, 182.0003414483169877 ) ) ;
#107284=CARTESIAN_POINT ( 'NONE',  ( -13.23821889442530697, 1443.160654751977518, 186.8362721621839455 ) ) ;
#107287=CARTESIAN_POINT ( 'NONE',  ( -0.1681681984989999989, 1420.016189442530049, 171.1670476502980023 ) ) ;
#107290=ADVANCED_FACE ( 'NONE', ( #78567 ), #102629, .T. ) ;
#107291=CARTESIAN_POINT ( 'NONE',  ( 24.69316157360000119, 1435.858930896569973, 137.7793382546979899 ) ) ;
#107294=VERTEX_POINT ( 'NONE', #11635 ) ;
#107300=ORIENTED_EDGE ( 'NONE', *, *, #22203, .F. ) ;
#107301=CARTESIAN_POINT ( 'NONE',  ( 16.78845670593169714, 1414.971513442450032, 209.5374550761620185 ) ) ;
#107302=CARTESIAN_POINT ( 'NONE',  ( 13.29979961619999962, 1509.142656770830172, 233.9102947482979857 ) ) ;
#107304=CARTESIAN_POINT ( 'NONE',  ( 29.77132726792740414, 1419.409540564665576, 269.4683900306495730 ) ) ;
#107305=CARTESIAN_POINT ( 'NONE',  ( -28.33103133910000082, 1450.578314054559769, 240.1819618728980004 ) ) ;
#107307=CARTESIAN_POINT ( 'NONE',  ( -11.89338303359999927, 1433.289361183159826, 150.1518857174980042 ) ) ;
#107309=CARTESIAN_POINT ( 'NONE',  ( -19.12425472950000227, 1486.130686572730156, 189.5132436031979921 ) ) ;
#107310=CARTESIAN_POINT ( 'NONE',  ( 24.40137257056360198, 1418.525752740940106, 209.6082346408329897 ) ) ;
#107311=CARTESIAN_POINT ( 'NONE',  ( -27.26752128509999906, 1441.515264747369883, 137.3262972417980166 ) ) ;
#107313=CARTESIAN_POINT ( 'NONE',  ( 7.134032011620000446, 1442.025630637640006, 154.4960302486979913 ) ) ;
#107317=CARTESIAN_POINT ( 'NONE',  ( 4.449893896030659734E-11, 1411.549994435260032, 254.7521586903190212 ) ) ;
#107318=ORIENTED_EDGE ( 'NONE', *, *, #55132, .F. ) ;
#107320=CARTESIAN_POINT ( 'NONE',  ( -11.86575960015439968, 1432.312193440490091, 149.9823566586960055 ) ) ;
#107322=CARTESIAN_POINT ( 'NONE',  ( -15.04635340419999956, 1470.707757194930082, 270.3649393566980166 ) ) ;
#107323=CARTESIAN_POINT ( 'NONE',  ( 13.31241404839999909, 1509.377940129630133, 234.8971984757980067 ) ) ;
#107327=B_SPLINE_CURVE_WITH_KNOTS ( 'NONE', 3,
 ( #103095, #31076, #75313, #5329, #9053, #676 ),
 .UNSPECIFIED., .F., .F.,
 ( 4, 2, 4 ),
 ( 0.000000000000000000, 0.002988018091905742402, 0.005976036183811482203 ),
 .UNSPECIFIED. ) ;
#107328=CARTESIAN_POINT ( 'NONE',  ( 0.3320937139126450277, 1450.964402829440132, 181.7697017419690155 ) ) ;
#107329=CARTESIAN_POINT ( 'NONE',  ( -13.23585369709999959, 1420.111225874029969, 228.0945412171980138 ) ) ;
#107332=CARTESIAN_POINT ( 'NONE',  ( -28.65682362046179676, 1414.257978759259913, 269.3829595885329695 ) ) ;
#107334=EDGE_LOOP ( 'NONE', ( #79975, #40009, #97020, #90242 ) ) ;
#107339=DIRECTION ( 'NONE',  ( 0.3363363969979660806, -0.9417419115949053898, 0.000000000000000000 ) ) ;
#107342=CARTESIAN_POINT ( 'NONE',  ( -16.80535727200000196, 1440.439471750479925, 190.3762289849980220 ) ) ;
#107344=CARTESIAN_POINT ( 'NONE',  ( -17.33645362950000290, 1414.996442546130083, 207.8511177337479978 ) ) ;
#107346=CARTESIAN_POINT ( 'NONE',  ( -26.64877008739999908, 1436.583672242290049, 136.7640741069980095 ) ) ;
#107348=B_SPLINE_CURVE_WITH_KNOTS ( 'NONE', 5,
 ( #93208, #32213, #76416, #100513, #16478, #7004 ),
 .UNSPECIFIED., .F., .F.,
 ( 6, 6 ),
 ( -107.3223151640000026, -30.86246213379999404 ),
 .UNSPECIFIED. ) ;
#107351=CARTESIAN_POINT ( 'NONE',  ( -35.01820525347180535, 1420.005377583910104, 270.2098316748109710 ) ) ;
#107353=CARTESIAN_POINT ( 'NONE',  ( -3.730240969670000073, 1396.578899543130092, 197.1274014984979885 ) ) ;
#107355=EDGE_LOOP ( 'NONE', ( #74176, #17186, #2453, #82289, #10239, #42765, #46776, #55941, #39301 ) ) ;
#107359=CARTESIAN_POINT ( 'NONE',  ( -14.58502509368319977, 1436.245402443870034, 149.8759987050300140 ) ) ;
#107366=CARTESIAN_POINT ( 'NONE',  ( 12.54563646380000108, 1416.254459047329874, 223.2775148006980146 ) ) ;
#107372=ORIENTED_EDGE ( 'NONE', *, *, #107785, .T. ) ;
#107374=CIRCLE ( 'NONE', #93062, 1.560060070890045836 ) ;
#107375=CARTESIAN_POINT ( 'NONE',  ( 25.32192960925430114, 1450.806448946380215, 137.4488745918710322 ) ) ;
#107376=CARTESIAN_POINT ( 'NONE',  ( -4.118002615245018205, 1440.027047901042351, 185.4484253817595629 ) ) ;
#107378=CARTESIAN_POINT ( 'NONE',  ( 20.28125875170000114, 1409.621297549229894, 202.2274701143080051 ) ) ;
#107379=CARTESIAN_POINT ( 'NONE',  ( -24.89775069963104315, 1442.835541681095037, 210.5176539881000508 ) ) ;
#107381=CARTESIAN_POINT ( 'NONE',  ( 4.247914338581740168, 1441.369206175110094, 161.4618793966889996 ) ) ;
#107386=CARTESIAN_POINT ( 'NONE',  ( 3.902542035141590038, 1426.015650130040058, 185.2953857556300079 ) ) ;
#107388=CARTESIAN_POINT ( 'NONE',  ( -11.73564150307709930, 1425.610157878649943, 144.1659385557379949 ) ) ;
#107390=CARTESIAN_POINT ( 'NONE',  ( 11.60004869885203860, 1425.871340881105198, 138.5940851285356530 ) ) ;
#107393=CARTESIAN_POINT ( 'NONE',  ( 17.99132714227145158, 1424.137213421525985, 225.5015134895514564 ) ) ;
#107395=CARTESIAN_POINT ( 'NONE',  ( -3.520303095042100390E-07, 1407.050513786409965, 222.1263857351630122 ) ) ;
#107396=B_SPLINE_SURFACE_WITH_KNOTS ( 'NONE', 5, 5, ( 
 ( #82220, #105796, #63796, #90618, #29077, #73845, #96842, #54844, #3897 ),
 ( #38026, #54302, #88430, #72205, #55391, #12813, #106864, #107419, #38559 ),
 ( #46993, #81116, #72738, #98468, #13342, #47534, #39105, #73282, #76445 ),
 ( #101620, #17049, #43411, #59662, #57051, #102188, #15962, #78100, #93770 ),
 ( #60782, #110050, #1402, #25468, #51246, #92686, #42854, #84826, #51812 ),
 ( #33882, #65453, #85379, #50165, #84293, #26585, #110599, #7584, #99561 ) ),
 .UNSPECIFIED., .F., .F., .F.,
 ( 6, 6 ),
 ( 6, 3, 6 ),
 ( 0.4666582264910000277, 2.797885342316130064 ),
 ( -1.082960613491289913E-05, 1.000000000000000000, 2.000000000000000000 ),
 .UNSPECIFIED. ) ;
#107397=CARTESIAN_POINT ( 'NONE',  ( 32.17164650389580061, 1440.913060383229777, 244.5574107866939926 ) ) ;
#107403=CARTESIAN_POINT ( 'NONE',  ( -19.07563200129111536, 1485.497391648796565, 189.6206291117065348 ) ) ;
#107404=CARTESIAN_POINT ( 'NONE',  ( 12.98226713004290112, 1414.913060387349788, 198.3280232619060257 ) ) ;
#107407=FACE_OUTER_BOUND ( 'NONE', #109273, .T. ) ;
#107411=CARTESIAN_POINT ( 'NONE',  ( -13.74793944760000031, 1453.152003546729929, 193.7924838359980129 ) ) ;
#107413=CARTESIAN_POINT ( 'NONE',  ( 2.750555178629999986, 1464.695220873430117, 236.8701282433979998 ) ) ;
#107415=ORIENTED_EDGE ( 'NONE', *, *, #96727, .T. ) ;
#107416=CARTESIAN_POINT ( 'NONE',  ( -0.4632198342000000135, 1452.646946044229935, 183.2964164767980151 ) ) ;
#107419=CARTESIAN_POINT ( 'NONE',  ( -18.23773974694429967, 1416.535698381769862, 208.9530515259610013 ) ) ;
#107420=ORIENTED_EDGE ( 'NONE', *, *, #91174, .F. ) ;
#107422=ORIENTED_EDGE ( 'NONE', *, *, #64561, .T. ) ;
#107429=CIRCLE ( 'NONE', #96750, 1.000000000000000000 ) ;
#107431=CARTESIAN_POINT ( 'NONE',  ( 3.610699138176100220, 1409.039148779609832, 194.5764597407000167 ) ) ;
#107432=CARTESIAN_POINT ( 'NONE',  ( 0.4274148046680000257, 1409.096031529930087, 185.6227931958979980 ) ) ;
#107435=CARTESIAN_POINT ( 'NONE',  ( 25.50064889474995411, 1507.958245409381789, 199.2056517364818262 ) ) ;
#107436=CARTESIAN_POINT ( 'NONE',  ( -2.304688949170010215, 1449.852729981760149, 182.9576120315739729 ) ) ;
#107438=CIRCLE ( 'NONE', #78855, 1.999999950040888708 ) ;
#107441=CARTESIAN_POINT ( 'NONE',  ( 19.24176482687100176, 1456.016048631040121, 226.4226196092550083 ) ) ;
#107442=CARTESIAN_POINT ( 'NONE',  ( -11.80724586129999842, 1434.031939626420126, 151.0333753425979921 ) ) ;
#107444=CARTESIAN_POINT ( 'NONE',  ( -4.333209346896190216E-10, 1466.864290985080061, 244.5380620273480190 ) ) ;
#107450=CARTESIAN_POINT ( 'NONE',  ( -45.66951489795039265, 1440.472176206239965, 266.1885706457709944 ) ) ;
#107451=CARTESIAN_POINT ( 'NONE',  ( 13.94437673319849935, 1452.624323591719985, 223.0644266127340245 ) ) ;
#107455=CARTESIAN_POINT ( 'NONE',  ( 2.589250188618630322, 1407.329176837810110, 221.9615471100440232 ) ) ;
#107456=CARTESIAN_POINT ( 'NONE',  ( -14.09108604789070185, 1436.127728589789967, 150.1512849377759835 ) ) ;
#107460=EDGE_LOOP ( 'NONE', ( #40219, #31317, #73917, #61804 ) ) ;
#107461=CARTESIAN_POINT ( 'NONE',  ( 31.18244400170000219, 1434.782053685459914, 244.2061907803979750 ) ) ;
#107463=CARTESIAN_POINT ( 'NONE',  ( 1.502583036259999894, 1464.119958549930061, 182.9892790823980135 ) ) ;
#107465=CARTESIAN_POINT ( 'NONE',  ( -44.93136215053984728, 1435.581077993269218, 269.6838109711935090 ) ) ;
#107466=CARTESIAN_POINT ( 'NONE',  ( -9.325404488320000240, 1417.437271135130004, 238.2842604422980060 ) ) ;
#107468=CARTESIAN_POINT ( 'NONE',  ( -15.48003957830860067, 1452.372485493469867, 147.5117064112409935 ) ) ;
#107469=CARTESIAN_POINT ( 'NONE',  ( -18.64646854149999911, 1416.843576337130116, 208.5596655672609927 ) ) ;
#107471=DIRECTION ( 'NONE',  ( 0.2857341030884418265, -0.9583089388770653638, 7.461198772136227059E-07 ) ) ;
#107473=CARTESIAN_POINT ( 'NONE',  ( 14.24651345449999873, 1509.423843874130171, 235.0733074521980086 ) ) ;
#107477=CARTESIAN_POINT ( 'NONE',  ( -24.11493509802720325, 1410.987047801660083, 208.7879060775239850 ) ) ;
#107479=CARTESIAN_POINT ( 'NONE',  ( -0.04536310503330000243, 1416.820969729929857, 227.2853261166980303 ) ) ;
#107482=CARTESIAN_POINT ( 'NONE',  ( -2.903514209118760014, 1462.727859335829862, 184.2752576602030103 ) ) ;
#107487=CARTESIAN_POINT ( 'NONE',  ( 45.51178678918370224, 1443.683907448070158, 268.9784073772149782 ) ) ;
#107489=CARTESIAN_POINT ( 'NONE',  ( -12.37273845018560081, 1415.932840154009909, 221.9815680357259851 ) ) ;
#107490=CARTESIAN_POINT ( 'NONE',  ( 0.1792131508849999777, 1419.175541713529810, 184.6431858978980074 ) ) ;
#107494=DIRECTION ( 'NONE',  ( 0.000000000000000000, 0.000000000000000000, 1.000000000000000000 ) ) ;
#107496=B_SPLINE_CURVE_WITH_KNOTS ( 'NONE', 3,
 ( #78345, #85616, #8359, #42527, #35790, #27381, #17291, #2217, #70526, #34126, #102423, #68314, #25704, #77252, #59357, #93465, #8916, #43091, #3318, #45863, #37995, #72709, #98438, #87866, #30126, #72178, #54810, #11155, #90031, #53728, #19522, #46419, #88938, #62684, #13308, #47503, #45316, #71078, #79454, #2765, #79996, #37445, #4403, #106832, #12229, #71643, #105763, #29048, #64317, #21708, #36885, #55913, #106297, #80551, #105203, #81627, #28492, #54272, #29580, #96807, #62121, #63765, #81086, #63234, #97879, #20077, #88397, #38531, #11688, #97340, #21155, #12786, #20610, #3867, #55360, #89492, #46965, #4929, #39073 ),
 .UNSPECIFIED., .F., .F.,
 ( 4, 3, 3, 3, 3, 3, 3, 3, 3, 3, 3, 3, 3, 3, 3, 3, 3, 3, 3, 3, 3, 3, 3, 3, 3, 3, 4 ),
 ( 0.000000000000000000, 0.4544021449487510300, 0.9179962495654619969, 1.396393621504530058, 1.883881772313160008, 2.384423073347710087, 2.507852632510000124, 3.024297152344930684, 3.546339487294009718, 4.069687867730900521, 4.589703316606949635, 5.097876012234750398, 5.597257678202040232, 6.082185787997209658, 6.405353355340000832, 7.038449128034610425, 7.690329614618261367, 8.360401334715410471, 9.048938637463850299, 9.739081358835889546, 10.41820253846390010, 10.57568948873339920, 11.41685275061539961, 12.28892242647819977, 13.18071908141179982, 14.10021730575109977, 14.18573955799999986 ),
 .UNSPECIFIED. ) ;
#107501=EDGE_CURVE ( 'NONE', #74953, #48466, #60471, .T. ) ;
#107504=EDGE_CURVE ( 'NONE', #52145, #99066, #32212, .T. ) ;
#107507=CARTESIAN_POINT ( 'NONE',  ( -1.657064955213390106E-05, 1410.034462405030126, 269.8654312530960055 ) ) ;
#107509=B_SPLINE_CURVE_WITH_KNOTS ( 'NONE', 3,
 ( #73000, #74654, #98731, #73559, #99265, #6330, #30976, #74105, #49452, #23114, #6870, #83575, #41027, #4681, #107692, #65152, #108235, #99822, #47239, #55660, #23673, #22543, #75205, #5795, #32083, #100388, #29872, #21993, #56185, #81926, #48912, #56745, #90881, #89782, #65702, #13052, #31523, #83039, #38820, #47789, #14168, #57318, #91445, #40481, #48353, #82493, #81367, #108791, #107134, #66271, #57856, #30426, #5229, #39936, #91985, #64613, #15260, #39382, #90322, #13602, #64060, #98179, #21449, #42695, #50551, #75749, #109894, #84675, #18020 ),
 .UNSPECIFIED., .F., .F.,
 ( 4, 2, 2, 1, 1, 2, 2, 2, 2, 1, 1, 1, 2, 2, 2, 2, 1, 1, 1, 2, 2, 2, 1, 1, 1, 1, 2, 2, 2, 1, 1, 1, 2, 2, 2, 1, 1, 2, 2, 2, 2, 2, 4 ),
 ( 0.000000000000000000, 0.06249999999907170090, 0.09374999999862482225, 0.1093749999984014037, 0.1171874999982728954, 0.1210937499981919879, 0.1249999999981110665, 0.1874999999972762066, 0.2187499999968588182, 0.2343749999966500963, 0.2421874999965457909, 0.2460937499965085429, 0.2480468749964898911, 0.2499999999964712116, 0.3124999999961673991, 0.3437499999960300090, 0.3593749999959603425, 0.3671874999959142127, 0.3710937499958910646, 0.3730468749958914532, 0.3749999999958918417, 0.4374999999964430120, 0.4687499999967315589, 0.4843749999968646747, 0.4921874999969201858, 0.4960937499969577114, 0.4980468749969765851, 0.4999999999969954034, 0.5624999999973115949, 0.5937499999974805709, 0.6093749999975639486, 0.6171874999976156850, 0.6210937499976517673, 0.6249999999976877385, 0.6874999999981096233, 0.7187499999983193444, 0.7343749999984254817, 0.7421874999984677812, 0.7499999999985099697, 0.8124999999988933297, 0.8437499999990838440, 0.8749999999992744693, 1.000000000000000000 ),
 .UNSPECIFIED. ) ;
#107510=CARTESIAN_POINT ( 'NONE',  ( -20.40003431008743462, 1509.667963569866515, 230.7573408031066720 ) ) ;
#107511=CARTESIAN_POINT ( 'NONE',  ( 0.01224639691883819444, 1408.939459843195209, 232.0643345525089103 ) ) ;
#107512=CARTESIAN_POINT ( 'NONE',  ( -16.77483171992739841, 1414.364824855560073, 191.6397021085149959 ) ) ;
#107517=CARTESIAN_POINT ( 'NONE',  ( 7.298550013359999866, 1430.724169039930075, 149.5003602673979799 ) ) ;
#107528=FACE_OUTER_BOUND ( 'NONE', #11366, .T. ) ;
#107529=CARTESIAN_POINT ( 'NONE',  ( -14.00913000090000082, 1416.839648763730111, 221.8523350387980031 ) ) ;
#107530=CARTESIAN_POINT ( 'NONE',  ( 11.55605632620000200, 1433.836531958829937, 151.2482139994980059 ) ) ;
#107531=CARTESIAN_POINT ( 'NONE',  ( 10.83195828224429214, 1414.913060387329779, 221.4508951956685792 ) ) ;
#107532=CARTESIAN_POINT ( 'NONE',  ( 12.40160425683189871, 1414.913057846380070, 197.9605655507020003 ) ) ;
#107533=EDGE_CURVE ( 'NONE', #48130, #63715, #8277, .T. ) ;
#107537=EDGE_CURVE ( 'NONE', #59101, #54399, #4351, .T. ) ;
#107538=CARTESIAN_POINT ( 'NONE',  ( 5.972257072449999704, 1422.095562574530049, 231.6255282193980065 ) ) ;
#107541=CARTESIAN_POINT ( 'NONE',  ( -17.26894667200000200, 1409.516105293429973, 223.1920633181979952 ) ) ;
#107543=EDGE_CURVE ( 'NONE', #88970, #94093, #109840, .T. ) ;
#107544=CARTESIAN_POINT ( 'NONE',  ( 20.19608870919999788, 1508.016571200030057, 189.3847908446980171 ) ) ;
#107546=CARTESIAN_POINT ( 'NONE',  ( -17.28494824625980186, 1410.440304317500022, 192.2716381327950046 ) ) ;
#107550=CARTESIAN_POINT ( 'NONE',  ( -10.26243781420000012, 1415.425644477229980, 223.2927970104979920 ) ) ;
#107552=CARTESIAN_POINT ( 'NONE',  ( -10.96539760289999954, 1409.236356875930142, 199.6509366764479694 ) ) ;
#107553=CARTESIAN_POINT ( 'NONE',  ( -16.73038498189999856, 1415.425582719929707, 203.0852499532379909 ) ) ;
#107555=CARTESIAN_POINT ( 'NONE',  ( -28.90421869647610009, 1509.875083456920038, 211.4900521685889885 ) ) ;
#107556=CARTESIAN_POINT ( 'NONE',  ( 13.19887955559999959, 1434.900409039649958, 147.6247122247980030 ) ) ;
#107557=CARTESIAN_POINT ( 'NONE',  ( -34.92262157014030066, 1435.778361307009845, 134.0999999978019730 ) ) ;
#107558=CARTESIAN_POINT ( 'NONE',  ( 4.053537042790000378, 1441.572390738320109, 183.3424090224980034 ) ) ;
#107565=CARTESIAN_POINT ( 'NONE',  ( 14.38486959344260008, 1507.535180641189982, 232.5758893386449984 ) ) ;
#107566=CARTESIAN_POINT ( 'NONE',  ( 27.40305221345824549, 1413.568219286974681, 269.4051270913062694 ) ) ;
#107567=CARTESIAN_POINT ( 'NONE',  ( 20.39519499389999879, 1453.159462793129933, 209.8471671030170000 ) ) ;
#107569=CARTESIAN_POINT ( 'NONE',  ( 2.661139925880000145, 1428.713487558729867, 184.2796365262979918 ) ) ;
#107574=CARTESIAN_POINT ( 'NONE',  ( -29.27865644980259674, 1509.812245390119870, 208.6395913010300092 ) ) ;
#107575=CARTESIAN_POINT ( 'NONE',  ( -6.754078978114156584, 1512.913060387330006, 184.4732361498326156 ) ) ;
#107576=CARTESIAN_POINT ( 'NONE',  ( -15.83290313645639991, 1409.465936823030006, 225.2763103180130031 ) ) ;
#107581=CARTESIAN_POINT ( 'NONE',  ( 23.10442899973940101, 1411.095127650270115, 207.3185325528490068 ) ) ;
#107583=CARTESIAN_POINT ( 'NONE',  ( -0.3973340087122340103, 1418.672806152889962, 184.7148007238050127 ) ) ;
#107584=CARTESIAN_POINT ( 'NONE',  ( -2.030806273019999773E-05, 1465.118916741829935, 238.1343320395980072 ) ) ;
#107585=CARTESIAN_POINT ( 'NONE',  ( 22.94835125820000243, 1411.074625106729854, 213.6345867971880068 ) ) ;
#107586=CARTESIAN_POINT ( 'NONE',  ( -2.668712174941869630, 1414.945758603789955, 186.3719431407839693 ) ) ;
#107591=CARTESIAN_POINT ( 'NONE',  ( 24.08291147301929769, 1411.090674609899906, 209.6339324557180248 ) ) ;
#107596=EDGE_CURVE ( 'NONE', #44597, #59669, #13622, .T. ) ;
#107599=CARTESIAN_POINT ( 'NONE',  ( -3.320716570817880076, 1484.261045064220070, 183.3706358249989989 ) ) ;
#107602=CARTESIAN_POINT ( 'NONE',  ( -4.227936195309520251, 1441.550847847370051, 165.4924148592990036 ) ) ;
#107605=ORIENTED_EDGE ( 'NONE', *, *, #101526, .F. ) ;
#107606=CARTESIAN_POINT ( 'NONE',  ( 28.01396353250000004, 1509.154209357430091, 211.9611640590480022 ) ) ;
#107609=CARTESIAN_POINT ( 'NONE',  ( -19.53984293939999972, 1410.902666576429965, 197.4202668715979883 ) ) ;
#107610=CARTESIAN_POINT ( 'NONE',  ( -11.73792004973664227, 1426.279486323856190, 144.2703440561577395 ) ) ;
#107611=CARTESIAN_POINT ( 'NONE',  ( 0.5133626083067620582, 1410.311097044259895, 185.0719925509139898 ) ) ;
#107613=( BOUNDED_CURVE ( )  B_SPLINE_CURVE ( 3, ( #44966, #61768, #105403, #20822 ),
 .UNSPECIFIED., .F., .T. ) 
 B_SPLINE_CURVE_WITH_KNOTS ( ( 4, 4 ),
 ( 2.550106748235465126, 2.860742008493075250 ),
 .UNSPECIFIED. ) 
 CURVE ( )  GEOMETRIC_REPRESENTATION_ITEM ( )  RATIONAL_B_SPLINE_CURVE ( ( 1.000000000000000000, 0.9919749634430294893, 0.9919749634430294893, 1.000000000000000000 ) ) 
 REPRESENTATION_ITEM ( '' )  );
#107615=ADVANCED_FACE ( 'NONE', ( #29530 ), #42760, .T. ) ;
#107616=CARTESIAN_POINT ( 'NONE',  ( -25.50355197240790162, 1451.146063814939907, 136.9902061369730291 ) ) ;
#107617=CARTESIAN_POINT ( 'NONE',  ( -11.73652925620000076, 1426.280330920429833, 144.1708004945979837 ) ) ;
#107622=B_SPLINE_CURVE_WITH_KNOTS ( 'NONE', 3,
 ( #108940, #92673, #50151, #7574, #75888, #25454, #23259 ),
 .UNSPECIFIED., .F., .F.,
 ( 4, 3, 4 ),
 ( -167.5289128750000032, -131.9184636301120008, -78.04659651044040913 ),
 .UNSPECIFIED. ) ;
#107623=CARTESIAN_POINT ( 'NONE',  ( -39.96762391852740137, 1441.625738433479910, 136.8927567948610147 ) ) ;
#107627=ORIENTED_EDGE ( 'NONE', *, *, #55579, .T. ) ;
#107629=CARTESIAN_POINT ( 'NONE',  ( 13.81770597796416666, 1410.768353600875116, 228.1343084947812088 ) ) ;
#107632=CARTESIAN_POINT ( 'NONE',  ( -3.127789639369999986, 1485.522978138030112, 182.9202317313979904 ) ) ;
#107633=CARTESIAN_POINT ( 'NONE',  ( -2.500000000000000000, 1439.522697816390064, 164.2180430355600151 ) ) ;
#107638=EDGE_CURVE ( 'NONE', #28487, #35481, #21558, .T. ) ;
#107640=CARTESIAN_POINT ( 'NONE',  ( 12.37274144529999909, 1415.932840167130053, 196.2621264754979791 ) ) ;
#107643=AXIS2_PLACEMENT_3D ( 'NONE', #74298, #30619, #55847 ) ;
#107647=CARTESIAN_POINT ( 'NONE',  ( 35.79086060848550233, 1440.913060387330006, 261.9942551139580473 ) ) ;
#107648=CARTESIAN_POINT ( 'NONE',  ( -0.0001992799835346449090, 1452.696936729286335, 153.3245174021012076 ) ) ;
#107650=CARTESIAN_POINT ( 'NONE',  ( -0.2439063137306309859, 1452.338815250500147, 183.2775397759450016 ) ) ;
#107653=CARTESIAN_POINT ( 'NONE',  ( -2.919621720534709919, 1419.522956690290130, 186.2043860719099939 ) ) ;
#107654=CARTESIAN_POINT ( 'NONE',  ( -13.04207679966010147, 1409.368499744919745, 225.9431846064669855 ) ) ;
#107656=CARTESIAN_POINT ( 'NONE',  ( -2.162510980229999991, 1508.218318618129842, 180.6352365529979807 ) ) ;
#107658=CARTESIAN_POINT ( 'NONE',  ( 26.11817593136069604, 1491.282851520119948, 206.2269962030060242 ) ) ;
#107659=ADVANCED_FACE ( 'NONE', ( #16553 ), #42343, .T. ) ;
#107660=CARTESIAN_POINT ( 'NONE',  ( 17.13490080239999713, 1458.470257116130142, 230.0791330072979974 ) ) ;
#107661=CARTESIAN_POINT ( 'NONE',  ( -11.60004869883471557, 1424.776443364156648, 137.5692383712261062 ) ) ;
#107662=CARTESIAN_POINT ( 'NONE',  ( -4.846113964861681112, 1422.339154117763201, 184.7758569840760572 ) ) ;
#107666=CARTESIAN_POINT ( 'NONE',  ( -0.1360155611962030053, 1507.785361668840096, 180.7547526672690026 ) ) ;
#107667=CARTESIAN_POINT ( 'NONE',  ( 18.49405840734494078, 1446.012071220772441, 215.4331772447790740 ) ) ;
#107670=CARTESIAN_POINT ( 'NONE',  ( 18.55728982200000132, 1509.324399912330136, 187.7614924380980028 ) ) ;
#107671=CARTESIAN_POINT ( 'NONE',  ( -11.60004869885203682, 1426.116538955981241, 139.0982239796293527 ) ) ;
#107676=CARTESIAN_POINT ( 'NONE',  ( -11.55594655870000054, 1430.767682321529946, 151.0182484257979922 ) ) ;
#107679=CARTESIAN_POINT ( 'NONE',  ( -20.22359736010910325, 1485.406499196400091, 187.9853393324099784 ) ) ;
#107683=CARTESIAN_POINT ( 'NONE',  ( -19.94616634080000139, 1444.802756643080102, 224.2822642680980039 ) ) ;
#107684=CARTESIAN_POINT ( 'NONE',  ( -3.187593557069610117, 1421.874555467776645, 137.0999999977043728 ) ) ;
#107685=CARTESIAN_POINT ( 'NONE',  ( -1.808741800610000006, 1485.212281157229882, 182.6012063751979895 ) ) ;
#107688=CARTESIAN_POINT ( 'NONE',  ( 4.970023385829999363, 1406.187660922729947, 266.9514890597980070 ) ) ;
#107691=CARTESIAN_POINT ( 'NONE',  ( 18.46986075919999948, 1410.877533305329962, 194.2880693953979971 ) ) ;
#107692=CARTESIAN_POINT ( 'NONE',  ( 24.29957117401547961, 1437.103412567565329, 213.1125009194426809 ) ) ;
#107694=CARTESIAN_POINT ( 'NONE',  ( 11.60004869885204037, 1423.119116085875930, 136.9990592530850506 ) ) ;
#107697=CARTESIAN_POINT ( 'NONE',  ( -0.8729612245483540089, 1450.882575899840049, 154.5162482229659986 ) ) ;
#107698=CARTESIAN_POINT ( 'NONE',  ( -12.29575077220000168, 1445.147283749560074, 186.2458169469979907 ) ) ;
#107699=CARTESIAN_POINT ( 'NONE',  ( -19.81676069552977282, 1485.772319128206391, 190.4006065858834518 ) ) ;
#107701=CYLINDRICAL_SURFACE ( 'NONE', #110455, 1.455175085940062507 ) ;
#107702=CARTESIAN_POINT ( 'NONE',  ( -15.71554773450000297, 1429.441490235930132, 224.8635562088979896 ) ) ;
#107704=CARTESIAN_POINT ( 'NONE',  ( 2.500000002460000204, 1440.023046414310102, 162.2537046324979997 ) ) ;
#107705=CARTESIAN_POINT ( 'NONE',  ( -2.772197528860000038, 1475.921741880330046, 267.2318177738980012 ) ) ;
#107706=CARTESIAN_POINT ( 'NONE',  ( -11.03641823134053723, 1425.191710119871232, 138.6345187158980252 ) ) ;
#107707=CARTESIAN_POINT ( 'NONE',  ( -17.63857530519999983, 1411.941882070129850, 193.4046992581980078 ) ) ;
#107710=CARTESIAN_POINT ( 'NONE',  ( 1.455000209906389896, 1507.073729425429974, 236.7651043255590082 ) ) ;
#107712=CARTESIAN_POINT ( 'NONE',  ( 12.24150297172569957, 1416.512142028610015, 223.5518725947510177 ) ) ;
#107715=CARTESIAN_POINT ( 'NONE',  ( -14.38276615813130022, 1509.537722091349906, 182.7943691049900110 ) ) ;
#107716=CARTESIAN_POINT ( 'NONE',  ( -19.69424761119999800, 1410.523354731429890, 197.7052557853979806 ) ) ;
#107717=B_SPLINE_CURVE_WITH_KNOTS ( 'NONE', 3,
 ( #74873, #32837, #109024, #33383, #77077, #40702, #101137, #24431, #59722, #15477 ),
 .UNSPECIFIED., .F., .F.,
 ( 4, 2, 2, 2, 4 ),
 ( -0.1358553352198900166, -0.1155267796648780099, -0.07212482838321790379, -0.03632190733730258914, -3.752851029936721261E-09 ),
 .UNSPECIFIED. ) ;
#107720=ORIENTED_EDGE ( 'NONE', *, *, #6539, .F. ) ;
#107723=CARTESIAN_POINT ( 'NONE',  ( 11.11916130470000041, 1425.182366623929965, 141.8404308875980178 ) ) ;
#107736=ORIENTED_EDGE ( 'NONE', *, *, #49063, .F. ) ;
#107738=CARTESIAN_POINT ( 'NONE',  ( -14.29155582609999975, 1442.454908126789860, 188.8169266407979876 ) ) ;
#107739=CARTESIAN_POINT ( 'NONE',  ( -20.92480426329999688, 1409.643770653630099, 213.2359878676279834 ) ) ;
#107741=CARTESIAN_POINT ( 'NONE',  ( -13.29164969346664193, 1444.599138759567268, 169.3795078411781105 ) ) ;
#107742=CARTESIAN_POINT ( 'NONE',  ( -25.31823295080000236, 1509.573488454329890, 197.1833682395979679 ) ) ;
#107745=CARTESIAN_POINT ( 'NONE',  ( -1.359675940647320003, 1412.718853561030073, 185.5028861769010007 ) ) ;
#107747=CARTESIAN_POINT ( 'NONE',  ( 2.642385910419999817, 1429.770789213729813, 184.7597551400980080 ) ) ;
#107748=CARTESIAN_POINT ( 'NONE',  ( -7.681064681269999639, 1415.931669658029932, 192.6807567567980186 ) ) ;
#107749=CARTESIAN_POINT ( 'NONE',  ( -40.94874006156769752, 1446.742020086070170, 136.1409490009270087 ) ) ;
#107751=CARTESIAN_POINT ( 'NONE',  ( 10.06792015711779875, 1396.264639913020119, 204.5271174533559986 ) ) ;
#107752=CARTESIAN_POINT ( 'NONE',  ( 0.7440358369610000633, 1416.274718422629803, 190.3966560648979964 ) ) ;
#107753=CARTESIAN_POINT ( 'NONE',  ( 11.75171807110000088, 1426.266890984929887, 145.3097295381980132 ) ) ;
#107754=CARTESIAN_POINT ( 'NONE',  ( 40.71506682779999409, 1443.618738319280055, 137.1015903996979830 ) ) ;
#107755=ORIENTED_EDGE ( 'NONE', *, *, #26767, .T. ) ;
#107759=ORIENTED_EDGE ( 'NONE', *, *, #103754, .T. ) ;
#107760=CARTESIAN_POINT ( 'NONE',  ( -38.60872993109999385, 1443.613625523540122, 137.1750381502980076 ) ) ;
#107762=CARTESIAN_POINT ( 'NONE',  ( -12.78657892559999887, 1416.813004075630033, 195.9657752819979919 ) ) ;
#107768=CARTESIAN_POINT ( 'NONE',  ( 2.500000000000000000, 1448.458776228290162, 161.2301877404750030 ) ) ;
#107770=CARTESIAN_POINT ( 'NONE',  ( 18.89907699009999931, 1416.828040557830036, 210.6687202295679811 ) ) ;
#107776=CARTESIAN_POINT ( 'NONE',  ( -16.20545877105858423, 1412.767257293050761, 269.3699492879471222 ) ) ;
#107777=CARTESIAN_POINT ( 'NONE',  ( -1.271723871399999872, 1409.895803293729841, 232.9734008183979768 ) ) ;
#107778=EDGE_CURVE ( 'NONE', #91418, #103319, #31104, .T. ) ;
#107779=CARTESIAN_POINT ( 'NONE',  ( -3.871411596960000256, 1475.513060387329915, 188.6584480527980077 ) ) ;
#107780=EDGE_LOOP ( 'NONE', ( #102865, #3183, #91155, #5841 ) ) ;
#107781=CARTESIAN_POINT ( 'NONE',  ( 2.500000000000000000, 1421.615752562629950, 151.7766360386979727 ) ) ;
#107782=CARTESIAN_POINT ( 'NONE',  ( -27.10898335609390131, 1440.913060414239908, 227.3295655018380046 ) ) ;
#107784=CARTESIAN_POINT ( 'NONE',  ( -0.2823795768692209940, 1467.126800852679935, 235.6211964996780068 ) ) ;
#107785=EDGE_CURVE ( 'NONE', #31171, #6800, #47801, .T. ) ;
#107786=CARTESIAN_POINT ( 'NONE',  ( 8.103047004457721414, 1409.756119192850065, 270.3694257726410228 ) ) ;
#107790=CARTESIAN_POINT ( 'NONE',  ( 24.09245823930000086, 1410.845047763129969, 209.4791609914190076 ) ) ;
#107791=CARTESIAN_POINT ( 'NONE',  ( -20.01067139950000140, 1507.877425041529932, 188.9709217985979706 ) ) ;
#107795=CARTESIAN_POINT ( 'NONE',  ( 0.3019365487449059970, 1424.316146906500080, 227.5104060230709990 ) ) ;
#107796=CARTESIAN_POINT ( 'NONE',  ( 15.08448175589999884, 1409.953164874830009, 191.7150831455979869 ) ) ;
#107799=ORIENTED_EDGE ( 'NONE', *, *, #55094, .T. ) ;
#107801=CARTESIAN_POINT ( 'NONE',  ( 0.7024623020930000905, 1417.310603422230088, 234.7649661555979890 ) ) ;
#107802=DIRECTION ( 'NONE',  ( -1.000000000000000000, 0.000000000000000000, 0.000000000000000000 ) ) ;
#107807=DIRECTION ( 'NONE',  ( -0.03489949451910427658, -0.1170788569999639955, 0.9925092274260693959 ) ) ;
#107812=EDGE_CURVE ( 'NONE', #98568, #79053, #71207, .T. ) ;
#107814=ORIENTED_EDGE ( 'NONE', *, *, #105925, .F. ) ;
#107816=CARTESIAN_POINT ( 'NONE',  ( 20.63350300269999948, 1453.978644282629830, 223.8963513020979974 ) ) ;
#107821=CARTESIAN_POINT ( 'NONE',  ( 16.02248003201332693, 1421.322728439146886, 227.4075243507649020 ) ) ;
#107822=CARTESIAN_POINT ( 'NONE',  ( -3.657345064219999831, 1446.327858494690190, 165.9157432180979868 ) ) ;
#107823=CARTESIAN_POINT ( 'NONE',  ( -19.44038716410000234, 1426.366113336930084, 223.7849254028979828 ) ) ;
#107824=CARTESIAN_POINT ( 'NONE',  ( -24.10732407660000121, 1435.765176705550175, 139.1454052177980145 ) ) ;
#107826=CARTESIAN_POINT ( 'NONE',  ( 19.29275756170000022, 1507.866073478030103, 188.6099784302979856 ) ) ;
#107828=CARTESIAN_POINT ( 'NONE',  ( -29.71179856916630158, 1462.459958223590093, 269.4677673287446282 ) ) ;
#107834=CARTESIAN_POINT ( 'NONE',  ( -0.2151303249849999821, 1415.407078916530054, 233.4369296871979884 ) ) ;
#107835=CARTESIAN_POINT ( 'NONE',  ( -13.49108505849066830, 1443.663885487968173, 187.1285806743424587 ) ) ;
#107837=CARTESIAN_POINT ( 'NONE',  ( -3.665627820750973598, 1507.166784779998579, 236.6858190950203493 ) ) ;
#107840=CARTESIAN_POINT ( 'NONE',  ( 17.04824238339829634, 1423.676546790900147, 228.9394188427949928 ) ) ;
#107841=CARTESIAN_POINT ( 'NONE',  ( -12.83622357435112527, 1442.860320894220195, 169.4450327812936052 ) ) ;
#107842=CARTESIAN_POINT ( 'NONE',  ( 18.00387273070569805, 1424.690294994519945, 226.0499844219949921 ) ) ;
#107846=EDGE_LOOP ( 'NONE', ( #12766, #5567, #29856, #66563 ) ) ;
#107848=CARTESIAN_POINT ( 'NONE',  ( 18.06717587838990013, 1416.826860677879949, 208.8995450462120118 ) ) ;
#107849=CARTESIAN_POINT ( 'NONE',  ( 12.95381060480000102, 1508.673484890930013, 233.5419616260979865 ) ) ;
#107851=CARTESIAN_POINT ( 'NONE',  ( -19.57999079410000220, 1459.737765216430034, 238.2202614069979916 ) ) ;
#107852=CARTESIAN_POINT ( 'NONE',  ( -19.39408456770000200, 1487.979652943030032, 189.5452868223979976 ) ) ;
#107853=CARTESIAN_POINT ( 'NONE',  ( -11.88208569280000049, 1433.207756250380044, 150.1653117102979991 ) ) ;
#107857=CARTESIAN_POINT ( 'NONE',  ( -26.44687317989999897, 1439.558179940190030, 137.2464839519979876 ) ) ;
#107859=CARTESIAN_POINT ( 'NONE',  ( 5.820774579480000099, 1441.874794564960212, 154.7773490369980038 ) ) ;
#107862=CARTESIAN_POINT ( 'NONE',  ( -2.612018202825398649, 1509.136298029517775, 239.0293567375654789 ) ) ;
#107863=CARTESIAN_POINT ( 'NONE',  ( 1.500377517123119864E-08, 1408.384000088409948, 262.1948535354470096 ) ) ;
#107865=ORIENTED_EDGE ( 'NONE', *, *, #45307, .F. ) ;
#107866=CARTESIAN_POINT ( 'NONE',  ( -11.86404314291600137, 1432.192232348270181, 149.9804585586999792 ) ) ;
#107869=CARTESIAN_POINT ( 'NONE',  ( -3.165485081419999958, 1473.508234980229872, 270.3910588708980640 ) ) ;
#107870=CARTESIAN_POINT ( 'NONE',  ( 12.72577279029999886, 1508.073447237130040, 233.4251884259979875 ) ) ;
#107878=CARTESIAN_POINT ( 'NONE',  ( -37.64115395575449696, 1420.091924967339992, 267.8855929252160308 ) ) ;
#107879=ORIENTED_EDGE ( 'NONE', *, *, #82871, .F. ) ;
#107882=ORIENTED_EDGE ( 'NONE', *, *, #24836, .F. ) ;
#107884=CARTESIAN_POINT ( 'NONE',  ( 34.00753574056176376, 1444.324653571831277, 154.9193549732159454 ) ) ;
#107885=DIRECTION ( 'NONE',  ( 0.03489949670251145386, -0.9993908270190954291, 0.000000000000000000 ) ) ;
#107887=CARTESIAN_POINT ( 'NONE',  ( -4.221362096953909848, 1441.596168439879875, 170.5366494805969921 ) ) ;
#107888=CARTESIAN_POINT ( 'NONE',  ( -17.05703394869999912, 1440.440300860529987, 190.5363989150980046 ) ) ;
#107889=B_SPLINE_CURVE_WITH_KNOTS ( 'NONE', 3,
 ( #279, #34950, #19231, #18140, #85337, #8634, #69134, #33843, #52336, #86459, #103820, #76970, #95422, #27119, #61304, #18685, #53440, #68034, #102143, #25424, #79739, #11967, #38259, #3047, #80281 ),
 .UNSPECIFIED., .F., .F.,
 ( 4, 3, 3, 3, 3, 3, 3, 3, 4 ),
 ( 80.62324409590000585, 83.04996275482889700, 85.46931539243300335, 87.87555010193320015, 89.44943093207820084, 91.83314302553000630, 94.22747645563690355, 96.63741502969980957, 98.11410426366440163 ),
 .UNSPECIFIED. ) ;
#107890=CARTESIAN_POINT ( 'NONE',  ( -2.349669919091817327, 1449.655171934847658, 182.9923140666560641 ) ) ;
#107891=VERTEX_POINT ( 'NONE', #65713 ) ;
#107892=CARTESIAN_POINT ( 'NONE',  ( -26.35025291359999855, 1436.552346511289898, 136.8052071317979994 ) ) ;
#107895=CARTESIAN_POINT ( 'NONE',  ( -40.23884947949994029, 1448.346529241730877, 135.0415268541977412 ) ) ;
#107897=CARTESIAN_POINT ( 'NONE',  ( 0.06979919672880000037, 1408.910622945630166, 194.1218459596979926 ) ) ;
#107899=CARTESIAN_POINT ( 'NONE',  ( -1.113853250640000070, 1395.951956999929962, 198.1149994302979849 ) ) ;
#107903=CARTESIAN_POINT ( 'NONE',  ( 0.3125186096800000035, 1450.902146997000045, 181.9094756310980188 ) ) ;
#107905=CARTESIAN_POINT ( 'NONE',  ( 29.84438983998366623, 1466.863671349131209, 269.3606549350047885 ) ) ;
#107906=FACE_OUTER_BOUND ( 'NONE', #45326, .T. ) ;
#107908=FACE_OUTER_BOUND ( 'NONE', #100545, .T. ) ;
#107917=ORIENTED_EDGE ( 'NONE', *, *, #80504, .T. ) ;
#107919=B_SPLINE_CURVE_WITH_KNOTS ( 'NONE', 5,
 ( #100890, #77243, #1094, #58374, #35780, #69407 ),
 .UNSPECIFIED., .F., .F.,
 ( 6, 6 ),
 ( -88.78633455690000176, -19.55448171529999968 ),
 .UNSPECIFIED. ) ;
#107921=CARTESIAN_POINT ( 'NONE',  ( -23.22468639008607383, 1449.418569010514830, 216.9711829936322829 ) ) ;
#107924=B_SPLINE_CURVE_WITH_KNOTS ( 'NONE', 3,
 ( #56469, #21721, #107403, #81639, #30699, #98992, #90601, #5503, #97894, #107956, #54285, #45875, #80564, #29593, #80010, #37457, #71659, #54828, #106309, #88951, #63777, #7700, #101190, #74387, #58126, #84414, #83309, #65990, #7159, #101747, #24487, #100112, #108512, #33436, #48630, #91709, #41316, #74933, #50816, #6053, #23394, #110715, #49726 ),
 .UNSPECIFIED., .F., .F.,
 ( 4, 2, 2, 2, 2, 2, 2, 2, 2, 1, 1, 2, 2, 2, 2, 2, 2, 1, 1, 1, 2, 2, 2, 4 ),
 ( 0.000000000000000000, 0.007812500000093510269, 0.01562500000018702054, 0.02343750000028053254, 0.03125000000037404108, 0.06250000000091890384, 0.1250000000021675994, 0.1875000000034163228, 0.2187500000040124293, 0.2343750000042608417, 0.2421875000043403892, 0.2460937500043932358, 0.2500000000044461101, 0.3125000000050295879, 0.3750000000056131211, 0.4375000000061965988, 0.4687500000065056849, 0.4843750000068736128, 0.4921875000067835737, 0.4960937500067363892, 0.4980468750067104100, 0.5000000000066844308, 0.7500000000033421044, 1.000000000000000000 ),
 .UNSPECIFIED. ) ;
#107926=ADVANCED_FACE ( 'NONE', ( #64072 ), #90245, .F. ) ;
#107927=CARTESIAN_POINT ( 'NONE',  ( 13.79047275900000002, 1415.263254653229978, 197.3591164767980217 ) ) ;
#107929=CARTESIAN_POINT ( 'NONE',  ( 20.27230674349999973, 1410.542376202429978, 198.0398506171979989 ) ) ;
#107933=CARTESIAN_POINT ( 'NONE',  ( -0.3821804589910179906, 1506.433683733660018, 187.1424611576989889 ) ) ;
#107934=CARTESIAN_POINT ( 'NONE',  ( 24.33873747859275483, 1445.475447480255298, 214.1757831162466630 ) ) ;
#107940=CARTESIAN_POINT ( 'NONE',  ( -3.565775599929999817, 1474.072336424830155, 270.1349117941979898 ) ) ;
#107941=CARTESIAN_POINT ( 'NONE',  ( -2.500000000000000000, 1448.577607907360061, 183.6861132275980140 ) ) ;
#107942=CARTESIAN_POINT ( 'NONE',  ( -11.00428676220000135, 1425.778354413130046, 91.15517427569778874 ) ) ;
#107945=CARTESIAN_POINT ( 'NONE',  ( 11.60004869885203682, 1426.459365826449584, 139.0214960885385551 ) ) ;
#107946=CARTESIAN_POINT ( 'NONE',  ( -38.64637139473789773, 1443.913060387190171, 137.1864063576500143 ) ) ;
#107947=CARTESIAN_POINT ( 'NONE',  ( -2.136599176237389930, 1477.791721619980081, 183.3770592319010007 ) ) ;
#107950=CARTESIAN_POINT ( 'NONE',  ( 32.66611766053999588, 1440.913060383240008, 245.7919428914240143 ) ) ;
#107954=ORIENTED_EDGE ( 'NONE', *, *, #9321, .F. ) ;
#107955=CARTESIAN_POINT ( 'NONE',  ( 12.45478753333600430, 1442.762691980110276, 150.7713593675359505 ) ) ;
#107956=CARTESIAN_POINT ( 'NONE',  ( -19.13255955744318726, 1485.540540826345932, 189.6605840472149964 ) ) ;
#107957=CARTESIAN_POINT ( 'NONE',  ( -27.85007288970000161, 1509.193792693030218, 210.7874566006480279 ) ) ;
#107960=CARTESIAN_POINT ( 'NONE',  ( -17.45336505325400012, 1413.337826481620141, 225.8632813675029922 ) ) ;
#107964=DIRECTION ( 'NONE',  ( -0.000000000000000000, -0.000000000000000000, 1.000000000000000000 ) ) ;
#107965=FACE_OUTER_BOUND ( 'NONE', #14498, .T. ) ;
#107966=CARTESIAN_POINT ( 'NONE',  ( 2.441369149599999844, 1464.626822193330099, 236.1885516863980001 ) ) ;
#107969=CARTESIAN_POINT ( 'NONE',  ( -1.031182265530000253, 1450.900347381030087, 182.2739190327980054 ) ) ;
#107977=CARTESIAN_POINT ( 'NONE',  ( 33.91369278643569629, 1437.010534640189690, 136.5611839302279691 ) ) ;
#107983=CARTESIAN_POINT ( 'NONE',  ( 10.82176781693950041, 1409.290964846770066, 198.8079905577820057 ) ) ;
#107984=CARTESIAN_POINT ( 'NONE',  ( 18.52259990968499892, 1425.592936175037948, 225.5468824535050203 ) ) ;
#107986=CARTESIAN_POINT ( 'NONE',  ( -18.93959894380000009, 1463.213399808430040, 190.7720972619979705 ) ) ;
#107989=CARTESIAN_POINT ( 'NONE',  ( -2.321573235545089986, 1449.941122205050078, 183.5337604117939918 ) ) ;
#107992=CARTESIAN_POINT ( 'NONE',  ( 18.98967647182920260, 1456.684695305999867, 227.0095329493280190 ) ) ;
#107993=FACE_OUTER_BOUND ( 'NONE', #1171, .T. ) ;
#107994=CARTESIAN_POINT ( 'NONE',  ( 6.763640255447179445E-10, 1465.118916387369836, 238.1343321182859825 ) ) ;
#107995=CARTESIAN_POINT ( 'NONE',  ( -20.42135399285539776, 1502.078354143829984, 190.5572915927370161 ) ) ;
#108000=CARTESIAN_POINT ( 'NONE',  ( -46.16084778820400203, 1440.247791815949995, 266.9716791494209929 ) ) ;
#108001=CARTESIAN_POINT ( 'NONE',  ( -19.40520978109999817, 1426.254488764730240, 225.7391413128980275 ) ) ;
#108005=CARTESIAN_POINT ( 'NONE',  ( 1.289002268286620012, 1407.277490461829984, 222.1229423106349827 ) ) ;
#108011=CARTESIAN_POINT ( 'NONE',  ( 34.48978217459999485, 1438.727114832149937, 250.0021841848979989 ) ) ;
#108012=CARTESIAN_POINT ( 'NONE',  ( -26.42702185619999966, 1508.126183420129792, 201.6901284736979960 ) ) ;
#108013=CARTESIAN_POINT ( 'NONE',  ( -0.4938787171589999470, 1469.871322339429980, 182.4160331598980065 ) ) ;
#108016=CARTESIAN_POINT ( 'NONE',  ( -14.01630619230000008, 1418.416544456529891, 240.3753821333979772 ) ) ;
#108018=CARTESIAN_POINT ( 'NONE',  ( -12.12288233474179933, 1452.489720007740061, 149.6117171413690130 ) ) ;
#108019=CARTESIAN_POINT ( 'NONE',  ( 27.02655771539999918, 1451.969198393830084, 135.3521981671979972 ) ) ;
#108022=CARTESIAN_POINT ( 'NONE',  ( 3.152372269302069840E-05, 1408.236641047440116, 270.3925689135490416 ) ) ;
#108023=CARTESIAN_POINT ( 'NONE',  ( 16.14572133049080094, 1423.056865153649824, 229.1739396973900114 ) ) ;
#108028=CARTESIAN_POINT ( 'NONE',  ( -24.10619303449700013, 1410.858805650359955, 208.8787671924330027 ) ) ;
#108029=ORIENTED_EDGE ( 'NONE', *, *, #18277, .F. ) ;
#108032=CARTESIAN_POINT ( 'NONE',  ( -7.500890280090000140, 1498.345403818429986, 235.0614749778980013 ) ) ;
#108034=ORIENTED_EDGE ( 'NONE', *, *, #27629, .F. ) ;
#108036=CARTESIAN_POINT ( 'NONE',  ( 43.01404880660360419, 1452.566160834499897, 269.0485511200449764 ) ) ;
#108037=CARTESIAN_POINT ( 'NONE',  ( -11.87146819872990022, 1414.971390223319986, 220.8694174431610122 ) ) ;
#108038=CARTESIAN_POINT ( 'NONE',  ( 0.03302424225530000562, 1420.442649414729885, 183.2904121144979683 ) ) ;
#108040=ORIENTED_EDGE ( 'NONE', *, *, #44047, .F. ) ;
#108043=CARTESIAN_POINT ( 'NONE',  ( 13.45635499389495848, 1443.545252278519229, 187.9751403306488555 ) ) ;
#108045=EDGE_LOOP ( 'NONE', ( #90011, #105061, #95359 ) ) ;
#108050=CARTESIAN_POINT ( 'NONE',  ( 6.700690081702690648, 1452.679067133560011, 151.6942415867249849 ) ) ;
#108056=FACE_OUTER_BOUND ( 'NONE', #38029, .T. ) ;
#108061=CARTESIAN_POINT ( 'NONE',  ( 9.660544699540000835, 1432.353341358199941, 148.7316627034979888 ) ) ;
#108062=ORIENTED_EDGE ( 'NONE', *, *, #35497, .T. ) ;
#108063=CARTESIAN_POINT ( 'NONE',  ( 11.69744348346759999, 1415.090956648730071, 222.2791104206980037 ) ) ;
#108064=AXIS2_PLACEMENT_3D ( 'NONE', #31561, #24790, #99857 ) ;
#108065=CARTESIAN_POINT ( 'NONE',  ( 0.000000000000000000, 1395.913060387330006, 201.1218459616980283 ) ) ;
#108067=B_SPLINE_SURFACE_WITH_KNOTS ( 'NONE', 5, 5, ( 
 ( #80326, #89266, #12562, #97123, #12012, #37769 ),
 ( #62452, #64090, #46192, #19848, #10917, #45092 ),
 ( #88179, #28259, #71962, #98212, #55145, #106072 ),
 ( #70859, #20392, #70304, #87629, #54595, #79232 ),
 ( #54053, #80873, #29897, #11471, #29352, #13085 ),
 ( #46742, #89814, #96013, #63552, #4172, #38302 ) ),
 .UNSPECIFIED., .F., .F., .F.,
 ( 6, 6 ),
 ( 6, 6 ),
 ( 8.898447406460000764, 11.87289910710000029 ),
 ( 0.000000000000000000, 1.449276807229999964 ),
 .UNSPECIFIED. ) ;
#108074=CARTESIAN_POINT ( 'NONE',  ( -14.20177183849999913, 1416.825532263429977, 221.7377879684979973 ) ) ;
#108075=CARTESIAN_POINT ( 'NONE',  ( 11.78366509199999967, 1433.667675045369833, 150.8308889936979824 ) ) ;
#108076=CARTESIAN_POINT ( 'NONE',  ( 8.881784197000000993E-16, 1472.413060387330006, 271.1218459616979999 ) ) ;
#108084=CARTESIAN_POINT ( 'NONE',  ( -18.18090960190000160, 1410.471885800429845, 224.4285890788979998 ) ) ;
#108086=CARTESIAN_POINT ( 'NONE',  ( -0.9052398807790000834, 1424.182955095330044, 228.3523643996979899 ) ) ;
#108088=CARTESIAN_POINT ( 'NONE',  ( -9.868474398105202994, 1442.396259418528871, 184.8303838034649118 ) ) ;
#108093=CARTESIAN_POINT ( 'NONE',  ( -12.13987719790000064, 1415.426210663629945, 221.7061748208979850 ) ) ;
#108095=CARTESIAN_POINT ( 'NONE',  ( 0.2130788428118109978, 1455.621404727349955, 183.1409395639289812 ) ) ;
#108096=CARTESIAN_POINT ( 'NONE',  ( -14.95126388759999969, 1409.435170027230015, 210.7295747781880095 ) ) ;
#108097=CARTESIAN_POINT ( 'NONE',  ( -14.46594802229999921, 1415.931784856029935, 198.6496374484979981 ) ) ;
#108099=CARTESIAN_POINT ( 'NONE',  ( 11.87555827259999930, 1433.006750501450142, 147.9453531988980046 ) ) ;
#108100=CARTESIAN_POINT ( 'NONE',  ( -36.12226356709360431, 1436.069430019170113, 134.0999999971620014 ) ) ;
#108101=CARTESIAN_POINT ( 'NONE',  ( 5.510472668829999421, 1441.112718070130086, 184.8635310645979928 ) ) ;
#108107=CARTESIAN_POINT ( 'NONE',  ( -0.7975830076839999228, 1452.841034471829971, 183.3931114573979926 ) ) ;
#108108=CARTESIAN_POINT ( 'NONE',  ( 14.14834384894100161, 1509.157209502659953, 233.5082961851909999 ) ) ;
#108110=CARTESIAN_POINT ( 'NONE',  ( -19.46057851763744395, 1490.124445399882006, 189.4835821391595516 ) ) ;
#108112=CARTESIAN_POINT ( 'NONE',  ( 3.920881188560000119, 1439.701871974669984, 184.6839050870979975 ) ) ;
#108117=CARTESIAN_POINT ( 'NONE',  ( -27.01382282590000017, 1451.969727051930022, 134.9184453750980026 ) ) ;
#108118=CARTESIAN_POINT ( 'NONE',  ( -16.10184242527700249, 1409.577400629780186, 225.8122160371329983 ) ) ;
#108119=CARTESIAN_POINT ( 'NONE',  ( 0.4905038111388070332, 1417.380665725640029, 184.7693946335109842 ) ) ;
#108120=EDGE_LOOP ( 'NONE', ( #72086, #25938, #27163, #5578 ) ) ;
#108123=ADVANCED_FACE ( 'NONE', ( #95861 ), #103710, .F. ) ;
#108126=CARTESIAN_POINT ( 'NONE',  ( -0.1826741778924199922, 1419.424196826690149, 184.4619947973449996 ) ) ;
#108127=CARTESIAN_POINT ( 'NONE',  ( 1.037447696609999914, 1466.935166012330001, 235.3575387440980080 ) ) ;
#108129=CARTESIAN_POINT ( 'NONE',  ( 20.51925379220000067, 1409.629608526529864, 217.0260594629280035 ) ) ;
#108131=ADVANCED_FACE ( 'NONE', ( #95315 ), #87696, .T. ) ;
#108133=CARTESIAN_POINT ( 'NONE',  ( -17.34583796720000137, 1423.871196963929833, 227.2247444212979985 ) ) ;
#108135=CARTESIAN_POINT ( 'NONE',  ( -4.155669664704369382, 1439.704322410719897, 185.4969487652249995 ) ) ;
#108136=CARTESIAN_POINT ( 'NONE',  ( 27.12645382674940109, 1488.751129074109940, 207.9500232232510086 ) ) ;
#108143=CARTESIAN_POINT ( 'NONE',  ( -6.512854995241789346, 1485.815955151150092, 183.1454636990030167 ) ) ;
#108144=ORIENTED_EDGE ( 'NONE', *, *, #61343, .T. ) ;
#108147=CARTESIAN_POINT ( 'NONE',  ( -4.250056676659310639, 1441.348028558830038, 161.1060492004820048 ) ) ;
#108150=ORIENTED_EDGE ( 'NONE', *, *, #34092, .T. ) ;
#108153=ORIENTED_EDGE ( 'NONE', *, *, #108912, .F. ) ;
#108156=CARTESIAN_POINT ( 'NONE',  ( -11.61544799517619886, 1425.877524782230012, 142.6765297559990131 ) ) ;
#108157=CARTESIAN_POINT ( 'NONE',  ( 15.79075242492770315, 1409.464554496639948, 192.8587461545550070 ) ) ;
#108166=CARTESIAN_POINT ( 'NONE',  ( -40.27281773781609786, 1443.421733393530303, 137.0938879172039719 ) ) ;
#108170=ORIENTED_EDGE ( 'NONE', *, *, #107638, .F. ) ;
#108171=CARTESIAN_POINT ( 'NONE',  ( 10.04954308034672650, 1410.638657478467394, 229.7980651590800960 ) ) ;
#108172=CARTESIAN_POINT ( 'NONE',  ( 0.009922064841440000546, 1452.352461717429833, 183.2658050908980272 ) ) ;
#108174=CARTESIAN_POINT ( 'NONE',  ( -2.500000000000000000, 1439.615672362369878, 170.5246407198980023 ) ) ;
#108176=CARTESIAN_POINT ( 'NONE',  ( 38.81202641429280220, 1436.797832205790201, 135.3769915889319861 ) ) ;
#108179=CARTESIAN_POINT ( 'NONE',  ( 25.87197768239999718, 1438.599946763920116, 137.3989826761979884 ) ) ;
#108186=CARTESIAN_POINT ( 'NONE',  ( 38.69786524538719874, 1440.913060387330006, 265.8278627617990537 ) ) ;
#108187=B_SPLINE_CURVE_WITH_KNOTS ( 'NONE', 3,
 ( #90093, #48682, #13376, #107451, #4992, #31852, #29644, #5559 ),
 .UNSPECIFIED., .F., .F.,
 ( 4, 2, 2, 4 ),
 ( -0.07898079781686900835, -0.04381124047686119766, -0.01845156514537110715, 0.000000000000000000 ),
 .UNSPECIFIED. ) ;
#108188=CARTESIAN_POINT ( 'NONE',  ( -0.0002161185356587633102, 1452.672516883277240, 153.3651468782901759 ) ) ;
#108189=EDGE_LOOP ( 'NONE', ( #3972, #64088, #103934, #84299 ) ) ;
#108190=CARTESIAN_POINT ( 'NONE',  ( -0.04116744988597149935, 1450.911622788300065, 181.8848909658740070 ) ) ;
#108191=ADVANCED_FACE ( 'NONE', ( #61738 ), #57920, .F. ) ;
#108192=CARTESIAN_POINT ( 'NONE',  ( -15.42891520709999931, 1409.953600697129787, 191.2302129608980010 ) ) ;
#108193=CARTESIAN_POINT ( 'NONE',  ( 0.000000000000000000, 1414.913060387329779, 209.1218459616979999 ) ) ;
#108196=FACE_OUTER_BOUND ( 'NONE', #38043, .T. ) ;
#108198=CARTESIAN_POINT ( 'NONE',  ( -1.517310980229999995, 1507.186118473530087, 180.8246499581979947 ) ) ;
#108199=CARTESIAN_POINT ( 'NONE',  ( -11.94157476580000043, 1433.614967702190143, 147.1502177932979976 ) ) ;
#108201=CARTESIAN_POINT ( 'NONE',  ( 12.32422840039999912, 1461.784851115730135, 233.7517049971980043 ) ) ;
#108202=CARTESIAN_POINT ( 'NONE',  ( -23.98820069242849939, 1430.810317484149891, 210.9021713681929953 ) ) ;
#108209=CARTESIAN_POINT ( 'NONE',  ( -0.07873616178531450682, 1508.524200534259990, 180.2296851813550234 ) ) ;
#108212=CARTESIAN_POINT ( 'NONE',  ( 18.65451744259999955, 1507.632629720729938, 188.5326157633979847 ) ) ;
#108213=CARTESIAN_POINT ( 'NONE',  ( -11.60004869885203682, 1426.445093601214467, 138.8745978379924679 ) ) ;
#108216=CARTESIAN_POINT ( 'NONE',  ( -20.15452302159999931, 1507.845791376729949, 228.9024215066979764 ) ) ;
#108218=CARTESIAN_POINT ( 'NONE',  ( -10.96178248360000040, 1431.789698015990098, 151.7500217919979661 ) ) ;
#108225=CARTESIAN_POINT ( 'NONE',  ( -19.65613647119999641, 1457.446755667530169, 225.8342101607980226 ) ) ;
#108230=CARTESIAN_POINT ( 'NONE',  ( 6.204532493290000339, 1406.059425862230000, 267.5209521470980008 ) ) ;
#108231=ADVANCED_FACE ( 'NONE', ( #85007, #26203 ), #18350, .T. ) ;
#108232=CARTESIAN_POINT ( 'NONE',  ( -0.3258850517759999676, 1410.291732226329941, 185.0570438166979841 ) ) ;
#108233=B_SPLINE_CURVE_WITH_KNOTS ( 'NONE', 3,
 ( #26804, #79430, #45289, #70502, #71055, #105178, #88374, #87842, #10563, #69391, #27354, #103502, #54248, #1078, #78887, #28469, #62098, #95117, #44175, #18381, #11130, #2193 ),
 .UNSPECIFIED., .F., .F.,
 ( 4, 2, 2, 1, 1, 1, 1, 2, 2, 2, 2, 2, 4 ),
 ( 0.000000000000000000, 0.2499999999997699618, 0.3749999999996527222, 0.4374999999995941025, 0.4687499999995649591, 0.4843749999995503597, 0.4921874999995429767, 0.4960937499995419775, 0.4999999999995410338, 0.7499999999997783995, 0.8124999999998353539, 0.8749999999998923084, 1.000000000000000000 ),
 .UNSPECIFIED. ) ;
#108235=CARTESIAN_POINT ( 'NONE',  ( 24.22202933080170340, 1436.664598046718766, 213.2981740296385453 ) ) ;
#108236=AXIS2_PLACEMENT_3D ( 'NONE', #32518, #109234, #67239 ) ;
#108237=CARTESIAN_POINT ( 'NONE',  ( -24.43498997089999847, 1452.059775937329960, 135.9951607580979953 ) ) ;
#108238=CARTESIAN_POINT ( 'NONE',  ( 27.44018068100522356, 1508.035990152466638, 213.3629281564213898 ) ) ;
#108240=CARTESIAN_POINT ( 'NONE',  ( -1.962873838212560118, 1450.341737221240010, 154.5188792923449910 ) ) ;
#108241=CARTESIAN_POINT ( 'NONE',  ( -12.36661650740000162, 1446.466068106850116, 187.6273874412979978 ) ) ;
#108242=CARTESIAN_POINT ( 'NONE',  ( -19.62491598524822578, 1486.234197820471536, 189.9488111625408351 ) ) ;
#108244=CARTESIAN_POINT ( 'NONE',  ( -14.31665923842830068, 1416.051481378920016, 221.2469180764289831 ) ) ;
#108247=CARTESIAN_POINT ( 'NONE',  ( -27.38276294334009719, 1507.983226544079798, 210.8770510937970073 ) ) ;
#108248=CARTESIAN_POINT ( 'NONE',  ( 2.499999942879999715, 1440.188278801189881, 170.5317984358979970 ) ) ;
#108249=CARTESIAN_POINT ( 'NONE',  ( -3.401812130889999786, 1475.226509619029912, 269.4945985741979939 ) ) ;
#108250=CARTESIAN_POINT ( 'NONE',  ( -4.223240706370930297, 1446.235532200490070, 167.1955850464350135 ) ) ;
#108251=CARTESIAN_POINT ( 'NONE',  ( -17.70270299129999714, 1414.019030144130056, 193.3444296426980316 ) ) ;
#108252=EDGE_CURVE ( 'NONE', #86845, #46740, #48373, .T. ) ;
#108259=CARTESIAN_POINT ( 'NONE',  ( -18.89905695062199698, 1416.828039266840278, 207.5749027128360069 ) ) ;
#108260=AXIS2_PLACEMENT_3D ( 'NONE', #108193, #13564, #12490 ) ;
#108262=CARTESIAN_POINT ( 'NONE',  ( -7.075873090581220301E-12, 1395.913060387330006, 220.1216245177919859 ) ) ;
#108263=( BOUNDED_CURVE ( )  B_SPLINE_CURVE ( 3, ( #7017, #68598, #26566, #51791 ),
 .UNSPECIFIED., .F., .T. ) 
 B_SPLINE_CURVE_WITH_KNOTS ( ( 4, 4 ),
 ( 1.036083218751772561, 2.105411800329895833 ),
 .UNSPECIFIED. ) 
 CURVE ( )  GEOMETRIC_REPRESENTATION_ITEM ( )  RATIONAL_B_SPLINE_CURVE ( ( 1.000000000000000000, 0.9069598260854428995, 0.9069598260854428995, 1.000000000000000000 ) ) 
 REPRESENTATION_ITEM ( '' )  );
#108266=CARTESIAN_POINT ( 'NONE',  ( -35.13956213160000175, 1419.958835960429951, 269.8639799881980252 ) ) ;
#108268=CARTESIAN_POINT ( 'NONE',  ( -2.276495432953816511, 1410.370859958793062, 232.7304497416644438 ) ) ;
#108280=CARTESIAN_POINT ( 'NONE',  ( -9.584198994920001269, 1428.531551829730233, 147.0197059986979866 ) ) ;
#108284=CARTESIAN_POINT ( 'NONE',  ( 20.51030872011919826, 1508.877646971749982, 228.8223684417449988 ) ) ;
#108287=ORIENTED_EDGE ( 'NONE', *, *, #20636, .F. ) ;
#108289=CARTESIAN_POINT ( 'NONE',  ( -11.56322555989999934, 1396.494206780630066, 212.6176595098179973 ) ) ;
#108290=CARTESIAN_POINT ( 'NONE',  ( -19.37964200209999888, 1409.589812403130054, 219.8414950337979974 ) ) ;
#108292=CARTESIAN_POINT ( 'NONE',  ( -12.97512972099614892, 1444.891494972908504, 169.4251994755254884 ) ) ;
#108293=CARTESIAN_POINT ( 'NONE',  ( -0.04548916784355099691, 1416.835419214280137, 227.2860346676060033 ) ) ;
#108294=LINE ( 'NONE', #83096, #51644 ) ;
#108296=CARTESIAN_POINT ( 'NONE',  ( 17.35196363740000081, 1421.690952144829907, 226.5939839563979774 ) ) ;
#108298=CARTESIAN_POINT ( 'NONE',  ( 1.616461792820000021, 1449.240018237009963, 183.6572643142980326 ) ) ;
#108301=CARTESIAN_POINT ( 'NONE',  ( 11.07060849806599911, 1396.299654554839890, 208.8974423235020197 ) ) ;
#108303=CARTESIAN_POINT ( 'NONE',  ( 1.556584322539999787, 1415.163755998629995, 191.2532905271980042 ) ) ;
#108304=CARTESIAN_POINT ( 'NONE',  ( 10.83255468690000001, 1424.906521154930033, 145.5564295056979915 ) ) ;
#108305=CARTESIAN_POINT ( 'NONE',  ( 17.11714618750000128, 1443.086052842849995, 162.7561046190980107 ) ) ;
#108306=VERTEX_POINT ( 'NONE', #79943 ) ;
#108307=CARTESIAN_POINT ( 'NONE',  ( 12.93434948142389906, 1435.679596294389967, 150.6798643324129898 ) ) ;
#108308=CARTESIAN_POINT ( 'NONE',  ( 2.062938842272421525, 1450.143278206232480, 181.9957652172806775 ) ) ;
#108311=ORIENTED_EDGE ( 'NONE', *, *, #110159, .F. ) ;
#108313=CARTESIAN_POINT ( 'NONE',  ( -15.74154650769999897, 1459.394320623929843, 230.7248345380980084 ) ) ;
#108318=ORIENTED_EDGE ( 'NONE', *, *, #33237, .T. ) ;
#108320=CARTESIAN_POINT ( 'NONE',  ( 2.500000000000000000, 1448.308226215490095, 164.1023061046490170 ) ) ;
#108325=ORIENTED_EDGE ( 'NONE', *, *, #15978, .F. ) ;
#108327=CARTESIAN_POINT ( 'NONE',  ( -21.39772452180000073, 1509.704964747930035, 229.7894198983979948 ) ) ;
#108328=B_SPLINE_SURFACE_WITH_KNOTS ( 'NONE', 5, 5, ( 
 ( #45392, #104714, #46492, #80625, #62763, #88477 ),
 ( #28007, #38605, #96880, #27453, #38067, #72244 ),
 ( #106371, #29658, #61637, #63844, #20149, #45931 ),
 ( #23458, #100708, #40264, #30200, #65492, #90661 ),
 ( #7224, #14501, #64391, #98512, #47575, #57652 ),
 ( #23989, #83920, #83362, #21780, #13944, #32425 ),
 ( #6108, #39721, #73885, #91220, #66604, #91764 ),
 ( #100173, #5570, #22885, #66050, #6662, #99602 ),
 ( #73328, #15040, #108013, #58185, #57095, #72785 ),
 ( #107463, #48691, #49239, #31309, #74447, #48134 ),
 ( #106912, #82815, #82272, #92313, #5007, #55982 ),
 ( #90105, #108573, #31862, #40815, #74994, #15584 ) ),
 .UNSPECIFIED., .F., .F., .F.,
 ( 6, 3, 3, 6 ),
 ( 6, 6 ),
 ( 31.69285121669999938, 50.14584306709999595, 68.35602240260000428, 108.8243570000000062 ),
 ( -9.967974889959999953E-09, 15.21005427680000111 ),
 .UNSPECIFIED. ) ;
#108329=CARTESIAN_POINT ( 'NONE',  ( -39.55833958944460704, 1430.592406935262488, 269.6025355008150655 ) ) ;
#108330=CARTESIAN_POINT ( 'NONE',  ( -2.069513320929999622, 1408.985329384930083, 231.7586132267979906 ) ) ;
#108331=CARTESIAN_POINT ( 'NONE',  ( 0.2465388108663439937, 1414.971349104640012, 225.7948585416679634 ) ) ;
#108332=ORIENTED_EDGE ( 'NONE', *, *, #94245, .F. ) ;
#108333=CARTESIAN_POINT ( 'NONE',  ( 24.57684123230000139, 1440.965828712510074, 212.8359049822580289 ) ) ;
#108334=CARTESIAN_POINT ( 'NONE',  ( -29.65916216564760077, 1440.913060386779989, 237.2382442218989809 ) ) ;
#108336=CARTESIAN_POINT ( 'NONE',  ( -0.1267477471548290047, 1466.039099894230048, 235.8527109107560022 ) ) ;
#108338=CARTESIAN_POINT ( 'NONE',  ( 13.03173489774369997, 1411.479542611389888, 269.8789902196239723 ) ) ;
#108340=CARTESIAN_POINT ( 'NONE',  ( 22.81565299040000028, 1409.709731146529975, 209.0774165718939912 ) ) ;
#108342=FACE_OUTER_BOUND ( 'NONE', #4450, .T. ) ;
#108344=CIRCLE ( 'NONE', #17103, 0.5000000000000000000 ) ;
#108347=CARTESIAN_POINT ( 'NONE',  ( -2.864433789270523167, 1447.807611701459109, 154.7916386383528504 ) ) ;
#108350=CARTESIAN_POINT ( 'NONE',  ( 10.97212503029999908, 1432.504868931790043, 151.7700489660979883 ) ) ;
#108354=CARTESIAN_POINT ( 'NONE',  ( 18.89942250099999654, 1416.835808384130132, 210.6687153374880097 ) ) ;
#108355=CARTESIAN_POINT ( 'NONE',  ( -17.17007368362429531, 1414.941152333210539, 207.7552173661434551 ) ) ;
#108357=FACE_OUTER_BOUND ( 'NONE', #5543, .T. ) ;
#108358=CARTESIAN_POINT ( 'NONE',  ( -5.411774941350000034, 1435.306181909920042, 154.6725816278979835 ) ) ;
#108361=ADVANCED_FACE ( 'NONE', ( #87236 ), #3259, .F. ) ;
#108370=CARTESIAN_POINT ( 'NONE',  ( -27.02655812420177028, 1451.969196582628911, 135.3522152283978528 ) ) ;
#108372=CARTESIAN_POINT ( 'NONE',  ( 7.151890254928414237, 1438.987468099824355, 154.0970018937933332 ) ) ;
#108375=CARTESIAN_POINT ( 'NONE',  ( 6.975311473106522442, 1416.765600848013037, 231.0738521692657059 ) ) ;
#108378=CARTESIAN_POINT ( 'NONE',  ( -18.92517849950000297, 1425.859884652129949, 225.1369558184979951 ) ) ;
#108381=CARTESIAN_POINT ( 'NONE',  ( 20.15502270700000054, 1507.862952647929887, 189.3407284623980047 ) ) ;
#108384=CARTESIAN_POINT ( 'NONE',  ( -31.28589133189229443, 1461.258894143585167, 269.4849877309756607 ) ) ;
#108385=VERTEX_POINT ( 'NONE', #3816 ) ;
#108387=EDGE_CURVE ( 'NONE', #7904, #21837, #73382, .T. ) ;
#108388=CARTESIAN_POINT ( 'NONE',  ( -33.30421208489385521, 1417.542625019127172, 269.2880441342906011 ) ) ;
#108390=CARTESIAN_POINT ( 'NONE',  ( -0.9766393796380001824, 1453.313060387329870, 229.7750655478980093 ) ) ;
#108392=CARTESIAN_POINT ( 'NONE',  ( -12.55703987801026500, 1442.777179238205917, 186.0009298388953880 ) ) ;
#108396=CARTESIAN_POINT ( 'NONE',  ( 24.45953054869999832, 1435.631735371460081, 137.6709130696980026 ) ) ;
#108397=CARTESIAN_POINT ( 'NONE',  ( -12.72569297477883588, 1442.818307999958733, 169.4573488157998611 ) ) ;
#108398=CARTESIAN_POINT ( 'NONE',  ( -15.06903107870000191, 1410.389868148830146, 226.7125060204980116 ) ) ;
#108402=CARTESIAN_POINT ( 'NONE',  ( -3.805207261640000116, 1409.045941153030071, 230.7650822874980179 ) ) ;
#108405=CARTESIAN_POINT ( 'NONE',  ( 16.06427069504690053, 1414.913060387399810, 208.9262394168359833 ) ) ;
#108408=CARTESIAN_POINT ( 'NONE',  ( -25.51518049010000055, 1444.285382571919854, 220.8700590728979876 ) ) ;
#108410=CARTESIAN_POINT ( 'NONE',  ( -11.46969010090000118, 1433.199005582570180, 151.2954870453980050 ) ) ;
#108411=ADVANCED_FACE ( 'NONE', ( #99470 ), #33012, .F. ) ;
#108414=CARTESIAN_POINT ( 'NONE',  ( -26.67861085519999875, 1438.479473329630082, 136.9888825721979799 ) ) ;
#108415=CARTESIAN_POINT ( 'NONE',  ( -24.46932507910000254, 1440.032561122739935, 210.9836422549680037 ) ) ;
#108417=CARTESIAN_POINT ( 'NONE',  ( 1.521080599399999844, 1450.730010003210054, 182.2924144091979883 ) ) ;
#108419=ADVANCED_FACE ( 'NONE', ( #106779 ), #56398, .F. ) ;
#108420=CARTESIAN_POINT ( 'NONE',  ( -11.05120362203290618, 1509.424098794511337, 237.0121822441638813 ) ) ;
#108421=CARTESIAN_POINT ( 'NONE',  ( -2.060856689691449839E-09, 1413.853476841760084, 248.1683309011359881 ) ) ;
#108424=CIRCLE ( 'NONE', #60164, 2.000000000000000000 ) ;
#108425=CARTESIAN_POINT ( 'NONE',  ( -11.86598650706779878, 1432.328056081479872, 149.9824201572170352 ) ) ;
#108427=CARTESIAN_POINT ( 'NONE',  ( -7.595213676849999374, 1473.705021973730027, 270.1248737330980134 ) ) ;
#108428=CARTESIAN_POINT ( 'NONE',  ( -14.87168881317970026, 1430.147188212150240, 221.8136313441650032 ) ) ;
#108429=CYLINDRICAL_SURFACE ( 'NONE', #11103, 10.00000000000000000 ) ;
#108430=CARTESIAN_POINT ( 'NONE',  ( 34.46379809770260039, 1450.419497442319880, 136.2296061301330212 ) ) ;
#108437=CARTESIAN_POINT ( 'NONE',  ( -33.64184985774720360, 1416.594321794520056, 267.0652993242159710 ) ) ;
#108438=ORIENTED_EDGE ( 'NONE', *, *, #78685, .T. ) ;
#108440=EDGE_CURVE ( 'NONE', #107891, #88507, #50939, .T. ) ;
#108441=EDGE_LOOP ( 'NONE', ( #36551, #52103, #26608, #23390 ) ) ;
#108442=ORIENTED_EDGE ( 'NONE', *, *, #32346, .T. ) ;
#108444=CARTESIAN_POINT ( 'NONE',  ( 4.608371281445468703, 1423.726610470979267, 183.8391095067188985 ) ) ;
#108445=CARTESIAN_POINT ( 'NONE',  ( -2.500000000000000000, 1436.878463555260169, 183.6520988947980015 ) ) ;
#108449=CARTESIAN_POINT ( 'NONE',  ( -17.25278045389999804, 1455.455490790330032, 189.9113160770979789 ) ) ;
#108451=CARTESIAN_POINT ( 'NONE',  ( -2.359913115097718617, 1449.630106320913455, 182.9978952858132004 ) ) ;
#108453=CARTESIAN_POINT ( 'NONE',  ( -26.07187536489999857, 1435.414138736239920, 135.5217793413980019 ) ) ;
#108455=CARTESIAN_POINT ( 'NONE',  ( -41.63813745289505164, 1444.512220545661876, 135.5979520083818954 ) ) ;
#108457=CARTESIAN_POINT ( 'NONE',  ( -40.61004888632240295, 1425.241059834939961, 269.7704499877880266 ) ) ;
#108459=CARTESIAN_POINT ( 'NONE',  ( -1.244837129730000047, 1397.637433091830189, 196.1147955250980033 ) ) ;
#108464=CARTESIAN_POINT ( 'NONE',  ( 1.704192342800000001E-13, 1475.048391919030109, 269.6500679772980220 ) ) ;
#108466=CARTESIAN_POINT ( 'NONE',  ( -14.58761689442209963, 1436.245193537610021, 149.8743049802889971 ) ) ;
#108467=CARTESIAN_POINT ( 'NONE',  ( -2.105916269280000197, 1485.584842596029830, 182.5101088919979873 ) ) ;
#108471=CARTESIAN_POINT ( 'NONE',  ( -14.42407037529999947, 1430.147381752329920, 222.2644859324980189 ) ) ;
#108472=CARTESIAN_POINT ( 'NONE',  ( 3.885349673800238879, 1440.907261985867081, 156.3247486698534487 ) ) ;
#108477=CARTESIAN_POINT ( 'NONE',  ( -36.37832868406120213, 1451.642701156830071, 135.3761648280290046 ) ) ;
#108479=CARTESIAN_POINT ( 'NONE',  ( -20.69466133717958911, 1455.350803762641135, 223.8685399355039465 ) ) ;
#108483=CARTESIAN_POINT ( 'NONE',  ( 12.92073010750949891, 1435.120627881940209, 150.2915359750790003 ) ) ;
#108484=CARTESIAN_POINT ( 'NONE',  ( 13.97021087459999933, 1416.254459046630018, 196.4665394535979885 ) ) ;
#108486=DIRECTION ( 'NONE',  ( 0.9483721503360844629, -0.1343667288060120535, 0.2872905265700261279 ) ) ;
#108487=CARTESIAN_POINT ( 'NONE',  ( 3.503183429743535804, 1450.836852080426297, 184.0621120680351339 ) ) ;
#108490=CARTESIAN_POINT ( 'NONE',  ( 23.79381763197114097, 1448.079399027135651, 216.0042285759331833 ) ) ;
#108491=CARTESIAN_POINT ( 'NONE',  ( -12.00000000000000000, 1443.913060387330006, 150.5878346084980137 ) ) ;
#108498=CARTESIAN_POINT ( 'NONE',  ( 1.366628593997903707, 1414.941152333447462, 191.9517722785298588 ) ) ;
#108499=CARTESIAN_POINT ( 'NONE',  ( -3.721063415729999695E-09, 1475.837061091930082, 266.9611530633980010 ) ) ;
#108500=CARTESIAN_POINT ( 'NONE',  ( 11.44982798326090290, 1425.806312135371854, 139.0983210244855854 ) ) ;
#108502=CARTESIAN_POINT ( 'NONE',  ( 17.98447767965197741, 1424.110086477602408, 225.5366282599816543 ) ) ;
#108505=CARTESIAN_POINT ( 'NONE',  ( 31.79362791131370258, 1440.913060383409857, 243.5716590067270033 ) ) ;
#108508=CARTESIAN_POINT ( 'NONE',  ( 13.11885828660000008, 1419.893985557330097, 221.7273098061980079 ) ) ;
#108512=CARTESIAN_POINT ( 'NONE',  ( -19.67602081376940859, 1485.246767906123978, 190.3296067428275649 ) ) ;
#108513=FACE_OUTER_BOUND ( 'NONE', #41142, .T. ) ;
#108516=CARTESIAN_POINT ( 'NONE',  ( -11.73701141503820011, 1426.696005490819971, 144.1689084034089774 ) ) ;
#108521=CARTESIAN_POINT ( 'NONE',  ( -0.2612772979118159755, 1416.851343897360039, 227.4677505453099968 ) ) ;
#108532=ORIENTED_EDGE ( 'NONE', *, *, #4133, .T. ) ;
#108542=CARTESIAN_POINT ( 'NONE',  ( 10.58919714376239973, 1409.282843299900151, 198.5624303964659987 ) ) ;
#108543=CARTESIAN_POINT ( 'NONE',  ( 18.80368963479999778, 1425.915429421829913, 225.1658117488979940 ) ) ;
#108546=CARTESIAN_POINT ( 'NONE',  ( -4.223640783000890409, 1441.596330317800039, 170.5493994362460057 ) ) ;
#108547=CIRCLE ( 'NONE', #28062, 2.000000000000068390 ) ;
#108550=EDGE_LOOP ( 'NONE', ( #21739, #43527, #793, #31719 ) ) ;
#108551=CARTESIAN_POINT ( 'NONE',  ( -1.623075365390000080, 1428.602351821930142, 149.4837496357980058 ) ) ;
#108552=CARTESIAN_POINT ( 'NONE',  ( 18.61188344111999982, 1458.579614889230015, 227.5056110255299870 ) ) ;
#108553=CARTESIAN_POINT ( 'NONE',  ( -11.39739833580000017, 1434.677645552710146, 151.4902371962980112 ) ) ;
#108555=CARTESIAN_POINT ( 'NONE',  ( -4.219438644781110526, 1441.595895916910195, 183.5288106640859951 ) ) ;
#108556=CARTESIAN_POINT ( 'NONE',  ( -24.92720798968933238, 1436.178265573613999, 137.8894290697291751 ) ) ;
#108558=CARTESIAN_POINT ( 'NONE',  ( -0.5561591756040000778, 1484.827948844329967, 181.8894219878979754 ) ) ;
#108560=CARTESIAN_POINT ( 'NONE',  ( -45.85227038866229776, 1440.469603780929901, 268.7564394150250564 ) ) ;
#108561=CARTESIAN_POINT ( 'NONE',  ( -19.04437315719999901, 1425.784752839030034, 226.3805134473980161 ) ) ;
#108562=CARTESIAN_POINT ( 'NONE',  ( -19.99778532869999736, 1488.358619900530130, 191.8244647984979849 ) ) ;
#108564=CARTESIAN_POINT ( 'NONE',  ( -25.07511837043467295, 1507.939514509590708, 198.1595777679482921 ) ) ;
#108568=CARTESIAN_POINT ( 'NONE',  ( 8.690383195619999057, 1424.104242789630007, 112.3001073638979932 ) ) ;
#108570=EDGE_LOOP ( 'NONE', ( #44178, #71977, #32451, #36916 ) ) ;
#108571=CARTESIAN_POINT ( 'NONE',  ( 14.01630619149999823, 1418.416544456529891, 240.3753821261979908 ) ) ;
#108572=CARTESIAN_POINT ( 'NONE',  ( -27.30475511710000092, 1508.128822472029924, 204.4091660346579999 ) ) ;
#108573=CARTESIAN_POINT ( 'NONE',  ( 0.5480496121420000977, 1452.697021778130193, 183.2754429902979894 ) ) ;
#108574=LINE ( 'NONE', #101246, #32024 ) ;
#108576=EDGE_CURVE ( 'NONE', #33227, #101013, #48375, .T. ) ;
#108577=CARTESIAN_POINT ( 'NONE',  ( -2.713387635329040037, 1419.520833911499949, 186.1633376940620224 ) ) ;
#108578=CARTESIAN_POINT ( 'NONE',  ( -19.57999073310000071, 1422.088355595230269, 238.2202611127979708 ) ) ;
#108580=CARTESIAN_POINT ( 'NONE',  ( -22.49711446700899842, 1452.127443838799991, 139.6705065661170124 ) ) ;
#108582=CARTESIAN_POINT ( 'NONE',  ( -18.89942250099999654, 1416.835808384130132, 207.5749765859080185 ) ) ;
#108584=CARTESIAN_POINT ( 'NONE',  ( -2.500000000000000000, 1419.382782049920024, 144.1108465772580018 ) ) ;
#108585=CARTESIAN_POINT ( 'NONE',  ( 2.603400736049609843E-05, 1407.928373405780121, 270.2926942668629522 ) ) ;
#108586=CARTESIAN_POINT ( 'NONE',  ( 15.52525468725849933, 1421.896024094239920, 227.9304414622129968 ) ) ;
#108591=CARTESIAN_POINT ( 'NONE',  ( -23.03704750979090221, 1409.747334528499778, 208.9847852389330001 ) ) ;
#108596=CARTESIAN_POINT ( 'NONE',  ( -2.896892187767880156, 1484.263391075600111, 183.3160938869699805 ) ) ;
#108597=CARTESIAN_POINT ( 'NONE',  ( -21.87294976469999952, 1415.845546353629970, 216.4166232744080105 ) ) ;
#108599=CARTESIAN_POINT ( 'NONE',  ( 46.01111071544060138, 1442.797791010789979, 266.6782117715599725 ) ) ;
#108606=CARTESIAN_POINT ( 'NONE',  ( 13.47882082157883232, 1444.213219860304434, 187.9195826302412229 ) ) ;
#108607=ORIENTED_EDGE ( 'NONE', *, *, #61935, .T. ) ;
#108609=CARTESIAN_POINT ( 'NONE',  ( 26.83363330979009831, 1450.700274826909890, 136.4563300885299668 ) ) ;
#108612=CARTESIAN_POINT ( 'NONE',  ( -1.681286490166120328E-05, 1409.206633381659913, 270.3713656704379673 ) ) ;
#108617=CARTESIAN_POINT ( 'NONE',  ( -13.13384863970290084, 1434.838379660660166, 149.0654039179239874 ) ) ;
#108624=CARTESIAN_POINT ( 'NONE',  ( 17.83186622659999898, 1434.542072767689888, 214.3676144197979738 ) ) ;
#108625=CARTESIAN_POINT ( 'NONE',  ( 0.000000000000000000, 0.000000000000000000, 137.0999999980979851 ) ) ;
#108629=CARTESIAN_POINT ( 'NONE',  ( 7.114141310732409629, 1427.484008838899626, 137.0999999980979567 ) ) ;
#108631=EDGE_LOOP ( 'NONE', ( #2871, #108144, #88406, #107882 ) ) ;
#108633=CARTESIAN_POINT ( 'NONE',  ( -3.034707026709789979, 1440.440247136690004, 157.2489849372729793 ) ) ;
#108635=CARTESIAN_POINT ( 'NONE',  ( 11.92075754520000075, 1433.502514733529779, 150.2427968400980092 ) ) ;
#108636=CARTESIAN_POINT ( 'NONE',  ( 6.832964021560000489, 1472.413060387330006, 271.1218459616979999 ) ) ;
#108642=CARTESIAN_POINT ( 'NONE',  ( 16.93584435349999850, 1422.112459457830028, 226.8792436412979896 ) ) ;
#108645=CARTESIAN_POINT ( 'NONE',  ( -17.85795099530000130, 1410.033484215229919, 224.6176101541979904 ) ) ;
#108647=CARTESIAN_POINT ( 'NONE',  ( 20.39632456690000240, 1508.015821253330159, 189.6607555625980126 ) ) ;
#108653=CARTESIAN_POINT ( 'NONE',  ( -11.61528297169999924, 1414.971352895729979, 221.0857775958980085 ) ) ;
#108654=CARTESIAN_POINT ( 'NONE',  ( 0.1719439918013369872, 1479.188729932770229, 182.1292389662029905 ) ) ;
#108657=CARTESIAN_POINT ( 'NONE',  ( -17.11714625305222981, 1444.740067931810927, 162.7561045841209193 ) ) ;
#108659=CARTESIAN_POINT ( 'NONE',  ( 12.40405681299999863, 1434.420100264380153, 149.4777463942980091 ) ) ;
#108660=CARTESIAN_POINT ( 'NONE',  ( -41.18215094384600405, 1440.963619929689912, 134.0999999980659823 ) ) ;
#108661=CARTESIAN_POINT ( 'NONE',  ( 5.605776958220000772, 1441.571049125840091, 184.4074510981980097 ) ) ;
#108664=CARTESIAN_POINT ( 'NONE',  ( 13.02322703161950024, 1416.825784015089994, 221.6328457863429833 ) ) ;
#108670=CARTESIAN_POINT ( 'NONE',  ( -22.52609270479999992, 1509.699688878229836, 208.9176257130850161 ) ) ;
#108672=CARTESIAN_POINT ( 'NONE',  ( 2.988808142889999520, 1436.945273251980097, 184.3538548285980028 ) ) ;
#108677=CARTESIAN_POINT ( 'NONE',  ( -29.03159036203449972, 1509.651961618060113, 208.6837609952029879 ) ) ;
#108678=CARTESIAN_POINT ( 'NONE',  ( -16.03542055943749745, 1410.434532276399977, 226.6320020206029824 ) ) ;
#108686=CARTESIAN_POINT ( 'NONE',  ( 1.963370033230000145, 1464.924280339329925, 237.5709149063980021 ) ) ;
#108688=CARTESIAN_POINT ( 'NONE',  ( 22.39508854780000036, 1411.055311095129809, 215.1301064521879880 ) ) ;
#108689=CARTESIAN_POINT ( 'NONE',  ( -2.419942311379319921, 1417.229693625109803, 186.1923575038539980 ) ) ;
#108690=CARTESIAN_POINT ( 'NONE',  ( -17.74698610909999985, 1424.418662807230021, 227.3573823931980087 ) ) ;
#108695=B_SPLINE_CURVE_WITH_KNOTS ( 'NONE', 3,
 ( #42025, #34166, #16778, #76722, #76173, #68352, #102458 ),
 .UNSPECIFIED., .F., .F.,
 ( 4, 3, 4 ),
 ( -157.7301682610000171, -100.4763595781870009, -30.40177460629999473 ),
 .UNSPECIFIED. ) ;
#108699=CARTESIAN_POINT ( 'NONE',  ( -4.461987601309290064, 1485.816428176619866, 182.7387781610549951 ) ) ;
#108702=FACE_OUTER_BOUND ( 'NONE', #42468, .T. ) ;
#108704=ORIENTED_EDGE ( 'NONE', *, *, #3633, .F. ) ;
#108705=ORIENTED_EDGE ( 'NONE', *, *, #76033, .F. ) ;
#108707=ORIENTED_EDGE ( 'NONE', *, *, #88133, .F. ) ;
#108711=CARTESIAN_POINT ( 'NONE',  ( -11.15639751152448511, 1425.159686727654162, 144.2660521923811530 ) ) ;
#108712=CARTESIAN_POINT ( 'NONE',  ( 15.82718059914979847, 1409.568640700319975, 192.3709770614890147 ) ) ;
#108714=CARTESIAN_POINT ( 'NONE',  ( 41.62259533861070082, 1442.636044721269855, 135.5651380244540007 ) ) ;
#108716=CARTESIAN_POINT ( 'NONE',  ( -3.310397198750480108, 1509.102546110879985, 179.4781337253649838 ) ) ;
#108719=CARTESIAN_POINT ( 'NONE',  ( 37.29624469549910515, 1450.849357696539982, 134.0999999986649698 ) ) ;
#108721=DIRECTION ( 'NONE',  ( -0.9993902469235412811, 0.03489947644508400310, 0.001077449749359510062 ) ) ;
#108724=CARTESIAN_POINT ( 'NONE',  ( -18.48828930349999666, 1458.367965555730052, 227.6410138353980130 ) ) ;
#108730=CIRCLE ( 'NONE', #15734, 2.000000000000000000 ) ;
#108732=CARTESIAN_POINT ( 'NONE',  ( -2.500000000000039968, 1439.311176619419939, 160.3626367463150189 ) ) ;
#108735=CARTESIAN_POINT ( 'NONE',  ( 38.81202644819820335, 1436.797832379770171, 134.4205481884810069 ) ) ;
#108736=CARTESIAN_POINT ( 'NONE',  ( 2.070960726044260181, 1421.152689218060004, 183.1770975898769791 ) ) ;
#108744=CARTESIAN_POINT ( 'NONE',  ( 37.64188185173559731, 1440.913060387330006, 264.5003480932859929 ) ) ;
#108745=CARTESIAN_POINT ( 'NONE',  ( -0.0001997011801151793269, 1452.268962891940419, 153.8032004743181176 ) ) ;
#108746=VERTEX_POINT ( 'NONE', #18771 ) ;
#108748=CARTESIAN_POINT ( 'NONE',  ( -15.26118644339999975, 1409.612623021030004, 191.5370205933980117 ) ) ;
#108751=CARTESIAN_POINT ( 'NONE',  ( 21.79577993357450083, 1409.838234761750073, 206.3155456279520195 ) ) ;
#108754=CARTESIAN_POINT ( 'NONE',  ( -12.91347167789999872, 1434.774310044260119, 146.4344527888979997 ) ) ;
#108755=CARTESIAN_POINT ( 'NONE',  ( 26.67729797004249903, 1503.852178143910123, 206.2304859205609944 ) ) ;
#108756=CARTESIAN_POINT ( 'NONE',  ( 15.04941445769999930, 1461.565441850729940, 229.9667256941980042 ) ) ;
#108757=PLANE ( 'NONE',  #54522 ) ;
#108758=CARTESIAN_POINT ( 'NONE',  ( -4.424915418274963486, 1421.993387322426543, 184.5440085787073770 ) ) ;
#108762=CARTESIAN_POINT ( 'NONE',  ( -1.004950505856348597, 1486.301326980616750, 181.7814475905654206 ) ) ;
#108763=CARTESIAN_POINT ( 'NONE',  ( -0.04975610472413720398, 1508.745098571959943, 179.9291894445549929 ) ) ;
#108766=CARTESIAN_POINT ( 'NONE',  ( 18.54307487750000050, 1508.238692192329836, 188.5097067394980002 ) ) ;
#108767=CARTESIAN_POINT ( 'NONE',  ( -0.3530891408735000181, 1467.116854267079816, 235.6078141451939985 ) ) ;
#108772=CARTESIAN_POINT ( 'NONE',  ( -11.76832574670000042, 1432.246854381219919, 150.8115016154980026 ) ) ;
#108775=CARTESIAN_POINT ( 'NONE',  ( 6.446325746348199104, 1432.345391573609959, 154.6647259147359819 ) ) ;
#108776=CARTESIAN_POINT ( 'NONE',  ( 20.02479433700000300, 1424.420966076929972, 224.6196048453980154 ) ) ;
#108780=CARTESIAN_POINT ( 'NONE',  ( -19.78242928659999933, 1495.375247112429861, 228.5198483940980054 ) ) ;
#108781=CARTESIAN_POINT ( 'NONE',  ( -4.332041340678299157, 1420.009902215498869, 137.0999999980978430 ) ) ;
#108782=CARTESIAN_POINT ( 'NONE',  ( -2.105918939980000015, 1485.584836081030062, 182.5101142617980088 ) ) ;
#108786=CARTESIAN_POINT ( 'NONE',  ( 14.63616075459999877, 1407.516636404930068, 267.4468191936979906 ) ) ;
#108787=CARTESIAN_POINT ( 'NONE',  ( 0.3096082303459999907, 1409.092176632029805, 185.5936471484980075 ) ) ;
#108791=CARTESIAN_POINT ( 'NONE',  ( 22.17856219145011210, 1430.336759468506671, 217.7288953034882013 ) ) ;
#108793=CARTESIAN_POINT ( 'NONE',  ( -12.78776258889159934, 1416.851343895820037, 195.9645815067300134 ) ) ;
#108794=AXIS2_PLACEMENT_3D ( 'NONE', #1047, #69355, #60959 ) ;
#108795=CARTESIAN_POINT ( 'NONE',  ( 0.000000000000000000, 1395.913060387330006, 215.6218459616979999 ) ) ;
#108797=CARTESIAN_POINT ( 'NONE',  ( -1.640778594498735421, 1450.655424612788693, 183.1975428507971628 ) ) ;
#108798=CARTESIAN_POINT ( 'NONE',  ( 0.5697989931917299966, 1450.893162568030220, 155.3351411520599754 ) ) ;
#108799=CARTESIAN_POINT ( 'NONE',  ( -14.30888197749849944, 1416.029511585999899, 221.2389454739920041 ) ) ;
#108802=CARTESIAN_POINT ( 'NONE',  ( -27.28973479252249845, 1507.987442490729791, 210.9867140273689756 ) ) ;
#108803=CARTESIAN_POINT ( 'NONE',  ( 2.705683380580000019, 1440.723906225590099, 165.1197260195979766 ) ) ;
#108804=CARTESIAN_POINT ( 'NONE',  ( -4.983379166339999777, 1475.784981106930218, 267.2248697199979688 ) ) ;
#108805=CARTESIAN_POINT ( 'NONE',  ( -11.64998282343909253, 1425.712254131211921, 138.1866827809310792 ) ) ;
#108811=CARTESIAN_POINT ( 'NONE',  ( 12.25713978260370141, 1416.640375556570007, 223.5670658059360107 ) ) ;
#108814=CARTESIAN_POINT ( 'NONE',  ( 24.27343987535987679, 1509.087591976627664, 195.8036345857676963 ) ) ;
#108816=CARTESIAN_POINT ( 'NONE',  ( -15.64852212096800166, 1421.346706121272064, 227.1284945715040067 ) ) ;
#108820=CARTESIAN_POINT ( 'NONE',  ( -6.373555541172550853, 1410.509728914295238, 231.3423281520361172 ) ) ;
#108830=CARTESIAN_POINT ( 'NONE',  ( -11.57397602220189725, 1398.256226300480648, 203.1998198725468114 ) ) ;
#108834=CARTESIAN_POINT ( 'NONE',  ( 20.59269091049739941, 1507.766057095049973, 227.7908381428599967 ) ) ;
#108838=CARTESIAN_POINT ( 'NONE',  ( 11.67990115640299997, 1434.088071600169769, 151.1483243173979929 ) ) ;
#108839=CARTESIAN_POINT ( 'NONE',  ( -9.361745962389999676, 1396.239979760129927, 215.6895990424980027 ) ) ;
#108840=CARTESIAN_POINT ( 'NONE',  ( -22.51990863569999846, 1410.619212186330060, 212.0399858907879889 ) ) ;
#108841=ORIENTED_EDGE ( 'NONE', *, *, #96638, .F. ) ;
#108842=CARTESIAN_POINT ( 'NONE',  ( -13.16099798814397204, 1444.747053629154379, 169.3968106364190191 ) ) ;
#108843=CARTESIAN_POINT ( 'NONE',  ( 20.59987592950000135, 1509.677367935830262, 230.5839143914980127 ) ) ;
#108844=CARTESIAN_POINT ( 'NONE',  ( -10.10004869884733125, 1422.222932908416851, 137.0999999980979851 ) ) ;
#108846=CARTESIAN_POINT ( 'NONE',  ( 17.85789328519999941, 1419.045775438330111, 225.4480613795979878 ) ) ;
#108847=CARTESIAN_POINT ( 'NONE',  ( 11.47832759589999974, 1468.696517459929964, 186.4345343207980079 ) ) ;
#108848=CARTESIAN_POINT ( 'NONE',  ( -7.561650701720000534, 1415.425582719929707, 193.0231593168980169 ) ) ;
#108851=B_SPLINE_SURFACE_WITH_KNOTS ( 'NONE', 5, 5, ( 
 ( #84451, #7737, #17203, #60367, #41898, #84982 ),
 ( #67672, #17760, #25070, #43561, #51964, #86105 ),
 ( #32398, #76600, #59273, #8278, #42442, #54739 ),
 ( #78818, #11613, #2132, #63158, #95611, #28413 ),
 ( #53639, #26744, #27858, #19999, #96726, #60933 ),
 ( #18877, #45789, #69331, #105687, #79372, #88868 ),
 ( #79924, #36256, #3238, #103438, #20535, #70444 ),
 ( #104564, #86651, #52520, #35699, #95062, #18329 ),
 ( #9947, #44119, #28968, #35147, #78254, #54191 ) ),
 .UNSPECIFIED., .F., .F., .F.,
 ( 6, 3, 6 ),
 ( 6, 6 ),
 ( 17.98520084990000001, 40.17980702489999345, 62.49762447089999995 ),
 ( 0.000000000000000000, 1.595529479780000148 ),
 .UNSPECIFIED. ) ;
#108852=CARTESIAN_POINT ( 'NONE',  ( 8.782767202921888838, 1396.219761434090060, 202.4073701858239929 ) ) ;
#108853=CARTESIAN_POINT ( 'NONE',  ( 1.441539353570000070, 1414.983773854429955, 191.7394860450980048 ) ) ;
#108854=CARTESIAN_POINT ( 'NONE',  ( 11.72512635530000047, 1429.059158185030128, 149.9312760468980059 ) ) ;
#108857=CARTESIAN_POINT ( 'NONE',  ( 13.12713025425550128, 1434.844877208209937, 149.2796170260219810 ) ) ;
#108858=ORIENTED_EDGE ( 'NONE', *, *, #53463, .F. ) ;
#108862=CARTESIAN_POINT ( 'NONE',  ( -9.200915198040000575, 1463.128421874929927, 234.0379130468980122 ) ) ;
#108876=ORIENTED_EDGE ( 'NONE', *, *, #75568, .F. ) ;
#108878=CARTESIAN_POINT ( 'NONE',  ( -20.52130963250000306, 1509.391296577229923, 229.7160214944979941 ) ) ;
#108879=CARTESIAN_POINT ( 'NONE',  ( -38.93016163265561147, 1429.415421242818866, 269.5917615160539640 ) ) ;
#108880=CARTESIAN_POINT ( 'NONE',  ( -1.169015704899999841, 1409.121795253429809, 232.4446791288980023 ) ) ;
#108881=CARTESIAN_POINT ( 'NONE',  ( -1.377258800830409857, 1414.913060387399810, 225.7566283813699783 ) ) ;
#108884=CARTESIAN_POINT ( 'NONE',  ( -30.79536835113719917, 1440.913060387759970, 240.7855773362489913 ) ) ;
#108886=CARTESIAN_POINT ( 'NONE',  ( -0.6774407473332200169, 1465.095561399730059, 238.0673353718009935 ) ) ;
#108887=CIRCLE ( 'NONE', #12320, 1.000000000000000000 ) ;
#108888=CARTESIAN_POINT ( 'NONE',  ( 10.80862676779999987, 1409.502744133030092, 270.4164080866979702 ) ) ;
#108890=CARTESIAN_POINT ( 'NONE',  ( 24.13936747690000217, 1411.115472691630202, 209.3334965061050070 ) ) ;
#108891=CARTESIAN_POINT ( 'NONE',  ( -21.24031773869999995, 1509.721128092229947, 188.1621763370980034 ) ) ;
#108896=EDGE_CURVE ( 'NONE', #33631, #6602, #50217, .T. ) ;
#108897=CARTESIAN_POINT ( 'NONE',  ( -3.812352470338788546, 1447.062376414930668, 154.8462586213417751 ) ) ;
#108898=CARTESIAN_POINT ( 'NONE',  ( 0.2538825943349999892, 1420.503732742429975, 182.7635796100980201 ) ) ;
#108899=CARTESIAN_POINT ( 'NONE',  ( -14.78542619307623873, 1486.064264431397760, 186.1959007592220701 ) ) ;
#108902=ORIENTED_EDGE ( 'NONE', *, *, #46642, .F. ) ;
#108904=CARTESIAN_POINT ( 'NONE',  ( 30.10642679900000118, 1468.180645040329864, 266.8105454816980000 ) ) ;
#108912=EDGE_CURVE ( 'NONE', #11504, #55526, #74727, .T. ) ;
#108915=CARTESIAN_POINT ( 'NONE',  ( -31.61373809194337170, 1450.520981466214153, 136.3130663088220160 ) ) ;
#108919=CARTESIAN_POINT ( 'NONE',  ( 11.94601693890058591, 1433.509856785846750, 149.8908047706937623 ) ) ;
#108920=CARTESIAN_POINT ( 'NONE',  ( 0.3722769094550000268, 1457.826255240429873, 228.9731060097980162 ) ) ;
#108924=CARTESIAN_POINT ( 'NONE',  ( -4.653281936863520762, 1425.827070423550140, 186.2156739099499987 ) ) ;
#108926=( BOUNDED_CURVE ( )  B_SPLINE_CURVE ( 3, ( #24153, #109843, #92468, #6274 ),
 .UNSPECIFIED., .F., .T. ) 
 B_SPLINE_CURVE_WITH_KNOTS ( ( 4, 4 ),
 ( 1.569654396653685113, 1.584183882043254998 ),
 .UNSPECIFIED. ) 
 CURVE ( )  GEOMETRIC_REPRESENTATION_ITEM ( )  RATIONAL_B_SPLINE_CURVE ( ( 1.000000000000000000, 0.9999824079152302980, 0.9999824079152302980, 1.000000000000000000 ) ) 
 REPRESENTATION_ITEM ( '' )  );
#108928=PLANE ( 'NONE',  #19218 ) ;
#108930=CARTESIAN_POINT ( 'NONE',  ( 39.92950177491940167, 1445.941520873710033, 136.8098320836529922 ) ) ;
#108931=CARTESIAN_POINT ( 'NONE',  ( -20.08890542589999839, 1427.297090845429921, 222.6039534643979891 ) ) ;
#108938=CARTESIAN_POINT ( 'NONE',  ( -32.70045657439047204, 1460.057872603863643, 269.5016316249235047 ) ) ;
#108940=CARTESIAN_POINT ( 'NONE',  ( -27.43355922089999765, 1507.980920696029898, 210.8261541407979962 ) ) ;
#108941=CARTESIAN_POINT ( 'NONE',  ( -42.04831442898936444, 1427.619777667461676, 269.0744805272954068 ) ) ;
#108942=ADVANCED_FACE ( 'NONE', ( #81991 ), #43674, .F. ) ;
#108946=CARTESIAN_POINT ( 'NONE',  ( -13.50801430494305144, 1444.065531194597725, 187.0996317180838560 ) ) ;
#108951=CARTESIAN_POINT ( 'NONE',  ( 0.000000000000000000, 1442.773887286369927, 126.8032249175980155 ) ) ;
#108954=LINE ( 'NONE', #31679, #33897 ) ;
#108956=CARTESIAN_POINT ( 'NONE',  ( -14.06840730360000080, 1410.335884372329929, 226.9421448683980032 ) ) ;
#108957=ORIENTED_EDGE ( 'NONE', *, *, #31790, .T. ) ;
#108959=CARTESIAN_POINT ( 'NONE',  ( 0.3166099824879999858, 1416.237488680629895, 190.8312741502979861 ) ) ;
#108960=CARTESIAN_POINT ( 'NONE',  ( 21.95218051589786157, 1509.537469184427891, 226.8469781385923909 ) ) ;
#108963=CARTESIAN_POINT ( 'NONE',  ( 17.90185111903100079, 1415.935475482089942, 209.1139596251610158 ) ) ;
#108966=CARTESIAN_POINT ( 'NONE',  ( 2.828023937740000225E-08, 1459.479586679530030, 211.7966661906679917 ) ) ;
#108967=CARTESIAN_POINT ( 'NONE',  ( -20.41479141479999981, 1507.904137136529926, 189.4586056721979901 ) ) ;
#108968=CARTESIAN_POINT ( 'NONE',  ( -11.81534876189999927, 1433.145554964519988, 150.5637033868979699 ) ) ;
#108973=CARTESIAN_POINT ( 'NONE',  ( -24.42533849189999984, 1437.817893690260235, 210.7709910404479956 ) ) ;
#108975=CARTESIAN_POINT ( 'NONE',  ( 1.885834960689999784, 1450.497026778770078, 182.4567463587980001 ) ) ;
#108977=CARTESIAN_POINT ( 'NONE',  ( -16.02051642983965252, 1509.593599257673759, 183.6930697544212023 ) ) ;
#108978=EDGE_CURVE ( 'NONE', #7065, #46444, #26938, .T. ) ;
#108981=ORIENTED_EDGE ( 'NONE', *, *, #25761, .F. ) ;
#108982=CARTESIAN_POINT ( 'NONE',  ( -11.75396294214339932, 1426.798760010640081, 145.3508344385039948 ) ) ;
#108985=CARTESIAN_POINT ( 'NONE',  ( -5.349258416210000533, 1473.354001796429884, 270.3881948814980092 ) ) ;
#108995=CARTESIAN_POINT ( 'NONE',  ( -41.65756761579879708, 1426.556841175060072, 269.0856960666789632 ) ) ;
#108998=B_SPLINE_SURFACE_WITH_KNOTS ( 'NONE', 5, 5, ( 
 ( #25537, #61401, #18793, #51307, #42925, #8742 ),
 ( #77082, #34510, #78164, #9860, #44027, #68687 ),
 ( #35608, #41807, #102793, #26090, #1476, #69803 ),
 ( #60279, #17677, #51880, #86016, #9316, #43479 ),
 ( #77624, #935, #21545, #80385, #3701, #72541 ),
 ( #78727, #27766, #2042, #89328, #10973, #54655 ) ),
 .UNSPECIFIED., .F., .F., .F.,
 ( 6, 6 ),
 ( 6, 6 ),
 ( 95.54053164052498914, 167.5214209060000030 ),
 ( -0.0006553164636343219865, 2.000655316463329836 ),
 .UNSPECIFIED. ) ;
#109003=CARTESIAN_POINT ( 'NONE',  ( 17.22592475669603473, 1443.913060387329097, 162.9227486557985003 ) ) ;
#109006=CARTESIAN_POINT ( 'NONE',  ( -2.370970874524634286, 1427.002265528474027, 134.0999999980980135 ) ) ;
#109007=CARTESIAN_POINT ( 'NONE',  ( -10.00325457980000010, 1455.444522322430203, 186.2569471202980083 ) ) ;
#109009=CARTESIAN_POINT ( 'NONE',  ( -17.64503295873700139, 1507.624289566409971, 229.7594340571970122 ) ) ;
#109012=CARTESIAN_POINT ( 'NONE',  ( -26.81252206619999967, 1435.744110061079937, 136.2294616770979871 ) ) ;
#109015=EDGE_CURVE ( 'NONE', #25299, #21185, #88415, .T. ) ;
#109016=B_SPLINE_SURFACE_WITH_KNOTS ( 'NONE', 5, 5, ( 
 ( #78389, #52645, #45363, #54317, #68912, #18446 ),
 ( #52095, #103579, #26309, #94623, #88446, #10071 ),
 ( #17898, #9517, #44246, #44805, #77836, #71124 ),
 ( #105245, #62165, #35277, #43685, #69462, #26881 ),
 ( #61070, #1697, #35838, #96291, #70021, #104135 ),
 ( #27421, #77295, #61604, #19001, #28536, #53201 ),
 ( #87342, #78958, #87910, #2265, #62737, #36379 ),
 ( #70568, #19570, #11199, #79502, #2809, #97386 ),
 ( #64914, #12826, #3910, #98483, #37488, #38574 ),
 ( #55953, #88983, #38040, #20657, #39119, #72219 ),
 ( #54859, #106880, #13914, #22860, #12271, #99025 ),
 ( #89537, #47006, #107986, #105811, #55405, #48099 ),
 ( #31283, #30171, #65467, #71692, #29627, #90075 ),
 ( #81130, #13358, #29090, #82239, #106341, #56504 ),
 ( #22301, #63275, #5540, #57066, #47549, #39691 ) ),
 .UNSPECIFIED., .F., .F., .F.,
 ( 6, 3, 3, 3, 6 ),
 ( 6, 6 ),
 ( 29.73194161469999841, 37.05188947199999916, 56.18585872479999921, 82.63977583489999290, 135.5476100549999785 ),
 ( -3.023210959359999692E-09, 2.000000000000000000 ),
 .UNSPECIFIED. ) ;
#109019=CARTESIAN_POINT ( 'NONE',  ( -44.93140602508920267, 1440.913053221170003, 269.6837651506019711 ) ) ;
#109021=DIRECTION ( 'NONE',  ( 4.440892098500004934E-16, 1.000000000000000000, -1.817990202819999994E-15 ) ) ;
#109022=CIRCLE ( 'NONE', #89349, 20.98341875040010507 ) ;
#109024=CARTESIAN_POINT ( 'NONE',  ( -38.57017548137279306, 1443.484401788910191, 137.1611502647359941 ) ) ;
#109027=CARTESIAN_POINT ( 'NONE',  ( 0.2421645026379999899, 1451.163597850030101, 182.5480897152980049 ) ) ;
#109030=CARTESIAN_POINT ( 'NONE',  ( -23.77614021810000011, 1435.333969175160064, 137.3595125206979901 ) ) ;
#109031=CARTESIAN_POINT ( 'NONE',  ( -24.90875591689999879, 1442.283708403439960, 210.4817964918080122 ) ) ;
#109036=CARTESIAN_POINT ( 'NONE',  ( -14.32036905050000009, 1426.820448865629942, 222.1614598904980085 ) ) ;
#109037=CARTESIAN_POINT ( 'NONE',  ( 3.646194203732994854, 1440.832530381142760, 156.5727254137537159 ) ) ;
#109043=CARTESIAN_POINT ( 'NONE',  ( -19.66086063814984186, 1456.978398402603716, 225.7864354487686285 ) ) ;
#109044=ORIENTED_EDGE ( 'NONE', *, *, #23088, .T. ) ;
#109047=DIRECTION ( 'NONE',  ( 0.8248189069719331634, 0.4629720251890361293, -0.3245468758037705626 ) ) ;
#109048=CARTESIAN_POINT ( 'NONE',  ( -4.113893833246661025, 1440.069258426123497, 185.4380465277182282 ) ) ;
#109049=CARTESIAN_POINT ( 'NONE',  ( 15.05358515032119904, 1410.831827804430077, 191.5175411757069810 ) ) ;
#109050=CARTESIAN_POINT ( 'NONE',  ( 2.500000000000000000, 1443.913060387330006, 150.6726614421979775 ) ) ;
#109053=CARTESIAN_POINT ( 'NONE',  ( 2.409586283469999923, 1426.663880916129983, 144.1938086916980239 ) ) ;
#109054=CARTESIAN_POINT ( 'NONE',  ( 22.06126275483152810, 1452.693645232389372, 220.1374946003218440 ) ) ;
#109055=EDGE_CURVE ( 'NONE', #83948, #31992, #21552, .T. ) ;
#109058=DIRECTION ( 'NONE',  ( 0.8730704095473449389, 0.4873619484741930075, 0.01504630028510589926 ) ) ;
#109061=CARTESIAN_POINT ( 'NONE',  ( -11.69744348347709995, 1415.090956648730071, 195.9645815027980120 ) ) ;
#109063=CARTESIAN_POINT ( 'NONE',  ( 0.2538967969029999883, 1420.503737814829947, 182.7635776114979933 ) ) ;
#109064=ADVANCED_FACE ( 'NONE', ( #57798 ), #91920, .T. ) ;
#109065=EDGE_CURVE ( 'NONE', #68085, #41682, #83511, .T. ) ;
#109067=CARTESIAN_POINT ( 'NONE',  ( -9816.840209716168829, 50.13405481564039690, 1424.308828391800034 ) ) ;
#109071=CARTESIAN_POINT ( 'NONE',  ( 17.20725958045629866, 1422.406334852679720, 226.7076084557567981 ) ) ;
#109074=CARTESIAN_POINT ( 'NONE',  ( 25.98102620618460179, 1446.564900598649956, 138.2990622187049894 ) ) ;
#109080=CARTESIAN_POINT ( 'NONE',  ( -27.01382282590000017, 1451.969727051930022, 134.9184453750980026 ) ) ;
#109081=CARTESIAN_POINT ( 'NONE',  ( -9.336114142359406287, 1506.539416414647121, 229.1226208970104494 ) ) ;
#109083=DIRECTION ( 'NONE',  ( -0.001078628244322317031, -3.766396416021244533E-05, -0.9999994175710984479 ) ) ;
#109085=EDGE_CURVE ( 'NONE', #56358, #2071, #25520, .T. ) ;
#109086=CARTESIAN_POINT ( 'NONE',  ( 27.53661718181439610, 1509.986717858917018, 221.0270820719949256 ) ) ;
#109100=CARTESIAN_POINT ( 'NONE',  ( -17.08792848909999762, 1409.509783999230194, 223.5124184947979984 ) ) ;
#109101=VERTEX_POINT ( 'NONE', #103062 ) ;
#109106=DIRECTION ( 'NONE',  ( -0.8023110876747339137, -0.5969061220947440294, 0.000000000000000000 ) ) ;
#109111=B_SPLINE_CURVE_WITH_KNOTS ( 'NONE', 3,
 ( #63240, #80003, #36892, #52609, #38002, #19529, #18411, #72184, #26842, #71085, #10597, #61028, #87872, #86747, #70532, #44208, #104650, #78351, #1660, #44769, #27946, #69981, #61567, #62127, #96254, #53735, #45323, #22260, #29587, #46971, #56461, #38538, #14426, #91701, #39652, #64324, #31242, #91150, #89501, #12793, #72715, #49170, #21161, #31792, #98447, #47510, #48622, #99533, #90594, #73822, #13871, #21715, #65426, #55919, #106838, #48057, #57024, #23386, #63771, #106303, #82192, #108505, #22817, #39079, #107397, #5495, #30693, #107950, #82754, #14975, #100105, #55368, #64879, #6046, #65982, #81093, #90038, #73257, #83302, #40197, #74380, #98986, #57576, #6597, #13315, #4409, #30132, #40747, #97887, #81633, #4935, #85486, #7151, #109613, #58666, #76005, #102839, #26133, #92253, #17719, #58119, #74924, #86064, #92802, #83851, #16612, #9359, #32886, #15523, #59230, #59774, #42968, #68192, #8232, #101740, #51921, #34552, #100638, #93347, #7693, #23925, #8786, #67079, #49719, #41850, #41307, #68735, #42399, #67626, #33999, #84939, #75480, #25028, #60322, #76553, #110709, #102296, #33429, #25581 ),
 .UNSPECIFIED., .F., .F.,
 ( 4, 3, 3, 3, 3, 3, 3, 3, 3, 3, 3, 3, 3, 3, 3, 3, 3, 3, 3, 3, 3, 3, 3, 3, 3, 3, 3, 3, 3, 3, 3, 3, 3, 3, 3, 3, 3, 3, 3, 3, 3, 3, 3, 3, 3, 3, 4 ),
 ( -28.53827112919999820, -26.45221505981819732, -24.01267252766740157, -21.74496381986899962, -19.71304886792480104, -17.83305997891750039, -16.05771537107780134, -14.36033624732730019, -12.75138636564559924, -11.18760895869190009, -9.657646656378112482, -8.173724279849281515, -6.990632790278482389, -5.760582367847380425, -4.497816196510928677, -3.242242590771951427, -1.969189602956539886, -0.6774439780757006702, 0.6566481976939542164, 1.992772157457029181, 3.367048238499528168, 4.341547002844251324, 5.758069219566863239, 7.176877794369772801, 8.618992616491055969, 9.956394040244987309, 11.39760739419979529, 12.72337739229750042, 14.29692855573880195, 15.67372473662510401, 16.59104555840569617, 17.57661266362431007, 18.56849156666920209, 19.56575179944280052, 20.56727088331129494, 21.57175587605299683, 22.57778385006959354, 23.58385892812350448, 24.58711680646079856, 25.58704511002700599, 26.58256055503940019, 27.57272639591489849, 28.57604209978619991, 29.55008166352749299, 30.56803543746379859, 31.52659850778239559, 31.58598921140000471 ),
 .UNSPECIFIED. ) ;
#109113=CARTESIAN_POINT ( 'NONE',  ( 9.063831788663421207, 1409.229576367929894, 197.2185231063879769 ) ) ;
#109114=CARTESIAN_POINT ( 'NONE',  ( 0.5238716732950000621, 1409.870337220530018, 185.0929749023979980 ) ) ;
#109116=FACE_OUTER_BOUND ( 'NONE', #71878, .T. ) ;
#109118=CARTESIAN_POINT ( 'NONE',  ( -13.62133678120479985, 1452.879579795280051, 223.2680741433150047 ) ) ;
#109120=B_SPLINE_CURVE_WITH_KNOTS ( 'NONE', 5,
 ( #83212, #73733, #40101, #30604, #31696, #58025 ),
 .UNSPECIFIED., .F., .F.,
 ( 6, 6 ),
 ( 0.000000000000000000, 1.000000000000000000 ),
 .UNSPECIFIED. ) ;
#109122=CARTESIAN_POINT ( 'NONE',  ( 18.38772902297059986, 1457.332268191050161, 228.4537576404730146 ) ) ;
#109123=CARTESIAN_POINT ( 'NONE',  ( -12.06208110920000109, 1434.483679219209989, 150.8899553371979891 ) ) ;
#109125=CARTESIAN_POINT ( 'NONE',  ( -6.553452772086439930E-09, 1475.392274334100193, 266.1199166997070051 ) ) ;
#109131=CARTESIAN_POINT ( 'NONE',  ( -46.02992379481870699, 1440.698477837170003, 268.4959868370419827 ) ) ;
#109132=CARTESIAN_POINT ( 'NONE',  ( 14.12038737319999804, 1509.406339941330089, 234.8413163218980060 ) ) ;
#109137=CARTESIAN_POINT ( 'NONE',  ( 5.451912722298930092, 1408.921438237069879, 222.1546799351359880 ) ) ;
#109139=CARTESIAN_POINT ( 'NONE',  ( 11.43480838300000002, 1425.837049133330083, 122.9428393764980001 ) ) ;
#109142=CARTESIAN_POINT ( 'NONE',  ( 8.200031714130000537, 1420.268578394229962, 225.6600891460980165 ) ) ;
#109144=CARTESIAN_POINT ( 'NONE',  ( -16.19188927940000156, 1409.478493620530116, 194.5079787952979871 ) ) ;
#109146=VECTOR ( 'NONE', #21026, 1000.000000000000114 ) ;
#109147=DIRECTION ( 'NONE',  ( 0.000000000000000000, 0.000000000000000000, -1.000000000000000000 ) ) ;
#109149=CARTESIAN_POINT ( 'NONE',  ( -1.463139458404679960, 1452.861966431559949, 152.4924432263949825 ) ) ;
#109150=CARTESIAN_POINT ( 'NONE',  ( -18.96325319869999859, 1416.831305841230005, 208.0005775078080035 ) ) ;
#109151=EDGE_LOOP ( 'NONE', ( #106785, #49689, #12686, #95532 ) ) ;
#109152=CARTESIAN_POINT ( 'NONE',  ( -2.500000000000000000, 1419.382958344190001, 144.1003752082409903 ) ) ;
#109153=CARTESIAN_POINT ( 'NONE',  ( 4.823329535264199886E-05, 1409.206609320529878, 270.3713713915270205 ) ) ;
#109154=CARTESIAN_POINT ( 'NONE',  ( 16.42440859496330319, 1423.292924526380148, 228.6634581238010071 ) ) ;
#109157=ORIENTED_EDGE ( 'NONE', *, *, #27042, .T. ) ;
#109159=CARTESIAN_POINT ( 'NONE',  ( -23.59803273300959958, 1410.014125045500123, 208.9302168428020252 ) ) ;
#109160=CARTESIAN_POINT ( 'NONE',  ( -3.903576985680000000, 1424.789296738229950, 185.8774067644979766 ) ) ;
#109163=CARTESIAN_POINT ( 'NONE',  ( -3.194354728630000029, 1498.350177541130051, 236.3803358245980064 ) ) ;
#109166=CARTESIAN_POINT ( 'NONE',  ( 43.55151698956129991, 1452.829994745100066, 267.0610574176429850 ) ) ;
#109168=CARTESIAN_POINT ( 'NONE',  ( -0.02483341509479999876, 1420.438468297229974, 183.3023409683979992 ) ) ;
#109171=CARTESIAN_POINT ( 'NONE',  ( 18.93983199967145126, 1457.591331553862574, 226.8224651722836995 ) ) ;
#109175=EDGE_LOOP ( 'NONE', ( #78873, #97560, #93373, #76377 ) ) ;
#109177=EDGE_CURVE ( 'NONE', #78889, #110373, #12247, .T. ) ;
#109178=CARTESIAN_POINT ( 'NONE',  ( 26.89135176257029869, 1451.907621766309830, 135.4131197746179964 ) ) ;
#109185=CARTESIAN_POINT ( 'NONE',  ( 1.871191615658170049, 1408.978403838410031, 186.8925371725070192 ) ) ;
#109186=CARTESIAN_POINT ( 'NONE',  ( -13.79715687802010038, 1434.979310490669832, 148.5442485412900169 ) ) ;
#109189=EDGE_CURVE ( 'NONE', #51052, #44714, #60263, .T. ) ;
#109195=CARTESIAN_POINT ( 'NONE',  ( 10.79382269979189957, 1414.913060387349788, 222.1041130917409987 ) ) ;
#109197=EDGE_CURVE ( 'NONE', #8806, #14678, #34858, .T. ) ;
#109202=CARTESIAN_POINT ( 'NONE',  ( 4.304798037349998904E-15, 1432.353341358199941, 150.3995506339979897 ) ) ;
#109205=CARTESIAN_POINT ( 'NONE',  ( 28.02005514660000074, 1440.913060387330006, 248.0989693021979861 ) ) ;
#109206=CARTESIAN_POINT ( 'NONE',  ( 13.15726442530000107, 1416.237488680629895, 196.4123356676979881 ) ) ;
#109207=VECTOR ( 'NONE', #92985, 1000.000000000000114 ) ;
#109212=CIRCLE ( 'NONE', #89532, 7.016581249619902039 ) ;
#109214=CARTESIAN_POINT ( 'NONE',  ( -17.22268207119999772, 1410.011820319130038, 225.6635735971980239 ) ) ;
#109216=CARTESIAN_POINT ( 'NONE',  ( 23.55087209250000058, 1410.914164809929844, 211.6928269362679771 ) ) ;
#109217=CARTESIAN_POINT ( 'NONE',  ( -17.31562880812650107, 1410.013633825039960, 192.7163598956479689 ) ) ;
#109222=CARTESIAN_POINT ( 'NONE',  ( -10.54743214440000010, 1416.216739748429973, 223.6935680435979918 ) ) ;
#109223=CARTESIAN_POINT ( 'NONE',  ( 0.1907346795993619948, 1468.290221018919965, 182.5972501460889816 ) ) ;
#109226=CARTESIAN_POINT ( 'NONE',  ( -23.84533141485470153, 1452.080363065020038, 136.9869391916130041 ) ) ;
#109227=AXIS2_PLACEMENT_3D ( 'NONE', #7131, #59751, #110684 ) ;
#109230=CARTESIAN_POINT ( 'NONE',  ( -41.34669637373799844, 1445.942886885710095, 134.0999999985539830 ) ) ;
#109234=DIRECTION ( 'NONE',  ( -0.7074300732573280959, 0.02470400251971149874, 0.7063514732133270302 ) ) ;
#109236=SPHERICAL_SURFACE ( 'NONE', #85633, 2.000000000000000000 ) ;
#109238=CARTESIAN_POINT ( 'NONE',  ( 40.50350722682676263, 1425.156443366132180, 269.1155502198245131 ) ) ;
#109241=DIRECTION ( 'NONE',  ( 0.000000000000000000, 8.545517954889998490E-18, 1.000000000000000000 ) ) ;
#109246=CARTESIAN_POINT ( 'NONE',  ( -32.05911432779999615, 1450.505517766510138, 136.2999930999980052 ) ) ;
#109247=CARTESIAN_POINT ( 'NONE',  ( -16.33521701716129826, 1410.862700950380031, 226.6351052317230028 ) ) ;
#109253=FACE_OUTER_BOUND ( 'NONE', #95088, .T. ) ;
#109255=CARTESIAN_POINT ( 'NONE',  ( -11.20854081390000090, 1414.996444526030018, 195.7122653627979787 ) ) ;
#109256=CARTESIAN_POINT ( 'NONE',  ( 23.20232703090000115, 1411.083540124029923, 212.8787804838979980 ) ) ;
#109258=CARTESIAN_POINT ( 'NONE',  ( -16.00015186889999796, 1423.003814079930180, 228.7447940140980052 ) ) ;
#109262=CARTESIAN_POINT ( 'NONE',  ( 3.487133837120000024, 1431.113060387329824, 227.6029907049980068 ) ) ;
#109265=CARTESIAN_POINT ( 'NONE',  ( 2.500000000000000000, 1448.229591938679960, 165.9681890900980079 ) ) ;
#109266=VERTEX_POINT ( 'NONE', #18784 ) ;
#109268=CARTESIAN_POINT ( 'NONE',  ( 16.87240902346729854, 1409.502257893559772, 222.1138755377239988 ) ) ;
#109269=DIRECTION ( 'NONE',  ( 0.6670494068259388287, 0.5110419776299538475, 0.5421080943439499089 ) ) ;
#109271=ORIENTED_EDGE ( 'NONE', *, *, #45240, .F. ) ;
#109272=CARTESIAN_POINT ( 'NONE',  ( -18.26675480510339966, 1424.840341062940070, 227.6848255537819909 ) ) ;
#109273=EDGE_LOOP ( 'NONE', ( #5391, #14233, #82414 ) ) ;
#109276=B_SPLINE_CURVE_WITH_KNOTS ( 'NONE', 3,
 ( #57714, #48757, #91830, #91286 ),
 .UNSPECIFIED., .F., .F.,
 ( 4, 4 ),
 ( 0.000000000000000000, 0.003000049121573633397 ),
 .UNSPECIFIED. ) ;
#109277=CARTESIAN_POINT ( 'NONE',  ( -11.41539857968949967, 1425.494006463380174, 142.6748587622950026 ) ) ;
#109278=CARTESIAN_POINT ( 'NONE',  ( 15.93865550815479892, 1409.469629138669916, 193.0036447647779880 ) ) ;
#109281=CARTESIAN_POINT ( 'NONE',  ( 39.08639746099999712, 1439.774711833670153, 136.7053848153979914 ) ) ;
#109282=CARTESIAN_POINT ( 'NONE',  ( -11.73702549210000079, 1426.695992139529835, 144.1699184476980236 ) ) ;
#109284=CARTESIAN_POINT ( 'NONE',  ( 2.902343876856320115, 1466.632250330839952, 234.1422825383600070 ) ) ;
#109285=CARTESIAN_POINT ( 'NONE',  ( 13.95592155805312906, 1416.839570625517808, 196.3344139125129857 ) ) ;
#109287=ORIENTED_EDGE ( 'NONE', *, *, #23751, .T. ) ;
#109292=CARTESIAN_POINT ( 'NONE',  ( -29.75012120250000081, 1509.993914124430148, 208.5595671623779879 ) ) ;
#109295=CARTESIAN_POINT ( 'NONE',  ( 0.1171482500689999956, 1451.168562942830249, 182.5358585629980155 ) ) ;
#109296=CARTESIAN_POINT ( 'NONE',  ( -3.321445554160000313, 1484.261041720429830, 183.3707341603979728 ) ) ;
#109297=DIRECTION ( 'NONE',  ( 0.000000000000000000, -1.000000000000000000, 0.000000000000000000 ) ) ;
#109300=CARTESIAN_POINT ( 'NONE',  ( 38.81202643689640297, 1436.797832322039994, 134.7402662745759869 ) ) ;
#109301=CARTESIAN_POINT ( 'NONE',  ( 2.116101361519879820, 1421.168810873590019, 183.1883719185100006 ) ) ;
#109302=CARTESIAN_POINT ( 'NONE',  ( 26.44808090420000113, 1439.564396612150176, 137.2471738511979993 ) ) ;
#109308=ORIENTED_EDGE ( 'NONE', *, *, #47446, .T. ) ;
#109310=AXIS2_PLACEMENT_3D ( 'NONE', #102166, #93751, #78641 ) ;
#109313=CARTESIAN_POINT ( 'NONE',  ( -13.29661090509999966, 1415.048591087029763, 220.6690200173979974 ) ) ;
#109314=EDGE_CURVE ( 'NONE', #34791, #81429, #52351, .T. ) ;
#109315=CARTESIAN_POINT ( 'NONE',  ( -11.72314552038290003, 1432.337468424269900, 150.7717712668979857 ) ) ;
#109316=CARTESIAN_POINT ( 'NONE',  ( -0.7950258152958181723, 1426.814114633998997, 137.0999999982234385 ) ) ;
#109319=CARTESIAN_POINT ( 'NONE',  ( -12.99738333980000071, 1429.131617844829861, 222.4366461256979903 ) ) ;
#109322=CARTESIAN_POINT ( 'NONE',  ( -14.20380459391698302, 1410.782058423236776, 190.3118870790858637 ) ) ;
#109323=CARTESIAN_POINT ( 'NONE',  ( -15.22920806200000143, 1462.589963187330113, 223.3216945802979865 ) ) ;
#109324=CARTESIAN_POINT ( 'NONE',  ( 16.63395562619999879, 1459.015801707430001, 231.1847121254979811 ) ) ;
#109326=CARTESIAN_POINT ( 'NONE',  ( -4.958647264046995851, 1422.537331718762516, 184.8308287925253524 ) ) ;
#109330=CARTESIAN_POINT ( 'NONE',  ( -22.70988283845126787, 1409.706100392974804, 208.9686675985246325 ) ) ;
#109332=EDGE_CURVE ( 'NONE', #10122, #55469, #17585, .T. ) ;
#109336=B_SPLINE_CURVE_WITH_KNOTS ( 'NONE', 3,
 ( #24946, #13935, #47566, #16540 ),
 .UNSPECIFIED., .F., .F.,
 ( 4, 4 ),
 ( -20.28790011219829736, -6.722899290939999162 ),
 .UNSPECIFIED. ) ;
#109339=CARTESIAN_POINT ( 'NONE',  ( 1.119642440080000023, 1434.994542537360076, 189.3593017752980074 ) ) ;
#109341=ADVANCED_FACE ( 'NONE', ( #255 ), #69647, .T. ) ;
#109342=CARTESIAN_POINT ( 'NONE',  ( -11.86543074620000127, 1432.295683013649978, 150.3972177407979984 ) ) ;
#109345=CARTESIAN_POINT ( 'NONE',  ( 3.134082760970000159, 1421.411057458130017, 144.1516174827979739 ) ) ;
#109347=CARTESIAN_POINT ( 'NONE',  ( 4.367506823990000342, 1410.393541147229826, 231.4170693631980100 ) ) ;
#109348=CARTESIAN_POINT ( 'NONE',  ( -23.05235012189999821, 1482.723166241629997, 221.7956923970979801 ) ) ;
#109349=CARTESIAN_POINT ( 'NONE',  ( -6.061273928713842629, 1422.611328064380359, 137.0999999980751340 ) ) ;
#109350=CARTESIAN_POINT ( 'NONE',  ( -28.77730030020000029, 1509.917985857730173, 212.2396942135479776 ) ) ;
#109353=CARTESIAN_POINT ( 'NONE',  ( 4.952595917969999206, 1406.456499948729970, 269.2856872263980108 ) ) ;
#109356=CARTESIAN_POINT ( 'NONE',  ( 21.09738187590000180, 1410.867002981430005, 200.0903158484080109 ) ) ;
#109364=CARTESIAN_POINT ( 'NONE',  ( -13.79526254970000032, 1445.853624484049760, 188.3960237689979920 ) ) ;
#109367=CARTESIAN_POINT ( 'NONE',  ( 3.196891693280000002, 1407.733286134229957, 270.1354749225980072 ) ) ;
#109370=CARTESIAN_POINT ( 'NONE',  ( 11.02941167081014484, 1424.908287015548240, 138.1869667496993088 ) ) ;
#109373=CARTESIAN_POINT ( 'NONE',  ( -2.778684086150000176, 1476.048032409329835, 267.8507713580979726 ) ) ;
#109374=CARTESIAN_POINT ( 'NONE',  ( -4.222051551403209757, 1446.225887192099890, 170.2164200388130268 ) ) ;
#109379=CARTESIAN_POINT ( 'NONE',  ( -6.655787406570000009, 1441.606255579999925, 154.8401361813980088 ) ) ;
#109382=CARTESIAN_POINT ( 'NONE',  ( -45.63712966311000230, 1440.913059426480004, 268.9747523979869470 ) ) ;
#109383=CARTESIAN_POINT ( 'NONE',  ( -21.36941021309999655, 1409.659296635530154, 204.4057705028979797 ) ) ;
#109385=CARTESIAN_POINT ( 'NONE',  ( -15.97531815300800062, 1420.724455713108000, 227.0315652133519961 ) ) ;
#109392=( BOUNDED_CURVE ( )  B_SPLINE_CURVE ( 3, ( #9312, #61952, #79837, #43474 ),
 .UNSPECIFIED., .F., .T. ) 
 B_SPLINE_CURVE_WITH_KNOTS ( ( 4, 4 ),
 ( 4.042232613224455484, 4.145962736327015286 ),
 .UNSPECIFIED. ) 
 CURVE ( )  GEOMETRIC_REPRESENTATION_ITEM ( )  RATIONAL_B_SPLINE_CURVE ( ( 1.000000000000000000, 0.9991035394458830377, 0.9991035394458830377, 1.000000000000000000 ) ) 
 REPRESENTATION_ITEM ( '' )  );
#109401=CARTESIAN_POINT ( 'NONE',  ( -11.68471933269640672, 1398.259520849452201, 203.4197633266676633 ) ) ;
#109405=CARTESIAN_POINT ( 'NONE',  ( 19.89552987158740294, 1507.835503131050018, 229.1917664541709883 ) ) ;
#109408=EDGE_LOOP ( 'NONE', ( #24101, #58313, #69934, #1064 ) ) ;
#109409=CARTESIAN_POINT ( 'NONE',  ( 12.00417144290479854, 1433.690309434259916, 149.9471367831160080 ) ) ;
#109410=CARTESIAN_POINT ( 'NONE',  ( -12.84602301340000174, 1397.681121324029846, 211.4929570555379996 ) ) ;
#109411=CARTESIAN_POINT ( 'NONE',  ( -20.70585539609999870, 1409.636124800530069, 216.1314882506880224 ) ) ;
#109412=VERTEX_POINT ( 'NONE', #89744 ) ;
#109413=CARTESIAN_POINT ( 'NONE',  ( -13.13987858127485531, 1444.766776377808810, 169.3999092927280117 ) ) ;
#109414=FACE_OUTER_BOUND ( 'NONE', #53624, .T. ) ;
#109417=CARTESIAN_POINT ( 'NONE',  ( -14.04733786781709881, 1509.155471822469963, 183.5477982220859872 ) ) ;
#109418=CARTESIAN_POINT ( 'NONE',  ( 1.819731560309999940, 1449.239545743680083, 183.7033410088979792 ) ) ;
#109420=DIRECTION ( 'NONE',  ( 0.7074300732573259864, -0.02470400251981139106, 0.7063514732133259200 ) ) ;
#109421=CARTESIAN_POINT ( 'NONE',  ( 6.882111520678369843, 1396.153389082980084, 200.4809898212910184 ) ) ;
#109422=CARTESIAN_POINT ( 'NONE',  ( 2.500000000000000000, 1419.493307454862588, 138.7644438434529377 ) ) ;
#109423=CARTESIAN_POINT ( 'NONE',  ( 11.86496431830000020, 1432.256597482460165, 149.9819972498980007 ) ) ;
#109424=CARTESIAN_POINT ( 'NONE',  ( 5.674678682617919634, 1509.116656018666845, 180.2329421256601449 ) ) ;
#109426=CARTESIAN_POINT ( 'NONE',  ( 13.06728979724060125, 1434.812079778950192, 149.1114618806330157 ) ) ;
#109427=VERTEX_POINT ( 'NONE', #30384 ) ;
#109428=VERTEX_POINT ( 'NONE', #72418 ) ;
#109429=CARTESIAN_POINT ( 'NONE',  ( 13.49167004114784163, 1444.154101332126402, 169.3566519967024533 ) ) ;
#109430=CARTESIAN_POINT ( 'NONE',  ( -13.14000772899999880, 1461.232465199529770, 232.8227670808980179 ) ) ;
#109436=CARTESIAN_POINT ( 'NONE',  ( -1.804213505890000180, 1410.351307731129964, 186.0507930254979954 ) ) ;
#109443=CARTESIAN_POINT ( 'NONE',  ( -11.00811277969999935, 1409.800196935129861, 189.0350722840979927 ) ) ;
#109445=CARTESIAN_POINT ( 'NONE',  ( 0.1956065449380390009, 1414.913060387399810, 225.1861166566439749 ) ) ;
#109447=CARTESIAN_POINT ( 'NONE',  ( 22.49274844409999830, 1431.770720225350033, 217.6924115464580041 ) ) ;
#109452=CARTESIAN_POINT ( 'NONE',  ( 5.319674812860000657, 1408.795128090730032, 270.4258975186979796 ) ) ;
#109454=CARTESIAN_POINT ( 'NONE',  ( 24.14539179490000365, 1411.115351439130109, 209.1808261004410099 ) ) ;
#109455=CARTESIAN_POINT ( 'NONE',  ( -20.61546995289999984, 1508.365016819430139, 190.3615313974979983 ) ) ;
#109457=CARTESIAN_POINT ( 'NONE',  ( -3.827327156165859723, 1424.046157831530081, 184.1455916618039907 ) ) ;
#109459=CARTESIAN_POINT ( 'NONE',  ( -2.738674389556827293, 1448.013728860840047, 154.7582013136732542 ) ) ;
#109460=CARTESIAN_POINT ( 'NONE',  ( 0.2110708091519999940, 1420.488442819130114, 182.7547195189980016 ) ) ;
#109461=CARTESIAN_POINT ( 'NONE',  ( 1.355725611670679509, 1410.152069949700717, 232.6326878827337339 ) ) ;
#109466=CARTESIAN_POINT ( 'NONE',  ( 18.64646854140000087, 1416.843576337130116, 209.6840263561229847 ) ) ;
#109469=CARTESIAN_POINT ( 'NONE',  ( -5.468507174450000896, 1438.698907215800091, 154.7381958892980265 ) ) ;
#109470=CARTESIAN_POINT ( 'NONE',  ( -22.74837831800000032, 1450.248907260850046, 218.8546552101780094 ) ) ;
#109479=CARTESIAN_POINT ( 'NONE',  ( -0.04719682667970000189, 1477.415580660429896, 229.9352398341980006 ) ) ;
#109480=CARTESIAN_POINT ( 'NONE',  ( 20.40554580410000085, 1454.562377498930118, 223.2165941418979855 ) ) ;
#109481=CARTESIAN_POINT ( 'NONE',  ( 7.129538283582470548, 1439.009953491013448, 154.1072895365704767 ) ) ;
#109482=CARTESIAN_POINT ( 'NONE',  ( -4.649632279085039954, 1420.176633138330089, 186.4708453798239987 ) ) ;
#109484=CARTESIAN_POINT ( 'NONE',  ( 15.29810743031686116, 1420.788480698754483, 227.8099671849163599 ) ) ;
#109485=CARTESIAN_POINT ( 'NONE',  ( 30.86131756593869824, 1435.574936792159860, 135.5979777996759879 ) ) ;
#109487=CARTESIAN_POINT ( 'NONE',  ( -22.59076341920000175, 1432.096319160770008, 217.4686915984279949 ) ) ;
#109488=CARTESIAN_POINT ( 'NONE',  ( -3.415174198469128619, 1451.477971282471344, 184.8447311170799594 ) ) ;
#109490=CARTESIAN_POINT ( 'NONE',  ( -15.82983165089999922, 1415.825112219430139, 226.8803080324979931 ) ) ;
#109495=CARTESIAN_POINT ( 'NONE',  ( 1.514738106409309948, 1507.606285602550088, 186.2052147526660235 ) ) ;
#109499=CARTESIAN_POINT ( 'NONE',  ( 11.60004869885203682, 1428.513469990230988, 134.1600495453299402 ) ) ;
#109500=CARTESIAN_POINT ( 'NONE',  ( -12.94242690632408710, 1444.911164871706660, 186.2050248885010433 ) ) ;
#109501=DIRECTION ( 'NONE',  ( -0.5161917810414702323, 0.8564730265368752926, 0.000000000000000000 ) ) ;
#109503=CARTESIAN_POINT ( 'NONE',  ( -6.462952837710792764, 1416.600481159538049, 231.5900835776368183 ) ) ;
#109504=CARTESIAN_POINT ( 'NONE',  ( -20.69862370072165447, 1450.958657178972317, 144.8102315378076526 ) ) ;
#109505=CARTESIAN_POINT ( 'NONE',  ( 25.56060455230000272, 1435.581316386610069, 136.3167502477979838 ) ) ;
#109506=CARTESIAN_POINT ( 'NONE',  ( -12.95247382709503547, 1442.920873375600650, 169.4286589542791432 ) ) ;
#109507=CARTESIAN_POINT ( 'NONE',  ( -13.86092848849999903, 1410.765486861730096, 227.1170286483979908 ) ) ;
#109509=CARTESIAN_POINT ( 'NONE',  ( 1.032249311045119855, 1415.090956648730071, 191.5469134311629773 ) ) ;
#109510=CARTESIAN_POINT ( 'NONE',  ( 21.47555099491460595, 1509.121809344517942, 226.4561570876979317 ) ) ;
#109512=VERTEX_POINT ( 'NONE', #82997 ) ;
#109515=CARTESIAN_POINT ( 'NONE',  ( -11.74015320060000001, 1428.979986575930070, 144.1938086916980239 ) ) ;
#109516=CARTESIAN_POINT ( 'NONE',  ( -25.90364837339999937, 1446.091283352949858, 225.2740410894980130 ) ) ;
#109518=CARTESIAN_POINT ( 'NONE',  ( -11.84754656309999987, 1433.385444766480077, 150.5314318111979901 ) ) ;
#109522=CARTESIAN_POINT ( 'NONE',  ( -24.86519793529999944, 1440.000684534039920, 210.4205762286579784 ) ) ;
#109524=CARTESIAN_POINT ( 'NONE',  ( 1.245430209930000087, 1451.852423490530100, 183.2837323295979957 ) ) ;
#109526=CARTESIAN_POINT ( 'NONE',  ( -26.22910734341959227, 1509.942088455394014, 194.4759448834997215 ) ) ;
#109527=CARTESIAN_POINT ( 'NONE',  ( -1.401184754297550056E-09, 1416.469379747089988, 239.0597315746249762 ) ) ;
#109528=ORIENTED_EDGE ( 'NONE', *, *, #69348, .F. ) ;
#109530=CARTESIAN_POINT ( 'NONE',  ( -11.79634470412839953, 1428.064288700699990, 147.9921703239390069 ) ) ;
#109532=EDGE_CURVE ( 'NONE', #67527, #105623, #72377, .T. ) ;
#109534=CARTESIAN_POINT ( 'NONE',  ( -6.330345537219999486, 1472.287844838930141, 270.3701849726979844 ) ) ;
#109537=CARTESIAN_POINT ( 'NONE',  ( 41.60492629830280720, 1445.157100822329994, 135.9429468860429893 ) ) ;
#109538=CARTESIAN_POINT ( 'NONE',  ( 18.48114474329999979, 1431.113060387329824, 205.6347121245780158 ) ) ;
#109539=EDGE_CURVE ( 'NONE', #57941, #43234, #88220, .T. ) ;
#109541=ADVANCED_FACE ( 'NONE', ( #49408 ), #37291, .F. ) ;
#109542=DIRECTION ( 'NONE',  ( 0.9894978258369474533, 0.04413734309288668695, -0.1376442792441983920 ) ) ;
#109545=CARTESIAN_POINT ( 'NONE',  ( -12.00303979631470064, 1407.670897247700168, 269.4483317826930033 ) ) ;
#109546=CARTESIAN_POINT ( 'NONE',  ( -13.07010703587889999, 1434.813263339430023, 149.2214592173789640 ) ) ;
#109552=CARTESIAN_POINT ( 'NONE',  ( 4.363122683464830232, 1421.971318488559973, 183.8271341761570170 ) ) ;
#109556=CARTESIAN_POINT ( 'NONE',  ( -16.86146284859999867, 1470.469775084729918, 188.9038085686979969 ) ) ;
#109557=CARTESIAN_POINT ( 'NONE',  ( -16.64506479750550128, 1498.345588598390123, 229.8579787729229906 ) ) ;
#109560=( BOUNDED_SURFACE ( )  B_SPLINE_SURFACE ( 2, 1, ( 
 ( #106842, #31249 ),
 ( #39659, #91156 ),
 ( #64884, #22824 ),
 ( #29591, #73828 ),
 ( #12242, #106308 ),
 ( #97352, #46975 ),
 ( #46431, #65432 ),
 ( #80563, #13877 ),
 ( #90043, #54827 ),
 ( #107955, #72189 ),
 ( #48062, #29060 ) ),
 .UNSPECIFIED., .T., .F., .F. ) 
 B_SPLINE_SURFACE_WITH_KNOTS ( ( 3, 2, 2, 2, 2, 3 ),
 ( 2, 2 ),
 ( 1.721761971665900504, 3.141592653589790007, 4.712388980384689674, 6.283185307179590673, 7.853981633974480125, 8.004947278845490288 ),
 ( -18.71423869390639894, 37.42847738632139709 ),
 .UNSPECIFIED. ) 
 GEOMETRIC_REPRESENTATION_ITEM ( )  RATIONAL_B_SPLINE_SURFACE ( (
 ( 0.9491121336701159317, 0.9491121336701159317),
 ( 0.7352560790313820149, 0.7352560790313820149),
 ( 1.000000000000000000, 1.000000000000000000),
 ( 0.7071067811865510144, 0.7071067811865510144),
 ( 1.000000000000000000, 1.000000000000000000),
 ( 0.7071067811865510144, 0.7071067811865510144),
 ( 1.000000000000000000, 1.000000000000000000),
 ( 0.7071067811865510144, 0.7071067811865510144),
 ( 1.000000000000000000, 1.000000000000000000),
 ( 0.9718507021551689995, 0.9718507021551689995),
 ( 0.9491121336701159317, 0.9491121336701159317) ) ) 
 REPRESENTATION_ITEM ( '' )  SURFACE ( )  );
#109563=CARTESIAN_POINT ( 'NONE',  ( 1.399926847669999974, 1507.072115598929940, 236.8180522793980174 ) ) ;
#109564=EDGE_CURVE ( 'NONE', #43369, #86466, #71666, .T. ) ;
#109566=CARTESIAN_POINT ( 'NONE',  ( -44.13014295924060093, 1440.913052153659919, 270.2165797975040391 ) ) ;
#109569=ORIENTED_EDGE ( 'NONE', *, *, #53884, .T. ) ;
#109571=CARTESIAN_POINT ( 'NONE',  ( 11.55169038159974271, 1474.014209610494845, 269.6090286003602614 ) ) ;
#109572=DIRECTION ( 'NONE',  ( 0.000000000000000000, 6.429975905516270088E-12, -1.000000000000000000 ) ) ;
#109573=FACE_OUTER_BOUND ( 'NONE', #51585, .T. ) ;
#109574=CARTESIAN_POINT ( 'NONE',  ( 0.1595995995380000143, 1486.508831850330125, 181.8147405652979671 ) ) ;
#109575=B_SPLINE_CURVE_WITH_KNOTS ( 'NONE', 5,
 ( #59522, #32100, #33738, #66829, #58964, #100935, #67932, #15809, #84693, #50014, #84146, #41610 ),
 .UNSPECIFIED., .F., .F.,
 ( 6, 3, 3, 6 ),
 ( 6.548035129179999636, 6.565483659539999906, 9.290526163740000953, 11.10277561180000028 ),
 .UNSPECIFIED. ) ;
#109578=CARTESIAN_POINT ( 'NONE',  ( -1.958690691882010393, 1484.245883193570080, 182.9456708303659696 ) ) ;
#109580=CARTESIAN_POINT ( 'NONE',  ( -13.10647016826960076, 1414.913527292460003, 220.1876821406260092 ) ) ;
#109582=ORIENTED_EDGE ( 'NONE', *, *, #12621, .T. ) ;
#109583=CARTESIAN_POINT ( 'NONE',  ( -36.37832874669049232, 1435.767865795990019, 134.4203393042459993 ) ) ;
#109586=CARTESIAN_POINT ( 'NONE',  ( -20.86320816170745474, 1455.053565070798186, 223.5191233675945739 ) ) ;
#109590=CARTESIAN_POINT ( 'NONE',  ( 12.80285994373759983, 1434.672508522010048, 149.2809111413529877 ) ) ;
#109591=CARTESIAN_POINT ( 'NONE',  ( -4.102557340004683084, 1441.363217865950901, 184.4172454785974367 ) ) ;
#109593=CARTESIAN_POINT ( 'NONE',  ( 2.455820327400000114, 1434.541746329560056, 150.3615916412979914 ) ) ;
#109596=CARTESIAN_POINT ( 'NONE',  ( 4.220605471363215067, 1441.596061467261961, 170.5366720304299974 ) ) ;
#109598=CARTESIAN_POINT ( 'NONE',  ( -11.86716023049999968, 1432.353341358199941, 147.6509521729980179 ) ) ;
#109602=CARTESIAN_POINT ( 'NONE',  ( -11.09581607415159965, 1414.913057834419988, 196.3422273742110065 ) ) ;
#109603=CARTESIAN_POINT ( 'NONE',  ( 15.73570983720359884, 1409.462563483369877, 192.9527024472970140 ) ) ;
#109604=CARTESIAN_POINT ( 'NONE',  ( 0.8523351540679999783, 1420.041841627029953, 184.5195079189979879 ) ) ;
#109611=CARTESIAN_POINT ( 'NONE',  ( 18.27629796897370440, 1425.362760113053127, 224.8572713904561624 ) ) ;
#109612=DIRECTION ( 'NONE',  ( 0.01559023541505519597, -0.9998783230245037457, -0.0005326400372547868437 ) ) ;
#109613=CARTESIAN_POINT ( 'NONE',  ( 37.44600398157700027, 1440.913060385919835, 255.3774732117640269 ) ) ;
#109616=CARTESIAN_POINT ( 'NONE',  ( 13.14582612660000116, 1426.028273205230107, 222.1471477697979822 ) ) ;
#109620=CARTESIAN_POINT ( 'NONE',  ( -11.11084040270383611, 1506.426094286139914, 228.0935513073362415 ) ) ;
#109621=CARTESIAN_POINT ( 'NONE',  ( -28.26671300199999948, 1509.671138065330069, 211.0443893778979998 ) ) ;
#109624=CARTESIAN_POINT ( 'NONE',  ( -12.74111629470790064, 1416.830086716310007, 221.9830696278120001 ) ) ;
#109627=LINE ( 'NONE', #100117, #104091 ) ;
#109630=CARTESIAN_POINT ( 'NONE',  ( 25.25200601139999890, 1450.804212501519942, 137.6134970599979965 ) ) ;
#109634=ORIENTED_EDGE ( 'NONE', *, *, #70906, .T. ) ;
#109635=CARTESIAN_POINT ( 'NONE',  ( -1.275851396490000011, 1451.568339848330197, 183.5777291321979874 ) ) ;
#109648=FACE_OUTER_BOUND ( 'NONE', #98339, .T. ) ;
#109650=CARTESIAN_POINT ( 'NONE',  ( 0.7028133466986099531, 1507.119929753229826, 180.9953409562019715 ) ) ;
#109652=CARTESIAN_POINT ( 'NONE',  ( 18.52299501639999946, 1425.669522579430122, 225.2536361859980047 ) ) ;
#109655=CARTESIAN_POINT ( 'NONE',  ( -2.499999926692149987, 1440.210506878179785, 168.7266372007799760 ) ) ;
#109656=CARTESIAN_POINT ( 'NONE',  ( -2.907244326632850040, 1451.960134957139871, 184.7555981325950256 ) ) ;
#109658=ADVANCED_FACE ( 'NONE', ( #71754 ), #56566, .F. ) ;
#109660=CARTESIAN_POINT ( 'NONE',  ( 18.39490484120650038, 1457.283212162220025, 229.1081970229850242 ) ) ;
#109661=B_SPLINE_CURVE_WITH_KNOTS ( 'NONE', 3,
 ( #52824, #35452, #102624, #70752, #25925, #26487, #86954, #19747, #95364, #79132 ),
 .UNSPECIFIED., .F., .F.,
 ( 4, 2, 2, 2, 4 ),
 ( -0.1158481289682099930, -0.06677386518054599651, -0.02553295751034780070, -0.01160833233004980591, -1.224380319353457480E-11 ),
 .UNSPECIFIED. ) ;
#109664=CARTESIAN_POINT ( 'NONE',  ( -8.904037867643029100E-09, 1472.816589274460057, 260.8417418167990149 ) ) ;
#109671=CARTESIAN_POINT ( 'NONE',  ( 14.06094701564179950, 1509.398387556550006, 234.7098584303389828 ) ) ;
#109675=CARTESIAN_POINT ( 'NONE',  ( -5.392707179739999468, 1433.241571820989975, 154.6274174169979858 ) ) ;
#109676=CARTESIAN_POINT ( 'NONE',  ( 11.00428676220000135, 1425.778354413130046, 91.15517427569778874 ) ) ;
#109679=CARTESIAN_POINT ( 'NONE',  ( -25.97192969330459889, 1450.951951750279932, 136.6899769078980000 ) ) ;
#109681=CARTESIAN_POINT ( 'NONE',  ( 27.37758288899999926, 1435.465027219049944, 231.9164972690979880 ) ) ;
#109683=CARTESIAN_POINT ( 'NONE',  ( -17.41030370700000063, 1410.018619281429892, 194.3499987567980156 ) ) ;
#109684=CARTESIAN_POINT ( 'NONE',  ( -1.987375205934570177, 1419.504246183010082, 185.8126813929330012 ) ) ;
#109687=CARTESIAN_POINT ( 'NONE',  ( -20.83123093438729967, 1452.185617773610147, 142.1974481988970069 ) ) ;
#109688=DIRECTION ( 'NONE',  ( 1.989737444810000148E-13, 6.825857443600000379E-15, -1.000000000000000000 ) ) ;
#109690=CARTESIAN_POINT ( 'NONE',  ( -4.438186827019999854E-16, 1395.913060387330006, 217.1218459616979999 ) ) ;
#109691=CARTESIAN_POINT ( 'NONE',  ( 15.69186927393040065, 1421.413580593060033, 227.6163148024349994 ) ) ;
#109693=ORIENTED_EDGE ( 'NONE', *, *, #20739, .F. ) ;
#109697=CARTESIAN_POINT ( 'NONE',  ( -23.32686250069690104, 1409.842844829079922, 209.2659248779790175 ) ) ;
#109698=EDGE_LOOP ( 'NONE', ( #38339, #59030, #5989, #61805, #40942 ) ) ;
#109700=CARTESIAN_POINT ( 'NONE',  ( -43.43522585315017892, 1430.093246065128596, 266.2528640357818404 ) ) ;
#109701=ADVANCED_FACE ( 'NONE', ( #6141 ), #44602, .T. ) ;
#109702=CARTESIAN_POINT ( 'NONE',  ( -2.843430457760000252, 1498.350673094430022, 236.4627852063980242 ) ) ;
#109703=CARTESIAN_POINT ( 'NONE',  ( -20.28645208769999897, 1410.869633620929790, 220.2088169694980024 ) ) ;
#109705=CARTESIAN_POINT ( 'NONE',  ( 43.63532980919219995, 1452.867011165669965, 267.6831642553480037 ) ) ;
#109707=CARTESIAN_POINT ( 'NONE',  ( -17.00189750847108172, 1422.035433323501366, 226.8094376528395344 ) ) ;
#109710=CARTESIAN_POINT ( 'NONE',  ( 18.99566638059803481, 1457.358491571087598, 226.5903252133678620 ) ) ;
#109715=CARTESIAN_POINT ( 'NONE',  ( 26.77909383400000110, 1451.812801000929994, 135.6496118224980023 ) ) ;
#109721=CARTESIAN_POINT ( 'NONE',  ( 6.511209069565670582, 1409.140436818330045, 188.5236114198380051 ) ) ;
#109725=B_SPLINE_CURVE_WITH_KNOTS ( 'NONE', 3,
 ( #93214, #7010, #23795, #93747, #41169, #15396, #7562, #50672, #76421, #65837, #8104, #16483, #91575 ),
 .UNSPECIFIED., .F., .F.,
 ( 4, 2, 2, 1, 2, 2, 4 ),
 ( 0.000000000000000000, 0.2499999999999756306, 0.3749999999999817368, 0.4374999999999787947, 0.4687499999999667488, 0.4999999999999547029, 1.000000000000000000 ),
 .UNSPECIFIED. ) ;
#109727=CARTESIAN_POINT ( 'NONE',  ( 11.43480838300000002, 1425.837049133330083, 122.9428393764980001 ) ) ;
#109729=CARTESIAN_POINT ( 'NONE',  ( 12.57878310069559902, 1415.943166310999914, 222.1097011578140155 ) ) ;
#109732=FACE_OUTER_BOUND ( 'NONE', #72664, .T. ) ;
#109736=CARTESIAN_POINT ( 'NONE',  ( -31.32742177469999945, 1440.913060387330006, 255.3819207742980097 ) ) ;
#109738=CARTESIAN_POINT ( 'NONE',  ( 11.70984135820000027, 1433.749505160629951, 151.0000356945979831 ) ) ;
#109739=CARTESIAN_POINT ( 'NONE',  ( 40.73184307449999864, 1445.563106277920042, 268.3665355199980240 ) ) ;
#109741=DIRECTION ( 'NONE',  ( 0.4547561197925752419, 0.8635678785390505929, 0.2178242196514530993 ) ) ;
#109745=B_SPLINE_CURVE_WITH_KNOTS ( 'NONE', 3,
 ( #56588, #64455, #81217, #89076, #12362, #31367 ),
 .UNSPECIFIED., .F., .F.,
 ( 4, 2, 4 ),
 ( 0.000000000000000000, 0.4999999999999998890, 1.000000000000000000 ),
 .UNSPECIFIED. ) ;
#109747=CARTESIAN_POINT ( 'NONE',  ( -18.85310169809999792, 1486.003537439730053, 189.4173365011979797 ) ) ;
#109748=CARTESIAN_POINT ( 'NONE',  ( -1.065774218729999975E-16, 1426.566393376330097, 144.1938086916980239 ) ) ;
#109749=CARTESIAN_POINT ( 'NONE',  ( -17.22714485659999895, 1409.679743144430176, 224.9962836928979755 ) ) ;
#109750=CARTESIAN_POINT ( 'NONE',  ( 23.51192877309999929, 1410.913812945130076, 211.8293362867379983 ) ) ;
#109751=VECTOR ( 'NONE', #10570, 1000.000000000000000 ) ;
#109757=CARTESIAN_POINT ( 'NONE',  ( -11.80290349340000056, 1415.088016306429836, 221.3076619498979767 ) ) ;
#109759=CARTESIAN_POINT ( 'NONE',  ( 0.2066550540702130068, 1459.231929753809936, 182.9860342603810182 ) ) ;
#109762=CARTESIAN_POINT ( 'NONE',  ( -27.73716673060003757, 1443.913060387329097, 175.8274728504979976 ) ) ;
#109763=EDGE_CURVE ( 'NONE', #17568, #85887, #2984, .T. ) ;
#109766=CARTESIAN_POINT ( 'NONE',  ( -41.56910739857319470, 1442.487573087369810, 134.0999999980959956 ) ) ;
#109768=EDGE_LOOP ( 'NONE', ( #11203, #106859, #62450, #66468, #90491 ) ) ;
#109769=B_SPLINE_CURVE_WITH_KNOTS ( 'NONE', 5,
 ( #29300, #64035, #87574, #80816, #71356, #11417 ),
 .UNSPECIFIED., .F., .F.,
 ( 6, 6 ),
 ( 0.000000000000000000, 1.000000000000000000 ),
 .UNSPECIFIED. ) ;
#109775=EDGE_CURVE ( 'NONE', #86349, #101781, #48156, .T. ) ;
#109778=CARTESIAN_POINT ( 'NONE',  ( 21.30047364570000212, 1471.312091223629977, 210.0334653296820022 ) ) ;
#109779=CARTESIAN_POINT ( 'NONE',  ( -5.362304121457834860, 1422.288402133340242, 142.1498578916476561 ) ) ;
#109786=CARTESIAN_POINT ( 'NONE',  ( -32.69751076149999847, 1451.617800104529806, 135.6222252852979864 ) ) ;
#109788=CARTESIAN_POINT ( 'NONE',  ( 2.370970874524633398, 1427.002265528473799, 137.0999999980980135 ) ) ;
#109789=ORIENTED_EDGE ( 'NONE', *, *, #34350, .F. ) ;
#109791=CARTESIAN_POINT ( 'NONE',  ( -19.66031314052480994, 1410.960623777707269, 221.6379339483827664 ) ) ;
#109795=CARTESIAN_POINT ( 'NONE',  ( 41.79939186130401652, 1444.333674645975179, 269.6436966550891157 ) ) ;
#109797=CARTESIAN_POINT ( 'NONE',  ( 17.96451342846462396, 1434.943382339013397, 215.4098532707286040 ) ) ;
#109806=FACE_OUTER_BOUND ( 'NONE', #104879, .T. ) ;
#109809=CARTESIAN_POINT ( 'NONE',  ( 14.00912983899999986, 1416.839648759230158, 196.3913567892980154 ) ) ;
#109811=ORIENTED_EDGE ( 'NONE', *, *, #69860, .T. ) ;
#109816=CARTESIAN_POINT ( 'NONE',  ( -23.61553526509999656, 1410.914738123429970, 206.7820667545679783 ) ) ;
#109817=CARTESIAN_POINT ( 'NONE',  ( -11.71570024223670003, 1426.293107577299907, 142.6799693210089970 ) ) ;
#109818=CARTESIAN_POINT ( 'NONE',  ( 16.23605858256030032, 1409.581384769300030, 192.4955713889560229 ) ) ;
#109820=CARTESIAN_POINT ( 'NONE',  ( 40.27308140560000282, 1443.612049536910035, 137.1163288290979949 ) ) ;
#109821=CARTESIAN_POINT ( 'NONE',  ( -19.16279443490000034, 1411.291491730330108, 262.3396854780979766 ) ) ;
#109822=DIRECTION ( 'NONE',  ( 0.000000000000000000, 1.000000000000000000, 0.000000000000000000 ) ) ;
#109823=CARTESIAN_POINT ( 'NONE',  ( 14.10180166660902046, 1462.573205505089845, 230.5089236422518582 ) ) ;
#109824=CARTESIAN_POINT ( 'NONE',  ( 34.94829774772319553, 1451.625365366340020, 134.0999999983029909 ) ) ;
#109825=CARTESIAN_POINT ( 'NONE',  ( -35.95777000360060072, 1437.416693626100141, 136.5372231441070028 ) ) ;
#109828=EDGE_CURVE ( 'NONE', #22768, #66538, #41321, .T. ) ;
#109834=CARTESIAN_POINT ( 'NONE',  ( 14.45119567767109992, 1485.899027755930092, 225.7245081177429995 ) ) ;
#109837=EDGE_CURVE ( 'NONE', #84627, #105413, #44197, .T. ) ;
#109840=B_SPLINE_CURVE_WITH_KNOTS ( 'NONE', 3,
 ( #57519, #64826, #4879, #99475, #55868, #56403, #46919, #108451, #107890, #82699, #13812, #14369, #48562, #65917, #31182, #65369, #13262, #5988, #30639, #39594, #81575, #40137, #90535, #5437, #14919 ),
 .UNSPECIFIED., .F., .F.,
 ( 4, 2, 2, 1, 1, 2, 2, 2, 2, 1, 1, 1, 2, 2, 4 ),
 ( 0.000000000000000000, 0.2499999999954249930, 0.3749999999931376005, 0.4374999999919982896, 0.4687499999916037163, 0.4843749999914018223, 0.4999999999911999282, 0.6249999999875969214, 0.6874999999857954736, 0.7187499999850445187, 0.7343749999848121490, 0.7421874999846904686, 0.7460937499846346244, 0.7499999999845787801, 1.000000000000000000 ),
 .UNSPECIFIED. ) ;
#109842=CARTESIAN_POINT ( 'NONE',  ( 33.91369114129039986, 1451.728768196330066, 134.7402677064790169 ) ) ;
#109843=CARTESIAN_POINT ( 'NONE',  ( 12.78752272718304184, 1416.843574568078566, 222.7044121896790898 ) ) ;
#109844=CARTESIAN_POINT ( 'NONE',  ( 26.26433425849999992, 1440.617482597780054, 137.6222147125980086 ) ) ;
#109845=ADVANCED_FACE ( 'NONE', ( #67051 ), #6020, .F. ) ;
#109848=VERTEX_POINT ( 'NONE', #69076 ) ;
#109851=VERTEX_POINT ( 'NONE', #47026 ) ;
#109852=CARTESIAN_POINT ( 'NONE',  ( 11.76320837242760042, 1426.958789830729984, 145.9773750732420012 ) ) ;
#109854=ORIENTED_EDGE ( 'NONE', *, *, #102818, .F. ) ;
#109855=CARTESIAN_POINT ( 'NONE',  ( -13.46339118210000052, 1415.263254644630024, 221.0797442403980142 ) ) ;
#109856=CARTESIAN_POINT ( 'NONE',  ( -14.26333330936780008, 1452.396687514240057, 223.0069981058830137 ) ) ;
#109858=CARTESIAN_POINT ( 'NONE',  ( 23.96695357696606266, 1411.114076150693109, 208.3039881944807803 ) ) ;
#109859=CARTESIAN_POINT ( 'NONE',  ( -13.15607067979999911, 1416.813004075730078, 221.9084248872979970 ) ) ;
#109862=CARTESIAN_POINT ( 'NONE',  ( -16.30342780150716209, 1410.854766001639064, 191.5161596899749838 ) ) ;
#109864=CARTESIAN_POINT ( 'NONE',  ( 22.94534059460660202, 1420.146124040419863, 206.2024909355390037 ) ) ;
#109865=CARTESIAN_POINT ( 'NONE',  ( 17.39940665230000150, 1459.341270389529882, 228.5023076377979976 ) ) ;
#109867=CARTESIAN_POINT ( 'NONE',  ( -4.785922751469102288, 1422.261607323150656, 184.7437580134849782 ) ) ;
#109869=VERTEX_POINT ( 'NONE', #4466 ) ;
#109870=CARTESIAN_POINT ( 'NONE',  ( 18.33041286839819861, 1424.507522803520033, 223.5605584007410016 ) ) ;
#109873=CARTESIAN_POINT ( 'NONE',  ( -3.011021552054556238, 1485.803647523245445, 182.4970978269045929 ) ) ;
#109874=CARTESIAN_POINT ( 'NONE',  ( -11.31259290968401743, 1425.497384986706493, 138.7251079064614032 ) ) ;
#109876=ORIENTED_EDGE ( 'NONE', *, *, #101553, .F. ) ;
#109879=CARTESIAN_POINT ( 'NONE',  ( -10.84157467490000037, 1425.079916389830032, 146.2720446874980098 ) ) ;
#109880=CARTESIAN_POINT ( 'NONE',  ( 19.04231260082879729, 1456.923026149589759, 225.4260409396169962 ) ) ;
#109881=DIRECTION ( 'NONE',  ( 0.000000000000000000, 1.000000000000000000, 0.000000000000000000 ) ) ;
#109884=CARTESIAN_POINT ( 'NONE',  ( 7.269326417459999412, 1410.392938076930022, 230.7475538776979818 ) ) ;
#109885=CARTESIAN_POINT ( 'NONE',  ( -23.22700599630000085, 1495.365700136630039, 222.7559110526980248 ) ) ;
#109886=CARTESIAN_POINT ( 'NONE',  ( -3.912719417411558709, 1422.010005319424181, 137.0999999983282862 ) ) ;
#109890=CARTESIAN_POINT ( 'NONE',  ( 6.204617315079999251, 1406.081877976730084, 268.4675683214979927 ) ) ;
#109892=B_SPLINE_SURFACE_WITH_KNOTS ( 'NONE', 5, 5, ( 
 ( #59729, #6557, #109030, #32313, #75965, #23884, #49679, #50765, #92211, #57536, #110117, #84362 ),
 ( #93849, #85445, #40708, #67036, #84900, #42926, #101143, #76512, #41263, #110662, #34511, #33955 ),
 ( #51308, #17120, #391, #24437, #68689, #91660, #14935, #15483, #83262, #74880, #100602, #66496 ),
 ( #58625, #92756, #35060, #95524, #1477, #27768, #27221, #70361, #36724, #94398, #78165, #61959 ),
 ( #52439, #78729, #61402, #87125, #18795, #26652, #44584, #60851, #937, #69804, #36177, #45148 ),
 ( #86567, #69242, #103922, #53547, #52991, #60280, #87694, #77625, #43480, #51881, #96074, #9861 ),
 ( #10414, #44029, #103350, #10975, #2044, #35609, #104474, #94976, #105034, #18244, #28324, #19348 ),
 ( #79289, #86017, #70918, #9317, #2599, #102794, #26091, #17678, #56961, #15470, #73202, #98391 ),
 ( #100039, #83247, #108453, #2840, #64828, #40140, #82701, #6542, #13814, #21661, #107892, #49665 ),
 ( #90537, #66479, #36963, #55870, #14371, #5439, #72658, #31734, #48564, #57521, #22757, #91646 ),
 ( #23329, #92197, #30641, #32295, #5990, #14921, #98936, #47999, #47453, #56405, #107346, #74323 ),
 ( #22210, #49115, #65919, #40694, #4881, #74866, #109012, #81577, #106786, #82138, #64268, #100588 ) ),
 .UNSPECIFIED., .F., .F., .F.,
 ( 6, 3, 3, 6 ),
 ( 6, 3, 3, 6 ),
 ( 12.92374750619999979, 13.99906740309999975, 15.76224410990000102, 17.24244726289999718 ),
 ( 0.000000000000000000, 0.3239695544339999955, 0.9719086633019999866, 1.551787865330000127 ),
 .UNSPECIFIED. ) ;
#109893=CARTESIAN_POINT ( 'NONE',  ( 19.90169804190000136, 1430.300817687629888, 195.1941537691980102 ) ) ;
#109894=CARTESIAN_POINT ( 'NONE',  ( 19.36767678366642897, 1425.674430346010013, 222.2074193912012277 ) ) ;
#109897=CARTESIAN_POINT ( 'NONE',  ( -1.584158815879999960, 1451.558453897129993, 184.0315954900979989 ) ) ;
#109900=CARTESIAN_POINT ( 'NONE',  ( -14.26903107030000051, 1444.886608432469984, 188.6883752183980221 ) ) ;
#109904=CARTESIAN_POINT ( 'NONE',  ( 1.458953924596269935, 1496.945680665030068, 181.5568043570760324 ) ) ;
#109909=CARTESIAN_POINT ( 'NONE',  ( -7.053447956369999439, 1475.362404503930065, 269.0260191948979696 ) ) ;
#109913=CARTESIAN_POINT ( 'NONE',  ( 17.60566278643909754, 1410.878816881569946, 223.9222694885750116 ) ) ;
#109916=AXIS2_PLACEMENT_3D ( 'NONE', #16365, #67929, #76307 ) ;
#109917=CARTESIAN_POINT ( 'NONE',  ( 12.15368974863659979, 1416.134159098650116, 223.4664122540619928 ) ) ;
#109918=B_SPLINE_SURFACE_WITH_KNOTS ( 'NONE', 5, 5, ( 
 ( #72059, #106175, #55799, #29455, #56331, #63651, #38408, #97766, #21038 ),
 ( #46845, #89374, #80974, #106712, #30002, #4804, #73129, #49592, #74792 ),
 ( #76428, #59642, #84811, #24891, #7570, #34427, #51228, #6471, #75884 ),
 ( #40621, #91581, #58543, #59098, #15946, #32767, #17030, #42833, #102168 ),
 ( #41724, #24357, #110032, #68057, #33308, #67502, #93222, #68600, #7019 ),
 ( #16489, #76994, #15403, #83181, #50679, #66950, #8656, #101606, #8110 ) ),
 .UNSPECIFIED., .F., .F., .F.,
 ( 6, 6 ),
 ( 6, 3, 6 ),
 ( 32.85731390589999990, 45.45696239520000148 ),
 ( 0.000000000000000000, 1.000000000000000000, 2.000000000000000000 ),
 .UNSPECIFIED. ) ;
#109922=CARTESIAN_POINT ( 'NONE',  ( -20.89362284670000136, 1409.642681774629864, 203.1985663301079796 ) ) ;
#109927=EDGE_CURVE ( 'NONE', #22669, #22237, #102988, .T. ) ;
#109929=CARTESIAN_POINT ( 'NONE',  ( 0.8167354255590000278, 1432.353341358199941, 150.3995506339979897 ) ) ;
#109935=CARTESIAN_POINT ( 'NONE',  ( 11.71530569028189994, 1426.709924042370176, 142.6142981130810199 ) ) ;
#109939=CARTESIAN_POINT ( 'NONE',  ( -17.12480635412540053, 1507.616838219199963, 224.4390396745509975 ) ) ;
#109942=CARTESIAN_POINT ( 'NONE',  ( -10.63125103579607078, 1398.228151311645888, 201.6093364865327544 ) ) ;
#109946=CARTESIAN_POINT ( 'NONE',  ( 20.84681744068790010, 1509.577347247510033, 229.6818225510970137 ) ) ;
#109950=CARTESIAN_POINT ( 'NONE',  ( 11.49040827066960091, 1434.209370592019923, 151.3710404996469947 ) ) ;
#109951=CARTESIAN_POINT ( 'NONE',  ( -4.919915858649999585, 1396.145435506330159, 220.1243708699980175 ) ) ;
#109955=CARTESIAN_POINT ( 'NONE',  ( 22.20822569604427343, 1509.700626114282386, 228.6180359268219320 ) ) ;
#109958=CARTESIAN_POINT ( 'NONE',  ( -14.35518320136639936, 1509.483853104240097, 182.9676327163749932 ) ) ;
#109960=CARTESIAN_POINT ( 'NONE',  ( 1.151973313230000073, 1429.774640056330099, 184.3913675471979730 ) ) ;
#109964=CARTESIAN_POINT ( 'NONE',  ( 3.572247405320189806, 1396.037806015820024, 198.6941501537289980 ) ) ;
#109965=CARTESIAN_POINT ( 'NONE',  ( 1.552659050380000183, 1415.628674276829770, 190.6570100179979761 ) ) ;
#109967=CARTESIAN_POINT ( 'NONE',  ( 11.29851010420000001, 1432.096855580479996, 151.5187265218980315 ) ) ;
#109968=CARTESIAN_POINT ( 'NONE',  ( 17.22592475670000312, 1443.501467202829872, 162.9227486557980171 ) ) ;
#109970=CARTESIAN_POINT ( 'NONE',  ( 13.09831360813569923, 1434.825884568560241, 149.1955092924029884 ) ) ;
#109972=ORIENTED_EDGE ( 'NONE', *, *, #18142, .T. ) ;
#109973=CARTESIAN_POINT ( 'NONE',  ( -18.54207416890000104, 1507.885690544229874, 229.7224895538980149 ) ) ;
#109974=CARTESIAN_POINT ( 'NONE',  ( -8.652254019400000828, 1463.299883665429888, 235.0794778895980244 ) ) ;
#109978=EDGE_CURVE ( 'NONE', #72755, #14771, #85999, .T. ) ;
#109983=ORIENTED_EDGE ( 'NONE', *, *, #61139, .T. ) ;
#109985=ORIENTED_EDGE ( 'NONE', *, *, #20651, .F. ) ;
#109987=CARTESIAN_POINT ( 'NONE',  ( -18.64442766460000200, 1507.939506224430033, 229.7217055948979976 ) ) ;
#109988=CARTESIAN_POINT ( 'NONE',  ( -2.747668638985504952, 1410.389839720919781, 269.3346462040586857 ) ) ;
#109990=CARTESIAN_POINT ( 'NONE',  ( -0.1222452018727299833, 1415.427621830080170, 226.6817715979609886 ) ) ;
#109992=CARTESIAN_POINT ( 'NONE',  ( 24.46211382750000141, 1438.319209241250064, 213.4123708239580139 ) ) ;
#109993=CARTESIAN_POINT ( 'NONE',  ( -0.03314839539225959697, 1508.987035968580130, 209.1276091456630013 ) ) ;
#109998=CARTESIAN_POINT ( 'NONE',  ( 24.05620271129999921, 1410.714389761430084, 209.4728325500950348 ) ) ;
#109999=CARTESIAN_POINT ( 'NONE',  ( -22.37111836880000126, 1509.698977978930088, 189.8981514860979871 ) ) ;
#110003=CARTESIAN_POINT ( 'NONE',  ( 0.06395050066389999788, 1420.208574609930110, 183.9020924998980036 ) ) ;
#110004=CARTESIAN_POINT ( 'NONE',  ( 0.9810389212584773588, 1409.219252835773659, 232.2248046168253381 ) ) ;
#110009=CARTESIAN_POINT ( 'NONE',  ( -1.621602494910000178E-09, 1472.348800621829923, 259.9484879168979887 ) ) ;
#110012=CARTESIAN_POINT ( 'NONE',  ( -5.429836194910000025, 1436.698278407169937, 154.7014982151980291 ) ) ;
#110013=CARTESIAN_POINT ( 'NONE',  ( -23.75643893390000017, 1446.680031664370063, 215.2230810373079919 ) ) ;
#110014=CARTESIAN_POINT ( 'NONE',  ( 4.363122647530000009, 1407.471318475729959, 121.6099336315979969 ) ) ;
#110019=EDGE_LOOP ( 'NONE', ( #91059, #65183, #12709, #96050 ) ) ;
#110021=CARTESIAN_POINT ( 'NONE',  ( 28.77213280029999964, 1509.917805404229966, 206.8662417159980293 ) ) ;
#110022=CARTESIAN_POINT ( 'NONE',  ( -4.494715636143079854E-06, 1472.045054924830083, 270.0713875376969781 ) ) ;
#110026=CARTESIAN_POINT ( 'NONE',  ( 14.68860525048159715, 1420.364114750980889, 228.1328174510751694 ) ) ;
#110027=CARTESIAN_POINT ( 'NONE',  ( 29.68682351698860344, 1436.863057280969997, 136.6924149577619971 ) ) ;
#110028=CARTESIAN_POINT ( 'NONE',  ( 39.55339567453099647, 1446.835654864889875, 136.6686472316449965 ) ) ;
#110029=CARTESIAN_POINT ( 'NONE',  ( 20.23078144684548718, 1506.575640308540414, 218.0217183349242589 ) ) ;
#110030=CARTESIAN_POINT ( 'NONE',  ( -43.12842832595762133, 1452.290486921479896, 269.0450826265717410 ) ) ;
#110032=CARTESIAN_POINT ( 'NONE',  ( 10.69931594910000072, 1509.229557744529984, 182.5718536335980104 ) ) ;
#110036=CARTESIAN_POINT ( 'NONE',  ( -38.81129961821237373, 1452.619208713947955, 269.5899325438009555 ) ) ;
#110039=CARTESIAN_POINT ( 'NONE',  ( -42.31040111291903827, 1428.094689011069022, 269.0673684584702414 ) ) ;
#110041=CARTESIAN_POINT ( 'NONE',  ( 16.74002313133309983, 1501.349413233449923, 188.2918665645719614 ) ) ;
#110042=CARTESIAN_POINT ( 'NONE',  ( -0.1199520561000000096, 1415.404073712830041, 233.4412207362979927 ) ) ;
#110044=CARTESIAN_POINT ( 'NONE',  ( -13.09467007730180832, 1444.805799845968522, 186.4212311027728219 ) ) ;
#110049=CARTESIAN_POINT ( 'NONE',  ( -7.843739966816699827, 1451.394674706588376, 152.9912049652007795 ) ) ;
#110050=CARTESIAN_POINT ( 'NONE',  ( -16.40028066370599902, 1414.913057860449953, 208.9659912899270182 ) ) ;
#110051=CARTESIAN_POINT ( 'NONE',  ( 25.44703061359999907, 1435.463407790350175, 136.0943506319979974 ) ) ;
#110054=CARTESIAN_POINT ( 'NONE',  ( -0.3610913072858399908, 1416.520646088689773, 191.0797031976740072 ) ) ;
#110057=ORIENTED_EDGE ( 'NONE', *, *, #13060, .F. ) ;
#110061=CARTESIAN_POINT ( 'NONE',  ( -27.78550214639999894, 1444.553010677309885, 231.7059331051979996 ) ) ;
#110062=CARTESIAN_POINT ( 'NONE',  ( -20.60186841840000227, 1507.925363662629934, 190.3874517655979730 ) ) ;
#110063=CARTESIAN_POINT ( 'NONE',  ( -0.2658540493943280514, 1507.120020986029886, 237.3289608297170048 ) ) ;
#110065=CARTESIAN_POINT ( 'NONE',  ( -2.497537340894446789, 1421.157573660655089, 184.9539988175752114 ) ) ;
#110067=CARTESIAN_POINT ( 'NONE',  ( -24.68077627620000314, 1437.736158917830153, 210.5119845518579780 ) ) ;
#110069=CARTESIAN_POINT ( 'NONE',  ( 1.812234975289999994, 1451.648984562529904, 183.4223051748979856 ) ) ;
#110074=ORIENTED_EDGE ( 'NONE', *, *, #77433, .F. ) ;
#110078=CARTESIAN_POINT ( 'NONE',  ( -4.112861762809999711, 1471.442216374229929, 269.6167275226979996 ) ) ;
#110079=CARTESIAN_POINT ( 'NONE',  ( 13.01067395679109318, 1434.788365234622461, 146.9710503661439134 ) ) ;
#110081=CARTESIAN_POINT ( 'NONE',  ( 17.23446452470000168, 1453.313060387329870, 198.3385369815979971 ) ) ;
#110083=ADVANCED_FACE ( 'NONE', ( #48684 ), #99881, .T. ) ;
#110084=B_SPLINE_SURFACE_WITH_KNOTS ( 'NONE', 5, 5, ( 
 ( #81313, #81865, #6808, #23050, #32579, #72938 ),
 ( #22485, #66755, #48852, #65644, #100329, #39876 ),
 ( #5166, #6269, #109295, #39324, #40967, #31464 ),
 ( #30915, #65094, #64555, #99206, #56685, #57258 ),
 ( #40416, #99760, #23614, #90264, #108172, #75147 ),
 ( #4628, #91923, #38764, #107078, #90821, #14103 ) ),
 .UNSPECIFIED., .F., .F., .F.,
 ( 6, 6 ),
 ( 6, 6 ),
 ( 0.8310181115189999579, 1.360694072900000107 ),
 ( 0.000000000000000000, 2.000000000000000000 ),
 .UNSPECIFIED. ) ;
#110085=CARTESIAN_POINT ( 'NONE',  ( 0.000000000000000000, 0.000000000000000000, 0.000000000000000000 ) ) ;
#110088=CARTESIAN_POINT ( 'NONE',  ( 28.77729953137099983, 1509.917985831029910, 206.0039978706130057 ) ) ;
#110089=CARTESIAN_POINT ( 'NONE',  ( -8.302495336826780203, 1407.043756550310036, 269.4752719639240013 ) ) ;
#110090=CARTESIAN_POINT ( 'NONE',  ( -13.47774476437770019, 1434.953314453749954, 149.0527405834899923 ) ) ;
#110091=ORIENTED_EDGE ( 'NONE', *, *, #44010, .F. ) ;
#110094=ORIENTED_EDGE ( 'NONE', *, *, #20171, .T. ) ;
#110095=CARTESIAN_POINT ( 'NONE',  ( 4.743542324458120518, 1422.215256140715837, 184.1963053778127914 ) ) ;
#110098=CARTESIAN_POINT ( 'NONE',  ( -18.56504074879999777, 1470.474274205130087, 190.0315648486979967 ) ) ;
#110099=CARTESIAN_POINT ( 'NONE',  ( -17.91320311087370243, 1507.617078275819949, 229.7141967011020256 ) ) ;
#110102=AXIS2_PLACEMENT_3D ( 'NONE', #103981, #61459, #86627 ) ;
#110104=B_SPLINE_CURVE_WITH_KNOTS ( 'NONE', 3,
 ( #39619, #100066, #16574, #108472, #41815, #74887, #16041, #15489, #109037, #84369, #75971, #75444, #6565 ),
 .UNSPECIFIED., .F., .F.,
 ( 4, 2, 2, 1, 2, 2, 4 ),
 ( 0.000000000000000000, 0.2500000000001970091, 0.3750000000002713385, 0.4375000000003243517, 0.4687500000002935430, 0.5000000000002627898, 1.000000000000000000 ),
 .UNSPECIFIED. ) ;
#110105=CARTESIAN_POINT ( 'NONE',  ( -27.89972997509999786, 1508.077281474930032, 206.8466243103179920 ) ) ;
#110106=CARTESIAN_POINT ( 'NONE',  ( -4.270560985520866382, 1421.938260711448493, 185.0877191533315909 ) ) ;
#110109=CARTESIAN_POINT ( 'NONE',  ( -5.563412915829999861, 1409.046699355029887, 195.8153601168980060 ) ) ;
#110111=DIRECTION ( 'NONE',  ( 0.000000000000000000, 0.000000000000000000, 1.000000000000000000 ) ) ;
#110114=CARTESIAN_POINT ( 'NONE',  ( 21.52036871800000029, 1488.680653137030049, 224.0828341895980031 ) ) ;
#110117=CARTESIAN_POINT ( 'NONE',  ( -24.97886932509999980, 1436.441184281979986, 137.9166797883979996 ) ) ;
#110118=CARTESIAN_POINT ( 'NONE',  ( -0.2610041142439999962, 1485.912415289430101, 181.7937759989980009 ) ) ;
#110121=CARTESIAN_POINT ( 'NONE',  ( 5.477776093029999238, 1439.067881875560033, 154.7441050454979745 ) ) ;
#110123=CARTESIAN_POINT ( 'NONE',  ( -13.20369377719999981, 1414.913528139930122, 220.1254046489979999 ) ) ;
#110126=CARTESIAN_POINT ( 'NONE',  ( -42.60628462810000627, 1443.705283505679745, 134.0999992373979808 ) ) ;
#110128=DIRECTION ( 'NONE',  ( 0.9995238204273075855, -0.03085664269485739394, -3.333398116331567129E-08 ) ) ;
#110131=CARTESIAN_POINT ( 'NONE',  ( -22.81398894436890856, 1509.728857822366308, 227.9950205443984714 ) ) ;
#110132=CARTESIAN_POINT ( 'NONE',  ( -4.094299838186481466, 1441.313231385115614, 184.5078324159681529 ) ) ;
#110134=DIRECTION ( 'NONE',  ( 0.1402804634178727861, 0.9901118076173351934, 0.000000000000000000 ) ) ;
#110137=CARTESIAN_POINT ( 'NONE',  ( -15.08447935729999934, 1409.953164787530113, 226.5286084827979778 ) ) ;
#110139=DIRECTION ( 'NONE',  ( 1.000000000000000000, 0.000000000000000000, 0.000000000000000000 ) ) ;
#110140=CARTESIAN_POINT ( 'NONE',  ( 20.28559703379999846, 1508.605287559729959, 189.2542286951979804 ) ) ;
#110143=CARTESIAN_POINT ( 'NONE',  ( -12.61618840270000064, 1416.831305841230005, 194.9199445040979981 ) ) ;
#110145=CARTESIAN_POINT ( 'NONE',  ( 0.8012822335670000129, 1420.474755016030258, 184.0519104804979804 ) ) ;
#110151=CARTESIAN_POINT ( 'NONE',  ( 8602.628222781668228, 50.13405481564041821, -10923.45535519340592 ) ) ;
#110155=EDGE_CURVE ( 'NONE', #40901, #76159, #102069, .T. ) ;
#110157=CARTESIAN_POINT ( 'NONE',  ( -11.94046459599999999, 1438.194204504490017, 147.6340003373980210 ) ) ;
#110158=DIRECTION ( 'NONE',  ( 0.9417419115949662300, -0.2378257470769920556, 0.2378257470769920556 ) ) ;
#110159=EDGE_CURVE ( 'NONE', #100575, #9577, #101462, .T. ) ;
#110162=ORIENTED_EDGE ( 'NONE', *, *, #34584, .T. ) ;
#110164=CARTESIAN_POINT ( 'NONE',  ( 1.546990765144379942, 1416.765224585179794, 190.2255853430220043 ) ) ;
#110166=CARTESIAN_POINT ( 'NONE',  ( -24.40604034560000102, 1441.493461323560041, 212.0691198047580031 ) ) ;
#110174=CARTESIAN_POINT ( 'NONE',  ( 7.282399919470000427, 1452.222616508330020, 153.1973960492980211 ) ) ;
#110175=CARTESIAN_POINT ( 'NONE',  ( -26.86204968941349946, 1508.007394745769943, 212.0120970035400205 ) ) ;
#110179=CARTESIAN_POINT ( 'NONE',  ( 12.78776258895000062, 1416.851343899079893, 222.7045348340550106 ) ) ;
#110184=CARTESIAN_POINT ( 'NONE',  ( 15.16579360867039838, 1509.443749158599985, 234.3045273943520215 ) ) ;
#110186=CARTESIAN_POINT ( 'NONE',  ( 40.00035472543419957, 1441.740890375260051, 136.9051897632780026 ) ) ;
#110191=CARTESIAN_POINT ( 'NONE',  ( -12.84238138274280061, 1435.935700660240400, 150.8114831378814245 ) ) ;
#110194=CARTESIAN_POINT ( 'NONE',  ( 2.776832761270000116, 1409.010029526630206, 186.6898676387980061 ) ) ;
#110196=CARTESIAN_POINT ( 'NONE',  ( -2.711917821514580051, 1440.323576713389912, 158.1830662651330215 ) ) ;
#110197=FACE_OUTER_BOUND ( 'NONE', #59647, .T. ) ;
#110201=CARTESIAN_POINT ( 'NONE',  ( -2.446787376320000096, 1432.353341358199941, 150.2884730787980061 ) ) ;
#110202=CARTESIAN_POINT ( 'NONE',  ( -23.69678315977305871, 1436.213473500231430, 212.2034013915424566 ) ) ;
#110203=CARTESIAN_POINT ( 'NONE',  ( 22.06852505278052234, 1506.535970898695041, 209.0957427188783981 ) ) ;
#110204=DIRECTION ( 'NONE',  ( 0.000000000000000000, 1.000000000000000000, 0.000000000000000000 ) ) ;
#110205=CARTESIAN_POINT ( 'NONE',  ( -3.496551860115360160E-09, 1471.729463454729967, 258.3617253003269525 ) ) ;
#110206=CARTESIAN_POINT ( 'NONE',  ( -19.96725921898470091, 1487.369853937069820, 190.9830490477359888 ) ) ;
#110209=CARTESIAN_POINT ( 'NONE',  ( -0.8130780850230000523, 1417.377578703830068, 235.4819908353979940 ) ) ;
#110214=CARTESIAN_POINT ( 'NONE',  ( -46.23755058181890121, 1439.409989939530078, 267.5908672125710268 ) ) ;
#110215=CARTESIAN_POINT ( 'NONE',  ( 13.50635050315699992, 1508.609632639959955, 233.4266690729490108 ) ) ;
#110218=CARTESIAN_POINT ( 'NONE',  ( 0.000000000000000000, 1413.913060387330006, 217.1218459616979999 ) ) ;
#110221=CARTESIAN_POINT ( 'NONE',  ( -26.59992281200619857, 1451.967265226159952, 135.1794589613959943 ) ) ;
#110223=CARTESIAN_POINT ( 'NONE',  ( 3.960029701070000296, 1420.509147081630090, 221.4103262571979940 ) ) ;
#110225=FACE_OUTER_BOUND ( 'NONE', #74725, .T. ) ;
#110226=CARTESIAN_POINT ( 'NONE',  ( 14.45750538832999865, 1416.828039266780024, 196.8520486936070029 ) ) ;
#110227=CARTESIAN_POINT ( 'NONE',  ( -7.332394679680000704E-08, 1421.529510530429889, 216.2239750317280311 ) ) ;
#110232=CARTESIAN_POINT ( 'NONE',  ( -1.204647661935780212, 1410.042122733069846, 269.8655116434729848 ) ) ;
#110233=CARTESIAN_POINT ( 'NONE',  ( 15.46640642006999933, 1422.315519798870127, 228.3555397929160051 ) ) ;
#110235=ORIENTED_EDGE ( 'NONE', *, *, #87921, .T. ) ;
#110237=CARTESIAN_POINT ( 'NONE',  ( -23.97615151247089926, 1411.113891529490047, 209.8899454678769985 ) ) ;
#110242=CARTESIAN_POINT ( 'NONE',  ( -20.44190531641500286, 1488.934990366839884, 192.7748267833920011 ) ) ;
#110243=CARTESIAN_POINT ( 'NONE',  ( -20.24945462270000007, 1415.849806780530116, 220.8573330491979902 ) ) ;
#110244=CIRCLE ( 'NONE', #101265, 7.975189853890007896 ) ;
#110246=CARTESIAN_POINT ( 'NONE',  ( 37.03850270579130211, 1462.024743436390054, 267.2720586370879801 ) ) ;
#110248=CARTESIAN_POINT ( 'NONE',  ( -16.45994915654801360, 1421.286113174233151, 226.9925930846744677 ) ) ;
#110250=ORIENTED_EDGE ( 'NONE', *, *, #55112, .F. ) ;
#110253=CARTESIAN_POINT ( 'NONE',  ( 22.71667399460000425, 1409.715173893529936, 208.6485712393049994 ) ) ;
#110254=VERTEX_POINT ( 'NONE', #205 ) ;
#110256=CARTESIAN_POINT ( 'NONE',  ( 27.01380162286760012, 1450.681224429609983, 136.4483868285099959 ) ) ;
#110262=CARTESIAN_POINT ( 'NONE',  ( 6.718545715849139732, 1409.147677173569946, 188.6149336500920128 ) ) ;
#110265=CARTESIAN_POINT ( 'NONE',  ( 1.131675640069840005, 1451.349608238679821, 182.9318126509270144 ) ) ;
#110269=ORIENTED_EDGE ( 'NONE', *, *, #35755, .T. ) ;
#110275=EDGE_CURVE ( 'NONE', #59045, #101455, #56081, .T. ) ;
#110277=B_SPLINE_CURVE_WITH_KNOTS ( 'NONE', 3,
 ( #90890, #14731, #14175, #4153, #48360, #74665, #6339, #46719, #82501, #80851, #65709, #5802, #29879, #108244, #108799, #5236, #64620, #90330, #72463, #39943, #4688, #21458, #74113, #99831, #23122, #48919, #83046, #63533, #20919, #38827, #89791, #55121, #89244, #98740, #12540, #38280, #106593, #22001, #13063, #47247, #56196, #91992, #42150 ),
 .UNSPECIFIED., .F., .F.,
 ( 4, 3, 3, 3, 3, 3, 3, 3, 3, 3, 3, 3, 3, 3, 4 ),
 ( 0.7655572723410000169, 0.9910019213816629868, 1.224379696548280050, 1.462078613726470078, 1.704827352691050013, 1.793853281190000093, 2.038466588041509819, 2.281256468864029330, 2.316155491860000026, 2.583989317140000352, 2.855920917859990027, 3.139267311770200131, 3.387490792979999554, 3.680707213613719553, 3.835724788389999418 ),
 .UNSPECIFIED. ) ;
#110279=EDGE_CURVE ( 'NONE', #28182, #105296, #10666, .T. ) ;
#110281=CARTESIAN_POINT ( 'NONE',  ( 3.108624468949999707E-15, 1472.413060387330006, 271.1218459616979999 ) ) ;
#110283=ADVANCED_FACE ( 'NONE', ( #102606 ), #47351, .F. ) ;
#110284=CARTESIAN_POINT ( 'NONE',  ( 11.11059101190000042, 1433.900907478189765, 151.6798154798979965 ) ) ;
#110285=CARTESIAN_POINT ( 'NONE',  ( 17.83186622649999720, 1447.284048007059937, 214.3676144203579952 ) ) ;
#110286=CARTESIAN_POINT ( 'NONE',  ( 12.56955872636179983, 1415.089118586289942, 197.3775234796719928 ) ) ;
#110293=CARTESIAN_POINT ( 'NONE',  ( -13.86092847646930082, 1410.765486861110048, 227.1170286572800023 ) ) ;
#110294=FACE_OUTER_BOUND ( 'NONE', #94839, .T. ) ;
#110295=CARTESIAN_POINT ( 'NONE',  ( 24.05801048009999832, 1430.354717876130053, 212.9167368799780036 ) ) ;
#110298=CARTESIAN_POINT ( 'NONE',  ( 3.530785927030000097E-16, 1427.166763959530044, 147.9649995502979891 ) ) ;
#110305=CARTESIAN_POINT ( 'NONE',  ( 0.2037710401876630106, 1460.860033808869957, 182.9161712545850094 ) ) ;
#110307=VERTEX_POINT ( 'NONE', #73464 ) ;
#110310=FACE_OUTER_BOUND ( 'NONE', #88264, .T. ) ;
#110311=CARTESIAN_POINT ( 'NONE',  ( -39.75236484342700294, 1448.901857781610261, 134.0999999981239910 ) ) ;
#110312=CARTESIAN_POINT ( 'NONE',  ( -31.06561261703210164, 1445.948172401960164, 137.1228040888619830 ) ) ;
#110314=CARTESIAN_POINT ( 'NONE',  ( 10.10004869885203682, 1422.222932908421853, 135.5999999980978430 ) ) ;
#110317=CARTESIAN_POINT ( 'NONE',  ( -14.45747005360000159, 1416.828040559430065, 221.3917074983979774 ) ) ;
#110331=CARTESIAN_POINT ( 'NONE',  ( -32.67729582440000513, 1451.771913520829912, 134.7516611205979871 ) ) ;
#110332=CARTESIAN_POINT ( 'NONE',  ( 17.11778670694504711, 1443.086052842848176, 162.7557629363845990 ) ) ;
#110333=DIRECTION ( 'NONE',  ( -1.000000000000000000, 0.000000000000000000, 0.000000000000000000 ) ) ;
#110334=VERTEX_POINT ( 'NONE', #57771 ) ;
#110339=CARTESIAN_POINT ( 'NONE',  ( 41.37929573993505983, 1446.359370807621190, 269.6357249233665812 ) ) ;
#110341=CARTESIAN_POINT ( 'NONE',  ( 18.04593430210184835, 1435.112856754830091, 215.2521370104431355 ) ) ;
#110342=FACE_OUTER_BOUND ( 'NONE', #17017, .T. ) ;
#110344=CARTESIAN_POINT ( 'NONE',  ( 11.34090880850000005, 1475.513060387329915, 227.1982711657979905 ) ) ;
#110347=VECTOR ( 'NONE', #35352, 1000.000000000000114 ) ;
#110348=CARTESIAN_POINT ( 'NONE',  ( 17.60627563539999940, 1410.895669412530196, 224.1775087544979783 ) ) ;
#110349=CARTESIAN_POINT ( 'NONE',  ( 1.341950105200000021, 1416.837177087930058, 190.1629993749980088 ) ) ;
#110357=CARTESIAN_POINT ( 'NONE',  ( -25.44333967360000059, 1449.802117277580010, 207.3037693659879892 ) ) ;
#110358=CARTESIAN_POINT ( 'NONE',  ( -11.10862876709039959, 1425.650570261519761, 121.9042659590140119 ) ) ;
#110359=CARTESIAN_POINT ( 'NONE',  ( 16.34779635269999787, 1409.733112109830017, 192.2574716150980123 ) ) ;
#110361=EDGE_CURVE ( 'NONE', #79447, #6969, #6683, .T. ) ;
#110362=CARTESIAN_POINT ( 'NONE',  ( 29.05308715847724699, 1510.038487003683258, 201.6439600875852420 ) ) ;
#110363=CARTESIAN_POINT ( 'NONE',  ( -18.89959452430000297, 1416.839692140830039, 207.5749784653779955 ) ) ;
#110364=CARTESIAN_POINT ( 'NONE',  ( 18.19796256645700083, 1509.563185887230020, 232.4213084367889905 ) ) ;
#110368=CARTESIAN_POINT ( 'NONE',  ( -37.75814923816869850, 1438.428394211809973, 136.5932668144599802 ) ) ;
#110370=CARTESIAN_POINT ( 'NONE',  ( 8.904014029423381160, 1397.867934375250115, 219.0684523409199755 ) ) ;
#110371=CARTESIAN_POINT ( 'NONE',  ( -18.87100397050000211, 1456.815141881530053, 228.5333397625980183 ) ) ;
#110373=VERTEX_POINT ( 'NONE', #68931 ) ;
#110376=CARTESIAN_POINT ( 'NONE',  ( -11.86590160489819823, 1432.348284114390026, 151.0567667500760081 ) ) ;
#110378=B_SPLINE_CURVE_WITH_KNOTS ( 'NONE', 3,
 ( #97505, #73964, #4017, #46573, #54975, #39804, #12931, #21314, #81238, #48217, #63925, #82356, #90184, #99681, #106997, #30838, #89645, #65014, #80708, #20774, #4554, #98594, #30286, #108095, #22973, #89100, #38687, #56611, #98040, #55517, #12388, #72862, #5087, #6190, #39240, #64478, #57179, #73415, #99131, #21858, #65570, #106455, #38143, #72325, #29738, #22409, #91301, #14584, #48773, #71802, #92388, #67772, #100783, #109759, #23537, #83440, #57729, #7299, #40893, #94049, #85094, #15661, #25730, #76157, #49314, #6735, #32508, #110305, #66678, #75074, #67228, #101885, #68338, #74523, #33580, #109223, #59932, #31941, #16221, #66136, #42554, #58809, #8385, #50966, #18, #34152, #100257, #33040, #50426, #49865, #85643, #25177, #51510, #41464, #91848, #92949, #108654, #16763, #76705, #84551, #83999, #102444, #75625, #24076, #42008, #40342, #15125, #59381, #101324, #58266, #24614, #7840, #93492, #17316, #102993, #27962, #104114, #2244, #27401, #44785, #105227, #44224, #60479, #573, #61584, #104667, #87889, #36357, #8943, #69440, #78935, #87322, #11180, #18425, #26290, #1676, #68891, #35256, #28514, #10617, #20103, #103555, #70548, #77816, #43116, #95717, #78368, #62145, #26858, #96271, #94597, #17876, #61046, #35816, #95169, #53755, #52625 ),
 .UNSPECIFIED., .F., .F.,
 ( 4, 3, 3, 3, 3, 3, 3, 3, 3, 3, 3, 3, 3, 3, 3, 3, 3, 3, 3, 3, 3, 3, 3, 3, 3, 3, 3, 3, 3, 3, 3, 3, 3, 3, 3, 3, 3, 3, 3, 3, 3, 3, 3, 3, 3, 3, 3, 3, 3, 3, 3, 3, 4 ),
 ( 24.28183316541300130, 24.71881649057640118, 25.16768965757360021, 25.63067172750350053, 26.11087491490579993, 26.61294145909250020, 27.16470443015920111, 27.77145901019460084, 28.47376813613320223, 29.29751198064149875, 29.94171883040609927, 30.50707339981829946, 31.03088294720540219, 31.53498744032980028, 32.00161556922130046, 32.45443727351199925, 32.89561208257300251, 33.32674843685160226, 33.76099105068869477, 34.17209352077410500, 34.57743404036049384, 34.97544006220940105, 35.06371889219999360, 39.13045466909090209, 43.63534274978590588, 49.28827455502730004, 54.45493433082799584, 58.82551417691030338, 62.91385627785520285, 66.62310817775708927, 67.00219837880000284, 67.58345923580628778, 68.17364255231809977, 68.77363305402450067, 69.38449005478119602, 70.00750236436559248, 70.64426827910560291, 71.29681654595110274, 71.96779783973650524, 72.67405307691460337, 73.40992868474920385, 74.18468017158738803, 75.01465558537010736, 75.96352105172489644, 77.28110059534179754, 78.31061113875900048, 79.18396656175289650, 79.98558190753520591, 80.73137701487929974, 81.44186439771650043, 82.13175408128769561, 82.79775432491919673, 82.96876233691149594 ),
 .UNSPECIFIED. ) ;
#110382=CIRCLE ( 'NONE', #74677, 39.61497827612718936 ) ;
#110384=CARTESIAN_POINT ( 'NONE',  ( 33.91369107978050579, 1451.728768198530133, 135.3769930381369875 ) ) ;
#110385=CARTESIAN_POINT ( 'NONE',  ( 0.4435022289555869968, 1418.672171135500093, 184.7048927309859891 ) ) ;
#110393=CARTESIAN_POINT ( 'NONE',  ( 11.79159303035750028, 1427.856769254729898, 147.7337906482489984 ) ) ;
#110394=EDGE_CURVE ( 'NONE', #64966, #75650, #81437, .T. ) ;
#110397=CARTESIAN_POINT ( 'NONE',  ( -14.00211218169999938, 1416.535385209229844, 221.8386906309980020 ) ) ;
#110398=CARTESIAN_POINT ( 'NONE',  ( -16.90742463042001376, 1442.831169986190844, 162.4348201727408991 ) ) ;
#110401=CARTESIAN_POINT ( 'NONE',  ( 21.90143050737389885, 1409.902695463000100, 206.2994855651969885 ) ) ;
#110402=EDGE_CURVE ( 'NONE', #59275, #101819, #13407, .T. ) ;
#110403=CARTESIAN_POINT ( 'NONE',  ( 14.36661330029840045, 1436.257348211630188, 150.0159985837800036 ) ) ;
#110407=CARTESIAN_POINT ( 'NONE',  ( -15.02388101939999920, 1462.596411967030008, 223.3218936951980140 ) ) ;
#110408=CARTESIAN_POINT ( 'NONE',  ( 17.24203588439999990, 1458.670886926930052, 229.0945275712979878 ) ) ;
#110410=CARTESIAN_POINT ( 'NONE',  ( -4.969838499002304566, 1423.248872364527642, 184.7412924219641184 ) ) ;
#110412=CARTESIAN_POINT ( 'NONE',  ( -5.468855732409769743, 1422.747406303380103, 121.8314839712469961 ) ) ;
#110417=EDGE_CURVE ( 'NONE', #91877, #31461, #92166, .T. ) ;
#110418=CARTESIAN_POINT ( 'NONE',  ( -2.901755129351373252, 1484.493861582726140, 183.2929701160953471 ) ) ;
#110419=CARTESIAN_POINT ( 'NONE',  ( -16.66101146819999812, 1410.867390116229899, 191.7375337716979971 ) ) ;
#110421=EDGE_LOOP ( 'NONE', ( #32052, #107759, #57399, #25812, #932 ) ) ;
#110425=CARTESIAN_POINT ( 'NONE',  ( -11.72873588490000074, 1429.311224835630128, 150.0544550291980102 ) ) ;
#110426=CARTESIAN_POINT ( 'NONE',  ( 19.27780332526499762, 1456.939258528880146, 224.7012343488810018 ) ) ;
#110430=CARTESIAN_POINT ( 'NONE',  ( 0.2681867035651760434, 1457.296285398379950, 189.0031676906399980 ) ) ;
#110432=CARTESIAN_POINT ( 'NONE',  ( -19.66165407200000104, 1482.732718108530207, 227.7681860883980107 ) ) ;
#110435=CARTESIAN_POINT ( 'NONE',  ( -16.78634058370699833, 1460.263302320530101, 228.3352825267500066 ) ) ;
#110438=CARTESIAN_POINT ( 'NONE',  ( 29.78004744509999924, 1414.955384726930106, 269.3615102554980467 ) ) ;
#110440=CARTESIAN_POINT ( 'NONE',  ( 18.44722761019999879, 1449.736698785399994, 191.1486972741980139 ) ) ;
#110442=EDGE_CURVE ( 'NONE', #68144, #7608, #94957, .T. ) ;
#110443=CARTESIAN_POINT ( 'NONE',  ( -0.01845360631625059950, 1508.137092213139795, 237.5627139155050145 ) ) ;
#110444=CARTESIAN_POINT ( 'NONE',  ( 15.95383384960000228, 1506.798305107329952, 193.5571554442980187 ) ) ;
#110445=CARTESIAN_POINT ( 'NONE',  ( -1.387227658650000084, 1451.254490850629963, 183.6670524069980104 ) ) ;
#110446=CARTESIAN_POINT ( 'NONE',  ( 17.69066643606209155, 1458.123854326780929, 230.3917304478115682 ) ) ;
#110448=CARTESIAN_POINT ( 'NONE',  ( -13.58279026639999998, 1443.465488095079991, 187.7936867102980045 ) ) ;
#110451=CARTESIAN_POINT ( 'NONE',  ( 5.035691840050000145, 1407.858053359329915, 270.1320510971980298 ) ) ;
#110452=CARTESIAN_POINT ( 'NONE',  ( 1.452806739154890003, 1502.997517574160156, 181.2928522130929991 ) ) ;
#110454=EDGE_CURVE ( 'NONE', #52345, #81409, #101676, .T. ) ;
#110455=AXIS2_PLACEMENT_3D ( 'NONE', #56197, #57865, #14732 ) ;
#110456=CARTESIAN_POINT ( 'NONE',  ( 11.45115712805808172, 1425.807404925399624, 139.1344848049184293 ) ) ;
#110458=CARTESIAN_POINT ( 'NONE',  ( -12.73803555039999935, 1474.798601776230043, 267.7854995676979684 ) ) ;
#110462=CARTESIAN_POINT ( 'NONE',  ( 18.42623971653249981, 1424.510075577899897, 223.4209876132420050 ) ) ;
#110465=CARTESIAN_POINT ( 'NONE',  ( -11.96661585360000046, 1440.449248668989867, 150.8629738177980073 ) ) ;
#110466=CARTESIAN_POINT ( 'NONE',  ( -24.64468664290339817, 1457.436562328650098, 211.7678147391609969 ) ) ;
#110467=CARTESIAN_POINT ( 'NONE',  ( -2.127049456059860066, 1416.948096802419968, 197.4354557404840307 ) ) ;
#110470=CARTESIAN_POINT ( 'NONE',  ( -23.36711103019999669, 1410.650541193030222, 205.9586710055679930 ) ) ;
#110474=FACE_OUTER_BOUND ( 'NONE', #108189, .T. ) ;
#110480=CARTESIAN_POINT ( 'NONE',  ( 11.69994194908459839, 1426.720164485290070, 141.5157594407809825 ) ) ;
#110488=CARTESIAN_POINT ( 'NONE',  ( -4.225531567558850732, 1398.039136736335195, 221.4159458655357753 ) ) ;
#110489=CARTESIAN_POINT ( 'NONE',  ( 1.547463896846929865, 1414.913060387349788, 192.3096116128920130 ) ) ;
#110494=ORIENTED_EDGE ( 'NONE', *, *, #31975, .F. ) ;
#110496=CARTESIAN_POINT ( 'NONE',  ( 11.82498356950000051, 1433.974774860679872, 150.8894406338980048 ) ) ;
#110497=CARTESIAN_POINT ( 'NONE',  ( -5.039302881340000262, 1396.270828050830005, 220.4040175563980313 ) ) ;
#110500=CARTESIAN_POINT ( 'NONE',  ( -23.45874307799999769, 1509.732257746930145, 193.0693562410979780 ) ) ;
#110502=CARTESIAN_POINT ( 'NONE',  ( 16.03737488143600132, 1422.958007463530294, 191.1431703812559988 ) ) ;
#110503=CARTESIAN_POINT ( 'NONE',  ( 17.83884855390000013, 1421.695374127529931, 225.9258521583979871 ) ) ;
#110504=CARTESIAN_POINT ( 'NONE',  ( 17.00378010880389823, 1488.410040644369928, 230.1592669151310133 ) ) ;
#110505=B_SPLINE_CURVE_WITH_KNOTS ( 'NONE', 5,
 ( #92013, #92549, #15817, #187, #42165, #84154 ),
 .UNSPECIFIED., .F., .F.,
 ( 6, 6 ),
 ( -95.99024502151270610, -20.17942402910439625 ),
 .UNSPECIFIED. ) ;
#110506=CARTESIAN_POINT ( 'NONE',  ( 4.549407228569999795, 1449.234560512250027, 184.4437958230980144 ) ) ;
#110507=CARTESIAN_POINT ( 'NONE',  ( -0.1955981715909999863, 1414.913060387329779, 193.0575580938979954 ) ) ;
#110508=CYLINDRICAL_SURFACE ( 'NONE', #96546, 2.000000000000022204 ) ;
#110509=CARTESIAN_POINT ( 'NONE',  ( 1.951953247971109917, 1395.981224096749884, 198.2838940656170053 ) ) ;
#110510=CARTESIAN_POINT ( 'NONE',  ( 14.41907353320999974, 1416.449138231070037, 196.8916081074650037 ) ) ;
#110511=CARTESIAN_POINT ( 'NONE',  ( 11.76661577670000014, 1432.114831257029891, 150.8088909320979951 ) ) ;
#110514=CARTESIAN_POINT ( 'NONE',  ( 13.52509826555950134, 1435.477190311279855, 150.1367605865879682 ) ) ;
#110515=B_SPLINE_CURVE_WITH_KNOTS ( 'NONE', 3,
 ( #49863, #23536, #49313, #65013 ),
 .UNSPECIFIED., .F., .F.,
 ( 4, 4 ),
 ( 0.000000000000000000, 1.000000000000000000 ),
 .UNSPECIFIED. ) ;
#110518=CARTESIAN_POINT ( 'NONE',  ( 13.50811536235293353, 1444.049332424179056, 169.3527944688763114 ) ) ;
#110519=CARTESIAN_POINT ( 'NONE',  ( -9.099053347499999944, 1464.323907318429974, 232.8359173459980127 ) ) ;
#110524=CARTESIAN_POINT ( 'NONE',  ( 2.500000000000000000, 1448.204022878760043, 169.8583767613770021 ) ) ;
#110529=CARTESIAN_POINT ( 'NONE',  ( 19.72684292035980036, 1440.913060387330006, 214.6106658576619850 ) ) ;
#110530=CARTESIAN_POINT ( 'NONE',  ( -19.48412118799999959, 1509.357564148129995, 230.4874557228980052 ) ) ;
#110531=CARTESIAN_POINT ( 'NONE',  ( -4.387270951399999674, 1410.444783042529934, 186.8284482498980026 ) ) ;
#110535=CARTESIAN_POINT ( 'NONE',  ( 21.70470943100000127, 1430.163002639730166, 219.7457352202980019 ) ) ;
#110536=DIRECTION ( 'NONE',  ( -0.7026931535931751904, 0.02432541744852609669, -0.7110770745560801576 ) ) ;
#110539=CARTESIAN_POINT ( 'NONE',  ( 0.003780032387689030195, 1466.769817337830091, 235.6257279122189914 ) ) ;
#110545=CARTESIAN_POINT ( 'NONE',  ( -20.59469742430000139, 1507.767255104930200, 190.2244918928979871 ) ) ;
#110546=AXIS2_PLACEMENT_3D ( 'NONE', #51459, #16175, #24020 ) ;
#110550=CARTESIAN_POINT ( 'NONE',  ( 14.72054272970000000, 1409.427113070929863, 192.5180613899979960 ) ) ;
#110551=( BOUNDED_CURVE ( )  B_SPLINE_CURVE ( 3, ( #61439, #44068, #63112, #53590 ),
 .UNSPECIFIED., .F., .T. ) 
 B_SPLINE_CURVE_WITH_KNOTS ( ( 4, 4 ),
 ( 4.243850967066803648, 4.610002426280772170 ),
 .UNSPECIFIED. ) 
 CURVE ( )  GEOMETRIC_REPRESENTATION_ITEM ( )  RATIONAL_B_SPLINE_CURVE ( ( 1.000000000000000000, 0.9888589289762730328, 0.9888589289762730328, 1.000000000000000000 ) ) 
 REPRESENTATION_ITEM ( '' )  );
#110552=CARTESIAN_POINT ( 'NONE',  ( 10.97130333569999827, 1432.456475934739956, 151.7700838859979910 ) ) ;
#110554=ORIENTED_EDGE ( 'NONE', *, *, #40661, .T. ) ;
#110556=CARTESIAN_POINT ( 'NONE',  ( 20.04382680870000044, 1471.636491243529917, 264.7217811306979911 ) ) ;
#110560=CARTESIAN_POINT ( 'NONE',  ( -23.89130367779999986, 1445.918201964170066, 214.2695373320979968 ) ) ;
#110561=CARTESIAN_POINT ( 'NONE',  ( -0.1681681984989999989, 1405.973120458229914, 146.1721969590979882 ) ) ;
#110563=CARTESIAN_POINT ( 'NONE',  ( 19.03110457509999875, 1457.047041243630019, 226.1578386332979846 ) ) ;
#110567=ORIENTED_EDGE ( 'NONE', *, *, #62887, .T. ) ;
#110569=CARTESIAN_POINT ( 'NONE',  ( 8.217213021130000279E-10, 1406.066315318429815, 269.0456997843980389 ) ) ;
#110570=CARTESIAN_POINT ( 'NONE',  ( -0.1675834497249999722, 1467.614897612030063, 229.5904413177980246 ) ) ;
#110572=CARTESIAN_POINT ( 'NONE',  ( 12.87923822840000021, 1419.814314491729874, 222.7980798877980249 ) ) ;
#110576=CARTESIAN_POINT ( 'NONE',  ( 15.06727053545517947, 1420.624436962964637, 227.9341869482010452 ) ) ;
#110577=CARTESIAN_POINT ( 'NONE',  ( 32.66532558909530337, 1435.798634193749876, 135.9825271959909969 ) ) ;
#110578=CARTESIAN_POINT ( 'NONE',  ( 40.04800941360640110, 1445.544085285030178, 136.8743094025140010 ) ) ;
#110579=CARTESIAN_POINT ( 'NONE',  ( 2.601599038695280157E-15, 1470.145267143019964, 266.9202418870810334 ) ) ;
#110583=CARTESIAN_POINT ( 'NONE',  ( -38.89734685438744322, 1452.468859951071181, 269.5913801711774340 ) ) ;
#110588=CARTESIAN_POINT ( 'NONE',  ( 15.56176417158150116, 1464.171868028719928, 189.4544269278800073 ) ) ;
#110589=CARTESIAN_POINT ( 'NONE',  ( -4.343257420380000298E-10, 1475.319450600630034, 269.4986873273979882 ) ) ;
#110592=CARTESIAN_POINT ( 'NONE',  ( -28.83249086449999865, 1509.587594257930050, 209.3213971828919853 ) ) ;
#110598=CARTESIAN_POINT ( 'NONE',  ( -7.331526522911103072, 1451.412073465244930, 153.1354536431154827 ) ) ;
#110599=CARTESIAN_POINT ( 'NONE',  ( -17.97082642953529685, 1416.218047878440075, 209.4769703680670148 ) ) ;
#110600=CARTESIAN_POINT ( 'NONE',  ( 24.58760858760000190, 1435.374942484849953, 136.3398539886979961 ) ) ;
#110601=CARTESIAN_POINT ( 'NONE',  ( -10.76975510178520068, 1396.289148523040012, 206.5700517074710092 ) ) ;
#110603=VERTEX_POINT ( 'NONE', #32278 ) ;
#110604=CARTESIAN_POINT ( 'NONE',  ( -0.3443494227043759626, 1415.932840154009909, 191.2798020189869987 ) ) ;
#110605=CARTESIAN_POINT ( 'NONE',  ( -9.486449711069932178, 1409.244334510940007, 228.2930016997800067 ) ) ;
#110610=CARTESIAN_POINT ( 'NONE',  ( 11.00605459009999976, 1426.944683675330225, 91.15821214469779932 ) ) ;
#110611=CARTESIAN_POINT ( 'NONE',  ( -23.73182569189999924, 1445.711889770029984, 212.0244532444880008 ) ) ;
#110613=CARTESIAN_POINT ( 'NONE',  ( -11.71362335670000121, 1433.059942302950276, 150.8500997151980130 ) ) ;
#110615=CARTESIAN_POINT ( 'NONE',  ( -2.617672629425792152, 1420.510773938307011, 185.8077901307954107 ) ) ;
#110617=CARTESIAN_POINT ( 'NONE',  ( -24.32551817709999753, 1439.446294773350019, 211.3365414780779759 ) ) ;
#110618=CARTESIAN_POINT ( 'NONE',  ( 8.878920243399999634, 1509.223121094930093, 181.5151187545980065 ) ) ;
#110619=CARTESIAN_POINT ( 'NONE',  ( 2.157135272340000132, 1450.193356149409965, 182.5998694718979891 ) ) ;
#110622=CARTESIAN_POINT ( 'NONE',  ( -27.93181393147919067, 1510.000215323476596, 198.1739204093250635 ) ) ;
#110625=ORIENTED_EDGE ( 'NONE', *, *, #30281, .F. ) ;
#110626=CARTESIAN_POINT ( 'NONE',  ( -11.78247531003460047, 1427.502628522240002, 147.2054527168990035 ) ) ;
#110628=FACE_OUTER_BOUND ( 'NONE', #63195, .T. ) ;
#110629=CARTESIAN_POINT ( 'NONE',  ( 12.90158639592108258, 1434.732194105914914, 147.0409106621408739 ) ) ;
#110631=CARTESIAN_POINT ( 'NONE',  ( 17.49001816009999999, 1408.913060387329779, 205.8268510044480024 ) ) ;
#110633=CARTESIAN_POINT ( 'NONE',  ( -18.37215797060000000, 1453.313060387329870, 201.1114320114980103 ) ) ;
#110636=CARTESIAN_POINT ( 'NONE',  ( -18.74185279165999773, 1409.000834736390061, 268.9060467476150507 ) ) ;
#110637=CARTESIAN_POINT ( 'NONE',  ( -13.86100052414289863, 1434.990764548580046, 148.7478939910440090 ) ) ;
#110640=CARTESIAN_POINT ( 'NONE',  ( 13.48810824839999967, 1444.252978269910045, 187.9321459801979870 ) ) ;
#110646=CARTESIAN_POINT ( 'NONE',  ( -15.16872267709999988, 1470.466736689130130, 187.9100041707980040 ) ) ;
#110647=CARTESIAN_POINT ( 'NONE',  ( 4.026786250540000722, 1408.413060387330006, 121.6099336315979969 ) ) ;
#110651=CARTESIAN_POINT ( 'NONE',  ( -28.19177135810000223, 1509.605818728229906, 205.1802907371279900 ) ) ;
#110652=CARTESIAN_POINT ( 'NONE',  ( -1.326199192210000044, 1477.815017677929973, 230.7694779113980132 ) ) ;
#110655=CARTESIAN_POINT ( 'NONE',  ( -13.30361621630000180, 1409.377632903229824, 226.2974586568980158 ) ) ;
#110658=CARTESIAN_POINT ( 'NONE',  ( -26.64852628982920280, 1469.324129686450078, 209.1558146821249977 ) ) ;
#110659=CARTESIAN_POINT ( 'NONE',  ( 26.16501621689999624, 1469.244469849229972, 211.4985517754080320 ) ) ;
#110662=CARTESIAN_POINT ( 'NONE',  ( -24.98051366310000176, 1436.289130477859999, 137.7795203887980051 ) ) ;
#110666=B_SPLINE_CURVE_WITH_KNOTS ( 'NONE', 3,
 ( #95589, #18858, #53054, #10484, #28389, #64632, #5816, #91464, #57876, #89803, #83595, #23692 ),
 .UNSPECIFIED., .F., .F.,
 ( 4, 2, 2, 2, 2, 4 ),
 ( -0.1123552058539349918, -0.09789079797621490220, -0.08345975750763819090, -0.05408602645632740180, -0.02844277172931640452, 0.000000000000000000 ),
 .UNSPECIFIED. ) ;
#110667=CARTESIAN_POINT ( 'NONE',  ( -14.09270673139999985, 1418.021918129430105, 227.3443978055980210 ) ) ;
#110671=CARTESIAN_POINT ( 'NONE',  ( -40.71747597329999735, 1438.773003763620181, 134.0999987698980078 ) ) ;
#110672=CARTESIAN_POINT ( 'NONE',  ( -10.25433319729999759, 1415.365669972130036, 229.7516580550980052 ) ) ;
#110673=CARTESIAN_POINT ( 'NONE',  ( -19.80317870211088760, 1456.769327258462909, 225.5394267937573716 ) ) ;
#110674=ORIENTED_EDGE ( 'NONE', *, *, #67834, .F. ) ;
#110676=AXIS2_PLACEMENT_3D ( 'NONE', #41061, #81392, #39413 ) ;
#110678=CARTESIAN_POINT ( 'NONE',  ( 12.65761277830709908, 1435.514348419339967, 150.7820475295659719 ) ) ;
#110679=B_SPLINE_SURFACE_WITH_KNOTS ( 'NONE', 5, 5, ( 
 ( #7426, #6865, #15258, #58946, #6327, #108232 ),
 ( #74102, #58397, #65700, #83037, #33171, #99818 ),
 ( #90878, #40477, #23112, #41025, #100912, #66811 ),
 ( #74651, #48351, #56742, #91982, #49448, #83573 ),
 ( #92522, #49991, #108787, #84127, #73556, #101459 ),
 ( #32079, #48909, #14166, #82491, #39934, #30973 ) ),
 .UNSPECIFIED., .F., .F., .F.,
 ( 6, 6 ),
 ( 6, 6 ),
 ( 7.505253243670000352, 8.371505715449998775 ),
 ( 0.000000000000000000, 1.425510291809999996 ),
 .UNSPECIFIED. ) ;
#110680=CARTESIAN_POINT ( 'NONE',  ( -4.127449627910051433, 1441.471781363327182, 184.1788307560163958 ) ) ;
#110682=DIRECTION ( 'NONE',  ( 0.6677681214262592979, -0.7443693545591762994, 0.000000000000000000 ) ) ;
#110684=DIRECTION ( 'NONE',  ( 0.3363363969979658030, 0.9417419115949056119, 0.000000000000000000 ) ) ;
#110685=CARTESIAN_POINT ( 'NONE',  ( -15.05358279999999915, 1410.831827720429828, 226.7261506157979909 ) ) ;
#110689=CARTESIAN_POINT ( 'NONE',  ( 19.97269026569999895, 1507.847566758330004, 189.1149477268980093 ) ) ;
#110693=CARTESIAN_POINT ( 'NONE',  ( 15.97957002059996157, 1409.471061922630497, 193.0247866931977114 ) ) ;
#110695=CARTESIAN_POINT ( 'NONE',  ( 1.959361663749999982, 1419.250139722030099, 185.0399661677979850 ) ) ;
#110700=B_SPLINE_CURVE_WITH_KNOTS ( 'NONE', 3,
 ( #18799, #80939, #105601, #29417, #95528, #70924, #53552, #38372, #27772, #52995, #63080, #4237, #87129, #2048, #88790 ),
 .UNSPECIFIED., .F., .F.,
 ( 4, 2, 2, 1, 1, 1, 2, 2, 4 ),
 ( 0.000000000000000000, 0.2499999999999507061, 0.3749999999999348299, 0.4374999999999256151, 0.4687499999999210076, 0.4843749999999186762, 0.4921874999999189537, 0.4999999999999191758, 1.000000000000000000 ),
 .UNSPECIFIED. ) ;
#110703=CARTESIAN_POINT ( 'NONE',  ( 1.823963636610874239, 1416.770504172074197, 232.7531906332400808 ) ) ;
#110704=CARTESIAN_POINT ( 'NONE',  ( 18.89315557560000158, 1416.535385209229844, 210.0306673353090048 ) ) ;
#110707=EDGE_CURVE ( 'NONE', #44597, #660, #73184, .T. ) ;
#110708=CARTESIAN_POINT ( 'NONE',  ( -2.471608048749999842, 1438.194204504490017, 150.4833623973980252 ) ) ;
#110709=CARTESIAN_POINT ( 'NONE',  ( 45.63129791352729825, 1440.913060379180024, 266.1458157647700205 ) ) ;
#110712=ORIENTED_EDGE ( 'NONE', *, *, #56860, .F. ) ;
#110713=ORIENTED_EDGE ( 'NONE', *, *, #13323, .T. ) ;
#110715=CARTESIAN_POINT ( 'NONE',  ( -19.87678393280335243, 1484.439226788044152, 191.0985201580460000 ) ) ;
#110717=CARTESIAN_POINT ( 'NONE',  ( 12.90804412569774762, 1410.732742728818266, 190.4223191256656094 ) ) ;
#110718=AXIS2_PLACEMENT_3D ( 'NONE', #23405, #107964, #82769 ) ;
#110720=B_SPLINE_SURFACE_WITH_KNOTS ( 'NONE', 4, 5, ( 
 ( #91341, #81821, #98627, #21894, #5124, #39280 ),
 ( #21349, #73455, #74556, #99718, #31424, #14063 ),
 ( #55556, #107586, #89681, #40378, #14623, #90220 ),
 ( #23572, #5692, #108689, #48252, #91884, #13505 ),
 ( #15157, #31981, #39836, #57765, #98078, #30872 ) ),
 .UNSPECIFIED., .F., .F., .F.,
 ( 5, 5 ),
 ( 6, 6 ),
 ( 23.77038316910000049, 36.72447201482209778 ),
 ( -0.0002035811339858509933, 2.000203581245860285 ),
 .UNSPECIFIED. ) ;
#110725=CARTESIAN_POINT ( 'NONE',  ( 6.976610649730000446, 1452.669431775030034, 151.9927557690980109 ) ) ;
#110726=CARTESIAN_POINT ( 'NONE',  ( 0.1681674884180490159, 1420.473121907760060, 182.7464979049940155 ) ) ;
#110729=CARTESIAN_POINT ( 'NONE',  ( 24.06669976739999939, 1509.724642860830045, 193.1379647362979881 ) ) ;
#110730=ORIENTED_EDGE ( 'NONE', *, *, #31026, .F. ) ;
#110733=CARTESIAN_POINT ( 'NONE',  ( -16.48213017202440156, 1409.488629055829961, 224.5375925732930114 ) ) ;
#110736=CARTESIAN_POINT ( 'NONE',  ( 12.20364748979999980, 1447.059433187239847, 188.0531537431980098 ) ) ;
#110738=CARTESIAN_POINT ( 'NONE',  ( 40.13353682310170001, 1442.269293553509897, 136.9628395507569962 ) ) ;
#110744=CARTESIAN_POINT ( 'NONE',  ( -12.64492061617493235, 1435.846068781982012, 150.8967598469849065 ) ) ;
#110746=B_SPLINE_CURVE_WITH_KNOTS ( 'NONE', 3,
 ( #90071, #38035, #72215, #20120, #82235, #80036, #106337, #64357, #55401, #73855, #3358, #99021, #89533, #4443, #13352, #41890, #16112 ),
 .UNSPECIFIED., .F., .F.,
 ( 4, 2, 2, 2, 2, 1, 2, 2, 4 ),
 ( 0.000000000000000000, 0.2499999999999915623, 0.3749999999999957812, 0.5000000000000000000, 0.6250000000000042188, 0.6875000000000049960, 0.7187500000000053291, 0.7500000000000057732, 1.000000000000000000 ),
 .UNSPECIFIED. ) ;
#110747=CARTESIAN_POINT ( 'NONE',  ( 5.118312429449999534, 1409.258938051830000, 187.0063209343980191 ) ) ;
#110748=CARTESIAN_POINT ( 'NONE',  ( 4.527354660830000377, 1423.822069290730269, 184.4238519299979941 ) ) ;
#110750=CARTESIAN_POINT ( 'NONE',  ( -3.141092941611050016, 1440.712674293340115, 157.0493854566300058 ) ) ;
#110752=CARTESIAN_POINT ( 'NONE',  ( -2.338064766694980090, 1451.283254387899888, 184.5359555560359865 ) ) ;
#110753=CARTESIAN_POINT ( 'NONE',  ( 1.406054942129999930, 1464.967845642129987, 236.6417686339979980 ) ) ;
#110754=ORIENTED_EDGE ( 'NONE', *, *, #40817, .F. ) ;
#110756=CARTESIAN_POINT ( 'NONE',  ( -1.628202555219999903, 1430.465083930730088, 150.2970716576980124 ) ) ;
#110759=CARTESIAN_POINT ( 'NONE',  ( 15.53740313620000180, 1449.513310617089928, 190.1957215746979841 ) ) ;
#110761=CARTESIAN_POINT ( 'NONE',  ( -2.034934016457660169E-12, 1470.108503626060156, 254.3105774012479685 ) ) ;
#110762=CARTESIAN_POINT ( 'NONE',  ( -19.90677659085769946, 1485.410772266320237, 191.0396054904460073 ) ) ;
#110763=CARTESIAN_POINT ( 'NONE',  ( -1.226570660889999997, 1415.553739809529816, 227.5749953283980176 ) ) ;
#110764=CARTESIAN_POINT ( 'NONE',  ( -6.356242932690000735, 1416.544486832730172, 231.6503315779980028 ) ) ;
#110767=CARTESIAN_POINT ( 'NONE',  ( -0.5856906059243432994, 1485.491362865349402, 181.9191849365466283 ) ) ;
#110769=CARTESIAN_POINT ( 'NONE',  ( -45.80170866997659829, 1439.242720596339950, 268.7579477620919874 ) ) ;
#110770=CARTESIAN_POINT ( 'NONE',  ( 13.69935640180099945, 1509.078849000180071, 233.8886703240220015 ) ) ;
#110771=CARTESIAN_POINT ( 'NONE',  ( -13.04908991647894290, 1414.913372219064286, 220.1077748470152642 ) ) ;
#110774=CARTESIAN_POINT ( 'NONE',  ( -2.478470422270000029, 1437.832529885160056, 157.6963859361979985 ) ) ;
#110778=CARTESIAN_POINT ( 'NONE',  ( -26.78870495038239952, 1451.977601232150164, 134.9148139021100121 ) ) ;
#110780=CARTESIAN_POINT ( 'NONE',  ( 4.694071620149999902, 1416.682256071730080, 238.2947578313980159 ) ) ;
#110783=CARTESIAN_POINT ( 'NONE',  ( -1.793335950739999962, 1419.496365638530051, 185.6406336190979971 ) ) ;
#110787=ORIENTED_EDGE ( 'NONE', *, *, #51620, .T. ) ;
#110788=CARTESIAN_POINT ( 'NONE',  ( -6.618142395782879994, 1410.137584300400022, 270.0732991173869664 ) ) ;
#110789=CARTESIAN_POINT ( 'NONE',  ( 10.63558804199830021, 1419.812302066319944, 231.2733509599579804 ) ) ;
#110792=VERTEX_POINT ( 'NONE', #85984 ) ;
#110793=CARTESIAN_POINT ( 'NONE',  ( -22.62006121466300002, 1409.702956284340189, 209.3923079909519913 ) ) ;
#110794=CARTESIAN_POINT ( 'NONE',  ( -4.447601775919999945, 1425.243076475230282, 186.2019964394980036 ) ) ;
#110797=CARTESIAN_POINT ( 'NONE',  ( -45.56249212406897442, 1438.493842798003470, 266.1916403547691061 ) ) ;
#110799=CARTESIAN_POINT ( 'NONE',  ( -21.03123196678649975, 1507.789098018889945, 192.1781278620359785 ) ) ;
#110801=CARTESIAN_POINT ( 'NONE',  ( 41.02605310493780166, 1456.755636601169954, 268.6565615534370295 ) ) ;
#110806=CARTESIAN_POINT ( 'NONE',  ( 18.43151930343191580, 1458.912353611211984, 227.6950766328336329 ) ) ;
#110809=ORIENTED_EDGE ( 'NONE', *, *, #12603, .F. ) ;
#110812=CARTESIAN_POINT ( 'NONE',  ( 27.02366518750249824, 1451.037975853650096, 136.3590651249419921 ) ) ;
#110819=CARTESIAN_POINT ( 'NONE',  ( 9.139323887128899315, 1409.232212610100078, 189.8042143963789954 ) ) ;
#110821=CARTESIAN_POINT ( 'NONE',  ( 11.60004869885203682, 1411.254281879943164, 135.5999999980979851 ) ) ;
#110822=CARTESIAN_POINT ( 'NONE',  ( 15.60455980150000066, 1409.457983623130076, 225.4781096464980124 ) ) ;
#110824=CARTESIAN_POINT ( 'NONE',  ( 14.83523515338253418, 1422.059756969527143, 230.2894810269289394 ) ) ;
#110826=CARTESIAN_POINT ( 'NONE',  ( 11.29419939621850055, 1414.913057855109855, 221.1598003036660032 ) ) ;
#110829=B_SPLINE_SURFACE_WITH_KNOTS ( 'NONE', 5, 5, ( 
 ( #32107, #68487, #7999, #66293, #100409, #23693 ),
 ( #57878, #110466, #49474, #92011, #32657, #33744 ),
 ( #15281, #67939, #83596, #6895, #41051, #66834 ),
 ( #58421, #727, #78531, #104279, #26450, #86920 ),
 ( #96433, #1276, #9111, #79647, #2951, #70716 ),
 ( #77969, #104830, #37070, #1842, #10211, #60643 ) ),
 .UNSPECIFIED., .F., .F., .F.,
 ( 6, 6 ),
 ( 6, 6 ),
 ( 78.04565204464360306, 167.5290185466710113 ),
 ( -0.0009444657940283349628, 2.000944465795519989 ),
 .UNSPECIFIED. ) ;
ENDSEC;
END-ISO-10303-21;
